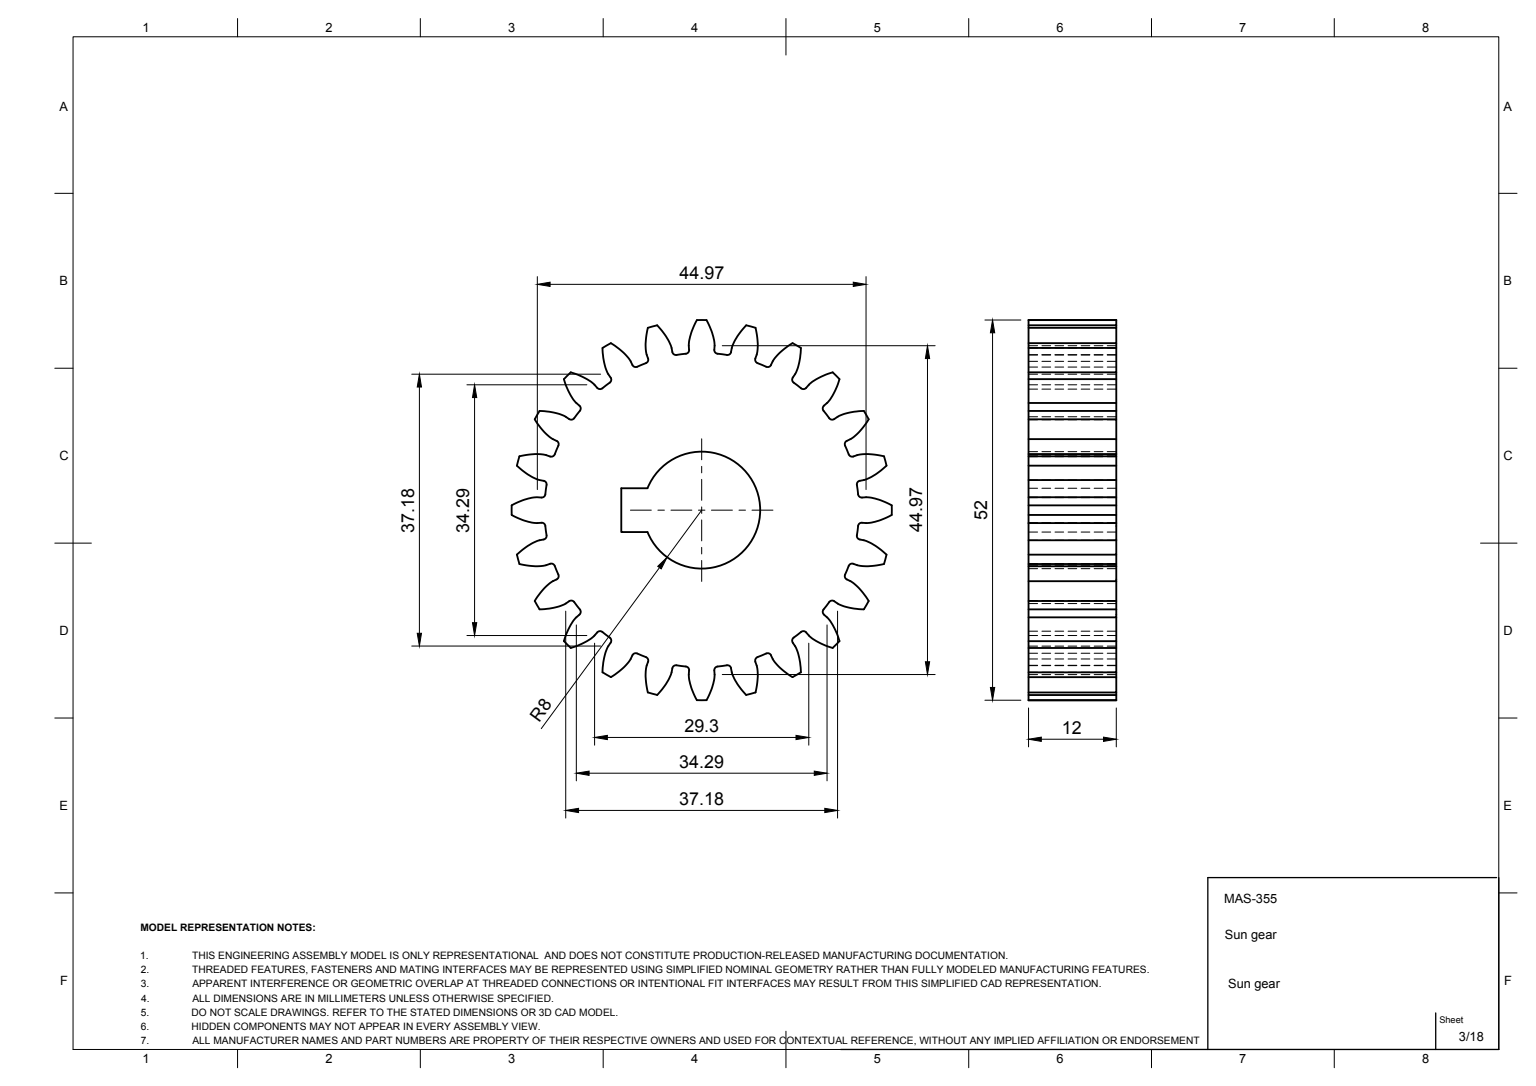
ISO-10303-21;
HEADER;
/* Generated by software containing ST-Developer
 * from STEP Tools, Inc. (www.steptools.com) 
 */

FILE_DESCRIPTION(
/* description */ ('Independent two-stage fixed-ring planetary gearbox,24/24/72 teeth,mod
ule2,20deg involutes,three planets per stage,4:1 x4:1=16:1. Native cut
-space/fillet/pattern tooth profiles derived from reusable gear blanks
; shared sun/planet/ring/carrier parts across both stages. Captured br
onze-journal input/carriers, headed retained planet pins, keyed inters
tage drive and modular keyed output interface. Native ideal gear links
; no torque, precision grade, production backlash/fits, lubrication, s
peed or life rating.'),
/* implementation_level */ '2;1');

FILE_NAME(
/* name */ 'Sun gear.step',
/* time_stamp */ '2026-11-08T19:10:00-08:00',
/* author */ (''),
/* organization */ (''),
/* preprocessor_version */ 'ST-DEVELOPER v20.2',
/* originating_system */ 'Autodesk Translation Framework v15.17.0.0',
/* authorisation */ '');

FILE_SCHEMA (('AUTOMOTIVE_DESIGN { 1 0 10303 214 3 1 1 }'));
ENDSEC;

DATA;
#10=MECHANICAL_DESIGN_GEOMETRIC_PRESENTATION_REPRESENTATION('',(#1168),#259224);
#691=(
BOUNDED_CURVE()
B_SPLINE_CURVE(5,(#175013,#175014,#175015,#175016,#175017,#175018,#175019,
#175020,#175021,#175022,#175023,#175024,#175025,#175026,#175027,#175028,
#175029,#175030,#175031,#175032,#175033,#175034,#175035,#175036,#175037,
#175038,#175039,#175040,#175041,#175042,#175043,#175044,#175045,#175046,
#175047,#175048,#175049,#175050,#175051,#175052,#175053,#175054,#175055,
#175056,#175057,#175058,#175059,#175060,#175061,#175062,#175063,#175064,
#175065,#175066,#175067,#175068,#175069,#175070,#175071,#175072,#175073,
#175074,#175075,#175076,#175077,#175078,#175079,#175080,#175081,#175082,
#175083,#175084,#175085,#175086,#175087,#175088,#175089,#175090,#175091,
#175092,#175093,#175094,#175095,#175096,#175097,#175098,#175099,#175100,
#175101,#175102,#175103,#175104,#175105,#175106,#175107,#175108,#175109,
#175110,#175111,#175112,#175113,#175114,#175115,#175116,#175117,#175118,
#175119,#175120,#175121,#175122,#175123,#175124,#175125,#175126,#175127,
#175128,#175129,#175130,#175131,#175132,#175133,#175134,#175135,#175136,
#175137,#175138,#175139,#175140,#175141,#175142,#175143,#175144,#175145,
#175146,#175147,#175148,#175149,#175150,#175151,#175152,#175153,#175154,
#175155,#175156,#175157,#175158,#175159,#175160,#175161,#175162,#175163,
#175164,#175165,#175166,#175167,#175168,#175169,#175170,#175171,#175172,
#175173,#175174,#175175,#175176,#175177,#175178,#175179,#175180,#175181,
#175182,#175183,#175184,#175185,#175186,#175187,#175188,#175189,#175190,
#175191,#175192,#175193,#175194,#175195,#175196,#175197,#175198,#175199,
#175200,#175201,#175202,#175203,#175204,#175205,#175206,#175207,#175208,
#175209,#175210,#175211,#175212,#175213,#175214,#175215,#175216,#175217),
 .UNSPECIFIED.,.F.,.F.)
B_SPLINE_CURVE_WITH_KNOTS((6,1,1,1,1,1,1,1,1,1,1,1,1,1,1,1,1,1,1,1,1,1,
1,1,1,1,1,1,1,1,1,1,1,1,1,1,1,1,1,1,1,1,1,1,1,1,1,1,1,1,1,1,1,1,1,1,1,1,
1,1,1,1,1,1,1,1,1,1,1,1,1,1,1,1,1,1,1,1,1,1,1,1,1,1,1,1,1,1,1,1,1,1,1,1,
1,1,1,1,1,1,1,1,1,1,1,1,1,1,1,1,1,1,1,1,1,1,1,1,1,1,1,1,1,1,1,1,1,1,1,1,
1,1,1,1,1,1,1,1,1,1,1,1,1,1,1,1,1,1,1,1,1,1,1,1,1,1,1,1,1,1,1,1,1,1,1,1,
1,1,1,1,1,1,1,1,1,1,1,1,1,1,1,1,1,1,1,1,1,1,1,1,1,1,1,1,1,1,1,1,1,1,6),
(0.,0.005,0.01,0.015,0.02,0.025,0.03,0.035,0.04,0.045,0.05,0.055,0.06,0.065,
0.07,0.075,0.08,0.085,0.09,0.095,0.1,0.105,0.11,0.115,0.12,0.125,0.13,0.135,
0.14,0.145,0.15,0.155,0.16,0.165,0.17,0.175,0.18,0.185,0.19,0.195,0.2,0.205,
0.21,0.215,0.22,0.225,0.23,0.235,0.24,0.245,0.25,0.255,0.26,0.265,0.27,
0.275,0.28,0.285,0.29,0.295,0.3,0.305,0.31,0.315,0.32,0.325,0.33,0.335,
0.34,0.345,0.35,0.355,0.36,0.365,0.37,0.375,0.38,0.385,0.39,0.395,0.4,0.405,
0.41,0.415,0.42,0.425,0.43,0.435,0.44,0.445,0.45,0.455,0.46,0.465,0.47,
0.475,0.48,0.485,0.49,0.495,0.5,0.505,0.51,0.515,0.52,0.525,0.53,0.535,
0.54,0.545,0.55,0.555,0.56,0.565,0.57,0.575,0.58,0.585,0.59,0.595,0.6,0.605,
0.61,0.615,0.62,0.625,0.63,0.635,0.64,0.645,0.65,0.655,0.66,0.665,0.67,
0.675,0.68,0.685,0.690000000000001,0.695000000000001,0.700000000000001,
0.705000000000001,0.710000000000001,0.715000000000001,0.720000000000001,
0.725000000000001,0.730000000000001,0.735000000000001,0.740000000000001,
0.745000000000001,0.750000000000001,0.755000000000001,0.760000000000001,
0.765000000000001,0.770000000000001,0.775000000000001,0.780000000000001,
0.785000000000001,0.790000000000001,0.795000000000001,0.800000000000001,
0.805000000000001,0.810000000000001,0.815000000000001,0.820000000000001,
0.825000000000001,0.830000000000001,0.835000000000001,0.840000000000001,
0.845000000000001,0.850000000000001,0.855000000000001,0.860000000000001,
0.865000000000001,0.870000000000001,0.875000000000001,0.880000000000001,
0.885000000000001,0.890000000000001,0.895000000000001,0.900000000000001,
0.905000000000001,0.910000000000001,0.915000000000001,0.920000000000001,
0.925000000000001,0.930000000000001,0.935000000000001,0.940000000000001,
0.945000000000001,0.950000000000001,0.955000000000001,0.960000000000001,
0.965000000000001,0.970000000000001,0.975000000000001,0.980000000000001,
0.985000000000001,0.990000000000001,0.995000000000001,1.),.UNSPECIFIED.)
CURVE()
GEOMETRIC_REPRESENTATION_ITEM()
RATIONAL_B_SPLINE_CURVE((1.,1.,1.,1.,1.,1.,1.,1.,1.,1.,1.,1.,1.,1.,1.,1.,
1.,1.,1.,1.,1.,1.,1.,1.,1.,1.,1.,1.,1.,1.,1.,1.,1.,1.,1.,1.,1.,1.,1.,1.,
1.,1.,1.,1.,1.,1.,1.,1.,1.,1.,1.,1.,1.,1.,1.,1.,1.,1.,1.,1.,1.,1.,1.,1.,
1.,1.,1.,1.,1.,1.,1.,1.,1.,1.,1.,1.,1.,1.,1.,1.,1.,1.,1.,1.,1.,1.,1.,1.,
1.,1.,1.,1.,1.,1.,1.,1.,1.,1.,1.,1.,1.,1.,1.,1.,1.,1.,1.,1.,1.,1.,1.,1.,
1.,1.,1.,1.,1.,1.,1.,1.,1.,1.,1.,1.,1.,1.,1.,1.,1.,1.,1.,1.,1.,1.,1.,1.,
1.,1.,1.,1.,1.,1.,1.,1.,1.,1.,1.,1.,1.,1.,1.,1.,1.,1.,1.,1.,1.,1.,1.,1.,
1.,1.,1.,1.,1.,1.,1.,1.,1.,1.,1.,1.,1.,1.,1.,1.,1.,1.,1.,1.,1.,1.,1.,1.,
1.,1.,1.,1.,1.,1.,1.,1.,1.,1.,1.,1.,1.,1.,1.,1.,1.,1.,1.,1.,1.))
REPRESENTATION_ITEM('')
);
#692=(
BOUNDED_CURVE()
B_SPLINE_CURVE(5,(#175221,#175222,#175223,#175224,#175225,#175226,#175227,
#175228,#175229,#175230,#175231,#175232,#175233,#175234,#175235,#175236,
#175237,#175238,#175239,#175240,#175241,#175242,#175243,#175244,#175245,
#175246,#175247,#175248,#175249,#175250,#175251,#175252,#175253,#175254,
#175255,#175256,#175257,#175258,#175259,#175260,#175261,#175262,#175263,
#175264,#175265,#175266,#175267,#175268,#175269,#175270,#175271,#175272,
#175273,#175274,#175275,#175276,#175277,#175278,#175279,#175280,#175281,
#175282,#175283,#175284,#175285,#175286,#175287,#175288,#175289,#175290,
#175291,#175292,#175293,#175294,#175295,#175296,#175297,#175298,#175299,
#175300,#175301,#175302,#175303,#175304,#175305,#175306,#175307,#175308,
#175309,#175310,#175311,#175312,#175313,#175314,#175315,#175316,#175317,
#175318,#175319,#175320,#175321,#175322,#175323,#175324,#175325,#175326,
#175327,#175328,#175329,#175330,#175331,#175332,#175333,#175334,#175335,
#175336,#175337,#175338,#175339,#175340,#175341,#175342,#175343,#175344,
#175345,#175346,#175347,#175348,#175349,#175350,#175351,#175352,#175353,
#175354,#175355,#175356,#175357,#175358,#175359,#175360,#175361,#175362,
#175363,#175364,#175365,#175366,#175367,#175368,#175369,#175370,#175371,
#175372,#175373,#175374,#175375,#175376,#175377,#175378,#175379,#175380,
#175381,#175382,#175383,#175384,#175385,#175386,#175387,#175388,#175389,
#175390,#175391,#175392,#175393,#175394,#175395,#175396,#175397,#175398,
#175399,#175400,#175401,#175402,#175403,#175404,#175405,#175406,#175407,
#175408,#175409,#175410,#175411,#175412,#175413,#175414,#175415,#175416,
#175417,#175418,#175419,#175420,#175421,#175422,#175423,#175424,#175425),
 .UNSPECIFIED.,.F.,.F.)
B_SPLINE_CURVE_WITH_KNOTS((6,1,1,1,1,1,1,1,1,1,1,1,1,1,1,1,1,1,1,1,1,1,
1,1,1,1,1,1,1,1,1,1,1,1,1,1,1,1,1,1,1,1,1,1,1,1,1,1,1,1,1,1,1,1,1,1,1,1,
1,1,1,1,1,1,1,1,1,1,1,1,1,1,1,1,1,1,1,1,1,1,1,1,1,1,1,1,1,1,1,1,1,1,1,1,
1,1,1,1,1,1,1,1,1,1,1,1,1,1,1,1,1,1,1,1,1,1,1,1,1,1,1,1,1,1,1,1,1,1,1,1,
1,1,1,1,1,1,1,1,1,1,1,1,1,1,1,1,1,1,1,1,1,1,1,1,1,1,1,1,1,1,1,1,1,1,1,1,
1,1,1,1,1,1,1,1,1,1,1,1,1,1,1,1,1,1,1,1,1,1,1,1,1,1,1,1,1,1,1,1,1,1,6),
(-1.,-0.995000000000001,-0.990000000000001,-0.985000000000001,-0.980000000000001,
-0.975000000000001,-0.970000000000001,-0.965000000000001,-0.960000000000001,
-0.955000000000001,-0.950000000000001,-0.945000000000001,-0.940000000000001,
-0.935000000000001,-0.930000000000001,-0.925000000000001,-0.920000000000001,
-0.915000000000001,-0.910000000000001,-0.905000000000001,-0.900000000000001,
-0.895000000000001,-0.890000000000001,-0.885000000000001,-0.880000000000001,
-0.875000000000001,-0.870000000000001,-0.865000000000001,-0.860000000000001,
-0.855000000000001,-0.850000000000001,-0.845000000000001,-0.840000000000001,
-0.835000000000001,-0.830000000000001,-0.825000000000001,-0.820000000000001,
-0.815000000000001,-0.810000000000001,-0.805000000000001,-0.800000000000001,
-0.795000000000001,-0.790000000000001,-0.785000000000001,-0.780000000000001,
-0.775000000000001,-0.770000000000001,-0.765000000000001,-0.760000000000001,
-0.755000000000001,-0.750000000000001,-0.745000000000001,-0.740000000000001,
-0.735000000000001,-0.730000000000001,-0.725000000000001,-0.720000000000001,
-0.715000000000001,-0.710000000000001,-0.705000000000001,-0.700000000000001,
-0.695000000000001,-0.690000000000001,-0.685,-0.68,-0.675,-0.67,-0.665,
-0.66,-0.655,-0.65,-0.645,-0.64,-0.635,-0.63,-0.625,-0.62,-0.615,-0.61,
-0.605,-0.6,-0.595,-0.59,-0.585,-0.58,-0.575,-0.57,-0.565,-0.56,-0.555,
-0.55,-0.545,-0.54,-0.535,-0.53,-0.525,-0.52,-0.515,-0.51,-0.505,-0.5,-0.495,
-0.49,-0.485,-0.48,-0.475,-0.47,-0.465,-0.46,-0.455,-0.45,-0.445,-0.44,
-0.435,-0.43,-0.425,-0.42,-0.415,-0.41,-0.405,-0.4,-0.395,-0.39,-0.385,
-0.38,-0.375,-0.37,-0.365,-0.36,-0.355,-0.35,-0.345,-0.34,-0.335,-0.33,
-0.325,-0.32,-0.315,-0.31,-0.305,-0.3,-0.295,-0.29,-0.285,-0.28,-0.275,
-0.27,-0.265,-0.26,-0.255,-0.25,-0.245,-0.24,-0.235,-0.23,-0.225,-0.22,
-0.215,-0.21,-0.205,-0.2,-0.195,-0.19,-0.185,-0.18,-0.175,-0.17,-0.165,
-0.16,-0.155,-0.15,-0.145,-0.14,-0.135,-0.13,-0.125,-0.12,-0.115,-0.11,
-0.105,-0.1,-0.095,-0.09,-0.085,-0.08,-0.075,-0.07,-0.065,-0.06,-0.055,
-0.05,-0.045,-0.04,-0.035,-0.03,-0.025,-0.02,-0.015,-0.01,-0.005,0.),
 .UNSPECIFIED.)
CURVE()
GEOMETRIC_REPRESENTATION_ITEM()
RATIONAL_B_SPLINE_CURVE((1.,1.,1.,1.,1.,1.,1.,1.,1.,1.,1.,1.,1.,1.,1.,1.,
1.,1.,1.,1.,1.,1.,1.,1.,1.,1.,1.,1.,1.,1.,1.,1.,1.,1.,1.,1.,1.,1.,1.,1.,
1.,1.,1.,1.,1.,1.,1.,1.,1.,1.,1.,1.,1.,1.,1.,1.,1.,1.,1.,1.,1.,1.,1.,1.,
1.,1.,1.,1.,1.,1.,1.,1.,1.,1.,1.,1.,1.,1.,1.,1.,1.,1.,1.,1.,1.,1.,1.,1.,
1.,1.,1.,1.,1.,1.,1.,1.,1.,1.,1.,1.,1.,1.,1.,1.,1.,1.,1.,1.,1.,1.,1.,1.,
1.,1.,1.,1.,1.,1.,1.,1.,1.,1.,1.,1.,1.,1.,1.,1.,1.,1.,1.,1.,1.,1.,1.,1.,
1.,1.,1.,1.,1.,1.,1.,1.,1.,1.,1.,1.,1.,1.,1.,1.,1.,1.,1.,1.,1.,1.,1.,1.,
1.,1.,1.,1.,1.,1.,1.,1.,1.,1.,1.,1.,1.,1.,1.,1.,1.,1.,1.,1.,1.,1.,1.,1.,
1.,1.,1.,1.,1.,1.,1.,1.,1.,1.,1.,1.,1.,1.,1.,1.,1.,1.,1.,1.,1.))
REPRESENTATION_ITEM('')
);
#693=(
BOUNDED_CURVE()
B_SPLINE_CURVE(5,(#175437,#175438,#175439,#175440,#175441,#175442,#175443,
#175444,#175445,#175446,#175447,#175448,#175449,#175450,#175451,#175452,
#175453,#175454,#175455,#175456,#175457,#175458,#175459,#175460,#175461,
#175462,#175463,#175464,#175465,#175466,#175467,#175468,#175469,#175470,
#175471,#175472,#175473,#175474,#175475,#175476,#175477,#175478,#175479,
#175480,#175481,#175482,#175483,#175484,#175485,#175486,#175487,#175488,
#175489,#175490,#175491,#175492,#175493,#175494,#175495,#175496,#175497,
#175498,#175499,#175500,#175501,#175502,#175503,#175504,#175505,#175506,
#175507,#175508,#175509,#175510,#175511,#175512,#175513,#175514,#175515,
#175516,#175517,#175518,#175519,#175520,#175521,#175522,#175523,#175524,
#175525,#175526,#175527,#175528,#175529,#175530,#175531,#175532,#175533,
#175534,#175535,#175536,#175537,#175538,#175539,#175540,#175541,#175542,
#175543,#175544,#175545,#175546,#175547,#175548,#175549,#175550,#175551,
#175552,#175553,#175554,#175555,#175556,#175557,#175558,#175559,#175560,
#175561,#175562,#175563,#175564,#175565,#175566,#175567,#175568,#175569,
#175570,#175571,#175572,#175573,#175574,#175575,#175576,#175577,#175578,
#175579,#175580,#175581,#175582,#175583,#175584,#175585,#175586,#175587,
#175588,#175589,#175590,#175591,#175592,#175593,#175594,#175595,#175596,
#175597,#175598,#175599,#175600,#175601,#175602,#175603,#175604,#175605,
#175606,#175607,#175608,#175609,#175610,#175611,#175612,#175613,#175614,
#175615,#175616,#175617,#175618,#175619,#175620,#175621,#175622,#175623,
#175624,#175625,#175626,#175627,#175628,#175629,#175630,#175631,#175632,
#175633,#175634,#175635,#175636,#175637,#175638,#175639,#175640,#175641),
 .UNSPECIFIED.,.F.,.F.)
B_SPLINE_CURVE_WITH_KNOTS((6,1,1,1,1,1,1,1,1,1,1,1,1,1,1,1,1,1,1,1,1,1,
1,1,1,1,1,1,1,1,1,1,1,1,1,1,1,1,1,1,1,1,1,1,1,1,1,1,1,1,1,1,1,1,1,1,1,1,
1,1,1,1,1,1,1,1,1,1,1,1,1,1,1,1,1,1,1,1,1,1,1,1,1,1,1,1,1,1,1,1,1,1,1,1,
1,1,1,1,1,1,1,1,1,1,1,1,1,1,1,1,1,1,1,1,1,1,1,1,1,1,1,1,1,1,1,1,1,1,1,1,
1,1,1,1,1,1,1,1,1,1,1,1,1,1,1,1,1,1,1,1,1,1,1,1,1,1,1,1,1,1,1,1,1,1,1,1,
1,1,1,1,1,1,1,1,1,1,1,1,1,1,1,1,1,1,1,1,1,1,1,1,1,1,1,1,1,1,1,1,1,1,6),
(0.,0.005,0.01,0.015,0.02,0.025,0.03,0.035,0.04,0.045,0.05,0.055,0.06,0.065,
0.07,0.075,0.08,0.085,0.09,0.095,0.1,0.105,0.11,0.115,0.12,0.125,0.13,0.135,
0.14,0.145,0.15,0.155,0.16,0.165,0.17,0.175,0.18,0.185,0.19,0.195,0.2,0.205,
0.21,0.215,0.22,0.225,0.23,0.235,0.24,0.245,0.25,0.255,0.26,0.265,0.27,
0.275,0.28,0.285,0.29,0.295,0.3,0.305,0.31,0.315,0.32,0.325,0.33,0.335,
0.34,0.345,0.35,0.355,0.36,0.365,0.37,0.375,0.38,0.385,0.39,0.395,0.4,0.405,
0.41,0.415,0.42,0.425,0.43,0.435,0.44,0.445,0.45,0.455,0.46,0.465,0.47,
0.475,0.48,0.485,0.49,0.495,0.5,0.505,0.51,0.515,0.52,0.525,0.53,0.535,
0.54,0.545,0.55,0.555,0.56,0.565,0.57,0.575,0.58,0.585,0.59,0.595,0.6,0.605,
0.61,0.615,0.62,0.625,0.63,0.635,0.64,0.645,0.65,0.655,0.66,0.665,0.67,
0.675,0.68,0.685,0.690000000000001,0.695000000000001,0.700000000000001,
0.705000000000001,0.710000000000001,0.715000000000001,0.720000000000001,
0.725000000000001,0.730000000000001,0.735000000000001,0.740000000000001,
0.745000000000001,0.750000000000001,0.755000000000001,0.760000000000001,
0.765000000000001,0.770000000000001,0.775000000000001,0.780000000000001,
0.785000000000001,0.790000000000001,0.795000000000001,0.800000000000001,
0.805000000000001,0.810000000000001,0.815000000000001,0.820000000000001,
0.825000000000001,0.830000000000001,0.835000000000001,0.840000000000001,
0.845000000000001,0.850000000000001,0.855000000000001,0.860000000000001,
0.865000000000001,0.870000000000001,0.875000000000001,0.880000000000001,
0.885000000000001,0.890000000000001,0.895000000000001,0.900000000000001,
0.905000000000001,0.910000000000001,0.915000000000001,0.920000000000001,
0.925000000000001,0.930000000000001,0.935000000000001,0.940000000000001,
0.945000000000001,0.950000000000001,0.955000000000001,0.960000000000001,
0.965000000000001,0.970000000000001,0.975000000000001,0.980000000000001,
0.985000000000001,0.990000000000001,0.995000000000001,1.),.UNSPECIFIED.)
CURVE()
GEOMETRIC_REPRESENTATION_ITEM()
RATIONAL_B_SPLINE_CURVE((1.,1.,1.,1.,1.,1.,1.,1.,1.,1.,1.,1.,1.,1.,1.,1.,
1.,1.,1.,1.,1.,1.,1.,1.,1.,1.,1.,1.,1.,1.,1.,1.,1.,1.,1.,1.,1.,1.,1.,1.,
1.,1.,1.,1.,1.,1.,1.,1.,1.,1.,1.,1.,1.,1.,1.,1.,1.,1.,1.,1.,1.,1.,1.,1.,
1.,1.,1.,1.,1.,1.,1.,1.,1.,1.,1.,1.,1.,1.,1.,1.,1.,1.,1.,1.,1.,1.,1.,1.,
1.,1.,1.,1.,1.,1.,1.,1.,1.,1.,1.,1.,1.,1.,1.,1.,1.,1.,1.,1.,1.,1.,1.,1.,
1.,1.,1.,1.,1.,1.,1.,1.,1.,1.,1.,1.,1.,1.,1.,1.,1.,1.,1.,1.,1.,1.,1.,1.,
1.,1.,1.,1.,1.,1.,1.,1.,1.,1.,1.,1.,1.,1.,1.,1.,1.,1.,1.,1.,1.,1.,1.,1.,
1.,1.,1.,1.,1.,1.,1.,1.,1.,1.,1.,1.,1.,1.,1.,1.,1.,1.,1.,1.,1.,1.,1.,1.,
1.,1.,1.,1.,1.,1.,1.,1.,1.,1.,1.,1.,1.,1.,1.,1.,1.,1.,1.,1.,1.))
REPRESENTATION_ITEM('')
);
#694=(
BOUNDED_CURVE()
B_SPLINE_CURVE(5,(#175645,#175646,#175647,#175648,#175649,#175650,#175651,
#175652,#175653,#175654,#175655,#175656,#175657,#175658,#175659,#175660,
#175661,#175662,#175663,#175664,#175665,#175666,#175667,#175668,#175669,
#175670,#175671,#175672,#175673,#175674,#175675,#175676,#175677,#175678,
#175679,#175680,#175681,#175682,#175683,#175684,#175685,#175686,#175687,
#175688,#175689,#175690,#175691,#175692,#175693,#175694,#175695,#175696,
#175697,#175698,#175699,#175700,#175701,#175702,#175703,#175704,#175705,
#175706,#175707,#175708,#175709,#175710,#175711,#175712,#175713,#175714,
#175715,#175716,#175717,#175718,#175719,#175720,#175721,#175722,#175723,
#175724,#175725,#175726,#175727,#175728,#175729,#175730,#175731,#175732,
#175733,#175734,#175735,#175736,#175737,#175738,#175739,#175740,#175741,
#175742,#175743,#175744,#175745,#175746,#175747,#175748,#175749,#175750,
#175751,#175752,#175753,#175754,#175755,#175756,#175757,#175758,#175759,
#175760,#175761,#175762,#175763,#175764,#175765,#175766,#175767,#175768,
#175769,#175770,#175771,#175772,#175773,#175774,#175775,#175776,#175777,
#175778,#175779,#175780,#175781,#175782,#175783,#175784,#175785,#175786,
#175787,#175788,#175789,#175790,#175791,#175792,#175793,#175794,#175795,
#175796,#175797,#175798,#175799,#175800,#175801,#175802,#175803,#175804,
#175805,#175806,#175807,#175808,#175809,#175810,#175811,#175812,#175813,
#175814,#175815,#175816,#175817,#175818,#175819,#175820,#175821,#175822,
#175823,#175824,#175825,#175826,#175827,#175828,#175829,#175830,#175831,
#175832,#175833,#175834,#175835,#175836,#175837,#175838,#175839,#175840,
#175841,#175842,#175843,#175844,#175845,#175846,#175847,#175848,#175849),
 .UNSPECIFIED.,.F.,.F.)
B_SPLINE_CURVE_WITH_KNOTS((6,1,1,1,1,1,1,1,1,1,1,1,1,1,1,1,1,1,1,1,1,1,
1,1,1,1,1,1,1,1,1,1,1,1,1,1,1,1,1,1,1,1,1,1,1,1,1,1,1,1,1,1,1,1,1,1,1,1,
1,1,1,1,1,1,1,1,1,1,1,1,1,1,1,1,1,1,1,1,1,1,1,1,1,1,1,1,1,1,1,1,1,1,1,1,
1,1,1,1,1,1,1,1,1,1,1,1,1,1,1,1,1,1,1,1,1,1,1,1,1,1,1,1,1,1,1,1,1,1,1,1,
1,1,1,1,1,1,1,1,1,1,1,1,1,1,1,1,1,1,1,1,1,1,1,1,1,1,1,1,1,1,1,1,1,1,1,1,
1,1,1,1,1,1,1,1,1,1,1,1,1,1,1,1,1,1,1,1,1,1,1,1,1,1,1,1,1,1,1,1,1,1,6),
(-1.,-0.995000000000001,-0.990000000000001,-0.985000000000001,-0.980000000000001,
-0.975000000000001,-0.970000000000001,-0.965000000000001,-0.960000000000001,
-0.955000000000001,-0.950000000000001,-0.945000000000001,-0.940000000000001,
-0.935000000000001,-0.930000000000001,-0.925000000000001,-0.920000000000001,
-0.915000000000001,-0.910000000000001,-0.905000000000001,-0.900000000000001,
-0.895000000000001,-0.890000000000001,-0.885000000000001,-0.880000000000001,
-0.875000000000001,-0.870000000000001,-0.865000000000001,-0.860000000000001,
-0.855000000000001,-0.850000000000001,-0.845000000000001,-0.840000000000001,
-0.835000000000001,-0.830000000000001,-0.825000000000001,-0.820000000000001,
-0.815000000000001,-0.810000000000001,-0.805000000000001,-0.800000000000001,
-0.795000000000001,-0.790000000000001,-0.785000000000001,-0.780000000000001,
-0.775000000000001,-0.770000000000001,-0.765000000000001,-0.760000000000001,
-0.755000000000001,-0.750000000000001,-0.745000000000001,-0.740000000000001,
-0.735000000000001,-0.730000000000001,-0.725000000000001,-0.720000000000001,
-0.715000000000001,-0.710000000000001,-0.705000000000001,-0.700000000000001,
-0.695000000000001,-0.690000000000001,-0.685,-0.68,-0.675,-0.67,-0.665,
-0.66,-0.655,-0.65,-0.645,-0.64,-0.635,-0.63,-0.625,-0.62,-0.615,-0.61,
-0.605,-0.6,-0.595,-0.59,-0.585,-0.58,-0.575,-0.57,-0.565,-0.56,-0.555,
-0.55,-0.545,-0.54,-0.535,-0.53,-0.525,-0.52,-0.515,-0.51,-0.505,-0.5,-0.495,
-0.49,-0.485,-0.48,-0.475,-0.47,-0.465,-0.46,-0.455,-0.45,-0.445,-0.44,
-0.435,-0.43,-0.425,-0.42,-0.415,-0.41,-0.405,-0.4,-0.395,-0.39,-0.385,
-0.38,-0.375,-0.37,-0.365,-0.36,-0.355,-0.35,-0.345,-0.34,-0.335,-0.33,
-0.325,-0.32,-0.315,-0.31,-0.305,-0.3,-0.295,-0.29,-0.285,-0.28,-0.275,
-0.27,-0.265,-0.26,-0.255,-0.25,-0.245,-0.24,-0.235,-0.23,-0.225,-0.22,
-0.215,-0.21,-0.205,-0.2,-0.195,-0.19,-0.185,-0.18,-0.175,-0.17,-0.165,
-0.16,-0.155,-0.15,-0.145,-0.14,-0.135,-0.13,-0.125,-0.12,-0.115,-0.11,
-0.105,-0.1,-0.095,-0.09,-0.085,-0.08,-0.075,-0.07,-0.065,-0.06,-0.055,
-0.05,-0.045,-0.04,-0.035,-0.03,-0.025,-0.02,-0.015,-0.01,-0.005,0.),
 .UNSPECIFIED.)
CURVE()
GEOMETRIC_REPRESENTATION_ITEM()
RATIONAL_B_SPLINE_CURVE((1.,1.,1.,1.,1.,1.,1.,1.,1.,1.,1.,1.,1.,1.,1.,1.,
1.,1.,1.,1.,1.,1.,1.,1.,1.,1.,1.,1.,1.,1.,1.,1.,1.,1.,1.,1.,1.,1.,1.,1.,
1.,1.,1.,1.,1.,1.,1.,1.,1.,1.,1.,1.,1.,1.,1.,1.,1.,1.,1.,1.,1.,1.,1.,1.,
1.,1.,1.,1.,1.,1.,1.,1.,1.,1.,1.,1.,1.,1.,1.,1.,1.,1.,1.,1.,1.,1.,1.,1.,
1.,1.,1.,1.,1.,1.,1.,1.,1.,1.,1.,1.,1.,1.,1.,1.,1.,1.,1.,1.,1.,1.,1.,1.,
1.,1.,1.,1.,1.,1.,1.,1.,1.,1.,1.,1.,1.,1.,1.,1.,1.,1.,1.,1.,1.,1.,1.,1.,
1.,1.,1.,1.,1.,1.,1.,1.,1.,1.,1.,1.,1.,1.,1.,1.,1.,1.,1.,1.,1.,1.,1.,1.,
1.,1.,1.,1.,1.,1.,1.,1.,1.,1.,1.,1.,1.,1.,1.,1.,1.,1.,1.,1.,1.,1.,1.,1.,
1.,1.,1.,1.,1.,1.,1.,1.,1.,1.,1.,1.,1.,1.,1.,1.,1.,1.,1.,1.,1.))
REPRESENTATION_ITEM('')
);
#695=(
BOUNDED_CURVE()
B_SPLINE_CURVE(5,(#175861,#175862,#175863,#175864,#175865,#175866,#175867,
#175868,#175869,#175870,#175871,#175872,#175873,#175874,#175875,#175876,
#175877,#175878,#175879,#175880,#175881,#175882,#175883,#175884,#175885,
#175886,#175887,#175888,#175889,#175890,#175891,#175892,#175893,#175894,
#175895,#175896,#175897,#175898,#175899,#175900,#175901,#175902,#175903,
#175904,#175905,#175906,#175907,#175908,#175909,#175910,#175911,#175912,
#175913,#175914,#175915,#175916,#175917,#175918,#175919,#175920,#175921,
#175922,#175923,#175924,#175925,#175926,#175927,#175928,#175929,#175930,
#175931,#175932,#175933,#175934,#175935,#175936,#175937,#175938,#175939,
#175940,#175941,#175942,#175943,#175944,#175945,#175946,#175947,#175948,
#175949,#175950,#175951,#175952,#175953,#175954,#175955,#175956,#175957,
#175958,#175959,#175960,#175961,#175962,#175963,#175964,#175965,#175966,
#175967,#175968,#175969,#175970,#175971,#175972,#175973,#175974,#175975,
#175976,#175977,#175978,#175979,#175980,#175981,#175982,#175983,#175984,
#175985,#175986,#175987,#175988,#175989,#175990,#175991,#175992,#175993,
#175994,#175995,#175996,#175997,#175998,#175999,#176000,#176001,#176002,
#176003,#176004,#176005,#176006,#176007,#176008,#176009,#176010,#176011,
#176012,#176013,#176014,#176015,#176016,#176017,#176018,#176019,#176020,
#176021,#176022,#176023,#176024,#176025,#176026,#176027,#176028,#176029,
#176030,#176031,#176032,#176033,#176034,#176035,#176036,#176037,#176038,
#176039,#176040,#176041,#176042,#176043,#176044,#176045,#176046,#176047,
#176048,#176049,#176050,#176051,#176052,#176053,#176054,#176055,#176056,
#176057,#176058,#176059,#176060,#176061,#176062,#176063,#176064,#176065),
 .UNSPECIFIED.,.F.,.F.)
B_SPLINE_CURVE_WITH_KNOTS((6,1,1,1,1,1,1,1,1,1,1,1,1,1,1,1,1,1,1,1,1,1,
1,1,1,1,1,1,1,1,1,1,1,1,1,1,1,1,1,1,1,1,1,1,1,1,1,1,1,1,1,1,1,1,1,1,1,1,
1,1,1,1,1,1,1,1,1,1,1,1,1,1,1,1,1,1,1,1,1,1,1,1,1,1,1,1,1,1,1,1,1,1,1,1,
1,1,1,1,1,1,1,1,1,1,1,1,1,1,1,1,1,1,1,1,1,1,1,1,1,1,1,1,1,1,1,1,1,1,1,1,
1,1,1,1,1,1,1,1,1,1,1,1,1,1,1,1,1,1,1,1,1,1,1,1,1,1,1,1,1,1,1,1,1,1,1,1,
1,1,1,1,1,1,1,1,1,1,1,1,1,1,1,1,1,1,1,1,1,1,1,1,1,1,1,1,1,1,1,1,1,1,6),
(0.,0.005,0.01,0.015,0.02,0.025,0.03,0.035,0.04,0.045,0.05,0.055,0.06,0.065,
0.07,0.075,0.08,0.085,0.09,0.095,0.1,0.105,0.11,0.115,0.12,0.125,0.13,0.135,
0.14,0.145,0.15,0.155,0.16,0.165,0.17,0.175,0.18,0.185,0.19,0.195,0.2,0.205,
0.21,0.215,0.22,0.225,0.23,0.235,0.24,0.245,0.25,0.255,0.26,0.265,0.27,
0.275,0.28,0.285,0.29,0.295,0.3,0.305,0.31,0.315,0.32,0.325,0.33,0.335,
0.34,0.345,0.35,0.355,0.36,0.365,0.37,0.375,0.38,0.385,0.39,0.395,0.4,0.405,
0.41,0.415,0.42,0.425,0.43,0.435,0.44,0.445,0.45,0.455,0.46,0.465,0.47,
0.475,0.48,0.485,0.49,0.495,0.5,0.505,0.51,0.515,0.52,0.525,0.53,0.535,
0.54,0.545,0.55,0.555,0.56,0.565,0.57,0.575,0.58,0.585,0.59,0.595,0.6,0.605,
0.61,0.615,0.62,0.625,0.63,0.635,0.64,0.645,0.65,0.655,0.66,0.665,0.67,
0.675,0.68,0.685,0.690000000000001,0.695000000000001,0.700000000000001,
0.705000000000001,0.710000000000001,0.715000000000001,0.720000000000001,
0.725000000000001,0.730000000000001,0.735000000000001,0.740000000000001,
0.745000000000001,0.750000000000001,0.755000000000001,0.760000000000001,
0.765000000000001,0.770000000000001,0.775000000000001,0.780000000000001,
0.785000000000001,0.790000000000001,0.795000000000001,0.800000000000001,
0.805000000000001,0.810000000000001,0.815000000000001,0.820000000000001,
0.825000000000001,0.830000000000001,0.835000000000001,0.840000000000001,
0.845000000000001,0.850000000000001,0.855000000000001,0.860000000000001,
0.865000000000001,0.870000000000001,0.875000000000001,0.880000000000001,
0.885000000000001,0.890000000000001,0.895000000000001,0.900000000000001,
0.905000000000001,0.910000000000001,0.915000000000001,0.920000000000001,
0.925000000000001,0.930000000000001,0.935000000000001,0.940000000000001,
0.945000000000001,0.950000000000001,0.955000000000001,0.960000000000001,
0.965000000000001,0.970000000000001,0.975000000000001,0.980000000000001,
0.985000000000001,0.990000000000001,0.995000000000001,1.),.UNSPECIFIED.)
CURVE()
GEOMETRIC_REPRESENTATION_ITEM()
RATIONAL_B_SPLINE_CURVE((1.,1.,1.,1.,1.,1.,1.,1.,1.,1.,1.,1.,1.,1.,1.,1.,
1.,1.,1.,1.,1.,1.,1.,1.,1.,1.,1.,1.,1.,1.,1.,1.,1.,1.,1.,1.,1.,1.,1.,1.,
1.,1.,1.,1.,1.,1.,1.,1.,1.,1.,1.,1.,1.,1.,1.,1.,1.,1.,1.,1.,1.,1.,1.,1.,
1.,1.,1.,1.,1.,1.,1.,1.,1.,1.,1.,1.,1.,1.,1.,1.,1.,1.,1.,1.,1.,1.,1.,1.,
1.,1.,1.,1.,1.,1.,1.,1.,1.,1.,1.,1.,1.,1.,1.,1.,1.,1.,1.,1.,1.,1.,1.,1.,
1.,1.,1.,1.,1.,1.,1.,1.,1.,1.,1.,1.,1.,1.,1.,1.,1.,1.,1.,1.,1.,1.,1.,1.,
1.,1.,1.,1.,1.,1.,1.,1.,1.,1.,1.,1.,1.,1.,1.,1.,1.,1.,1.,1.,1.,1.,1.,1.,
1.,1.,1.,1.,1.,1.,1.,1.,1.,1.,1.,1.,1.,1.,1.,1.,1.,1.,1.,1.,1.,1.,1.,1.,
1.,1.,1.,1.,1.,1.,1.,1.,1.,1.,1.,1.,1.,1.,1.,1.,1.,1.,1.,1.,1.))
REPRESENTATION_ITEM('')
);
#696=(
BOUNDED_CURVE()
B_SPLINE_CURVE(5,(#176069,#176070,#176071,#176072,#176073,#176074,#176075,
#176076,#176077,#176078,#176079,#176080,#176081,#176082,#176083,#176084,
#176085,#176086,#176087,#176088,#176089,#176090,#176091,#176092,#176093,
#176094,#176095,#176096,#176097,#176098,#176099,#176100,#176101,#176102,
#176103,#176104,#176105,#176106,#176107,#176108,#176109,#176110,#176111,
#176112,#176113,#176114,#176115,#176116,#176117,#176118,#176119,#176120,
#176121,#176122,#176123,#176124,#176125,#176126,#176127,#176128,#176129,
#176130,#176131,#176132,#176133,#176134,#176135,#176136,#176137,#176138,
#176139,#176140,#176141,#176142,#176143,#176144,#176145,#176146,#176147,
#176148,#176149,#176150,#176151,#176152,#176153,#176154,#176155,#176156,
#176157,#176158,#176159,#176160,#176161,#176162,#176163,#176164,#176165,
#176166,#176167,#176168,#176169,#176170,#176171,#176172,#176173,#176174,
#176175,#176176,#176177,#176178,#176179,#176180,#176181,#176182,#176183,
#176184,#176185,#176186,#176187,#176188,#176189,#176190,#176191,#176192,
#176193,#176194,#176195,#176196,#176197,#176198,#176199,#176200,#176201,
#176202,#176203,#176204,#176205,#176206,#176207,#176208,#176209,#176210,
#176211,#176212,#176213,#176214,#176215,#176216,#176217,#176218,#176219,
#176220,#176221,#176222,#176223,#176224,#176225,#176226,#176227,#176228,
#176229,#176230,#176231,#176232,#176233,#176234,#176235,#176236,#176237,
#176238,#176239,#176240,#176241,#176242,#176243,#176244,#176245,#176246,
#176247,#176248,#176249,#176250,#176251,#176252,#176253,#176254,#176255,
#176256,#176257,#176258,#176259,#176260,#176261,#176262,#176263,#176264,
#176265,#176266,#176267,#176268,#176269,#176270,#176271,#176272,#176273),
 .UNSPECIFIED.,.F.,.F.)
B_SPLINE_CURVE_WITH_KNOTS((6,1,1,1,1,1,1,1,1,1,1,1,1,1,1,1,1,1,1,1,1,1,
1,1,1,1,1,1,1,1,1,1,1,1,1,1,1,1,1,1,1,1,1,1,1,1,1,1,1,1,1,1,1,1,1,1,1,1,
1,1,1,1,1,1,1,1,1,1,1,1,1,1,1,1,1,1,1,1,1,1,1,1,1,1,1,1,1,1,1,1,1,1,1,1,
1,1,1,1,1,1,1,1,1,1,1,1,1,1,1,1,1,1,1,1,1,1,1,1,1,1,1,1,1,1,1,1,1,1,1,1,
1,1,1,1,1,1,1,1,1,1,1,1,1,1,1,1,1,1,1,1,1,1,1,1,1,1,1,1,1,1,1,1,1,1,1,1,
1,1,1,1,1,1,1,1,1,1,1,1,1,1,1,1,1,1,1,1,1,1,1,1,1,1,1,1,1,1,1,1,1,1,6),
(-1.,-0.995000000000001,-0.990000000000001,-0.985000000000001,-0.980000000000001,
-0.975000000000001,-0.970000000000001,-0.965000000000001,-0.960000000000001,
-0.955000000000001,-0.950000000000001,-0.945000000000001,-0.940000000000001,
-0.935000000000001,-0.930000000000001,-0.925000000000001,-0.920000000000001,
-0.915000000000001,-0.910000000000001,-0.905000000000001,-0.900000000000001,
-0.895000000000001,-0.890000000000001,-0.885000000000001,-0.880000000000001,
-0.875000000000001,-0.870000000000001,-0.865000000000001,-0.860000000000001,
-0.855000000000001,-0.850000000000001,-0.845000000000001,-0.840000000000001,
-0.835000000000001,-0.830000000000001,-0.825000000000001,-0.820000000000001,
-0.815000000000001,-0.810000000000001,-0.805000000000001,-0.800000000000001,
-0.795000000000001,-0.790000000000001,-0.785000000000001,-0.780000000000001,
-0.775000000000001,-0.770000000000001,-0.765000000000001,-0.760000000000001,
-0.755000000000001,-0.750000000000001,-0.745000000000001,-0.740000000000001,
-0.735000000000001,-0.730000000000001,-0.725000000000001,-0.720000000000001,
-0.715000000000001,-0.710000000000001,-0.705000000000001,-0.700000000000001,
-0.695000000000001,-0.690000000000001,-0.685,-0.68,-0.675,-0.67,-0.665,
-0.66,-0.655,-0.65,-0.645,-0.64,-0.635,-0.63,-0.625,-0.62,-0.615,-0.61,
-0.605,-0.6,-0.595,-0.59,-0.585,-0.58,-0.575,-0.57,-0.565,-0.56,-0.555,
-0.55,-0.545,-0.54,-0.535,-0.53,-0.525,-0.52,-0.515,-0.51,-0.505,-0.5,-0.495,
-0.49,-0.485,-0.48,-0.475,-0.47,-0.465,-0.46,-0.455,-0.45,-0.445,-0.44,
-0.435,-0.43,-0.425,-0.42,-0.415,-0.41,-0.405,-0.4,-0.395,-0.39,-0.385,
-0.38,-0.375,-0.37,-0.365,-0.36,-0.355,-0.35,-0.345,-0.34,-0.335,-0.33,
-0.325,-0.32,-0.315,-0.31,-0.305,-0.3,-0.295,-0.29,-0.285,-0.28,-0.275,
-0.27,-0.265,-0.26,-0.255,-0.25,-0.245,-0.24,-0.235,-0.23,-0.225,-0.22,
-0.215,-0.21,-0.205,-0.2,-0.195,-0.19,-0.185,-0.18,-0.175,-0.17,-0.165,
-0.16,-0.155,-0.15,-0.145,-0.14,-0.135,-0.13,-0.125,-0.12,-0.115,-0.11,
-0.105,-0.1,-0.095,-0.09,-0.085,-0.08,-0.075,-0.07,-0.065,-0.06,-0.055,
-0.05,-0.045,-0.04,-0.035,-0.03,-0.025,-0.02,-0.015,-0.01,-0.005,0.),
 .UNSPECIFIED.)
CURVE()
GEOMETRIC_REPRESENTATION_ITEM()
RATIONAL_B_SPLINE_CURVE((1.,1.,1.,1.,1.,1.,1.,1.,1.,1.,1.,1.,1.,1.,1.,1.,
1.,1.,1.,1.,1.,1.,1.,1.,1.,1.,1.,1.,1.,1.,1.,1.,1.,1.,1.,1.,1.,1.,1.,1.,
1.,1.,1.,1.,1.,1.,1.,1.,1.,1.,1.,1.,1.,1.,1.,1.,1.,1.,1.,1.,1.,1.,1.,1.,
1.,1.,1.,1.,1.,1.,1.,1.,1.,1.,1.,1.,1.,1.,1.,1.,1.,1.,1.,1.,1.,1.,1.,1.,
1.,1.,1.,1.,1.,1.,1.,1.,1.,1.,1.,1.,1.,1.,1.,1.,1.,1.,1.,1.,1.,1.,1.,1.,
1.,1.,1.,1.,1.,1.,1.,1.,1.,1.,1.,1.,1.,1.,1.,1.,1.,1.,1.,1.,1.,1.,1.,1.,
1.,1.,1.,1.,1.,1.,1.,1.,1.,1.,1.,1.,1.,1.,1.,1.,1.,1.,1.,1.,1.,1.,1.,1.,
1.,1.,1.,1.,1.,1.,1.,1.,1.,1.,1.,1.,1.,1.,1.,1.,1.,1.,1.,1.,1.,1.,1.,1.,
1.,1.,1.,1.,1.,1.,1.,1.,1.,1.,1.,1.,1.,1.,1.,1.,1.,1.,1.,1.,1.))
REPRESENTATION_ITEM('')
);
#697=(
BOUNDED_CURVE()
B_SPLINE_CURVE(5,(#176285,#176286,#176287,#176288,#176289,#176290,#176291,
#176292,#176293,#176294,#176295,#176296,#176297,#176298,#176299,#176300,
#176301,#176302,#176303,#176304,#176305,#176306,#176307,#176308,#176309,
#176310,#176311,#176312,#176313,#176314,#176315,#176316,#176317,#176318,
#176319,#176320,#176321,#176322,#176323,#176324,#176325,#176326,#176327,
#176328,#176329,#176330,#176331,#176332,#176333,#176334,#176335,#176336,
#176337,#176338,#176339,#176340,#176341,#176342,#176343,#176344,#176345,
#176346,#176347,#176348,#176349,#176350,#176351,#176352,#176353,#176354,
#176355,#176356,#176357,#176358,#176359,#176360,#176361,#176362,#176363,
#176364,#176365,#176366,#176367,#176368,#176369,#176370,#176371,#176372,
#176373,#176374,#176375,#176376,#176377,#176378,#176379,#176380,#176381,
#176382,#176383,#176384,#176385,#176386,#176387,#176388,#176389,#176390,
#176391,#176392,#176393,#176394,#176395,#176396,#176397,#176398,#176399,
#176400,#176401,#176402,#176403,#176404,#176405,#176406,#176407,#176408,
#176409,#176410,#176411,#176412,#176413,#176414,#176415,#176416,#176417,
#176418,#176419,#176420,#176421,#176422,#176423,#176424,#176425,#176426,
#176427,#176428,#176429,#176430,#176431,#176432,#176433,#176434,#176435,
#176436,#176437,#176438,#176439,#176440,#176441,#176442,#176443,#176444,
#176445,#176446,#176447,#176448,#176449,#176450,#176451,#176452,#176453,
#176454,#176455,#176456,#176457,#176458,#176459,#176460,#176461,#176462,
#176463,#176464,#176465,#176466,#176467,#176468,#176469,#176470,#176471,
#176472,#176473,#176474,#176475,#176476,#176477,#176478,#176479,#176480,
#176481,#176482,#176483,#176484,#176485,#176486,#176487,#176488,#176489),
 .UNSPECIFIED.,.F.,.F.)
B_SPLINE_CURVE_WITH_KNOTS((6,1,1,1,1,1,1,1,1,1,1,1,1,1,1,1,1,1,1,1,1,1,
1,1,1,1,1,1,1,1,1,1,1,1,1,1,1,1,1,1,1,1,1,1,1,1,1,1,1,1,1,1,1,1,1,1,1,1,
1,1,1,1,1,1,1,1,1,1,1,1,1,1,1,1,1,1,1,1,1,1,1,1,1,1,1,1,1,1,1,1,1,1,1,1,
1,1,1,1,1,1,1,1,1,1,1,1,1,1,1,1,1,1,1,1,1,1,1,1,1,1,1,1,1,1,1,1,1,1,1,1,
1,1,1,1,1,1,1,1,1,1,1,1,1,1,1,1,1,1,1,1,1,1,1,1,1,1,1,1,1,1,1,1,1,1,1,1,
1,1,1,1,1,1,1,1,1,1,1,1,1,1,1,1,1,1,1,1,1,1,1,1,1,1,1,1,1,1,1,1,1,1,6),
(0.,0.005,0.01,0.015,0.02,0.025,0.03,0.035,0.04,0.045,0.05,0.055,0.06,0.065,
0.07,0.075,0.08,0.085,0.09,0.095,0.1,0.105,0.11,0.115,0.12,0.125,0.13,0.135,
0.14,0.145,0.15,0.155,0.16,0.165,0.17,0.175,0.18,0.185,0.19,0.195,0.2,0.205,
0.21,0.215,0.22,0.225,0.23,0.235,0.24,0.245,0.25,0.255,0.26,0.265,0.27,
0.275,0.28,0.285,0.29,0.295,0.3,0.305,0.31,0.315,0.32,0.325,0.33,0.335,
0.34,0.345,0.35,0.355,0.36,0.365,0.37,0.375,0.38,0.385,0.39,0.395,0.4,0.405,
0.41,0.415,0.42,0.425,0.43,0.435,0.44,0.445,0.45,0.455,0.46,0.465,0.47,
0.475,0.48,0.485,0.49,0.495,0.5,0.505,0.51,0.515,0.52,0.525,0.53,0.535,
0.54,0.545,0.55,0.555,0.56,0.565,0.57,0.575,0.58,0.585,0.59,0.595,0.6,0.605,
0.61,0.615,0.62,0.625,0.63,0.635,0.64,0.645,0.65,0.655,0.66,0.665,0.67,
0.675,0.68,0.685,0.690000000000001,0.695000000000001,0.700000000000001,
0.705000000000001,0.710000000000001,0.715000000000001,0.720000000000001,
0.725000000000001,0.730000000000001,0.735000000000001,0.740000000000001,
0.745000000000001,0.750000000000001,0.755000000000001,0.760000000000001,
0.765000000000001,0.770000000000001,0.775000000000001,0.780000000000001,
0.785000000000001,0.790000000000001,0.795000000000001,0.800000000000001,
0.805000000000001,0.810000000000001,0.815000000000001,0.820000000000001,
0.825000000000001,0.830000000000001,0.835000000000001,0.840000000000001,
0.845000000000001,0.850000000000001,0.855000000000001,0.860000000000001,
0.865000000000001,0.870000000000001,0.875000000000001,0.880000000000001,
0.885000000000001,0.890000000000001,0.895000000000001,0.900000000000001,
0.905000000000001,0.910000000000001,0.915000000000001,0.920000000000001,
0.925000000000001,0.930000000000001,0.935000000000001,0.940000000000001,
0.945000000000001,0.950000000000001,0.955000000000001,0.960000000000001,
0.965000000000001,0.970000000000001,0.975000000000001,0.980000000000001,
0.985000000000001,0.990000000000001,0.995000000000001,1.),.UNSPECIFIED.)
CURVE()
GEOMETRIC_REPRESENTATION_ITEM()
RATIONAL_B_SPLINE_CURVE((1.,1.,1.,1.,1.,1.,1.,1.,1.,1.,1.,1.,1.,1.,1.,1.,
1.,1.,1.,1.,1.,1.,1.,1.,1.,1.,1.,1.,1.,1.,1.,1.,1.,1.,1.,1.,1.,1.,1.,1.,
1.,1.,1.,1.,1.,1.,1.,1.,1.,1.,1.,1.,1.,1.,1.,1.,1.,1.,1.,1.,1.,1.,1.,1.,
1.,1.,1.,1.,1.,1.,1.,1.,1.,1.,1.,1.,1.,1.,1.,1.,1.,1.,1.,1.,1.,1.,1.,1.,
1.,1.,1.,1.,1.,1.,1.,1.,1.,1.,1.,1.,1.,1.,1.,1.,1.,1.,1.,1.,1.,1.,1.,1.,
1.,1.,1.,1.,1.,1.,1.,1.,1.,1.,1.,1.,1.,1.,1.,1.,1.,1.,1.,1.,1.,1.,1.,1.,
1.,1.,1.,1.,1.,1.,1.,1.,1.,1.,1.,1.,1.,1.,1.,1.,1.,1.,1.,1.,1.,1.,1.,1.,
1.,1.,1.,1.,1.,1.,1.,1.,1.,1.,1.,1.,1.,1.,1.,1.,1.,1.,1.,1.,1.,1.,1.,1.,
1.,1.,1.,1.,1.,1.,1.,1.,1.,1.,1.,1.,1.,1.,1.,1.,1.,1.,1.,1.,1.))
REPRESENTATION_ITEM('')
);
#698=(
BOUNDED_CURVE()
B_SPLINE_CURVE(5,(#176493,#176494,#176495,#176496,#176497,#176498,#176499,
#176500,#176501,#176502,#176503,#176504,#176505,#176506,#176507,#176508,
#176509,#176510,#176511,#176512,#176513,#176514,#176515,#176516,#176517,
#176518,#176519,#176520,#176521,#176522,#176523,#176524,#176525,#176526,
#176527,#176528,#176529,#176530,#176531,#176532,#176533,#176534,#176535,
#176536,#176537,#176538,#176539,#176540,#176541,#176542,#176543,#176544,
#176545,#176546,#176547,#176548,#176549,#176550,#176551,#176552,#176553,
#176554,#176555,#176556,#176557,#176558,#176559,#176560,#176561,#176562,
#176563,#176564,#176565,#176566,#176567,#176568,#176569,#176570,#176571,
#176572,#176573,#176574,#176575,#176576,#176577,#176578,#176579,#176580,
#176581,#176582,#176583,#176584,#176585,#176586,#176587,#176588,#176589,
#176590,#176591,#176592,#176593,#176594,#176595,#176596,#176597,#176598,
#176599,#176600,#176601,#176602,#176603,#176604,#176605,#176606,#176607,
#176608,#176609,#176610,#176611,#176612,#176613,#176614,#176615,#176616,
#176617,#176618,#176619,#176620,#176621,#176622,#176623,#176624,#176625,
#176626,#176627,#176628,#176629,#176630,#176631,#176632,#176633,#176634,
#176635,#176636,#176637,#176638,#176639,#176640,#176641,#176642,#176643,
#176644,#176645,#176646,#176647,#176648,#176649,#176650,#176651,#176652,
#176653,#176654,#176655,#176656,#176657,#176658,#176659,#176660,#176661,
#176662,#176663,#176664,#176665,#176666,#176667,#176668,#176669,#176670,
#176671,#176672,#176673,#176674,#176675,#176676,#176677,#176678,#176679,
#176680,#176681,#176682,#176683,#176684,#176685,#176686,#176687,#176688,
#176689,#176690,#176691,#176692,#176693,#176694,#176695,#176696,#176697),
 .UNSPECIFIED.,.F.,.F.)
B_SPLINE_CURVE_WITH_KNOTS((6,1,1,1,1,1,1,1,1,1,1,1,1,1,1,1,1,1,1,1,1,1,
1,1,1,1,1,1,1,1,1,1,1,1,1,1,1,1,1,1,1,1,1,1,1,1,1,1,1,1,1,1,1,1,1,1,1,1,
1,1,1,1,1,1,1,1,1,1,1,1,1,1,1,1,1,1,1,1,1,1,1,1,1,1,1,1,1,1,1,1,1,1,1,1,
1,1,1,1,1,1,1,1,1,1,1,1,1,1,1,1,1,1,1,1,1,1,1,1,1,1,1,1,1,1,1,1,1,1,1,1,
1,1,1,1,1,1,1,1,1,1,1,1,1,1,1,1,1,1,1,1,1,1,1,1,1,1,1,1,1,1,1,1,1,1,1,1,
1,1,1,1,1,1,1,1,1,1,1,1,1,1,1,1,1,1,1,1,1,1,1,1,1,1,1,1,1,1,1,1,1,1,6),
(-1.,-0.995000000000001,-0.990000000000001,-0.985000000000001,-0.980000000000001,
-0.975000000000001,-0.970000000000001,-0.965000000000001,-0.960000000000001,
-0.955000000000001,-0.950000000000001,-0.945000000000001,-0.940000000000001,
-0.935000000000001,-0.930000000000001,-0.925000000000001,-0.920000000000001,
-0.915000000000001,-0.910000000000001,-0.905000000000001,-0.900000000000001,
-0.895000000000001,-0.890000000000001,-0.885000000000001,-0.880000000000001,
-0.875000000000001,-0.870000000000001,-0.865000000000001,-0.860000000000001,
-0.855000000000001,-0.850000000000001,-0.845000000000001,-0.840000000000001,
-0.835000000000001,-0.830000000000001,-0.825000000000001,-0.820000000000001,
-0.815000000000001,-0.810000000000001,-0.805000000000001,-0.800000000000001,
-0.795000000000001,-0.790000000000001,-0.785000000000001,-0.780000000000001,
-0.775000000000001,-0.770000000000001,-0.765000000000001,-0.760000000000001,
-0.755000000000001,-0.750000000000001,-0.745000000000001,-0.740000000000001,
-0.735000000000001,-0.730000000000001,-0.725000000000001,-0.720000000000001,
-0.715000000000001,-0.710000000000001,-0.705000000000001,-0.700000000000001,
-0.695000000000001,-0.690000000000001,-0.685,-0.68,-0.675,-0.67,-0.665,
-0.66,-0.655,-0.65,-0.645,-0.64,-0.635,-0.63,-0.625,-0.62,-0.615,-0.61,
-0.605,-0.6,-0.595,-0.59,-0.585,-0.58,-0.575,-0.57,-0.565,-0.56,-0.555,
-0.55,-0.545,-0.54,-0.535,-0.53,-0.525,-0.52,-0.515,-0.51,-0.505,-0.5,-0.495,
-0.49,-0.485,-0.48,-0.475,-0.47,-0.465,-0.46,-0.455,-0.45,-0.445,-0.44,
-0.435,-0.43,-0.425,-0.42,-0.415,-0.41,-0.405,-0.4,-0.395,-0.39,-0.385,
-0.38,-0.375,-0.37,-0.365,-0.36,-0.355,-0.35,-0.345,-0.34,-0.335,-0.33,
-0.325,-0.32,-0.315,-0.31,-0.305,-0.3,-0.295,-0.29,-0.285,-0.28,-0.275,
-0.27,-0.265,-0.26,-0.255,-0.25,-0.245,-0.24,-0.235,-0.23,-0.225,-0.22,
-0.215,-0.21,-0.205,-0.2,-0.195,-0.19,-0.185,-0.18,-0.175,-0.17,-0.165,
-0.16,-0.155,-0.15,-0.145,-0.14,-0.135,-0.13,-0.125,-0.12,-0.115,-0.11,
-0.105,-0.1,-0.095,-0.09,-0.085,-0.08,-0.075,-0.07,-0.065,-0.06,-0.055,
-0.05,-0.045,-0.04,-0.035,-0.03,-0.025,-0.02,-0.015,-0.01,-0.005,0.),
 .UNSPECIFIED.)
CURVE()
GEOMETRIC_REPRESENTATION_ITEM()
RATIONAL_B_SPLINE_CURVE((1.,1.,1.,1.,1.,1.,1.,1.,1.,1.,1.,1.,1.,1.,1.,1.,
1.,1.,1.,1.,1.,1.,1.,1.,1.,1.,1.,1.,1.,1.,1.,1.,1.,1.,1.,1.,1.,1.,1.,1.,
1.,1.,1.,1.,1.,1.,1.,1.,1.,1.,1.,1.,1.,1.,1.,1.,1.,1.,1.,1.,1.,1.,1.,1.,
1.,1.,1.,1.,1.,1.,1.,1.,1.,1.,1.,1.,1.,1.,1.,1.,1.,1.,1.,1.,1.,1.,1.,1.,
1.,1.,1.,1.,1.,1.,1.,1.,1.,1.,1.,1.,1.,1.,1.,1.,1.,1.,1.,1.,1.,1.,1.,1.,
1.,1.,1.,1.,1.,1.,1.,1.,1.,1.,1.,1.,1.,1.,1.,1.,1.,1.,1.,1.,1.,1.,1.,1.,
1.,1.,1.,1.,1.,1.,1.,1.,1.,1.,1.,1.,1.,1.,1.,1.,1.,1.,1.,1.,1.,1.,1.,1.,
1.,1.,1.,1.,1.,1.,1.,1.,1.,1.,1.,1.,1.,1.,1.,1.,1.,1.,1.,1.,1.,1.,1.,1.,
1.,1.,1.,1.,1.,1.,1.,1.,1.,1.,1.,1.,1.,1.,1.,1.,1.,1.,1.,1.,1.))
REPRESENTATION_ITEM('')
);
#699=(
BOUNDED_CURVE()
B_SPLINE_CURVE(5,(#176709,#176710,#176711,#176712,#176713,#176714,#176715,
#176716,#176717,#176718,#176719,#176720,#176721,#176722,#176723,#176724,
#176725,#176726,#176727,#176728,#176729,#176730,#176731,#176732,#176733,
#176734,#176735,#176736,#176737,#176738,#176739,#176740,#176741,#176742,
#176743,#176744,#176745,#176746,#176747,#176748,#176749,#176750,#176751,
#176752,#176753,#176754,#176755,#176756,#176757,#176758,#176759,#176760,
#176761,#176762,#176763,#176764,#176765,#176766,#176767,#176768,#176769,
#176770,#176771,#176772,#176773,#176774,#176775,#176776,#176777,#176778,
#176779,#176780,#176781,#176782,#176783,#176784,#176785,#176786,#176787,
#176788,#176789,#176790,#176791,#176792,#176793,#176794,#176795,#176796,
#176797,#176798,#176799,#176800,#176801,#176802,#176803,#176804,#176805,
#176806,#176807,#176808,#176809,#176810,#176811,#176812,#176813,#176814,
#176815,#176816,#176817,#176818,#176819,#176820,#176821,#176822,#176823,
#176824,#176825,#176826,#176827,#176828,#176829,#176830,#176831,#176832,
#176833,#176834,#176835,#176836,#176837,#176838,#176839,#176840,#176841,
#176842,#176843,#176844,#176845,#176846,#176847,#176848,#176849,#176850,
#176851,#176852,#176853,#176854,#176855,#176856,#176857,#176858,#176859,
#176860,#176861,#176862,#176863,#176864,#176865,#176866,#176867,#176868,
#176869,#176870,#176871,#176872,#176873,#176874,#176875,#176876,#176877,
#176878,#176879,#176880,#176881,#176882,#176883,#176884,#176885,#176886,
#176887,#176888,#176889,#176890,#176891,#176892,#176893,#176894,#176895,
#176896,#176897,#176898,#176899,#176900,#176901,#176902,#176903,#176904,
#176905,#176906,#176907,#176908,#176909,#176910,#176911,#176912,#176913),
 .UNSPECIFIED.,.F.,.F.)
B_SPLINE_CURVE_WITH_KNOTS((6,1,1,1,1,1,1,1,1,1,1,1,1,1,1,1,1,1,1,1,1,1,
1,1,1,1,1,1,1,1,1,1,1,1,1,1,1,1,1,1,1,1,1,1,1,1,1,1,1,1,1,1,1,1,1,1,1,1,
1,1,1,1,1,1,1,1,1,1,1,1,1,1,1,1,1,1,1,1,1,1,1,1,1,1,1,1,1,1,1,1,1,1,1,1,
1,1,1,1,1,1,1,1,1,1,1,1,1,1,1,1,1,1,1,1,1,1,1,1,1,1,1,1,1,1,1,1,1,1,1,1,
1,1,1,1,1,1,1,1,1,1,1,1,1,1,1,1,1,1,1,1,1,1,1,1,1,1,1,1,1,1,1,1,1,1,1,1,
1,1,1,1,1,1,1,1,1,1,1,1,1,1,1,1,1,1,1,1,1,1,1,1,1,1,1,1,1,1,1,1,1,1,6),
(0.,0.005,0.01,0.015,0.02,0.025,0.03,0.035,0.04,0.045,0.05,0.055,0.06,0.065,
0.07,0.075,0.08,0.085,0.09,0.095,0.1,0.105,0.11,0.115,0.12,0.125,0.13,0.135,
0.14,0.145,0.15,0.155,0.16,0.165,0.17,0.175,0.18,0.185,0.19,0.195,0.2,0.205,
0.21,0.215,0.22,0.225,0.23,0.235,0.24,0.245,0.25,0.255,0.26,0.265,0.27,
0.275,0.28,0.285,0.29,0.295,0.3,0.305,0.31,0.315,0.32,0.325,0.33,0.335,
0.34,0.345,0.35,0.355,0.36,0.365,0.37,0.375,0.38,0.385,0.39,0.395,0.4,0.405,
0.41,0.415,0.42,0.425,0.43,0.435,0.44,0.445,0.45,0.455,0.46,0.465,0.47,
0.475,0.48,0.485,0.49,0.495,0.5,0.505,0.51,0.515,0.52,0.525,0.53,0.535,
0.54,0.545,0.55,0.555,0.56,0.565,0.57,0.575,0.58,0.585,0.59,0.595,0.6,0.605,
0.61,0.615,0.62,0.625,0.63,0.635,0.64,0.645,0.65,0.655,0.66,0.665,0.67,
0.675,0.68,0.685,0.690000000000001,0.695000000000001,0.700000000000001,
0.705000000000001,0.710000000000001,0.715000000000001,0.720000000000001,
0.725000000000001,0.730000000000001,0.735000000000001,0.740000000000001,
0.745000000000001,0.750000000000001,0.755000000000001,0.760000000000001,
0.765000000000001,0.770000000000001,0.775000000000001,0.780000000000001,
0.785000000000001,0.790000000000001,0.795000000000001,0.800000000000001,
0.805000000000001,0.810000000000001,0.815000000000001,0.820000000000001,
0.825000000000001,0.830000000000001,0.835000000000001,0.840000000000001,
0.845000000000001,0.850000000000001,0.855000000000001,0.860000000000001,
0.865000000000001,0.870000000000001,0.875000000000001,0.880000000000001,
0.885000000000001,0.890000000000001,0.895000000000001,0.900000000000001,
0.905000000000001,0.910000000000001,0.915000000000001,0.920000000000001,
0.925000000000001,0.930000000000001,0.935000000000001,0.940000000000001,
0.945000000000001,0.950000000000001,0.955000000000001,0.960000000000001,
0.965000000000001,0.970000000000001,0.975000000000001,0.980000000000001,
0.985000000000001,0.990000000000001,0.995000000000001,1.),.UNSPECIFIED.)
CURVE()
GEOMETRIC_REPRESENTATION_ITEM()
RATIONAL_B_SPLINE_CURVE((1.,1.,1.,1.,1.,1.,1.,1.,1.,1.,1.,1.,1.,1.,1.,1.,
1.,1.,1.,1.,1.,1.,1.,1.,1.,1.,1.,1.,1.,1.,1.,1.,1.,1.,1.,1.,1.,1.,1.,1.,
1.,1.,1.,1.,1.,1.,1.,1.,1.,1.,1.,1.,1.,1.,1.,1.,1.,1.,1.,1.,1.,1.,1.,1.,
1.,1.,1.,1.,1.,1.,1.,1.,1.,1.,1.,1.,1.,1.,1.,1.,1.,1.,1.,1.,1.,1.,1.,1.,
1.,1.,1.,1.,1.,1.,1.,1.,1.,1.,1.,1.,1.,1.,1.,1.,1.,1.,1.,1.,1.,1.,1.,1.,
1.,1.,1.,1.,1.,1.,1.,1.,1.,1.,1.,1.,1.,1.,1.,1.,1.,1.,1.,1.,1.,1.,1.,1.,
1.,1.,1.,1.,1.,1.,1.,1.,1.,1.,1.,1.,1.,1.,1.,1.,1.,1.,1.,1.,1.,1.,1.,1.,
1.,1.,1.,1.,1.,1.,1.,1.,1.,1.,1.,1.,1.,1.,1.,1.,1.,1.,1.,1.,1.,1.,1.,1.,
1.,1.,1.,1.,1.,1.,1.,1.,1.,1.,1.,1.,1.,1.,1.,1.,1.,1.,1.,1.,1.))
REPRESENTATION_ITEM('')
);
#700=(
BOUNDED_CURVE()
B_SPLINE_CURVE(5,(#176917,#176918,#176919,#176920,#176921,#176922,#176923,
#176924,#176925,#176926,#176927,#176928,#176929,#176930,#176931,#176932,
#176933,#176934,#176935,#176936,#176937,#176938,#176939,#176940,#176941,
#176942,#176943,#176944,#176945,#176946,#176947,#176948,#176949,#176950,
#176951,#176952,#176953,#176954,#176955,#176956,#176957,#176958,#176959,
#176960,#176961,#176962,#176963,#176964,#176965,#176966,#176967,#176968,
#176969,#176970,#176971,#176972,#176973,#176974,#176975,#176976,#176977,
#176978,#176979,#176980,#176981,#176982,#176983,#176984,#176985,#176986,
#176987,#176988,#176989,#176990,#176991,#176992,#176993,#176994,#176995,
#176996,#176997,#176998,#176999,#177000,#177001,#177002,#177003,#177004,
#177005,#177006,#177007,#177008,#177009,#177010,#177011,#177012,#177013,
#177014,#177015,#177016,#177017,#177018,#177019,#177020,#177021,#177022,
#177023,#177024,#177025,#177026,#177027,#177028,#177029,#177030,#177031,
#177032,#177033,#177034,#177035,#177036,#177037,#177038,#177039,#177040,
#177041,#177042,#177043,#177044,#177045,#177046,#177047,#177048,#177049,
#177050,#177051,#177052,#177053,#177054,#177055,#177056,#177057,#177058,
#177059,#177060,#177061,#177062,#177063,#177064,#177065,#177066,#177067,
#177068,#177069,#177070,#177071,#177072,#177073,#177074,#177075,#177076,
#177077,#177078,#177079,#177080,#177081,#177082,#177083,#177084,#177085,
#177086,#177087,#177088,#177089,#177090,#177091,#177092,#177093,#177094,
#177095,#177096,#177097,#177098,#177099,#177100,#177101,#177102,#177103,
#177104,#177105,#177106,#177107,#177108,#177109,#177110,#177111,#177112,
#177113,#177114,#177115,#177116,#177117,#177118,#177119,#177120,#177121),
 .UNSPECIFIED.,.F.,.F.)
B_SPLINE_CURVE_WITH_KNOTS((6,1,1,1,1,1,1,1,1,1,1,1,1,1,1,1,1,1,1,1,1,1,
1,1,1,1,1,1,1,1,1,1,1,1,1,1,1,1,1,1,1,1,1,1,1,1,1,1,1,1,1,1,1,1,1,1,1,1,
1,1,1,1,1,1,1,1,1,1,1,1,1,1,1,1,1,1,1,1,1,1,1,1,1,1,1,1,1,1,1,1,1,1,1,1,
1,1,1,1,1,1,1,1,1,1,1,1,1,1,1,1,1,1,1,1,1,1,1,1,1,1,1,1,1,1,1,1,1,1,1,1,
1,1,1,1,1,1,1,1,1,1,1,1,1,1,1,1,1,1,1,1,1,1,1,1,1,1,1,1,1,1,1,1,1,1,1,1,
1,1,1,1,1,1,1,1,1,1,1,1,1,1,1,1,1,1,1,1,1,1,1,1,1,1,1,1,1,1,1,1,1,1,6),
(-1.,-0.995000000000001,-0.990000000000001,-0.985000000000001,-0.980000000000001,
-0.975000000000001,-0.970000000000001,-0.965000000000001,-0.960000000000001,
-0.955000000000001,-0.950000000000001,-0.945000000000001,-0.940000000000001,
-0.935000000000001,-0.930000000000001,-0.925000000000001,-0.920000000000001,
-0.915000000000001,-0.910000000000001,-0.905000000000001,-0.900000000000001,
-0.895000000000001,-0.890000000000001,-0.885000000000001,-0.880000000000001,
-0.875000000000001,-0.870000000000001,-0.865000000000001,-0.860000000000001,
-0.855000000000001,-0.850000000000001,-0.845000000000001,-0.840000000000001,
-0.835000000000001,-0.830000000000001,-0.825000000000001,-0.820000000000001,
-0.815000000000001,-0.810000000000001,-0.805000000000001,-0.800000000000001,
-0.795000000000001,-0.790000000000001,-0.785000000000001,-0.780000000000001,
-0.775000000000001,-0.770000000000001,-0.765000000000001,-0.760000000000001,
-0.755000000000001,-0.750000000000001,-0.745000000000001,-0.740000000000001,
-0.735000000000001,-0.730000000000001,-0.725000000000001,-0.720000000000001,
-0.715000000000001,-0.710000000000001,-0.705000000000001,-0.700000000000001,
-0.695000000000001,-0.690000000000001,-0.685,-0.68,-0.675,-0.67,-0.665,
-0.66,-0.655,-0.65,-0.645,-0.64,-0.635,-0.63,-0.625,-0.62,-0.615,-0.61,
-0.605,-0.6,-0.595,-0.59,-0.585,-0.58,-0.575,-0.57,-0.565,-0.56,-0.555,
-0.55,-0.545,-0.54,-0.535,-0.53,-0.525,-0.52,-0.515,-0.51,-0.505,-0.5,-0.495,
-0.49,-0.485,-0.48,-0.475,-0.47,-0.465,-0.46,-0.455,-0.45,-0.445,-0.44,
-0.435,-0.43,-0.425,-0.42,-0.415,-0.41,-0.405,-0.4,-0.395,-0.39,-0.385,
-0.38,-0.375,-0.37,-0.365,-0.36,-0.355,-0.35,-0.345,-0.34,-0.335,-0.33,
-0.325,-0.32,-0.315,-0.31,-0.305,-0.3,-0.295,-0.29,-0.285,-0.28,-0.275,
-0.27,-0.265,-0.26,-0.255,-0.25,-0.245,-0.24,-0.235,-0.23,-0.225,-0.22,
-0.215,-0.21,-0.205,-0.2,-0.195,-0.19,-0.185,-0.18,-0.175,-0.17,-0.165,
-0.16,-0.155,-0.15,-0.145,-0.14,-0.135,-0.13,-0.125,-0.12,-0.115,-0.11,
-0.105,-0.1,-0.095,-0.09,-0.085,-0.08,-0.075,-0.07,-0.065,-0.06,-0.055,
-0.05,-0.045,-0.04,-0.035,-0.03,-0.025,-0.02,-0.015,-0.01,-0.005,0.),
 .UNSPECIFIED.)
CURVE()
GEOMETRIC_REPRESENTATION_ITEM()
RATIONAL_B_SPLINE_CURVE((1.,1.,1.,1.,1.,1.,1.,1.,1.,1.,1.,1.,1.,1.,1.,1.,
1.,1.,1.,1.,1.,1.,1.,1.,1.,1.,1.,1.,1.,1.,1.,1.,1.,1.,1.,1.,1.,1.,1.,1.,
1.,1.,1.,1.,1.,1.,1.,1.,1.,1.,1.,1.,1.,1.,1.,1.,1.,1.,1.,1.,1.,1.,1.,1.,
1.,1.,1.,1.,1.,1.,1.,1.,1.,1.,1.,1.,1.,1.,1.,1.,1.,1.,1.,1.,1.,1.,1.,1.,
1.,1.,1.,1.,1.,1.,1.,1.,1.,1.,1.,1.,1.,1.,1.,1.,1.,1.,1.,1.,1.,1.,1.,1.,
1.,1.,1.,1.,1.,1.,1.,1.,1.,1.,1.,1.,1.,1.,1.,1.,1.,1.,1.,1.,1.,1.,1.,1.,
1.,1.,1.,1.,1.,1.,1.,1.,1.,1.,1.,1.,1.,1.,1.,1.,1.,1.,1.,1.,1.,1.,1.,1.,
1.,1.,1.,1.,1.,1.,1.,1.,1.,1.,1.,1.,1.,1.,1.,1.,1.,1.,1.,1.,1.,1.,1.,1.,
1.,1.,1.,1.,1.,1.,1.,1.,1.,1.,1.,1.,1.,1.,1.,1.,1.,1.,1.,1.,1.))
REPRESENTATION_ITEM('')
);
#701=(
BOUNDED_CURVE()
B_SPLINE_CURVE(5,(#177133,#177134,#177135,#177136,#177137,#177138,#177139,
#177140,#177141,#177142,#177143,#177144,#177145,#177146,#177147,#177148,
#177149,#177150,#177151,#177152,#177153,#177154,#177155,#177156,#177157,
#177158,#177159,#177160,#177161,#177162,#177163,#177164,#177165,#177166,
#177167,#177168,#177169,#177170,#177171,#177172,#177173,#177174,#177175,
#177176,#177177,#177178,#177179,#177180,#177181,#177182,#177183,#177184,
#177185,#177186,#177187,#177188,#177189,#177190,#177191,#177192,#177193,
#177194,#177195,#177196,#177197,#177198,#177199,#177200,#177201,#177202,
#177203,#177204,#177205,#177206,#177207,#177208,#177209,#177210,#177211,
#177212,#177213,#177214,#177215,#177216,#177217,#177218,#177219,#177220,
#177221,#177222,#177223,#177224,#177225,#177226,#177227,#177228,#177229,
#177230,#177231,#177232,#177233,#177234,#177235,#177236,#177237,#177238,
#177239,#177240,#177241,#177242,#177243,#177244,#177245,#177246,#177247,
#177248,#177249,#177250,#177251,#177252,#177253,#177254,#177255,#177256,
#177257,#177258,#177259,#177260,#177261,#177262,#177263,#177264,#177265,
#177266,#177267,#177268,#177269,#177270,#177271,#177272,#177273,#177274,
#177275,#177276,#177277,#177278,#177279,#177280,#177281,#177282,#177283,
#177284,#177285,#177286,#177287,#177288,#177289,#177290,#177291,#177292,
#177293,#177294,#177295,#177296,#177297,#177298,#177299,#177300,#177301,
#177302,#177303,#177304,#177305,#177306,#177307,#177308,#177309,#177310,
#177311,#177312,#177313,#177314,#177315,#177316,#177317,#177318,#177319,
#177320,#177321,#177322,#177323,#177324,#177325,#177326,#177327,#177328,
#177329,#177330,#177331,#177332,#177333,#177334,#177335,#177336,#177337),
 .UNSPECIFIED.,.F.,.F.)
B_SPLINE_CURVE_WITH_KNOTS((6,1,1,1,1,1,1,1,1,1,1,1,1,1,1,1,1,1,1,1,1,1,
1,1,1,1,1,1,1,1,1,1,1,1,1,1,1,1,1,1,1,1,1,1,1,1,1,1,1,1,1,1,1,1,1,1,1,1,
1,1,1,1,1,1,1,1,1,1,1,1,1,1,1,1,1,1,1,1,1,1,1,1,1,1,1,1,1,1,1,1,1,1,1,1,
1,1,1,1,1,1,1,1,1,1,1,1,1,1,1,1,1,1,1,1,1,1,1,1,1,1,1,1,1,1,1,1,1,1,1,1,
1,1,1,1,1,1,1,1,1,1,1,1,1,1,1,1,1,1,1,1,1,1,1,1,1,1,1,1,1,1,1,1,1,1,1,1,
1,1,1,1,1,1,1,1,1,1,1,1,1,1,1,1,1,1,1,1,1,1,1,1,1,1,1,1,1,1,1,1,1,1,6),
(0.,0.005,0.01,0.015,0.02,0.025,0.03,0.035,0.04,0.045,0.05,0.055,0.06,0.065,
0.07,0.075,0.08,0.085,0.09,0.095,0.1,0.105,0.11,0.115,0.12,0.125,0.13,0.135,
0.14,0.145,0.15,0.155,0.16,0.165,0.17,0.175,0.18,0.185,0.19,0.195,0.2,0.205,
0.21,0.215,0.22,0.225,0.23,0.235,0.24,0.245,0.25,0.255,0.26,0.265,0.27,
0.275,0.28,0.285,0.29,0.295,0.3,0.305,0.31,0.315,0.32,0.325,0.33,0.335,
0.34,0.345,0.35,0.355,0.36,0.365,0.37,0.375,0.38,0.385,0.39,0.395,0.4,0.405,
0.41,0.415,0.42,0.425,0.43,0.435,0.44,0.445,0.45,0.455,0.46,0.465,0.47,
0.475,0.48,0.485,0.49,0.495,0.5,0.505,0.51,0.515,0.52,0.525,0.53,0.535,
0.54,0.545,0.55,0.555,0.56,0.565,0.57,0.575,0.58,0.585,0.59,0.595,0.6,0.605,
0.61,0.615,0.62,0.625,0.63,0.635,0.64,0.645,0.65,0.655,0.66,0.665,0.67,
0.675,0.68,0.685,0.690000000000001,0.695000000000001,0.700000000000001,
0.705000000000001,0.710000000000001,0.715000000000001,0.720000000000001,
0.725000000000001,0.730000000000001,0.735000000000001,0.740000000000001,
0.745000000000001,0.750000000000001,0.755000000000001,0.760000000000001,
0.765000000000001,0.770000000000001,0.775000000000001,0.780000000000001,
0.785000000000001,0.790000000000001,0.795000000000001,0.800000000000001,
0.805000000000001,0.810000000000001,0.815000000000001,0.820000000000001,
0.825000000000001,0.830000000000001,0.835000000000001,0.840000000000001,
0.845000000000001,0.850000000000001,0.855000000000001,0.860000000000001,
0.865000000000001,0.870000000000001,0.875000000000001,0.880000000000001,
0.885000000000001,0.890000000000001,0.895000000000001,0.900000000000001,
0.905000000000001,0.910000000000001,0.915000000000001,0.920000000000001,
0.925000000000001,0.930000000000001,0.935000000000001,0.940000000000001,
0.945000000000001,0.950000000000001,0.955000000000001,0.960000000000001,
0.965000000000001,0.970000000000001,0.975000000000001,0.980000000000001,
0.985000000000001,0.990000000000001,0.995000000000001,1.),.UNSPECIFIED.)
CURVE()
GEOMETRIC_REPRESENTATION_ITEM()
RATIONAL_B_SPLINE_CURVE((1.,1.,1.,1.,1.,1.,1.,1.,1.,1.,1.,1.,1.,1.,1.,1.,
1.,1.,1.,1.,1.,1.,1.,1.,1.,1.,1.,1.,1.,1.,1.,1.,1.,1.,1.,1.,1.,1.,1.,1.,
1.,1.,1.,1.,1.,1.,1.,1.,1.,1.,1.,1.,1.,1.,1.,1.,1.,1.,1.,1.,1.,1.,1.,1.,
1.,1.,1.,1.,1.,1.,1.,1.,1.,1.,1.,1.,1.,1.,1.,1.,1.,1.,1.,1.,1.,1.,1.,1.,
1.,1.,1.,1.,1.,1.,1.,1.,1.,1.,1.,1.,1.,1.,1.,1.,1.,1.,1.,1.,1.,1.,1.,1.,
1.,1.,1.,1.,1.,1.,1.,1.,1.,1.,1.,1.,1.,1.,1.,1.,1.,1.,1.,1.,1.,1.,1.,1.,
1.,1.,1.,1.,1.,1.,1.,1.,1.,1.,1.,1.,1.,1.,1.,1.,1.,1.,1.,1.,1.,1.,1.,1.,
1.,1.,1.,1.,1.,1.,1.,1.,1.,1.,1.,1.,1.,1.,1.,1.,1.,1.,1.,1.,1.,1.,1.,1.,
1.,1.,1.,1.,1.,1.,1.,1.,1.,1.,1.,1.,1.,1.,1.,1.,1.,1.,1.,1.,1.))
REPRESENTATION_ITEM('')
);
#702=(
BOUNDED_CURVE()
B_SPLINE_CURVE(5,(#177341,#177342,#177343,#177344,#177345,#177346,#177347,
#177348,#177349,#177350,#177351,#177352,#177353,#177354,#177355,#177356,
#177357,#177358,#177359,#177360,#177361,#177362,#177363,#177364,#177365,
#177366,#177367,#177368,#177369,#177370,#177371,#177372,#177373,#177374,
#177375,#177376,#177377,#177378,#177379,#177380,#177381,#177382,#177383,
#177384,#177385,#177386,#177387,#177388,#177389,#177390,#177391,#177392,
#177393,#177394,#177395,#177396,#177397,#177398,#177399,#177400,#177401,
#177402,#177403,#177404,#177405,#177406,#177407,#177408,#177409,#177410,
#177411,#177412,#177413,#177414,#177415,#177416,#177417,#177418,#177419,
#177420,#177421,#177422,#177423,#177424,#177425,#177426,#177427,#177428,
#177429,#177430,#177431,#177432,#177433,#177434,#177435,#177436,#177437,
#177438,#177439,#177440,#177441,#177442,#177443,#177444,#177445,#177446,
#177447,#177448,#177449,#177450,#177451,#177452,#177453,#177454,#177455,
#177456,#177457,#177458,#177459,#177460,#177461,#177462,#177463,#177464,
#177465,#177466,#177467,#177468,#177469,#177470,#177471,#177472,#177473,
#177474,#177475,#177476,#177477,#177478,#177479,#177480,#177481,#177482,
#177483,#177484,#177485,#177486,#177487,#177488,#177489,#177490,#177491,
#177492,#177493,#177494,#177495,#177496,#177497,#177498,#177499,#177500,
#177501,#177502,#177503,#177504,#177505,#177506,#177507,#177508,#177509,
#177510,#177511,#177512,#177513,#177514,#177515,#177516,#177517,#177518,
#177519,#177520,#177521,#177522,#177523,#177524,#177525,#177526,#177527,
#177528,#177529,#177530,#177531,#177532,#177533,#177534,#177535,#177536,
#177537,#177538,#177539,#177540,#177541,#177542,#177543,#177544,#177545),
 .UNSPECIFIED.,.F.,.F.)
B_SPLINE_CURVE_WITH_KNOTS((6,1,1,1,1,1,1,1,1,1,1,1,1,1,1,1,1,1,1,1,1,1,
1,1,1,1,1,1,1,1,1,1,1,1,1,1,1,1,1,1,1,1,1,1,1,1,1,1,1,1,1,1,1,1,1,1,1,1,
1,1,1,1,1,1,1,1,1,1,1,1,1,1,1,1,1,1,1,1,1,1,1,1,1,1,1,1,1,1,1,1,1,1,1,1,
1,1,1,1,1,1,1,1,1,1,1,1,1,1,1,1,1,1,1,1,1,1,1,1,1,1,1,1,1,1,1,1,1,1,1,1,
1,1,1,1,1,1,1,1,1,1,1,1,1,1,1,1,1,1,1,1,1,1,1,1,1,1,1,1,1,1,1,1,1,1,1,1,
1,1,1,1,1,1,1,1,1,1,1,1,1,1,1,1,1,1,1,1,1,1,1,1,1,1,1,1,1,1,1,1,1,1,6),
(-1.,-0.995000000000001,-0.990000000000001,-0.985000000000001,-0.980000000000001,
-0.975000000000001,-0.970000000000001,-0.965000000000001,-0.960000000000001,
-0.955000000000001,-0.950000000000001,-0.945000000000001,-0.940000000000001,
-0.935000000000001,-0.930000000000001,-0.925000000000001,-0.920000000000001,
-0.915000000000001,-0.910000000000001,-0.905000000000001,-0.900000000000001,
-0.895000000000001,-0.890000000000001,-0.885000000000001,-0.880000000000001,
-0.875000000000001,-0.870000000000001,-0.865000000000001,-0.860000000000001,
-0.855000000000001,-0.850000000000001,-0.845000000000001,-0.840000000000001,
-0.835000000000001,-0.830000000000001,-0.825000000000001,-0.820000000000001,
-0.815000000000001,-0.810000000000001,-0.805000000000001,-0.800000000000001,
-0.795000000000001,-0.790000000000001,-0.785000000000001,-0.780000000000001,
-0.775000000000001,-0.770000000000001,-0.765000000000001,-0.760000000000001,
-0.755000000000001,-0.750000000000001,-0.745000000000001,-0.740000000000001,
-0.735000000000001,-0.730000000000001,-0.725000000000001,-0.720000000000001,
-0.715000000000001,-0.710000000000001,-0.705000000000001,-0.700000000000001,
-0.695000000000001,-0.690000000000001,-0.685,-0.68,-0.675,-0.67,-0.665,
-0.66,-0.655,-0.65,-0.645,-0.64,-0.635,-0.63,-0.625,-0.62,-0.615,-0.61,
-0.605,-0.6,-0.595,-0.59,-0.585,-0.58,-0.575,-0.57,-0.565,-0.56,-0.555,
-0.55,-0.545,-0.54,-0.535,-0.53,-0.525,-0.52,-0.515,-0.51,-0.505,-0.5,-0.495,
-0.49,-0.485,-0.48,-0.475,-0.47,-0.465,-0.46,-0.455,-0.45,-0.445,-0.44,
-0.435,-0.43,-0.425,-0.42,-0.415,-0.41,-0.405,-0.4,-0.395,-0.39,-0.385,
-0.38,-0.375,-0.37,-0.365,-0.36,-0.355,-0.35,-0.345,-0.34,-0.335,-0.33,
-0.325,-0.32,-0.315,-0.31,-0.305,-0.3,-0.295,-0.29,-0.285,-0.28,-0.275,
-0.27,-0.265,-0.26,-0.255,-0.25,-0.245,-0.24,-0.235,-0.23,-0.225,-0.22,
-0.215,-0.21,-0.205,-0.2,-0.195,-0.19,-0.185,-0.18,-0.175,-0.17,-0.165,
-0.16,-0.155,-0.15,-0.145,-0.14,-0.135,-0.13,-0.125,-0.12,-0.115,-0.11,
-0.105,-0.1,-0.095,-0.09,-0.085,-0.08,-0.075,-0.07,-0.065,-0.06,-0.055,
-0.05,-0.045,-0.04,-0.035,-0.03,-0.025,-0.02,-0.015,-0.01,-0.005,0.),
 .UNSPECIFIED.)
CURVE()
GEOMETRIC_REPRESENTATION_ITEM()
RATIONAL_B_SPLINE_CURVE((1.,1.,1.,1.,1.,1.,1.,1.,1.,1.,1.,1.,1.,1.,1.,1.,
1.,1.,1.,1.,1.,1.,1.,1.,1.,1.,1.,1.,1.,1.,1.,1.,1.,1.,1.,1.,1.,1.,1.,1.,
1.,1.,1.,1.,1.,1.,1.,1.,1.,1.,1.,1.,1.,1.,1.,1.,1.,1.,1.,1.,1.,1.,1.,1.,
1.,1.,1.,1.,1.,1.,1.,1.,1.,1.,1.,1.,1.,1.,1.,1.,1.,1.,1.,1.,1.,1.,1.,1.,
1.,1.,1.,1.,1.,1.,1.,1.,1.,1.,1.,1.,1.,1.,1.,1.,1.,1.,1.,1.,1.,1.,1.,1.,
1.,1.,1.,1.,1.,1.,1.,1.,1.,1.,1.,1.,1.,1.,1.,1.,1.,1.,1.,1.,1.,1.,1.,1.,
1.,1.,1.,1.,1.,1.,1.,1.,1.,1.,1.,1.,1.,1.,1.,1.,1.,1.,1.,1.,1.,1.,1.,1.,
1.,1.,1.,1.,1.,1.,1.,1.,1.,1.,1.,1.,1.,1.,1.,1.,1.,1.,1.,1.,1.,1.,1.,1.,
1.,1.,1.,1.,1.,1.,1.,1.,1.,1.,1.,1.,1.,1.,1.,1.,1.,1.,1.,1.,1.))
REPRESENTATION_ITEM('')
);
#703=(
BOUNDED_CURVE()
B_SPLINE_CURVE(5,(#177557,#177558,#177559,#177560,#177561,#177562,#177563,
#177564,#177565,#177566,#177567,#177568,#177569,#177570,#177571,#177572,
#177573,#177574,#177575,#177576,#177577,#177578,#177579,#177580,#177581,
#177582,#177583,#177584,#177585,#177586,#177587,#177588,#177589,#177590,
#177591,#177592,#177593,#177594,#177595,#177596,#177597,#177598,#177599,
#177600,#177601,#177602,#177603,#177604,#177605,#177606,#177607,#177608,
#177609,#177610,#177611,#177612,#177613,#177614,#177615,#177616,#177617,
#177618,#177619,#177620,#177621,#177622,#177623,#177624,#177625,#177626,
#177627,#177628,#177629,#177630,#177631,#177632,#177633,#177634,#177635,
#177636,#177637,#177638,#177639,#177640,#177641,#177642,#177643,#177644,
#177645,#177646,#177647,#177648,#177649,#177650,#177651,#177652,#177653,
#177654,#177655,#177656,#177657,#177658,#177659,#177660,#177661,#177662,
#177663,#177664,#177665,#177666,#177667,#177668,#177669,#177670,#177671,
#177672,#177673,#177674,#177675,#177676,#177677,#177678,#177679,#177680,
#177681,#177682,#177683,#177684,#177685,#177686,#177687,#177688,#177689,
#177690,#177691,#177692,#177693,#177694,#177695,#177696,#177697,#177698,
#177699,#177700,#177701,#177702,#177703,#177704,#177705,#177706,#177707,
#177708,#177709,#177710,#177711,#177712,#177713,#177714,#177715,#177716,
#177717,#177718,#177719,#177720,#177721,#177722,#177723,#177724,#177725,
#177726,#177727,#177728,#177729,#177730,#177731,#177732,#177733,#177734,
#177735,#177736,#177737,#177738,#177739,#177740,#177741,#177742,#177743,
#177744,#177745,#177746,#177747,#177748,#177749,#177750,#177751,#177752,
#177753,#177754,#177755,#177756,#177757,#177758,#177759,#177760,#177761),
 .UNSPECIFIED.,.F.,.F.)
B_SPLINE_CURVE_WITH_KNOTS((6,1,1,1,1,1,1,1,1,1,1,1,1,1,1,1,1,1,1,1,1,1,
1,1,1,1,1,1,1,1,1,1,1,1,1,1,1,1,1,1,1,1,1,1,1,1,1,1,1,1,1,1,1,1,1,1,1,1,
1,1,1,1,1,1,1,1,1,1,1,1,1,1,1,1,1,1,1,1,1,1,1,1,1,1,1,1,1,1,1,1,1,1,1,1,
1,1,1,1,1,1,1,1,1,1,1,1,1,1,1,1,1,1,1,1,1,1,1,1,1,1,1,1,1,1,1,1,1,1,1,1,
1,1,1,1,1,1,1,1,1,1,1,1,1,1,1,1,1,1,1,1,1,1,1,1,1,1,1,1,1,1,1,1,1,1,1,1,
1,1,1,1,1,1,1,1,1,1,1,1,1,1,1,1,1,1,1,1,1,1,1,1,1,1,1,1,1,1,1,1,1,1,6),
(0.,0.005,0.01,0.015,0.02,0.025,0.03,0.035,0.04,0.045,0.05,0.055,0.06,0.065,
0.07,0.075,0.08,0.085,0.09,0.095,0.1,0.105,0.11,0.115,0.12,0.125,0.13,0.135,
0.14,0.145,0.15,0.155,0.16,0.165,0.17,0.175,0.18,0.185,0.19,0.195,0.2,0.205,
0.21,0.215,0.22,0.225,0.23,0.235,0.24,0.245,0.25,0.255,0.26,0.265,0.27,
0.275,0.28,0.285,0.29,0.295,0.3,0.305,0.31,0.315,0.32,0.325,0.33,0.335,
0.34,0.345,0.35,0.355,0.36,0.365,0.37,0.375,0.38,0.385,0.39,0.395,0.4,0.405,
0.41,0.415,0.42,0.425,0.43,0.435,0.44,0.445,0.45,0.455,0.46,0.465,0.47,
0.475,0.48,0.485,0.49,0.495,0.5,0.505,0.51,0.515,0.52,0.525,0.53,0.535,
0.54,0.545,0.55,0.555,0.56,0.565,0.57,0.575,0.58,0.585,0.59,0.595,0.6,0.605,
0.61,0.615,0.62,0.625,0.63,0.635,0.64,0.645,0.65,0.655,0.66,0.665,0.67,
0.675,0.68,0.685,0.690000000000001,0.695000000000001,0.700000000000001,
0.705000000000001,0.710000000000001,0.715000000000001,0.720000000000001,
0.725000000000001,0.730000000000001,0.735000000000001,0.740000000000001,
0.745000000000001,0.750000000000001,0.755000000000001,0.760000000000001,
0.765000000000001,0.770000000000001,0.775000000000001,0.780000000000001,
0.785000000000001,0.790000000000001,0.795000000000001,0.800000000000001,
0.805000000000001,0.810000000000001,0.815000000000001,0.820000000000001,
0.825000000000001,0.830000000000001,0.835000000000001,0.840000000000001,
0.845000000000001,0.850000000000001,0.855000000000001,0.860000000000001,
0.865000000000001,0.870000000000001,0.875000000000001,0.880000000000001,
0.885000000000001,0.890000000000001,0.895000000000001,0.900000000000001,
0.905000000000001,0.910000000000001,0.915000000000001,0.920000000000001,
0.925000000000001,0.930000000000001,0.935000000000001,0.940000000000001,
0.945000000000001,0.950000000000001,0.955000000000001,0.960000000000001,
0.965000000000001,0.970000000000001,0.975000000000001,0.980000000000001,
0.985000000000001,0.990000000000001,0.995000000000001,1.),.UNSPECIFIED.)
CURVE()
GEOMETRIC_REPRESENTATION_ITEM()
RATIONAL_B_SPLINE_CURVE((1.,1.,1.,1.,1.,1.,1.,1.,1.,1.,1.,1.,1.,1.,1.,1.,
1.,1.,1.,1.,1.,1.,1.,1.,1.,1.,1.,1.,1.,1.,1.,1.,1.,1.,1.,1.,1.,1.,1.,1.,
1.,1.,1.,1.,1.,1.,1.,1.,1.,1.,1.,1.,1.,1.,1.,1.,1.,1.,1.,1.,1.,1.,1.,1.,
1.,1.,1.,1.,1.,1.,1.,1.,1.,1.,1.,1.,1.,1.,1.,1.,1.,1.,1.,1.,1.,1.,1.,1.,
1.,1.,1.,1.,1.,1.,1.,1.,1.,1.,1.,1.,1.,1.,1.,1.,1.,1.,1.,1.,1.,1.,1.,1.,
1.,1.,1.,1.,1.,1.,1.,1.,1.,1.,1.,1.,1.,1.,1.,1.,1.,1.,1.,1.,1.,1.,1.,1.,
1.,1.,1.,1.,1.,1.,1.,1.,1.,1.,1.,1.,1.,1.,1.,1.,1.,1.,1.,1.,1.,1.,1.,1.,
1.,1.,1.,1.,1.,1.,1.,1.,1.,1.,1.,1.,1.,1.,1.,1.,1.,1.,1.,1.,1.,1.,1.,1.,
1.,1.,1.,1.,1.,1.,1.,1.,1.,1.,1.,1.,1.,1.,1.,1.,1.,1.,1.,1.,1.))
REPRESENTATION_ITEM('')
);
#704=(
BOUNDED_CURVE()
B_SPLINE_CURVE(5,(#177765,#177766,#177767,#177768,#177769,#177770,#177771,
#177772,#177773,#177774,#177775,#177776,#177777,#177778,#177779,#177780,
#177781,#177782,#177783,#177784,#177785,#177786,#177787,#177788,#177789,
#177790,#177791,#177792,#177793,#177794,#177795,#177796,#177797,#177798,
#177799,#177800,#177801,#177802,#177803,#177804,#177805,#177806,#177807,
#177808,#177809,#177810,#177811,#177812,#177813,#177814,#177815,#177816,
#177817,#177818,#177819,#177820,#177821,#177822,#177823,#177824,#177825,
#177826,#177827,#177828,#177829,#177830,#177831,#177832,#177833,#177834,
#177835,#177836,#177837,#177838,#177839,#177840,#177841,#177842,#177843,
#177844,#177845,#177846,#177847,#177848,#177849,#177850,#177851,#177852,
#177853,#177854,#177855,#177856,#177857,#177858,#177859,#177860,#177861,
#177862,#177863,#177864,#177865,#177866,#177867,#177868,#177869,#177870,
#177871,#177872,#177873,#177874,#177875,#177876,#177877,#177878,#177879,
#177880,#177881,#177882,#177883,#177884,#177885,#177886,#177887,#177888,
#177889,#177890,#177891,#177892,#177893,#177894,#177895,#177896,#177897,
#177898,#177899,#177900,#177901,#177902,#177903,#177904,#177905,#177906,
#177907,#177908,#177909,#177910,#177911,#177912,#177913,#177914,#177915,
#177916,#177917,#177918,#177919,#177920,#177921,#177922,#177923,#177924,
#177925,#177926,#177927,#177928,#177929,#177930,#177931,#177932,#177933,
#177934,#177935,#177936,#177937,#177938,#177939,#177940,#177941,#177942,
#177943,#177944,#177945,#177946,#177947,#177948,#177949,#177950,#177951,
#177952,#177953,#177954,#177955,#177956,#177957,#177958,#177959,#177960,
#177961,#177962,#177963,#177964,#177965,#177966,#177967,#177968,#177969),
 .UNSPECIFIED.,.F.,.F.)
B_SPLINE_CURVE_WITH_KNOTS((6,1,1,1,1,1,1,1,1,1,1,1,1,1,1,1,1,1,1,1,1,1,
1,1,1,1,1,1,1,1,1,1,1,1,1,1,1,1,1,1,1,1,1,1,1,1,1,1,1,1,1,1,1,1,1,1,1,1,
1,1,1,1,1,1,1,1,1,1,1,1,1,1,1,1,1,1,1,1,1,1,1,1,1,1,1,1,1,1,1,1,1,1,1,1,
1,1,1,1,1,1,1,1,1,1,1,1,1,1,1,1,1,1,1,1,1,1,1,1,1,1,1,1,1,1,1,1,1,1,1,1,
1,1,1,1,1,1,1,1,1,1,1,1,1,1,1,1,1,1,1,1,1,1,1,1,1,1,1,1,1,1,1,1,1,1,1,1,
1,1,1,1,1,1,1,1,1,1,1,1,1,1,1,1,1,1,1,1,1,1,1,1,1,1,1,1,1,1,1,1,1,1,6),
(-1.,-0.995000000000001,-0.990000000000001,-0.985000000000001,-0.980000000000001,
-0.975000000000001,-0.970000000000001,-0.965000000000001,-0.960000000000001,
-0.955000000000001,-0.950000000000001,-0.945000000000001,-0.940000000000001,
-0.935000000000001,-0.930000000000001,-0.925000000000001,-0.920000000000001,
-0.915000000000001,-0.910000000000001,-0.905000000000001,-0.900000000000001,
-0.895000000000001,-0.890000000000001,-0.885000000000001,-0.880000000000001,
-0.875000000000001,-0.870000000000001,-0.865000000000001,-0.860000000000001,
-0.855000000000001,-0.850000000000001,-0.845000000000001,-0.840000000000001,
-0.835000000000001,-0.830000000000001,-0.825000000000001,-0.820000000000001,
-0.815000000000001,-0.810000000000001,-0.805000000000001,-0.800000000000001,
-0.795000000000001,-0.790000000000001,-0.785000000000001,-0.780000000000001,
-0.775000000000001,-0.770000000000001,-0.765000000000001,-0.760000000000001,
-0.755000000000001,-0.750000000000001,-0.745000000000001,-0.740000000000001,
-0.735000000000001,-0.730000000000001,-0.725000000000001,-0.720000000000001,
-0.715000000000001,-0.710000000000001,-0.705000000000001,-0.700000000000001,
-0.695000000000001,-0.690000000000001,-0.685,-0.68,-0.675,-0.67,-0.665,
-0.66,-0.655,-0.65,-0.645,-0.64,-0.635,-0.63,-0.625,-0.62,-0.615,-0.61,
-0.605,-0.6,-0.595,-0.59,-0.585,-0.58,-0.575,-0.57,-0.565,-0.56,-0.555,
-0.55,-0.545,-0.54,-0.535,-0.53,-0.525,-0.52,-0.515,-0.51,-0.505,-0.5,-0.495,
-0.49,-0.485,-0.48,-0.475,-0.47,-0.465,-0.46,-0.455,-0.45,-0.445,-0.44,
-0.435,-0.43,-0.425,-0.42,-0.415,-0.41,-0.405,-0.4,-0.395,-0.39,-0.385,
-0.38,-0.375,-0.37,-0.365,-0.36,-0.355,-0.35,-0.345,-0.34,-0.335,-0.33,
-0.325,-0.32,-0.315,-0.31,-0.305,-0.3,-0.295,-0.29,-0.285,-0.28,-0.275,
-0.27,-0.265,-0.26,-0.255,-0.25,-0.245,-0.24,-0.235,-0.23,-0.225,-0.22,
-0.215,-0.21,-0.205,-0.2,-0.195,-0.19,-0.185,-0.18,-0.175,-0.17,-0.165,
-0.16,-0.155,-0.15,-0.145,-0.14,-0.135,-0.13,-0.125,-0.12,-0.115,-0.11,
-0.105,-0.1,-0.095,-0.09,-0.085,-0.08,-0.075,-0.07,-0.065,-0.06,-0.055,
-0.05,-0.045,-0.04,-0.035,-0.03,-0.025,-0.02,-0.015,-0.01,-0.005,0.),
 .UNSPECIFIED.)
CURVE()
GEOMETRIC_REPRESENTATION_ITEM()
RATIONAL_B_SPLINE_CURVE((1.,1.,1.,1.,1.,1.,1.,1.,1.,1.,1.,1.,1.,1.,1.,1.,
1.,1.,1.,1.,1.,1.,1.,1.,1.,1.,1.,1.,1.,1.,1.,1.,1.,1.,1.,1.,1.,1.,1.,1.,
1.,1.,1.,1.,1.,1.,1.,1.,1.,1.,1.,1.,1.,1.,1.,1.,1.,1.,1.,1.,1.,1.,1.,1.,
1.,1.,1.,1.,1.,1.,1.,1.,1.,1.,1.,1.,1.,1.,1.,1.,1.,1.,1.,1.,1.,1.,1.,1.,
1.,1.,1.,1.,1.,1.,1.,1.,1.,1.,1.,1.,1.,1.,1.,1.,1.,1.,1.,1.,1.,1.,1.,1.,
1.,1.,1.,1.,1.,1.,1.,1.,1.,1.,1.,1.,1.,1.,1.,1.,1.,1.,1.,1.,1.,1.,1.,1.,
1.,1.,1.,1.,1.,1.,1.,1.,1.,1.,1.,1.,1.,1.,1.,1.,1.,1.,1.,1.,1.,1.,1.,1.,
1.,1.,1.,1.,1.,1.,1.,1.,1.,1.,1.,1.,1.,1.,1.,1.,1.,1.,1.,1.,1.,1.,1.,1.,
1.,1.,1.,1.,1.,1.,1.,1.,1.,1.,1.,1.,1.,1.,1.,1.,1.,1.,1.,1.,1.))
REPRESENTATION_ITEM('')
);
#705=(
BOUNDED_CURVE()
B_SPLINE_CURVE(5,(#177981,#177982,#177983,#177984,#177985,#177986,#177987,
#177988,#177989,#177990,#177991,#177992,#177993,#177994,#177995,#177996,
#177997,#177998,#177999,#178000,#178001,#178002,#178003,#178004,#178005,
#178006,#178007,#178008,#178009,#178010,#178011,#178012,#178013,#178014,
#178015,#178016,#178017,#178018,#178019,#178020,#178021,#178022,#178023,
#178024,#178025,#178026,#178027,#178028,#178029,#178030,#178031,#178032,
#178033,#178034,#178035,#178036,#178037,#178038,#178039,#178040,#178041,
#178042,#178043,#178044,#178045,#178046,#178047,#178048,#178049,#178050,
#178051,#178052,#178053,#178054,#178055,#178056,#178057,#178058,#178059,
#178060,#178061,#178062,#178063,#178064,#178065,#178066,#178067,#178068,
#178069,#178070,#178071,#178072,#178073,#178074,#178075,#178076,#178077,
#178078,#178079,#178080,#178081,#178082,#178083,#178084,#178085,#178086,
#178087,#178088,#178089,#178090,#178091,#178092,#178093,#178094,#178095,
#178096,#178097,#178098,#178099,#178100,#178101,#178102,#178103,#178104,
#178105,#178106,#178107,#178108,#178109,#178110,#178111,#178112,#178113,
#178114,#178115,#178116,#178117,#178118,#178119,#178120,#178121,#178122,
#178123,#178124,#178125,#178126,#178127,#178128,#178129,#178130,#178131,
#178132,#178133,#178134,#178135,#178136,#178137,#178138,#178139,#178140,
#178141,#178142,#178143,#178144,#178145,#178146,#178147,#178148,#178149,
#178150,#178151,#178152,#178153,#178154,#178155,#178156,#178157,#178158,
#178159,#178160,#178161,#178162,#178163,#178164,#178165,#178166,#178167,
#178168,#178169,#178170,#178171,#178172,#178173,#178174,#178175,#178176,
#178177,#178178,#178179,#178180,#178181,#178182,#178183,#178184,#178185),
 .UNSPECIFIED.,.F.,.F.)
B_SPLINE_CURVE_WITH_KNOTS((6,1,1,1,1,1,1,1,1,1,1,1,1,1,1,1,1,1,1,1,1,1,
1,1,1,1,1,1,1,1,1,1,1,1,1,1,1,1,1,1,1,1,1,1,1,1,1,1,1,1,1,1,1,1,1,1,1,1,
1,1,1,1,1,1,1,1,1,1,1,1,1,1,1,1,1,1,1,1,1,1,1,1,1,1,1,1,1,1,1,1,1,1,1,1,
1,1,1,1,1,1,1,1,1,1,1,1,1,1,1,1,1,1,1,1,1,1,1,1,1,1,1,1,1,1,1,1,1,1,1,1,
1,1,1,1,1,1,1,1,1,1,1,1,1,1,1,1,1,1,1,1,1,1,1,1,1,1,1,1,1,1,1,1,1,1,1,1,
1,1,1,1,1,1,1,1,1,1,1,1,1,1,1,1,1,1,1,1,1,1,1,1,1,1,1,1,1,1,1,1,1,1,6),
(0.,0.005,0.01,0.015,0.02,0.025,0.03,0.035,0.04,0.045,0.05,0.055,0.06,0.065,
0.07,0.075,0.08,0.085,0.09,0.095,0.1,0.105,0.11,0.115,0.12,0.125,0.13,0.135,
0.14,0.145,0.15,0.155,0.16,0.165,0.17,0.175,0.18,0.185,0.19,0.195,0.2,0.205,
0.21,0.215,0.22,0.225,0.23,0.235,0.24,0.245,0.25,0.255,0.26,0.265,0.27,
0.275,0.28,0.285,0.29,0.295,0.3,0.305,0.31,0.315,0.32,0.325,0.33,0.335,
0.34,0.345,0.35,0.355,0.36,0.365,0.37,0.375,0.38,0.385,0.39,0.395,0.4,0.405,
0.41,0.415,0.42,0.425,0.43,0.435,0.44,0.445,0.45,0.455,0.46,0.465,0.47,
0.475,0.48,0.485,0.49,0.495,0.5,0.505,0.51,0.515,0.52,0.525,0.53,0.535,
0.54,0.545,0.55,0.555,0.56,0.565,0.57,0.575,0.58,0.585,0.59,0.595,0.6,0.605,
0.61,0.615,0.62,0.625,0.63,0.635,0.64,0.645,0.65,0.655,0.66,0.665,0.67,
0.675,0.68,0.685,0.690000000000001,0.695000000000001,0.700000000000001,
0.705000000000001,0.710000000000001,0.715000000000001,0.720000000000001,
0.725000000000001,0.730000000000001,0.735000000000001,0.740000000000001,
0.745000000000001,0.750000000000001,0.755000000000001,0.760000000000001,
0.765000000000001,0.770000000000001,0.775000000000001,0.780000000000001,
0.785000000000001,0.790000000000001,0.795000000000001,0.800000000000001,
0.805000000000001,0.810000000000001,0.815000000000001,0.820000000000001,
0.825000000000001,0.830000000000001,0.835000000000001,0.840000000000001,
0.845000000000001,0.850000000000001,0.855000000000001,0.860000000000001,
0.865000000000001,0.870000000000001,0.875000000000001,0.880000000000001,
0.885000000000001,0.890000000000001,0.895000000000001,0.900000000000001,
0.905000000000001,0.910000000000001,0.915000000000001,0.920000000000001,
0.925000000000001,0.930000000000001,0.935000000000001,0.940000000000001,
0.945000000000001,0.950000000000001,0.955000000000001,0.960000000000001,
0.965000000000001,0.970000000000001,0.975000000000001,0.980000000000001,
0.985000000000001,0.990000000000001,0.995000000000001,1.),.UNSPECIFIED.)
CURVE()
GEOMETRIC_REPRESENTATION_ITEM()
RATIONAL_B_SPLINE_CURVE((1.,1.,1.,1.,1.,1.,1.,1.,1.,1.,1.,1.,1.,1.,1.,1.,
1.,1.,1.,1.,1.,1.,1.,1.,1.,1.,1.,1.,1.,1.,1.,1.,1.,1.,1.,1.,1.,1.,1.,1.,
1.,1.,1.,1.,1.,1.,1.,1.,1.,1.,1.,1.,1.,1.,1.,1.,1.,1.,1.,1.,1.,1.,1.,1.,
1.,1.,1.,1.,1.,1.,1.,1.,1.,1.,1.,1.,1.,1.,1.,1.,1.,1.,1.,1.,1.,1.,1.,1.,
1.,1.,1.,1.,1.,1.,1.,1.,1.,1.,1.,1.,1.,1.,1.,1.,1.,1.,1.,1.,1.,1.,1.,1.,
1.,1.,1.,1.,1.,1.,1.,1.,1.,1.,1.,1.,1.,1.,1.,1.,1.,1.,1.,1.,1.,1.,1.,1.,
1.,1.,1.,1.,1.,1.,1.,1.,1.,1.,1.,1.,1.,1.,1.,1.,1.,1.,1.,1.,1.,1.,1.,1.,
1.,1.,1.,1.,1.,1.,1.,1.,1.,1.,1.,1.,1.,1.,1.,1.,1.,1.,1.,1.,1.,1.,1.,1.,
1.,1.,1.,1.,1.,1.,1.,1.,1.,1.,1.,1.,1.,1.,1.,1.,1.,1.,1.,1.,1.))
REPRESENTATION_ITEM('')
);
#706=(
BOUNDED_CURVE()
B_SPLINE_CURVE(5,(#178189,#178190,#178191,#178192,#178193,#178194,#178195,
#178196,#178197,#178198,#178199,#178200,#178201,#178202,#178203,#178204,
#178205,#178206,#178207,#178208,#178209,#178210,#178211,#178212,#178213,
#178214,#178215,#178216,#178217,#178218,#178219,#178220,#178221,#178222,
#178223,#178224,#178225,#178226,#178227,#178228,#178229,#178230,#178231,
#178232,#178233,#178234,#178235,#178236,#178237,#178238,#178239,#178240,
#178241,#178242,#178243,#178244,#178245,#178246,#178247,#178248,#178249,
#178250,#178251,#178252,#178253,#178254,#178255,#178256,#178257,#178258,
#178259,#178260,#178261,#178262,#178263,#178264,#178265,#178266,#178267,
#178268,#178269,#178270,#178271,#178272,#178273,#178274,#178275,#178276,
#178277,#178278,#178279,#178280,#178281,#178282,#178283,#178284,#178285,
#178286,#178287,#178288,#178289,#178290,#178291,#178292,#178293,#178294,
#178295,#178296,#178297,#178298,#178299,#178300,#178301,#178302,#178303,
#178304,#178305,#178306,#178307,#178308,#178309,#178310,#178311,#178312,
#178313,#178314,#178315,#178316,#178317,#178318,#178319,#178320,#178321,
#178322,#178323,#178324,#178325,#178326,#178327,#178328,#178329,#178330,
#178331,#178332,#178333,#178334,#178335,#178336,#178337,#178338,#178339,
#178340,#178341,#178342,#178343,#178344,#178345,#178346,#178347,#178348,
#178349,#178350,#178351,#178352,#178353,#178354,#178355,#178356,#178357,
#178358,#178359,#178360,#178361,#178362,#178363,#178364,#178365,#178366,
#178367,#178368,#178369,#178370,#178371,#178372,#178373,#178374,#178375,
#178376,#178377,#178378,#178379,#178380,#178381,#178382,#178383,#178384,
#178385,#178386,#178387,#178388,#178389,#178390,#178391,#178392,#178393),
 .UNSPECIFIED.,.F.,.F.)
B_SPLINE_CURVE_WITH_KNOTS((6,1,1,1,1,1,1,1,1,1,1,1,1,1,1,1,1,1,1,1,1,1,
1,1,1,1,1,1,1,1,1,1,1,1,1,1,1,1,1,1,1,1,1,1,1,1,1,1,1,1,1,1,1,1,1,1,1,1,
1,1,1,1,1,1,1,1,1,1,1,1,1,1,1,1,1,1,1,1,1,1,1,1,1,1,1,1,1,1,1,1,1,1,1,1,
1,1,1,1,1,1,1,1,1,1,1,1,1,1,1,1,1,1,1,1,1,1,1,1,1,1,1,1,1,1,1,1,1,1,1,1,
1,1,1,1,1,1,1,1,1,1,1,1,1,1,1,1,1,1,1,1,1,1,1,1,1,1,1,1,1,1,1,1,1,1,1,1,
1,1,1,1,1,1,1,1,1,1,1,1,1,1,1,1,1,1,1,1,1,1,1,1,1,1,1,1,1,1,1,1,1,1,6),
(-1.,-0.995000000000001,-0.990000000000001,-0.985000000000001,-0.980000000000001,
-0.975000000000001,-0.970000000000001,-0.965000000000001,-0.960000000000001,
-0.955000000000001,-0.950000000000001,-0.945000000000001,-0.940000000000001,
-0.935000000000001,-0.930000000000001,-0.925000000000001,-0.920000000000001,
-0.915000000000001,-0.910000000000001,-0.905000000000001,-0.900000000000001,
-0.895000000000001,-0.890000000000001,-0.885000000000001,-0.880000000000001,
-0.875000000000001,-0.870000000000001,-0.865000000000001,-0.860000000000001,
-0.855000000000001,-0.850000000000001,-0.845000000000001,-0.840000000000001,
-0.835000000000001,-0.830000000000001,-0.825000000000001,-0.820000000000001,
-0.815000000000001,-0.810000000000001,-0.805000000000001,-0.800000000000001,
-0.795000000000001,-0.790000000000001,-0.785000000000001,-0.780000000000001,
-0.775000000000001,-0.770000000000001,-0.765000000000001,-0.760000000000001,
-0.755000000000001,-0.750000000000001,-0.745000000000001,-0.740000000000001,
-0.735000000000001,-0.730000000000001,-0.725000000000001,-0.720000000000001,
-0.715000000000001,-0.710000000000001,-0.705000000000001,-0.700000000000001,
-0.695000000000001,-0.690000000000001,-0.685,-0.68,-0.675,-0.67,-0.665,
-0.66,-0.655,-0.65,-0.645,-0.64,-0.635,-0.63,-0.625,-0.62,-0.615,-0.61,
-0.605,-0.6,-0.595,-0.59,-0.585,-0.58,-0.575,-0.57,-0.565,-0.56,-0.555,
-0.55,-0.545,-0.54,-0.535,-0.53,-0.525,-0.52,-0.515,-0.51,-0.505,-0.5,-0.495,
-0.49,-0.485,-0.48,-0.475,-0.47,-0.465,-0.46,-0.455,-0.45,-0.445,-0.44,
-0.435,-0.43,-0.425,-0.42,-0.415,-0.41,-0.405,-0.4,-0.395,-0.39,-0.385,
-0.38,-0.375,-0.37,-0.365,-0.36,-0.355,-0.35,-0.345,-0.34,-0.335,-0.33,
-0.325,-0.32,-0.315,-0.31,-0.305,-0.3,-0.295,-0.29,-0.285,-0.28,-0.275,
-0.27,-0.265,-0.26,-0.255,-0.25,-0.245,-0.24,-0.235,-0.23,-0.225,-0.22,
-0.215,-0.21,-0.205,-0.2,-0.195,-0.19,-0.185,-0.18,-0.175,-0.17,-0.165,
-0.16,-0.155,-0.15,-0.145,-0.14,-0.135,-0.13,-0.125,-0.12,-0.115,-0.11,
-0.105,-0.1,-0.095,-0.09,-0.085,-0.08,-0.075,-0.07,-0.065,-0.06,-0.055,
-0.05,-0.045,-0.04,-0.035,-0.03,-0.025,-0.02,-0.015,-0.01,-0.005,0.),
 .UNSPECIFIED.)
CURVE()
GEOMETRIC_REPRESENTATION_ITEM()
RATIONAL_B_SPLINE_CURVE((1.,1.,1.,1.,1.,1.,1.,1.,1.,1.,1.,1.,1.,1.,1.,1.,
1.,1.,1.,1.,1.,1.,1.,1.,1.,1.,1.,1.,1.,1.,1.,1.,1.,1.,1.,1.,1.,1.,1.,1.,
1.,1.,1.,1.,1.,1.,1.,1.,1.,1.,1.,1.,1.,1.,1.,1.,1.,1.,1.,1.,1.,1.,1.,1.,
1.,1.,1.,1.,1.,1.,1.,1.,1.,1.,1.,1.,1.,1.,1.,1.,1.,1.,1.,1.,1.,1.,1.,1.,
1.,1.,1.,1.,1.,1.,1.,1.,1.,1.,1.,1.,1.,1.,1.,1.,1.,1.,1.,1.,1.,1.,1.,1.,
1.,1.,1.,1.,1.,1.,1.,1.,1.,1.,1.,1.,1.,1.,1.,1.,1.,1.,1.,1.,1.,1.,1.,1.,
1.,1.,1.,1.,1.,1.,1.,1.,1.,1.,1.,1.,1.,1.,1.,1.,1.,1.,1.,1.,1.,1.,1.,1.,
1.,1.,1.,1.,1.,1.,1.,1.,1.,1.,1.,1.,1.,1.,1.,1.,1.,1.,1.,1.,1.,1.,1.,1.,
1.,1.,1.,1.,1.,1.,1.,1.,1.,1.,1.,1.,1.,1.,1.,1.,1.,1.,1.,1.,1.))
REPRESENTATION_ITEM('')
);
#707=(
BOUNDED_CURVE()
B_SPLINE_CURVE(5,(#178405,#178406,#178407,#178408,#178409,#178410,#178411,
#178412,#178413,#178414,#178415,#178416,#178417,#178418,#178419,#178420,
#178421,#178422,#178423,#178424,#178425,#178426,#178427,#178428,#178429,
#178430,#178431,#178432,#178433,#178434,#178435,#178436,#178437,#178438,
#178439,#178440,#178441,#178442,#178443,#178444,#178445,#178446,#178447,
#178448,#178449,#178450,#178451,#178452,#178453,#178454,#178455,#178456,
#178457,#178458,#178459,#178460,#178461,#178462,#178463,#178464,#178465,
#178466,#178467,#178468,#178469,#178470,#178471,#178472,#178473,#178474,
#178475,#178476,#178477,#178478,#178479,#178480,#178481,#178482,#178483,
#178484,#178485,#178486,#178487,#178488,#178489,#178490,#178491,#178492,
#178493,#178494,#178495,#178496,#178497,#178498,#178499,#178500,#178501,
#178502,#178503,#178504,#178505,#178506,#178507,#178508,#178509,#178510,
#178511,#178512,#178513,#178514,#178515,#178516,#178517,#178518,#178519,
#178520,#178521,#178522,#178523,#178524,#178525,#178526,#178527,#178528,
#178529,#178530,#178531,#178532,#178533,#178534,#178535,#178536,#178537,
#178538,#178539,#178540,#178541,#178542,#178543,#178544,#178545,#178546,
#178547,#178548,#178549,#178550,#178551,#178552,#178553,#178554,#178555,
#178556,#178557,#178558,#178559,#178560,#178561,#178562,#178563,#178564,
#178565,#178566,#178567,#178568,#178569,#178570,#178571,#178572,#178573,
#178574,#178575,#178576,#178577,#178578,#178579,#178580,#178581,#178582,
#178583,#178584,#178585,#178586,#178587,#178588,#178589,#178590,#178591,
#178592,#178593,#178594,#178595,#178596,#178597,#178598,#178599,#178600,
#178601,#178602,#178603,#178604,#178605,#178606,#178607,#178608,#178609),
 .UNSPECIFIED.,.F.,.F.)
B_SPLINE_CURVE_WITH_KNOTS((6,1,1,1,1,1,1,1,1,1,1,1,1,1,1,1,1,1,1,1,1,1,
1,1,1,1,1,1,1,1,1,1,1,1,1,1,1,1,1,1,1,1,1,1,1,1,1,1,1,1,1,1,1,1,1,1,1,1,
1,1,1,1,1,1,1,1,1,1,1,1,1,1,1,1,1,1,1,1,1,1,1,1,1,1,1,1,1,1,1,1,1,1,1,1,
1,1,1,1,1,1,1,1,1,1,1,1,1,1,1,1,1,1,1,1,1,1,1,1,1,1,1,1,1,1,1,1,1,1,1,1,
1,1,1,1,1,1,1,1,1,1,1,1,1,1,1,1,1,1,1,1,1,1,1,1,1,1,1,1,1,1,1,1,1,1,1,1,
1,1,1,1,1,1,1,1,1,1,1,1,1,1,1,1,1,1,1,1,1,1,1,1,1,1,1,1,1,1,1,1,1,1,6),
(0.,0.005,0.01,0.015,0.02,0.025,0.03,0.035,0.04,0.045,0.05,0.055,0.06,0.065,
0.07,0.075,0.08,0.085,0.09,0.095,0.1,0.105,0.11,0.115,0.12,0.125,0.13,0.135,
0.14,0.145,0.15,0.155,0.16,0.165,0.17,0.175,0.18,0.185,0.19,0.195,0.2,0.205,
0.21,0.215,0.22,0.225,0.23,0.235,0.24,0.245,0.25,0.255,0.26,0.265,0.27,
0.275,0.28,0.285,0.29,0.295,0.3,0.305,0.31,0.315,0.32,0.325,0.33,0.335,
0.34,0.345,0.35,0.355,0.36,0.365,0.37,0.375,0.38,0.385,0.39,0.395,0.4,0.405,
0.41,0.415,0.42,0.425,0.43,0.435,0.44,0.445,0.45,0.455,0.46,0.465,0.47,
0.475,0.48,0.485,0.49,0.495,0.5,0.505,0.51,0.515,0.52,0.525,0.53,0.535,
0.54,0.545,0.55,0.555,0.56,0.565,0.57,0.575,0.58,0.585,0.59,0.595,0.6,0.605,
0.61,0.615,0.62,0.625,0.63,0.635,0.64,0.645,0.65,0.655,0.66,0.665,0.67,
0.675,0.68,0.685,0.690000000000001,0.695000000000001,0.700000000000001,
0.705000000000001,0.710000000000001,0.715000000000001,0.720000000000001,
0.725000000000001,0.730000000000001,0.735000000000001,0.740000000000001,
0.745000000000001,0.750000000000001,0.755000000000001,0.760000000000001,
0.765000000000001,0.770000000000001,0.775000000000001,0.780000000000001,
0.785000000000001,0.790000000000001,0.795000000000001,0.800000000000001,
0.805000000000001,0.810000000000001,0.815000000000001,0.820000000000001,
0.825000000000001,0.830000000000001,0.835000000000001,0.840000000000001,
0.845000000000001,0.850000000000001,0.855000000000001,0.860000000000001,
0.865000000000001,0.870000000000001,0.875000000000001,0.880000000000001,
0.885000000000001,0.890000000000001,0.895000000000001,0.900000000000001,
0.905000000000001,0.910000000000001,0.915000000000001,0.920000000000001,
0.925000000000001,0.930000000000001,0.935000000000001,0.940000000000001,
0.945000000000001,0.950000000000001,0.955000000000001,0.960000000000001,
0.965000000000001,0.970000000000001,0.975000000000001,0.980000000000001,
0.985000000000001,0.990000000000001,0.995000000000001,1.),.UNSPECIFIED.)
CURVE()
GEOMETRIC_REPRESENTATION_ITEM()
RATIONAL_B_SPLINE_CURVE((1.,1.,1.,1.,1.,1.,1.,1.,1.,1.,1.,1.,1.,1.,1.,1.,
1.,1.,1.,1.,1.,1.,1.,1.,1.,1.,1.,1.,1.,1.,1.,1.,1.,1.,1.,1.,1.,1.,1.,1.,
1.,1.,1.,1.,1.,1.,1.,1.,1.,1.,1.,1.,1.,1.,1.,1.,1.,1.,1.,1.,1.,1.,1.,1.,
1.,1.,1.,1.,1.,1.,1.,1.,1.,1.,1.,1.,1.,1.,1.,1.,1.,1.,1.,1.,1.,1.,1.,1.,
1.,1.,1.,1.,1.,1.,1.,1.,1.,1.,1.,1.,1.,1.,1.,1.,1.,1.,1.,1.,1.,1.,1.,1.,
1.,1.,1.,1.,1.,1.,1.,1.,1.,1.,1.,1.,1.,1.,1.,1.,1.,1.,1.,1.,1.,1.,1.,1.,
1.,1.,1.,1.,1.,1.,1.,1.,1.,1.,1.,1.,1.,1.,1.,1.,1.,1.,1.,1.,1.,1.,1.,1.,
1.,1.,1.,1.,1.,1.,1.,1.,1.,1.,1.,1.,1.,1.,1.,1.,1.,1.,1.,1.,1.,1.,1.,1.,
1.,1.,1.,1.,1.,1.,1.,1.,1.,1.,1.,1.,1.,1.,1.,1.,1.,1.,1.,1.,1.))
REPRESENTATION_ITEM('')
);
#708=(
BOUNDED_CURVE()
B_SPLINE_CURVE(5,(#178613,#178614,#178615,#178616,#178617,#178618,#178619,
#178620,#178621,#178622,#178623,#178624,#178625,#178626,#178627,#178628,
#178629,#178630,#178631,#178632,#178633,#178634,#178635,#178636,#178637,
#178638,#178639,#178640,#178641,#178642,#178643,#178644,#178645,#178646,
#178647,#178648,#178649,#178650,#178651,#178652,#178653,#178654,#178655,
#178656,#178657,#178658,#178659,#178660,#178661,#178662,#178663,#178664,
#178665,#178666,#178667,#178668,#178669,#178670,#178671,#178672,#178673,
#178674,#178675,#178676,#178677,#178678,#178679,#178680,#178681,#178682,
#178683,#178684,#178685,#178686,#178687,#178688,#178689,#178690,#178691,
#178692,#178693,#178694,#178695,#178696,#178697,#178698,#178699,#178700,
#178701,#178702,#178703,#178704,#178705,#178706,#178707,#178708,#178709,
#178710,#178711,#178712,#178713,#178714,#178715,#178716,#178717,#178718,
#178719,#178720,#178721,#178722,#178723,#178724,#178725,#178726,#178727,
#178728,#178729,#178730,#178731,#178732,#178733,#178734,#178735,#178736,
#178737,#178738,#178739,#178740,#178741,#178742,#178743,#178744,#178745,
#178746,#178747,#178748,#178749,#178750,#178751,#178752,#178753,#178754,
#178755,#178756,#178757,#178758,#178759,#178760,#178761,#178762,#178763,
#178764,#178765,#178766,#178767,#178768,#178769,#178770,#178771,#178772,
#178773,#178774,#178775,#178776,#178777,#178778,#178779,#178780,#178781,
#178782,#178783,#178784,#178785,#178786,#178787,#178788,#178789,#178790,
#178791,#178792,#178793,#178794,#178795,#178796,#178797,#178798,#178799,
#178800,#178801,#178802,#178803,#178804,#178805,#178806,#178807,#178808,
#178809,#178810,#178811,#178812,#178813,#178814,#178815,#178816,#178817),
 .UNSPECIFIED.,.F.,.F.)
B_SPLINE_CURVE_WITH_KNOTS((6,1,1,1,1,1,1,1,1,1,1,1,1,1,1,1,1,1,1,1,1,1,
1,1,1,1,1,1,1,1,1,1,1,1,1,1,1,1,1,1,1,1,1,1,1,1,1,1,1,1,1,1,1,1,1,1,1,1,
1,1,1,1,1,1,1,1,1,1,1,1,1,1,1,1,1,1,1,1,1,1,1,1,1,1,1,1,1,1,1,1,1,1,1,1,
1,1,1,1,1,1,1,1,1,1,1,1,1,1,1,1,1,1,1,1,1,1,1,1,1,1,1,1,1,1,1,1,1,1,1,1,
1,1,1,1,1,1,1,1,1,1,1,1,1,1,1,1,1,1,1,1,1,1,1,1,1,1,1,1,1,1,1,1,1,1,1,1,
1,1,1,1,1,1,1,1,1,1,1,1,1,1,1,1,1,1,1,1,1,1,1,1,1,1,1,1,1,1,1,1,1,1,6),
(-1.,-0.995000000000001,-0.990000000000001,-0.985000000000001,-0.980000000000001,
-0.975000000000001,-0.970000000000001,-0.965000000000001,-0.960000000000001,
-0.955000000000001,-0.950000000000001,-0.945000000000001,-0.940000000000001,
-0.935000000000001,-0.930000000000001,-0.925000000000001,-0.920000000000001,
-0.915000000000001,-0.910000000000001,-0.905000000000001,-0.900000000000001,
-0.895000000000001,-0.890000000000001,-0.885000000000001,-0.880000000000001,
-0.875000000000001,-0.870000000000001,-0.865000000000001,-0.860000000000001,
-0.855000000000001,-0.850000000000001,-0.845000000000001,-0.840000000000001,
-0.835000000000001,-0.830000000000001,-0.825000000000001,-0.820000000000001,
-0.815000000000001,-0.810000000000001,-0.805000000000001,-0.800000000000001,
-0.795000000000001,-0.790000000000001,-0.785000000000001,-0.780000000000001,
-0.775000000000001,-0.770000000000001,-0.765000000000001,-0.760000000000001,
-0.755000000000001,-0.750000000000001,-0.745000000000001,-0.740000000000001,
-0.735000000000001,-0.730000000000001,-0.725000000000001,-0.720000000000001,
-0.715000000000001,-0.710000000000001,-0.705000000000001,-0.700000000000001,
-0.695000000000001,-0.690000000000001,-0.685,-0.68,-0.675,-0.67,-0.665,
-0.66,-0.655,-0.65,-0.645,-0.64,-0.635,-0.63,-0.625,-0.62,-0.615,-0.61,
-0.605,-0.6,-0.595,-0.59,-0.585,-0.58,-0.575,-0.57,-0.565,-0.56,-0.555,
-0.55,-0.545,-0.54,-0.535,-0.53,-0.525,-0.52,-0.515,-0.51,-0.505,-0.5,-0.495,
-0.49,-0.485,-0.48,-0.475,-0.47,-0.465,-0.46,-0.455,-0.45,-0.445,-0.44,
-0.435,-0.43,-0.425,-0.42,-0.415,-0.41,-0.405,-0.4,-0.395,-0.39,-0.385,
-0.38,-0.375,-0.37,-0.365,-0.36,-0.355,-0.35,-0.345,-0.34,-0.335,-0.33,
-0.325,-0.32,-0.315,-0.31,-0.305,-0.3,-0.295,-0.29,-0.285,-0.28,-0.275,
-0.27,-0.265,-0.26,-0.255,-0.25,-0.245,-0.24,-0.235,-0.23,-0.225,-0.22,
-0.215,-0.21,-0.205,-0.2,-0.195,-0.19,-0.185,-0.18,-0.175,-0.17,-0.165,
-0.16,-0.155,-0.15,-0.145,-0.14,-0.135,-0.13,-0.125,-0.12,-0.115,-0.11,
-0.105,-0.1,-0.095,-0.09,-0.085,-0.08,-0.075,-0.07,-0.065,-0.06,-0.055,
-0.05,-0.045,-0.04,-0.035,-0.03,-0.025,-0.02,-0.015,-0.01,-0.005,0.),
 .UNSPECIFIED.)
CURVE()
GEOMETRIC_REPRESENTATION_ITEM()
RATIONAL_B_SPLINE_CURVE((1.,1.,1.,1.,1.,1.,1.,1.,1.,1.,1.,1.,1.,1.,1.,1.,
1.,1.,1.,1.,1.,1.,1.,1.,1.,1.,1.,1.,1.,1.,1.,1.,1.,1.,1.,1.,1.,1.,1.,1.,
1.,1.,1.,1.,1.,1.,1.,1.,1.,1.,1.,1.,1.,1.,1.,1.,1.,1.,1.,1.,1.,1.,1.,1.,
1.,1.,1.,1.,1.,1.,1.,1.,1.,1.,1.,1.,1.,1.,1.,1.,1.,1.,1.,1.,1.,1.,1.,1.,
1.,1.,1.,1.,1.,1.,1.,1.,1.,1.,1.,1.,1.,1.,1.,1.,1.,1.,1.,1.,1.,1.,1.,1.,
1.,1.,1.,1.,1.,1.,1.,1.,1.,1.,1.,1.,1.,1.,1.,1.,1.,1.,1.,1.,1.,1.,1.,1.,
1.,1.,1.,1.,1.,1.,1.,1.,1.,1.,1.,1.,1.,1.,1.,1.,1.,1.,1.,1.,1.,1.,1.,1.,
1.,1.,1.,1.,1.,1.,1.,1.,1.,1.,1.,1.,1.,1.,1.,1.,1.,1.,1.,1.,1.,1.,1.,1.,
1.,1.,1.,1.,1.,1.,1.,1.,1.,1.,1.,1.,1.,1.,1.,1.,1.,1.,1.,1.,1.))
REPRESENTATION_ITEM('')
);
#709=(
BOUNDED_CURVE()
B_SPLINE_CURVE(5,(#178829,#178830,#178831,#178832,#178833,#178834,#178835,
#178836,#178837,#178838,#178839,#178840,#178841,#178842,#178843,#178844,
#178845,#178846,#178847,#178848,#178849,#178850,#178851,#178852,#178853,
#178854,#178855,#178856,#178857,#178858,#178859,#178860,#178861,#178862,
#178863,#178864,#178865,#178866,#178867,#178868,#178869,#178870,#178871,
#178872,#178873,#178874,#178875,#178876,#178877,#178878,#178879,#178880,
#178881,#178882,#178883,#178884,#178885,#178886,#178887,#178888,#178889,
#178890,#178891,#178892,#178893,#178894,#178895,#178896,#178897,#178898,
#178899,#178900,#178901,#178902,#178903,#178904,#178905,#178906,#178907,
#178908,#178909,#178910,#178911,#178912,#178913,#178914,#178915,#178916,
#178917,#178918,#178919,#178920,#178921,#178922,#178923,#178924,#178925,
#178926,#178927,#178928,#178929,#178930,#178931,#178932,#178933,#178934,
#178935,#178936,#178937,#178938,#178939,#178940,#178941,#178942,#178943,
#178944,#178945,#178946,#178947,#178948,#178949,#178950,#178951,#178952,
#178953,#178954,#178955,#178956,#178957,#178958,#178959,#178960,#178961,
#178962,#178963,#178964,#178965,#178966,#178967,#178968,#178969,#178970,
#178971,#178972,#178973,#178974,#178975,#178976,#178977,#178978,#178979,
#178980,#178981,#178982,#178983,#178984,#178985,#178986,#178987,#178988,
#178989,#178990,#178991,#178992,#178993,#178994,#178995,#178996,#178997,
#178998,#178999,#179000,#179001,#179002,#179003,#179004,#179005,#179006,
#179007,#179008,#179009,#179010,#179011,#179012,#179013,#179014,#179015,
#179016,#179017,#179018,#179019,#179020,#179021,#179022,#179023,#179024,
#179025,#179026,#179027,#179028,#179029,#179030,#179031,#179032,#179033),
 .UNSPECIFIED.,.F.,.F.)
B_SPLINE_CURVE_WITH_KNOTS((6,1,1,1,1,1,1,1,1,1,1,1,1,1,1,1,1,1,1,1,1,1,
1,1,1,1,1,1,1,1,1,1,1,1,1,1,1,1,1,1,1,1,1,1,1,1,1,1,1,1,1,1,1,1,1,1,1,1,
1,1,1,1,1,1,1,1,1,1,1,1,1,1,1,1,1,1,1,1,1,1,1,1,1,1,1,1,1,1,1,1,1,1,1,1,
1,1,1,1,1,1,1,1,1,1,1,1,1,1,1,1,1,1,1,1,1,1,1,1,1,1,1,1,1,1,1,1,1,1,1,1,
1,1,1,1,1,1,1,1,1,1,1,1,1,1,1,1,1,1,1,1,1,1,1,1,1,1,1,1,1,1,1,1,1,1,1,1,
1,1,1,1,1,1,1,1,1,1,1,1,1,1,1,1,1,1,1,1,1,1,1,1,1,1,1,1,1,1,1,1,1,1,6),
(0.,0.005,0.01,0.015,0.02,0.025,0.03,0.035,0.04,0.045,0.05,0.055,0.06,0.065,
0.07,0.075,0.08,0.085,0.09,0.095,0.1,0.105,0.11,0.115,0.12,0.125,0.13,0.135,
0.14,0.145,0.15,0.155,0.16,0.165,0.17,0.175,0.18,0.185,0.19,0.195,0.2,0.205,
0.21,0.215,0.22,0.225,0.23,0.235,0.24,0.245,0.25,0.255,0.26,0.265,0.27,
0.275,0.28,0.285,0.29,0.295,0.3,0.305,0.31,0.315,0.32,0.325,0.33,0.335,
0.34,0.345,0.35,0.355,0.36,0.365,0.37,0.375,0.38,0.385,0.39,0.395,0.4,0.405,
0.41,0.415,0.42,0.425,0.43,0.435,0.44,0.445,0.45,0.455,0.46,0.465,0.47,
0.475,0.48,0.485,0.49,0.495,0.5,0.505,0.51,0.515,0.52,0.525,0.53,0.535,
0.54,0.545,0.55,0.555,0.56,0.565,0.57,0.575,0.58,0.585,0.59,0.595,0.6,0.605,
0.61,0.615,0.62,0.625,0.63,0.635,0.64,0.645,0.65,0.655,0.66,0.665,0.67,
0.675,0.68,0.685,0.690000000000001,0.695000000000001,0.700000000000001,
0.705000000000001,0.710000000000001,0.715000000000001,0.720000000000001,
0.725000000000001,0.730000000000001,0.735000000000001,0.740000000000001,
0.745000000000001,0.750000000000001,0.755000000000001,0.760000000000001,
0.765000000000001,0.770000000000001,0.775000000000001,0.780000000000001,
0.785000000000001,0.790000000000001,0.795000000000001,0.800000000000001,
0.805000000000001,0.810000000000001,0.815000000000001,0.820000000000001,
0.825000000000001,0.830000000000001,0.835000000000001,0.840000000000001,
0.845000000000001,0.850000000000001,0.855000000000001,0.860000000000001,
0.865000000000001,0.870000000000001,0.875000000000001,0.880000000000001,
0.885000000000001,0.890000000000001,0.895000000000001,0.900000000000001,
0.905000000000001,0.910000000000001,0.915000000000001,0.920000000000001,
0.925000000000001,0.930000000000001,0.935000000000001,0.940000000000001,
0.945000000000001,0.950000000000001,0.955000000000001,0.960000000000001,
0.965000000000001,0.970000000000001,0.975000000000001,0.980000000000001,
0.985000000000001,0.990000000000001,0.995000000000001,1.),.UNSPECIFIED.)
CURVE()
GEOMETRIC_REPRESENTATION_ITEM()
RATIONAL_B_SPLINE_CURVE((1.,1.,1.,1.,1.,1.,1.,1.,1.,1.,1.,1.,1.,1.,1.,1.,
1.,1.,1.,1.,1.,1.,1.,1.,1.,1.,1.,1.,1.,1.,1.,1.,1.,1.,1.,1.,1.,1.,1.,1.,
1.,1.,1.,1.,1.,1.,1.,1.,1.,1.,1.,1.,1.,1.,1.,1.,1.,1.,1.,1.,1.,1.,1.,1.,
1.,1.,1.,1.,1.,1.,1.,1.,1.,1.,1.,1.,1.,1.,1.,1.,1.,1.,1.,1.,1.,1.,1.,1.,
1.,1.,1.,1.,1.,1.,1.,1.,1.,1.,1.,1.,1.,1.,1.,1.,1.,1.,1.,1.,1.,1.,1.,1.,
1.,1.,1.,1.,1.,1.,1.,1.,1.,1.,1.,1.,1.,1.,1.,1.,1.,1.,1.,1.,1.,1.,1.,1.,
1.,1.,1.,1.,1.,1.,1.,1.,1.,1.,1.,1.,1.,1.,1.,1.,1.,1.,1.,1.,1.,1.,1.,1.,
1.,1.,1.,1.,1.,1.,1.,1.,1.,1.,1.,1.,1.,1.,1.,1.,1.,1.,1.,1.,1.,1.,1.,1.,
1.,1.,1.,1.,1.,1.,1.,1.,1.,1.,1.,1.,1.,1.,1.,1.,1.,1.,1.,1.,1.))
REPRESENTATION_ITEM('')
);
#710=(
BOUNDED_CURVE()
B_SPLINE_CURVE(5,(#179037,#179038,#179039,#179040,#179041,#179042,#179043,
#179044,#179045,#179046,#179047,#179048,#179049,#179050,#179051,#179052,
#179053,#179054,#179055,#179056,#179057,#179058,#179059,#179060,#179061,
#179062,#179063,#179064,#179065,#179066,#179067,#179068,#179069,#179070,
#179071,#179072,#179073,#179074,#179075,#179076,#179077,#179078,#179079,
#179080,#179081,#179082,#179083,#179084,#179085,#179086,#179087,#179088,
#179089,#179090,#179091,#179092,#179093,#179094,#179095,#179096,#179097,
#179098,#179099,#179100,#179101,#179102,#179103,#179104,#179105,#179106,
#179107,#179108,#179109,#179110,#179111,#179112,#179113,#179114,#179115,
#179116,#179117,#179118,#179119,#179120,#179121,#179122,#179123,#179124,
#179125,#179126,#179127,#179128,#179129,#179130,#179131,#179132,#179133,
#179134,#179135,#179136,#179137,#179138,#179139,#179140,#179141,#179142,
#179143,#179144,#179145,#179146,#179147,#179148,#179149,#179150,#179151,
#179152,#179153,#179154,#179155,#179156,#179157,#179158,#179159,#179160,
#179161,#179162,#179163,#179164,#179165,#179166,#179167,#179168,#179169,
#179170,#179171,#179172,#179173,#179174,#179175,#179176,#179177,#179178,
#179179,#179180,#179181,#179182,#179183,#179184,#179185,#179186,#179187,
#179188,#179189,#179190,#179191,#179192,#179193,#179194,#179195,#179196,
#179197,#179198,#179199,#179200,#179201,#179202,#179203,#179204,#179205,
#179206,#179207,#179208,#179209,#179210,#179211,#179212,#179213,#179214,
#179215,#179216,#179217,#179218,#179219,#179220,#179221,#179222,#179223,
#179224,#179225,#179226,#179227,#179228,#179229,#179230,#179231,#179232,
#179233,#179234,#179235,#179236,#179237,#179238,#179239,#179240,#179241),
 .UNSPECIFIED.,.F.,.F.)
B_SPLINE_CURVE_WITH_KNOTS((6,1,1,1,1,1,1,1,1,1,1,1,1,1,1,1,1,1,1,1,1,1,
1,1,1,1,1,1,1,1,1,1,1,1,1,1,1,1,1,1,1,1,1,1,1,1,1,1,1,1,1,1,1,1,1,1,1,1,
1,1,1,1,1,1,1,1,1,1,1,1,1,1,1,1,1,1,1,1,1,1,1,1,1,1,1,1,1,1,1,1,1,1,1,1,
1,1,1,1,1,1,1,1,1,1,1,1,1,1,1,1,1,1,1,1,1,1,1,1,1,1,1,1,1,1,1,1,1,1,1,1,
1,1,1,1,1,1,1,1,1,1,1,1,1,1,1,1,1,1,1,1,1,1,1,1,1,1,1,1,1,1,1,1,1,1,1,1,
1,1,1,1,1,1,1,1,1,1,1,1,1,1,1,1,1,1,1,1,1,1,1,1,1,1,1,1,1,1,1,1,1,1,6),
(-1.,-0.995000000000001,-0.990000000000001,-0.985000000000001,-0.980000000000001,
-0.975000000000001,-0.970000000000001,-0.965000000000001,-0.960000000000001,
-0.955000000000001,-0.950000000000001,-0.945000000000001,-0.940000000000001,
-0.935000000000001,-0.930000000000001,-0.925000000000001,-0.920000000000001,
-0.915000000000001,-0.910000000000001,-0.905000000000001,-0.900000000000001,
-0.895000000000001,-0.890000000000001,-0.885000000000001,-0.880000000000001,
-0.875000000000001,-0.870000000000001,-0.865000000000001,-0.860000000000001,
-0.855000000000001,-0.850000000000001,-0.845000000000001,-0.840000000000001,
-0.835000000000001,-0.830000000000001,-0.825000000000001,-0.820000000000001,
-0.815000000000001,-0.810000000000001,-0.805000000000001,-0.800000000000001,
-0.795000000000001,-0.790000000000001,-0.785000000000001,-0.780000000000001,
-0.775000000000001,-0.770000000000001,-0.765000000000001,-0.760000000000001,
-0.755000000000001,-0.750000000000001,-0.745000000000001,-0.740000000000001,
-0.735000000000001,-0.730000000000001,-0.725000000000001,-0.720000000000001,
-0.715000000000001,-0.710000000000001,-0.705000000000001,-0.700000000000001,
-0.695000000000001,-0.690000000000001,-0.685,-0.68,-0.675,-0.67,-0.665,
-0.66,-0.655,-0.65,-0.645,-0.64,-0.635,-0.63,-0.625,-0.62,-0.615,-0.61,
-0.605,-0.6,-0.595,-0.59,-0.585,-0.58,-0.575,-0.57,-0.565,-0.56,-0.555,
-0.55,-0.545,-0.54,-0.535,-0.53,-0.525,-0.52,-0.515,-0.51,-0.505,-0.5,-0.495,
-0.49,-0.485,-0.48,-0.475,-0.47,-0.465,-0.46,-0.455,-0.45,-0.445,-0.44,
-0.435,-0.43,-0.425,-0.42,-0.415,-0.41,-0.405,-0.4,-0.395,-0.39,-0.385,
-0.38,-0.375,-0.37,-0.365,-0.36,-0.355,-0.35,-0.345,-0.34,-0.335,-0.33,
-0.325,-0.32,-0.315,-0.31,-0.305,-0.3,-0.295,-0.29,-0.285,-0.28,-0.275,
-0.27,-0.265,-0.26,-0.255,-0.25,-0.245,-0.24,-0.235,-0.23,-0.225,-0.22,
-0.215,-0.21,-0.205,-0.2,-0.195,-0.19,-0.185,-0.18,-0.175,-0.17,-0.165,
-0.16,-0.155,-0.15,-0.145,-0.14,-0.135,-0.13,-0.125,-0.12,-0.115,-0.11,
-0.105,-0.1,-0.095,-0.09,-0.085,-0.08,-0.075,-0.07,-0.065,-0.06,-0.055,
-0.05,-0.045,-0.04,-0.035,-0.03,-0.025,-0.02,-0.015,-0.01,-0.005,0.),
 .UNSPECIFIED.)
CURVE()
GEOMETRIC_REPRESENTATION_ITEM()
RATIONAL_B_SPLINE_CURVE((1.,1.,1.,1.,1.,1.,1.,1.,1.,1.,1.,1.,1.,1.,1.,1.,
1.,1.,1.,1.,1.,1.,1.,1.,1.,1.,1.,1.,1.,1.,1.,1.,1.,1.,1.,1.,1.,1.,1.,1.,
1.,1.,1.,1.,1.,1.,1.,1.,1.,1.,1.,1.,1.,1.,1.,1.,1.,1.,1.,1.,1.,1.,1.,1.,
1.,1.,1.,1.,1.,1.,1.,1.,1.,1.,1.,1.,1.,1.,1.,1.,1.,1.,1.,1.,1.,1.,1.,1.,
1.,1.,1.,1.,1.,1.,1.,1.,1.,1.,1.,1.,1.,1.,1.,1.,1.,1.,1.,1.,1.,1.,1.,1.,
1.,1.,1.,1.,1.,1.,1.,1.,1.,1.,1.,1.,1.,1.,1.,1.,1.,1.,1.,1.,1.,1.,1.,1.,
1.,1.,1.,1.,1.,1.,1.,1.,1.,1.,1.,1.,1.,1.,1.,1.,1.,1.,1.,1.,1.,1.,1.,1.,
1.,1.,1.,1.,1.,1.,1.,1.,1.,1.,1.,1.,1.,1.,1.,1.,1.,1.,1.,1.,1.,1.,1.,1.,
1.,1.,1.,1.,1.,1.,1.,1.,1.,1.,1.,1.,1.,1.,1.,1.,1.,1.,1.,1.,1.))
REPRESENTATION_ITEM('')
);
#711=(
BOUNDED_CURVE()
B_SPLINE_CURVE(5,(#179253,#179254,#179255,#179256,#179257,#179258,#179259,
#179260,#179261,#179262,#179263,#179264,#179265,#179266,#179267,#179268,
#179269,#179270,#179271,#179272,#179273,#179274,#179275,#179276,#179277,
#179278,#179279,#179280,#179281,#179282,#179283,#179284,#179285,#179286,
#179287,#179288,#179289,#179290,#179291,#179292,#179293,#179294,#179295,
#179296,#179297,#179298,#179299,#179300,#179301,#179302,#179303,#179304,
#179305,#179306,#179307,#179308,#179309,#179310,#179311,#179312,#179313,
#179314,#179315,#179316,#179317,#179318,#179319,#179320,#179321,#179322,
#179323,#179324,#179325,#179326,#179327,#179328,#179329,#179330,#179331,
#179332,#179333,#179334,#179335,#179336,#179337,#179338,#179339,#179340,
#179341,#179342,#179343,#179344,#179345,#179346,#179347,#179348,#179349,
#179350,#179351,#179352,#179353,#179354,#179355,#179356,#179357,#179358,
#179359,#179360,#179361,#179362,#179363,#179364,#179365,#179366,#179367,
#179368,#179369,#179370,#179371,#179372,#179373,#179374,#179375,#179376,
#179377,#179378,#179379,#179380,#179381,#179382,#179383,#179384,#179385,
#179386,#179387,#179388,#179389,#179390,#179391,#179392,#179393,#179394,
#179395,#179396,#179397,#179398,#179399,#179400,#179401,#179402,#179403,
#179404,#179405,#179406,#179407,#179408,#179409,#179410,#179411,#179412,
#179413,#179414,#179415,#179416,#179417,#179418,#179419,#179420,#179421,
#179422,#179423,#179424,#179425,#179426,#179427,#179428,#179429,#179430,
#179431,#179432,#179433,#179434,#179435,#179436,#179437,#179438,#179439,
#179440,#179441,#179442,#179443,#179444,#179445,#179446,#179447,#179448,
#179449,#179450,#179451,#179452,#179453,#179454,#179455,#179456,#179457),
 .UNSPECIFIED.,.F.,.F.)
B_SPLINE_CURVE_WITH_KNOTS((6,1,1,1,1,1,1,1,1,1,1,1,1,1,1,1,1,1,1,1,1,1,
1,1,1,1,1,1,1,1,1,1,1,1,1,1,1,1,1,1,1,1,1,1,1,1,1,1,1,1,1,1,1,1,1,1,1,1,
1,1,1,1,1,1,1,1,1,1,1,1,1,1,1,1,1,1,1,1,1,1,1,1,1,1,1,1,1,1,1,1,1,1,1,1,
1,1,1,1,1,1,1,1,1,1,1,1,1,1,1,1,1,1,1,1,1,1,1,1,1,1,1,1,1,1,1,1,1,1,1,1,
1,1,1,1,1,1,1,1,1,1,1,1,1,1,1,1,1,1,1,1,1,1,1,1,1,1,1,1,1,1,1,1,1,1,1,1,
1,1,1,1,1,1,1,1,1,1,1,1,1,1,1,1,1,1,1,1,1,1,1,1,1,1,1,1,1,1,1,1,1,1,6),
(0.,0.005,0.01,0.015,0.02,0.025,0.03,0.035,0.04,0.045,0.05,0.055,0.06,0.065,
0.07,0.075,0.08,0.085,0.09,0.095,0.1,0.105,0.11,0.115,0.12,0.125,0.13,0.135,
0.14,0.145,0.15,0.155,0.16,0.165,0.17,0.175,0.18,0.185,0.19,0.195,0.2,0.205,
0.21,0.215,0.22,0.225,0.23,0.235,0.24,0.245,0.25,0.255,0.26,0.265,0.27,
0.275,0.28,0.285,0.29,0.295,0.3,0.305,0.31,0.315,0.32,0.325,0.33,0.335,
0.34,0.345,0.35,0.355,0.36,0.365,0.37,0.375,0.38,0.385,0.39,0.395,0.4,0.405,
0.41,0.415,0.42,0.425,0.43,0.435,0.44,0.445,0.45,0.455,0.46,0.465,0.47,
0.475,0.48,0.485,0.49,0.495,0.5,0.505,0.51,0.515,0.52,0.525,0.53,0.535,
0.54,0.545,0.55,0.555,0.56,0.565,0.57,0.575,0.58,0.585,0.59,0.595,0.6,0.605,
0.61,0.615,0.62,0.625,0.63,0.635,0.64,0.645,0.65,0.655,0.66,0.665,0.67,
0.675,0.68,0.685,0.690000000000001,0.695000000000001,0.700000000000001,
0.705000000000001,0.710000000000001,0.715000000000001,0.720000000000001,
0.725000000000001,0.730000000000001,0.735000000000001,0.740000000000001,
0.745000000000001,0.750000000000001,0.755000000000001,0.760000000000001,
0.765000000000001,0.770000000000001,0.775000000000001,0.780000000000001,
0.785000000000001,0.790000000000001,0.795000000000001,0.800000000000001,
0.805000000000001,0.810000000000001,0.815000000000001,0.820000000000001,
0.825000000000001,0.830000000000001,0.835000000000001,0.840000000000001,
0.845000000000001,0.850000000000001,0.855000000000001,0.860000000000001,
0.865000000000001,0.870000000000001,0.875000000000001,0.880000000000001,
0.885000000000001,0.890000000000001,0.895000000000001,0.900000000000001,
0.905000000000001,0.910000000000001,0.915000000000001,0.920000000000001,
0.925000000000001,0.930000000000001,0.935000000000001,0.940000000000001,
0.945000000000001,0.950000000000001,0.955000000000001,0.960000000000001,
0.965000000000001,0.970000000000001,0.975000000000001,0.980000000000001,
0.985000000000001,0.990000000000001,0.995000000000001,1.),.UNSPECIFIED.)
CURVE()
GEOMETRIC_REPRESENTATION_ITEM()
RATIONAL_B_SPLINE_CURVE((1.,1.,1.,1.,1.,1.,1.,1.,1.,1.,1.,1.,1.,1.,1.,1.,
1.,1.,1.,1.,1.,1.,1.,1.,1.,1.,1.,1.,1.,1.,1.,1.,1.,1.,1.,1.,1.,1.,1.,1.,
1.,1.,1.,1.,1.,1.,1.,1.,1.,1.,1.,1.,1.,1.,1.,1.,1.,1.,1.,1.,1.,1.,1.,1.,
1.,1.,1.,1.,1.,1.,1.,1.,1.,1.,1.,1.,1.,1.,1.,1.,1.,1.,1.,1.,1.,1.,1.,1.,
1.,1.,1.,1.,1.,1.,1.,1.,1.,1.,1.,1.,1.,1.,1.,1.,1.,1.,1.,1.,1.,1.,1.,1.,
1.,1.,1.,1.,1.,1.,1.,1.,1.,1.,1.,1.,1.,1.,1.,1.,1.,1.,1.,1.,1.,1.,1.,1.,
1.,1.,1.,1.,1.,1.,1.,1.,1.,1.,1.,1.,1.,1.,1.,1.,1.,1.,1.,1.,1.,1.,1.,1.,
1.,1.,1.,1.,1.,1.,1.,1.,1.,1.,1.,1.,1.,1.,1.,1.,1.,1.,1.,1.,1.,1.,1.,1.,
1.,1.,1.,1.,1.,1.,1.,1.,1.,1.,1.,1.,1.,1.,1.,1.,1.,1.,1.,1.,1.))
REPRESENTATION_ITEM('')
);
#712=(
BOUNDED_CURVE()
B_SPLINE_CURVE(5,(#179461,#179462,#179463,#179464,#179465,#179466,#179467,
#179468,#179469,#179470,#179471,#179472,#179473,#179474,#179475,#179476,
#179477,#179478,#179479,#179480,#179481,#179482,#179483,#179484,#179485,
#179486,#179487,#179488,#179489,#179490,#179491,#179492,#179493,#179494,
#179495,#179496,#179497,#179498,#179499,#179500,#179501,#179502,#179503,
#179504,#179505,#179506,#179507,#179508,#179509,#179510,#179511,#179512,
#179513,#179514,#179515,#179516,#179517,#179518,#179519,#179520,#179521,
#179522,#179523,#179524,#179525,#179526,#179527,#179528,#179529,#179530,
#179531,#179532,#179533,#179534,#179535,#179536,#179537,#179538,#179539,
#179540,#179541,#179542,#179543,#179544,#179545,#179546,#179547,#179548,
#179549,#179550,#179551,#179552,#179553,#179554,#179555,#179556,#179557,
#179558,#179559,#179560,#179561,#179562,#179563,#179564,#179565,#179566,
#179567,#179568,#179569,#179570,#179571,#179572,#179573,#179574,#179575,
#179576,#179577,#179578,#179579,#179580,#179581,#179582,#179583,#179584,
#179585,#179586,#179587,#179588,#179589,#179590,#179591,#179592,#179593,
#179594,#179595,#179596,#179597,#179598,#179599,#179600,#179601,#179602,
#179603,#179604,#179605,#179606,#179607,#179608,#179609,#179610,#179611,
#179612,#179613,#179614,#179615,#179616,#179617,#179618,#179619,#179620,
#179621,#179622,#179623,#179624,#179625,#179626,#179627,#179628,#179629,
#179630,#179631,#179632,#179633,#179634,#179635,#179636,#179637,#179638,
#179639,#179640,#179641,#179642,#179643,#179644,#179645,#179646,#179647,
#179648,#179649,#179650,#179651,#179652,#179653,#179654,#179655,#179656,
#179657,#179658,#179659,#179660,#179661,#179662,#179663,#179664,#179665),
 .UNSPECIFIED.,.F.,.F.)
B_SPLINE_CURVE_WITH_KNOTS((6,1,1,1,1,1,1,1,1,1,1,1,1,1,1,1,1,1,1,1,1,1,
1,1,1,1,1,1,1,1,1,1,1,1,1,1,1,1,1,1,1,1,1,1,1,1,1,1,1,1,1,1,1,1,1,1,1,1,
1,1,1,1,1,1,1,1,1,1,1,1,1,1,1,1,1,1,1,1,1,1,1,1,1,1,1,1,1,1,1,1,1,1,1,1,
1,1,1,1,1,1,1,1,1,1,1,1,1,1,1,1,1,1,1,1,1,1,1,1,1,1,1,1,1,1,1,1,1,1,1,1,
1,1,1,1,1,1,1,1,1,1,1,1,1,1,1,1,1,1,1,1,1,1,1,1,1,1,1,1,1,1,1,1,1,1,1,1,
1,1,1,1,1,1,1,1,1,1,1,1,1,1,1,1,1,1,1,1,1,1,1,1,1,1,1,1,1,1,1,1,1,1,6),
(-1.,-0.995000000000001,-0.990000000000001,-0.985000000000001,-0.980000000000001,
-0.975000000000001,-0.970000000000001,-0.965000000000001,-0.960000000000001,
-0.955000000000001,-0.950000000000001,-0.945000000000001,-0.940000000000001,
-0.935000000000001,-0.930000000000001,-0.925000000000001,-0.920000000000001,
-0.915000000000001,-0.910000000000001,-0.905000000000001,-0.900000000000001,
-0.895000000000001,-0.890000000000001,-0.885000000000001,-0.880000000000001,
-0.875000000000001,-0.870000000000001,-0.865000000000001,-0.860000000000001,
-0.855000000000001,-0.850000000000001,-0.845000000000001,-0.840000000000001,
-0.835000000000001,-0.830000000000001,-0.825000000000001,-0.820000000000001,
-0.815000000000001,-0.810000000000001,-0.805000000000001,-0.800000000000001,
-0.795000000000001,-0.790000000000001,-0.785000000000001,-0.780000000000001,
-0.775000000000001,-0.770000000000001,-0.765000000000001,-0.760000000000001,
-0.755000000000001,-0.750000000000001,-0.745000000000001,-0.740000000000001,
-0.735000000000001,-0.730000000000001,-0.725000000000001,-0.720000000000001,
-0.715000000000001,-0.710000000000001,-0.705000000000001,-0.700000000000001,
-0.695000000000001,-0.690000000000001,-0.685,-0.68,-0.675,-0.67,-0.665,
-0.66,-0.655,-0.65,-0.645,-0.64,-0.635,-0.63,-0.625,-0.62,-0.615,-0.61,
-0.605,-0.6,-0.595,-0.59,-0.585,-0.58,-0.575,-0.57,-0.565,-0.56,-0.555,
-0.55,-0.545,-0.54,-0.535,-0.53,-0.525,-0.52,-0.515,-0.51,-0.505,-0.5,-0.495,
-0.49,-0.485,-0.48,-0.475,-0.47,-0.465,-0.46,-0.455,-0.45,-0.445,-0.44,
-0.435,-0.43,-0.425,-0.42,-0.415,-0.41,-0.405,-0.4,-0.395,-0.39,-0.385,
-0.38,-0.375,-0.37,-0.365,-0.36,-0.355,-0.35,-0.345,-0.34,-0.335,-0.33,
-0.325,-0.32,-0.315,-0.31,-0.305,-0.3,-0.295,-0.29,-0.285,-0.28,-0.275,
-0.27,-0.265,-0.26,-0.255,-0.25,-0.245,-0.24,-0.235,-0.23,-0.225,-0.22,
-0.215,-0.21,-0.205,-0.2,-0.195,-0.19,-0.185,-0.18,-0.175,-0.17,-0.165,
-0.16,-0.155,-0.15,-0.145,-0.14,-0.135,-0.13,-0.125,-0.12,-0.115,-0.11,
-0.105,-0.1,-0.095,-0.09,-0.085,-0.08,-0.075,-0.07,-0.065,-0.06,-0.055,
-0.05,-0.045,-0.04,-0.035,-0.03,-0.025,-0.02,-0.015,-0.01,-0.005,0.),
 .UNSPECIFIED.)
CURVE()
GEOMETRIC_REPRESENTATION_ITEM()
RATIONAL_B_SPLINE_CURVE((1.,1.,1.,1.,1.,1.,1.,1.,1.,1.,1.,1.,1.,1.,1.,1.,
1.,1.,1.,1.,1.,1.,1.,1.,1.,1.,1.,1.,1.,1.,1.,1.,1.,1.,1.,1.,1.,1.,1.,1.,
1.,1.,1.,1.,1.,1.,1.,1.,1.,1.,1.,1.,1.,1.,1.,1.,1.,1.,1.,1.,1.,1.,1.,1.,
1.,1.,1.,1.,1.,1.,1.,1.,1.,1.,1.,1.,1.,1.,1.,1.,1.,1.,1.,1.,1.,1.,1.,1.,
1.,1.,1.,1.,1.,1.,1.,1.,1.,1.,1.,1.,1.,1.,1.,1.,1.,1.,1.,1.,1.,1.,1.,1.,
1.,1.,1.,1.,1.,1.,1.,1.,1.,1.,1.,1.,1.,1.,1.,1.,1.,1.,1.,1.,1.,1.,1.,1.,
1.,1.,1.,1.,1.,1.,1.,1.,1.,1.,1.,1.,1.,1.,1.,1.,1.,1.,1.,1.,1.,1.,1.,1.,
1.,1.,1.,1.,1.,1.,1.,1.,1.,1.,1.,1.,1.,1.,1.,1.,1.,1.,1.,1.,1.,1.,1.,1.,
1.,1.,1.,1.,1.,1.,1.,1.,1.,1.,1.,1.,1.,1.,1.,1.,1.,1.,1.,1.,1.))
REPRESENTATION_ITEM('')
);
#713=(
BOUNDED_CURVE()
B_SPLINE_CURVE(5,(#179677,#179678,#179679,#179680,#179681,#179682,#179683,
#179684,#179685,#179686,#179687,#179688,#179689,#179690,#179691,#179692,
#179693,#179694,#179695,#179696,#179697,#179698,#179699,#179700,#179701,
#179702,#179703,#179704,#179705,#179706,#179707,#179708,#179709,#179710,
#179711,#179712,#179713,#179714,#179715,#179716,#179717,#179718,#179719,
#179720,#179721,#179722,#179723,#179724,#179725,#179726,#179727,#179728,
#179729,#179730,#179731,#179732,#179733,#179734,#179735,#179736,#179737,
#179738,#179739,#179740,#179741,#179742,#179743,#179744,#179745,#179746,
#179747,#179748,#179749,#179750,#179751,#179752,#179753,#179754,#179755,
#179756,#179757,#179758,#179759,#179760,#179761,#179762,#179763,#179764,
#179765,#179766,#179767,#179768,#179769,#179770,#179771,#179772,#179773,
#179774,#179775,#179776,#179777,#179778,#179779,#179780,#179781,#179782,
#179783,#179784,#179785,#179786,#179787,#179788,#179789,#179790,#179791,
#179792,#179793,#179794,#179795,#179796,#179797,#179798,#179799,#179800,
#179801,#179802,#179803,#179804,#179805,#179806,#179807,#179808,#179809,
#179810,#179811,#179812,#179813,#179814,#179815,#179816,#179817,#179818,
#179819,#179820,#179821,#179822,#179823,#179824,#179825,#179826,#179827,
#179828,#179829,#179830,#179831,#179832,#179833,#179834,#179835,#179836,
#179837,#179838,#179839,#179840,#179841,#179842,#179843,#179844,#179845,
#179846,#179847,#179848,#179849,#179850,#179851,#179852,#179853,#179854,
#179855,#179856,#179857,#179858,#179859,#179860,#179861,#179862,#179863,
#179864,#179865,#179866,#179867,#179868,#179869,#179870,#179871,#179872,
#179873,#179874,#179875,#179876,#179877,#179878,#179879,#179880,#179881),
 .UNSPECIFIED.,.F.,.F.)
B_SPLINE_CURVE_WITH_KNOTS((6,1,1,1,1,1,1,1,1,1,1,1,1,1,1,1,1,1,1,1,1,1,
1,1,1,1,1,1,1,1,1,1,1,1,1,1,1,1,1,1,1,1,1,1,1,1,1,1,1,1,1,1,1,1,1,1,1,1,
1,1,1,1,1,1,1,1,1,1,1,1,1,1,1,1,1,1,1,1,1,1,1,1,1,1,1,1,1,1,1,1,1,1,1,1,
1,1,1,1,1,1,1,1,1,1,1,1,1,1,1,1,1,1,1,1,1,1,1,1,1,1,1,1,1,1,1,1,1,1,1,1,
1,1,1,1,1,1,1,1,1,1,1,1,1,1,1,1,1,1,1,1,1,1,1,1,1,1,1,1,1,1,1,1,1,1,1,1,
1,1,1,1,1,1,1,1,1,1,1,1,1,1,1,1,1,1,1,1,1,1,1,1,1,1,1,1,1,1,1,1,1,1,6),
(0.,0.005,0.01,0.015,0.02,0.025,0.03,0.035,0.04,0.045,0.05,0.055,0.06,0.065,
0.07,0.075,0.08,0.085,0.09,0.095,0.1,0.105,0.11,0.115,0.12,0.125,0.13,0.135,
0.14,0.145,0.15,0.155,0.16,0.165,0.17,0.175,0.18,0.185,0.19,0.195,0.2,0.205,
0.21,0.215,0.22,0.225,0.23,0.235,0.24,0.245,0.25,0.255,0.26,0.265,0.27,
0.275,0.28,0.285,0.29,0.295,0.3,0.305,0.31,0.315,0.32,0.325,0.33,0.335,
0.34,0.345,0.35,0.355,0.36,0.365,0.37,0.375,0.38,0.385,0.39,0.395,0.4,0.405,
0.41,0.415,0.42,0.425,0.43,0.435,0.44,0.445,0.45,0.455,0.46,0.465,0.47,
0.475,0.48,0.485,0.49,0.495,0.5,0.505,0.51,0.515,0.52,0.525,0.53,0.535,
0.54,0.545,0.55,0.555,0.56,0.565,0.57,0.575,0.58,0.585,0.59,0.595,0.6,0.605,
0.61,0.615,0.62,0.625,0.63,0.635,0.64,0.645,0.65,0.655,0.66,0.665,0.67,
0.675,0.68,0.685,0.690000000000001,0.695000000000001,0.700000000000001,
0.705000000000001,0.710000000000001,0.715000000000001,0.720000000000001,
0.725000000000001,0.730000000000001,0.735000000000001,0.740000000000001,
0.745000000000001,0.750000000000001,0.755000000000001,0.760000000000001,
0.765000000000001,0.770000000000001,0.775000000000001,0.780000000000001,
0.785000000000001,0.790000000000001,0.795000000000001,0.800000000000001,
0.805000000000001,0.810000000000001,0.815000000000001,0.820000000000001,
0.825000000000001,0.830000000000001,0.835000000000001,0.840000000000001,
0.845000000000001,0.850000000000001,0.855000000000001,0.860000000000001,
0.865000000000001,0.870000000000001,0.875000000000001,0.880000000000001,
0.885000000000001,0.890000000000001,0.895000000000001,0.900000000000001,
0.905000000000001,0.910000000000001,0.915000000000001,0.920000000000001,
0.925000000000001,0.930000000000001,0.935000000000001,0.940000000000001,
0.945000000000001,0.950000000000001,0.955000000000001,0.960000000000001,
0.965000000000001,0.970000000000001,0.975000000000001,0.980000000000001,
0.985000000000001,0.990000000000001,0.995000000000001,1.),.UNSPECIFIED.)
CURVE()
GEOMETRIC_REPRESENTATION_ITEM()
RATIONAL_B_SPLINE_CURVE((1.,1.,1.,1.,1.,1.,1.,1.,1.,1.,1.,1.,1.,1.,1.,1.,
1.,1.,1.,1.,1.,1.,1.,1.,1.,1.,1.,1.,1.,1.,1.,1.,1.,1.,1.,1.,1.,1.,1.,1.,
1.,1.,1.,1.,1.,1.,1.,1.,1.,1.,1.,1.,1.,1.,1.,1.,1.,1.,1.,1.,1.,1.,1.,1.,
1.,1.,1.,1.,1.,1.,1.,1.,1.,1.,1.,1.,1.,1.,1.,1.,1.,1.,1.,1.,1.,1.,1.,1.,
1.,1.,1.,1.,1.,1.,1.,1.,1.,1.,1.,1.,1.,1.,1.,1.,1.,1.,1.,1.,1.,1.,1.,1.,
1.,1.,1.,1.,1.,1.,1.,1.,1.,1.,1.,1.,1.,1.,1.,1.,1.,1.,1.,1.,1.,1.,1.,1.,
1.,1.,1.,1.,1.,1.,1.,1.,1.,1.,1.,1.,1.,1.,1.,1.,1.,1.,1.,1.,1.,1.,1.,1.,
1.,1.,1.,1.,1.,1.,1.,1.,1.,1.,1.,1.,1.,1.,1.,1.,1.,1.,1.,1.,1.,1.,1.,1.,
1.,1.,1.,1.,1.,1.,1.,1.,1.,1.,1.,1.,1.,1.,1.,1.,1.,1.,1.,1.,1.))
REPRESENTATION_ITEM('')
);
#714=(
BOUNDED_CURVE()
B_SPLINE_CURVE(5,(#179885,#179886,#179887,#179888,#179889,#179890,#179891,
#179892,#179893,#179894,#179895,#179896,#179897,#179898,#179899,#179900,
#179901,#179902,#179903,#179904,#179905,#179906,#179907,#179908,#179909,
#179910,#179911,#179912,#179913,#179914,#179915,#179916,#179917,#179918,
#179919,#179920,#179921,#179922,#179923,#179924,#179925,#179926,#179927,
#179928,#179929,#179930,#179931,#179932,#179933,#179934,#179935,#179936,
#179937,#179938,#179939,#179940,#179941,#179942,#179943,#179944,#179945,
#179946,#179947,#179948,#179949,#179950,#179951,#179952,#179953,#179954,
#179955,#179956,#179957,#179958,#179959,#179960,#179961,#179962,#179963,
#179964,#179965,#179966,#179967,#179968,#179969,#179970,#179971,#179972,
#179973,#179974,#179975,#179976,#179977,#179978,#179979,#179980,#179981,
#179982,#179983,#179984,#179985,#179986,#179987,#179988,#179989,#179990,
#179991,#179992,#179993,#179994,#179995,#179996,#179997,#179998,#179999,
#180000,#180001,#180002,#180003,#180004,#180005,#180006,#180007,#180008,
#180009,#180010,#180011,#180012,#180013,#180014,#180015,#180016,#180017,
#180018,#180019,#180020,#180021,#180022,#180023,#180024,#180025,#180026,
#180027,#180028,#180029,#180030,#180031,#180032,#180033,#180034,#180035,
#180036,#180037,#180038,#180039,#180040,#180041,#180042,#180043,#180044,
#180045,#180046,#180047,#180048,#180049,#180050,#180051,#180052,#180053,
#180054,#180055,#180056,#180057,#180058,#180059,#180060,#180061,#180062,
#180063,#180064,#180065,#180066,#180067,#180068,#180069,#180070,#180071,
#180072,#180073,#180074,#180075,#180076,#180077,#180078,#180079,#180080,
#180081,#180082,#180083,#180084,#180085,#180086,#180087,#180088,#180089),
 .UNSPECIFIED.,.F.,.F.)
B_SPLINE_CURVE_WITH_KNOTS((6,1,1,1,1,1,1,1,1,1,1,1,1,1,1,1,1,1,1,1,1,1,
1,1,1,1,1,1,1,1,1,1,1,1,1,1,1,1,1,1,1,1,1,1,1,1,1,1,1,1,1,1,1,1,1,1,1,1,
1,1,1,1,1,1,1,1,1,1,1,1,1,1,1,1,1,1,1,1,1,1,1,1,1,1,1,1,1,1,1,1,1,1,1,1,
1,1,1,1,1,1,1,1,1,1,1,1,1,1,1,1,1,1,1,1,1,1,1,1,1,1,1,1,1,1,1,1,1,1,1,1,
1,1,1,1,1,1,1,1,1,1,1,1,1,1,1,1,1,1,1,1,1,1,1,1,1,1,1,1,1,1,1,1,1,1,1,1,
1,1,1,1,1,1,1,1,1,1,1,1,1,1,1,1,1,1,1,1,1,1,1,1,1,1,1,1,1,1,1,1,1,1,6),
(-1.,-0.995000000000001,-0.990000000000001,-0.985000000000001,-0.980000000000001,
-0.975000000000001,-0.970000000000001,-0.965000000000001,-0.960000000000001,
-0.955000000000001,-0.950000000000001,-0.945000000000001,-0.940000000000001,
-0.935000000000001,-0.930000000000001,-0.925000000000001,-0.920000000000001,
-0.915000000000001,-0.910000000000001,-0.905000000000001,-0.900000000000001,
-0.895000000000001,-0.890000000000001,-0.885000000000001,-0.880000000000001,
-0.875000000000001,-0.870000000000001,-0.865000000000001,-0.860000000000001,
-0.855000000000001,-0.850000000000001,-0.845000000000001,-0.840000000000001,
-0.835000000000001,-0.830000000000001,-0.825000000000001,-0.820000000000001,
-0.815000000000001,-0.810000000000001,-0.805000000000001,-0.800000000000001,
-0.795000000000001,-0.790000000000001,-0.785000000000001,-0.780000000000001,
-0.775000000000001,-0.770000000000001,-0.765000000000001,-0.760000000000001,
-0.755000000000001,-0.750000000000001,-0.745000000000001,-0.740000000000001,
-0.735000000000001,-0.730000000000001,-0.725000000000001,-0.720000000000001,
-0.715000000000001,-0.710000000000001,-0.705000000000001,-0.700000000000001,
-0.695000000000001,-0.690000000000001,-0.685,-0.68,-0.675,-0.67,-0.665,
-0.66,-0.655,-0.65,-0.645,-0.64,-0.635,-0.63,-0.625,-0.62,-0.615,-0.61,
-0.605,-0.6,-0.595,-0.59,-0.585,-0.58,-0.575,-0.57,-0.565,-0.56,-0.555,
-0.55,-0.545,-0.54,-0.535,-0.53,-0.525,-0.52,-0.515,-0.51,-0.505,-0.5,-0.495,
-0.49,-0.485,-0.48,-0.475,-0.47,-0.465,-0.46,-0.455,-0.45,-0.445,-0.44,
-0.435,-0.43,-0.425,-0.42,-0.415,-0.41,-0.405,-0.4,-0.395,-0.39,-0.385,
-0.38,-0.375,-0.37,-0.365,-0.36,-0.355,-0.35,-0.345,-0.34,-0.335,-0.33,
-0.325,-0.32,-0.315,-0.31,-0.305,-0.3,-0.295,-0.29,-0.285,-0.28,-0.275,
-0.27,-0.265,-0.26,-0.255,-0.25,-0.245,-0.24,-0.235,-0.23,-0.225,-0.22,
-0.215,-0.21,-0.205,-0.2,-0.195,-0.19,-0.185,-0.18,-0.175,-0.17,-0.165,
-0.16,-0.155,-0.15,-0.145,-0.14,-0.135,-0.13,-0.125,-0.12,-0.115,-0.11,
-0.105,-0.1,-0.095,-0.09,-0.085,-0.08,-0.075,-0.07,-0.065,-0.06,-0.055,
-0.05,-0.045,-0.04,-0.035,-0.03,-0.025,-0.02,-0.015,-0.01,-0.005,0.),
 .UNSPECIFIED.)
CURVE()
GEOMETRIC_REPRESENTATION_ITEM()
RATIONAL_B_SPLINE_CURVE((1.,1.,1.,1.,1.,1.,1.,1.,1.,1.,1.,1.,1.,1.,1.,1.,
1.,1.,1.,1.,1.,1.,1.,1.,1.,1.,1.,1.,1.,1.,1.,1.,1.,1.,1.,1.,1.,1.,1.,1.,
1.,1.,1.,1.,1.,1.,1.,1.,1.,1.,1.,1.,1.,1.,1.,1.,1.,1.,1.,1.,1.,1.,1.,1.,
1.,1.,1.,1.,1.,1.,1.,1.,1.,1.,1.,1.,1.,1.,1.,1.,1.,1.,1.,1.,1.,1.,1.,1.,
1.,1.,1.,1.,1.,1.,1.,1.,1.,1.,1.,1.,1.,1.,1.,1.,1.,1.,1.,1.,1.,1.,1.,1.,
1.,1.,1.,1.,1.,1.,1.,1.,1.,1.,1.,1.,1.,1.,1.,1.,1.,1.,1.,1.,1.,1.,1.,1.,
1.,1.,1.,1.,1.,1.,1.,1.,1.,1.,1.,1.,1.,1.,1.,1.,1.,1.,1.,1.,1.,1.,1.,1.,
1.,1.,1.,1.,1.,1.,1.,1.,1.,1.,1.,1.,1.,1.,1.,1.,1.,1.,1.,1.,1.,1.,1.,1.,
1.,1.,1.,1.,1.,1.,1.,1.,1.,1.,1.,1.,1.,1.,1.,1.,1.,1.,1.,1.,1.))
REPRESENTATION_ITEM('')
);
#715=(
BOUNDED_CURVE()
B_SPLINE_CURVE(5,(#180101,#180102,#180103,#180104,#180105,#180106,#180107,
#180108,#180109,#180110,#180111,#180112,#180113,#180114,#180115,#180116,
#180117,#180118,#180119,#180120,#180121,#180122,#180123,#180124,#180125,
#180126,#180127,#180128,#180129,#180130,#180131,#180132,#180133,#180134,
#180135,#180136,#180137,#180138,#180139,#180140,#180141,#180142,#180143,
#180144,#180145,#180146,#180147,#180148,#180149,#180150,#180151,#180152,
#180153,#180154,#180155,#180156,#180157,#180158,#180159,#180160,#180161,
#180162,#180163,#180164,#180165,#180166,#180167,#180168,#180169,#180170,
#180171,#180172,#180173,#180174,#180175,#180176,#180177,#180178,#180179,
#180180,#180181,#180182,#180183,#180184,#180185,#180186,#180187,#180188,
#180189,#180190,#180191,#180192,#180193,#180194,#180195,#180196,#180197,
#180198,#180199,#180200,#180201,#180202,#180203,#180204,#180205,#180206,
#180207,#180208,#180209,#180210,#180211,#180212,#180213,#180214,#180215,
#180216,#180217,#180218,#180219,#180220,#180221,#180222,#180223,#180224,
#180225,#180226,#180227,#180228,#180229,#180230,#180231,#180232,#180233,
#180234,#180235,#180236,#180237,#180238,#180239,#180240,#180241,#180242,
#180243,#180244,#180245,#180246,#180247,#180248,#180249,#180250,#180251,
#180252,#180253,#180254,#180255,#180256,#180257,#180258,#180259,#180260,
#180261,#180262,#180263,#180264,#180265,#180266,#180267,#180268,#180269,
#180270,#180271,#180272,#180273,#180274,#180275,#180276,#180277,#180278,
#180279,#180280,#180281,#180282,#180283,#180284,#180285,#180286,#180287,
#180288,#180289,#180290,#180291,#180292,#180293,#180294,#180295,#180296,
#180297,#180298,#180299,#180300,#180301,#180302,#180303,#180304,#180305),
 .UNSPECIFIED.,.F.,.F.)
B_SPLINE_CURVE_WITH_KNOTS((6,1,1,1,1,1,1,1,1,1,1,1,1,1,1,1,1,1,1,1,1,1,
1,1,1,1,1,1,1,1,1,1,1,1,1,1,1,1,1,1,1,1,1,1,1,1,1,1,1,1,1,1,1,1,1,1,1,1,
1,1,1,1,1,1,1,1,1,1,1,1,1,1,1,1,1,1,1,1,1,1,1,1,1,1,1,1,1,1,1,1,1,1,1,1,
1,1,1,1,1,1,1,1,1,1,1,1,1,1,1,1,1,1,1,1,1,1,1,1,1,1,1,1,1,1,1,1,1,1,1,1,
1,1,1,1,1,1,1,1,1,1,1,1,1,1,1,1,1,1,1,1,1,1,1,1,1,1,1,1,1,1,1,1,1,1,1,1,
1,1,1,1,1,1,1,1,1,1,1,1,1,1,1,1,1,1,1,1,1,1,1,1,1,1,1,1,1,1,1,1,1,1,6),
(0.,0.005,0.01,0.015,0.02,0.025,0.03,0.035,0.04,0.045,0.05,0.055,0.06,0.065,
0.07,0.075,0.08,0.085,0.09,0.095,0.1,0.105,0.11,0.115,0.12,0.125,0.13,0.135,
0.14,0.145,0.15,0.155,0.16,0.165,0.17,0.175,0.18,0.185,0.19,0.195,0.2,0.205,
0.21,0.215,0.22,0.225,0.23,0.235,0.24,0.245,0.25,0.255,0.26,0.265,0.27,
0.275,0.28,0.285,0.29,0.295,0.3,0.305,0.31,0.315,0.32,0.325,0.33,0.335,
0.34,0.345,0.35,0.355,0.36,0.365,0.37,0.375,0.38,0.385,0.39,0.395,0.4,0.405,
0.41,0.415,0.42,0.425,0.43,0.435,0.44,0.445,0.45,0.455,0.46,0.465,0.47,
0.475,0.48,0.485,0.49,0.495,0.5,0.505,0.51,0.515,0.52,0.525,0.53,0.535,
0.54,0.545,0.55,0.555,0.56,0.565,0.57,0.575,0.58,0.585,0.59,0.595,0.6,0.605,
0.61,0.615,0.62,0.625,0.63,0.635,0.64,0.645,0.65,0.655,0.66,0.665,0.67,
0.675,0.68,0.685,0.690000000000001,0.695000000000001,0.700000000000001,
0.705000000000001,0.710000000000001,0.715000000000001,0.720000000000001,
0.725000000000001,0.730000000000001,0.735000000000001,0.740000000000001,
0.745000000000001,0.750000000000001,0.755000000000001,0.760000000000001,
0.765000000000001,0.770000000000001,0.775000000000001,0.780000000000001,
0.785000000000001,0.790000000000001,0.795000000000001,0.800000000000001,
0.805000000000001,0.810000000000001,0.815000000000001,0.820000000000001,
0.825000000000001,0.830000000000001,0.835000000000001,0.840000000000001,
0.845000000000001,0.850000000000001,0.855000000000001,0.860000000000001,
0.865000000000001,0.870000000000001,0.875000000000001,0.880000000000001,
0.885000000000001,0.890000000000001,0.895000000000001,0.900000000000001,
0.905000000000001,0.910000000000001,0.915000000000001,0.920000000000001,
0.925000000000001,0.930000000000001,0.935000000000001,0.940000000000001,
0.945000000000001,0.950000000000001,0.955000000000001,0.960000000000001,
0.965000000000001,0.970000000000001,0.975000000000001,0.980000000000001,
0.985000000000001,0.990000000000001,0.995000000000001,1.),.UNSPECIFIED.)
CURVE()
GEOMETRIC_REPRESENTATION_ITEM()
RATIONAL_B_SPLINE_CURVE((1.,1.,1.,1.,1.,1.,1.,1.,1.,1.,1.,1.,1.,1.,1.,1.,
1.,1.,1.,1.,1.,1.,1.,1.,1.,1.,1.,1.,1.,1.,1.,1.,1.,1.,1.,1.,1.,1.,1.,1.,
1.,1.,1.,1.,1.,1.,1.,1.,1.,1.,1.,1.,1.,1.,1.,1.,1.,1.,1.,1.,1.,1.,1.,1.,
1.,1.,1.,1.,1.,1.,1.,1.,1.,1.,1.,1.,1.,1.,1.,1.,1.,1.,1.,1.,1.,1.,1.,1.,
1.,1.,1.,1.,1.,1.,1.,1.,1.,1.,1.,1.,1.,1.,1.,1.,1.,1.,1.,1.,1.,1.,1.,1.,
1.,1.,1.,1.,1.,1.,1.,1.,1.,1.,1.,1.,1.,1.,1.,1.,1.,1.,1.,1.,1.,1.,1.,1.,
1.,1.,1.,1.,1.,1.,1.,1.,1.,1.,1.,1.,1.,1.,1.,1.,1.,1.,1.,1.,1.,1.,1.,1.,
1.,1.,1.,1.,1.,1.,1.,1.,1.,1.,1.,1.,1.,1.,1.,1.,1.,1.,1.,1.,1.,1.,1.,1.,
1.,1.,1.,1.,1.,1.,1.,1.,1.,1.,1.,1.,1.,1.,1.,1.,1.,1.,1.,1.,1.))
REPRESENTATION_ITEM('')
);
#716=(
BOUNDED_CURVE()
B_SPLINE_CURVE(5,(#180309,#180310,#180311,#180312,#180313,#180314,#180315,
#180316,#180317,#180318,#180319,#180320,#180321,#180322,#180323,#180324,
#180325,#180326,#180327,#180328,#180329,#180330,#180331,#180332,#180333,
#180334,#180335,#180336,#180337,#180338,#180339,#180340,#180341,#180342,
#180343,#180344,#180345,#180346,#180347,#180348,#180349,#180350,#180351,
#180352,#180353,#180354,#180355,#180356,#180357,#180358,#180359,#180360,
#180361,#180362,#180363,#180364,#180365,#180366,#180367,#180368,#180369,
#180370,#180371,#180372,#180373,#180374,#180375,#180376,#180377,#180378,
#180379,#180380,#180381,#180382,#180383,#180384,#180385,#180386,#180387,
#180388,#180389,#180390,#180391,#180392,#180393,#180394,#180395,#180396,
#180397,#180398,#180399,#180400,#180401,#180402,#180403,#180404,#180405,
#180406,#180407,#180408,#180409,#180410,#180411,#180412,#180413,#180414,
#180415,#180416,#180417,#180418,#180419,#180420,#180421,#180422,#180423,
#180424,#180425,#180426,#180427,#180428,#180429,#180430,#180431,#180432,
#180433,#180434,#180435,#180436,#180437,#180438,#180439,#180440,#180441,
#180442,#180443,#180444,#180445,#180446,#180447,#180448,#180449,#180450,
#180451,#180452,#180453,#180454,#180455,#180456,#180457,#180458,#180459,
#180460,#180461,#180462,#180463,#180464,#180465,#180466,#180467,#180468,
#180469,#180470,#180471,#180472,#180473,#180474,#180475,#180476,#180477,
#180478,#180479,#180480,#180481,#180482,#180483,#180484,#180485,#180486,
#180487,#180488,#180489,#180490,#180491,#180492,#180493,#180494,#180495,
#180496,#180497,#180498,#180499,#180500,#180501,#180502,#180503,#180504,
#180505,#180506,#180507,#180508,#180509,#180510,#180511,#180512,#180513),
 .UNSPECIFIED.,.F.,.F.)
B_SPLINE_CURVE_WITH_KNOTS((6,1,1,1,1,1,1,1,1,1,1,1,1,1,1,1,1,1,1,1,1,1,
1,1,1,1,1,1,1,1,1,1,1,1,1,1,1,1,1,1,1,1,1,1,1,1,1,1,1,1,1,1,1,1,1,1,1,1,
1,1,1,1,1,1,1,1,1,1,1,1,1,1,1,1,1,1,1,1,1,1,1,1,1,1,1,1,1,1,1,1,1,1,1,1,
1,1,1,1,1,1,1,1,1,1,1,1,1,1,1,1,1,1,1,1,1,1,1,1,1,1,1,1,1,1,1,1,1,1,1,1,
1,1,1,1,1,1,1,1,1,1,1,1,1,1,1,1,1,1,1,1,1,1,1,1,1,1,1,1,1,1,1,1,1,1,1,1,
1,1,1,1,1,1,1,1,1,1,1,1,1,1,1,1,1,1,1,1,1,1,1,1,1,1,1,1,1,1,1,1,1,1,6),
(-1.,-0.995000000000001,-0.990000000000001,-0.985000000000001,-0.980000000000001,
-0.975000000000001,-0.970000000000001,-0.965000000000001,-0.960000000000001,
-0.955000000000001,-0.950000000000001,-0.945000000000001,-0.940000000000001,
-0.935000000000001,-0.930000000000001,-0.925000000000001,-0.920000000000001,
-0.915000000000001,-0.910000000000001,-0.905000000000001,-0.900000000000001,
-0.895000000000001,-0.890000000000001,-0.885000000000001,-0.880000000000001,
-0.875000000000001,-0.870000000000001,-0.865000000000001,-0.860000000000001,
-0.855000000000001,-0.850000000000001,-0.845000000000001,-0.840000000000001,
-0.835000000000001,-0.830000000000001,-0.825000000000001,-0.820000000000001,
-0.815000000000001,-0.810000000000001,-0.805000000000001,-0.800000000000001,
-0.795000000000001,-0.790000000000001,-0.785000000000001,-0.780000000000001,
-0.775000000000001,-0.770000000000001,-0.765000000000001,-0.760000000000001,
-0.755000000000001,-0.750000000000001,-0.745000000000001,-0.740000000000001,
-0.735000000000001,-0.730000000000001,-0.725000000000001,-0.720000000000001,
-0.715000000000001,-0.710000000000001,-0.705000000000001,-0.700000000000001,
-0.695000000000001,-0.690000000000001,-0.685,-0.68,-0.675,-0.67,-0.665,
-0.66,-0.655,-0.65,-0.645,-0.64,-0.635,-0.63,-0.625,-0.62,-0.615,-0.61,
-0.605,-0.6,-0.595,-0.59,-0.585,-0.58,-0.575,-0.57,-0.565,-0.56,-0.555,
-0.55,-0.545,-0.54,-0.535,-0.53,-0.525,-0.52,-0.515,-0.51,-0.505,-0.5,-0.495,
-0.49,-0.485,-0.48,-0.475,-0.47,-0.465,-0.46,-0.455,-0.45,-0.445,-0.44,
-0.435,-0.43,-0.425,-0.42,-0.415,-0.41,-0.405,-0.4,-0.395,-0.39,-0.385,
-0.38,-0.375,-0.37,-0.365,-0.36,-0.355,-0.35,-0.345,-0.34,-0.335,-0.33,
-0.325,-0.32,-0.315,-0.31,-0.305,-0.3,-0.295,-0.29,-0.285,-0.28,-0.275,
-0.27,-0.265,-0.26,-0.255,-0.25,-0.245,-0.24,-0.235,-0.23,-0.225,-0.22,
-0.215,-0.21,-0.205,-0.2,-0.195,-0.19,-0.185,-0.18,-0.175,-0.17,-0.165,
-0.16,-0.155,-0.15,-0.145,-0.14,-0.135,-0.13,-0.125,-0.12,-0.115,-0.11,
-0.105,-0.1,-0.095,-0.09,-0.085,-0.08,-0.075,-0.07,-0.065,-0.06,-0.055,
-0.05,-0.045,-0.04,-0.035,-0.03,-0.025,-0.02,-0.015,-0.01,-0.005,0.),
 .UNSPECIFIED.)
CURVE()
GEOMETRIC_REPRESENTATION_ITEM()
RATIONAL_B_SPLINE_CURVE((1.,1.,1.,1.,1.,1.,1.,1.,1.,1.,1.,1.,1.,1.,1.,1.,
1.,1.,1.,1.,1.,1.,1.,1.,1.,1.,1.,1.,1.,1.,1.,1.,1.,1.,1.,1.,1.,1.,1.,1.,
1.,1.,1.,1.,1.,1.,1.,1.,1.,1.,1.,1.,1.,1.,1.,1.,1.,1.,1.,1.,1.,1.,1.,1.,
1.,1.,1.,1.,1.,1.,1.,1.,1.,1.,1.,1.,1.,1.,1.,1.,1.,1.,1.,1.,1.,1.,1.,1.,
1.,1.,1.,1.,1.,1.,1.,1.,1.,1.,1.,1.,1.,1.,1.,1.,1.,1.,1.,1.,1.,1.,1.,1.,
1.,1.,1.,1.,1.,1.,1.,1.,1.,1.,1.,1.,1.,1.,1.,1.,1.,1.,1.,1.,1.,1.,1.,1.,
1.,1.,1.,1.,1.,1.,1.,1.,1.,1.,1.,1.,1.,1.,1.,1.,1.,1.,1.,1.,1.,1.,1.,1.,
1.,1.,1.,1.,1.,1.,1.,1.,1.,1.,1.,1.,1.,1.,1.,1.,1.,1.,1.,1.,1.,1.,1.,1.,
1.,1.,1.,1.,1.,1.,1.,1.,1.,1.,1.,1.,1.,1.,1.,1.,1.,1.,1.,1.,1.))
REPRESENTATION_ITEM('')
);
#717=(
BOUNDED_CURVE()
B_SPLINE_CURVE(5,(#180525,#180526,#180527,#180528,#180529,#180530,#180531,
#180532,#180533,#180534,#180535,#180536,#180537,#180538,#180539,#180540,
#180541,#180542,#180543,#180544,#180545,#180546,#180547,#180548,#180549,
#180550,#180551,#180552,#180553,#180554,#180555,#180556,#180557,#180558,
#180559,#180560,#180561,#180562,#180563,#180564,#180565,#180566,#180567,
#180568,#180569,#180570,#180571,#180572,#180573,#180574,#180575,#180576,
#180577,#180578,#180579,#180580,#180581,#180582,#180583,#180584,#180585,
#180586,#180587,#180588,#180589,#180590,#180591,#180592,#180593,#180594,
#180595,#180596,#180597,#180598,#180599,#180600,#180601,#180602,#180603,
#180604,#180605,#180606,#180607,#180608,#180609,#180610,#180611,#180612,
#180613,#180614,#180615,#180616,#180617,#180618,#180619,#180620,#180621,
#180622,#180623,#180624,#180625,#180626,#180627,#180628,#180629,#180630,
#180631,#180632,#180633,#180634,#180635,#180636,#180637,#180638,#180639,
#180640,#180641,#180642,#180643,#180644,#180645,#180646,#180647,#180648,
#180649,#180650,#180651,#180652,#180653,#180654,#180655,#180656,#180657,
#180658,#180659,#180660,#180661,#180662,#180663,#180664,#180665,#180666,
#180667,#180668,#180669,#180670,#180671,#180672,#180673,#180674,#180675,
#180676,#180677,#180678,#180679,#180680,#180681,#180682,#180683,#180684,
#180685,#180686,#180687,#180688,#180689,#180690,#180691,#180692,#180693,
#180694,#180695,#180696,#180697,#180698,#180699,#180700,#180701,#180702,
#180703,#180704,#180705,#180706,#180707,#180708,#180709,#180710,#180711,
#180712,#180713,#180714,#180715,#180716,#180717,#180718,#180719,#180720,
#180721,#180722,#180723,#180724,#180725,#180726,#180727,#180728,#180729),
 .UNSPECIFIED.,.F.,.F.)
B_SPLINE_CURVE_WITH_KNOTS((6,1,1,1,1,1,1,1,1,1,1,1,1,1,1,1,1,1,1,1,1,1,
1,1,1,1,1,1,1,1,1,1,1,1,1,1,1,1,1,1,1,1,1,1,1,1,1,1,1,1,1,1,1,1,1,1,1,1,
1,1,1,1,1,1,1,1,1,1,1,1,1,1,1,1,1,1,1,1,1,1,1,1,1,1,1,1,1,1,1,1,1,1,1,1,
1,1,1,1,1,1,1,1,1,1,1,1,1,1,1,1,1,1,1,1,1,1,1,1,1,1,1,1,1,1,1,1,1,1,1,1,
1,1,1,1,1,1,1,1,1,1,1,1,1,1,1,1,1,1,1,1,1,1,1,1,1,1,1,1,1,1,1,1,1,1,1,1,
1,1,1,1,1,1,1,1,1,1,1,1,1,1,1,1,1,1,1,1,1,1,1,1,1,1,1,1,1,1,1,1,1,1,6),
(0.,0.005,0.01,0.015,0.02,0.025,0.03,0.035,0.04,0.045,0.05,0.055,0.06,0.065,
0.07,0.075,0.08,0.085,0.09,0.095,0.1,0.105,0.11,0.115,0.12,0.125,0.13,0.135,
0.14,0.145,0.15,0.155,0.16,0.165,0.17,0.175,0.18,0.185,0.19,0.195,0.2,0.205,
0.21,0.215,0.22,0.225,0.23,0.235,0.24,0.245,0.25,0.255,0.26,0.265,0.27,
0.275,0.28,0.285,0.29,0.295,0.3,0.305,0.31,0.315,0.32,0.325,0.33,0.335,
0.34,0.345,0.35,0.355,0.36,0.365,0.37,0.375,0.38,0.385,0.39,0.395,0.4,0.405,
0.41,0.415,0.42,0.425,0.43,0.435,0.44,0.445,0.45,0.455,0.46,0.465,0.47,
0.475,0.48,0.485,0.49,0.495,0.5,0.505,0.51,0.515,0.52,0.525,0.53,0.535,
0.54,0.545,0.55,0.555,0.56,0.565,0.57,0.575,0.58,0.585,0.59,0.595,0.6,0.605,
0.61,0.615,0.62,0.625,0.63,0.635,0.64,0.645,0.65,0.655,0.66,0.665,0.67,
0.675,0.68,0.685,0.690000000000001,0.695000000000001,0.700000000000001,
0.705000000000001,0.710000000000001,0.715000000000001,0.720000000000001,
0.725000000000001,0.730000000000001,0.735000000000001,0.740000000000001,
0.745000000000001,0.750000000000001,0.755000000000001,0.760000000000001,
0.765000000000001,0.770000000000001,0.775000000000001,0.780000000000001,
0.785000000000001,0.790000000000001,0.795000000000001,0.800000000000001,
0.805000000000001,0.810000000000001,0.815000000000001,0.820000000000001,
0.825000000000001,0.830000000000001,0.835000000000001,0.840000000000001,
0.845000000000001,0.850000000000001,0.855000000000001,0.860000000000001,
0.865000000000001,0.870000000000001,0.875000000000001,0.880000000000001,
0.885000000000001,0.890000000000001,0.895000000000001,0.900000000000001,
0.905000000000001,0.910000000000001,0.915000000000001,0.920000000000001,
0.925000000000001,0.930000000000001,0.935000000000001,0.940000000000001,
0.945000000000001,0.950000000000001,0.955000000000001,0.960000000000001,
0.965000000000001,0.970000000000001,0.975000000000001,0.980000000000001,
0.985000000000001,0.990000000000001,0.995000000000001,1.),.UNSPECIFIED.)
CURVE()
GEOMETRIC_REPRESENTATION_ITEM()
RATIONAL_B_SPLINE_CURVE((1.,1.,1.,1.,1.,1.,1.,1.,1.,1.,1.,1.,1.,1.,1.,1.,
1.,1.,1.,1.,1.,1.,1.,1.,1.,1.,1.,1.,1.,1.,1.,1.,1.,1.,1.,1.,1.,1.,1.,1.,
1.,1.,1.,1.,1.,1.,1.,1.,1.,1.,1.,1.,1.,1.,1.,1.,1.,1.,1.,1.,1.,1.,1.,1.,
1.,1.,1.,1.,1.,1.,1.,1.,1.,1.,1.,1.,1.,1.,1.,1.,1.,1.,1.,1.,1.,1.,1.,1.,
1.,1.,1.,1.,1.,1.,1.,1.,1.,1.,1.,1.,1.,1.,1.,1.,1.,1.,1.,1.,1.,1.,1.,1.,
1.,1.,1.,1.,1.,1.,1.,1.,1.,1.,1.,1.,1.,1.,1.,1.,1.,1.,1.,1.,1.,1.,1.,1.,
1.,1.,1.,1.,1.,1.,1.,1.,1.,1.,1.,1.,1.,1.,1.,1.,1.,1.,1.,1.,1.,1.,1.,1.,
1.,1.,1.,1.,1.,1.,1.,1.,1.,1.,1.,1.,1.,1.,1.,1.,1.,1.,1.,1.,1.,1.,1.,1.,
1.,1.,1.,1.,1.,1.,1.,1.,1.,1.,1.,1.,1.,1.,1.,1.,1.,1.,1.,1.,1.))
REPRESENTATION_ITEM('')
);
#718=(
BOUNDED_CURVE()
B_SPLINE_CURVE(5,(#180733,#180734,#180735,#180736,#180737,#180738,#180739,
#180740,#180741,#180742,#180743,#180744,#180745,#180746,#180747,#180748,
#180749,#180750,#180751,#180752,#180753,#180754,#180755,#180756,#180757,
#180758,#180759,#180760,#180761,#180762,#180763,#180764,#180765,#180766,
#180767,#180768,#180769,#180770,#180771,#180772,#180773,#180774,#180775,
#180776,#180777,#180778,#180779,#180780,#180781,#180782,#180783,#180784,
#180785,#180786,#180787,#180788,#180789,#180790,#180791,#180792,#180793,
#180794,#180795,#180796,#180797,#180798,#180799,#180800,#180801,#180802,
#180803,#180804,#180805,#180806,#180807,#180808,#180809,#180810,#180811,
#180812,#180813,#180814,#180815,#180816,#180817,#180818,#180819,#180820,
#180821,#180822,#180823,#180824,#180825,#180826,#180827,#180828,#180829,
#180830,#180831,#180832,#180833,#180834,#180835,#180836,#180837,#180838,
#180839,#180840,#180841,#180842,#180843,#180844,#180845,#180846,#180847,
#180848,#180849,#180850,#180851,#180852,#180853,#180854,#180855,#180856,
#180857,#180858,#180859,#180860,#180861,#180862,#180863,#180864,#180865,
#180866,#180867,#180868,#180869,#180870,#180871,#180872,#180873,#180874,
#180875,#180876,#180877,#180878,#180879,#180880,#180881,#180882,#180883,
#180884,#180885,#180886,#180887,#180888,#180889,#180890,#180891,#180892,
#180893,#180894,#180895,#180896,#180897,#180898,#180899,#180900,#180901,
#180902,#180903,#180904,#180905,#180906,#180907,#180908,#180909,#180910,
#180911,#180912,#180913,#180914,#180915,#180916,#180917,#180918,#180919,
#180920,#180921,#180922,#180923,#180924,#180925,#180926,#180927,#180928,
#180929,#180930,#180931,#180932,#180933,#180934,#180935,#180936,#180937),
 .UNSPECIFIED.,.F.,.F.)
B_SPLINE_CURVE_WITH_KNOTS((6,1,1,1,1,1,1,1,1,1,1,1,1,1,1,1,1,1,1,1,1,1,
1,1,1,1,1,1,1,1,1,1,1,1,1,1,1,1,1,1,1,1,1,1,1,1,1,1,1,1,1,1,1,1,1,1,1,1,
1,1,1,1,1,1,1,1,1,1,1,1,1,1,1,1,1,1,1,1,1,1,1,1,1,1,1,1,1,1,1,1,1,1,1,1,
1,1,1,1,1,1,1,1,1,1,1,1,1,1,1,1,1,1,1,1,1,1,1,1,1,1,1,1,1,1,1,1,1,1,1,1,
1,1,1,1,1,1,1,1,1,1,1,1,1,1,1,1,1,1,1,1,1,1,1,1,1,1,1,1,1,1,1,1,1,1,1,1,
1,1,1,1,1,1,1,1,1,1,1,1,1,1,1,1,1,1,1,1,1,1,1,1,1,1,1,1,1,1,1,1,1,1,6),
(-1.,-0.995000000000001,-0.990000000000001,-0.985000000000001,-0.980000000000001,
-0.975000000000001,-0.970000000000001,-0.965000000000001,-0.960000000000001,
-0.955000000000001,-0.950000000000001,-0.945000000000001,-0.940000000000001,
-0.935000000000001,-0.930000000000001,-0.925000000000001,-0.920000000000001,
-0.915000000000001,-0.910000000000001,-0.905000000000001,-0.900000000000001,
-0.895000000000001,-0.890000000000001,-0.885000000000001,-0.880000000000001,
-0.875000000000001,-0.870000000000001,-0.865000000000001,-0.860000000000001,
-0.855000000000001,-0.850000000000001,-0.845000000000001,-0.840000000000001,
-0.835000000000001,-0.830000000000001,-0.825000000000001,-0.820000000000001,
-0.815000000000001,-0.810000000000001,-0.805000000000001,-0.800000000000001,
-0.795000000000001,-0.790000000000001,-0.785000000000001,-0.780000000000001,
-0.775000000000001,-0.770000000000001,-0.765000000000001,-0.760000000000001,
-0.755000000000001,-0.750000000000001,-0.745000000000001,-0.740000000000001,
-0.735000000000001,-0.730000000000001,-0.725000000000001,-0.720000000000001,
-0.715000000000001,-0.710000000000001,-0.705000000000001,-0.700000000000001,
-0.695000000000001,-0.690000000000001,-0.685,-0.68,-0.675,-0.67,-0.665,
-0.66,-0.655,-0.65,-0.645,-0.64,-0.635,-0.63,-0.625,-0.62,-0.615,-0.61,
-0.605,-0.6,-0.595,-0.59,-0.585,-0.58,-0.575,-0.57,-0.565,-0.56,-0.555,
-0.55,-0.545,-0.54,-0.535,-0.53,-0.525,-0.52,-0.515,-0.51,-0.505,-0.5,-0.495,
-0.49,-0.485,-0.48,-0.475,-0.47,-0.465,-0.46,-0.455,-0.45,-0.445,-0.44,
-0.435,-0.43,-0.425,-0.42,-0.415,-0.41,-0.405,-0.4,-0.395,-0.39,-0.385,
-0.38,-0.375,-0.37,-0.365,-0.36,-0.355,-0.35,-0.345,-0.34,-0.335,-0.33,
-0.325,-0.32,-0.315,-0.31,-0.305,-0.3,-0.295,-0.29,-0.285,-0.28,-0.275,
-0.27,-0.265,-0.26,-0.255,-0.25,-0.245,-0.24,-0.235,-0.23,-0.225,-0.22,
-0.215,-0.21,-0.205,-0.2,-0.195,-0.19,-0.185,-0.18,-0.175,-0.17,-0.165,
-0.16,-0.155,-0.15,-0.145,-0.14,-0.135,-0.13,-0.125,-0.12,-0.115,-0.11,
-0.105,-0.1,-0.095,-0.09,-0.085,-0.08,-0.075,-0.07,-0.065,-0.06,-0.055,
-0.05,-0.045,-0.04,-0.035,-0.03,-0.025,-0.02,-0.015,-0.01,-0.005,0.),
 .UNSPECIFIED.)
CURVE()
GEOMETRIC_REPRESENTATION_ITEM()
RATIONAL_B_SPLINE_CURVE((1.,1.,1.,1.,1.,1.,1.,1.,1.,1.,1.,1.,1.,1.,1.,1.,
1.,1.,1.,1.,1.,1.,1.,1.,1.,1.,1.,1.,1.,1.,1.,1.,1.,1.,1.,1.,1.,1.,1.,1.,
1.,1.,1.,1.,1.,1.,1.,1.,1.,1.,1.,1.,1.,1.,1.,1.,1.,1.,1.,1.,1.,1.,1.,1.,
1.,1.,1.,1.,1.,1.,1.,1.,1.,1.,1.,1.,1.,1.,1.,1.,1.,1.,1.,1.,1.,1.,1.,1.,
1.,1.,1.,1.,1.,1.,1.,1.,1.,1.,1.,1.,1.,1.,1.,1.,1.,1.,1.,1.,1.,1.,1.,1.,
1.,1.,1.,1.,1.,1.,1.,1.,1.,1.,1.,1.,1.,1.,1.,1.,1.,1.,1.,1.,1.,1.,1.,1.,
1.,1.,1.,1.,1.,1.,1.,1.,1.,1.,1.,1.,1.,1.,1.,1.,1.,1.,1.,1.,1.,1.,1.,1.,
1.,1.,1.,1.,1.,1.,1.,1.,1.,1.,1.,1.,1.,1.,1.,1.,1.,1.,1.,1.,1.,1.,1.,1.,
1.,1.,1.,1.,1.,1.,1.,1.,1.,1.,1.,1.,1.,1.,1.,1.,1.,1.,1.,1.,1.))
REPRESENTATION_ITEM('')
);
#719=(
BOUNDED_CURVE()
B_SPLINE_CURVE(5,(#180949,#180950,#180951,#180952,#180953,#180954,#180955,
#180956,#180957,#180958,#180959,#180960,#180961,#180962,#180963,#180964,
#180965,#180966,#180967,#180968,#180969,#180970,#180971,#180972,#180973,
#180974,#180975,#180976,#180977,#180978,#180979,#180980,#180981,#180982,
#180983,#180984,#180985,#180986,#180987,#180988,#180989,#180990,#180991,
#180992,#180993,#180994,#180995,#180996,#180997,#180998,#180999,#181000,
#181001,#181002,#181003,#181004,#181005,#181006,#181007,#181008,#181009,
#181010,#181011,#181012,#181013,#181014,#181015,#181016,#181017,#181018,
#181019,#181020,#181021,#181022,#181023,#181024,#181025,#181026,#181027,
#181028,#181029,#181030,#181031,#181032,#181033,#181034,#181035,#181036,
#181037,#181038,#181039,#181040,#181041,#181042,#181043,#181044,#181045,
#181046,#181047,#181048,#181049,#181050,#181051,#181052,#181053,#181054,
#181055,#181056,#181057,#181058,#181059,#181060,#181061,#181062,#181063,
#181064,#181065,#181066,#181067,#181068,#181069,#181070,#181071,#181072,
#181073,#181074,#181075,#181076,#181077,#181078,#181079,#181080,#181081,
#181082,#181083,#181084,#181085,#181086,#181087,#181088,#181089,#181090,
#181091,#181092,#181093,#181094,#181095,#181096,#181097,#181098,#181099,
#181100,#181101,#181102,#181103,#181104,#181105,#181106,#181107,#181108,
#181109,#181110,#181111,#181112,#181113,#181114,#181115,#181116,#181117,
#181118,#181119,#181120,#181121,#181122,#181123,#181124,#181125,#181126,
#181127,#181128,#181129,#181130,#181131,#181132,#181133,#181134,#181135,
#181136,#181137,#181138,#181139,#181140,#181141,#181142,#181143,#181144,
#181145,#181146,#181147,#181148,#181149,#181150,#181151,#181152,#181153),
 .UNSPECIFIED.,.F.,.F.)
B_SPLINE_CURVE_WITH_KNOTS((6,1,1,1,1,1,1,1,1,1,1,1,1,1,1,1,1,1,1,1,1,1,
1,1,1,1,1,1,1,1,1,1,1,1,1,1,1,1,1,1,1,1,1,1,1,1,1,1,1,1,1,1,1,1,1,1,1,1,
1,1,1,1,1,1,1,1,1,1,1,1,1,1,1,1,1,1,1,1,1,1,1,1,1,1,1,1,1,1,1,1,1,1,1,1,
1,1,1,1,1,1,1,1,1,1,1,1,1,1,1,1,1,1,1,1,1,1,1,1,1,1,1,1,1,1,1,1,1,1,1,1,
1,1,1,1,1,1,1,1,1,1,1,1,1,1,1,1,1,1,1,1,1,1,1,1,1,1,1,1,1,1,1,1,1,1,1,1,
1,1,1,1,1,1,1,1,1,1,1,1,1,1,1,1,1,1,1,1,1,1,1,1,1,1,1,1,1,1,1,1,1,1,6),
(0.,0.005,0.01,0.015,0.02,0.025,0.03,0.035,0.04,0.045,0.05,0.055,0.06,0.065,
0.07,0.075,0.08,0.085,0.09,0.095,0.1,0.105,0.11,0.115,0.12,0.125,0.13,0.135,
0.14,0.145,0.15,0.155,0.16,0.165,0.17,0.175,0.18,0.185,0.19,0.195,0.2,0.205,
0.21,0.215,0.22,0.225,0.23,0.235,0.24,0.245,0.25,0.255,0.26,0.265,0.27,
0.275,0.28,0.285,0.29,0.295,0.3,0.305,0.31,0.315,0.32,0.325,0.33,0.335,
0.34,0.345,0.35,0.355,0.36,0.365,0.37,0.375,0.38,0.385,0.39,0.395,0.4,0.405,
0.41,0.415,0.42,0.425,0.43,0.435,0.44,0.445,0.45,0.455,0.46,0.465,0.47,
0.475,0.48,0.485,0.49,0.495,0.5,0.505,0.51,0.515,0.52,0.525,0.53,0.535,
0.54,0.545,0.55,0.555,0.56,0.565,0.57,0.575,0.58,0.585,0.59,0.595,0.6,0.605,
0.61,0.615,0.62,0.625,0.63,0.635,0.64,0.645,0.65,0.655,0.66,0.665,0.67,
0.675,0.68,0.685,0.690000000000001,0.695000000000001,0.700000000000001,
0.705000000000001,0.710000000000001,0.715000000000001,0.720000000000001,
0.725000000000001,0.730000000000001,0.735000000000001,0.740000000000001,
0.745000000000001,0.750000000000001,0.755000000000001,0.760000000000001,
0.765000000000001,0.770000000000001,0.775000000000001,0.780000000000001,
0.785000000000001,0.790000000000001,0.795000000000001,0.800000000000001,
0.805000000000001,0.810000000000001,0.815000000000001,0.820000000000001,
0.825000000000001,0.830000000000001,0.835000000000001,0.840000000000001,
0.845000000000001,0.850000000000001,0.855000000000001,0.860000000000001,
0.865000000000001,0.870000000000001,0.875000000000001,0.880000000000001,
0.885000000000001,0.890000000000001,0.895000000000001,0.900000000000001,
0.905000000000001,0.910000000000001,0.915000000000001,0.920000000000001,
0.925000000000001,0.930000000000001,0.935000000000001,0.940000000000001,
0.945000000000001,0.950000000000001,0.955000000000001,0.960000000000001,
0.965000000000001,0.970000000000001,0.975000000000001,0.980000000000001,
0.985000000000001,0.990000000000001,0.995000000000001,1.),.UNSPECIFIED.)
CURVE()
GEOMETRIC_REPRESENTATION_ITEM()
RATIONAL_B_SPLINE_CURVE((1.,1.,1.,1.,1.,1.,1.,1.,1.,1.,1.,1.,1.,1.,1.,1.,
1.,1.,1.,1.,1.,1.,1.,1.,1.,1.,1.,1.,1.,1.,1.,1.,1.,1.,1.,1.,1.,1.,1.,1.,
1.,1.,1.,1.,1.,1.,1.,1.,1.,1.,1.,1.,1.,1.,1.,1.,1.,1.,1.,1.,1.,1.,1.,1.,
1.,1.,1.,1.,1.,1.,1.,1.,1.,1.,1.,1.,1.,1.,1.,1.,1.,1.,1.,1.,1.,1.,1.,1.,
1.,1.,1.,1.,1.,1.,1.,1.,1.,1.,1.,1.,1.,1.,1.,1.,1.,1.,1.,1.,1.,1.,1.,1.,
1.,1.,1.,1.,1.,1.,1.,1.,1.,1.,1.,1.,1.,1.,1.,1.,1.,1.,1.,1.,1.,1.,1.,1.,
1.,1.,1.,1.,1.,1.,1.,1.,1.,1.,1.,1.,1.,1.,1.,1.,1.,1.,1.,1.,1.,1.,1.,1.,
1.,1.,1.,1.,1.,1.,1.,1.,1.,1.,1.,1.,1.,1.,1.,1.,1.,1.,1.,1.,1.,1.,1.,1.,
1.,1.,1.,1.,1.,1.,1.,1.,1.,1.,1.,1.,1.,1.,1.,1.,1.,1.,1.,1.,1.))
REPRESENTATION_ITEM('')
);
#720=(
BOUNDED_CURVE()
B_SPLINE_CURVE(5,(#181157,#181158,#181159,#181160,#181161,#181162,#181163,
#181164,#181165,#181166,#181167,#181168,#181169,#181170,#181171,#181172,
#181173,#181174,#181175,#181176,#181177,#181178,#181179,#181180,#181181,
#181182,#181183,#181184,#181185,#181186,#181187,#181188,#181189,#181190,
#181191,#181192,#181193,#181194,#181195,#181196,#181197,#181198,#181199,
#181200,#181201,#181202,#181203,#181204,#181205,#181206,#181207,#181208,
#181209,#181210,#181211,#181212,#181213,#181214,#181215,#181216,#181217,
#181218,#181219,#181220,#181221,#181222,#181223,#181224,#181225,#181226,
#181227,#181228,#181229,#181230,#181231,#181232,#181233,#181234,#181235,
#181236,#181237,#181238,#181239,#181240,#181241,#181242,#181243,#181244,
#181245,#181246,#181247,#181248,#181249,#181250,#181251,#181252,#181253,
#181254,#181255,#181256,#181257,#181258,#181259,#181260,#181261,#181262,
#181263,#181264,#181265,#181266,#181267,#181268,#181269,#181270,#181271,
#181272,#181273,#181274,#181275,#181276,#181277,#181278,#181279,#181280,
#181281,#181282,#181283,#181284,#181285,#181286,#181287,#181288,#181289,
#181290,#181291,#181292,#181293,#181294,#181295,#181296,#181297,#181298,
#181299,#181300,#181301,#181302,#181303,#181304,#181305,#181306,#181307,
#181308,#181309,#181310,#181311,#181312,#181313,#181314,#181315,#181316,
#181317,#181318,#181319,#181320,#181321,#181322,#181323,#181324,#181325,
#181326,#181327,#181328,#181329,#181330,#181331,#181332,#181333,#181334,
#181335,#181336,#181337,#181338,#181339,#181340,#181341,#181342,#181343,
#181344,#181345,#181346,#181347,#181348,#181349,#181350,#181351,#181352,
#181353,#181354,#181355,#181356,#181357,#181358,#181359,#181360,#181361),
 .UNSPECIFIED.,.F.,.F.)
B_SPLINE_CURVE_WITH_KNOTS((6,1,1,1,1,1,1,1,1,1,1,1,1,1,1,1,1,1,1,1,1,1,
1,1,1,1,1,1,1,1,1,1,1,1,1,1,1,1,1,1,1,1,1,1,1,1,1,1,1,1,1,1,1,1,1,1,1,1,
1,1,1,1,1,1,1,1,1,1,1,1,1,1,1,1,1,1,1,1,1,1,1,1,1,1,1,1,1,1,1,1,1,1,1,1,
1,1,1,1,1,1,1,1,1,1,1,1,1,1,1,1,1,1,1,1,1,1,1,1,1,1,1,1,1,1,1,1,1,1,1,1,
1,1,1,1,1,1,1,1,1,1,1,1,1,1,1,1,1,1,1,1,1,1,1,1,1,1,1,1,1,1,1,1,1,1,1,1,
1,1,1,1,1,1,1,1,1,1,1,1,1,1,1,1,1,1,1,1,1,1,1,1,1,1,1,1,1,1,1,1,1,1,6),
(-1.,-0.995000000000001,-0.990000000000001,-0.985000000000001,-0.980000000000001,
-0.975000000000001,-0.970000000000001,-0.965000000000001,-0.960000000000001,
-0.955000000000001,-0.950000000000001,-0.945000000000001,-0.940000000000001,
-0.935000000000001,-0.930000000000001,-0.925000000000001,-0.920000000000001,
-0.915000000000001,-0.910000000000001,-0.905000000000001,-0.900000000000001,
-0.895000000000001,-0.890000000000001,-0.885000000000001,-0.880000000000001,
-0.875000000000001,-0.870000000000001,-0.865000000000001,-0.860000000000001,
-0.855000000000001,-0.850000000000001,-0.845000000000001,-0.840000000000001,
-0.835000000000001,-0.830000000000001,-0.825000000000001,-0.820000000000001,
-0.815000000000001,-0.810000000000001,-0.805000000000001,-0.800000000000001,
-0.795000000000001,-0.790000000000001,-0.785000000000001,-0.780000000000001,
-0.775000000000001,-0.770000000000001,-0.765000000000001,-0.760000000000001,
-0.755000000000001,-0.750000000000001,-0.745000000000001,-0.740000000000001,
-0.735000000000001,-0.730000000000001,-0.725000000000001,-0.720000000000001,
-0.715000000000001,-0.710000000000001,-0.705000000000001,-0.700000000000001,
-0.695000000000001,-0.690000000000001,-0.685,-0.68,-0.675,-0.67,-0.665,
-0.66,-0.655,-0.65,-0.645,-0.64,-0.635,-0.63,-0.625,-0.62,-0.615,-0.61,
-0.605,-0.6,-0.595,-0.59,-0.585,-0.58,-0.575,-0.57,-0.565,-0.56,-0.555,
-0.55,-0.545,-0.54,-0.535,-0.53,-0.525,-0.52,-0.515,-0.51,-0.505,-0.5,-0.495,
-0.49,-0.485,-0.48,-0.475,-0.47,-0.465,-0.46,-0.455,-0.45,-0.445,-0.44,
-0.435,-0.43,-0.425,-0.42,-0.415,-0.41,-0.405,-0.4,-0.395,-0.39,-0.385,
-0.38,-0.375,-0.37,-0.365,-0.36,-0.355,-0.35,-0.345,-0.34,-0.335,-0.33,
-0.325,-0.32,-0.315,-0.31,-0.305,-0.3,-0.295,-0.29,-0.285,-0.28,-0.275,
-0.27,-0.265,-0.26,-0.255,-0.25,-0.245,-0.24,-0.235,-0.23,-0.225,-0.22,
-0.215,-0.21,-0.205,-0.2,-0.195,-0.19,-0.185,-0.18,-0.175,-0.17,-0.165,
-0.16,-0.155,-0.15,-0.145,-0.14,-0.135,-0.13,-0.125,-0.12,-0.115,-0.11,
-0.105,-0.1,-0.095,-0.09,-0.085,-0.08,-0.075,-0.07,-0.065,-0.06,-0.055,
-0.05,-0.045,-0.04,-0.035,-0.03,-0.025,-0.02,-0.015,-0.01,-0.005,0.),
 .UNSPECIFIED.)
CURVE()
GEOMETRIC_REPRESENTATION_ITEM()
RATIONAL_B_SPLINE_CURVE((1.,1.,1.,1.,1.,1.,1.,1.,1.,1.,1.,1.,1.,1.,1.,1.,
1.,1.,1.,1.,1.,1.,1.,1.,1.,1.,1.,1.,1.,1.,1.,1.,1.,1.,1.,1.,1.,1.,1.,1.,
1.,1.,1.,1.,1.,1.,1.,1.,1.,1.,1.,1.,1.,1.,1.,1.,1.,1.,1.,1.,1.,1.,1.,1.,
1.,1.,1.,1.,1.,1.,1.,1.,1.,1.,1.,1.,1.,1.,1.,1.,1.,1.,1.,1.,1.,1.,1.,1.,
1.,1.,1.,1.,1.,1.,1.,1.,1.,1.,1.,1.,1.,1.,1.,1.,1.,1.,1.,1.,1.,1.,1.,1.,
1.,1.,1.,1.,1.,1.,1.,1.,1.,1.,1.,1.,1.,1.,1.,1.,1.,1.,1.,1.,1.,1.,1.,1.,
1.,1.,1.,1.,1.,1.,1.,1.,1.,1.,1.,1.,1.,1.,1.,1.,1.,1.,1.,1.,1.,1.,1.,1.,
1.,1.,1.,1.,1.,1.,1.,1.,1.,1.,1.,1.,1.,1.,1.,1.,1.,1.,1.,1.,1.,1.,1.,1.,
1.,1.,1.,1.,1.,1.,1.,1.,1.,1.,1.,1.,1.,1.,1.,1.,1.,1.,1.,1.,1.))
REPRESENTATION_ITEM('')
);
#721=(
BOUNDED_CURVE()
B_SPLINE_CURVE(5,(#181373,#181374,#181375,#181376,#181377,#181378,#181379,
#181380,#181381,#181382,#181383,#181384,#181385,#181386,#181387,#181388,
#181389,#181390,#181391,#181392,#181393,#181394,#181395,#181396,#181397,
#181398,#181399,#181400,#181401,#181402,#181403,#181404,#181405,#181406,
#181407,#181408,#181409,#181410,#181411,#181412,#181413,#181414,#181415,
#181416,#181417,#181418,#181419,#181420,#181421,#181422,#181423,#181424,
#181425,#181426,#181427,#181428,#181429,#181430,#181431,#181432,#181433,
#181434,#181435,#181436,#181437,#181438,#181439,#181440,#181441,#181442,
#181443,#181444,#181445,#181446,#181447,#181448,#181449,#181450,#181451,
#181452,#181453,#181454,#181455,#181456,#181457,#181458,#181459,#181460,
#181461,#181462,#181463,#181464,#181465,#181466,#181467,#181468,#181469,
#181470,#181471,#181472,#181473,#181474,#181475,#181476,#181477,#181478,
#181479,#181480,#181481,#181482,#181483,#181484,#181485,#181486,#181487,
#181488,#181489,#181490,#181491,#181492,#181493,#181494,#181495,#181496,
#181497,#181498,#181499,#181500,#181501,#181502,#181503,#181504,#181505,
#181506,#181507,#181508,#181509,#181510,#181511,#181512,#181513,#181514,
#181515,#181516,#181517,#181518,#181519,#181520,#181521,#181522,#181523,
#181524,#181525,#181526,#181527,#181528,#181529,#181530,#181531,#181532,
#181533,#181534,#181535,#181536,#181537,#181538,#181539,#181540,#181541,
#181542,#181543,#181544,#181545,#181546,#181547,#181548,#181549,#181550,
#181551,#181552,#181553,#181554,#181555,#181556,#181557,#181558,#181559,
#181560,#181561,#181562,#181563,#181564,#181565,#181566,#181567,#181568,
#181569,#181570,#181571,#181572,#181573,#181574,#181575,#181576,#181577),
 .UNSPECIFIED.,.F.,.F.)
B_SPLINE_CURVE_WITH_KNOTS((6,1,1,1,1,1,1,1,1,1,1,1,1,1,1,1,1,1,1,1,1,1,
1,1,1,1,1,1,1,1,1,1,1,1,1,1,1,1,1,1,1,1,1,1,1,1,1,1,1,1,1,1,1,1,1,1,1,1,
1,1,1,1,1,1,1,1,1,1,1,1,1,1,1,1,1,1,1,1,1,1,1,1,1,1,1,1,1,1,1,1,1,1,1,1,
1,1,1,1,1,1,1,1,1,1,1,1,1,1,1,1,1,1,1,1,1,1,1,1,1,1,1,1,1,1,1,1,1,1,1,1,
1,1,1,1,1,1,1,1,1,1,1,1,1,1,1,1,1,1,1,1,1,1,1,1,1,1,1,1,1,1,1,1,1,1,1,1,
1,1,1,1,1,1,1,1,1,1,1,1,1,1,1,1,1,1,1,1,1,1,1,1,1,1,1,1,1,1,1,1,1,1,6),
(0.,0.005,0.01,0.015,0.02,0.025,0.03,0.035,0.04,0.045,0.05,0.055,0.06,0.065,
0.07,0.075,0.08,0.085,0.09,0.095,0.1,0.105,0.11,0.115,0.12,0.125,0.13,0.135,
0.14,0.145,0.15,0.155,0.16,0.165,0.17,0.175,0.18,0.185,0.19,0.195,0.2,0.205,
0.21,0.215,0.22,0.225,0.23,0.235,0.24,0.245,0.25,0.255,0.26,0.265,0.27,
0.275,0.28,0.285,0.29,0.295,0.3,0.305,0.31,0.315,0.32,0.325,0.33,0.335,
0.34,0.345,0.35,0.355,0.36,0.365,0.37,0.375,0.38,0.385,0.39,0.395,0.4,0.405,
0.41,0.415,0.42,0.425,0.43,0.435,0.44,0.445,0.45,0.455,0.46,0.465,0.47,
0.475,0.48,0.485,0.49,0.495,0.5,0.505,0.51,0.515,0.52,0.525,0.53,0.535,
0.54,0.545,0.55,0.555,0.56,0.565,0.57,0.575,0.58,0.585,0.59,0.595,0.6,0.605,
0.61,0.615,0.62,0.625,0.63,0.635,0.64,0.645,0.65,0.655,0.66,0.665,0.67,
0.675,0.68,0.685,0.690000000000001,0.695000000000001,0.700000000000001,
0.705000000000001,0.710000000000001,0.715000000000001,0.720000000000001,
0.725000000000001,0.730000000000001,0.735000000000001,0.740000000000001,
0.745000000000001,0.750000000000001,0.755000000000001,0.760000000000001,
0.765000000000001,0.770000000000001,0.775000000000001,0.780000000000001,
0.785000000000001,0.790000000000001,0.795000000000001,0.800000000000001,
0.805000000000001,0.810000000000001,0.815000000000001,0.820000000000001,
0.825000000000001,0.830000000000001,0.835000000000001,0.840000000000001,
0.845000000000001,0.850000000000001,0.855000000000001,0.860000000000001,
0.865000000000001,0.870000000000001,0.875000000000001,0.880000000000001,
0.885000000000001,0.890000000000001,0.895000000000001,0.900000000000001,
0.905000000000001,0.910000000000001,0.915000000000001,0.920000000000001,
0.925000000000001,0.930000000000001,0.935000000000001,0.940000000000001,
0.945000000000001,0.950000000000001,0.955000000000001,0.960000000000001,
0.965000000000001,0.970000000000001,0.975000000000001,0.980000000000001,
0.985000000000001,0.990000000000001,0.995000000000001,1.),.UNSPECIFIED.)
CURVE()
GEOMETRIC_REPRESENTATION_ITEM()
RATIONAL_B_SPLINE_CURVE((1.,1.,1.,1.,1.,1.,1.,1.,1.,1.,1.,1.,1.,1.,1.,1.,
1.,1.,1.,1.,1.,1.,1.,1.,1.,1.,1.,1.,1.,1.,1.,1.,1.,1.,1.,1.,1.,1.,1.,1.,
1.,1.,1.,1.,1.,1.,1.,1.,1.,1.,1.,1.,1.,1.,1.,1.,1.,1.,1.,1.,1.,1.,1.,1.,
1.,1.,1.,1.,1.,1.,1.,1.,1.,1.,1.,1.,1.,1.,1.,1.,1.,1.,1.,1.,1.,1.,1.,1.,
1.,1.,1.,1.,1.,1.,1.,1.,1.,1.,1.,1.,1.,1.,1.,1.,1.,1.,1.,1.,1.,1.,1.,1.,
1.,1.,1.,1.,1.,1.,1.,1.,1.,1.,1.,1.,1.,1.,1.,1.,1.,1.,1.,1.,1.,1.,1.,1.,
1.,1.,1.,1.,1.,1.,1.,1.,1.,1.,1.,1.,1.,1.,1.,1.,1.,1.,1.,1.,1.,1.,1.,1.,
1.,1.,1.,1.,1.,1.,1.,1.,1.,1.,1.,1.,1.,1.,1.,1.,1.,1.,1.,1.,1.,1.,1.,1.,
1.,1.,1.,1.,1.,1.,1.,1.,1.,1.,1.,1.,1.,1.,1.,1.,1.,1.,1.,1.,1.))
REPRESENTATION_ITEM('')
);
#722=(
BOUNDED_CURVE()
B_SPLINE_CURVE(5,(#181581,#181582,#181583,#181584,#181585,#181586,#181587,
#181588,#181589,#181590,#181591,#181592,#181593,#181594,#181595,#181596,
#181597,#181598,#181599,#181600,#181601,#181602,#181603,#181604,#181605,
#181606,#181607,#181608,#181609,#181610,#181611,#181612,#181613,#181614,
#181615,#181616,#181617,#181618,#181619,#181620,#181621,#181622,#181623,
#181624,#181625,#181626,#181627,#181628,#181629,#181630,#181631,#181632,
#181633,#181634,#181635,#181636,#181637,#181638,#181639,#181640,#181641,
#181642,#181643,#181644,#181645,#181646,#181647,#181648,#181649,#181650,
#181651,#181652,#181653,#181654,#181655,#181656,#181657,#181658,#181659,
#181660,#181661,#181662,#181663,#181664,#181665,#181666,#181667,#181668,
#181669,#181670,#181671,#181672,#181673,#181674,#181675,#181676,#181677,
#181678,#181679,#181680,#181681,#181682,#181683,#181684,#181685,#181686,
#181687,#181688,#181689,#181690,#181691,#181692,#181693,#181694,#181695,
#181696,#181697,#181698,#181699,#181700,#181701,#181702,#181703,#181704,
#181705,#181706,#181707,#181708,#181709,#181710,#181711,#181712,#181713,
#181714,#181715,#181716,#181717,#181718,#181719,#181720,#181721,#181722,
#181723,#181724,#181725,#181726,#181727,#181728,#181729,#181730,#181731,
#181732,#181733,#181734,#181735,#181736,#181737,#181738,#181739,#181740,
#181741,#181742,#181743,#181744,#181745,#181746,#181747,#181748,#181749,
#181750,#181751,#181752,#181753,#181754,#181755,#181756,#181757,#181758,
#181759,#181760,#181761,#181762,#181763,#181764,#181765,#181766,#181767,
#181768,#181769,#181770,#181771,#181772,#181773,#181774,#181775,#181776,
#181777,#181778,#181779,#181780,#181781,#181782,#181783,#181784,#181785),
 .UNSPECIFIED.,.F.,.F.)
B_SPLINE_CURVE_WITH_KNOTS((6,1,1,1,1,1,1,1,1,1,1,1,1,1,1,1,1,1,1,1,1,1,
1,1,1,1,1,1,1,1,1,1,1,1,1,1,1,1,1,1,1,1,1,1,1,1,1,1,1,1,1,1,1,1,1,1,1,1,
1,1,1,1,1,1,1,1,1,1,1,1,1,1,1,1,1,1,1,1,1,1,1,1,1,1,1,1,1,1,1,1,1,1,1,1,
1,1,1,1,1,1,1,1,1,1,1,1,1,1,1,1,1,1,1,1,1,1,1,1,1,1,1,1,1,1,1,1,1,1,1,1,
1,1,1,1,1,1,1,1,1,1,1,1,1,1,1,1,1,1,1,1,1,1,1,1,1,1,1,1,1,1,1,1,1,1,1,1,
1,1,1,1,1,1,1,1,1,1,1,1,1,1,1,1,1,1,1,1,1,1,1,1,1,1,1,1,1,1,1,1,1,1,6),
(-1.,-0.995000000000001,-0.990000000000001,-0.985000000000001,-0.980000000000001,
-0.975000000000001,-0.970000000000001,-0.965000000000001,-0.960000000000001,
-0.955000000000001,-0.950000000000001,-0.945000000000001,-0.940000000000001,
-0.935000000000001,-0.930000000000001,-0.925000000000001,-0.920000000000001,
-0.915000000000001,-0.910000000000001,-0.905000000000001,-0.900000000000001,
-0.895000000000001,-0.890000000000001,-0.885000000000001,-0.880000000000001,
-0.875000000000001,-0.870000000000001,-0.865000000000001,-0.860000000000001,
-0.855000000000001,-0.850000000000001,-0.845000000000001,-0.840000000000001,
-0.835000000000001,-0.830000000000001,-0.825000000000001,-0.820000000000001,
-0.815000000000001,-0.810000000000001,-0.805000000000001,-0.800000000000001,
-0.795000000000001,-0.790000000000001,-0.785000000000001,-0.780000000000001,
-0.775000000000001,-0.770000000000001,-0.765000000000001,-0.760000000000001,
-0.755000000000001,-0.750000000000001,-0.745000000000001,-0.740000000000001,
-0.735000000000001,-0.730000000000001,-0.725000000000001,-0.720000000000001,
-0.715000000000001,-0.710000000000001,-0.705000000000001,-0.700000000000001,
-0.695000000000001,-0.690000000000001,-0.685,-0.68,-0.675,-0.67,-0.665,
-0.66,-0.655,-0.65,-0.645,-0.64,-0.635,-0.63,-0.625,-0.62,-0.615,-0.61,
-0.605,-0.6,-0.595,-0.59,-0.585,-0.58,-0.575,-0.57,-0.565,-0.56,-0.555,
-0.55,-0.545,-0.54,-0.535,-0.53,-0.525,-0.52,-0.515,-0.51,-0.505,-0.5,-0.495,
-0.49,-0.485,-0.48,-0.475,-0.47,-0.465,-0.46,-0.455,-0.45,-0.445,-0.44,
-0.435,-0.43,-0.425,-0.42,-0.415,-0.41,-0.405,-0.4,-0.395,-0.39,-0.385,
-0.38,-0.375,-0.37,-0.365,-0.36,-0.355,-0.35,-0.345,-0.34,-0.335,-0.33,
-0.325,-0.32,-0.315,-0.31,-0.305,-0.3,-0.295,-0.29,-0.285,-0.28,-0.275,
-0.27,-0.265,-0.26,-0.255,-0.25,-0.245,-0.24,-0.235,-0.23,-0.225,-0.22,
-0.215,-0.21,-0.205,-0.2,-0.195,-0.19,-0.185,-0.18,-0.175,-0.17,-0.165,
-0.16,-0.155,-0.15,-0.145,-0.14,-0.135,-0.13,-0.125,-0.12,-0.115,-0.11,
-0.105,-0.1,-0.095,-0.09,-0.085,-0.08,-0.075,-0.07,-0.065,-0.06,-0.055,
-0.05,-0.045,-0.04,-0.035,-0.03,-0.025,-0.02,-0.015,-0.01,-0.005,0.),
 .UNSPECIFIED.)
CURVE()
GEOMETRIC_REPRESENTATION_ITEM()
RATIONAL_B_SPLINE_CURVE((1.,1.,1.,1.,1.,1.,1.,1.,1.,1.,1.,1.,1.,1.,1.,1.,
1.,1.,1.,1.,1.,1.,1.,1.,1.,1.,1.,1.,1.,1.,1.,1.,1.,1.,1.,1.,1.,1.,1.,1.,
1.,1.,1.,1.,1.,1.,1.,1.,1.,1.,1.,1.,1.,1.,1.,1.,1.,1.,1.,1.,1.,1.,1.,1.,
1.,1.,1.,1.,1.,1.,1.,1.,1.,1.,1.,1.,1.,1.,1.,1.,1.,1.,1.,1.,1.,1.,1.,1.,
1.,1.,1.,1.,1.,1.,1.,1.,1.,1.,1.,1.,1.,1.,1.,1.,1.,1.,1.,1.,1.,1.,1.,1.,
1.,1.,1.,1.,1.,1.,1.,1.,1.,1.,1.,1.,1.,1.,1.,1.,1.,1.,1.,1.,1.,1.,1.,1.,
1.,1.,1.,1.,1.,1.,1.,1.,1.,1.,1.,1.,1.,1.,1.,1.,1.,1.,1.,1.,1.,1.,1.,1.,
1.,1.,1.,1.,1.,1.,1.,1.,1.,1.,1.,1.,1.,1.,1.,1.,1.,1.,1.,1.,1.,1.,1.,1.,
1.,1.,1.,1.,1.,1.,1.,1.,1.,1.,1.,1.,1.,1.,1.,1.,1.,1.,1.,1.,1.))
REPRESENTATION_ITEM('')
);
#723=(
BOUNDED_CURVE()
B_SPLINE_CURVE(5,(#181797,#181798,#181799,#181800,#181801,#181802,#181803,
#181804,#181805,#181806,#181807,#181808,#181809,#181810,#181811,#181812,
#181813,#181814,#181815,#181816,#181817,#181818,#181819,#181820,#181821,
#181822,#181823,#181824,#181825,#181826,#181827,#181828,#181829,#181830,
#181831,#181832,#181833,#181834,#181835,#181836,#181837,#181838,#181839,
#181840,#181841,#181842,#181843,#181844,#181845,#181846,#181847,#181848,
#181849,#181850,#181851,#181852,#181853,#181854,#181855,#181856,#181857,
#181858,#181859,#181860,#181861,#181862,#181863,#181864,#181865,#181866,
#181867,#181868,#181869,#181870,#181871,#181872,#181873,#181874,#181875,
#181876,#181877,#181878,#181879,#181880,#181881,#181882,#181883,#181884,
#181885,#181886,#181887,#181888,#181889,#181890,#181891,#181892,#181893,
#181894,#181895,#181896,#181897,#181898,#181899,#181900,#181901,#181902,
#181903,#181904,#181905,#181906,#181907,#181908,#181909,#181910,#181911,
#181912,#181913,#181914,#181915,#181916,#181917,#181918,#181919,#181920,
#181921,#181922,#181923,#181924,#181925,#181926,#181927,#181928,#181929,
#181930,#181931,#181932,#181933,#181934,#181935,#181936,#181937,#181938,
#181939,#181940,#181941,#181942,#181943,#181944,#181945,#181946,#181947,
#181948,#181949,#181950,#181951,#181952,#181953,#181954,#181955,#181956,
#181957,#181958,#181959,#181960,#181961,#181962,#181963,#181964,#181965,
#181966,#181967,#181968,#181969,#181970,#181971,#181972,#181973,#181974,
#181975,#181976,#181977,#181978,#181979,#181980,#181981,#181982,#181983,
#181984,#181985,#181986,#181987,#181988,#181989,#181990,#181991,#181992,
#181993,#181994,#181995,#181996,#181997,#181998,#181999,#182000,#182001),
 .UNSPECIFIED.,.F.,.F.)
B_SPLINE_CURVE_WITH_KNOTS((6,1,1,1,1,1,1,1,1,1,1,1,1,1,1,1,1,1,1,1,1,1,
1,1,1,1,1,1,1,1,1,1,1,1,1,1,1,1,1,1,1,1,1,1,1,1,1,1,1,1,1,1,1,1,1,1,1,1,
1,1,1,1,1,1,1,1,1,1,1,1,1,1,1,1,1,1,1,1,1,1,1,1,1,1,1,1,1,1,1,1,1,1,1,1,
1,1,1,1,1,1,1,1,1,1,1,1,1,1,1,1,1,1,1,1,1,1,1,1,1,1,1,1,1,1,1,1,1,1,1,1,
1,1,1,1,1,1,1,1,1,1,1,1,1,1,1,1,1,1,1,1,1,1,1,1,1,1,1,1,1,1,1,1,1,1,1,1,
1,1,1,1,1,1,1,1,1,1,1,1,1,1,1,1,1,1,1,1,1,1,1,1,1,1,1,1,1,1,1,1,1,1,6),
(0.,0.005,0.01,0.015,0.02,0.025,0.03,0.035,0.04,0.045,0.05,0.055,0.06,0.065,
0.07,0.075,0.08,0.085,0.09,0.095,0.1,0.105,0.11,0.115,0.12,0.125,0.13,0.135,
0.14,0.145,0.15,0.155,0.16,0.165,0.17,0.175,0.18,0.185,0.19,0.195,0.2,0.205,
0.21,0.215,0.22,0.225,0.23,0.235,0.24,0.245,0.25,0.255,0.26,0.265,0.27,
0.275,0.28,0.285,0.29,0.295,0.3,0.305,0.31,0.315,0.32,0.325,0.33,0.335,
0.34,0.345,0.35,0.355,0.36,0.365,0.37,0.375,0.38,0.385,0.39,0.395,0.4,0.405,
0.41,0.415,0.42,0.425,0.43,0.435,0.44,0.445,0.45,0.455,0.46,0.465,0.47,
0.475,0.48,0.485,0.49,0.495,0.5,0.505,0.51,0.515,0.52,0.525,0.53,0.535,
0.54,0.545,0.55,0.555,0.56,0.565,0.57,0.575,0.58,0.585,0.59,0.595,0.6,0.605,
0.61,0.615,0.62,0.625,0.63,0.635,0.64,0.645,0.65,0.655,0.66,0.665,0.67,
0.675,0.68,0.685,0.690000000000001,0.695000000000001,0.700000000000001,
0.705000000000001,0.710000000000001,0.715000000000001,0.720000000000001,
0.725000000000001,0.730000000000001,0.735000000000001,0.740000000000001,
0.745000000000001,0.750000000000001,0.755000000000001,0.760000000000001,
0.765000000000001,0.770000000000001,0.775000000000001,0.780000000000001,
0.785000000000001,0.790000000000001,0.795000000000001,0.800000000000001,
0.805000000000001,0.810000000000001,0.815000000000001,0.820000000000001,
0.825000000000001,0.830000000000001,0.835000000000001,0.840000000000001,
0.845000000000001,0.850000000000001,0.855000000000001,0.860000000000001,
0.865000000000001,0.870000000000001,0.875000000000001,0.880000000000001,
0.885000000000001,0.890000000000001,0.895000000000001,0.900000000000001,
0.905000000000001,0.910000000000001,0.915000000000001,0.920000000000001,
0.925000000000001,0.930000000000001,0.935000000000001,0.940000000000001,
0.945000000000001,0.950000000000001,0.955000000000001,0.960000000000001,
0.965000000000001,0.970000000000001,0.975000000000001,0.980000000000001,
0.985000000000001,0.990000000000001,0.995000000000001,1.),.UNSPECIFIED.)
CURVE()
GEOMETRIC_REPRESENTATION_ITEM()
RATIONAL_B_SPLINE_CURVE((1.,1.,1.,1.,1.,1.,1.,1.,1.,1.,1.,1.,1.,1.,1.,1.,
1.,1.,1.,1.,1.,1.,1.,1.,1.,1.,1.,1.,1.,1.,1.,1.,1.,1.,1.,1.,1.,1.,1.,1.,
1.,1.,1.,1.,1.,1.,1.,1.,1.,1.,1.,1.,1.,1.,1.,1.,1.,1.,1.,1.,1.,1.,1.,1.,
1.,1.,1.,1.,1.,1.,1.,1.,1.,1.,1.,1.,1.,1.,1.,1.,1.,1.,1.,1.,1.,1.,1.,1.,
1.,1.,1.,1.,1.,1.,1.,1.,1.,1.,1.,1.,1.,1.,1.,1.,1.,1.,1.,1.,1.,1.,1.,1.,
1.,1.,1.,1.,1.,1.,1.,1.,1.,1.,1.,1.,1.,1.,1.,1.,1.,1.,1.,1.,1.,1.,1.,1.,
1.,1.,1.,1.,1.,1.,1.,1.,1.,1.,1.,1.,1.,1.,1.,1.,1.,1.,1.,1.,1.,1.,1.,1.,
1.,1.,1.,1.,1.,1.,1.,1.,1.,1.,1.,1.,1.,1.,1.,1.,1.,1.,1.,1.,1.,1.,1.,1.,
1.,1.,1.,1.,1.,1.,1.,1.,1.,1.,1.,1.,1.,1.,1.,1.,1.,1.,1.,1.,1.))
REPRESENTATION_ITEM('')
);
#724=(
BOUNDED_CURVE()
B_SPLINE_CURVE(5,(#182005,#182006,#182007,#182008,#182009,#182010,#182011,
#182012,#182013,#182014,#182015,#182016,#182017,#182018,#182019,#182020,
#182021,#182022,#182023,#182024,#182025,#182026,#182027,#182028,#182029,
#182030,#182031,#182032,#182033,#182034,#182035,#182036,#182037,#182038,
#182039,#182040,#182041,#182042,#182043,#182044,#182045,#182046,#182047,
#182048,#182049,#182050,#182051,#182052,#182053,#182054,#182055,#182056,
#182057,#182058,#182059,#182060,#182061,#182062,#182063,#182064,#182065,
#182066,#182067,#182068,#182069,#182070,#182071,#182072,#182073,#182074,
#182075,#182076,#182077,#182078,#182079,#182080,#182081,#182082,#182083,
#182084,#182085,#182086,#182087,#182088,#182089,#182090,#182091,#182092,
#182093,#182094,#182095,#182096,#182097,#182098,#182099,#182100,#182101,
#182102,#182103,#182104,#182105,#182106,#182107,#182108,#182109,#182110,
#182111,#182112,#182113,#182114,#182115,#182116,#182117,#182118,#182119,
#182120,#182121,#182122,#182123,#182124,#182125,#182126,#182127,#182128,
#182129,#182130,#182131,#182132,#182133,#182134,#182135,#182136,#182137,
#182138,#182139,#182140,#182141,#182142,#182143,#182144,#182145,#182146,
#182147,#182148,#182149,#182150,#182151,#182152,#182153,#182154,#182155,
#182156,#182157,#182158,#182159,#182160,#182161,#182162,#182163,#182164,
#182165,#182166,#182167,#182168,#182169,#182170,#182171,#182172,#182173,
#182174,#182175,#182176,#182177,#182178,#182179,#182180,#182181,#182182,
#182183,#182184,#182185,#182186,#182187,#182188,#182189,#182190,#182191,
#182192,#182193,#182194,#182195,#182196,#182197,#182198,#182199,#182200,
#182201,#182202,#182203,#182204,#182205,#182206,#182207,#182208,#182209),
 .UNSPECIFIED.,.F.,.F.)
B_SPLINE_CURVE_WITH_KNOTS((6,1,1,1,1,1,1,1,1,1,1,1,1,1,1,1,1,1,1,1,1,1,
1,1,1,1,1,1,1,1,1,1,1,1,1,1,1,1,1,1,1,1,1,1,1,1,1,1,1,1,1,1,1,1,1,1,1,1,
1,1,1,1,1,1,1,1,1,1,1,1,1,1,1,1,1,1,1,1,1,1,1,1,1,1,1,1,1,1,1,1,1,1,1,1,
1,1,1,1,1,1,1,1,1,1,1,1,1,1,1,1,1,1,1,1,1,1,1,1,1,1,1,1,1,1,1,1,1,1,1,1,
1,1,1,1,1,1,1,1,1,1,1,1,1,1,1,1,1,1,1,1,1,1,1,1,1,1,1,1,1,1,1,1,1,1,1,1,
1,1,1,1,1,1,1,1,1,1,1,1,1,1,1,1,1,1,1,1,1,1,1,1,1,1,1,1,1,1,1,1,1,1,6),
(-1.,-0.995000000000001,-0.990000000000001,-0.985000000000001,-0.980000000000001,
-0.975000000000001,-0.970000000000001,-0.965000000000001,-0.960000000000001,
-0.955000000000001,-0.950000000000001,-0.945000000000001,-0.940000000000001,
-0.935000000000001,-0.930000000000001,-0.925000000000001,-0.920000000000001,
-0.915000000000001,-0.910000000000001,-0.905000000000001,-0.900000000000001,
-0.895000000000001,-0.890000000000001,-0.885000000000001,-0.880000000000001,
-0.875000000000001,-0.870000000000001,-0.865000000000001,-0.860000000000001,
-0.855000000000001,-0.850000000000001,-0.845000000000001,-0.840000000000001,
-0.835000000000001,-0.830000000000001,-0.825000000000001,-0.820000000000001,
-0.815000000000001,-0.810000000000001,-0.805000000000001,-0.800000000000001,
-0.795000000000001,-0.790000000000001,-0.785000000000001,-0.780000000000001,
-0.775000000000001,-0.770000000000001,-0.765000000000001,-0.760000000000001,
-0.755000000000001,-0.750000000000001,-0.745000000000001,-0.740000000000001,
-0.735000000000001,-0.730000000000001,-0.725000000000001,-0.720000000000001,
-0.715000000000001,-0.710000000000001,-0.705000000000001,-0.700000000000001,
-0.695000000000001,-0.690000000000001,-0.685,-0.68,-0.675,-0.67,-0.665,
-0.66,-0.655,-0.65,-0.645,-0.64,-0.635,-0.63,-0.625,-0.62,-0.615,-0.61,
-0.605,-0.6,-0.595,-0.59,-0.585,-0.58,-0.575,-0.57,-0.565,-0.56,-0.555,
-0.55,-0.545,-0.54,-0.535,-0.53,-0.525,-0.52,-0.515,-0.51,-0.505,-0.5,-0.495,
-0.49,-0.485,-0.48,-0.475,-0.47,-0.465,-0.46,-0.455,-0.45,-0.445,-0.44,
-0.435,-0.43,-0.425,-0.42,-0.415,-0.41,-0.405,-0.4,-0.395,-0.39,-0.385,
-0.38,-0.375,-0.37,-0.365,-0.36,-0.355,-0.35,-0.345,-0.34,-0.335,-0.33,
-0.325,-0.32,-0.315,-0.31,-0.305,-0.3,-0.295,-0.29,-0.285,-0.28,-0.275,
-0.27,-0.265,-0.26,-0.255,-0.25,-0.245,-0.24,-0.235,-0.23,-0.225,-0.22,
-0.215,-0.21,-0.205,-0.2,-0.195,-0.19,-0.185,-0.18,-0.175,-0.17,-0.165,
-0.16,-0.155,-0.15,-0.145,-0.14,-0.135,-0.13,-0.125,-0.12,-0.115,-0.11,
-0.105,-0.1,-0.095,-0.09,-0.085,-0.08,-0.075,-0.07,-0.065,-0.06,-0.055,
-0.05,-0.045,-0.04,-0.035,-0.03,-0.025,-0.02,-0.015,-0.01,-0.005,0.),
 .UNSPECIFIED.)
CURVE()
GEOMETRIC_REPRESENTATION_ITEM()
RATIONAL_B_SPLINE_CURVE((1.,1.,1.,1.,1.,1.,1.,1.,1.,1.,1.,1.,1.,1.,1.,1.,
1.,1.,1.,1.,1.,1.,1.,1.,1.,1.,1.,1.,1.,1.,1.,1.,1.,1.,1.,1.,1.,1.,1.,1.,
1.,1.,1.,1.,1.,1.,1.,1.,1.,1.,1.,1.,1.,1.,1.,1.,1.,1.,1.,1.,1.,1.,1.,1.,
1.,1.,1.,1.,1.,1.,1.,1.,1.,1.,1.,1.,1.,1.,1.,1.,1.,1.,1.,1.,1.,1.,1.,1.,
1.,1.,1.,1.,1.,1.,1.,1.,1.,1.,1.,1.,1.,1.,1.,1.,1.,1.,1.,1.,1.,1.,1.,1.,
1.,1.,1.,1.,1.,1.,1.,1.,1.,1.,1.,1.,1.,1.,1.,1.,1.,1.,1.,1.,1.,1.,1.,1.,
1.,1.,1.,1.,1.,1.,1.,1.,1.,1.,1.,1.,1.,1.,1.,1.,1.,1.,1.,1.,1.,1.,1.,1.,
1.,1.,1.,1.,1.,1.,1.,1.,1.,1.,1.,1.,1.,1.,1.,1.,1.,1.,1.,1.,1.,1.,1.,1.,
1.,1.,1.,1.,1.,1.,1.,1.,1.,1.,1.,1.,1.,1.,1.,1.,1.,1.,1.,1.,1.))
REPRESENTATION_ITEM('')
);
#725=(
BOUNDED_CURVE()
B_SPLINE_CURVE(5,(#182221,#182222,#182223,#182224,#182225,#182226,#182227,
#182228,#182229,#182230,#182231,#182232,#182233,#182234,#182235,#182236,
#182237,#182238,#182239,#182240,#182241,#182242,#182243,#182244,#182245,
#182246,#182247,#182248,#182249,#182250,#182251,#182252,#182253,#182254,
#182255,#182256,#182257,#182258,#182259,#182260,#182261,#182262,#182263,
#182264,#182265,#182266,#182267,#182268,#182269,#182270,#182271,#182272,
#182273,#182274,#182275,#182276,#182277,#182278,#182279,#182280,#182281,
#182282,#182283,#182284,#182285,#182286,#182287,#182288,#182289,#182290,
#182291,#182292,#182293,#182294,#182295,#182296,#182297,#182298,#182299,
#182300,#182301,#182302,#182303,#182304,#182305,#182306,#182307,#182308,
#182309,#182310,#182311,#182312,#182313,#182314,#182315,#182316,#182317,
#182318,#182319,#182320,#182321,#182322,#182323,#182324,#182325,#182326,
#182327,#182328,#182329,#182330,#182331,#182332,#182333,#182334,#182335,
#182336,#182337,#182338,#182339,#182340,#182341,#182342,#182343,#182344,
#182345,#182346,#182347,#182348,#182349,#182350,#182351,#182352,#182353,
#182354,#182355,#182356,#182357,#182358,#182359,#182360,#182361,#182362,
#182363,#182364,#182365,#182366,#182367,#182368,#182369,#182370,#182371,
#182372,#182373,#182374,#182375,#182376,#182377,#182378,#182379,#182380,
#182381,#182382,#182383,#182384,#182385,#182386,#182387,#182388,#182389,
#182390,#182391,#182392,#182393,#182394,#182395,#182396,#182397,#182398,
#182399,#182400,#182401,#182402,#182403,#182404,#182405,#182406,#182407,
#182408,#182409,#182410,#182411,#182412,#182413,#182414,#182415,#182416,
#182417,#182418,#182419,#182420,#182421,#182422,#182423,#182424,#182425),
 .UNSPECIFIED.,.F.,.F.)
B_SPLINE_CURVE_WITH_KNOTS((6,1,1,1,1,1,1,1,1,1,1,1,1,1,1,1,1,1,1,1,1,1,
1,1,1,1,1,1,1,1,1,1,1,1,1,1,1,1,1,1,1,1,1,1,1,1,1,1,1,1,1,1,1,1,1,1,1,1,
1,1,1,1,1,1,1,1,1,1,1,1,1,1,1,1,1,1,1,1,1,1,1,1,1,1,1,1,1,1,1,1,1,1,1,1,
1,1,1,1,1,1,1,1,1,1,1,1,1,1,1,1,1,1,1,1,1,1,1,1,1,1,1,1,1,1,1,1,1,1,1,1,
1,1,1,1,1,1,1,1,1,1,1,1,1,1,1,1,1,1,1,1,1,1,1,1,1,1,1,1,1,1,1,1,1,1,1,1,
1,1,1,1,1,1,1,1,1,1,1,1,1,1,1,1,1,1,1,1,1,1,1,1,1,1,1,1,1,1,1,1,1,1,6),
(0.,0.005,0.01,0.015,0.02,0.025,0.03,0.035,0.04,0.045,0.05,0.055,0.06,0.065,
0.07,0.075,0.08,0.085,0.09,0.095,0.1,0.105,0.11,0.115,0.12,0.125,0.13,0.135,
0.14,0.145,0.15,0.155,0.16,0.165,0.17,0.175,0.18,0.185,0.19,0.195,0.2,0.205,
0.21,0.215,0.22,0.225,0.23,0.235,0.24,0.245,0.25,0.255,0.26,0.265,0.27,
0.275,0.28,0.285,0.29,0.295,0.3,0.305,0.31,0.315,0.32,0.325,0.33,0.335,
0.34,0.345,0.35,0.355,0.36,0.365,0.37,0.375,0.38,0.385,0.39,0.395,0.4,0.405,
0.41,0.415,0.42,0.425,0.43,0.435,0.44,0.445,0.45,0.455,0.46,0.465,0.47,
0.475,0.48,0.485,0.49,0.495,0.5,0.505,0.51,0.515,0.52,0.525,0.53,0.535,
0.54,0.545,0.55,0.555,0.56,0.565,0.57,0.575,0.58,0.585,0.59,0.595,0.6,0.605,
0.61,0.615,0.62,0.625,0.63,0.635,0.64,0.645,0.65,0.655,0.66,0.665,0.67,
0.675,0.68,0.685,0.690000000000001,0.695000000000001,0.700000000000001,
0.705000000000001,0.710000000000001,0.715000000000001,0.720000000000001,
0.725000000000001,0.730000000000001,0.735000000000001,0.740000000000001,
0.745000000000001,0.750000000000001,0.755000000000001,0.760000000000001,
0.765000000000001,0.770000000000001,0.775000000000001,0.780000000000001,
0.785000000000001,0.790000000000001,0.795000000000001,0.800000000000001,
0.805000000000001,0.810000000000001,0.815000000000001,0.820000000000001,
0.825000000000001,0.830000000000001,0.835000000000001,0.840000000000001,
0.845000000000001,0.850000000000001,0.855000000000001,0.860000000000001,
0.865000000000001,0.870000000000001,0.875000000000001,0.880000000000001,
0.885000000000001,0.890000000000001,0.895000000000001,0.900000000000001,
0.905000000000001,0.910000000000001,0.915000000000001,0.920000000000001,
0.925000000000001,0.930000000000001,0.935000000000001,0.940000000000001,
0.945000000000001,0.950000000000001,0.955000000000001,0.960000000000001,
0.965000000000001,0.970000000000001,0.975000000000001,0.980000000000001,
0.985000000000001,0.990000000000001,0.995000000000001,1.),.UNSPECIFIED.)
CURVE()
GEOMETRIC_REPRESENTATION_ITEM()
RATIONAL_B_SPLINE_CURVE((1.,1.,1.,1.,1.,1.,1.,1.,1.,1.,1.,1.,1.,1.,1.,1.,
1.,1.,1.,1.,1.,1.,1.,1.,1.,1.,1.,1.,1.,1.,1.,1.,1.,1.,1.,1.,1.,1.,1.,1.,
1.,1.,1.,1.,1.,1.,1.,1.,1.,1.,1.,1.,1.,1.,1.,1.,1.,1.,1.,1.,1.,1.,1.,1.,
1.,1.,1.,1.,1.,1.,1.,1.,1.,1.,1.,1.,1.,1.,1.,1.,1.,1.,1.,1.,1.,1.,1.,1.,
1.,1.,1.,1.,1.,1.,1.,1.,1.,1.,1.,1.,1.,1.,1.,1.,1.,1.,1.,1.,1.,1.,1.,1.,
1.,1.,1.,1.,1.,1.,1.,1.,1.,1.,1.,1.,1.,1.,1.,1.,1.,1.,1.,1.,1.,1.,1.,1.,
1.,1.,1.,1.,1.,1.,1.,1.,1.,1.,1.,1.,1.,1.,1.,1.,1.,1.,1.,1.,1.,1.,1.,1.,
1.,1.,1.,1.,1.,1.,1.,1.,1.,1.,1.,1.,1.,1.,1.,1.,1.,1.,1.,1.,1.,1.,1.,1.,
1.,1.,1.,1.,1.,1.,1.,1.,1.,1.,1.,1.,1.,1.,1.,1.,1.,1.,1.,1.,1.))
REPRESENTATION_ITEM('')
);
#726=(
BOUNDED_CURVE()
B_SPLINE_CURVE(5,(#182429,#182430,#182431,#182432,#182433,#182434,#182435,
#182436,#182437,#182438,#182439,#182440,#182441,#182442,#182443,#182444,
#182445,#182446,#182447,#182448,#182449,#182450,#182451,#182452,#182453,
#182454,#182455,#182456,#182457,#182458,#182459,#182460,#182461,#182462,
#182463,#182464,#182465,#182466,#182467,#182468,#182469,#182470,#182471,
#182472,#182473,#182474,#182475,#182476,#182477,#182478,#182479,#182480,
#182481,#182482,#182483,#182484,#182485,#182486,#182487,#182488,#182489,
#182490,#182491,#182492,#182493,#182494,#182495,#182496,#182497,#182498,
#182499,#182500,#182501,#182502,#182503,#182504,#182505,#182506,#182507,
#182508,#182509,#182510,#182511,#182512,#182513,#182514,#182515,#182516,
#182517,#182518,#182519,#182520,#182521,#182522,#182523,#182524,#182525,
#182526,#182527,#182528,#182529,#182530,#182531,#182532,#182533,#182534,
#182535,#182536,#182537,#182538,#182539,#182540,#182541,#182542,#182543,
#182544,#182545,#182546,#182547,#182548,#182549,#182550,#182551,#182552,
#182553,#182554,#182555,#182556,#182557,#182558,#182559,#182560,#182561,
#182562,#182563,#182564,#182565,#182566,#182567,#182568,#182569,#182570,
#182571,#182572,#182573,#182574,#182575,#182576,#182577,#182578,#182579,
#182580,#182581,#182582,#182583,#182584,#182585,#182586,#182587,#182588,
#182589,#182590,#182591,#182592,#182593,#182594,#182595,#182596,#182597,
#182598,#182599,#182600,#182601,#182602,#182603,#182604,#182605,#182606,
#182607,#182608,#182609,#182610,#182611,#182612,#182613,#182614,#182615,
#182616,#182617,#182618,#182619,#182620,#182621,#182622,#182623,#182624,
#182625,#182626,#182627,#182628,#182629,#182630,#182631,#182632,#182633),
 .UNSPECIFIED.,.F.,.F.)
B_SPLINE_CURVE_WITH_KNOTS((6,1,1,1,1,1,1,1,1,1,1,1,1,1,1,1,1,1,1,1,1,1,
1,1,1,1,1,1,1,1,1,1,1,1,1,1,1,1,1,1,1,1,1,1,1,1,1,1,1,1,1,1,1,1,1,1,1,1,
1,1,1,1,1,1,1,1,1,1,1,1,1,1,1,1,1,1,1,1,1,1,1,1,1,1,1,1,1,1,1,1,1,1,1,1,
1,1,1,1,1,1,1,1,1,1,1,1,1,1,1,1,1,1,1,1,1,1,1,1,1,1,1,1,1,1,1,1,1,1,1,1,
1,1,1,1,1,1,1,1,1,1,1,1,1,1,1,1,1,1,1,1,1,1,1,1,1,1,1,1,1,1,1,1,1,1,1,1,
1,1,1,1,1,1,1,1,1,1,1,1,1,1,1,1,1,1,1,1,1,1,1,1,1,1,1,1,1,1,1,1,1,1,6),
(-1.,-0.995000000000001,-0.990000000000001,-0.985000000000001,-0.980000000000001,
-0.975000000000001,-0.970000000000001,-0.965000000000001,-0.960000000000001,
-0.955000000000001,-0.950000000000001,-0.945000000000001,-0.940000000000001,
-0.935000000000001,-0.930000000000001,-0.925000000000001,-0.920000000000001,
-0.915000000000001,-0.910000000000001,-0.905000000000001,-0.900000000000001,
-0.895000000000001,-0.890000000000001,-0.885000000000001,-0.880000000000001,
-0.875000000000001,-0.870000000000001,-0.865000000000001,-0.860000000000001,
-0.855000000000001,-0.850000000000001,-0.845000000000001,-0.840000000000001,
-0.835000000000001,-0.830000000000001,-0.825000000000001,-0.820000000000001,
-0.815000000000001,-0.810000000000001,-0.805000000000001,-0.800000000000001,
-0.795000000000001,-0.790000000000001,-0.785000000000001,-0.780000000000001,
-0.775000000000001,-0.770000000000001,-0.765000000000001,-0.760000000000001,
-0.755000000000001,-0.750000000000001,-0.745000000000001,-0.740000000000001,
-0.735000000000001,-0.730000000000001,-0.725000000000001,-0.720000000000001,
-0.715000000000001,-0.710000000000001,-0.705000000000001,-0.700000000000001,
-0.695000000000001,-0.690000000000001,-0.685,-0.68,-0.675,-0.67,-0.665,
-0.66,-0.655,-0.65,-0.645,-0.64,-0.635,-0.63,-0.625,-0.62,-0.615,-0.61,
-0.605,-0.6,-0.595,-0.59,-0.585,-0.58,-0.575,-0.57,-0.565,-0.56,-0.555,
-0.55,-0.545,-0.54,-0.535,-0.53,-0.525,-0.52,-0.515,-0.51,-0.505,-0.5,-0.495,
-0.49,-0.485,-0.48,-0.475,-0.47,-0.465,-0.46,-0.455,-0.45,-0.445,-0.44,
-0.435,-0.43,-0.425,-0.42,-0.415,-0.41,-0.405,-0.4,-0.395,-0.39,-0.385,
-0.38,-0.375,-0.37,-0.365,-0.36,-0.355,-0.35,-0.345,-0.34,-0.335,-0.33,
-0.325,-0.32,-0.315,-0.31,-0.305,-0.3,-0.295,-0.29,-0.285,-0.28,-0.275,
-0.27,-0.265,-0.26,-0.255,-0.25,-0.245,-0.24,-0.235,-0.23,-0.225,-0.22,
-0.215,-0.21,-0.205,-0.2,-0.195,-0.19,-0.185,-0.18,-0.175,-0.17,-0.165,
-0.16,-0.155,-0.15,-0.145,-0.14,-0.135,-0.13,-0.125,-0.12,-0.115,-0.11,
-0.105,-0.1,-0.095,-0.09,-0.085,-0.08,-0.075,-0.07,-0.065,-0.06,-0.055,
-0.05,-0.045,-0.04,-0.035,-0.03,-0.025,-0.02,-0.015,-0.01,-0.005,0.),
 .UNSPECIFIED.)
CURVE()
GEOMETRIC_REPRESENTATION_ITEM()
RATIONAL_B_SPLINE_CURVE((1.,1.,1.,1.,1.,1.,1.,1.,1.,1.,1.,1.,1.,1.,1.,1.,
1.,1.,1.,1.,1.,1.,1.,1.,1.,1.,1.,1.,1.,1.,1.,1.,1.,1.,1.,1.,1.,1.,1.,1.,
1.,1.,1.,1.,1.,1.,1.,1.,1.,1.,1.,1.,1.,1.,1.,1.,1.,1.,1.,1.,1.,1.,1.,1.,
1.,1.,1.,1.,1.,1.,1.,1.,1.,1.,1.,1.,1.,1.,1.,1.,1.,1.,1.,1.,1.,1.,1.,1.,
1.,1.,1.,1.,1.,1.,1.,1.,1.,1.,1.,1.,1.,1.,1.,1.,1.,1.,1.,1.,1.,1.,1.,1.,
1.,1.,1.,1.,1.,1.,1.,1.,1.,1.,1.,1.,1.,1.,1.,1.,1.,1.,1.,1.,1.,1.,1.,1.,
1.,1.,1.,1.,1.,1.,1.,1.,1.,1.,1.,1.,1.,1.,1.,1.,1.,1.,1.,1.,1.,1.,1.,1.,
1.,1.,1.,1.,1.,1.,1.,1.,1.,1.,1.,1.,1.,1.,1.,1.,1.,1.,1.,1.,1.,1.,1.,1.,
1.,1.,1.,1.,1.,1.,1.,1.,1.,1.,1.,1.,1.,1.,1.,1.,1.,1.,1.,1.,1.))
REPRESENTATION_ITEM('')
);
#727=(
BOUNDED_CURVE()
B_SPLINE_CURVE(5,(#182645,#182646,#182647,#182648,#182649,#182650,#182651,
#182652,#182653,#182654,#182655,#182656,#182657,#182658,#182659,#182660,
#182661,#182662,#182663,#182664,#182665,#182666,#182667,#182668,#182669,
#182670,#182671,#182672,#182673,#182674,#182675,#182676,#182677,#182678,
#182679,#182680,#182681,#182682,#182683,#182684,#182685,#182686,#182687,
#182688,#182689,#182690,#182691,#182692,#182693,#182694,#182695,#182696,
#182697,#182698,#182699,#182700,#182701,#182702,#182703,#182704,#182705,
#182706,#182707,#182708,#182709,#182710,#182711,#182712,#182713,#182714,
#182715,#182716,#182717,#182718,#182719,#182720,#182721,#182722,#182723,
#182724,#182725,#182726,#182727,#182728,#182729,#182730,#182731,#182732,
#182733,#182734,#182735,#182736,#182737,#182738,#182739,#182740,#182741,
#182742,#182743,#182744,#182745,#182746,#182747,#182748,#182749,#182750,
#182751,#182752,#182753,#182754,#182755,#182756,#182757,#182758,#182759,
#182760,#182761,#182762,#182763,#182764,#182765,#182766,#182767,#182768,
#182769,#182770,#182771,#182772,#182773,#182774,#182775,#182776,#182777,
#182778,#182779,#182780,#182781,#182782,#182783,#182784,#182785,#182786,
#182787,#182788,#182789,#182790,#182791,#182792,#182793,#182794,#182795,
#182796,#182797,#182798,#182799,#182800,#182801,#182802,#182803,#182804,
#182805,#182806,#182807,#182808,#182809,#182810,#182811,#182812,#182813,
#182814,#182815,#182816,#182817,#182818,#182819,#182820,#182821,#182822,
#182823,#182824,#182825,#182826,#182827,#182828,#182829,#182830,#182831,
#182832,#182833,#182834,#182835,#182836,#182837,#182838,#182839,#182840,
#182841,#182842,#182843,#182844,#182845,#182846,#182847,#182848,#182849),
 .UNSPECIFIED.,.F.,.F.)
B_SPLINE_CURVE_WITH_KNOTS((6,1,1,1,1,1,1,1,1,1,1,1,1,1,1,1,1,1,1,1,1,1,
1,1,1,1,1,1,1,1,1,1,1,1,1,1,1,1,1,1,1,1,1,1,1,1,1,1,1,1,1,1,1,1,1,1,1,1,
1,1,1,1,1,1,1,1,1,1,1,1,1,1,1,1,1,1,1,1,1,1,1,1,1,1,1,1,1,1,1,1,1,1,1,1,
1,1,1,1,1,1,1,1,1,1,1,1,1,1,1,1,1,1,1,1,1,1,1,1,1,1,1,1,1,1,1,1,1,1,1,1,
1,1,1,1,1,1,1,1,1,1,1,1,1,1,1,1,1,1,1,1,1,1,1,1,1,1,1,1,1,1,1,1,1,1,1,1,
1,1,1,1,1,1,1,1,1,1,1,1,1,1,1,1,1,1,1,1,1,1,1,1,1,1,1,1,1,1,1,1,1,1,6),
(0.,0.005,0.01,0.015,0.02,0.025,0.03,0.035,0.04,0.045,0.05,0.055,0.06,0.065,
0.07,0.075,0.08,0.085,0.09,0.095,0.1,0.105,0.11,0.115,0.12,0.125,0.13,0.135,
0.14,0.145,0.15,0.155,0.16,0.165,0.17,0.175,0.18,0.185,0.19,0.195,0.2,0.205,
0.21,0.215,0.22,0.225,0.23,0.235,0.24,0.245,0.25,0.255,0.26,0.265,0.27,
0.275,0.28,0.285,0.29,0.295,0.3,0.305,0.31,0.315,0.32,0.325,0.33,0.335,
0.34,0.345,0.35,0.355,0.36,0.365,0.37,0.375,0.38,0.385,0.39,0.395,0.4,0.405,
0.41,0.415,0.42,0.425,0.43,0.435,0.44,0.445,0.45,0.455,0.46,0.465,0.47,
0.475,0.48,0.485,0.49,0.495,0.5,0.505,0.51,0.515,0.52,0.525,0.53,0.535,
0.54,0.545,0.55,0.555,0.56,0.565,0.57,0.575,0.58,0.585,0.59,0.595,0.6,0.605,
0.61,0.615,0.62,0.625,0.63,0.635,0.64,0.645,0.65,0.655,0.66,0.665,0.67,
0.675,0.68,0.685,0.690000000000001,0.695000000000001,0.700000000000001,
0.705000000000001,0.710000000000001,0.715000000000001,0.720000000000001,
0.725000000000001,0.730000000000001,0.735000000000001,0.740000000000001,
0.745000000000001,0.750000000000001,0.755000000000001,0.760000000000001,
0.765000000000001,0.770000000000001,0.775000000000001,0.780000000000001,
0.785000000000001,0.790000000000001,0.795000000000001,0.800000000000001,
0.805000000000001,0.810000000000001,0.815000000000001,0.820000000000001,
0.825000000000001,0.830000000000001,0.835000000000001,0.840000000000001,
0.845000000000001,0.850000000000001,0.855000000000001,0.860000000000001,
0.865000000000001,0.870000000000001,0.875000000000001,0.880000000000001,
0.885000000000001,0.890000000000001,0.895000000000001,0.900000000000001,
0.905000000000001,0.910000000000001,0.915000000000001,0.920000000000001,
0.925000000000001,0.930000000000001,0.935000000000001,0.940000000000001,
0.945000000000001,0.950000000000001,0.955000000000001,0.960000000000001,
0.965000000000001,0.970000000000001,0.975000000000001,0.980000000000001,
0.985000000000001,0.990000000000001,0.995000000000001,1.),.UNSPECIFIED.)
CURVE()
GEOMETRIC_REPRESENTATION_ITEM()
RATIONAL_B_SPLINE_CURVE((1.,1.,1.,1.,1.,1.,1.,1.,1.,1.,1.,1.,1.,1.,1.,1.,
1.,1.,1.,1.,1.,1.,1.,1.,1.,1.,1.,1.,1.,1.,1.,1.,1.,1.,1.,1.,1.,1.,1.,1.,
1.,1.,1.,1.,1.,1.,1.,1.,1.,1.,1.,1.,1.,1.,1.,1.,1.,1.,1.,1.,1.,1.,1.,1.,
1.,1.,1.,1.,1.,1.,1.,1.,1.,1.,1.,1.,1.,1.,1.,1.,1.,1.,1.,1.,1.,1.,1.,1.,
1.,1.,1.,1.,1.,1.,1.,1.,1.,1.,1.,1.,1.,1.,1.,1.,1.,1.,1.,1.,1.,1.,1.,1.,
1.,1.,1.,1.,1.,1.,1.,1.,1.,1.,1.,1.,1.,1.,1.,1.,1.,1.,1.,1.,1.,1.,1.,1.,
1.,1.,1.,1.,1.,1.,1.,1.,1.,1.,1.,1.,1.,1.,1.,1.,1.,1.,1.,1.,1.,1.,1.,1.,
1.,1.,1.,1.,1.,1.,1.,1.,1.,1.,1.,1.,1.,1.,1.,1.,1.,1.,1.,1.,1.,1.,1.,1.,
1.,1.,1.,1.,1.,1.,1.,1.,1.,1.,1.,1.,1.,1.,1.,1.,1.,1.,1.,1.,1.))
REPRESENTATION_ITEM('')
);
#728=(
BOUNDED_CURVE()
B_SPLINE_CURVE(5,(#182853,#182854,#182855,#182856,#182857,#182858,#182859,
#182860,#182861,#182862,#182863,#182864,#182865,#182866,#182867,#182868,
#182869,#182870,#182871,#182872,#182873,#182874,#182875,#182876,#182877,
#182878,#182879,#182880,#182881,#182882,#182883,#182884,#182885,#182886,
#182887,#182888,#182889,#182890,#182891,#182892,#182893,#182894,#182895,
#182896,#182897,#182898,#182899,#182900,#182901,#182902,#182903,#182904,
#182905,#182906,#182907,#182908,#182909,#182910,#182911,#182912,#182913,
#182914,#182915,#182916,#182917,#182918,#182919,#182920,#182921,#182922,
#182923,#182924,#182925,#182926,#182927,#182928,#182929,#182930,#182931,
#182932,#182933,#182934,#182935,#182936,#182937,#182938,#182939,#182940,
#182941,#182942,#182943,#182944,#182945,#182946,#182947,#182948,#182949,
#182950,#182951,#182952,#182953,#182954,#182955,#182956,#182957,#182958,
#182959,#182960,#182961,#182962,#182963,#182964,#182965,#182966,#182967,
#182968,#182969,#182970,#182971,#182972,#182973,#182974,#182975,#182976,
#182977,#182978,#182979,#182980,#182981,#182982,#182983,#182984,#182985,
#182986,#182987,#182988,#182989,#182990,#182991,#182992,#182993,#182994,
#182995,#182996,#182997,#182998,#182999,#183000,#183001,#183002,#183003,
#183004,#183005,#183006,#183007,#183008,#183009,#183010,#183011,#183012,
#183013,#183014,#183015,#183016,#183017,#183018,#183019,#183020,#183021,
#183022,#183023,#183024,#183025,#183026,#183027,#183028,#183029,#183030,
#183031,#183032,#183033,#183034,#183035,#183036,#183037,#183038,#183039,
#183040,#183041,#183042,#183043,#183044,#183045,#183046,#183047,#183048,
#183049,#183050,#183051,#183052,#183053,#183054,#183055,#183056,#183057),
 .UNSPECIFIED.,.F.,.F.)
B_SPLINE_CURVE_WITH_KNOTS((6,1,1,1,1,1,1,1,1,1,1,1,1,1,1,1,1,1,1,1,1,1,
1,1,1,1,1,1,1,1,1,1,1,1,1,1,1,1,1,1,1,1,1,1,1,1,1,1,1,1,1,1,1,1,1,1,1,1,
1,1,1,1,1,1,1,1,1,1,1,1,1,1,1,1,1,1,1,1,1,1,1,1,1,1,1,1,1,1,1,1,1,1,1,1,
1,1,1,1,1,1,1,1,1,1,1,1,1,1,1,1,1,1,1,1,1,1,1,1,1,1,1,1,1,1,1,1,1,1,1,1,
1,1,1,1,1,1,1,1,1,1,1,1,1,1,1,1,1,1,1,1,1,1,1,1,1,1,1,1,1,1,1,1,1,1,1,1,
1,1,1,1,1,1,1,1,1,1,1,1,1,1,1,1,1,1,1,1,1,1,1,1,1,1,1,1,1,1,1,1,1,1,6),
(-1.,-0.995000000000001,-0.990000000000001,-0.985000000000001,-0.980000000000001,
-0.975000000000001,-0.970000000000001,-0.965000000000001,-0.960000000000001,
-0.955000000000001,-0.950000000000001,-0.945000000000001,-0.940000000000001,
-0.935000000000001,-0.930000000000001,-0.925000000000001,-0.920000000000001,
-0.915000000000001,-0.910000000000001,-0.905000000000001,-0.900000000000001,
-0.895000000000001,-0.890000000000001,-0.885000000000001,-0.880000000000001,
-0.875000000000001,-0.870000000000001,-0.865000000000001,-0.860000000000001,
-0.855000000000001,-0.850000000000001,-0.845000000000001,-0.840000000000001,
-0.835000000000001,-0.830000000000001,-0.825000000000001,-0.820000000000001,
-0.815000000000001,-0.810000000000001,-0.805000000000001,-0.800000000000001,
-0.795000000000001,-0.790000000000001,-0.785000000000001,-0.780000000000001,
-0.775000000000001,-0.770000000000001,-0.765000000000001,-0.760000000000001,
-0.755000000000001,-0.750000000000001,-0.745000000000001,-0.740000000000001,
-0.735000000000001,-0.730000000000001,-0.725000000000001,-0.720000000000001,
-0.715000000000001,-0.710000000000001,-0.705000000000001,-0.700000000000001,
-0.695000000000001,-0.690000000000001,-0.685,-0.68,-0.675,-0.67,-0.665,
-0.66,-0.655,-0.65,-0.645,-0.64,-0.635,-0.63,-0.625,-0.62,-0.615,-0.61,
-0.605,-0.6,-0.595,-0.59,-0.585,-0.58,-0.575,-0.57,-0.565,-0.56,-0.555,
-0.55,-0.545,-0.54,-0.535,-0.53,-0.525,-0.52,-0.515,-0.51,-0.505,-0.5,-0.495,
-0.49,-0.485,-0.48,-0.475,-0.47,-0.465,-0.46,-0.455,-0.45,-0.445,-0.44,
-0.435,-0.43,-0.425,-0.42,-0.415,-0.41,-0.405,-0.4,-0.395,-0.39,-0.385,
-0.38,-0.375,-0.37,-0.365,-0.36,-0.355,-0.35,-0.345,-0.34,-0.335,-0.33,
-0.325,-0.32,-0.315,-0.31,-0.305,-0.3,-0.295,-0.29,-0.285,-0.28,-0.275,
-0.27,-0.265,-0.26,-0.255,-0.25,-0.245,-0.24,-0.235,-0.23,-0.225,-0.22,
-0.215,-0.21,-0.205,-0.2,-0.195,-0.19,-0.185,-0.18,-0.175,-0.17,-0.165,
-0.16,-0.155,-0.15,-0.145,-0.14,-0.135,-0.13,-0.125,-0.12,-0.115,-0.11,
-0.105,-0.1,-0.095,-0.09,-0.085,-0.08,-0.075,-0.07,-0.065,-0.06,-0.055,
-0.05,-0.045,-0.04,-0.035,-0.03,-0.025,-0.02,-0.015,-0.01,-0.005,0.),
 .UNSPECIFIED.)
CURVE()
GEOMETRIC_REPRESENTATION_ITEM()
RATIONAL_B_SPLINE_CURVE((1.,1.,1.,1.,1.,1.,1.,1.,1.,1.,1.,1.,1.,1.,1.,1.,
1.,1.,1.,1.,1.,1.,1.,1.,1.,1.,1.,1.,1.,1.,1.,1.,1.,1.,1.,1.,1.,1.,1.,1.,
1.,1.,1.,1.,1.,1.,1.,1.,1.,1.,1.,1.,1.,1.,1.,1.,1.,1.,1.,1.,1.,1.,1.,1.,
1.,1.,1.,1.,1.,1.,1.,1.,1.,1.,1.,1.,1.,1.,1.,1.,1.,1.,1.,1.,1.,1.,1.,1.,
1.,1.,1.,1.,1.,1.,1.,1.,1.,1.,1.,1.,1.,1.,1.,1.,1.,1.,1.,1.,1.,1.,1.,1.,
1.,1.,1.,1.,1.,1.,1.,1.,1.,1.,1.,1.,1.,1.,1.,1.,1.,1.,1.,1.,1.,1.,1.,1.,
1.,1.,1.,1.,1.,1.,1.,1.,1.,1.,1.,1.,1.,1.,1.,1.,1.,1.,1.,1.,1.,1.,1.,1.,
1.,1.,1.,1.,1.,1.,1.,1.,1.,1.,1.,1.,1.,1.,1.,1.,1.,1.,1.,1.,1.,1.,1.,1.,
1.,1.,1.,1.,1.,1.,1.,1.,1.,1.,1.,1.,1.,1.,1.,1.,1.,1.,1.,1.,1.))
REPRESENTATION_ITEM('')
);
#729=(
BOUNDED_CURVE()
B_SPLINE_CURVE(5,(#183069,#183070,#183071,#183072,#183073,#183074,#183075,
#183076,#183077,#183078,#183079,#183080,#183081,#183082,#183083,#183084,
#183085,#183086,#183087,#183088,#183089,#183090,#183091,#183092,#183093,
#183094,#183095,#183096,#183097,#183098,#183099,#183100,#183101,#183102,
#183103,#183104,#183105,#183106,#183107,#183108,#183109,#183110,#183111,
#183112,#183113,#183114,#183115,#183116,#183117,#183118,#183119,#183120,
#183121,#183122,#183123,#183124,#183125,#183126,#183127,#183128,#183129,
#183130,#183131,#183132,#183133,#183134,#183135,#183136,#183137,#183138,
#183139,#183140,#183141,#183142,#183143,#183144,#183145,#183146,#183147,
#183148,#183149,#183150,#183151,#183152,#183153,#183154,#183155,#183156,
#183157,#183158,#183159,#183160,#183161,#183162,#183163,#183164,#183165,
#183166,#183167,#183168,#183169,#183170,#183171,#183172,#183173,#183174,
#183175,#183176,#183177,#183178,#183179,#183180,#183181,#183182,#183183,
#183184,#183185,#183186,#183187,#183188,#183189,#183190,#183191,#183192,
#183193,#183194,#183195,#183196,#183197,#183198,#183199,#183200,#183201,
#183202,#183203,#183204,#183205,#183206,#183207,#183208,#183209,#183210,
#183211,#183212,#183213,#183214,#183215,#183216,#183217,#183218,#183219,
#183220,#183221,#183222,#183223,#183224,#183225,#183226,#183227,#183228,
#183229,#183230,#183231,#183232,#183233,#183234,#183235,#183236,#183237,
#183238,#183239,#183240,#183241,#183242,#183243,#183244,#183245,#183246,
#183247,#183248,#183249,#183250,#183251,#183252,#183253,#183254,#183255,
#183256,#183257,#183258,#183259,#183260,#183261,#183262,#183263,#183264,
#183265,#183266,#183267,#183268,#183269,#183270,#183271,#183272,#183273),
 .UNSPECIFIED.,.F.,.F.)
B_SPLINE_CURVE_WITH_KNOTS((6,1,1,1,1,1,1,1,1,1,1,1,1,1,1,1,1,1,1,1,1,1,
1,1,1,1,1,1,1,1,1,1,1,1,1,1,1,1,1,1,1,1,1,1,1,1,1,1,1,1,1,1,1,1,1,1,1,1,
1,1,1,1,1,1,1,1,1,1,1,1,1,1,1,1,1,1,1,1,1,1,1,1,1,1,1,1,1,1,1,1,1,1,1,1,
1,1,1,1,1,1,1,1,1,1,1,1,1,1,1,1,1,1,1,1,1,1,1,1,1,1,1,1,1,1,1,1,1,1,1,1,
1,1,1,1,1,1,1,1,1,1,1,1,1,1,1,1,1,1,1,1,1,1,1,1,1,1,1,1,1,1,1,1,1,1,1,1,
1,1,1,1,1,1,1,1,1,1,1,1,1,1,1,1,1,1,1,1,1,1,1,1,1,1,1,1,1,1,1,1,1,1,6),
(0.,0.005,0.01,0.015,0.02,0.025,0.03,0.035,0.04,0.045,0.05,0.055,0.06,0.065,
0.07,0.075,0.08,0.085,0.09,0.095,0.1,0.105,0.11,0.115,0.12,0.125,0.13,0.135,
0.14,0.145,0.15,0.155,0.16,0.165,0.17,0.175,0.18,0.185,0.19,0.195,0.2,0.205,
0.21,0.215,0.22,0.225,0.23,0.235,0.24,0.245,0.25,0.255,0.26,0.265,0.27,
0.275,0.28,0.285,0.29,0.295,0.3,0.305,0.31,0.315,0.32,0.325,0.33,0.335,
0.34,0.345,0.35,0.355,0.36,0.365,0.37,0.375,0.38,0.385,0.39,0.395,0.4,0.405,
0.41,0.415,0.42,0.425,0.43,0.435,0.44,0.445,0.45,0.455,0.46,0.465,0.47,
0.475,0.48,0.485,0.49,0.495,0.5,0.505,0.51,0.515,0.52,0.525,0.53,0.535,
0.54,0.545,0.55,0.555,0.56,0.565,0.57,0.575,0.58,0.585,0.59,0.595,0.6,0.605,
0.61,0.615,0.62,0.625,0.63,0.635,0.64,0.645,0.65,0.655,0.66,0.665,0.67,
0.675,0.68,0.685,0.690000000000001,0.695000000000001,0.700000000000001,
0.705000000000001,0.710000000000001,0.715000000000001,0.720000000000001,
0.725000000000001,0.730000000000001,0.735000000000001,0.740000000000001,
0.745000000000001,0.750000000000001,0.755000000000001,0.760000000000001,
0.765000000000001,0.770000000000001,0.775000000000001,0.780000000000001,
0.785000000000001,0.790000000000001,0.795000000000001,0.800000000000001,
0.805000000000001,0.810000000000001,0.815000000000001,0.820000000000001,
0.825000000000001,0.830000000000001,0.835000000000001,0.840000000000001,
0.845000000000001,0.850000000000001,0.855000000000001,0.860000000000001,
0.865000000000001,0.870000000000001,0.875000000000001,0.880000000000001,
0.885000000000001,0.890000000000001,0.895000000000001,0.900000000000001,
0.905000000000001,0.910000000000001,0.915000000000001,0.920000000000001,
0.925000000000001,0.930000000000001,0.935000000000001,0.940000000000001,
0.945000000000001,0.950000000000001,0.955000000000001,0.960000000000001,
0.965000000000001,0.970000000000001,0.975000000000001,0.980000000000001,
0.985000000000001,0.990000000000001,0.995000000000001,1.),.UNSPECIFIED.)
CURVE()
GEOMETRIC_REPRESENTATION_ITEM()
RATIONAL_B_SPLINE_CURVE((1.,1.,1.,1.,1.,1.,1.,1.,1.,1.,1.,1.,1.,1.,1.,1.,
1.,1.,1.,1.,1.,1.,1.,1.,1.,1.,1.,1.,1.,1.,1.,1.,1.,1.,1.,1.,1.,1.,1.,1.,
1.,1.,1.,1.,1.,1.,1.,1.,1.,1.,1.,1.,1.,1.,1.,1.,1.,1.,1.,1.,1.,1.,1.,1.,
1.,1.,1.,1.,1.,1.,1.,1.,1.,1.,1.,1.,1.,1.,1.,1.,1.,1.,1.,1.,1.,1.,1.,1.,
1.,1.,1.,1.,1.,1.,1.,1.,1.,1.,1.,1.,1.,1.,1.,1.,1.,1.,1.,1.,1.,1.,1.,1.,
1.,1.,1.,1.,1.,1.,1.,1.,1.,1.,1.,1.,1.,1.,1.,1.,1.,1.,1.,1.,1.,1.,1.,1.,
1.,1.,1.,1.,1.,1.,1.,1.,1.,1.,1.,1.,1.,1.,1.,1.,1.,1.,1.,1.,1.,1.,1.,1.,
1.,1.,1.,1.,1.,1.,1.,1.,1.,1.,1.,1.,1.,1.,1.,1.,1.,1.,1.,1.,1.,1.,1.,1.,
1.,1.,1.,1.,1.,1.,1.,1.,1.,1.,1.,1.,1.,1.,1.,1.,1.,1.,1.,1.,1.))
REPRESENTATION_ITEM('')
);
#730=(
BOUNDED_CURVE()
B_SPLINE_CURVE(5,(#183277,#183278,#183279,#183280,#183281,#183282,#183283,
#183284,#183285,#183286,#183287,#183288,#183289,#183290,#183291,#183292,
#183293,#183294,#183295,#183296,#183297,#183298,#183299,#183300,#183301,
#183302,#183303,#183304,#183305,#183306,#183307,#183308,#183309,#183310,
#183311,#183312,#183313,#183314,#183315,#183316,#183317,#183318,#183319,
#183320,#183321,#183322,#183323,#183324,#183325,#183326,#183327,#183328,
#183329,#183330,#183331,#183332,#183333,#183334,#183335,#183336,#183337,
#183338,#183339,#183340,#183341,#183342,#183343,#183344,#183345,#183346,
#183347,#183348,#183349,#183350,#183351,#183352,#183353,#183354,#183355,
#183356,#183357,#183358,#183359,#183360,#183361,#183362,#183363,#183364,
#183365,#183366,#183367,#183368,#183369,#183370,#183371,#183372,#183373,
#183374,#183375,#183376,#183377,#183378,#183379,#183380,#183381,#183382,
#183383,#183384,#183385,#183386,#183387,#183388,#183389,#183390,#183391,
#183392,#183393,#183394,#183395,#183396,#183397,#183398,#183399,#183400,
#183401,#183402,#183403,#183404,#183405,#183406,#183407,#183408,#183409,
#183410,#183411,#183412,#183413,#183414,#183415,#183416,#183417,#183418,
#183419,#183420,#183421,#183422,#183423,#183424,#183425,#183426,#183427,
#183428,#183429,#183430,#183431,#183432,#183433,#183434,#183435,#183436,
#183437,#183438,#183439,#183440,#183441,#183442,#183443,#183444,#183445,
#183446,#183447,#183448,#183449,#183450,#183451,#183452,#183453,#183454,
#183455,#183456,#183457,#183458,#183459,#183460,#183461,#183462,#183463,
#183464,#183465,#183466,#183467,#183468,#183469,#183470,#183471,#183472,
#183473,#183474,#183475,#183476,#183477,#183478,#183479,#183480,#183481),
 .UNSPECIFIED.,.F.,.F.)
B_SPLINE_CURVE_WITH_KNOTS((6,1,1,1,1,1,1,1,1,1,1,1,1,1,1,1,1,1,1,1,1,1,
1,1,1,1,1,1,1,1,1,1,1,1,1,1,1,1,1,1,1,1,1,1,1,1,1,1,1,1,1,1,1,1,1,1,1,1,
1,1,1,1,1,1,1,1,1,1,1,1,1,1,1,1,1,1,1,1,1,1,1,1,1,1,1,1,1,1,1,1,1,1,1,1,
1,1,1,1,1,1,1,1,1,1,1,1,1,1,1,1,1,1,1,1,1,1,1,1,1,1,1,1,1,1,1,1,1,1,1,1,
1,1,1,1,1,1,1,1,1,1,1,1,1,1,1,1,1,1,1,1,1,1,1,1,1,1,1,1,1,1,1,1,1,1,1,1,
1,1,1,1,1,1,1,1,1,1,1,1,1,1,1,1,1,1,1,1,1,1,1,1,1,1,1,1,1,1,1,1,1,1,6),
(-1.,-0.995000000000001,-0.990000000000001,-0.985000000000001,-0.980000000000001,
-0.975000000000001,-0.970000000000001,-0.965000000000001,-0.960000000000001,
-0.955000000000001,-0.950000000000001,-0.945000000000001,-0.940000000000001,
-0.935000000000001,-0.930000000000001,-0.925000000000001,-0.920000000000001,
-0.915000000000001,-0.910000000000001,-0.905000000000001,-0.900000000000001,
-0.895000000000001,-0.890000000000001,-0.885000000000001,-0.880000000000001,
-0.875000000000001,-0.870000000000001,-0.865000000000001,-0.860000000000001,
-0.855000000000001,-0.850000000000001,-0.845000000000001,-0.840000000000001,
-0.835000000000001,-0.830000000000001,-0.825000000000001,-0.820000000000001,
-0.815000000000001,-0.810000000000001,-0.805000000000001,-0.800000000000001,
-0.795000000000001,-0.790000000000001,-0.785000000000001,-0.780000000000001,
-0.775000000000001,-0.770000000000001,-0.765000000000001,-0.760000000000001,
-0.755000000000001,-0.750000000000001,-0.745000000000001,-0.740000000000001,
-0.735000000000001,-0.730000000000001,-0.725000000000001,-0.720000000000001,
-0.715000000000001,-0.710000000000001,-0.705000000000001,-0.700000000000001,
-0.695000000000001,-0.690000000000001,-0.685,-0.68,-0.675,-0.67,-0.665,
-0.66,-0.655,-0.65,-0.645,-0.64,-0.635,-0.63,-0.625,-0.62,-0.615,-0.61,
-0.605,-0.6,-0.595,-0.59,-0.585,-0.58,-0.575,-0.57,-0.565,-0.56,-0.555,
-0.55,-0.545,-0.54,-0.535,-0.53,-0.525,-0.52,-0.515,-0.51,-0.505,-0.5,-0.495,
-0.49,-0.485,-0.48,-0.475,-0.47,-0.465,-0.46,-0.455,-0.45,-0.445,-0.44,
-0.435,-0.43,-0.425,-0.42,-0.415,-0.41,-0.405,-0.4,-0.395,-0.39,-0.385,
-0.38,-0.375,-0.37,-0.365,-0.36,-0.355,-0.35,-0.345,-0.34,-0.335,-0.33,
-0.325,-0.32,-0.315,-0.31,-0.305,-0.3,-0.295,-0.29,-0.285,-0.28,-0.275,
-0.27,-0.265,-0.26,-0.255,-0.25,-0.245,-0.24,-0.235,-0.23,-0.225,-0.22,
-0.215,-0.21,-0.205,-0.2,-0.195,-0.19,-0.185,-0.18,-0.175,-0.17,-0.165,
-0.16,-0.155,-0.15,-0.145,-0.14,-0.135,-0.13,-0.125,-0.12,-0.115,-0.11,
-0.105,-0.1,-0.095,-0.09,-0.085,-0.08,-0.075,-0.07,-0.065,-0.06,-0.055,
-0.05,-0.045,-0.04,-0.035,-0.03,-0.025,-0.02,-0.015,-0.01,-0.005,0.),
 .UNSPECIFIED.)
CURVE()
GEOMETRIC_REPRESENTATION_ITEM()
RATIONAL_B_SPLINE_CURVE((1.,1.,1.,1.,1.,1.,1.,1.,1.,1.,1.,1.,1.,1.,1.,1.,
1.,1.,1.,1.,1.,1.,1.,1.,1.,1.,1.,1.,1.,1.,1.,1.,1.,1.,1.,1.,1.,1.,1.,1.,
1.,1.,1.,1.,1.,1.,1.,1.,1.,1.,1.,1.,1.,1.,1.,1.,1.,1.,1.,1.,1.,1.,1.,1.,
1.,1.,1.,1.,1.,1.,1.,1.,1.,1.,1.,1.,1.,1.,1.,1.,1.,1.,1.,1.,1.,1.,1.,1.,
1.,1.,1.,1.,1.,1.,1.,1.,1.,1.,1.,1.,1.,1.,1.,1.,1.,1.,1.,1.,1.,1.,1.,1.,
1.,1.,1.,1.,1.,1.,1.,1.,1.,1.,1.,1.,1.,1.,1.,1.,1.,1.,1.,1.,1.,1.,1.,1.,
1.,1.,1.,1.,1.,1.,1.,1.,1.,1.,1.,1.,1.,1.,1.,1.,1.,1.,1.,1.,1.,1.,1.,1.,
1.,1.,1.,1.,1.,1.,1.,1.,1.,1.,1.,1.,1.,1.,1.,1.,1.,1.,1.,1.,1.,1.,1.,1.,
1.,1.,1.,1.,1.,1.,1.,1.,1.,1.,1.,1.,1.,1.,1.,1.,1.,1.,1.,1.,1.))
REPRESENTATION_ITEM('')
);
#731=(
BOUNDED_CURVE()
B_SPLINE_CURVE(5,(#183493,#183494,#183495,#183496,#183497,#183498,#183499,
#183500,#183501,#183502,#183503,#183504,#183505,#183506,#183507,#183508,
#183509,#183510,#183511,#183512,#183513,#183514,#183515,#183516,#183517,
#183518,#183519,#183520,#183521,#183522,#183523,#183524,#183525,#183526,
#183527,#183528,#183529,#183530,#183531,#183532,#183533,#183534,#183535,
#183536,#183537,#183538,#183539,#183540,#183541,#183542,#183543,#183544,
#183545,#183546,#183547,#183548,#183549,#183550,#183551,#183552,#183553,
#183554,#183555,#183556,#183557,#183558,#183559,#183560,#183561,#183562,
#183563,#183564,#183565,#183566,#183567,#183568,#183569,#183570,#183571,
#183572,#183573,#183574,#183575,#183576,#183577,#183578,#183579,#183580,
#183581,#183582,#183583,#183584,#183585,#183586,#183587,#183588,#183589,
#183590,#183591,#183592,#183593,#183594,#183595,#183596,#183597,#183598,
#183599,#183600,#183601,#183602,#183603,#183604,#183605,#183606,#183607,
#183608,#183609,#183610,#183611,#183612,#183613,#183614,#183615,#183616,
#183617,#183618,#183619,#183620,#183621,#183622,#183623,#183624,#183625,
#183626,#183627,#183628,#183629,#183630,#183631,#183632,#183633,#183634,
#183635,#183636,#183637,#183638,#183639,#183640,#183641,#183642,#183643,
#183644,#183645,#183646,#183647,#183648,#183649,#183650,#183651,#183652,
#183653,#183654,#183655,#183656,#183657,#183658,#183659,#183660,#183661,
#183662,#183663,#183664,#183665,#183666,#183667,#183668,#183669,#183670,
#183671,#183672,#183673,#183674,#183675,#183676,#183677,#183678,#183679,
#183680,#183681,#183682,#183683,#183684,#183685,#183686,#183687,#183688,
#183689,#183690,#183691,#183692,#183693,#183694,#183695,#183696,#183697),
 .UNSPECIFIED.,.F.,.F.)
B_SPLINE_CURVE_WITH_KNOTS((6,1,1,1,1,1,1,1,1,1,1,1,1,1,1,1,1,1,1,1,1,1,
1,1,1,1,1,1,1,1,1,1,1,1,1,1,1,1,1,1,1,1,1,1,1,1,1,1,1,1,1,1,1,1,1,1,1,1,
1,1,1,1,1,1,1,1,1,1,1,1,1,1,1,1,1,1,1,1,1,1,1,1,1,1,1,1,1,1,1,1,1,1,1,1,
1,1,1,1,1,1,1,1,1,1,1,1,1,1,1,1,1,1,1,1,1,1,1,1,1,1,1,1,1,1,1,1,1,1,1,1,
1,1,1,1,1,1,1,1,1,1,1,1,1,1,1,1,1,1,1,1,1,1,1,1,1,1,1,1,1,1,1,1,1,1,1,1,
1,1,1,1,1,1,1,1,1,1,1,1,1,1,1,1,1,1,1,1,1,1,1,1,1,1,1,1,1,1,1,1,1,1,6),
(0.,0.005,0.01,0.015,0.02,0.025,0.03,0.035,0.04,0.045,0.05,0.055,0.06,0.065,
0.07,0.075,0.08,0.085,0.09,0.095,0.1,0.105,0.11,0.115,0.12,0.125,0.13,0.135,
0.14,0.145,0.15,0.155,0.16,0.165,0.17,0.175,0.18,0.185,0.19,0.195,0.2,0.205,
0.21,0.215,0.22,0.225,0.23,0.235,0.24,0.245,0.25,0.255,0.26,0.265,0.27,
0.275,0.28,0.285,0.29,0.295,0.3,0.305,0.31,0.315,0.32,0.325,0.33,0.335,
0.34,0.345,0.35,0.355,0.36,0.365,0.37,0.375,0.38,0.385,0.39,0.395,0.4,0.405,
0.41,0.415,0.42,0.425,0.43,0.435,0.44,0.445,0.45,0.455,0.46,0.465,0.47,
0.475,0.48,0.485,0.49,0.495,0.5,0.505,0.51,0.515,0.52,0.525,0.53,0.535,
0.54,0.545,0.55,0.555,0.56,0.565,0.57,0.575,0.58,0.585,0.59,0.595,0.6,0.605,
0.61,0.615,0.62,0.625,0.63,0.635,0.64,0.645,0.65,0.655,0.66,0.665,0.67,
0.675,0.68,0.685,0.690000000000001,0.695000000000001,0.700000000000001,
0.705000000000001,0.710000000000001,0.715000000000001,0.720000000000001,
0.725000000000001,0.730000000000001,0.735000000000001,0.740000000000001,
0.745000000000001,0.750000000000001,0.755000000000001,0.760000000000001,
0.765000000000001,0.770000000000001,0.775000000000001,0.780000000000001,
0.785000000000001,0.790000000000001,0.795000000000001,0.800000000000001,
0.805000000000001,0.810000000000001,0.815000000000001,0.820000000000001,
0.825000000000001,0.830000000000001,0.835000000000001,0.840000000000001,
0.845000000000001,0.850000000000001,0.855000000000001,0.860000000000001,
0.865000000000001,0.870000000000001,0.875000000000001,0.880000000000001,
0.885000000000001,0.890000000000001,0.895000000000001,0.900000000000001,
0.905000000000001,0.910000000000001,0.915000000000001,0.920000000000001,
0.925000000000001,0.930000000000001,0.935000000000001,0.940000000000001,
0.945000000000001,0.950000000000001,0.955000000000001,0.960000000000001,
0.965000000000001,0.970000000000001,0.975000000000001,0.980000000000001,
0.985000000000001,0.990000000000001,0.995000000000001,1.),.UNSPECIFIED.)
CURVE()
GEOMETRIC_REPRESENTATION_ITEM()
RATIONAL_B_SPLINE_CURVE((1.,1.,1.,1.,1.,1.,1.,1.,1.,1.,1.,1.,1.,1.,1.,1.,
1.,1.,1.,1.,1.,1.,1.,1.,1.,1.,1.,1.,1.,1.,1.,1.,1.,1.,1.,1.,1.,1.,1.,1.,
1.,1.,1.,1.,1.,1.,1.,1.,1.,1.,1.,1.,1.,1.,1.,1.,1.,1.,1.,1.,1.,1.,1.,1.,
1.,1.,1.,1.,1.,1.,1.,1.,1.,1.,1.,1.,1.,1.,1.,1.,1.,1.,1.,1.,1.,1.,1.,1.,
1.,1.,1.,1.,1.,1.,1.,1.,1.,1.,1.,1.,1.,1.,1.,1.,1.,1.,1.,1.,1.,1.,1.,1.,
1.,1.,1.,1.,1.,1.,1.,1.,1.,1.,1.,1.,1.,1.,1.,1.,1.,1.,1.,1.,1.,1.,1.,1.,
1.,1.,1.,1.,1.,1.,1.,1.,1.,1.,1.,1.,1.,1.,1.,1.,1.,1.,1.,1.,1.,1.,1.,1.,
1.,1.,1.,1.,1.,1.,1.,1.,1.,1.,1.,1.,1.,1.,1.,1.,1.,1.,1.,1.,1.,1.,1.,1.,
1.,1.,1.,1.,1.,1.,1.,1.,1.,1.,1.,1.,1.,1.,1.,1.,1.,1.,1.,1.,1.))
REPRESENTATION_ITEM('')
);
#732=(
BOUNDED_CURVE()
B_SPLINE_CURVE(5,(#183701,#183702,#183703,#183704,#183705,#183706,#183707,
#183708,#183709,#183710,#183711,#183712,#183713,#183714,#183715,#183716,
#183717,#183718,#183719,#183720,#183721,#183722,#183723,#183724,#183725,
#183726,#183727,#183728,#183729,#183730,#183731,#183732,#183733,#183734,
#183735,#183736,#183737,#183738,#183739,#183740,#183741,#183742,#183743,
#183744,#183745,#183746,#183747,#183748,#183749,#183750,#183751,#183752,
#183753,#183754,#183755,#183756,#183757,#183758,#183759,#183760,#183761,
#183762,#183763,#183764,#183765,#183766,#183767,#183768,#183769,#183770,
#183771,#183772,#183773,#183774,#183775,#183776,#183777,#183778,#183779,
#183780,#183781,#183782,#183783,#183784,#183785,#183786,#183787,#183788,
#183789,#183790,#183791,#183792,#183793,#183794,#183795,#183796,#183797,
#183798,#183799,#183800,#183801,#183802,#183803,#183804,#183805,#183806,
#183807,#183808,#183809,#183810,#183811,#183812,#183813,#183814,#183815,
#183816,#183817,#183818,#183819,#183820,#183821,#183822,#183823,#183824,
#183825,#183826,#183827,#183828,#183829,#183830,#183831,#183832,#183833,
#183834,#183835,#183836,#183837,#183838,#183839,#183840,#183841,#183842,
#183843,#183844,#183845,#183846,#183847,#183848,#183849,#183850,#183851,
#183852,#183853,#183854,#183855,#183856,#183857,#183858,#183859,#183860,
#183861,#183862,#183863,#183864,#183865,#183866,#183867,#183868,#183869,
#183870,#183871,#183872,#183873,#183874,#183875,#183876,#183877,#183878,
#183879,#183880,#183881,#183882,#183883,#183884,#183885,#183886,#183887,
#183888,#183889,#183890,#183891,#183892,#183893,#183894,#183895,#183896,
#183897,#183898,#183899,#183900,#183901,#183902,#183903,#183904,#183905),
 .UNSPECIFIED.,.F.,.F.)
B_SPLINE_CURVE_WITH_KNOTS((6,1,1,1,1,1,1,1,1,1,1,1,1,1,1,1,1,1,1,1,1,1,
1,1,1,1,1,1,1,1,1,1,1,1,1,1,1,1,1,1,1,1,1,1,1,1,1,1,1,1,1,1,1,1,1,1,1,1,
1,1,1,1,1,1,1,1,1,1,1,1,1,1,1,1,1,1,1,1,1,1,1,1,1,1,1,1,1,1,1,1,1,1,1,1,
1,1,1,1,1,1,1,1,1,1,1,1,1,1,1,1,1,1,1,1,1,1,1,1,1,1,1,1,1,1,1,1,1,1,1,1,
1,1,1,1,1,1,1,1,1,1,1,1,1,1,1,1,1,1,1,1,1,1,1,1,1,1,1,1,1,1,1,1,1,1,1,1,
1,1,1,1,1,1,1,1,1,1,1,1,1,1,1,1,1,1,1,1,1,1,1,1,1,1,1,1,1,1,1,1,1,1,6),
(-1.,-0.995000000000001,-0.990000000000001,-0.985000000000001,-0.980000000000001,
-0.975000000000001,-0.970000000000001,-0.965000000000001,-0.960000000000001,
-0.955000000000001,-0.950000000000001,-0.945000000000001,-0.940000000000001,
-0.935000000000001,-0.930000000000001,-0.925000000000001,-0.920000000000001,
-0.915000000000001,-0.910000000000001,-0.905000000000001,-0.900000000000001,
-0.895000000000001,-0.890000000000001,-0.885000000000001,-0.880000000000001,
-0.875000000000001,-0.870000000000001,-0.865000000000001,-0.860000000000001,
-0.855000000000001,-0.850000000000001,-0.845000000000001,-0.840000000000001,
-0.835000000000001,-0.830000000000001,-0.825000000000001,-0.820000000000001,
-0.815000000000001,-0.810000000000001,-0.805000000000001,-0.800000000000001,
-0.795000000000001,-0.790000000000001,-0.785000000000001,-0.780000000000001,
-0.775000000000001,-0.770000000000001,-0.765000000000001,-0.760000000000001,
-0.755000000000001,-0.750000000000001,-0.745000000000001,-0.740000000000001,
-0.735000000000001,-0.730000000000001,-0.725000000000001,-0.720000000000001,
-0.715000000000001,-0.710000000000001,-0.705000000000001,-0.700000000000001,
-0.695000000000001,-0.690000000000001,-0.685,-0.68,-0.675,-0.67,-0.665,
-0.66,-0.655,-0.65,-0.645,-0.64,-0.635,-0.63,-0.625,-0.62,-0.615,-0.61,
-0.605,-0.6,-0.595,-0.59,-0.585,-0.58,-0.575,-0.57,-0.565,-0.56,-0.555,
-0.55,-0.545,-0.54,-0.535,-0.53,-0.525,-0.52,-0.515,-0.51,-0.505,-0.5,-0.495,
-0.49,-0.485,-0.48,-0.475,-0.47,-0.465,-0.46,-0.455,-0.45,-0.445,-0.44,
-0.435,-0.43,-0.425,-0.42,-0.415,-0.41,-0.405,-0.4,-0.395,-0.39,-0.385,
-0.38,-0.375,-0.37,-0.365,-0.36,-0.355,-0.35,-0.345,-0.34,-0.335,-0.33,
-0.325,-0.32,-0.315,-0.31,-0.305,-0.3,-0.295,-0.29,-0.285,-0.28,-0.275,
-0.27,-0.265,-0.26,-0.255,-0.25,-0.245,-0.24,-0.235,-0.23,-0.225,-0.22,
-0.215,-0.21,-0.205,-0.2,-0.195,-0.19,-0.185,-0.18,-0.175,-0.17,-0.165,
-0.16,-0.155,-0.15,-0.145,-0.14,-0.135,-0.13,-0.125,-0.12,-0.115,-0.11,
-0.105,-0.1,-0.095,-0.09,-0.085,-0.08,-0.075,-0.07,-0.065,-0.06,-0.055,
-0.05,-0.045,-0.04,-0.035,-0.03,-0.025,-0.02,-0.015,-0.01,-0.005,0.),
 .UNSPECIFIED.)
CURVE()
GEOMETRIC_REPRESENTATION_ITEM()
RATIONAL_B_SPLINE_CURVE((1.,1.,1.,1.,1.,1.,1.,1.,1.,1.,1.,1.,1.,1.,1.,1.,
1.,1.,1.,1.,1.,1.,1.,1.,1.,1.,1.,1.,1.,1.,1.,1.,1.,1.,1.,1.,1.,1.,1.,1.,
1.,1.,1.,1.,1.,1.,1.,1.,1.,1.,1.,1.,1.,1.,1.,1.,1.,1.,1.,1.,1.,1.,1.,1.,
1.,1.,1.,1.,1.,1.,1.,1.,1.,1.,1.,1.,1.,1.,1.,1.,1.,1.,1.,1.,1.,1.,1.,1.,
1.,1.,1.,1.,1.,1.,1.,1.,1.,1.,1.,1.,1.,1.,1.,1.,1.,1.,1.,1.,1.,1.,1.,1.,
1.,1.,1.,1.,1.,1.,1.,1.,1.,1.,1.,1.,1.,1.,1.,1.,1.,1.,1.,1.,1.,1.,1.,1.,
1.,1.,1.,1.,1.,1.,1.,1.,1.,1.,1.,1.,1.,1.,1.,1.,1.,1.,1.,1.,1.,1.,1.,1.,
1.,1.,1.,1.,1.,1.,1.,1.,1.,1.,1.,1.,1.,1.,1.,1.,1.,1.,1.,1.,1.,1.,1.,1.,
1.,1.,1.,1.,1.,1.,1.,1.,1.,1.,1.,1.,1.,1.,1.,1.,1.,1.,1.,1.,1.))
REPRESENTATION_ITEM('')
);
#733=(
BOUNDED_CURVE()
B_SPLINE_CURVE(5,(#183917,#183918,#183919,#183920,#183921,#183922,#183923,
#183924,#183925,#183926,#183927,#183928,#183929,#183930,#183931,#183932,
#183933,#183934,#183935,#183936,#183937,#183938,#183939,#183940,#183941,
#183942,#183943,#183944,#183945,#183946,#183947,#183948,#183949,#183950,
#183951,#183952,#183953,#183954,#183955,#183956,#183957,#183958,#183959,
#183960,#183961,#183962,#183963,#183964,#183965,#183966,#183967,#183968,
#183969,#183970,#183971,#183972,#183973,#183974,#183975,#183976,#183977,
#183978,#183979,#183980,#183981,#183982,#183983,#183984,#183985,#183986,
#183987,#183988,#183989,#183990,#183991,#183992,#183993,#183994,#183995,
#183996,#183997,#183998,#183999,#184000,#184001,#184002,#184003,#184004,
#184005,#184006,#184007,#184008,#184009,#184010,#184011,#184012,#184013,
#184014,#184015,#184016,#184017,#184018,#184019,#184020,#184021,#184022,
#184023,#184024,#184025,#184026,#184027,#184028,#184029,#184030,#184031,
#184032,#184033,#184034,#184035,#184036,#184037,#184038,#184039,#184040,
#184041,#184042,#184043,#184044,#184045,#184046,#184047,#184048,#184049,
#184050,#184051,#184052,#184053,#184054,#184055,#184056,#184057,#184058,
#184059,#184060,#184061,#184062,#184063,#184064,#184065,#184066,#184067,
#184068,#184069,#184070,#184071,#184072,#184073,#184074,#184075,#184076,
#184077,#184078,#184079,#184080,#184081,#184082,#184083,#184084,#184085,
#184086,#184087,#184088,#184089,#184090,#184091,#184092,#184093,#184094,
#184095,#184096,#184097,#184098,#184099,#184100,#184101,#184102,#184103,
#184104,#184105,#184106,#184107,#184108,#184109,#184110,#184111,#184112,
#184113,#184114,#184115,#184116,#184117,#184118,#184119,#184120,#184121),
 .UNSPECIFIED.,.F.,.F.)
B_SPLINE_CURVE_WITH_KNOTS((6,1,1,1,1,1,1,1,1,1,1,1,1,1,1,1,1,1,1,1,1,1,
1,1,1,1,1,1,1,1,1,1,1,1,1,1,1,1,1,1,1,1,1,1,1,1,1,1,1,1,1,1,1,1,1,1,1,1,
1,1,1,1,1,1,1,1,1,1,1,1,1,1,1,1,1,1,1,1,1,1,1,1,1,1,1,1,1,1,1,1,1,1,1,1,
1,1,1,1,1,1,1,1,1,1,1,1,1,1,1,1,1,1,1,1,1,1,1,1,1,1,1,1,1,1,1,1,1,1,1,1,
1,1,1,1,1,1,1,1,1,1,1,1,1,1,1,1,1,1,1,1,1,1,1,1,1,1,1,1,1,1,1,1,1,1,1,1,
1,1,1,1,1,1,1,1,1,1,1,1,1,1,1,1,1,1,1,1,1,1,1,1,1,1,1,1,1,1,1,1,1,1,6),
(0.,0.005,0.01,0.015,0.02,0.025,0.03,0.035,0.04,0.045,0.05,0.055,0.06,0.065,
0.07,0.075,0.08,0.085,0.09,0.095,0.1,0.105,0.11,0.115,0.12,0.125,0.13,0.135,
0.14,0.145,0.15,0.155,0.16,0.165,0.17,0.175,0.18,0.185,0.19,0.195,0.2,0.205,
0.21,0.215,0.22,0.225,0.23,0.235,0.24,0.245,0.25,0.255,0.26,0.265,0.27,
0.275,0.28,0.285,0.29,0.295,0.3,0.305,0.31,0.315,0.32,0.325,0.33,0.335,
0.34,0.345,0.35,0.355,0.36,0.365,0.37,0.375,0.38,0.385,0.39,0.395,0.4,0.405,
0.41,0.415,0.42,0.425,0.43,0.435,0.44,0.445,0.45,0.455,0.46,0.465,0.47,
0.475,0.48,0.485,0.49,0.495,0.5,0.505,0.51,0.515,0.52,0.525,0.53,0.535,
0.54,0.545,0.55,0.555,0.56,0.565,0.57,0.575,0.58,0.585,0.59,0.595,0.6,0.605,
0.61,0.615,0.62,0.625,0.63,0.635,0.64,0.645,0.65,0.655,0.66,0.665,0.67,
0.675,0.68,0.685,0.690000000000001,0.695000000000001,0.700000000000001,
0.705000000000001,0.710000000000001,0.715000000000001,0.720000000000001,
0.725000000000001,0.730000000000001,0.735000000000001,0.740000000000001,
0.745000000000001,0.750000000000001,0.755000000000001,0.760000000000001,
0.765000000000001,0.770000000000001,0.775000000000001,0.780000000000001,
0.785000000000001,0.790000000000001,0.795000000000001,0.800000000000001,
0.805000000000001,0.810000000000001,0.815000000000001,0.820000000000001,
0.825000000000001,0.830000000000001,0.835000000000001,0.840000000000001,
0.845000000000001,0.850000000000001,0.855000000000001,0.860000000000001,
0.865000000000001,0.870000000000001,0.875000000000001,0.880000000000001,
0.885000000000001,0.890000000000001,0.895000000000001,0.900000000000001,
0.905000000000001,0.910000000000001,0.915000000000001,0.920000000000001,
0.925000000000001,0.930000000000001,0.935000000000001,0.940000000000001,
0.945000000000001,0.950000000000001,0.955000000000001,0.960000000000001,
0.965000000000001,0.970000000000001,0.975000000000001,0.980000000000001,
0.985000000000001,0.990000000000001,0.995000000000001,1.),.UNSPECIFIED.)
CURVE()
GEOMETRIC_REPRESENTATION_ITEM()
RATIONAL_B_SPLINE_CURVE((1.,1.,1.,1.,1.,1.,1.,1.,1.,1.,1.,1.,1.,1.,1.,1.,
1.,1.,1.,1.,1.,1.,1.,1.,1.,1.,1.,1.,1.,1.,1.,1.,1.,1.,1.,1.,1.,1.,1.,1.,
1.,1.,1.,1.,1.,1.,1.,1.,1.,1.,1.,1.,1.,1.,1.,1.,1.,1.,1.,1.,1.,1.,1.,1.,
1.,1.,1.,1.,1.,1.,1.,1.,1.,1.,1.,1.,1.,1.,1.,1.,1.,1.,1.,1.,1.,1.,1.,1.,
1.,1.,1.,1.,1.,1.,1.,1.,1.,1.,1.,1.,1.,1.,1.,1.,1.,1.,1.,1.,1.,1.,1.,1.,
1.,1.,1.,1.,1.,1.,1.,1.,1.,1.,1.,1.,1.,1.,1.,1.,1.,1.,1.,1.,1.,1.,1.,1.,
1.,1.,1.,1.,1.,1.,1.,1.,1.,1.,1.,1.,1.,1.,1.,1.,1.,1.,1.,1.,1.,1.,1.,1.,
1.,1.,1.,1.,1.,1.,1.,1.,1.,1.,1.,1.,1.,1.,1.,1.,1.,1.,1.,1.,1.,1.,1.,1.,
1.,1.,1.,1.,1.,1.,1.,1.,1.,1.,1.,1.,1.,1.,1.,1.,1.,1.,1.,1.,1.))
REPRESENTATION_ITEM('')
);
#734=(
BOUNDED_CURVE()
B_SPLINE_CURVE(5,(#184125,#184126,#184127,#184128,#184129,#184130,#184131,
#184132,#184133,#184134,#184135,#184136,#184137,#184138,#184139,#184140,
#184141,#184142,#184143,#184144,#184145,#184146,#184147,#184148,#184149,
#184150,#184151,#184152,#184153,#184154,#184155,#184156,#184157,#184158,
#184159,#184160,#184161,#184162,#184163,#184164,#184165,#184166,#184167,
#184168,#184169,#184170,#184171,#184172,#184173,#184174,#184175,#184176,
#184177,#184178,#184179,#184180,#184181,#184182,#184183,#184184,#184185,
#184186,#184187,#184188,#184189,#184190,#184191,#184192,#184193,#184194,
#184195,#184196,#184197,#184198,#184199,#184200,#184201,#184202,#184203,
#184204,#184205,#184206,#184207,#184208,#184209,#184210,#184211,#184212,
#184213,#184214,#184215,#184216,#184217,#184218,#184219,#184220,#184221,
#184222,#184223,#184224,#184225,#184226,#184227,#184228,#184229,#184230,
#184231,#184232,#184233,#184234,#184235,#184236,#184237,#184238,#184239,
#184240,#184241,#184242,#184243,#184244,#184245,#184246,#184247,#184248,
#184249,#184250,#184251,#184252,#184253,#184254,#184255,#184256,#184257,
#184258,#184259,#184260,#184261,#184262,#184263,#184264,#184265,#184266,
#184267,#184268,#184269,#184270,#184271,#184272,#184273,#184274,#184275,
#184276,#184277,#184278,#184279,#184280,#184281,#184282,#184283,#184284,
#184285,#184286,#184287,#184288,#184289,#184290,#184291,#184292,#184293,
#184294,#184295,#184296,#184297,#184298,#184299,#184300,#184301,#184302,
#184303,#184304,#184305,#184306,#184307,#184308,#184309,#184310,#184311,
#184312,#184313,#184314,#184315,#184316,#184317,#184318,#184319,#184320,
#184321,#184322,#184323,#184324,#184325,#184326,#184327,#184328,#184329),
 .UNSPECIFIED.,.F.,.F.)
B_SPLINE_CURVE_WITH_KNOTS((6,1,1,1,1,1,1,1,1,1,1,1,1,1,1,1,1,1,1,1,1,1,
1,1,1,1,1,1,1,1,1,1,1,1,1,1,1,1,1,1,1,1,1,1,1,1,1,1,1,1,1,1,1,1,1,1,1,1,
1,1,1,1,1,1,1,1,1,1,1,1,1,1,1,1,1,1,1,1,1,1,1,1,1,1,1,1,1,1,1,1,1,1,1,1,
1,1,1,1,1,1,1,1,1,1,1,1,1,1,1,1,1,1,1,1,1,1,1,1,1,1,1,1,1,1,1,1,1,1,1,1,
1,1,1,1,1,1,1,1,1,1,1,1,1,1,1,1,1,1,1,1,1,1,1,1,1,1,1,1,1,1,1,1,1,1,1,1,
1,1,1,1,1,1,1,1,1,1,1,1,1,1,1,1,1,1,1,1,1,1,1,1,1,1,1,1,1,1,1,1,1,1,6),
(-1.,-0.995000000000001,-0.990000000000001,-0.985000000000001,-0.980000000000001,
-0.975000000000001,-0.970000000000001,-0.965000000000001,-0.960000000000001,
-0.955000000000001,-0.950000000000001,-0.945000000000001,-0.940000000000001,
-0.935000000000001,-0.930000000000001,-0.925000000000001,-0.920000000000001,
-0.915000000000001,-0.910000000000001,-0.905000000000001,-0.900000000000001,
-0.895000000000001,-0.890000000000001,-0.885000000000001,-0.880000000000001,
-0.875000000000001,-0.870000000000001,-0.865000000000001,-0.860000000000001,
-0.855000000000001,-0.850000000000001,-0.845000000000001,-0.840000000000001,
-0.835000000000001,-0.830000000000001,-0.825000000000001,-0.820000000000001,
-0.815000000000001,-0.810000000000001,-0.805000000000001,-0.800000000000001,
-0.795000000000001,-0.790000000000001,-0.785000000000001,-0.780000000000001,
-0.775000000000001,-0.770000000000001,-0.765000000000001,-0.760000000000001,
-0.755000000000001,-0.750000000000001,-0.745000000000001,-0.740000000000001,
-0.735000000000001,-0.730000000000001,-0.725000000000001,-0.720000000000001,
-0.715000000000001,-0.710000000000001,-0.705000000000001,-0.700000000000001,
-0.695000000000001,-0.690000000000001,-0.685,-0.68,-0.675,-0.67,-0.665,
-0.66,-0.655,-0.65,-0.645,-0.64,-0.635,-0.63,-0.625,-0.62,-0.615,-0.61,
-0.605,-0.6,-0.595,-0.59,-0.585,-0.58,-0.575,-0.57,-0.565,-0.56,-0.555,
-0.55,-0.545,-0.54,-0.535,-0.53,-0.525,-0.52,-0.515,-0.51,-0.505,-0.5,-0.495,
-0.49,-0.485,-0.48,-0.475,-0.47,-0.465,-0.46,-0.455,-0.45,-0.445,-0.44,
-0.435,-0.43,-0.425,-0.42,-0.415,-0.41,-0.405,-0.4,-0.395,-0.39,-0.385,
-0.38,-0.375,-0.37,-0.365,-0.36,-0.355,-0.35,-0.345,-0.34,-0.335,-0.33,
-0.325,-0.32,-0.315,-0.31,-0.305,-0.3,-0.295,-0.29,-0.285,-0.28,-0.275,
-0.27,-0.265,-0.26,-0.255,-0.25,-0.245,-0.24,-0.235,-0.23,-0.225,-0.22,
-0.215,-0.21,-0.205,-0.2,-0.195,-0.19,-0.185,-0.18,-0.175,-0.17,-0.165,
-0.16,-0.155,-0.15,-0.145,-0.14,-0.135,-0.13,-0.125,-0.12,-0.115,-0.11,
-0.105,-0.1,-0.095,-0.09,-0.085,-0.08,-0.075,-0.07,-0.065,-0.06,-0.055,
-0.05,-0.045,-0.04,-0.035,-0.03,-0.025,-0.02,-0.015,-0.01,-0.005,0.),
 .UNSPECIFIED.)
CURVE()
GEOMETRIC_REPRESENTATION_ITEM()
RATIONAL_B_SPLINE_CURVE((1.,1.,1.,1.,1.,1.,1.,1.,1.,1.,1.,1.,1.,1.,1.,1.,
1.,1.,1.,1.,1.,1.,1.,1.,1.,1.,1.,1.,1.,1.,1.,1.,1.,1.,1.,1.,1.,1.,1.,1.,
1.,1.,1.,1.,1.,1.,1.,1.,1.,1.,1.,1.,1.,1.,1.,1.,1.,1.,1.,1.,1.,1.,1.,1.,
1.,1.,1.,1.,1.,1.,1.,1.,1.,1.,1.,1.,1.,1.,1.,1.,1.,1.,1.,1.,1.,1.,1.,1.,
1.,1.,1.,1.,1.,1.,1.,1.,1.,1.,1.,1.,1.,1.,1.,1.,1.,1.,1.,1.,1.,1.,1.,1.,
1.,1.,1.,1.,1.,1.,1.,1.,1.,1.,1.,1.,1.,1.,1.,1.,1.,1.,1.,1.,1.,1.,1.,1.,
1.,1.,1.,1.,1.,1.,1.,1.,1.,1.,1.,1.,1.,1.,1.,1.,1.,1.,1.,1.,1.,1.,1.,1.,
1.,1.,1.,1.,1.,1.,1.,1.,1.,1.,1.,1.,1.,1.,1.,1.,1.,1.,1.,1.,1.,1.,1.,1.,
1.,1.,1.,1.,1.,1.,1.,1.,1.,1.,1.,1.,1.,1.,1.,1.,1.,1.,1.,1.,1.))
REPRESENTATION_ITEM('')
);
#735=(
BOUNDED_CURVE()
B_SPLINE_CURVE(5,(#184341,#184342,#184343,#184344,#184345,#184346,#184347,
#184348,#184349,#184350,#184351,#184352,#184353,#184354,#184355,#184356,
#184357,#184358,#184359,#184360,#184361,#184362,#184363,#184364,#184365,
#184366,#184367,#184368,#184369,#184370,#184371,#184372,#184373,#184374,
#184375,#184376,#184377,#184378,#184379,#184380,#184381,#184382,#184383,
#184384,#184385,#184386,#184387,#184388,#184389,#184390,#184391,#184392,
#184393,#184394,#184395,#184396,#184397,#184398,#184399,#184400,#184401,
#184402,#184403,#184404,#184405,#184406,#184407,#184408,#184409,#184410,
#184411,#184412,#184413,#184414,#184415,#184416,#184417,#184418,#184419,
#184420,#184421,#184422,#184423,#184424,#184425,#184426,#184427,#184428,
#184429,#184430,#184431,#184432,#184433,#184434,#184435,#184436,#184437,
#184438,#184439,#184440,#184441,#184442,#184443,#184444,#184445,#184446,
#184447,#184448,#184449,#184450,#184451,#184452,#184453,#184454,#184455,
#184456,#184457,#184458,#184459,#184460,#184461,#184462,#184463,#184464,
#184465,#184466,#184467,#184468,#184469,#184470,#184471,#184472,#184473,
#184474,#184475,#184476,#184477,#184478,#184479,#184480,#184481,#184482,
#184483,#184484,#184485,#184486,#184487,#184488,#184489,#184490,#184491,
#184492,#184493,#184494,#184495,#184496,#184497,#184498,#184499,#184500,
#184501,#184502,#184503,#184504,#184505,#184506,#184507,#184508,#184509,
#184510,#184511,#184512,#184513,#184514,#184515,#184516,#184517,#184518,
#184519,#184520,#184521,#184522,#184523,#184524,#184525,#184526,#184527,
#184528,#184529,#184530,#184531,#184532,#184533,#184534,#184535,#184536,
#184537,#184538,#184539,#184540,#184541,#184542,#184543,#184544,#184545),
 .UNSPECIFIED.,.F.,.F.)
B_SPLINE_CURVE_WITH_KNOTS((6,1,1,1,1,1,1,1,1,1,1,1,1,1,1,1,1,1,1,1,1,1,
1,1,1,1,1,1,1,1,1,1,1,1,1,1,1,1,1,1,1,1,1,1,1,1,1,1,1,1,1,1,1,1,1,1,1,1,
1,1,1,1,1,1,1,1,1,1,1,1,1,1,1,1,1,1,1,1,1,1,1,1,1,1,1,1,1,1,1,1,1,1,1,1,
1,1,1,1,1,1,1,1,1,1,1,1,1,1,1,1,1,1,1,1,1,1,1,1,1,1,1,1,1,1,1,1,1,1,1,1,
1,1,1,1,1,1,1,1,1,1,1,1,1,1,1,1,1,1,1,1,1,1,1,1,1,1,1,1,1,1,1,1,1,1,1,1,
1,1,1,1,1,1,1,1,1,1,1,1,1,1,1,1,1,1,1,1,1,1,1,1,1,1,1,1,1,1,1,1,1,1,6),
(0.,0.005,0.01,0.015,0.02,0.025,0.03,0.035,0.04,0.045,0.05,0.055,0.06,0.065,
0.07,0.075,0.08,0.085,0.09,0.095,0.1,0.105,0.11,0.115,0.12,0.125,0.13,0.135,
0.14,0.145,0.15,0.155,0.16,0.165,0.17,0.175,0.18,0.185,0.19,0.195,0.2,0.205,
0.21,0.215,0.22,0.225,0.23,0.235,0.24,0.245,0.25,0.255,0.26,0.265,0.27,
0.275,0.28,0.285,0.29,0.295,0.3,0.305,0.31,0.315,0.32,0.325,0.33,0.335,
0.34,0.345,0.35,0.355,0.36,0.365,0.37,0.375,0.38,0.385,0.39,0.395,0.4,0.405,
0.41,0.415,0.42,0.425,0.43,0.435,0.44,0.445,0.45,0.455,0.46,0.465,0.47,
0.475,0.48,0.485,0.49,0.495,0.5,0.505,0.51,0.515,0.52,0.525,0.53,0.535,
0.54,0.545,0.55,0.555,0.56,0.565,0.57,0.575,0.58,0.585,0.59,0.595,0.6,0.605,
0.61,0.615,0.62,0.625,0.63,0.635,0.64,0.645,0.65,0.655,0.66,0.665,0.67,
0.675,0.68,0.685,0.690000000000001,0.695000000000001,0.700000000000001,
0.705000000000001,0.710000000000001,0.715000000000001,0.720000000000001,
0.725000000000001,0.730000000000001,0.735000000000001,0.740000000000001,
0.745000000000001,0.750000000000001,0.755000000000001,0.760000000000001,
0.765000000000001,0.770000000000001,0.775000000000001,0.780000000000001,
0.785000000000001,0.790000000000001,0.795000000000001,0.800000000000001,
0.805000000000001,0.810000000000001,0.815000000000001,0.820000000000001,
0.825000000000001,0.830000000000001,0.835000000000001,0.840000000000001,
0.845000000000001,0.850000000000001,0.855000000000001,0.860000000000001,
0.865000000000001,0.870000000000001,0.875000000000001,0.880000000000001,
0.885000000000001,0.890000000000001,0.895000000000001,0.900000000000001,
0.905000000000001,0.910000000000001,0.915000000000001,0.920000000000001,
0.925000000000001,0.930000000000001,0.935000000000001,0.940000000000001,
0.945000000000001,0.950000000000001,0.955000000000001,0.960000000000001,
0.965000000000001,0.970000000000001,0.975000000000001,0.980000000000001,
0.985000000000001,0.990000000000001,0.995000000000001,1.),.UNSPECIFIED.)
CURVE()
GEOMETRIC_REPRESENTATION_ITEM()
RATIONAL_B_SPLINE_CURVE((1.,1.,1.,1.,1.,1.,1.,1.,1.,1.,1.,1.,1.,1.,1.,1.,
1.,1.,1.,1.,1.,1.,1.,1.,1.,1.,1.,1.,1.,1.,1.,1.,1.,1.,1.,1.,1.,1.,1.,1.,
1.,1.,1.,1.,1.,1.,1.,1.,1.,1.,1.,1.,1.,1.,1.,1.,1.,1.,1.,1.,1.,1.,1.,1.,
1.,1.,1.,1.,1.,1.,1.,1.,1.,1.,1.,1.,1.,1.,1.,1.,1.,1.,1.,1.,1.,1.,1.,1.,
1.,1.,1.,1.,1.,1.,1.,1.,1.,1.,1.,1.,1.,1.,1.,1.,1.,1.,1.,1.,1.,1.,1.,1.,
1.,1.,1.,1.,1.,1.,1.,1.,1.,1.,1.,1.,1.,1.,1.,1.,1.,1.,1.,1.,1.,1.,1.,1.,
1.,1.,1.,1.,1.,1.,1.,1.,1.,1.,1.,1.,1.,1.,1.,1.,1.,1.,1.,1.,1.,1.,1.,1.,
1.,1.,1.,1.,1.,1.,1.,1.,1.,1.,1.,1.,1.,1.,1.,1.,1.,1.,1.,1.,1.,1.,1.,1.,
1.,1.,1.,1.,1.,1.,1.,1.,1.,1.,1.,1.,1.,1.,1.,1.,1.,1.,1.,1.,1.))
REPRESENTATION_ITEM('')
);
#736=(
BOUNDED_CURVE()
B_SPLINE_CURVE(5,(#184549,#184550,#184551,#184552,#184553,#184554,#184555,
#184556,#184557,#184558,#184559,#184560,#184561,#184562,#184563,#184564,
#184565,#184566,#184567,#184568,#184569,#184570,#184571,#184572,#184573,
#184574,#184575,#184576,#184577,#184578,#184579,#184580,#184581,#184582,
#184583,#184584,#184585,#184586,#184587,#184588,#184589,#184590,#184591,
#184592,#184593,#184594,#184595,#184596,#184597,#184598,#184599,#184600,
#184601,#184602,#184603,#184604,#184605,#184606,#184607,#184608,#184609,
#184610,#184611,#184612,#184613,#184614,#184615,#184616,#184617,#184618,
#184619,#184620,#184621,#184622,#184623,#184624,#184625,#184626,#184627,
#184628,#184629,#184630,#184631,#184632,#184633,#184634,#184635,#184636,
#184637,#184638,#184639,#184640,#184641,#184642,#184643,#184644,#184645,
#184646,#184647,#184648,#184649,#184650,#184651,#184652,#184653,#184654,
#184655,#184656,#184657,#184658,#184659,#184660,#184661,#184662,#184663,
#184664,#184665,#184666,#184667,#184668,#184669,#184670,#184671,#184672,
#184673,#184674,#184675,#184676,#184677,#184678,#184679,#184680,#184681,
#184682,#184683,#184684,#184685,#184686,#184687,#184688,#184689,#184690,
#184691,#184692,#184693,#184694,#184695,#184696,#184697,#184698,#184699,
#184700,#184701,#184702,#184703,#184704,#184705,#184706,#184707,#184708,
#184709,#184710,#184711,#184712,#184713,#184714,#184715,#184716,#184717,
#184718,#184719,#184720,#184721,#184722,#184723,#184724,#184725,#184726,
#184727,#184728,#184729,#184730,#184731,#184732,#184733,#184734,#184735,
#184736,#184737,#184738,#184739,#184740,#184741,#184742,#184743,#184744,
#184745,#184746,#184747,#184748,#184749,#184750,#184751,#184752,#184753),
 .UNSPECIFIED.,.F.,.F.)
B_SPLINE_CURVE_WITH_KNOTS((6,1,1,1,1,1,1,1,1,1,1,1,1,1,1,1,1,1,1,1,1,1,
1,1,1,1,1,1,1,1,1,1,1,1,1,1,1,1,1,1,1,1,1,1,1,1,1,1,1,1,1,1,1,1,1,1,1,1,
1,1,1,1,1,1,1,1,1,1,1,1,1,1,1,1,1,1,1,1,1,1,1,1,1,1,1,1,1,1,1,1,1,1,1,1,
1,1,1,1,1,1,1,1,1,1,1,1,1,1,1,1,1,1,1,1,1,1,1,1,1,1,1,1,1,1,1,1,1,1,1,1,
1,1,1,1,1,1,1,1,1,1,1,1,1,1,1,1,1,1,1,1,1,1,1,1,1,1,1,1,1,1,1,1,1,1,1,1,
1,1,1,1,1,1,1,1,1,1,1,1,1,1,1,1,1,1,1,1,1,1,1,1,1,1,1,1,1,1,1,1,1,1,6),
(-1.,-0.995000000000001,-0.990000000000001,-0.985000000000001,-0.980000000000001,
-0.975000000000001,-0.970000000000001,-0.965000000000001,-0.960000000000001,
-0.955000000000001,-0.950000000000001,-0.945000000000001,-0.940000000000001,
-0.935000000000001,-0.930000000000001,-0.925000000000001,-0.920000000000001,
-0.915000000000001,-0.910000000000001,-0.905000000000001,-0.900000000000001,
-0.895000000000001,-0.890000000000001,-0.885000000000001,-0.880000000000001,
-0.875000000000001,-0.870000000000001,-0.865000000000001,-0.860000000000001,
-0.855000000000001,-0.850000000000001,-0.845000000000001,-0.840000000000001,
-0.835000000000001,-0.830000000000001,-0.825000000000001,-0.820000000000001,
-0.815000000000001,-0.810000000000001,-0.805000000000001,-0.800000000000001,
-0.795000000000001,-0.790000000000001,-0.785000000000001,-0.780000000000001,
-0.775000000000001,-0.770000000000001,-0.765000000000001,-0.760000000000001,
-0.755000000000001,-0.750000000000001,-0.745000000000001,-0.740000000000001,
-0.735000000000001,-0.730000000000001,-0.725000000000001,-0.720000000000001,
-0.715000000000001,-0.710000000000001,-0.705000000000001,-0.700000000000001,
-0.695000000000001,-0.690000000000001,-0.685,-0.68,-0.675,-0.67,-0.665,
-0.66,-0.655,-0.65,-0.645,-0.64,-0.635,-0.63,-0.625,-0.62,-0.615,-0.61,
-0.605,-0.6,-0.595,-0.59,-0.585,-0.58,-0.575,-0.57,-0.565,-0.56,-0.555,
-0.55,-0.545,-0.54,-0.535,-0.53,-0.525,-0.52,-0.515,-0.51,-0.505,-0.5,-0.495,
-0.49,-0.485,-0.48,-0.475,-0.47,-0.465,-0.46,-0.455,-0.45,-0.445,-0.44,
-0.435,-0.43,-0.425,-0.42,-0.415,-0.41,-0.405,-0.4,-0.395,-0.39,-0.385,
-0.38,-0.375,-0.37,-0.365,-0.36,-0.355,-0.35,-0.345,-0.34,-0.335,-0.33,
-0.325,-0.32,-0.315,-0.31,-0.305,-0.3,-0.295,-0.29,-0.285,-0.28,-0.275,
-0.27,-0.265,-0.26,-0.255,-0.25,-0.245,-0.24,-0.235,-0.23,-0.225,-0.22,
-0.215,-0.21,-0.205,-0.2,-0.195,-0.19,-0.185,-0.18,-0.175,-0.17,-0.165,
-0.16,-0.155,-0.15,-0.145,-0.14,-0.135,-0.13,-0.125,-0.12,-0.115,-0.11,
-0.105,-0.1,-0.095,-0.09,-0.085,-0.08,-0.075,-0.07,-0.065,-0.06,-0.055,
-0.05,-0.045,-0.04,-0.035,-0.03,-0.025,-0.02,-0.015,-0.01,-0.005,0.),
 .UNSPECIFIED.)
CURVE()
GEOMETRIC_REPRESENTATION_ITEM()
RATIONAL_B_SPLINE_CURVE((1.,1.,1.,1.,1.,1.,1.,1.,1.,1.,1.,1.,1.,1.,1.,1.,
1.,1.,1.,1.,1.,1.,1.,1.,1.,1.,1.,1.,1.,1.,1.,1.,1.,1.,1.,1.,1.,1.,1.,1.,
1.,1.,1.,1.,1.,1.,1.,1.,1.,1.,1.,1.,1.,1.,1.,1.,1.,1.,1.,1.,1.,1.,1.,1.,
1.,1.,1.,1.,1.,1.,1.,1.,1.,1.,1.,1.,1.,1.,1.,1.,1.,1.,1.,1.,1.,1.,1.,1.,
1.,1.,1.,1.,1.,1.,1.,1.,1.,1.,1.,1.,1.,1.,1.,1.,1.,1.,1.,1.,1.,1.,1.,1.,
1.,1.,1.,1.,1.,1.,1.,1.,1.,1.,1.,1.,1.,1.,1.,1.,1.,1.,1.,1.,1.,1.,1.,1.,
1.,1.,1.,1.,1.,1.,1.,1.,1.,1.,1.,1.,1.,1.,1.,1.,1.,1.,1.,1.,1.,1.,1.,1.,
1.,1.,1.,1.,1.,1.,1.,1.,1.,1.,1.,1.,1.,1.,1.,1.,1.,1.,1.,1.,1.,1.,1.,1.,
1.,1.,1.,1.,1.,1.,1.,1.,1.,1.,1.,1.,1.,1.,1.,1.,1.,1.,1.,1.,1.))
REPRESENTATION_ITEM('')
);
#737=(
BOUNDED_CURVE()
B_SPLINE_CURVE(5,(#184765,#184766,#184767,#184768,#184769,#184770,#184771,
#184772,#184773,#184774,#184775,#184776,#184777,#184778,#184779,#184780,
#184781,#184782,#184783,#184784,#184785,#184786,#184787,#184788,#184789,
#184790,#184791,#184792,#184793,#184794,#184795,#184796,#184797,#184798,
#184799,#184800,#184801,#184802,#184803,#184804,#184805,#184806,#184807,
#184808,#184809,#184810,#184811,#184812,#184813,#184814,#184815,#184816,
#184817,#184818,#184819,#184820,#184821,#184822,#184823,#184824,#184825,
#184826,#184827,#184828,#184829,#184830,#184831,#184832,#184833,#184834,
#184835,#184836,#184837,#184838,#184839,#184840,#184841,#184842,#184843,
#184844,#184845,#184846,#184847,#184848,#184849,#184850,#184851,#184852,
#184853,#184854,#184855,#184856,#184857,#184858,#184859,#184860,#184861,
#184862,#184863,#184864,#184865,#184866,#184867,#184868,#184869,#184870,
#184871,#184872,#184873,#184874,#184875,#184876,#184877,#184878,#184879,
#184880,#184881,#184882,#184883,#184884,#184885,#184886,#184887,#184888,
#184889,#184890,#184891,#184892,#184893,#184894,#184895,#184896,#184897,
#184898,#184899,#184900,#184901,#184902,#184903,#184904,#184905,#184906,
#184907,#184908,#184909,#184910,#184911,#184912,#184913,#184914,#184915,
#184916,#184917,#184918,#184919,#184920,#184921,#184922,#184923,#184924,
#184925,#184926,#184927,#184928,#184929,#184930,#184931,#184932,#184933,
#184934,#184935,#184936,#184937,#184938,#184939,#184940,#184941,#184942,
#184943,#184944,#184945,#184946,#184947,#184948,#184949,#184950,#184951,
#184952,#184953,#184954,#184955,#184956,#184957,#184958,#184959,#184960,
#184961,#184962,#184963,#184964,#184965,#184966,#184967,#184968,#184969),
 .UNSPECIFIED.,.F.,.F.)
B_SPLINE_CURVE_WITH_KNOTS((6,1,1,1,1,1,1,1,1,1,1,1,1,1,1,1,1,1,1,1,1,1,
1,1,1,1,1,1,1,1,1,1,1,1,1,1,1,1,1,1,1,1,1,1,1,1,1,1,1,1,1,1,1,1,1,1,1,1,
1,1,1,1,1,1,1,1,1,1,1,1,1,1,1,1,1,1,1,1,1,1,1,1,1,1,1,1,1,1,1,1,1,1,1,1,
1,1,1,1,1,1,1,1,1,1,1,1,1,1,1,1,1,1,1,1,1,1,1,1,1,1,1,1,1,1,1,1,1,1,1,1,
1,1,1,1,1,1,1,1,1,1,1,1,1,1,1,1,1,1,1,1,1,1,1,1,1,1,1,1,1,1,1,1,1,1,1,1,
1,1,1,1,1,1,1,1,1,1,1,1,1,1,1,1,1,1,1,1,1,1,1,1,1,1,1,1,1,1,1,1,1,1,6),
(0.,0.005,0.01,0.015,0.02,0.025,0.03,0.035,0.04,0.045,0.05,0.055,0.06,0.065,
0.07,0.075,0.08,0.085,0.09,0.095,0.1,0.105,0.11,0.115,0.12,0.125,0.13,0.135,
0.14,0.145,0.15,0.155,0.16,0.165,0.17,0.175,0.18,0.185,0.19,0.195,0.2,0.205,
0.21,0.215,0.22,0.225,0.23,0.235,0.24,0.245,0.25,0.255,0.26,0.265,0.27,
0.275,0.28,0.285,0.29,0.295,0.3,0.305,0.31,0.315,0.32,0.325,0.33,0.335,
0.34,0.345,0.35,0.355,0.36,0.365,0.37,0.375,0.38,0.385,0.39,0.395,0.4,0.405,
0.41,0.415,0.42,0.425,0.43,0.435,0.44,0.445,0.45,0.455,0.46,0.465,0.47,
0.475,0.48,0.485,0.49,0.495,0.5,0.505,0.51,0.515,0.52,0.525,0.53,0.535,
0.54,0.545,0.55,0.555,0.56,0.565,0.57,0.575,0.58,0.585,0.59,0.595,0.6,0.605,
0.61,0.615,0.62,0.625,0.63,0.635,0.64,0.645,0.65,0.655,0.66,0.665,0.67,
0.675,0.68,0.685,0.690000000000001,0.695000000000001,0.700000000000001,
0.705000000000001,0.710000000000001,0.715000000000001,0.720000000000001,
0.725000000000001,0.730000000000001,0.735000000000001,0.740000000000001,
0.745000000000001,0.750000000000001,0.755000000000001,0.760000000000001,
0.765000000000001,0.770000000000001,0.775000000000001,0.780000000000001,
0.785000000000001,0.790000000000001,0.795000000000001,0.800000000000001,
0.805000000000001,0.810000000000001,0.815000000000001,0.820000000000001,
0.825000000000001,0.830000000000001,0.835000000000001,0.840000000000001,
0.845000000000001,0.850000000000001,0.855000000000001,0.860000000000001,
0.865000000000001,0.870000000000001,0.875000000000001,0.880000000000001,
0.885000000000001,0.890000000000001,0.895000000000001,0.900000000000001,
0.905000000000001,0.910000000000001,0.915000000000001,0.920000000000001,
0.925000000000001,0.930000000000001,0.935000000000001,0.940000000000001,
0.945000000000001,0.950000000000001,0.955000000000001,0.960000000000001,
0.965000000000001,0.970000000000001,0.975000000000001,0.980000000000001,
0.985000000000001,0.990000000000001,0.995000000000001,1.),.UNSPECIFIED.)
CURVE()
GEOMETRIC_REPRESENTATION_ITEM()
RATIONAL_B_SPLINE_CURVE((1.,1.,1.,1.,1.,1.,1.,1.,1.,1.,1.,1.,1.,1.,1.,1.,
1.,1.,1.,1.,1.,1.,1.,1.,1.,1.,1.,1.,1.,1.,1.,1.,1.,1.,1.,1.,1.,1.,1.,1.,
1.,1.,1.,1.,1.,1.,1.,1.,1.,1.,1.,1.,1.,1.,1.,1.,1.,1.,1.,1.,1.,1.,1.,1.,
1.,1.,1.,1.,1.,1.,1.,1.,1.,1.,1.,1.,1.,1.,1.,1.,1.,1.,1.,1.,1.,1.,1.,1.,
1.,1.,1.,1.,1.,1.,1.,1.,1.,1.,1.,1.,1.,1.,1.,1.,1.,1.,1.,1.,1.,1.,1.,1.,
1.,1.,1.,1.,1.,1.,1.,1.,1.,1.,1.,1.,1.,1.,1.,1.,1.,1.,1.,1.,1.,1.,1.,1.,
1.,1.,1.,1.,1.,1.,1.,1.,1.,1.,1.,1.,1.,1.,1.,1.,1.,1.,1.,1.,1.,1.,1.,1.,
1.,1.,1.,1.,1.,1.,1.,1.,1.,1.,1.,1.,1.,1.,1.,1.,1.,1.,1.,1.,1.,1.,1.,1.,
1.,1.,1.,1.,1.,1.,1.,1.,1.,1.,1.,1.,1.,1.,1.,1.,1.,1.,1.,1.,1.))
REPRESENTATION_ITEM('')
);
#738=(
BOUNDED_CURVE()
B_SPLINE_CURVE(5,(#184973,#184974,#184975,#184976,#184977,#184978,#184979,
#184980,#184981,#184982,#184983,#184984,#184985,#184986,#184987,#184988,
#184989,#184990,#184991,#184992,#184993,#184994,#184995,#184996,#184997,
#184998,#184999,#185000,#185001,#185002,#185003,#185004,#185005,#185006,
#185007,#185008,#185009,#185010,#185011,#185012,#185013,#185014,#185015,
#185016,#185017,#185018,#185019,#185020,#185021,#185022,#185023,#185024,
#185025,#185026,#185027,#185028,#185029,#185030,#185031,#185032,#185033,
#185034,#185035,#185036,#185037,#185038,#185039,#185040,#185041,#185042,
#185043,#185044,#185045,#185046,#185047,#185048,#185049,#185050,#185051,
#185052,#185053,#185054,#185055,#185056,#185057,#185058,#185059,#185060,
#185061,#185062,#185063,#185064,#185065,#185066,#185067,#185068,#185069,
#185070,#185071,#185072,#185073,#185074,#185075,#185076,#185077,#185078,
#185079,#185080,#185081,#185082,#185083,#185084,#185085,#185086,#185087,
#185088,#185089,#185090,#185091,#185092,#185093,#185094,#185095,#185096,
#185097,#185098,#185099,#185100,#185101,#185102,#185103,#185104,#185105,
#185106,#185107,#185108,#185109,#185110,#185111,#185112,#185113,#185114,
#185115,#185116,#185117,#185118,#185119,#185120,#185121,#185122,#185123,
#185124,#185125,#185126,#185127,#185128,#185129,#185130,#185131,#185132,
#185133,#185134,#185135,#185136,#185137,#185138,#185139,#185140,#185141,
#185142,#185143,#185144,#185145,#185146,#185147,#185148,#185149,#185150,
#185151,#185152,#185153,#185154,#185155,#185156,#185157,#185158,#185159,
#185160,#185161,#185162,#185163,#185164,#185165,#185166,#185167,#185168,
#185169,#185170,#185171,#185172,#185173,#185174,#185175,#185176,#185177),
 .UNSPECIFIED.,.F.,.F.)
B_SPLINE_CURVE_WITH_KNOTS((6,1,1,1,1,1,1,1,1,1,1,1,1,1,1,1,1,1,1,1,1,1,
1,1,1,1,1,1,1,1,1,1,1,1,1,1,1,1,1,1,1,1,1,1,1,1,1,1,1,1,1,1,1,1,1,1,1,1,
1,1,1,1,1,1,1,1,1,1,1,1,1,1,1,1,1,1,1,1,1,1,1,1,1,1,1,1,1,1,1,1,1,1,1,1,
1,1,1,1,1,1,1,1,1,1,1,1,1,1,1,1,1,1,1,1,1,1,1,1,1,1,1,1,1,1,1,1,1,1,1,1,
1,1,1,1,1,1,1,1,1,1,1,1,1,1,1,1,1,1,1,1,1,1,1,1,1,1,1,1,1,1,1,1,1,1,1,1,
1,1,1,1,1,1,1,1,1,1,1,1,1,1,1,1,1,1,1,1,1,1,1,1,1,1,1,1,1,1,1,1,1,1,6),
(-1.,-0.995000000000001,-0.990000000000001,-0.985000000000001,-0.980000000000001,
-0.975000000000001,-0.970000000000001,-0.965000000000001,-0.960000000000001,
-0.955000000000001,-0.950000000000001,-0.945000000000001,-0.940000000000001,
-0.935000000000001,-0.930000000000001,-0.925000000000001,-0.920000000000001,
-0.915000000000001,-0.910000000000001,-0.905000000000001,-0.900000000000001,
-0.895000000000001,-0.890000000000001,-0.885000000000001,-0.880000000000001,
-0.875000000000001,-0.870000000000001,-0.865000000000001,-0.860000000000001,
-0.855000000000001,-0.850000000000001,-0.845000000000001,-0.840000000000001,
-0.835000000000001,-0.830000000000001,-0.825000000000001,-0.820000000000001,
-0.815000000000001,-0.810000000000001,-0.805000000000001,-0.800000000000001,
-0.795000000000001,-0.790000000000001,-0.785000000000001,-0.780000000000001,
-0.775000000000001,-0.770000000000001,-0.765000000000001,-0.760000000000001,
-0.755000000000001,-0.750000000000001,-0.745000000000001,-0.740000000000001,
-0.735000000000001,-0.730000000000001,-0.725000000000001,-0.720000000000001,
-0.715000000000001,-0.710000000000001,-0.705000000000001,-0.700000000000001,
-0.695000000000001,-0.690000000000001,-0.685,-0.68,-0.675,-0.67,-0.665,
-0.66,-0.655,-0.65,-0.645,-0.64,-0.635,-0.63,-0.625,-0.62,-0.615,-0.61,
-0.605,-0.6,-0.595,-0.59,-0.585,-0.58,-0.575,-0.57,-0.565,-0.56,-0.555,
-0.55,-0.545,-0.54,-0.535,-0.53,-0.525,-0.52,-0.515,-0.51,-0.505,-0.5,-0.495,
-0.49,-0.485,-0.48,-0.475,-0.47,-0.465,-0.46,-0.455,-0.45,-0.445,-0.44,
-0.435,-0.43,-0.425,-0.42,-0.415,-0.41,-0.405,-0.4,-0.395,-0.39,-0.385,
-0.38,-0.375,-0.37,-0.365,-0.36,-0.355,-0.35,-0.345,-0.34,-0.335,-0.33,
-0.325,-0.32,-0.315,-0.31,-0.305,-0.3,-0.295,-0.29,-0.285,-0.28,-0.275,
-0.27,-0.265,-0.26,-0.255,-0.25,-0.245,-0.24,-0.235,-0.23,-0.225,-0.22,
-0.215,-0.21,-0.205,-0.2,-0.195,-0.19,-0.185,-0.18,-0.175,-0.17,-0.165,
-0.16,-0.155,-0.15,-0.145,-0.14,-0.135,-0.13,-0.125,-0.12,-0.115,-0.11,
-0.105,-0.1,-0.095,-0.09,-0.085,-0.08,-0.075,-0.07,-0.065,-0.06,-0.055,
-0.05,-0.045,-0.04,-0.035,-0.03,-0.025,-0.02,-0.015,-0.01,-0.005,0.),
 .UNSPECIFIED.)
CURVE()
GEOMETRIC_REPRESENTATION_ITEM()
RATIONAL_B_SPLINE_CURVE((1.,1.,1.,1.,1.,1.,1.,1.,1.,1.,1.,1.,1.,1.,1.,1.,
1.,1.,1.,1.,1.,1.,1.,1.,1.,1.,1.,1.,1.,1.,1.,1.,1.,1.,1.,1.,1.,1.,1.,1.,
1.,1.,1.,1.,1.,1.,1.,1.,1.,1.,1.,1.,1.,1.,1.,1.,1.,1.,1.,1.,1.,1.,1.,1.,
1.,1.,1.,1.,1.,1.,1.,1.,1.,1.,1.,1.,1.,1.,1.,1.,1.,1.,1.,1.,1.,1.,1.,1.,
1.,1.,1.,1.,1.,1.,1.,1.,1.,1.,1.,1.,1.,1.,1.,1.,1.,1.,1.,1.,1.,1.,1.,1.,
1.,1.,1.,1.,1.,1.,1.,1.,1.,1.,1.,1.,1.,1.,1.,1.,1.,1.,1.,1.,1.,1.,1.,1.,
1.,1.,1.,1.,1.,1.,1.,1.,1.,1.,1.,1.,1.,1.,1.,1.,1.,1.,1.,1.,1.,1.,1.,1.,
1.,1.,1.,1.,1.,1.,1.,1.,1.,1.,1.,1.,1.,1.,1.,1.,1.,1.,1.,1.,1.,1.,1.,1.,
1.,1.,1.,1.,1.,1.,1.,1.,1.,1.,1.,1.,1.,1.,1.,1.,1.,1.,1.,1.,1.))
REPRESENTATION_ITEM('')
);
#739=(
BOUNDED_CURVE()
B_SPLINE_CURVE(5,(#186016,#186017,#186018,#186019,#186020,#186021,#186022,
#186023,#186024,#186025,#186026,#186027,#186028,#186029,#186030,#186031,
#186032,#186033,#186034,#186035,#186036,#186037,#186038,#186039,#186040,
#186041,#186042,#186043,#186044,#186045,#186046,#186047,#186048,#186049,
#186050,#186051,#186052,#186053,#186054,#186055,#186056,#186057,#186058,
#186059,#186060,#186061,#186062,#186063,#186064,#186065,#186066,#186067,
#186068,#186069,#186070,#186071,#186072,#186073,#186074,#186075,#186076,
#186077,#186078,#186079,#186080,#186081,#186082,#186083,#186084,#186085,
#186086,#186087,#186088,#186089,#186090,#186091,#186092,#186093,#186094,
#186095,#186096,#186097,#186098,#186099,#186100,#186101,#186102,#186103,
#186104,#186105,#186106,#186107,#186108,#186109,#186110,#186111,#186112,
#186113,#186114,#186115,#186116,#186117,#186118,#186119,#186120,#186121,
#186122,#186123,#186124,#186125,#186126,#186127,#186128,#186129,#186130,
#186131,#186132,#186133,#186134,#186135,#186136,#186137,#186138,#186139,
#186140,#186141,#186142,#186143,#186144,#186145,#186146,#186147,#186148,
#186149,#186150,#186151,#186152,#186153,#186154,#186155,#186156,#186157,
#186158,#186159,#186160,#186161,#186162,#186163,#186164,#186165,#186166,
#186167,#186168,#186169,#186170,#186171,#186172,#186173,#186174,#186175,
#186176,#186177,#186178,#186179,#186180,#186181,#186182,#186183,#186184,
#186185,#186186,#186187,#186188,#186189,#186190,#186191,#186192,#186193,
#186194,#186195,#186196,#186197,#186198,#186199,#186200,#186201,#186202,
#186203,#186204,#186205,#186206,#186207,#186208,#186209,#186210,#186211,
#186212,#186213,#186214,#186215,#186216,#186217,#186218,#186219,#186220),
 .UNSPECIFIED.,.F.,.F.)
B_SPLINE_CURVE_WITH_KNOTS((6,1,1,1,1,1,1,1,1,1,1,1,1,1,1,1,1,1,1,1,1,1,
1,1,1,1,1,1,1,1,1,1,1,1,1,1,1,1,1,1,1,1,1,1,1,1,1,1,1,1,1,1,1,1,1,1,1,1,
1,1,1,1,1,1,1,1,1,1,1,1,1,1,1,1,1,1,1,1,1,1,1,1,1,1,1,1,1,1,1,1,1,1,1,1,
1,1,1,1,1,1,1,1,1,1,1,1,1,1,1,1,1,1,1,1,1,1,1,1,1,1,1,1,1,1,1,1,1,1,1,1,
1,1,1,1,1,1,1,1,1,1,1,1,1,1,1,1,1,1,1,1,1,1,1,1,1,1,1,1,1,1,1,1,1,1,1,1,
1,1,1,1,1,1,1,1,1,1,1,1,1,1,1,1,1,1,1,1,1,1,1,1,1,1,1,1,1,1,1,1,1,1,6),
(-1.,-0.995000000000001,-0.990000000000001,-0.985000000000001,-0.980000000000001,
-0.975000000000001,-0.970000000000001,-0.965000000000001,-0.960000000000001,
-0.955000000000001,-0.950000000000001,-0.945000000000001,-0.940000000000001,
-0.935000000000001,-0.930000000000001,-0.925000000000001,-0.920000000000001,
-0.915000000000001,-0.910000000000001,-0.905000000000001,-0.900000000000001,
-0.895000000000001,-0.890000000000001,-0.885000000000001,-0.880000000000001,
-0.875000000000001,-0.870000000000001,-0.865000000000001,-0.860000000000001,
-0.855000000000001,-0.850000000000001,-0.845000000000001,-0.840000000000001,
-0.835000000000001,-0.830000000000001,-0.825000000000001,-0.820000000000001,
-0.815000000000001,-0.810000000000001,-0.805000000000001,-0.800000000000001,
-0.795000000000001,-0.790000000000001,-0.785000000000001,-0.780000000000001,
-0.775000000000001,-0.770000000000001,-0.765000000000001,-0.760000000000001,
-0.755000000000001,-0.750000000000001,-0.745000000000001,-0.740000000000001,
-0.735000000000001,-0.730000000000001,-0.725000000000001,-0.720000000000001,
-0.715000000000001,-0.710000000000001,-0.705000000000001,-0.700000000000001,
-0.695000000000001,-0.690000000000001,-0.685,-0.68,-0.675,-0.67,-0.665,
-0.66,-0.655,-0.65,-0.645,-0.64,-0.635,-0.63,-0.625,-0.62,-0.615,-0.61,
-0.605,-0.6,-0.595,-0.59,-0.585,-0.58,-0.575,-0.57,-0.565,-0.56,-0.555,
-0.55,-0.545,-0.54,-0.535,-0.53,-0.525,-0.52,-0.515,-0.51,-0.505,-0.5,-0.495,
-0.49,-0.485,-0.48,-0.475,-0.47,-0.465,-0.46,-0.455,-0.45,-0.445,-0.44,
-0.435,-0.43,-0.425,-0.42,-0.415,-0.41,-0.405,-0.4,-0.395,-0.39,-0.385,
-0.38,-0.375,-0.37,-0.365,-0.36,-0.355,-0.35,-0.345,-0.34,-0.335,-0.33,
-0.325,-0.32,-0.315,-0.31,-0.305,-0.3,-0.295,-0.29,-0.285,-0.28,-0.275,
-0.27,-0.265,-0.26,-0.255,-0.25,-0.245,-0.24,-0.235,-0.23,-0.225,-0.22,
-0.215,-0.21,-0.205,-0.2,-0.195,-0.19,-0.185,-0.18,-0.175,-0.17,-0.165,
-0.16,-0.155,-0.15,-0.145,-0.14,-0.135,-0.13,-0.125,-0.12,-0.115,-0.11,
-0.105,-0.1,-0.095,-0.09,-0.085,-0.08,-0.075,-0.07,-0.065,-0.06,-0.055,
-0.05,-0.045,-0.04,-0.035,-0.03,-0.025,-0.02,-0.015,-0.01,-0.005,0.),
 .UNSPECIFIED.)
CURVE()
GEOMETRIC_REPRESENTATION_ITEM()
RATIONAL_B_SPLINE_CURVE((1.,1.,1.,1.,1.,1.,1.,1.,1.,1.,1.,1.,1.,1.,1.,1.,
1.,1.,1.,1.,1.,1.,1.,1.,1.,1.,1.,1.,1.,1.,1.,1.,1.,1.,1.,1.,1.,1.,1.,1.,
1.,1.,1.,1.,1.,1.,1.,1.,1.,1.,1.,1.,1.,1.,1.,1.,1.,1.,1.,1.,1.,1.,1.,1.,
1.,1.,1.,1.,1.,1.,1.,1.,1.,1.,1.,1.,1.,1.,1.,1.,1.,1.,1.,1.,1.,1.,1.,1.,
1.,1.,1.,1.,1.,1.,1.,1.,1.,1.,1.,1.,1.,1.,1.,1.,1.,1.,1.,1.,1.,1.,1.,1.,
1.,1.,1.,1.,1.,1.,1.,1.,1.,1.,1.,1.,1.,1.,1.,1.,1.,1.,1.,1.,1.,1.,1.,1.,
1.,1.,1.,1.,1.,1.,1.,1.,1.,1.,1.,1.,1.,1.,1.,1.,1.,1.,1.,1.,1.,1.,1.,1.,
1.,1.,1.,1.,1.,1.,1.,1.,1.,1.,1.,1.,1.,1.,1.,1.,1.,1.,1.,1.,1.,1.,1.,1.,
1.,1.,1.,1.,1.,1.,1.,1.,1.,1.,1.,1.,1.,1.,1.,1.,1.,1.,1.,1.,1.))
REPRESENTATION_ITEM('')
);
#740=(
BOUNDED_CURVE()
B_SPLINE_CURVE(5,(#186633,#186634,#186635,#186636,#186637,#186638,#186639,
#186640,#186641,#186642,#186643,#186644,#186645,#186646,#186647,#186648,
#186649,#186650,#186651,#186652,#186653,#186654,#186655,#186656,#186657,
#186658,#186659,#186660,#186661,#186662,#186663,#186664,#186665,#186666,
#186667,#186668,#186669,#186670,#186671,#186672,#186673,#186674,#186675,
#186676,#186677,#186678,#186679,#186680,#186681,#186682,#186683,#186684,
#186685,#186686,#186687,#186688,#186689,#186690,#186691,#186692,#186693,
#186694,#186695,#186696,#186697,#186698,#186699,#186700,#186701,#186702,
#186703,#186704,#186705,#186706,#186707,#186708,#186709,#186710,#186711,
#186712,#186713,#186714,#186715,#186716,#186717,#186718,#186719,#186720,
#186721,#186722,#186723,#186724,#186725,#186726,#186727,#186728,#186729,
#186730,#186731,#186732,#186733,#186734,#186735,#186736,#186737,#186738,
#186739,#186740,#186741,#186742,#186743,#186744,#186745,#186746,#186747,
#186748,#186749,#186750,#186751,#186752,#186753,#186754,#186755,#186756,
#186757,#186758,#186759,#186760,#186761,#186762,#186763,#186764,#186765,
#186766,#186767,#186768,#186769,#186770,#186771,#186772,#186773,#186774,
#186775,#186776,#186777,#186778,#186779,#186780,#186781,#186782,#186783,
#186784,#186785,#186786,#186787,#186788,#186789,#186790,#186791,#186792,
#186793,#186794,#186795,#186796,#186797,#186798,#186799,#186800,#186801,
#186802,#186803,#186804,#186805,#186806,#186807,#186808,#186809,#186810,
#186811,#186812,#186813,#186814,#186815,#186816,#186817,#186818,#186819,
#186820,#186821,#186822,#186823,#186824,#186825,#186826,#186827,#186828,
#186829,#186830,#186831,#186832,#186833,#186834,#186835,#186836,#186837),
 .UNSPECIFIED.,.F.,.F.)
B_SPLINE_CURVE_WITH_KNOTS((6,1,1,1,1,1,1,1,1,1,1,1,1,1,1,1,1,1,1,1,1,1,
1,1,1,1,1,1,1,1,1,1,1,1,1,1,1,1,1,1,1,1,1,1,1,1,1,1,1,1,1,1,1,1,1,1,1,1,
1,1,1,1,1,1,1,1,1,1,1,1,1,1,1,1,1,1,1,1,1,1,1,1,1,1,1,1,1,1,1,1,1,1,1,1,
1,1,1,1,1,1,1,1,1,1,1,1,1,1,1,1,1,1,1,1,1,1,1,1,1,1,1,1,1,1,1,1,1,1,1,1,
1,1,1,1,1,1,1,1,1,1,1,1,1,1,1,1,1,1,1,1,1,1,1,1,1,1,1,1,1,1,1,1,1,1,1,1,
1,1,1,1,1,1,1,1,1,1,1,1,1,1,1,1,1,1,1,1,1,1,1,1,1,1,1,1,1,1,1,1,1,1,6),
(0.,0.005,0.01,0.015,0.02,0.025,0.03,0.035,0.04,0.045,0.05,0.055,0.06,0.065,
0.07,0.075,0.08,0.085,0.09,0.095,0.1,0.105,0.11,0.115,0.12,0.125,0.13,0.135,
0.14,0.145,0.15,0.155,0.16,0.165,0.17,0.175,0.18,0.185,0.19,0.195,0.2,0.205,
0.21,0.215,0.22,0.225,0.23,0.235,0.24,0.245,0.25,0.255,0.26,0.265,0.27,
0.275,0.28,0.285,0.29,0.295,0.3,0.305,0.31,0.315,0.32,0.325,0.33,0.335,
0.34,0.345,0.35,0.355,0.36,0.365,0.37,0.375,0.38,0.385,0.39,0.395,0.4,0.405,
0.41,0.415,0.42,0.425,0.43,0.435,0.44,0.445,0.45,0.455,0.46,0.465,0.47,
0.475,0.48,0.485,0.49,0.495,0.5,0.505,0.51,0.515,0.52,0.525,0.53,0.535,
0.54,0.545,0.55,0.555,0.56,0.565,0.57,0.575,0.58,0.585,0.59,0.595,0.6,0.605,
0.61,0.615,0.62,0.625,0.63,0.635,0.64,0.645,0.65,0.655,0.66,0.665,0.67,
0.675,0.68,0.685,0.690000000000001,0.695000000000001,0.700000000000001,
0.705000000000001,0.710000000000001,0.715000000000001,0.720000000000001,
0.725000000000001,0.730000000000001,0.735000000000001,0.740000000000001,
0.745000000000001,0.750000000000001,0.755000000000001,0.760000000000001,
0.765000000000001,0.770000000000001,0.775000000000001,0.780000000000001,
0.785000000000001,0.790000000000001,0.795000000000001,0.800000000000001,
0.805000000000001,0.810000000000001,0.815000000000001,0.820000000000001,
0.825000000000001,0.830000000000001,0.835000000000001,0.840000000000001,
0.845000000000001,0.850000000000001,0.855000000000001,0.860000000000001,
0.865000000000001,0.870000000000001,0.875000000000001,0.880000000000001,
0.885000000000001,0.890000000000001,0.895000000000001,0.900000000000001,
0.905000000000001,0.910000000000001,0.915000000000001,0.920000000000001,
0.925000000000001,0.930000000000001,0.935000000000001,0.940000000000001,
0.945000000000001,0.950000000000001,0.955000000000001,0.960000000000001,
0.965000000000001,0.970000000000001,0.975000000000001,0.980000000000001,
0.985000000000001,0.990000000000001,0.995000000000001,1.),.UNSPECIFIED.)
CURVE()
GEOMETRIC_REPRESENTATION_ITEM()
RATIONAL_B_SPLINE_CURVE((1.,1.,1.,1.,1.,1.,1.,1.,1.,1.,1.,1.,1.,1.,1.,1.,
1.,1.,1.,1.,1.,1.,1.,1.,1.,1.,1.,1.,1.,1.,1.,1.,1.,1.,1.,1.,1.,1.,1.,1.,
1.,1.,1.,1.,1.,1.,1.,1.,1.,1.,1.,1.,1.,1.,1.,1.,1.,1.,1.,1.,1.,1.,1.,1.,
1.,1.,1.,1.,1.,1.,1.,1.,1.,1.,1.,1.,1.,1.,1.,1.,1.,1.,1.,1.,1.,1.,1.,1.,
1.,1.,1.,1.,1.,1.,1.,1.,1.,1.,1.,1.,1.,1.,1.,1.,1.,1.,1.,1.,1.,1.,1.,1.,
1.,1.,1.,1.,1.,1.,1.,1.,1.,1.,1.,1.,1.,1.,1.,1.,1.,1.,1.,1.,1.,1.,1.,1.,
1.,1.,1.,1.,1.,1.,1.,1.,1.,1.,1.,1.,1.,1.,1.,1.,1.,1.,1.,1.,1.,1.,1.,1.,
1.,1.,1.,1.,1.,1.,1.,1.,1.,1.,1.,1.,1.,1.,1.,1.,1.,1.,1.,1.,1.,1.,1.,1.,
1.,1.,1.,1.,1.,1.,1.,1.,1.,1.,1.,1.,1.,1.,1.,1.,1.,1.,1.,1.,1.))
REPRESENTATION_ITEM('')
);
#741=(
BOUNDED_CURVE()
B_SPLINE_CURVE(5,(#187254,#187255,#187256,#187257,#187258,#187259,#187260,
#187261,#187262,#187263,#187264,#187265,#187266,#187267,#187268,#187269,
#187270,#187271,#187272,#187273,#187274,#187275,#187276,#187277,#187278,
#187279,#187280,#187281,#187282,#187283,#187284,#187285,#187286,#187287,
#187288,#187289,#187290,#187291,#187292,#187293,#187294,#187295,#187296,
#187297,#187298,#187299,#187300,#187301,#187302,#187303,#187304,#187305,
#187306,#187307,#187308,#187309,#187310,#187311,#187312,#187313,#187314,
#187315,#187316,#187317,#187318,#187319,#187320,#187321,#187322,#187323,
#187324,#187325,#187326,#187327,#187328,#187329,#187330,#187331,#187332,
#187333,#187334,#187335,#187336,#187337,#187338,#187339,#187340,#187341,
#187342,#187343,#187344,#187345,#187346,#187347,#187348,#187349,#187350,
#187351,#187352,#187353,#187354,#187355,#187356,#187357,#187358,#187359,
#187360,#187361,#187362,#187363,#187364,#187365,#187366,#187367,#187368,
#187369,#187370,#187371,#187372,#187373,#187374,#187375,#187376,#187377,
#187378,#187379,#187380,#187381,#187382,#187383,#187384,#187385,#187386,
#187387,#187388,#187389,#187390,#187391,#187392,#187393,#187394,#187395,
#187396,#187397,#187398,#187399,#187400,#187401,#187402,#187403,#187404,
#187405,#187406,#187407,#187408,#187409,#187410,#187411,#187412,#187413,
#187414,#187415,#187416,#187417,#187418,#187419,#187420,#187421,#187422,
#187423,#187424,#187425,#187426,#187427,#187428,#187429,#187430,#187431,
#187432,#187433,#187434,#187435,#187436,#187437,#187438,#187439,#187440,
#187441,#187442,#187443,#187444,#187445,#187446,#187447,#187448,#187449,
#187450,#187451,#187452,#187453,#187454,#187455,#187456,#187457,#187458),
 .UNSPECIFIED.,.F.,.F.)
B_SPLINE_CURVE_WITH_KNOTS((6,1,1,1,1,1,1,1,1,1,1,1,1,1,1,1,1,1,1,1,1,1,
1,1,1,1,1,1,1,1,1,1,1,1,1,1,1,1,1,1,1,1,1,1,1,1,1,1,1,1,1,1,1,1,1,1,1,1,
1,1,1,1,1,1,1,1,1,1,1,1,1,1,1,1,1,1,1,1,1,1,1,1,1,1,1,1,1,1,1,1,1,1,1,1,
1,1,1,1,1,1,1,1,1,1,1,1,1,1,1,1,1,1,1,1,1,1,1,1,1,1,1,1,1,1,1,1,1,1,1,1,
1,1,1,1,1,1,1,1,1,1,1,1,1,1,1,1,1,1,1,1,1,1,1,1,1,1,1,1,1,1,1,1,1,1,1,1,
1,1,1,1,1,1,1,1,1,1,1,1,1,1,1,1,1,1,1,1,1,1,1,1,1,1,1,1,1,1,1,1,1,1,6),
(-1.,-0.995000000000001,-0.990000000000001,-0.985000000000001,-0.980000000000001,
-0.975000000000001,-0.970000000000001,-0.965000000000001,-0.960000000000001,
-0.955000000000001,-0.950000000000001,-0.945000000000001,-0.940000000000001,
-0.935000000000001,-0.930000000000001,-0.925000000000001,-0.920000000000001,
-0.915000000000001,-0.910000000000001,-0.905000000000001,-0.900000000000001,
-0.895000000000001,-0.890000000000001,-0.885000000000001,-0.880000000000001,
-0.875000000000001,-0.870000000000001,-0.865000000000001,-0.860000000000001,
-0.855000000000001,-0.850000000000001,-0.845000000000001,-0.840000000000001,
-0.835000000000001,-0.830000000000001,-0.825000000000001,-0.820000000000001,
-0.815000000000001,-0.810000000000001,-0.805000000000001,-0.800000000000001,
-0.795000000000001,-0.790000000000001,-0.785000000000001,-0.780000000000001,
-0.775000000000001,-0.770000000000001,-0.765000000000001,-0.760000000000001,
-0.755000000000001,-0.750000000000001,-0.745000000000001,-0.740000000000001,
-0.735000000000001,-0.730000000000001,-0.725000000000001,-0.720000000000001,
-0.715000000000001,-0.710000000000001,-0.705000000000001,-0.700000000000001,
-0.695000000000001,-0.690000000000001,-0.685,-0.68,-0.675,-0.67,-0.665,
-0.66,-0.655,-0.65,-0.645,-0.64,-0.635,-0.63,-0.625,-0.62,-0.615,-0.61,
-0.605,-0.6,-0.595,-0.59,-0.585,-0.58,-0.575,-0.57,-0.565,-0.56,-0.555,
-0.55,-0.545,-0.54,-0.535,-0.53,-0.525,-0.52,-0.515,-0.51,-0.505,-0.5,-0.495,
-0.49,-0.485,-0.48,-0.475,-0.47,-0.465,-0.46,-0.455,-0.45,-0.445,-0.44,
-0.435,-0.43,-0.425,-0.42,-0.415,-0.41,-0.405,-0.4,-0.395,-0.39,-0.385,
-0.38,-0.375,-0.37,-0.365,-0.36,-0.355,-0.35,-0.345,-0.34,-0.335,-0.33,
-0.325,-0.32,-0.315,-0.31,-0.305,-0.3,-0.295,-0.29,-0.285,-0.28,-0.275,
-0.27,-0.265,-0.26,-0.255,-0.25,-0.245,-0.24,-0.235,-0.23,-0.225,-0.22,
-0.215,-0.21,-0.205,-0.2,-0.195,-0.19,-0.185,-0.18,-0.175,-0.17,-0.165,
-0.16,-0.155,-0.15,-0.145,-0.14,-0.135,-0.13,-0.125,-0.12,-0.115,-0.11,
-0.105,-0.1,-0.095,-0.09,-0.085,-0.08,-0.075,-0.07,-0.065,-0.06,-0.055,
-0.05,-0.045,-0.04,-0.035,-0.03,-0.025,-0.02,-0.015,-0.01,-0.005,0.),
 .UNSPECIFIED.)
CURVE()
GEOMETRIC_REPRESENTATION_ITEM()
RATIONAL_B_SPLINE_CURVE((1.,1.,1.,1.,1.,1.,1.,1.,1.,1.,1.,1.,1.,1.,1.,1.,
1.,1.,1.,1.,1.,1.,1.,1.,1.,1.,1.,1.,1.,1.,1.,1.,1.,1.,1.,1.,1.,1.,1.,1.,
1.,1.,1.,1.,1.,1.,1.,1.,1.,1.,1.,1.,1.,1.,1.,1.,1.,1.,1.,1.,1.,1.,1.,1.,
1.,1.,1.,1.,1.,1.,1.,1.,1.,1.,1.,1.,1.,1.,1.,1.,1.,1.,1.,1.,1.,1.,1.,1.,
1.,1.,1.,1.,1.,1.,1.,1.,1.,1.,1.,1.,1.,1.,1.,1.,1.,1.,1.,1.,1.,1.,1.,1.,
1.,1.,1.,1.,1.,1.,1.,1.,1.,1.,1.,1.,1.,1.,1.,1.,1.,1.,1.,1.,1.,1.,1.,1.,
1.,1.,1.,1.,1.,1.,1.,1.,1.,1.,1.,1.,1.,1.,1.,1.,1.,1.,1.,1.,1.,1.,1.,1.,
1.,1.,1.,1.,1.,1.,1.,1.,1.,1.,1.,1.,1.,1.,1.,1.,1.,1.,1.,1.,1.,1.,1.,1.,
1.,1.,1.,1.,1.,1.,1.,1.,1.,1.,1.,1.,1.,1.,1.,1.,1.,1.,1.,1.,1.))
REPRESENTATION_ITEM('')
);
#742=(
BOUNDED_CURVE()
B_SPLINE_CURVE(5,(#187871,#187872,#187873,#187874,#187875,#187876,#187877,
#187878,#187879,#187880,#187881,#187882,#187883,#187884,#187885,#187886,
#187887,#187888,#187889,#187890,#187891,#187892,#187893,#187894,#187895,
#187896,#187897,#187898,#187899,#187900,#187901,#187902,#187903,#187904,
#187905,#187906,#187907,#187908,#187909,#187910,#187911,#187912,#187913,
#187914,#187915,#187916,#187917,#187918,#187919,#187920,#187921,#187922,
#187923,#187924,#187925,#187926,#187927,#187928,#187929,#187930,#187931,
#187932,#187933,#187934,#187935,#187936,#187937,#187938,#187939,#187940,
#187941,#187942,#187943,#187944,#187945,#187946,#187947,#187948,#187949,
#187950,#187951,#187952,#187953,#187954,#187955,#187956,#187957,#187958,
#187959,#187960,#187961,#187962,#187963,#187964,#187965,#187966,#187967,
#187968,#187969,#187970,#187971,#187972,#187973,#187974,#187975,#187976,
#187977,#187978,#187979,#187980,#187981,#187982,#187983,#187984,#187985,
#187986,#187987,#187988,#187989,#187990,#187991,#187992,#187993,#187994,
#187995,#187996,#187997,#187998,#187999,#188000,#188001,#188002,#188003,
#188004,#188005,#188006,#188007,#188008,#188009,#188010,#188011,#188012,
#188013,#188014,#188015,#188016,#188017,#188018,#188019,#188020,#188021,
#188022,#188023,#188024,#188025,#188026,#188027,#188028,#188029,#188030,
#188031,#188032,#188033,#188034,#188035,#188036,#188037,#188038,#188039,
#188040,#188041,#188042,#188043,#188044,#188045,#188046,#188047,#188048,
#188049,#188050,#188051,#188052,#188053,#188054,#188055,#188056,#188057,
#188058,#188059,#188060,#188061,#188062,#188063,#188064,#188065,#188066,
#188067,#188068,#188069,#188070,#188071,#188072,#188073,#188074,#188075),
 .UNSPECIFIED.,.F.,.F.)
B_SPLINE_CURVE_WITH_KNOTS((6,1,1,1,1,1,1,1,1,1,1,1,1,1,1,1,1,1,1,1,1,1,
1,1,1,1,1,1,1,1,1,1,1,1,1,1,1,1,1,1,1,1,1,1,1,1,1,1,1,1,1,1,1,1,1,1,1,1,
1,1,1,1,1,1,1,1,1,1,1,1,1,1,1,1,1,1,1,1,1,1,1,1,1,1,1,1,1,1,1,1,1,1,1,1,
1,1,1,1,1,1,1,1,1,1,1,1,1,1,1,1,1,1,1,1,1,1,1,1,1,1,1,1,1,1,1,1,1,1,1,1,
1,1,1,1,1,1,1,1,1,1,1,1,1,1,1,1,1,1,1,1,1,1,1,1,1,1,1,1,1,1,1,1,1,1,1,1,
1,1,1,1,1,1,1,1,1,1,1,1,1,1,1,1,1,1,1,1,1,1,1,1,1,1,1,1,1,1,1,1,1,1,6),
(0.,0.005,0.01,0.015,0.02,0.025,0.03,0.035,0.04,0.045,0.05,0.055,0.06,0.065,
0.07,0.075,0.08,0.085,0.09,0.095,0.1,0.105,0.11,0.115,0.12,0.125,0.13,0.135,
0.14,0.145,0.15,0.155,0.16,0.165,0.17,0.175,0.18,0.185,0.19,0.195,0.2,0.205,
0.21,0.215,0.22,0.225,0.23,0.235,0.24,0.245,0.25,0.255,0.26,0.265,0.27,
0.275,0.28,0.285,0.29,0.295,0.3,0.305,0.31,0.315,0.32,0.325,0.33,0.335,
0.34,0.345,0.35,0.355,0.36,0.365,0.37,0.375,0.38,0.385,0.39,0.395,0.4,0.405,
0.41,0.415,0.42,0.425,0.43,0.435,0.44,0.445,0.45,0.455,0.46,0.465,0.47,
0.475,0.48,0.485,0.49,0.495,0.5,0.505,0.51,0.515,0.52,0.525,0.53,0.535,
0.54,0.545,0.55,0.555,0.56,0.565,0.57,0.575,0.58,0.585,0.59,0.595,0.6,0.605,
0.61,0.615,0.62,0.625,0.63,0.635,0.64,0.645,0.65,0.655,0.66,0.665,0.67,
0.675,0.68,0.685,0.690000000000001,0.695000000000001,0.700000000000001,
0.705000000000001,0.710000000000001,0.715000000000001,0.720000000000001,
0.725000000000001,0.730000000000001,0.735000000000001,0.740000000000001,
0.745000000000001,0.750000000000001,0.755000000000001,0.760000000000001,
0.765000000000001,0.770000000000001,0.775000000000001,0.780000000000001,
0.785000000000001,0.790000000000001,0.795000000000001,0.800000000000001,
0.805000000000001,0.810000000000001,0.815000000000001,0.820000000000001,
0.825000000000001,0.830000000000001,0.835000000000001,0.840000000000001,
0.845000000000001,0.850000000000001,0.855000000000001,0.860000000000001,
0.865000000000001,0.870000000000001,0.875000000000001,0.880000000000001,
0.885000000000001,0.890000000000001,0.895000000000001,0.900000000000001,
0.905000000000001,0.910000000000001,0.915000000000001,0.920000000000001,
0.925000000000001,0.930000000000001,0.935000000000001,0.940000000000001,
0.945000000000001,0.950000000000001,0.955000000000001,0.960000000000001,
0.965000000000001,0.970000000000001,0.975000000000001,0.980000000000001,
0.985000000000001,0.990000000000001,0.995000000000001,1.),.UNSPECIFIED.)
CURVE()
GEOMETRIC_REPRESENTATION_ITEM()
RATIONAL_B_SPLINE_CURVE((1.,1.,1.,1.,1.,1.,1.,1.,1.,1.,1.,1.,1.,1.,1.,1.,
1.,1.,1.,1.,1.,1.,1.,1.,1.,1.,1.,1.,1.,1.,1.,1.,1.,1.,1.,1.,1.,1.,1.,1.,
1.,1.,1.,1.,1.,1.,1.,1.,1.,1.,1.,1.,1.,1.,1.,1.,1.,1.,1.,1.,1.,1.,1.,1.,
1.,1.,1.,1.,1.,1.,1.,1.,1.,1.,1.,1.,1.,1.,1.,1.,1.,1.,1.,1.,1.,1.,1.,1.,
1.,1.,1.,1.,1.,1.,1.,1.,1.,1.,1.,1.,1.,1.,1.,1.,1.,1.,1.,1.,1.,1.,1.,1.,
1.,1.,1.,1.,1.,1.,1.,1.,1.,1.,1.,1.,1.,1.,1.,1.,1.,1.,1.,1.,1.,1.,1.,1.,
1.,1.,1.,1.,1.,1.,1.,1.,1.,1.,1.,1.,1.,1.,1.,1.,1.,1.,1.,1.,1.,1.,1.,1.,
1.,1.,1.,1.,1.,1.,1.,1.,1.,1.,1.,1.,1.,1.,1.,1.,1.,1.,1.,1.,1.,1.,1.,1.,
1.,1.,1.,1.,1.,1.,1.,1.,1.,1.,1.,1.,1.,1.,1.,1.,1.,1.,1.,1.,1.))
REPRESENTATION_ITEM('')
);
#743=(
BOUNDED_CURVE()
B_SPLINE_CURVE(5,(#188492,#188493,#188494,#188495,#188496,#188497,#188498,
#188499,#188500,#188501,#188502,#188503,#188504,#188505,#188506,#188507,
#188508,#188509,#188510,#188511,#188512,#188513,#188514,#188515,#188516,
#188517,#188518,#188519,#188520,#188521,#188522,#188523,#188524,#188525,
#188526,#188527,#188528,#188529,#188530,#188531,#188532,#188533,#188534,
#188535,#188536,#188537,#188538,#188539,#188540,#188541,#188542,#188543,
#188544,#188545,#188546,#188547,#188548,#188549,#188550,#188551,#188552,
#188553,#188554,#188555,#188556,#188557,#188558,#188559,#188560,#188561,
#188562,#188563,#188564,#188565,#188566,#188567,#188568,#188569,#188570,
#188571,#188572,#188573,#188574,#188575,#188576,#188577,#188578,#188579,
#188580,#188581,#188582,#188583,#188584,#188585,#188586,#188587,#188588,
#188589,#188590,#188591,#188592,#188593,#188594,#188595,#188596,#188597,
#188598,#188599,#188600,#188601,#188602,#188603,#188604,#188605,#188606,
#188607,#188608,#188609,#188610,#188611,#188612,#188613,#188614,#188615,
#188616,#188617,#188618,#188619,#188620,#188621,#188622,#188623,#188624,
#188625,#188626,#188627,#188628,#188629,#188630,#188631,#188632,#188633,
#188634,#188635,#188636,#188637,#188638,#188639,#188640,#188641,#188642,
#188643,#188644,#188645,#188646,#188647,#188648,#188649,#188650,#188651,
#188652,#188653,#188654,#188655,#188656,#188657,#188658,#188659,#188660,
#188661,#188662,#188663,#188664,#188665,#188666,#188667,#188668,#188669,
#188670,#188671,#188672,#188673,#188674,#188675,#188676,#188677,#188678,
#188679,#188680,#188681,#188682,#188683,#188684,#188685,#188686,#188687,
#188688,#188689,#188690,#188691,#188692,#188693,#188694,#188695,#188696),
 .UNSPECIFIED.,.F.,.F.)
B_SPLINE_CURVE_WITH_KNOTS((6,1,1,1,1,1,1,1,1,1,1,1,1,1,1,1,1,1,1,1,1,1,
1,1,1,1,1,1,1,1,1,1,1,1,1,1,1,1,1,1,1,1,1,1,1,1,1,1,1,1,1,1,1,1,1,1,1,1,
1,1,1,1,1,1,1,1,1,1,1,1,1,1,1,1,1,1,1,1,1,1,1,1,1,1,1,1,1,1,1,1,1,1,1,1,
1,1,1,1,1,1,1,1,1,1,1,1,1,1,1,1,1,1,1,1,1,1,1,1,1,1,1,1,1,1,1,1,1,1,1,1,
1,1,1,1,1,1,1,1,1,1,1,1,1,1,1,1,1,1,1,1,1,1,1,1,1,1,1,1,1,1,1,1,1,1,1,1,
1,1,1,1,1,1,1,1,1,1,1,1,1,1,1,1,1,1,1,1,1,1,1,1,1,1,1,1,1,1,1,1,1,1,6),
(-1.,-0.995000000000001,-0.990000000000001,-0.985000000000001,-0.980000000000001,
-0.975000000000001,-0.970000000000001,-0.965000000000001,-0.960000000000001,
-0.955000000000001,-0.950000000000001,-0.945000000000001,-0.940000000000001,
-0.935000000000001,-0.930000000000001,-0.925000000000001,-0.920000000000001,
-0.915000000000001,-0.910000000000001,-0.905000000000001,-0.900000000000001,
-0.895000000000001,-0.890000000000001,-0.885000000000001,-0.880000000000001,
-0.875000000000001,-0.870000000000001,-0.865000000000001,-0.860000000000001,
-0.855000000000001,-0.850000000000001,-0.845000000000001,-0.840000000000001,
-0.835000000000001,-0.830000000000001,-0.825000000000001,-0.820000000000001,
-0.815000000000001,-0.810000000000001,-0.805000000000001,-0.800000000000001,
-0.795000000000001,-0.790000000000001,-0.785000000000001,-0.780000000000001,
-0.775000000000001,-0.770000000000001,-0.765000000000001,-0.760000000000001,
-0.755000000000001,-0.750000000000001,-0.745000000000001,-0.740000000000001,
-0.735000000000001,-0.730000000000001,-0.725000000000001,-0.720000000000001,
-0.715000000000001,-0.710000000000001,-0.705000000000001,-0.700000000000001,
-0.695000000000001,-0.690000000000001,-0.685,-0.68,-0.675,-0.67,-0.665,
-0.66,-0.655,-0.65,-0.645,-0.64,-0.635,-0.63,-0.625,-0.62,-0.615,-0.61,
-0.605,-0.6,-0.595,-0.59,-0.585,-0.58,-0.575,-0.57,-0.565,-0.56,-0.555,
-0.55,-0.545,-0.54,-0.535,-0.53,-0.525,-0.52,-0.515,-0.51,-0.505,-0.5,-0.495,
-0.49,-0.485,-0.48,-0.475,-0.47,-0.465,-0.46,-0.455,-0.45,-0.445,-0.44,
-0.435,-0.43,-0.425,-0.42,-0.415,-0.41,-0.405,-0.4,-0.395,-0.39,-0.385,
-0.38,-0.375,-0.37,-0.365,-0.36,-0.355,-0.35,-0.345,-0.34,-0.335,-0.33,
-0.325,-0.32,-0.315,-0.31,-0.305,-0.3,-0.295,-0.29,-0.285,-0.28,-0.275,
-0.27,-0.265,-0.26,-0.255,-0.25,-0.245,-0.24,-0.235,-0.23,-0.225,-0.22,
-0.215,-0.21,-0.205,-0.2,-0.195,-0.19,-0.185,-0.18,-0.175,-0.17,-0.165,
-0.16,-0.155,-0.15,-0.145,-0.14,-0.135,-0.13,-0.125,-0.12,-0.115,-0.11,
-0.105,-0.1,-0.095,-0.09,-0.085,-0.08,-0.075,-0.07,-0.065,-0.06,-0.055,
-0.05,-0.045,-0.04,-0.035,-0.03,-0.025,-0.02,-0.015,-0.01,-0.005,0.),
 .UNSPECIFIED.)
CURVE()
GEOMETRIC_REPRESENTATION_ITEM()
RATIONAL_B_SPLINE_CURVE((1.,1.,1.,1.,1.,1.,1.,1.,1.,1.,1.,1.,1.,1.,1.,1.,
1.,1.,1.,1.,1.,1.,1.,1.,1.,1.,1.,1.,1.,1.,1.,1.,1.,1.,1.,1.,1.,1.,1.,1.,
1.,1.,1.,1.,1.,1.,1.,1.,1.,1.,1.,1.,1.,1.,1.,1.,1.,1.,1.,1.,1.,1.,1.,1.,
1.,1.,1.,1.,1.,1.,1.,1.,1.,1.,1.,1.,1.,1.,1.,1.,1.,1.,1.,1.,1.,1.,1.,1.,
1.,1.,1.,1.,1.,1.,1.,1.,1.,1.,1.,1.,1.,1.,1.,1.,1.,1.,1.,1.,1.,1.,1.,1.,
1.,1.,1.,1.,1.,1.,1.,1.,1.,1.,1.,1.,1.,1.,1.,1.,1.,1.,1.,1.,1.,1.,1.,1.,
1.,1.,1.,1.,1.,1.,1.,1.,1.,1.,1.,1.,1.,1.,1.,1.,1.,1.,1.,1.,1.,1.,1.,1.,
1.,1.,1.,1.,1.,1.,1.,1.,1.,1.,1.,1.,1.,1.,1.,1.,1.,1.,1.,1.,1.,1.,1.,1.,
1.,1.,1.,1.,1.,1.,1.,1.,1.,1.,1.,1.,1.,1.,1.,1.,1.,1.,1.,1.,1.))
REPRESENTATION_ITEM('')
);
#744=(
BOUNDED_CURVE()
B_SPLINE_CURVE(5,(#189109,#189110,#189111,#189112,#189113,#189114,#189115,
#189116,#189117,#189118,#189119,#189120,#189121,#189122,#189123,#189124,
#189125,#189126,#189127,#189128,#189129,#189130,#189131,#189132,#189133,
#189134,#189135,#189136,#189137,#189138,#189139,#189140,#189141,#189142,
#189143,#189144,#189145,#189146,#189147,#189148,#189149,#189150,#189151,
#189152,#189153,#189154,#189155,#189156,#189157,#189158,#189159,#189160,
#189161,#189162,#189163,#189164,#189165,#189166,#189167,#189168,#189169,
#189170,#189171,#189172,#189173,#189174,#189175,#189176,#189177,#189178,
#189179,#189180,#189181,#189182,#189183,#189184,#189185,#189186,#189187,
#189188,#189189,#189190,#189191,#189192,#189193,#189194,#189195,#189196,
#189197,#189198,#189199,#189200,#189201,#189202,#189203,#189204,#189205,
#189206,#189207,#189208,#189209,#189210,#189211,#189212,#189213,#189214,
#189215,#189216,#189217,#189218,#189219,#189220,#189221,#189222,#189223,
#189224,#189225,#189226,#189227,#189228,#189229,#189230,#189231,#189232,
#189233,#189234,#189235,#189236,#189237,#189238,#189239,#189240,#189241,
#189242,#189243,#189244,#189245,#189246,#189247,#189248,#189249,#189250,
#189251,#189252,#189253,#189254,#189255,#189256,#189257,#189258,#189259,
#189260,#189261,#189262,#189263,#189264,#189265,#189266,#189267,#189268,
#189269,#189270,#189271,#189272,#189273,#189274,#189275,#189276,#189277,
#189278,#189279,#189280,#189281,#189282,#189283,#189284,#189285,#189286,
#189287,#189288,#189289,#189290,#189291,#189292,#189293,#189294,#189295,
#189296,#189297,#189298,#189299,#189300,#189301,#189302,#189303,#189304,
#189305,#189306,#189307,#189308,#189309,#189310,#189311,#189312,#189313),
 .UNSPECIFIED.,.F.,.F.)
B_SPLINE_CURVE_WITH_KNOTS((6,1,1,1,1,1,1,1,1,1,1,1,1,1,1,1,1,1,1,1,1,1,
1,1,1,1,1,1,1,1,1,1,1,1,1,1,1,1,1,1,1,1,1,1,1,1,1,1,1,1,1,1,1,1,1,1,1,1,
1,1,1,1,1,1,1,1,1,1,1,1,1,1,1,1,1,1,1,1,1,1,1,1,1,1,1,1,1,1,1,1,1,1,1,1,
1,1,1,1,1,1,1,1,1,1,1,1,1,1,1,1,1,1,1,1,1,1,1,1,1,1,1,1,1,1,1,1,1,1,1,1,
1,1,1,1,1,1,1,1,1,1,1,1,1,1,1,1,1,1,1,1,1,1,1,1,1,1,1,1,1,1,1,1,1,1,1,1,
1,1,1,1,1,1,1,1,1,1,1,1,1,1,1,1,1,1,1,1,1,1,1,1,1,1,1,1,1,1,1,1,1,1,6),
(0.,0.005,0.01,0.015,0.02,0.025,0.03,0.035,0.04,0.045,0.05,0.055,0.06,0.065,
0.07,0.075,0.08,0.085,0.09,0.095,0.1,0.105,0.11,0.115,0.12,0.125,0.13,0.135,
0.14,0.145,0.15,0.155,0.16,0.165,0.17,0.175,0.18,0.185,0.19,0.195,0.2,0.205,
0.21,0.215,0.22,0.225,0.23,0.235,0.24,0.245,0.25,0.255,0.26,0.265,0.27,
0.275,0.28,0.285,0.29,0.295,0.3,0.305,0.31,0.315,0.32,0.325,0.33,0.335,
0.34,0.345,0.35,0.355,0.36,0.365,0.37,0.375,0.38,0.385,0.39,0.395,0.4,0.405,
0.41,0.415,0.42,0.425,0.43,0.435,0.44,0.445,0.45,0.455,0.46,0.465,0.47,
0.475,0.48,0.485,0.49,0.495,0.5,0.505,0.51,0.515,0.52,0.525,0.53,0.535,
0.54,0.545,0.55,0.555,0.56,0.565,0.57,0.575,0.58,0.585,0.59,0.595,0.6,0.605,
0.61,0.615,0.62,0.625,0.63,0.635,0.64,0.645,0.65,0.655,0.66,0.665,0.67,
0.675,0.68,0.685,0.690000000000001,0.695000000000001,0.700000000000001,
0.705000000000001,0.710000000000001,0.715000000000001,0.720000000000001,
0.725000000000001,0.730000000000001,0.735000000000001,0.740000000000001,
0.745000000000001,0.750000000000001,0.755000000000001,0.760000000000001,
0.765000000000001,0.770000000000001,0.775000000000001,0.780000000000001,
0.785000000000001,0.790000000000001,0.795000000000001,0.800000000000001,
0.805000000000001,0.810000000000001,0.815000000000001,0.820000000000001,
0.825000000000001,0.830000000000001,0.835000000000001,0.840000000000001,
0.845000000000001,0.850000000000001,0.855000000000001,0.860000000000001,
0.865000000000001,0.870000000000001,0.875000000000001,0.880000000000001,
0.885000000000001,0.890000000000001,0.895000000000001,0.900000000000001,
0.905000000000001,0.910000000000001,0.915000000000001,0.920000000000001,
0.925000000000001,0.930000000000001,0.935000000000001,0.940000000000001,
0.945000000000001,0.950000000000001,0.955000000000001,0.960000000000001,
0.965000000000001,0.970000000000001,0.975000000000001,0.980000000000001,
0.985000000000001,0.990000000000001,0.995000000000001,1.),.UNSPECIFIED.)
CURVE()
GEOMETRIC_REPRESENTATION_ITEM()
RATIONAL_B_SPLINE_CURVE((1.,1.,1.,1.,1.,1.,1.,1.,1.,1.,1.,1.,1.,1.,1.,1.,
1.,1.,1.,1.,1.,1.,1.,1.,1.,1.,1.,1.,1.,1.,1.,1.,1.,1.,1.,1.,1.,1.,1.,1.,
1.,1.,1.,1.,1.,1.,1.,1.,1.,1.,1.,1.,1.,1.,1.,1.,1.,1.,1.,1.,1.,1.,1.,1.,
1.,1.,1.,1.,1.,1.,1.,1.,1.,1.,1.,1.,1.,1.,1.,1.,1.,1.,1.,1.,1.,1.,1.,1.,
1.,1.,1.,1.,1.,1.,1.,1.,1.,1.,1.,1.,1.,1.,1.,1.,1.,1.,1.,1.,1.,1.,1.,1.,
1.,1.,1.,1.,1.,1.,1.,1.,1.,1.,1.,1.,1.,1.,1.,1.,1.,1.,1.,1.,1.,1.,1.,1.,
1.,1.,1.,1.,1.,1.,1.,1.,1.,1.,1.,1.,1.,1.,1.,1.,1.,1.,1.,1.,1.,1.,1.,1.,
1.,1.,1.,1.,1.,1.,1.,1.,1.,1.,1.,1.,1.,1.,1.,1.,1.,1.,1.,1.,1.,1.,1.,1.,
1.,1.,1.,1.,1.,1.,1.,1.,1.,1.,1.,1.,1.,1.,1.,1.,1.,1.,1.,1.,1.))
REPRESENTATION_ITEM('')
);
#745=(
BOUNDED_CURVE()
B_SPLINE_CURVE(5,(#189730,#189731,#189732,#189733,#189734,#189735,#189736,
#189737,#189738,#189739,#189740,#189741,#189742,#189743,#189744,#189745,
#189746,#189747,#189748,#189749,#189750,#189751,#189752,#189753,#189754,
#189755,#189756,#189757,#189758,#189759,#189760,#189761,#189762,#189763,
#189764,#189765,#189766,#189767,#189768,#189769,#189770,#189771,#189772,
#189773,#189774,#189775,#189776,#189777,#189778,#189779,#189780,#189781,
#189782,#189783,#189784,#189785,#189786,#189787,#189788,#189789,#189790,
#189791,#189792,#189793,#189794,#189795,#189796,#189797,#189798,#189799,
#189800,#189801,#189802,#189803,#189804,#189805,#189806,#189807,#189808,
#189809,#189810,#189811,#189812,#189813,#189814,#189815,#189816,#189817,
#189818,#189819,#189820,#189821,#189822,#189823,#189824,#189825,#189826,
#189827,#189828,#189829,#189830,#189831,#189832,#189833,#189834,#189835,
#189836,#189837,#189838,#189839,#189840,#189841,#189842,#189843,#189844,
#189845,#189846,#189847,#189848,#189849,#189850,#189851,#189852,#189853,
#189854,#189855,#189856,#189857,#189858,#189859,#189860,#189861,#189862,
#189863,#189864,#189865,#189866,#189867,#189868,#189869,#189870,#189871,
#189872,#189873,#189874,#189875,#189876,#189877,#189878,#189879,#189880,
#189881,#189882,#189883,#189884,#189885,#189886,#189887,#189888,#189889,
#189890,#189891,#189892,#189893,#189894,#189895,#189896,#189897,#189898,
#189899,#189900,#189901,#189902,#189903,#189904,#189905,#189906,#189907,
#189908,#189909,#189910,#189911,#189912,#189913,#189914,#189915,#189916,
#189917,#189918,#189919,#189920,#189921,#189922,#189923,#189924,#189925,
#189926,#189927,#189928,#189929,#189930,#189931,#189932,#189933,#189934),
 .UNSPECIFIED.,.F.,.F.)
B_SPLINE_CURVE_WITH_KNOTS((6,1,1,1,1,1,1,1,1,1,1,1,1,1,1,1,1,1,1,1,1,1,
1,1,1,1,1,1,1,1,1,1,1,1,1,1,1,1,1,1,1,1,1,1,1,1,1,1,1,1,1,1,1,1,1,1,1,1,
1,1,1,1,1,1,1,1,1,1,1,1,1,1,1,1,1,1,1,1,1,1,1,1,1,1,1,1,1,1,1,1,1,1,1,1,
1,1,1,1,1,1,1,1,1,1,1,1,1,1,1,1,1,1,1,1,1,1,1,1,1,1,1,1,1,1,1,1,1,1,1,1,
1,1,1,1,1,1,1,1,1,1,1,1,1,1,1,1,1,1,1,1,1,1,1,1,1,1,1,1,1,1,1,1,1,1,1,1,
1,1,1,1,1,1,1,1,1,1,1,1,1,1,1,1,1,1,1,1,1,1,1,1,1,1,1,1,1,1,1,1,1,1,6),
(-1.,-0.995000000000001,-0.990000000000001,-0.985000000000001,-0.980000000000001,
-0.975000000000001,-0.970000000000001,-0.965000000000001,-0.960000000000001,
-0.955000000000001,-0.950000000000001,-0.945000000000001,-0.940000000000001,
-0.935000000000001,-0.930000000000001,-0.925000000000001,-0.920000000000001,
-0.915000000000001,-0.910000000000001,-0.905000000000001,-0.900000000000001,
-0.895000000000001,-0.890000000000001,-0.885000000000001,-0.880000000000001,
-0.875000000000001,-0.870000000000001,-0.865000000000001,-0.860000000000001,
-0.855000000000001,-0.850000000000001,-0.845000000000001,-0.840000000000001,
-0.835000000000001,-0.830000000000001,-0.825000000000001,-0.820000000000001,
-0.815000000000001,-0.810000000000001,-0.805000000000001,-0.800000000000001,
-0.795000000000001,-0.790000000000001,-0.785000000000001,-0.780000000000001,
-0.775000000000001,-0.770000000000001,-0.765000000000001,-0.760000000000001,
-0.755000000000001,-0.750000000000001,-0.745000000000001,-0.740000000000001,
-0.735000000000001,-0.730000000000001,-0.725000000000001,-0.720000000000001,
-0.715000000000001,-0.710000000000001,-0.705000000000001,-0.700000000000001,
-0.695000000000001,-0.690000000000001,-0.685,-0.68,-0.675,-0.67,-0.665,
-0.66,-0.655,-0.65,-0.645,-0.64,-0.635,-0.63,-0.625,-0.62,-0.615,-0.61,
-0.605,-0.6,-0.595,-0.59,-0.585,-0.58,-0.575,-0.57,-0.565,-0.56,-0.555,
-0.55,-0.545,-0.54,-0.535,-0.53,-0.525,-0.52,-0.515,-0.51,-0.505,-0.5,-0.495,
-0.49,-0.485,-0.48,-0.475,-0.47,-0.465,-0.46,-0.455,-0.45,-0.445,-0.44,
-0.435,-0.43,-0.425,-0.42,-0.415,-0.41,-0.405,-0.4,-0.395,-0.39,-0.385,
-0.38,-0.375,-0.37,-0.365,-0.36,-0.355,-0.35,-0.345,-0.34,-0.335,-0.33,
-0.325,-0.32,-0.315,-0.31,-0.305,-0.3,-0.295,-0.29,-0.285,-0.28,-0.275,
-0.27,-0.265,-0.26,-0.255,-0.25,-0.245,-0.24,-0.235,-0.23,-0.225,-0.22,
-0.215,-0.21,-0.205,-0.2,-0.195,-0.19,-0.185,-0.18,-0.175,-0.17,-0.165,
-0.16,-0.155,-0.15,-0.145,-0.14,-0.135,-0.13,-0.125,-0.12,-0.115,-0.11,
-0.105,-0.1,-0.095,-0.09,-0.085,-0.08,-0.075,-0.07,-0.065,-0.06,-0.055,
-0.05,-0.045,-0.04,-0.035,-0.03,-0.025,-0.02,-0.015,-0.01,-0.005,0.),
 .UNSPECIFIED.)
CURVE()
GEOMETRIC_REPRESENTATION_ITEM()
RATIONAL_B_SPLINE_CURVE((1.,1.,1.,1.,1.,1.,1.,1.,1.,1.,1.,1.,1.,1.,1.,1.,
1.,1.,1.,1.,1.,1.,1.,1.,1.,1.,1.,1.,1.,1.,1.,1.,1.,1.,1.,1.,1.,1.,1.,1.,
1.,1.,1.,1.,1.,1.,1.,1.,1.,1.,1.,1.,1.,1.,1.,1.,1.,1.,1.,1.,1.,1.,1.,1.,
1.,1.,1.,1.,1.,1.,1.,1.,1.,1.,1.,1.,1.,1.,1.,1.,1.,1.,1.,1.,1.,1.,1.,1.,
1.,1.,1.,1.,1.,1.,1.,1.,1.,1.,1.,1.,1.,1.,1.,1.,1.,1.,1.,1.,1.,1.,1.,1.,
1.,1.,1.,1.,1.,1.,1.,1.,1.,1.,1.,1.,1.,1.,1.,1.,1.,1.,1.,1.,1.,1.,1.,1.,
1.,1.,1.,1.,1.,1.,1.,1.,1.,1.,1.,1.,1.,1.,1.,1.,1.,1.,1.,1.,1.,1.,1.,1.,
1.,1.,1.,1.,1.,1.,1.,1.,1.,1.,1.,1.,1.,1.,1.,1.,1.,1.,1.,1.,1.,1.,1.,1.,
1.,1.,1.,1.,1.,1.,1.,1.,1.,1.,1.,1.,1.,1.,1.,1.,1.,1.,1.,1.,1.))
REPRESENTATION_ITEM('')
);
#746=(
BOUNDED_CURVE()
B_SPLINE_CURVE(5,(#190347,#190348,#190349,#190350,#190351,#190352,#190353,
#190354,#190355,#190356,#190357,#190358,#190359,#190360,#190361,#190362,
#190363,#190364,#190365,#190366,#190367,#190368,#190369,#190370,#190371,
#190372,#190373,#190374,#190375,#190376,#190377,#190378,#190379,#190380,
#190381,#190382,#190383,#190384,#190385,#190386,#190387,#190388,#190389,
#190390,#190391,#190392,#190393,#190394,#190395,#190396,#190397,#190398,
#190399,#190400,#190401,#190402,#190403,#190404,#190405,#190406,#190407,
#190408,#190409,#190410,#190411,#190412,#190413,#190414,#190415,#190416,
#190417,#190418,#190419,#190420,#190421,#190422,#190423,#190424,#190425,
#190426,#190427,#190428,#190429,#190430,#190431,#190432,#190433,#190434,
#190435,#190436,#190437,#190438,#190439,#190440,#190441,#190442,#190443,
#190444,#190445,#190446,#190447,#190448,#190449,#190450,#190451,#190452,
#190453,#190454,#190455,#190456,#190457,#190458,#190459,#190460,#190461,
#190462,#190463,#190464,#190465,#190466,#190467,#190468,#190469,#190470,
#190471,#190472,#190473,#190474,#190475,#190476,#190477,#190478,#190479,
#190480,#190481,#190482,#190483,#190484,#190485,#190486,#190487,#190488,
#190489,#190490,#190491,#190492,#190493,#190494,#190495,#190496,#190497,
#190498,#190499,#190500,#190501,#190502,#190503,#190504,#190505,#190506,
#190507,#190508,#190509,#190510,#190511,#190512,#190513,#190514,#190515,
#190516,#190517,#190518,#190519,#190520,#190521,#190522,#190523,#190524,
#190525,#190526,#190527,#190528,#190529,#190530,#190531,#190532,#190533,
#190534,#190535,#190536,#190537,#190538,#190539,#190540,#190541,#190542,
#190543,#190544,#190545,#190546,#190547,#190548,#190549,#190550,#190551),
 .UNSPECIFIED.,.F.,.F.)
B_SPLINE_CURVE_WITH_KNOTS((6,1,1,1,1,1,1,1,1,1,1,1,1,1,1,1,1,1,1,1,1,1,
1,1,1,1,1,1,1,1,1,1,1,1,1,1,1,1,1,1,1,1,1,1,1,1,1,1,1,1,1,1,1,1,1,1,1,1,
1,1,1,1,1,1,1,1,1,1,1,1,1,1,1,1,1,1,1,1,1,1,1,1,1,1,1,1,1,1,1,1,1,1,1,1,
1,1,1,1,1,1,1,1,1,1,1,1,1,1,1,1,1,1,1,1,1,1,1,1,1,1,1,1,1,1,1,1,1,1,1,1,
1,1,1,1,1,1,1,1,1,1,1,1,1,1,1,1,1,1,1,1,1,1,1,1,1,1,1,1,1,1,1,1,1,1,1,1,
1,1,1,1,1,1,1,1,1,1,1,1,1,1,1,1,1,1,1,1,1,1,1,1,1,1,1,1,1,1,1,1,1,1,6),
(0.,0.005,0.01,0.015,0.02,0.025,0.03,0.035,0.04,0.045,0.05,0.055,0.06,0.065,
0.07,0.075,0.08,0.085,0.09,0.095,0.1,0.105,0.11,0.115,0.12,0.125,0.13,0.135,
0.14,0.145,0.15,0.155,0.16,0.165,0.17,0.175,0.18,0.185,0.19,0.195,0.2,0.205,
0.21,0.215,0.22,0.225,0.23,0.235,0.24,0.245,0.25,0.255,0.26,0.265,0.27,
0.275,0.28,0.285,0.29,0.295,0.3,0.305,0.31,0.315,0.32,0.325,0.33,0.335,
0.34,0.345,0.35,0.355,0.36,0.365,0.37,0.375,0.38,0.385,0.39,0.395,0.4,0.405,
0.41,0.415,0.42,0.425,0.43,0.435,0.44,0.445,0.45,0.455,0.46,0.465,0.47,
0.475,0.48,0.485,0.49,0.495,0.5,0.505,0.51,0.515,0.52,0.525,0.53,0.535,
0.54,0.545,0.55,0.555,0.56,0.565,0.57,0.575,0.58,0.585,0.59,0.595,0.6,0.605,
0.61,0.615,0.62,0.625,0.63,0.635,0.64,0.645,0.65,0.655,0.66,0.665,0.67,
0.675,0.68,0.685,0.690000000000001,0.695000000000001,0.700000000000001,
0.705000000000001,0.710000000000001,0.715000000000001,0.720000000000001,
0.725000000000001,0.730000000000001,0.735000000000001,0.740000000000001,
0.745000000000001,0.750000000000001,0.755000000000001,0.760000000000001,
0.765000000000001,0.770000000000001,0.775000000000001,0.780000000000001,
0.785000000000001,0.790000000000001,0.795000000000001,0.800000000000001,
0.805000000000001,0.810000000000001,0.815000000000001,0.820000000000001,
0.825000000000001,0.830000000000001,0.835000000000001,0.840000000000001,
0.845000000000001,0.850000000000001,0.855000000000001,0.860000000000001,
0.865000000000001,0.870000000000001,0.875000000000001,0.880000000000001,
0.885000000000001,0.890000000000001,0.895000000000001,0.900000000000001,
0.905000000000001,0.910000000000001,0.915000000000001,0.920000000000001,
0.925000000000001,0.930000000000001,0.935000000000001,0.940000000000001,
0.945000000000001,0.950000000000001,0.955000000000001,0.960000000000001,
0.965000000000001,0.970000000000001,0.975000000000001,0.980000000000001,
0.985000000000001,0.990000000000001,0.995000000000001,1.),.UNSPECIFIED.)
CURVE()
GEOMETRIC_REPRESENTATION_ITEM()
RATIONAL_B_SPLINE_CURVE((1.,1.,1.,1.,1.,1.,1.,1.,1.,1.,1.,1.,1.,1.,1.,1.,
1.,1.,1.,1.,1.,1.,1.,1.,1.,1.,1.,1.,1.,1.,1.,1.,1.,1.,1.,1.,1.,1.,1.,1.,
1.,1.,1.,1.,1.,1.,1.,1.,1.,1.,1.,1.,1.,1.,1.,1.,1.,1.,1.,1.,1.,1.,1.,1.,
1.,1.,1.,1.,1.,1.,1.,1.,1.,1.,1.,1.,1.,1.,1.,1.,1.,1.,1.,1.,1.,1.,1.,1.,
1.,1.,1.,1.,1.,1.,1.,1.,1.,1.,1.,1.,1.,1.,1.,1.,1.,1.,1.,1.,1.,1.,1.,1.,
1.,1.,1.,1.,1.,1.,1.,1.,1.,1.,1.,1.,1.,1.,1.,1.,1.,1.,1.,1.,1.,1.,1.,1.,
1.,1.,1.,1.,1.,1.,1.,1.,1.,1.,1.,1.,1.,1.,1.,1.,1.,1.,1.,1.,1.,1.,1.,1.,
1.,1.,1.,1.,1.,1.,1.,1.,1.,1.,1.,1.,1.,1.,1.,1.,1.,1.,1.,1.,1.,1.,1.,1.,
1.,1.,1.,1.,1.,1.,1.,1.,1.,1.,1.,1.,1.,1.,1.,1.,1.,1.,1.,1.,1.))
REPRESENTATION_ITEM('')
);
#747=(
BOUNDED_CURVE()
B_SPLINE_CURVE(5,(#190968,#190969,#190970,#190971,#190972,#190973,#190974,
#190975,#190976,#190977,#190978,#190979,#190980,#190981,#190982,#190983,
#190984,#190985,#190986,#190987,#190988,#190989,#190990,#190991,#190992,
#190993,#190994,#190995,#190996,#190997,#190998,#190999,#191000,#191001,
#191002,#191003,#191004,#191005,#191006,#191007,#191008,#191009,#191010,
#191011,#191012,#191013,#191014,#191015,#191016,#191017,#191018,#191019,
#191020,#191021,#191022,#191023,#191024,#191025,#191026,#191027,#191028,
#191029,#191030,#191031,#191032,#191033,#191034,#191035,#191036,#191037,
#191038,#191039,#191040,#191041,#191042,#191043,#191044,#191045,#191046,
#191047,#191048,#191049,#191050,#191051,#191052,#191053,#191054,#191055,
#191056,#191057,#191058,#191059,#191060,#191061,#191062,#191063,#191064,
#191065,#191066,#191067,#191068,#191069,#191070,#191071,#191072,#191073,
#191074,#191075,#191076,#191077,#191078,#191079,#191080,#191081,#191082,
#191083,#191084,#191085,#191086,#191087,#191088,#191089,#191090,#191091,
#191092,#191093,#191094,#191095,#191096,#191097,#191098,#191099,#191100,
#191101,#191102,#191103,#191104,#191105,#191106,#191107,#191108,#191109,
#191110,#191111,#191112,#191113,#191114,#191115,#191116,#191117,#191118,
#191119,#191120,#191121,#191122,#191123,#191124,#191125,#191126,#191127,
#191128,#191129,#191130,#191131,#191132,#191133,#191134,#191135,#191136,
#191137,#191138,#191139,#191140,#191141,#191142,#191143,#191144,#191145,
#191146,#191147,#191148,#191149,#191150,#191151,#191152,#191153,#191154,
#191155,#191156,#191157,#191158,#191159,#191160,#191161,#191162,#191163,
#191164,#191165,#191166,#191167,#191168,#191169,#191170,#191171,#191172),
 .UNSPECIFIED.,.F.,.F.)
B_SPLINE_CURVE_WITH_KNOTS((6,1,1,1,1,1,1,1,1,1,1,1,1,1,1,1,1,1,1,1,1,1,
1,1,1,1,1,1,1,1,1,1,1,1,1,1,1,1,1,1,1,1,1,1,1,1,1,1,1,1,1,1,1,1,1,1,1,1,
1,1,1,1,1,1,1,1,1,1,1,1,1,1,1,1,1,1,1,1,1,1,1,1,1,1,1,1,1,1,1,1,1,1,1,1,
1,1,1,1,1,1,1,1,1,1,1,1,1,1,1,1,1,1,1,1,1,1,1,1,1,1,1,1,1,1,1,1,1,1,1,1,
1,1,1,1,1,1,1,1,1,1,1,1,1,1,1,1,1,1,1,1,1,1,1,1,1,1,1,1,1,1,1,1,1,1,1,1,
1,1,1,1,1,1,1,1,1,1,1,1,1,1,1,1,1,1,1,1,1,1,1,1,1,1,1,1,1,1,1,1,1,1,6),
(-1.,-0.995000000000001,-0.990000000000001,-0.985000000000001,-0.980000000000001,
-0.975000000000001,-0.970000000000001,-0.965000000000001,-0.960000000000001,
-0.955000000000001,-0.950000000000001,-0.945000000000001,-0.940000000000001,
-0.935000000000001,-0.930000000000001,-0.925000000000001,-0.920000000000001,
-0.915000000000001,-0.910000000000001,-0.905000000000001,-0.900000000000001,
-0.895000000000001,-0.890000000000001,-0.885000000000001,-0.880000000000001,
-0.875000000000001,-0.870000000000001,-0.865000000000001,-0.860000000000001,
-0.855000000000001,-0.850000000000001,-0.845000000000001,-0.840000000000001,
-0.835000000000001,-0.830000000000001,-0.825000000000001,-0.820000000000001,
-0.815000000000001,-0.810000000000001,-0.805000000000001,-0.800000000000001,
-0.795000000000001,-0.790000000000001,-0.785000000000001,-0.780000000000001,
-0.775000000000001,-0.770000000000001,-0.765000000000001,-0.760000000000001,
-0.755000000000001,-0.750000000000001,-0.745000000000001,-0.740000000000001,
-0.735000000000001,-0.730000000000001,-0.725000000000001,-0.720000000000001,
-0.715000000000001,-0.710000000000001,-0.705000000000001,-0.700000000000001,
-0.695000000000001,-0.690000000000001,-0.685,-0.68,-0.675,-0.67,-0.665,
-0.66,-0.655,-0.65,-0.645,-0.64,-0.635,-0.63,-0.625,-0.62,-0.615,-0.61,
-0.605,-0.6,-0.595,-0.59,-0.585,-0.58,-0.575,-0.57,-0.565,-0.56,-0.555,
-0.55,-0.545,-0.54,-0.535,-0.53,-0.525,-0.52,-0.515,-0.51,-0.505,-0.5,-0.495,
-0.49,-0.485,-0.48,-0.475,-0.47,-0.465,-0.46,-0.455,-0.45,-0.445,-0.44,
-0.435,-0.43,-0.425,-0.42,-0.415,-0.41,-0.405,-0.4,-0.395,-0.39,-0.385,
-0.38,-0.375,-0.37,-0.365,-0.36,-0.355,-0.35,-0.345,-0.34,-0.335,-0.33,
-0.325,-0.32,-0.315,-0.31,-0.305,-0.3,-0.295,-0.29,-0.285,-0.28,-0.275,
-0.27,-0.265,-0.26,-0.255,-0.25,-0.245,-0.24,-0.235,-0.23,-0.225,-0.22,
-0.215,-0.21,-0.205,-0.2,-0.195,-0.19,-0.185,-0.18,-0.175,-0.17,-0.165,
-0.16,-0.155,-0.15,-0.145,-0.14,-0.135,-0.13,-0.125,-0.12,-0.115,-0.11,
-0.105,-0.1,-0.095,-0.09,-0.085,-0.08,-0.075,-0.07,-0.065,-0.06,-0.055,
-0.05,-0.045,-0.04,-0.035,-0.03,-0.025,-0.02,-0.015,-0.01,-0.005,0.),
 .UNSPECIFIED.)
CURVE()
GEOMETRIC_REPRESENTATION_ITEM()
RATIONAL_B_SPLINE_CURVE((1.,1.,1.,1.,1.,1.,1.,1.,1.,1.,1.,1.,1.,1.,1.,1.,
1.,1.,1.,1.,1.,1.,1.,1.,1.,1.,1.,1.,1.,1.,1.,1.,1.,1.,1.,1.,1.,1.,1.,1.,
1.,1.,1.,1.,1.,1.,1.,1.,1.,1.,1.,1.,1.,1.,1.,1.,1.,1.,1.,1.,1.,1.,1.,1.,
1.,1.,1.,1.,1.,1.,1.,1.,1.,1.,1.,1.,1.,1.,1.,1.,1.,1.,1.,1.,1.,1.,1.,1.,
1.,1.,1.,1.,1.,1.,1.,1.,1.,1.,1.,1.,1.,1.,1.,1.,1.,1.,1.,1.,1.,1.,1.,1.,
1.,1.,1.,1.,1.,1.,1.,1.,1.,1.,1.,1.,1.,1.,1.,1.,1.,1.,1.,1.,1.,1.,1.,1.,
1.,1.,1.,1.,1.,1.,1.,1.,1.,1.,1.,1.,1.,1.,1.,1.,1.,1.,1.,1.,1.,1.,1.,1.,
1.,1.,1.,1.,1.,1.,1.,1.,1.,1.,1.,1.,1.,1.,1.,1.,1.,1.,1.,1.,1.,1.,1.,1.,
1.,1.,1.,1.,1.,1.,1.,1.,1.,1.,1.,1.,1.,1.,1.,1.,1.,1.,1.,1.,1.))
REPRESENTATION_ITEM('')
);
#748=(
BOUNDED_CURVE()
B_SPLINE_CURVE(5,(#191585,#191586,#191587,#191588,#191589,#191590,#191591,
#191592,#191593,#191594,#191595,#191596,#191597,#191598,#191599,#191600,
#191601,#191602,#191603,#191604,#191605,#191606,#191607,#191608,#191609,
#191610,#191611,#191612,#191613,#191614,#191615,#191616,#191617,#191618,
#191619,#191620,#191621,#191622,#191623,#191624,#191625,#191626,#191627,
#191628,#191629,#191630,#191631,#191632,#191633,#191634,#191635,#191636,
#191637,#191638,#191639,#191640,#191641,#191642,#191643,#191644,#191645,
#191646,#191647,#191648,#191649,#191650,#191651,#191652,#191653,#191654,
#191655,#191656,#191657,#191658,#191659,#191660,#191661,#191662,#191663,
#191664,#191665,#191666,#191667,#191668,#191669,#191670,#191671,#191672,
#191673,#191674,#191675,#191676,#191677,#191678,#191679,#191680,#191681,
#191682,#191683,#191684,#191685,#191686,#191687,#191688,#191689,#191690,
#191691,#191692,#191693,#191694,#191695,#191696,#191697,#191698,#191699,
#191700,#191701,#191702,#191703,#191704,#191705,#191706,#191707,#191708,
#191709,#191710,#191711,#191712,#191713,#191714,#191715,#191716,#191717,
#191718,#191719,#191720,#191721,#191722,#191723,#191724,#191725,#191726,
#191727,#191728,#191729,#191730,#191731,#191732,#191733,#191734,#191735,
#191736,#191737,#191738,#191739,#191740,#191741,#191742,#191743,#191744,
#191745,#191746,#191747,#191748,#191749,#191750,#191751,#191752,#191753,
#191754,#191755,#191756,#191757,#191758,#191759,#191760,#191761,#191762,
#191763,#191764,#191765,#191766,#191767,#191768,#191769,#191770,#191771,
#191772,#191773,#191774,#191775,#191776,#191777,#191778,#191779,#191780,
#191781,#191782,#191783,#191784,#191785,#191786,#191787,#191788,#191789),
 .UNSPECIFIED.,.F.,.F.)
B_SPLINE_CURVE_WITH_KNOTS((6,1,1,1,1,1,1,1,1,1,1,1,1,1,1,1,1,1,1,1,1,1,
1,1,1,1,1,1,1,1,1,1,1,1,1,1,1,1,1,1,1,1,1,1,1,1,1,1,1,1,1,1,1,1,1,1,1,1,
1,1,1,1,1,1,1,1,1,1,1,1,1,1,1,1,1,1,1,1,1,1,1,1,1,1,1,1,1,1,1,1,1,1,1,1,
1,1,1,1,1,1,1,1,1,1,1,1,1,1,1,1,1,1,1,1,1,1,1,1,1,1,1,1,1,1,1,1,1,1,1,1,
1,1,1,1,1,1,1,1,1,1,1,1,1,1,1,1,1,1,1,1,1,1,1,1,1,1,1,1,1,1,1,1,1,1,1,1,
1,1,1,1,1,1,1,1,1,1,1,1,1,1,1,1,1,1,1,1,1,1,1,1,1,1,1,1,1,1,1,1,1,1,6),
(0.,0.005,0.01,0.015,0.02,0.025,0.03,0.035,0.04,0.045,0.05,0.055,0.06,0.065,
0.07,0.075,0.08,0.085,0.09,0.095,0.1,0.105,0.11,0.115,0.12,0.125,0.13,0.135,
0.14,0.145,0.15,0.155,0.16,0.165,0.17,0.175,0.18,0.185,0.19,0.195,0.2,0.205,
0.21,0.215,0.22,0.225,0.23,0.235,0.24,0.245,0.25,0.255,0.26,0.265,0.27,
0.275,0.28,0.285,0.29,0.295,0.3,0.305,0.31,0.315,0.32,0.325,0.33,0.335,
0.34,0.345,0.35,0.355,0.36,0.365,0.37,0.375,0.38,0.385,0.39,0.395,0.4,0.405,
0.41,0.415,0.42,0.425,0.43,0.435,0.44,0.445,0.45,0.455,0.46,0.465,0.47,
0.475,0.48,0.485,0.49,0.495,0.5,0.505,0.51,0.515,0.52,0.525,0.53,0.535,
0.54,0.545,0.55,0.555,0.56,0.565,0.57,0.575,0.58,0.585,0.59,0.595,0.6,0.605,
0.61,0.615,0.62,0.625,0.63,0.635,0.64,0.645,0.65,0.655,0.66,0.665,0.67,
0.675,0.68,0.685,0.690000000000001,0.695000000000001,0.700000000000001,
0.705000000000001,0.710000000000001,0.715000000000001,0.720000000000001,
0.725000000000001,0.730000000000001,0.735000000000001,0.740000000000001,
0.745000000000001,0.750000000000001,0.755000000000001,0.760000000000001,
0.765000000000001,0.770000000000001,0.775000000000001,0.780000000000001,
0.785000000000001,0.790000000000001,0.795000000000001,0.800000000000001,
0.805000000000001,0.810000000000001,0.815000000000001,0.820000000000001,
0.825000000000001,0.830000000000001,0.835000000000001,0.840000000000001,
0.845000000000001,0.850000000000001,0.855000000000001,0.860000000000001,
0.865000000000001,0.870000000000001,0.875000000000001,0.880000000000001,
0.885000000000001,0.890000000000001,0.895000000000001,0.900000000000001,
0.905000000000001,0.910000000000001,0.915000000000001,0.920000000000001,
0.925000000000001,0.930000000000001,0.935000000000001,0.940000000000001,
0.945000000000001,0.950000000000001,0.955000000000001,0.960000000000001,
0.965000000000001,0.970000000000001,0.975000000000001,0.980000000000001,
0.985000000000001,0.990000000000001,0.995000000000001,1.),.UNSPECIFIED.)
CURVE()
GEOMETRIC_REPRESENTATION_ITEM()
RATIONAL_B_SPLINE_CURVE((1.,1.,1.,1.,1.,1.,1.,1.,1.,1.,1.,1.,1.,1.,1.,1.,
1.,1.,1.,1.,1.,1.,1.,1.,1.,1.,1.,1.,1.,1.,1.,1.,1.,1.,1.,1.,1.,1.,1.,1.,
1.,1.,1.,1.,1.,1.,1.,1.,1.,1.,1.,1.,1.,1.,1.,1.,1.,1.,1.,1.,1.,1.,1.,1.,
1.,1.,1.,1.,1.,1.,1.,1.,1.,1.,1.,1.,1.,1.,1.,1.,1.,1.,1.,1.,1.,1.,1.,1.,
1.,1.,1.,1.,1.,1.,1.,1.,1.,1.,1.,1.,1.,1.,1.,1.,1.,1.,1.,1.,1.,1.,1.,1.,
1.,1.,1.,1.,1.,1.,1.,1.,1.,1.,1.,1.,1.,1.,1.,1.,1.,1.,1.,1.,1.,1.,1.,1.,
1.,1.,1.,1.,1.,1.,1.,1.,1.,1.,1.,1.,1.,1.,1.,1.,1.,1.,1.,1.,1.,1.,1.,1.,
1.,1.,1.,1.,1.,1.,1.,1.,1.,1.,1.,1.,1.,1.,1.,1.,1.,1.,1.,1.,1.,1.,1.,1.,
1.,1.,1.,1.,1.,1.,1.,1.,1.,1.,1.,1.,1.,1.,1.,1.,1.,1.,1.,1.,1.))
REPRESENTATION_ITEM('')
);
#749=(
BOUNDED_CURVE()
B_SPLINE_CURVE(5,(#192206,#192207,#192208,#192209,#192210,#192211,#192212,
#192213,#192214,#192215,#192216,#192217,#192218,#192219,#192220,#192221,
#192222,#192223,#192224,#192225,#192226,#192227,#192228,#192229,#192230,
#192231,#192232,#192233,#192234,#192235,#192236,#192237,#192238,#192239,
#192240,#192241,#192242,#192243,#192244,#192245,#192246,#192247,#192248,
#192249,#192250,#192251,#192252,#192253,#192254,#192255,#192256,#192257,
#192258,#192259,#192260,#192261,#192262,#192263,#192264,#192265,#192266,
#192267,#192268,#192269,#192270,#192271,#192272,#192273,#192274,#192275,
#192276,#192277,#192278,#192279,#192280,#192281,#192282,#192283,#192284,
#192285,#192286,#192287,#192288,#192289,#192290,#192291,#192292,#192293,
#192294,#192295,#192296,#192297,#192298,#192299,#192300,#192301,#192302,
#192303,#192304,#192305,#192306,#192307,#192308,#192309,#192310,#192311,
#192312,#192313,#192314,#192315,#192316,#192317,#192318,#192319,#192320,
#192321,#192322,#192323,#192324,#192325,#192326,#192327,#192328,#192329,
#192330,#192331,#192332,#192333,#192334,#192335,#192336,#192337,#192338,
#192339,#192340,#192341,#192342,#192343,#192344,#192345,#192346,#192347,
#192348,#192349,#192350,#192351,#192352,#192353,#192354,#192355,#192356,
#192357,#192358,#192359,#192360,#192361,#192362,#192363,#192364,#192365,
#192366,#192367,#192368,#192369,#192370,#192371,#192372,#192373,#192374,
#192375,#192376,#192377,#192378,#192379,#192380,#192381,#192382,#192383,
#192384,#192385,#192386,#192387,#192388,#192389,#192390,#192391,#192392,
#192393,#192394,#192395,#192396,#192397,#192398,#192399,#192400,#192401,
#192402,#192403,#192404,#192405,#192406,#192407,#192408,#192409,#192410),
 .UNSPECIFIED.,.F.,.F.)
B_SPLINE_CURVE_WITH_KNOTS((6,1,1,1,1,1,1,1,1,1,1,1,1,1,1,1,1,1,1,1,1,1,
1,1,1,1,1,1,1,1,1,1,1,1,1,1,1,1,1,1,1,1,1,1,1,1,1,1,1,1,1,1,1,1,1,1,1,1,
1,1,1,1,1,1,1,1,1,1,1,1,1,1,1,1,1,1,1,1,1,1,1,1,1,1,1,1,1,1,1,1,1,1,1,1,
1,1,1,1,1,1,1,1,1,1,1,1,1,1,1,1,1,1,1,1,1,1,1,1,1,1,1,1,1,1,1,1,1,1,1,1,
1,1,1,1,1,1,1,1,1,1,1,1,1,1,1,1,1,1,1,1,1,1,1,1,1,1,1,1,1,1,1,1,1,1,1,1,
1,1,1,1,1,1,1,1,1,1,1,1,1,1,1,1,1,1,1,1,1,1,1,1,1,1,1,1,1,1,1,1,1,1,6),
(-1.,-0.995000000000001,-0.990000000000001,-0.985000000000001,-0.980000000000001,
-0.975000000000001,-0.970000000000001,-0.965000000000001,-0.960000000000001,
-0.955000000000001,-0.950000000000001,-0.945000000000001,-0.940000000000001,
-0.935000000000001,-0.930000000000001,-0.925000000000001,-0.920000000000001,
-0.915000000000001,-0.910000000000001,-0.905000000000001,-0.900000000000001,
-0.895000000000001,-0.890000000000001,-0.885000000000001,-0.880000000000001,
-0.875000000000001,-0.870000000000001,-0.865000000000001,-0.860000000000001,
-0.855000000000001,-0.850000000000001,-0.845000000000001,-0.840000000000001,
-0.835000000000001,-0.830000000000001,-0.825000000000001,-0.820000000000001,
-0.815000000000001,-0.810000000000001,-0.805000000000001,-0.800000000000001,
-0.795000000000001,-0.790000000000001,-0.785000000000001,-0.780000000000001,
-0.775000000000001,-0.770000000000001,-0.765000000000001,-0.760000000000001,
-0.755000000000001,-0.750000000000001,-0.745000000000001,-0.740000000000001,
-0.735000000000001,-0.730000000000001,-0.725000000000001,-0.720000000000001,
-0.715000000000001,-0.710000000000001,-0.705000000000001,-0.700000000000001,
-0.695000000000001,-0.690000000000001,-0.685,-0.68,-0.675,-0.67,-0.665,
-0.66,-0.655,-0.65,-0.645,-0.64,-0.635,-0.63,-0.625,-0.62,-0.615,-0.61,
-0.605,-0.6,-0.595,-0.59,-0.585,-0.58,-0.575,-0.57,-0.565,-0.56,-0.555,
-0.55,-0.545,-0.54,-0.535,-0.53,-0.525,-0.52,-0.515,-0.51,-0.505,-0.5,-0.495,
-0.49,-0.485,-0.48,-0.475,-0.47,-0.465,-0.46,-0.455,-0.45,-0.445,-0.44,
-0.435,-0.43,-0.425,-0.42,-0.415,-0.41,-0.405,-0.4,-0.395,-0.39,-0.385,
-0.38,-0.375,-0.37,-0.365,-0.36,-0.355,-0.35,-0.345,-0.34,-0.335,-0.33,
-0.325,-0.32,-0.315,-0.31,-0.305,-0.3,-0.295,-0.29,-0.285,-0.28,-0.275,
-0.27,-0.265,-0.26,-0.255,-0.25,-0.245,-0.24,-0.235,-0.23,-0.225,-0.22,
-0.215,-0.21,-0.205,-0.2,-0.195,-0.19,-0.185,-0.18,-0.175,-0.17,-0.165,
-0.16,-0.155,-0.15,-0.145,-0.14,-0.135,-0.13,-0.125,-0.12,-0.115,-0.11,
-0.105,-0.1,-0.095,-0.09,-0.085,-0.08,-0.075,-0.07,-0.065,-0.06,-0.055,
-0.05,-0.045,-0.04,-0.035,-0.03,-0.025,-0.02,-0.015,-0.01,-0.005,0.),
 .UNSPECIFIED.)
CURVE()
GEOMETRIC_REPRESENTATION_ITEM()
RATIONAL_B_SPLINE_CURVE((1.,1.,1.,1.,1.,1.,1.,1.,1.,1.,1.,1.,1.,1.,1.,1.,
1.,1.,1.,1.,1.,1.,1.,1.,1.,1.,1.,1.,1.,1.,1.,1.,1.,1.,1.,1.,1.,1.,1.,1.,
1.,1.,1.,1.,1.,1.,1.,1.,1.,1.,1.,1.,1.,1.,1.,1.,1.,1.,1.,1.,1.,1.,1.,1.,
1.,1.,1.,1.,1.,1.,1.,1.,1.,1.,1.,1.,1.,1.,1.,1.,1.,1.,1.,1.,1.,1.,1.,1.,
1.,1.,1.,1.,1.,1.,1.,1.,1.,1.,1.,1.,1.,1.,1.,1.,1.,1.,1.,1.,1.,1.,1.,1.,
1.,1.,1.,1.,1.,1.,1.,1.,1.,1.,1.,1.,1.,1.,1.,1.,1.,1.,1.,1.,1.,1.,1.,1.,
1.,1.,1.,1.,1.,1.,1.,1.,1.,1.,1.,1.,1.,1.,1.,1.,1.,1.,1.,1.,1.,1.,1.,1.,
1.,1.,1.,1.,1.,1.,1.,1.,1.,1.,1.,1.,1.,1.,1.,1.,1.,1.,1.,1.,1.,1.,1.,1.,
1.,1.,1.,1.,1.,1.,1.,1.,1.,1.,1.,1.,1.,1.,1.,1.,1.,1.,1.,1.,1.))
REPRESENTATION_ITEM('')
);
#750=(
BOUNDED_CURVE()
B_SPLINE_CURVE(5,(#192823,#192824,#192825,#192826,#192827,#192828,#192829,
#192830,#192831,#192832,#192833,#192834,#192835,#192836,#192837,#192838,
#192839,#192840,#192841,#192842,#192843,#192844,#192845,#192846,#192847,
#192848,#192849,#192850,#192851,#192852,#192853,#192854,#192855,#192856,
#192857,#192858,#192859,#192860,#192861,#192862,#192863,#192864,#192865,
#192866,#192867,#192868,#192869,#192870,#192871,#192872,#192873,#192874,
#192875,#192876,#192877,#192878,#192879,#192880,#192881,#192882,#192883,
#192884,#192885,#192886,#192887,#192888,#192889,#192890,#192891,#192892,
#192893,#192894,#192895,#192896,#192897,#192898,#192899,#192900,#192901,
#192902,#192903,#192904,#192905,#192906,#192907,#192908,#192909,#192910,
#192911,#192912,#192913,#192914,#192915,#192916,#192917,#192918,#192919,
#192920,#192921,#192922,#192923,#192924,#192925,#192926,#192927,#192928,
#192929,#192930,#192931,#192932,#192933,#192934,#192935,#192936,#192937,
#192938,#192939,#192940,#192941,#192942,#192943,#192944,#192945,#192946,
#192947,#192948,#192949,#192950,#192951,#192952,#192953,#192954,#192955,
#192956,#192957,#192958,#192959,#192960,#192961,#192962,#192963,#192964,
#192965,#192966,#192967,#192968,#192969,#192970,#192971,#192972,#192973,
#192974,#192975,#192976,#192977,#192978,#192979,#192980,#192981,#192982,
#192983,#192984,#192985,#192986,#192987,#192988,#192989,#192990,#192991,
#192992,#192993,#192994,#192995,#192996,#192997,#192998,#192999,#193000,
#193001,#193002,#193003,#193004,#193005,#193006,#193007,#193008,#193009,
#193010,#193011,#193012,#193013,#193014,#193015,#193016,#193017,#193018,
#193019,#193020,#193021,#193022,#193023,#193024,#193025,#193026,#193027),
 .UNSPECIFIED.,.F.,.F.)
B_SPLINE_CURVE_WITH_KNOTS((6,1,1,1,1,1,1,1,1,1,1,1,1,1,1,1,1,1,1,1,1,1,
1,1,1,1,1,1,1,1,1,1,1,1,1,1,1,1,1,1,1,1,1,1,1,1,1,1,1,1,1,1,1,1,1,1,1,1,
1,1,1,1,1,1,1,1,1,1,1,1,1,1,1,1,1,1,1,1,1,1,1,1,1,1,1,1,1,1,1,1,1,1,1,1,
1,1,1,1,1,1,1,1,1,1,1,1,1,1,1,1,1,1,1,1,1,1,1,1,1,1,1,1,1,1,1,1,1,1,1,1,
1,1,1,1,1,1,1,1,1,1,1,1,1,1,1,1,1,1,1,1,1,1,1,1,1,1,1,1,1,1,1,1,1,1,1,1,
1,1,1,1,1,1,1,1,1,1,1,1,1,1,1,1,1,1,1,1,1,1,1,1,1,1,1,1,1,1,1,1,1,1,6),
(0.,0.005,0.01,0.015,0.02,0.025,0.03,0.035,0.04,0.045,0.05,0.055,0.06,0.065,
0.07,0.075,0.08,0.085,0.09,0.095,0.1,0.105,0.11,0.115,0.12,0.125,0.13,0.135,
0.14,0.145,0.15,0.155,0.16,0.165,0.17,0.175,0.18,0.185,0.19,0.195,0.2,0.205,
0.21,0.215,0.22,0.225,0.23,0.235,0.24,0.245,0.25,0.255,0.26,0.265,0.27,
0.275,0.28,0.285,0.29,0.295,0.3,0.305,0.31,0.315,0.32,0.325,0.33,0.335,
0.34,0.345,0.35,0.355,0.36,0.365,0.37,0.375,0.38,0.385,0.39,0.395,0.4,0.405,
0.41,0.415,0.42,0.425,0.43,0.435,0.44,0.445,0.45,0.455,0.46,0.465,0.47,
0.475,0.48,0.485,0.49,0.495,0.5,0.505,0.51,0.515,0.52,0.525,0.53,0.535,
0.54,0.545,0.55,0.555,0.56,0.565,0.57,0.575,0.58,0.585,0.59,0.595,0.6,0.605,
0.61,0.615,0.62,0.625,0.63,0.635,0.64,0.645,0.65,0.655,0.66,0.665,0.67,
0.675,0.68,0.685,0.690000000000001,0.695000000000001,0.700000000000001,
0.705000000000001,0.710000000000001,0.715000000000001,0.720000000000001,
0.725000000000001,0.730000000000001,0.735000000000001,0.740000000000001,
0.745000000000001,0.750000000000001,0.755000000000001,0.760000000000001,
0.765000000000001,0.770000000000001,0.775000000000001,0.780000000000001,
0.785000000000001,0.790000000000001,0.795000000000001,0.800000000000001,
0.805000000000001,0.810000000000001,0.815000000000001,0.820000000000001,
0.825000000000001,0.830000000000001,0.835000000000001,0.840000000000001,
0.845000000000001,0.850000000000001,0.855000000000001,0.860000000000001,
0.865000000000001,0.870000000000001,0.875000000000001,0.880000000000001,
0.885000000000001,0.890000000000001,0.895000000000001,0.900000000000001,
0.905000000000001,0.910000000000001,0.915000000000001,0.920000000000001,
0.925000000000001,0.930000000000001,0.935000000000001,0.940000000000001,
0.945000000000001,0.950000000000001,0.955000000000001,0.960000000000001,
0.965000000000001,0.970000000000001,0.975000000000001,0.980000000000001,
0.985000000000001,0.990000000000001,0.995000000000001,1.),.UNSPECIFIED.)
CURVE()
GEOMETRIC_REPRESENTATION_ITEM()
RATIONAL_B_SPLINE_CURVE((1.,1.,1.,1.,1.,1.,1.,1.,1.,1.,1.,1.,1.,1.,1.,1.,
1.,1.,1.,1.,1.,1.,1.,1.,1.,1.,1.,1.,1.,1.,1.,1.,1.,1.,1.,1.,1.,1.,1.,1.,
1.,1.,1.,1.,1.,1.,1.,1.,1.,1.,1.,1.,1.,1.,1.,1.,1.,1.,1.,1.,1.,1.,1.,1.,
1.,1.,1.,1.,1.,1.,1.,1.,1.,1.,1.,1.,1.,1.,1.,1.,1.,1.,1.,1.,1.,1.,1.,1.,
1.,1.,1.,1.,1.,1.,1.,1.,1.,1.,1.,1.,1.,1.,1.,1.,1.,1.,1.,1.,1.,1.,1.,1.,
1.,1.,1.,1.,1.,1.,1.,1.,1.,1.,1.,1.,1.,1.,1.,1.,1.,1.,1.,1.,1.,1.,1.,1.,
1.,1.,1.,1.,1.,1.,1.,1.,1.,1.,1.,1.,1.,1.,1.,1.,1.,1.,1.,1.,1.,1.,1.,1.,
1.,1.,1.,1.,1.,1.,1.,1.,1.,1.,1.,1.,1.,1.,1.,1.,1.,1.,1.,1.,1.,1.,1.,1.,
1.,1.,1.,1.,1.,1.,1.,1.,1.,1.,1.,1.,1.,1.,1.,1.,1.,1.,1.,1.,1.))
REPRESENTATION_ITEM('')
);
#751=(
BOUNDED_CURVE()
B_SPLINE_CURVE(5,(#193444,#193445,#193446,#193447,#193448,#193449,#193450,
#193451,#193452,#193453,#193454,#193455,#193456,#193457,#193458,#193459,
#193460,#193461,#193462,#193463,#193464,#193465,#193466,#193467,#193468,
#193469,#193470,#193471,#193472,#193473,#193474,#193475,#193476,#193477,
#193478,#193479,#193480,#193481,#193482,#193483,#193484,#193485,#193486,
#193487,#193488,#193489,#193490,#193491,#193492,#193493,#193494,#193495,
#193496,#193497,#193498,#193499,#193500,#193501,#193502,#193503,#193504,
#193505,#193506,#193507,#193508,#193509,#193510,#193511,#193512,#193513,
#193514,#193515,#193516,#193517,#193518,#193519,#193520,#193521,#193522,
#193523,#193524,#193525,#193526,#193527,#193528,#193529,#193530,#193531,
#193532,#193533,#193534,#193535,#193536,#193537,#193538,#193539,#193540,
#193541,#193542,#193543,#193544,#193545,#193546,#193547,#193548,#193549,
#193550,#193551,#193552,#193553,#193554,#193555,#193556,#193557,#193558,
#193559,#193560,#193561,#193562,#193563,#193564,#193565,#193566,#193567,
#193568,#193569,#193570,#193571,#193572,#193573,#193574,#193575,#193576,
#193577,#193578,#193579,#193580,#193581,#193582,#193583,#193584,#193585,
#193586,#193587,#193588,#193589,#193590,#193591,#193592,#193593,#193594,
#193595,#193596,#193597,#193598,#193599,#193600,#193601,#193602,#193603,
#193604,#193605,#193606,#193607,#193608,#193609,#193610,#193611,#193612,
#193613,#193614,#193615,#193616,#193617,#193618,#193619,#193620,#193621,
#193622,#193623,#193624,#193625,#193626,#193627,#193628,#193629,#193630,
#193631,#193632,#193633,#193634,#193635,#193636,#193637,#193638,#193639,
#193640,#193641,#193642,#193643,#193644,#193645,#193646,#193647,#193648),
 .UNSPECIFIED.,.F.,.F.)
B_SPLINE_CURVE_WITH_KNOTS((6,1,1,1,1,1,1,1,1,1,1,1,1,1,1,1,1,1,1,1,1,1,
1,1,1,1,1,1,1,1,1,1,1,1,1,1,1,1,1,1,1,1,1,1,1,1,1,1,1,1,1,1,1,1,1,1,1,1,
1,1,1,1,1,1,1,1,1,1,1,1,1,1,1,1,1,1,1,1,1,1,1,1,1,1,1,1,1,1,1,1,1,1,1,1,
1,1,1,1,1,1,1,1,1,1,1,1,1,1,1,1,1,1,1,1,1,1,1,1,1,1,1,1,1,1,1,1,1,1,1,1,
1,1,1,1,1,1,1,1,1,1,1,1,1,1,1,1,1,1,1,1,1,1,1,1,1,1,1,1,1,1,1,1,1,1,1,1,
1,1,1,1,1,1,1,1,1,1,1,1,1,1,1,1,1,1,1,1,1,1,1,1,1,1,1,1,1,1,1,1,1,1,6),
(-1.,-0.995000000000001,-0.990000000000001,-0.985000000000001,-0.980000000000001,
-0.975000000000001,-0.970000000000001,-0.965000000000001,-0.960000000000001,
-0.955000000000001,-0.950000000000001,-0.945000000000001,-0.940000000000001,
-0.935000000000001,-0.930000000000001,-0.925000000000001,-0.920000000000001,
-0.915000000000001,-0.910000000000001,-0.905000000000001,-0.900000000000001,
-0.895000000000001,-0.890000000000001,-0.885000000000001,-0.880000000000001,
-0.875000000000001,-0.870000000000001,-0.865000000000001,-0.860000000000001,
-0.855000000000001,-0.850000000000001,-0.845000000000001,-0.840000000000001,
-0.835000000000001,-0.830000000000001,-0.825000000000001,-0.820000000000001,
-0.815000000000001,-0.810000000000001,-0.805000000000001,-0.800000000000001,
-0.795000000000001,-0.790000000000001,-0.785000000000001,-0.780000000000001,
-0.775000000000001,-0.770000000000001,-0.765000000000001,-0.760000000000001,
-0.755000000000001,-0.750000000000001,-0.745000000000001,-0.740000000000001,
-0.735000000000001,-0.730000000000001,-0.725000000000001,-0.720000000000001,
-0.715000000000001,-0.710000000000001,-0.705000000000001,-0.700000000000001,
-0.695000000000001,-0.690000000000001,-0.685,-0.68,-0.675,-0.67,-0.665,
-0.66,-0.655,-0.65,-0.645,-0.64,-0.635,-0.63,-0.625,-0.62,-0.615,-0.61,
-0.605,-0.6,-0.595,-0.59,-0.585,-0.58,-0.575,-0.57,-0.565,-0.56,-0.555,
-0.55,-0.545,-0.54,-0.535,-0.53,-0.525,-0.52,-0.515,-0.51,-0.505,-0.5,-0.495,
-0.49,-0.485,-0.48,-0.475,-0.47,-0.465,-0.46,-0.455,-0.45,-0.445,-0.44,
-0.435,-0.43,-0.425,-0.42,-0.415,-0.41,-0.405,-0.4,-0.395,-0.39,-0.385,
-0.38,-0.375,-0.37,-0.365,-0.36,-0.355,-0.35,-0.345,-0.34,-0.335,-0.33,
-0.325,-0.32,-0.315,-0.31,-0.305,-0.3,-0.295,-0.29,-0.285,-0.28,-0.275,
-0.27,-0.265,-0.26,-0.255,-0.25,-0.245,-0.24,-0.235,-0.23,-0.225,-0.22,
-0.215,-0.21,-0.205,-0.2,-0.195,-0.19,-0.185,-0.18,-0.175,-0.17,-0.165,
-0.16,-0.155,-0.15,-0.145,-0.14,-0.135,-0.13,-0.125,-0.12,-0.115,-0.11,
-0.105,-0.1,-0.095,-0.09,-0.085,-0.08,-0.075,-0.07,-0.065,-0.06,-0.055,
-0.05,-0.045,-0.04,-0.035,-0.03,-0.025,-0.02,-0.015,-0.01,-0.005,0.),
 .UNSPECIFIED.)
CURVE()
GEOMETRIC_REPRESENTATION_ITEM()
RATIONAL_B_SPLINE_CURVE((1.,1.,1.,1.,1.,1.,1.,1.,1.,1.,1.,1.,1.,1.,1.,1.,
1.,1.,1.,1.,1.,1.,1.,1.,1.,1.,1.,1.,1.,1.,1.,1.,1.,1.,1.,1.,1.,1.,1.,1.,
1.,1.,1.,1.,1.,1.,1.,1.,1.,1.,1.,1.,1.,1.,1.,1.,1.,1.,1.,1.,1.,1.,1.,1.,
1.,1.,1.,1.,1.,1.,1.,1.,1.,1.,1.,1.,1.,1.,1.,1.,1.,1.,1.,1.,1.,1.,1.,1.,
1.,1.,1.,1.,1.,1.,1.,1.,1.,1.,1.,1.,1.,1.,1.,1.,1.,1.,1.,1.,1.,1.,1.,1.,
1.,1.,1.,1.,1.,1.,1.,1.,1.,1.,1.,1.,1.,1.,1.,1.,1.,1.,1.,1.,1.,1.,1.,1.,
1.,1.,1.,1.,1.,1.,1.,1.,1.,1.,1.,1.,1.,1.,1.,1.,1.,1.,1.,1.,1.,1.,1.,1.,
1.,1.,1.,1.,1.,1.,1.,1.,1.,1.,1.,1.,1.,1.,1.,1.,1.,1.,1.,1.,1.,1.,1.,1.,
1.,1.,1.,1.,1.,1.,1.,1.,1.,1.,1.,1.,1.,1.,1.,1.,1.,1.,1.,1.,1.))
REPRESENTATION_ITEM('')
);
#752=(
BOUNDED_CURVE()
B_SPLINE_CURVE(5,(#194061,#194062,#194063,#194064,#194065,#194066,#194067,
#194068,#194069,#194070,#194071,#194072,#194073,#194074,#194075,#194076,
#194077,#194078,#194079,#194080,#194081,#194082,#194083,#194084,#194085,
#194086,#194087,#194088,#194089,#194090,#194091,#194092,#194093,#194094,
#194095,#194096,#194097,#194098,#194099,#194100,#194101,#194102,#194103,
#194104,#194105,#194106,#194107,#194108,#194109,#194110,#194111,#194112,
#194113,#194114,#194115,#194116,#194117,#194118,#194119,#194120,#194121,
#194122,#194123,#194124,#194125,#194126,#194127,#194128,#194129,#194130,
#194131,#194132,#194133,#194134,#194135,#194136,#194137,#194138,#194139,
#194140,#194141,#194142,#194143,#194144,#194145,#194146,#194147,#194148,
#194149,#194150,#194151,#194152,#194153,#194154,#194155,#194156,#194157,
#194158,#194159,#194160,#194161,#194162,#194163,#194164,#194165,#194166,
#194167,#194168,#194169,#194170,#194171,#194172,#194173,#194174,#194175,
#194176,#194177,#194178,#194179,#194180,#194181,#194182,#194183,#194184,
#194185,#194186,#194187,#194188,#194189,#194190,#194191,#194192,#194193,
#194194,#194195,#194196,#194197,#194198,#194199,#194200,#194201,#194202,
#194203,#194204,#194205,#194206,#194207,#194208,#194209,#194210,#194211,
#194212,#194213,#194214,#194215,#194216,#194217,#194218,#194219,#194220,
#194221,#194222,#194223,#194224,#194225,#194226,#194227,#194228,#194229,
#194230,#194231,#194232,#194233,#194234,#194235,#194236,#194237,#194238,
#194239,#194240,#194241,#194242,#194243,#194244,#194245,#194246,#194247,
#194248,#194249,#194250,#194251,#194252,#194253,#194254,#194255,#194256,
#194257,#194258,#194259,#194260,#194261,#194262,#194263,#194264,#194265),
 .UNSPECIFIED.,.F.,.F.)
B_SPLINE_CURVE_WITH_KNOTS((6,1,1,1,1,1,1,1,1,1,1,1,1,1,1,1,1,1,1,1,1,1,
1,1,1,1,1,1,1,1,1,1,1,1,1,1,1,1,1,1,1,1,1,1,1,1,1,1,1,1,1,1,1,1,1,1,1,1,
1,1,1,1,1,1,1,1,1,1,1,1,1,1,1,1,1,1,1,1,1,1,1,1,1,1,1,1,1,1,1,1,1,1,1,1,
1,1,1,1,1,1,1,1,1,1,1,1,1,1,1,1,1,1,1,1,1,1,1,1,1,1,1,1,1,1,1,1,1,1,1,1,
1,1,1,1,1,1,1,1,1,1,1,1,1,1,1,1,1,1,1,1,1,1,1,1,1,1,1,1,1,1,1,1,1,1,1,1,
1,1,1,1,1,1,1,1,1,1,1,1,1,1,1,1,1,1,1,1,1,1,1,1,1,1,1,1,1,1,1,1,1,1,6),
(0.,0.005,0.01,0.015,0.02,0.025,0.03,0.035,0.04,0.045,0.05,0.055,0.06,0.065,
0.07,0.075,0.08,0.085,0.09,0.095,0.1,0.105,0.11,0.115,0.12,0.125,0.13,0.135,
0.14,0.145,0.15,0.155,0.16,0.165,0.17,0.175,0.18,0.185,0.19,0.195,0.2,0.205,
0.21,0.215,0.22,0.225,0.23,0.235,0.24,0.245,0.25,0.255,0.26,0.265,0.27,
0.275,0.28,0.285,0.29,0.295,0.3,0.305,0.31,0.315,0.32,0.325,0.33,0.335,
0.34,0.345,0.35,0.355,0.36,0.365,0.37,0.375,0.38,0.385,0.39,0.395,0.4,0.405,
0.41,0.415,0.42,0.425,0.43,0.435,0.44,0.445,0.45,0.455,0.46,0.465,0.47,
0.475,0.48,0.485,0.49,0.495,0.5,0.505,0.51,0.515,0.52,0.525,0.53,0.535,
0.54,0.545,0.55,0.555,0.56,0.565,0.57,0.575,0.58,0.585,0.59,0.595,0.6,0.605,
0.61,0.615,0.62,0.625,0.63,0.635,0.64,0.645,0.65,0.655,0.66,0.665,0.67,
0.675,0.68,0.685,0.690000000000001,0.695000000000001,0.700000000000001,
0.705000000000001,0.710000000000001,0.715000000000001,0.720000000000001,
0.725000000000001,0.730000000000001,0.735000000000001,0.740000000000001,
0.745000000000001,0.750000000000001,0.755000000000001,0.760000000000001,
0.765000000000001,0.770000000000001,0.775000000000001,0.780000000000001,
0.785000000000001,0.790000000000001,0.795000000000001,0.800000000000001,
0.805000000000001,0.810000000000001,0.815000000000001,0.820000000000001,
0.825000000000001,0.830000000000001,0.835000000000001,0.840000000000001,
0.845000000000001,0.850000000000001,0.855000000000001,0.860000000000001,
0.865000000000001,0.870000000000001,0.875000000000001,0.880000000000001,
0.885000000000001,0.890000000000001,0.895000000000001,0.900000000000001,
0.905000000000001,0.910000000000001,0.915000000000001,0.920000000000001,
0.925000000000001,0.930000000000001,0.935000000000001,0.940000000000001,
0.945000000000001,0.950000000000001,0.955000000000001,0.960000000000001,
0.965000000000001,0.970000000000001,0.975000000000001,0.980000000000001,
0.985000000000001,0.990000000000001,0.995000000000001,1.),.UNSPECIFIED.)
CURVE()
GEOMETRIC_REPRESENTATION_ITEM()
RATIONAL_B_SPLINE_CURVE((1.,1.,1.,1.,1.,1.,1.,1.,1.,1.,1.,1.,1.,1.,1.,1.,
1.,1.,1.,1.,1.,1.,1.,1.,1.,1.,1.,1.,1.,1.,1.,1.,1.,1.,1.,1.,1.,1.,1.,1.,
1.,1.,1.,1.,1.,1.,1.,1.,1.,1.,1.,1.,1.,1.,1.,1.,1.,1.,1.,1.,1.,1.,1.,1.,
1.,1.,1.,1.,1.,1.,1.,1.,1.,1.,1.,1.,1.,1.,1.,1.,1.,1.,1.,1.,1.,1.,1.,1.,
1.,1.,1.,1.,1.,1.,1.,1.,1.,1.,1.,1.,1.,1.,1.,1.,1.,1.,1.,1.,1.,1.,1.,1.,
1.,1.,1.,1.,1.,1.,1.,1.,1.,1.,1.,1.,1.,1.,1.,1.,1.,1.,1.,1.,1.,1.,1.,1.,
1.,1.,1.,1.,1.,1.,1.,1.,1.,1.,1.,1.,1.,1.,1.,1.,1.,1.,1.,1.,1.,1.,1.,1.,
1.,1.,1.,1.,1.,1.,1.,1.,1.,1.,1.,1.,1.,1.,1.,1.,1.,1.,1.,1.,1.,1.,1.,1.,
1.,1.,1.,1.,1.,1.,1.,1.,1.,1.,1.,1.,1.,1.,1.,1.,1.,1.,1.,1.,1.))
REPRESENTATION_ITEM('')
);
#753=(
BOUNDED_CURVE()
B_SPLINE_CURVE(5,(#194682,#194683,#194684,#194685,#194686,#194687,#194688,
#194689,#194690,#194691,#194692,#194693,#194694,#194695,#194696,#194697,
#194698,#194699,#194700,#194701,#194702,#194703,#194704,#194705,#194706,
#194707,#194708,#194709,#194710,#194711,#194712,#194713,#194714,#194715,
#194716,#194717,#194718,#194719,#194720,#194721,#194722,#194723,#194724,
#194725,#194726,#194727,#194728,#194729,#194730,#194731,#194732,#194733,
#194734,#194735,#194736,#194737,#194738,#194739,#194740,#194741,#194742,
#194743,#194744,#194745,#194746,#194747,#194748,#194749,#194750,#194751,
#194752,#194753,#194754,#194755,#194756,#194757,#194758,#194759,#194760,
#194761,#194762,#194763,#194764,#194765,#194766,#194767,#194768,#194769,
#194770,#194771,#194772,#194773,#194774,#194775,#194776,#194777,#194778,
#194779,#194780,#194781,#194782,#194783,#194784,#194785,#194786,#194787,
#194788,#194789,#194790,#194791,#194792,#194793,#194794,#194795,#194796,
#194797,#194798,#194799,#194800,#194801,#194802,#194803,#194804,#194805,
#194806,#194807,#194808,#194809,#194810,#194811,#194812,#194813,#194814,
#194815,#194816,#194817,#194818,#194819,#194820,#194821,#194822,#194823,
#194824,#194825,#194826,#194827,#194828,#194829,#194830,#194831,#194832,
#194833,#194834,#194835,#194836,#194837,#194838,#194839,#194840,#194841,
#194842,#194843,#194844,#194845,#194846,#194847,#194848,#194849,#194850,
#194851,#194852,#194853,#194854,#194855,#194856,#194857,#194858,#194859,
#194860,#194861,#194862,#194863,#194864,#194865,#194866,#194867,#194868,
#194869,#194870,#194871,#194872,#194873,#194874,#194875,#194876,#194877,
#194878,#194879,#194880,#194881,#194882,#194883,#194884,#194885,#194886),
 .UNSPECIFIED.,.F.,.F.)
B_SPLINE_CURVE_WITH_KNOTS((6,1,1,1,1,1,1,1,1,1,1,1,1,1,1,1,1,1,1,1,1,1,
1,1,1,1,1,1,1,1,1,1,1,1,1,1,1,1,1,1,1,1,1,1,1,1,1,1,1,1,1,1,1,1,1,1,1,1,
1,1,1,1,1,1,1,1,1,1,1,1,1,1,1,1,1,1,1,1,1,1,1,1,1,1,1,1,1,1,1,1,1,1,1,1,
1,1,1,1,1,1,1,1,1,1,1,1,1,1,1,1,1,1,1,1,1,1,1,1,1,1,1,1,1,1,1,1,1,1,1,1,
1,1,1,1,1,1,1,1,1,1,1,1,1,1,1,1,1,1,1,1,1,1,1,1,1,1,1,1,1,1,1,1,1,1,1,1,
1,1,1,1,1,1,1,1,1,1,1,1,1,1,1,1,1,1,1,1,1,1,1,1,1,1,1,1,1,1,1,1,1,1,6),
(-1.,-0.995000000000001,-0.990000000000001,-0.985000000000001,-0.980000000000001,
-0.975000000000001,-0.970000000000001,-0.965000000000001,-0.960000000000001,
-0.955000000000001,-0.950000000000001,-0.945000000000001,-0.940000000000001,
-0.935000000000001,-0.930000000000001,-0.925000000000001,-0.920000000000001,
-0.915000000000001,-0.910000000000001,-0.905000000000001,-0.900000000000001,
-0.895000000000001,-0.890000000000001,-0.885000000000001,-0.880000000000001,
-0.875000000000001,-0.870000000000001,-0.865000000000001,-0.860000000000001,
-0.855000000000001,-0.850000000000001,-0.845000000000001,-0.840000000000001,
-0.835000000000001,-0.830000000000001,-0.825000000000001,-0.820000000000001,
-0.815000000000001,-0.810000000000001,-0.805000000000001,-0.800000000000001,
-0.795000000000001,-0.790000000000001,-0.785000000000001,-0.780000000000001,
-0.775000000000001,-0.770000000000001,-0.765000000000001,-0.760000000000001,
-0.755000000000001,-0.750000000000001,-0.745000000000001,-0.740000000000001,
-0.735000000000001,-0.730000000000001,-0.725000000000001,-0.720000000000001,
-0.715000000000001,-0.710000000000001,-0.705000000000001,-0.700000000000001,
-0.695000000000001,-0.690000000000001,-0.685,-0.68,-0.675,-0.67,-0.665,
-0.66,-0.655,-0.65,-0.645,-0.64,-0.635,-0.63,-0.625,-0.62,-0.615,-0.61,
-0.605,-0.6,-0.595,-0.59,-0.585,-0.58,-0.575,-0.57,-0.565,-0.56,-0.555,
-0.55,-0.545,-0.54,-0.535,-0.53,-0.525,-0.52,-0.515,-0.51,-0.505,-0.5,-0.495,
-0.49,-0.485,-0.48,-0.475,-0.47,-0.465,-0.46,-0.455,-0.45,-0.445,-0.44,
-0.435,-0.43,-0.425,-0.42,-0.415,-0.41,-0.405,-0.4,-0.395,-0.39,-0.385,
-0.38,-0.375,-0.37,-0.365,-0.36,-0.355,-0.35,-0.345,-0.34,-0.335,-0.33,
-0.325,-0.32,-0.315,-0.31,-0.305,-0.3,-0.295,-0.29,-0.285,-0.28,-0.275,
-0.27,-0.265,-0.26,-0.255,-0.25,-0.245,-0.24,-0.235,-0.23,-0.225,-0.22,
-0.215,-0.21,-0.205,-0.2,-0.195,-0.19,-0.185,-0.18,-0.175,-0.17,-0.165,
-0.16,-0.155,-0.15,-0.145,-0.14,-0.135,-0.13,-0.125,-0.12,-0.115,-0.11,
-0.105,-0.1,-0.095,-0.09,-0.085,-0.08,-0.075,-0.07,-0.065,-0.06,-0.055,
-0.05,-0.045,-0.04,-0.035,-0.03,-0.025,-0.02,-0.015,-0.01,-0.005,0.),
 .UNSPECIFIED.)
CURVE()
GEOMETRIC_REPRESENTATION_ITEM()
RATIONAL_B_SPLINE_CURVE((1.,1.,1.,1.,1.,1.,1.,1.,1.,1.,1.,1.,1.,1.,1.,1.,
1.,1.,1.,1.,1.,1.,1.,1.,1.,1.,1.,1.,1.,1.,1.,1.,1.,1.,1.,1.,1.,1.,1.,1.,
1.,1.,1.,1.,1.,1.,1.,1.,1.,1.,1.,1.,1.,1.,1.,1.,1.,1.,1.,1.,1.,1.,1.,1.,
1.,1.,1.,1.,1.,1.,1.,1.,1.,1.,1.,1.,1.,1.,1.,1.,1.,1.,1.,1.,1.,1.,1.,1.,
1.,1.,1.,1.,1.,1.,1.,1.,1.,1.,1.,1.,1.,1.,1.,1.,1.,1.,1.,1.,1.,1.,1.,1.,
1.,1.,1.,1.,1.,1.,1.,1.,1.,1.,1.,1.,1.,1.,1.,1.,1.,1.,1.,1.,1.,1.,1.,1.,
1.,1.,1.,1.,1.,1.,1.,1.,1.,1.,1.,1.,1.,1.,1.,1.,1.,1.,1.,1.,1.,1.,1.,1.,
1.,1.,1.,1.,1.,1.,1.,1.,1.,1.,1.,1.,1.,1.,1.,1.,1.,1.,1.,1.,1.,1.,1.,1.,
1.,1.,1.,1.,1.,1.,1.,1.,1.,1.,1.,1.,1.,1.,1.,1.,1.,1.,1.,1.,1.))
REPRESENTATION_ITEM('')
);
#754=(
BOUNDED_CURVE()
B_SPLINE_CURVE(5,(#195299,#195300,#195301,#195302,#195303,#195304,#195305,
#195306,#195307,#195308,#195309,#195310,#195311,#195312,#195313,#195314,
#195315,#195316,#195317,#195318,#195319,#195320,#195321,#195322,#195323,
#195324,#195325,#195326,#195327,#195328,#195329,#195330,#195331,#195332,
#195333,#195334,#195335,#195336,#195337,#195338,#195339,#195340,#195341,
#195342,#195343,#195344,#195345,#195346,#195347,#195348,#195349,#195350,
#195351,#195352,#195353,#195354,#195355,#195356,#195357,#195358,#195359,
#195360,#195361,#195362,#195363,#195364,#195365,#195366,#195367,#195368,
#195369,#195370,#195371,#195372,#195373,#195374,#195375,#195376,#195377,
#195378,#195379,#195380,#195381,#195382,#195383,#195384,#195385,#195386,
#195387,#195388,#195389,#195390,#195391,#195392,#195393,#195394,#195395,
#195396,#195397,#195398,#195399,#195400,#195401,#195402,#195403,#195404,
#195405,#195406,#195407,#195408,#195409,#195410,#195411,#195412,#195413,
#195414,#195415,#195416,#195417,#195418,#195419,#195420,#195421,#195422,
#195423,#195424,#195425,#195426,#195427,#195428,#195429,#195430,#195431,
#195432,#195433,#195434,#195435,#195436,#195437,#195438,#195439,#195440,
#195441,#195442,#195443,#195444,#195445,#195446,#195447,#195448,#195449,
#195450,#195451,#195452,#195453,#195454,#195455,#195456,#195457,#195458,
#195459,#195460,#195461,#195462,#195463,#195464,#195465,#195466,#195467,
#195468,#195469,#195470,#195471,#195472,#195473,#195474,#195475,#195476,
#195477,#195478,#195479,#195480,#195481,#195482,#195483,#195484,#195485,
#195486,#195487,#195488,#195489,#195490,#195491,#195492,#195493,#195494,
#195495,#195496,#195497,#195498,#195499,#195500,#195501,#195502,#195503),
 .UNSPECIFIED.,.F.,.F.)
B_SPLINE_CURVE_WITH_KNOTS((6,1,1,1,1,1,1,1,1,1,1,1,1,1,1,1,1,1,1,1,1,1,
1,1,1,1,1,1,1,1,1,1,1,1,1,1,1,1,1,1,1,1,1,1,1,1,1,1,1,1,1,1,1,1,1,1,1,1,
1,1,1,1,1,1,1,1,1,1,1,1,1,1,1,1,1,1,1,1,1,1,1,1,1,1,1,1,1,1,1,1,1,1,1,1,
1,1,1,1,1,1,1,1,1,1,1,1,1,1,1,1,1,1,1,1,1,1,1,1,1,1,1,1,1,1,1,1,1,1,1,1,
1,1,1,1,1,1,1,1,1,1,1,1,1,1,1,1,1,1,1,1,1,1,1,1,1,1,1,1,1,1,1,1,1,1,1,1,
1,1,1,1,1,1,1,1,1,1,1,1,1,1,1,1,1,1,1,1,1,1,1,1,1,1,1,1,1,1,1,1,1,1,6),
(0.,0.005,0.01,0.015,0.02,0.025,0.03,0.035,0.04,0.045,0.05,0.055,0.06,0.065,
0.07,0.075,0.08,0.085,0.09,0.095,0.1,0.105,0.11,0.115,0.12,0.125,0.13,0.135,
0.14,0.145,0.15,0.155,0.16,0.165,0.17,0.175,0.18,0.185,0.19,0.195,0.2,0.205,
0.21,0.215,0.22,0.225,0.23,0.235,0.24,0.245,0.25,0.255,0.26,0.265,0.27,
0.275,0.28,0.285,0.29,0.295,0.3,0.305,0.31,0.315,0.32,0.325,0.33,0.335,
0.34,0.345,0.35,0.355,0.36,0.365,0.37,0.375,0.38,0.385,0.39,0.395,0.4,0.405,
0.41,0.415,0.42,0.425,0.43,0.435,0.44,0.445,0.45,0.455,0.46,0.465,0.47,
0.475,0.48,0.485,0.49,0.495,0.5,0.505,0.51,0.515,0.52,0.525,0.53,0.535,
0.54,0.545,0.55,0.555,0.56,0.565,0.57,0.575,0.58,0.585,0.59,0.595,0.6,0.605,
0.61,0.615,0.62,0.625,0.63,0.635,0.64,0.645,0.65,0.655,0.66,0.665,0.67,
0.675,0.68,0.685,0.690000000000001,0.695000000000001,0.700000000000001,
0.705000000000001,0.710000000000001,0.715000000000001,0.720000000000001,
0.725000000000001,0.730000000000001,0.735000000000001,0.740000000000001,
0.745000000000001,0.750000000000001,0.755000000000001,0.760000000000001,
0.765000000000001,0.770000000000001,0.775000000000001,0.780000000000001,
0.785000000000001,0.790000000000001,0.795000000000001,0.800000000000001,
0.805000000000001,0.810000000000001,0.815000000000001,0.820000000000001,
0.825000000000001,0.830000000000001,0.835000000000001,0.840000000000001,
0.845000000000001,0.850000000000001,0.855000000000001,0.860000000000001,
0.865000000000001,0.870000000000001,0.875000000000001,0.880000000000001,
0.885000000000001,0.890000000000001,0.895000000000001,0.900000000000001,
0.905000000000001,0.910000000000001,0.915000000000001,0.920000000000001,
0.925000000000001,0.930000000000001,0.935000000000001,0.940000000000001,
0.945000000000001,0.950000000000001,0.955000000000001,0.960000000000001,
0.965000000000001,0.970000000000001,0.975000000000001,0.980000000000001,
0.985000000000001,0.990000000000001,0.995000000000001,1.),.UNSPECIFIED.)
CURVE()
GEOMETRIC_REPRESENTATION_ITEM()
RATIONAL_B_SPLINE_CURVE((1.,1.,1.,1.,1.,1.,1.,1.,1.,1.,1.,1.,1.,1.,1.,1.,
1.,1.,1.,1.,1.,1.,1.,1.,1.,1.,1.,1.,1.,1.,1.,1.,1.,1.,1.,1.,1.,1.,1.,1.,
1.,1.,1.,1.,1.,1.,1.,1.,1.,1.,1.,1.,1.,1.,1.,1.,1.,1.,1.,1.,1.,1.,1.,1.,
1.,1.,1.,1.,1.,1.,1.,1.,1.,1.,1.,1.,1.,1.,1.,1.,1.,1.,1.,1.,1.,1.,1.,1.,
1.,1.,1.,1.,1.,1.,1.,1.,1.,1.,1.,1.,1.,1.,1.,1.,1.,1.,1.,1.,1.,1.,1.,1.,
1.,1.,1.,1.,1.,1.,1.,1.,1.,1.,1.,1.,1.,1.,1.,1.,1.,1.,1.,1.,1.,1.,1.,1.,
1.,1.,1.,1.,1.,1.,1.,1.,1.,1.,1.,1.,1.,1.,1.,1.,1.,1.,1.,1.,1.,1.,1.,1.,
1.,1.,1.,1.,1.,1.,1.,1.,1.,1.,1.,1.,1.,1.,1.,1.,1.,1.,1.,1.,1.,1.,1.,1.,
1.,1.,1.,1.,1.,1.,1.,1.,1.,1.,1.,1.,1.,1.,1.,1.,1.,1.,1.,1.,1.))
REPRESENTATION_ITEM('')
);
#755=(
BOUNDED_CURVE()
B_SPLINE_CURVE(5,(#195920,#195921,#195922,#195923,#195924,#195925,#195926,
#195927,#195928,#195929,#195930,#195931,#195932,#195933,#195934,#195935,
#195936,#195937,#195938,#195939,#195940,#195941,#195942,#195943,#195944,
#195945,#195946,#195947,#195948,#195949,#195950,#195951,#195952,#195953,
#195954,#195955,#195956,#195957,#195958,#195959,#195960,#195961,#195962,
#195963,#195964,#195965,#195966,#195967,#195968,#195969,#195970,#195971,
#195972,#195973,#195974,#195975,#195976,#195977,#195978,#195979,#195980,
#195981,#195982,#195983,#195984,#195985,#195986,#195987,#195988,#195989,
#195990,#195991,#195992,#195993,#195994,#195995,#195996,#195997,#195998,
#195999,#196000,#196001,#196002,#196003,#196004,#196005,#196006,#196007,
#196008,#196009,#196010,#196011,#196012,#196013,#196014,#196015,#196016,
#196017,#196018,#196019,#196020,#196021,#196022,#196023,#196024,#196025,
#196026,#196027,#196028,#196029,#196030,#196031,#196032,#196033,#196034,
#196035,#196036,#196037,#196038,#196039,#196040,#196041,#196042,#196043,
#196044,#196045,#196046,#196047,#196048,#196049,#196050,#196051,#196052,
#196053,#196054,#196055,#196056,#196057,#196058,#196059,#196060,#196061,
#196062,#196063,#196064,#196065,#196066,#196067,#196068,#196069,#196070,
#196071,#196072,#196073,#196074,#196075,#196076,#196077,#196078,#196079,
#196080,#196081,#196082,#196083,#196084,#196085,#196086,#196087,#196088,
#196089,#196090,#196091,#196092,#196093,#196094,#196095,#196096,#196097,
#196098,#196099,#196100,#196101,#196102,#196103,#196104,#196105,#196106,
#196107,#196108,#196109,#196110,#196111,#196112,#196113,#196114,#196115,
#196116,#196117,#196118,#196119,#196120,#196121,#196122,#196123,#196124),
 .UNSPECIFIED.,.F.,.F.)
B_SPLINE_CURVE_WITH_KNOTS((6,1,1,1,1,1,1,1,1,1,1,1,1,1,1,1,1,1,1,1,1,1,
1,1,1,1,1,1,1,1,1,1,1,1,1,1,1,1,1,1,1,1,1,1,1,1,1,1,1,1,1,1,1,1,1,1,1,1,
1,1,1,1,1,1,1,1,1,1,1,1,1,1,1,1,1,1,1,1,1,1,1,1,1,1,1,1,1,1,1,1,1,1,1,1,
1,1,1,1,1,1,1,1,1,1,1,1,1,1,1,1,1,1,1,1,1,1,1,1,1,1,1,1,1,1,1,1,1,1,1,1,
1,1,1,1,1,1,1,1,1,1,1,1,1,1,1,1,1,1,1,1,1,1,1,1,1,1,1,1,1,1,1,1,1,1,1,1,
1,1,1,1,1,1,1,1,1,1,1,1,1,1,1,1,1,1,1,1,1,1,1,1,1,1,1,1,1,1,1,1,1,1,6),
(-1.,-0.995000000000001,-0.990000000000001,-0.985000000000001,-0.980000000000001,
-0.975000000000001,-0.970000000000001,-0.965000000000001,-0.960000000000001,
-0.955000000000001,-0.950000000000001,-0.945000000000001,-0.940000000000001,
-0.935000000000001,-0.930000000000001,-0.925000000000001,-0.920000000000001,
-0.915000000000001,-0.910000000000001,-0.905000000000001,-0.900000000000001,
-0.895000000000001,-0.890000000000001,-0.885000000000001,-0.880000000000001,
-0.875000000000001,-0.870000000000001,-0.865000000000001,-0.860000000000001,
-0.855000000000001,-0.850000000000001,-0.845000000000001,-0.840000000000001,
-0.835000000000001,-0.830000000000001,-0.825000000000001,-0.820000000000001,
-0.815000000000001,-0.810000000000001,-0.805000000000001,-0.800000000000001,
-0.795000000000001,-0.790000000000001,-0.785000000000001,-0.780000000000001,
-0.775000000000001,-0.770000000000001,-0.765000000000001,-0.760000000000001,
-0.755000000000001,-0.750000000000001,-0.745000000000001,-0.740000000000001,
-0.735000000000001,-0.730000000000001,-0.725000000000001,-0.720000000000001,
-0.715000000000001,-0.710000000000001,-0.705000000000001,-0.700000000000001,
-0.695000000000001,-0.690000000000001,-0.685,-0.68,-0.675,-0.67,-0.665,
-0.66,-0.655,-0.65,-0.645,-0.64,-0.635,-0.63,-0.625,-0.62,-0.615,-0.61,
-0.605,-0.6,-0.595,-0.59,-0.585,-0.58,-0.575,-0.57,-0.565,-0.56,-0.555,
-0.55,-0.545,-0.54,-0.535,-0.53,-0.525,-0.52,-0.515,-0.51,-0.505,-0.5,-0.495,
-0.49,-0.485,-0.48,-0.475,-0.47,-0.465,-0.46,-0.455,-0.45,-0.445,-0.44,
-0.435,-0.43,-0.425,-0.42,-0.415,-0.41,-0.405,-0.4,-0.395,-0.39,-0.385,
-0.38,-0.375,-0.37,-0.365,-0.36,-0.355,-0.35,-0.345,-0.34,-0.335,-0.33,
-0.325,-0.32,-0.315,-0.31,-0.305,-0.3,-0.295,-0.29,-0.285,-0.28,-0.275,
-0.27,-0.265,-0.26,-0.255,-0.25,-0.245,-0.24,-0.235,-0.23,-0.225,-0.22,
-0.215,-0.21,-0.205,-0.2,-0.195,-0.19,-0.185,-0.18,-0.175,-0.17,-0.165,
-0.16,-0.155,-0.15,-0.145,-0.14,-0.135,-0.13,-0.125,-0.12,-0.115,-0.11,
-0.105,-0.1,-0.095,-0.09,-0.085,-0.08,-0.075,-0.07,-0.065,-0.06,-0.055,
-0.05,-0.045,-0.04,-0.035,-0.03,-0.025,-0.02,-0.015,-0.01,-0.005,0.),
 .UNSPECIFIED.)
CURVE()
GEOMETRIC_REPRESENTATION_ITEM()
RATIONAL_B_SPLINE_CURVE((1.,1.,1.,1.,1.,1.,1.,1.,1.,1.,1.,1.,1.,1.,1.,1.,
1.,1.,1.,1.,1.,1.,1.,1.,1.,1.,1.,1.,1.,1.,1.,1.,1.,1.,1.,1.,1.,1.,1.,1.,
1.,1.,1.,1.,1.,1.,1.,1.,1.,1.,1.,1.,1.,1.,1.,1.,1.,1.,1.,1.,1.,1.,1.,1.,
1.,1.,1.,1.,1.,1.,1.,1.,1.,1.,1.,1.,1.,1.,1.,1.,1.,1.,1.,1.,1.,1.,1.,1.,
1.,1.,1.,1.,1.,1.,1.,1.,1.,1.,1.,1.,1.,1.,1.,1.,1.,1.,1.,1.,1.,1.,1.,1.,
1.,1.,1.,1.,1.,1.,1.,1.,1.,1.,1.,1.,1.,1.,1.,1.,1.,1.,1.,1.,1.,1.,1.,1.,
1.,1.,1.,1.,1.,1.,1.,1.,1.,1.,1.,1.,1.,1.,1.,1.,1.,1.,1.,1.,1.,1.,1.,1.,
1.,1.,1.,1.,1.,1.,1.,1.,1.,1.,1.,1.,1.,1.,1.,1.,1.,1.,1.,1.,1.,1.,1.,1.,
1.,1.,1.,1.,1.,1.,1.,1.,1.,1.,1.,1.,1.,1.,1.,1.,1.,1.,1.,1.,1.))
REPRESENTATION_ITEM('')
);
#756=(
BOUNDED_CURVE()
B_SPLINE_CURVE(5,(#196537,#196538,#196539,#196540,#196541,#196542,#196543,
#196544,#196545,#196546,#196547,#196548,#196549,#196550,#196551,#196552,
#196553,#196554,#196555,#196556,#196557,#196558,#196559,#196560,#196561,
#196562,#196563,#196564,#196565,#196566,#196567,#196568,#196569,#196570,
#196571,#196572,#196573,#196574,#196575,#196576,#196577,#196578,#196579,
#196580,#196581,#196582,#196583,#196584,#196585,#196586,#196587,#196588,
#196589,#196590,#196591,#196592,#196593,#196594,#196595,#196596,#196597,
#196598,#196599,#196600,#196601,#196602,#196603,#196604,#196605,#196606,
#196607,#196608,#196609,#196610,#196611,#196612,#196613,#196614,#196615,
#196616,#196617,#196618,#196619,#196620,#196621,#196622,#196623,#196624,
#196625,#196626,#196627,#196628,#196629,#196630,#196631,#196632,#196633,
#196634,#196635,#196636,#196637,#196638,#196639,#196640,#196641,#196642,
#196643,#196644,#196645,#196646,#196647,#196648,#196649,#196650,#196651,
#196652,#196653,#196654,#196655,#196656,#196657,#196658,#196659,#196660,
#196661,#196662,#196663,#196664,#196665,#196666,#196667,#196668,#196669,
#196670,#196671,#196672,#196673,#196674,#196675,#196676,#196677,#196678,
#196679,#196680,#196681,#196682,#196683,#196684,#196685,#196686,#196687,
#196688,#196689,#196690,#196691,#196692,#196693,#196694,#196695,#196696,
#196697,#196698,#196699,#196700,#196701,#196702,#196703,#196704,#196705,
#196706,#196707,#196708,#196709,#196710,#196711,#196712,#196713,#196714,
#196715,#196716,#196717,#196718,#196719,#196720,#196721,#196722,#196723,
#196724,#196725,#196726,#196727,#196728,#196729,#196730,#196731,#196732,
#196733,#196734,#196735,#196736,#196737,#196738,#196739,#196740,#196741),
 .UNSPECIFIED.,.F.,.F.)
B_SPLINE_CURVE_WITH_KNOTS((6,1,1,1,1,1,1,1,1,1,1,1,1,1,1,1,1,1,1,1,1,1,
1,1,1,1,1,1,1,1,1,1,1,1,1,1,1,1,1,1,1,1,1,1,1,1,1,1,1,1,1,1,1,1,1,1,1,1,
1,1,1,1,1,1,1,1,1,1,1,1,1,1,1,1,1,1,1,1,1,1,1,1,1,1,1,1,1,1,1,1,1,1,1,1,
1,1,1,1,1,1,1,1,1,1,1,1,1,1,1,1,1,1,1,1,1,1,1,1,1,1,1,1,1,1,1,1,1,1,1,1,
1,1,1,1,1,1,1,1,1,1,1,1,1,1,1,1,1,1,1,1,1,1,1,1,1,1,1,1,1,1,1,1,1,1,1,1,
1,1,1,1,1,1,1,1,1,1,1,1,1,1,1,1,1,1,1,1,1,1,1,1,1,1,1,1,1,1,1,1,1,1,6),
(0.,0.005,0.01,0.015,0.02,0.025,0.03,0.035,0.04,0.045,0.05,0.055,0.06,0.065,
0.07,0.075,0.08,0.085,0.09,0.095,0.1,0.105,0.11,0.115,0.12,0.125,0.13,0.135,
0.14,0.145,0.15,0.155,0.16,0.165,0.17,0.175,0.18,0.185,0.19,0.195,0.2,0.205,
0.21,0.215,0.22,0.225,0.23,0.235,0.24,0.245,0.25,0.255,0.26,0.265,0.27,
0.275,0.28,0.285,0.29,0.295,0.3,0.305,0.31,0.315,0.32,0.325,0.33,0.335,
0.34,0.345,0.35,0.355,0.36,0.365,0.37,0.375,0.38,0.385,0.39,0.395,0.4,0.405,
0.41,0.415,0.42,0.425,0.43,0.435,0.44,0.445,0.45,0.455,0.46,0.465,0.47,
0.475,0.48,0.485,0.49,0.495,0.5,0.505,0.51,0.515,0.52,0.525,0.53,0.535,
0.54,0.545,0.55,0.555,0.56,0.565,0.57,0.575,0.58,0.585,0.59,0.595,0.6,0.605,
0.61,0.615,0.62,0.625,0.63,0.635,0.64,0.645,0.65,0.655,0.66,0.665,0.67,
0.675,0.68,0.685,0.690000000000001,0.695000000000001,0.700000000000001,
0.705000000000001,0.710000000000001,0.715000000000001,0.720000000000001,
0.725000000000001,0.730000000000001,0.735000000000001,0.740000000000001,
0.745000000000001,0.750000000000001,0.755000000000001,0.760000000000001,
0.765000000000001,0.770000000000001,0.775000000000001,0.780000000000001,
0.785000000000001,0.790000000000001,0.795000000000001,0.800000000000001,
0.805000000000001,0.810000000000001,0.815000000000001,0.820000000000001,
0.825000000000001,0.830000000000001,0.835000000000001,0.840000000000001,
0.845000000000001,0.850000000000001,0.855000000000001,0.860000000000001,
0.865000000000001,0.870000000000001,0.875000000000001,0.880000000000001,
0.885000000000001,0.890000000000001,0.895000000000001,0.900000000000001,
0.905000000000001,0.910000000000001,0.915000000000001,0.920000000000001,
0.925000000000001,0.930000000000001,0.935000000000001,0.940000000000001,
0.945000000000001,0.950000000000001,0.955000000000001,0.960000000000001,
0.965000000000001,0.970000000000001,0.975000000000001,0.980000000000001,
0.985000000000001,0.990000000000001,0.995000000000001,1.),.UNSPECIFIED.)
CURVE()
GEOMETRIC_REPRESENTATION_ITEM()
RATIONAL_B_SPLINE_CURVE((1.,1.,1.,1.,1.,1.,1.,1.,1.,1.,1.,1.,1.,1.,1.,1.,
1.,1.,1.,1.,1.,1.,1.,1.,1.,1.,1.,1.,1.,1.,1.,1.,1.,1.,1.,1.,1.,1.,1.,1.,
1.,1.,1.,1.,1.,1.,1.,1.,1.,1.,1.,1.,1.,1.,1.,1.,1.,1.,1.,1.,1.,1.,1.,1.,
1.,1.,1.,1.,1.,1.,1.,1.,1.,1.,1.,1.,1.,1.,1.,1.,1.,1.,1.,1.,1.,1.,1.,1.,
1.,1.,1.,1.,1.,1.,1.,1.,1.,1.,1.,1.,1.,1.,1.,1.,1.,1.,1.,1.,1.,1.,1.,1.,
1.,1.,1.,1.,1.,1.,1.,1.,1.,1.,1.,1.,1.,1.,1.,1.,1.,1.,1.,1.,1.,1.,1.,1.,
1.,1.,1.,1.,1.,1.,1.,1.,1.,1.,1.,1.,1.,1.,1.,1.,1.,1.,1.,1.,1.,1.,1.,1.,
1.,1.,1.,1.,1.,1.,1.,1.,1.,1.,1.,1.,1.,1.,1.,1.,1.,1.,1.,1.,1.,1.,1.,1.,
1.,1.,1.,1.,1.,1.,1.,1.,1.,1.,1.,1.,1.,1.,1.,1.,1.,1.,1.,1.,1.))
REPRESENTATION_ITEM('')
);
#757=(
BOUNDED_CURVE()
B_SPLINE_CURVE(5,(#197158,#197159,#197160,#197161,#197162,#197163,#197164,
#197165,#197166,#197167,#197168,#197169,#197170,#197171,#197172,#197173,
#197174,#197175,#197176,#197177,#197178,#197179,#197180,#197181,#197182,
#197183,#197184,#197185,#197186,#197187,#197188,#197189,#197190,#197191,
#197192,#197193,#197194,#197195,#197196,#197197,#197198,#197199,#197200,
#197201,#197202,#197203,#197204,#197205,#197206,#197207,#197208,#197209,
#197210,#197211,#197212,#197213,#197214,#197215,#197216,#197217,#197218,
#197219,#197220,#197221,#197222,#197223,#197224,#197225,#197226,#197227,
#197228,#197229,#197230,#197231,#197232,#197233,#197234,#197235,#197236,
#197237,#197238,#197239,#197240,#197241,#197242,#197243,#197244,#197245,
#197246,#197247,#197248,#197249,#197250,#197251,#197252,#197253,#197254,
#197255,#197256,#197257,#197258,#197259,#197260,#197261,#197262,#197263,
#197264,#197265,#197266,#197267,#197268,#197269,#197270,#197271,#197272,
#197273,#197274,#197275,#197276,#197277,#197278,#197279,#197280,#197281,
#197282,#197283,#197284,#197285,#197286,#197287,#197288,#197289,#197290,
#197291,#197292,#197293,#197294,#197295,#197296,#197297,#197298,#197299,
#197300,#197301,#197302,#197303,#197304,#197305,#197306,#197307,#197308,
#197309,#197310,#197311,#197312,#197313,#197314,#197315,#197316,#197317,
#197318,#197319,#197320,#197321,#197322,#197323,#197324,#197325,#197326,
#197327,#197328,#197329,#197330,#197331,#197332,#197333,#197334,#197335,
#197336,#197337,#197338,#197339,#197340,#197341,#197342,#197343,#197344,
#197345,#197346,#197347,#197348,#197349,#197350,#197351,#197352,#197353,
#197354,#197355,#197356,#197357,#197358,#197359,#197360,#197361,#197362),
 .UNSPECIFIED.,.F.,.F.)
B_SPLINE_CURVE_WITH_KNOTS((6,1,1,1,1,1,1,1,1,1,1,1,1,1,1,1,1,1,1,1,1,1,
1,1,1,1,1,1,1,1,1,1,1,1,1,1,1,1,1,1,1,1,1,1,1,1,1,1,1,1,1,1,1,1,1,1,1,1,
1,1,1,1,1,1,1,1,1,1,1,1,1,1,1,1,1,1,1,1,1,1,1,1,1,1,1,1,1,1,1,1,1,1,1,1,
1,1,1,1,1,1,1,1,1,1,1,1,1,1,1,1,1,1,1,1,1,1,1,1,1,1,1,1,1,1,1,1,1,1,1,1,
1,1,1,1,1,1,1,1,1,1,1,1,1,1,1,1,1,1,1,1,1,1,1,1,1,1,1,1,1,1,1,1,1,1,1,1,
1,1,1,1,1,1,1,1,1,1,1,1,1,1,1,1,1,1,1,1,1,1,1,1,1,1,1,1,1,1,1,1,1,1,6),
(-1.,-0.995000000000001,-0.990000000000001,-0.985000000000001,-0.980000000000001,
-0.975000000000001,-0.970000000000001,-0.965000000000001,-0.960000000000001,
-0.955000000000001,-0.950000000000001,-0.945000000000001,-0.940000000000001,
-0.935000000000001,-0.930000000000001,-0.925000000000001,-0.920000000000001,
-0.915000000000001,-0.910000000000001,-0.905000000000001,-0.900000000000001,
-0.895000000000001,-0.890000000000001,-0.885000000000001,-0.880000000000001,
-0.875000000000001,-0.870000000000001,-0.865000000000001,-0.860000000000001,
-0.855000000000001,-0.850000000000001,-0.845000000000001,-0.840000000000001,
-0.835000000000001,-0.830000000000001,-0.825000000000001,-0.820000000000001,
-0.815000000000001,-0.810000000000001,-0.805000000000001,-0.800000000000001,
-0.795000000000001,-0.790000000000001,-0.785000000000001,-0.780000000000001,
-0.775000000000001,-0.770000000000001,-0.765000000000001,-0.760000000000001,
-0.755000000000001,-0.750000000000001,-0.745000000000001,-0.740000000000001,
-0.735000000000001,-0.730000000000001,-0.725000000000001,-0.720000000000001,
-0.715000000000001,-0.710000000000001,-0.705000000000001,-0.700000000000001,
-0.695000000000001,-0.690000000000001,-0.685,-0.68,-0.675,-0.67,-0.665,
-0.66,-0.655,-0.65,-0.645,-0.64,-0.635,-0.63,-0.625,-0.62,-0.615,-0.61,
-0.605,-0.6,-0.595,-0.59,-0.585,-0.58,-0.575,-0.57,-0.565,-0.56,-0.555,
-0.55,-0.545,-0.54,-0.535,-0.53,-0.525,-0.52,-0.515,-0.51,-0.505,-0.5,-0.495,
-0.49,-0.485,-0.48,-0.475,-0.47,-0.465,-0.46,-0.455,-0.45,-0.445,-0.44,
-0.435,-0.43,-0.425,-0.42,-0.415,-0.41,-0.405,-0.4,-0.395,-0.39,-0.385,
-0.38,-0.375,-0.37,-0.365,-0.36,-0.355,-0.35,-0.345,-0.34,-0.335,-0.33,
-0.325,-0.32,-0.315,-0.31,-0.305,-0.3,-0.295,-0.29,-0.285,-0.28,-0.275,
-0.27,-0.265,-0.26,-0.255,-0.25,-0.245,-0.24,-0.235,-0.23,-0.225,-0.22,
-0.215,-0.21,-0.205,-0.2,-0.195,-0.19,-0.185,-0.18,-0.175,-0.17,-0.165,
-0.16,-0.155,-0.15,-0.145,-0.14,-0.135,-0.13,-0.125,-0.12,-0.115,-0.11,
-0.105,-0.1,-0.095,-0.09,-0.085,-0.08,-0.075,-0.07,-0.065,-0.06,-0.055,
-0.05,-0.045,-0.04,-0.035,-0.03,-0.025,-0.02,-0.015,-0.01,-0.005,0.),
 .UNSPECIFIED.)
CURVE()
GEOMETRIC_REPRESENTATION_ITEM()
RATIONAL_B_SPLINE_CURVE((1.,1.,1.,1.,1.,1.,1.,1.,1.,1.,1.,1.,1.,1.,1.,1.,
1.,1.,1.,1.,1.,1.,1.,1.,1.,1.,1.,1.,1.,1.,1.,1.,1.,1.,1.,1.,1.,1.,1.,1.,
1.,1.,1.,1.,1.,1.,1.,1.,1.,1.,1.,1.,1.,1.,1.,1.,1.,1.,1.,1.,1.,1.,1.,1.,
1.,1.,1.,1.,1.,1.,1.,1.,1.,1.,1.,1.,1.,1.,1.,1.,1.,1.,1.,1.,1.,1.,1.,1.,
1.,1.,1.,1.,1.,1.,1.,1.,1.,1.,1.,1.,1.,1.,1.,1.,1.,1.,1.,1.,1.,1.,1.,1.,
1.,1.,1.,1.,1.,1.,1.,1.,1.,1.,1.,1.,1.,1.,1.,1.,1.,1.,1.,1.,1.,1.,1.,1.,
1.,1.,1.,1.,1.,1.,1.,1.,1.,1.,1.,1.,1.,1.,1.,1.,1.,1.,1.,1.,1.,1.,1.,1.,
1.,1.,1.,1.,1.,1.,1.,1.,1.,1.,1.,1.,1.,1.,1.,1.,1.,1.,1.,1.,1.,1.,1.,1.,
1.,1.,1.,1.,1.,1.,1.,1.,1.,1.,1.,1.,1.,1.,1.,1.,1.,1.,1.,1.,1.))
REPRESENTATION_ITEM('')
);
#758=(
BOUNDED_CURVE()
B_SPLINE_CURVE(5,(#197775,#197776,#197777,#197778,#197779,#197780,#197781,
#197782,#197783,#197784,#197785,#197786,#197787,#197788,#197789,#197790,
#197791,#197792,#197793,#197794,#197795,#197796,#197797,#197798,#197799,
#197800,#197801,#197802,#197803,#197804,#197805,#197806,#197807,#197808,
#197809,#197810,#197811,#197812,#197813,#197814,#197815,#197816,#197817,
#197818,#197819,#197820,#197821,#197822,#197823,#197824,#197825,#197826,
#197827,#197828,#197829,#197830,#197831,#197832,#197833,#197834,#197835,
#197836,#197837,#197838,#197839,#197840,#197841,#197842,#197843,#197844,
#197845,#197846,#197847,#197848,#197849,#197850,#197851,#197852,#197853,
#197854,#197855,#197856,#197857,#197858,#197859,#197860,#197861,#197862,
#197863,#197864,#197865,#197866,#197867,#197868,#197869,#197870,#197871,
#197872,#197873,#197874,#197875,#197876,#197877,#197878,#197879,#197880,
#197881,#197882,#197883,#197884,#197885,#197886,#197887,#197888,#197889,
#197890,#197891,#197892,#197893,#197894,#197895,#197896,#197897,#197898,
#197899,#197900,#197901,#197902,#197903,#197904,#197905,#197906,#197907,
#197908,#197909,#197910,#197911,#197912,#197913,#197914,#197915,#197916,
#197917,#197918,#197919,#197920,#197921,#197922,#197923,#197924,#197925,
#197926,#197927,#197928,#197929,#197930,#197931,#197932,#197933,#197934,
#197935,#197936,#197937,#197938,#197939,#197940,#197941,#197942,#197943,
#197944,#197945,#197946,#197947,#197948,#197949,#197950,#197951,#197952,
#197953,#197954,#197955,#197956,#197957,#197958,#197959,#197960,#197961,
#197962,#197963,#197964,#197965,#197966,#197967,#197968,#197969,#197970,
#197971,#197972,#197973,#197974,#197975,#197976,#197977,#197978,#197979),
 .UNSPECIFIED.,.F.,.F.)
B_SPLINE_CURVE_WITH_KNOTS((6,1,1,1,1,1,1,1,1,1,1,1,1,1,1,1,1,1,1,1,1,1,
1,1,1,1,1,1,1,1,1,1,1,1,1,1,1,1,1,1,1,1,1,1,1,1,1,1,1,1,1,1,1,1,1,1,1,1,
1,1,1,1,1,1,1,1,1,1,1,1,1,1,1,1,1,1,1,1,1,1,1,1,1,1,1,1,1,1,1,1,1,1,1,1,
1,1,1,1,1,1,1,1,1,1,1,1,1,1,1,1,1,1,1,1,1,1,1,1,1,1,1,1,1,1,1,1,1,1,1,1,
1,1,1,1,1,1,1,1,1,1,1,1,1,1,1,1,1,1,1,1,1,1,1,1,1,1,1,1,1,1,1,1,1,1,1,1,
1,1,1,1,1,1,1,1,1,1,1,1,1,1,1,1,1,1,1,1,1,1,1,1,1,1,1,1,1,1,1,1,1,1,6),
(0.,0.005,0.01,0.015,0.02,0.025,0.03,0.035,0.04,0.045,0.05,0.055,0.06,0.065,
0.07,0.075,0.08,0.085,0.09,0.095,0.1,0.105,0.11,0.115,0.12,0.125,0.13,0.135,
0.14,0.145,0.15,0.155,0.16,0.165,0.17,0.175,0.18,0.185,0.19,0.195,0.2,0.205,
0.21,0.215,0.22,0.225,0.23,0.235,0.24,0.245,0.25,0.255,0.26,0.265,0.27,
0.275,0.28,0.285,0.29,0.295,0.3,0.305,0.31,0.315,0.32,0.325,0.33,0.335,
0.34,0.345,0.35,0.355,0.36,0.365,0.37,0.375,0.38,0.385,0.39,0.395,0.4,0.405,
0.41,0.415,0.42,0.425,0.43,0.435,0.44,0.445,0.45,0.455,0.46,0.465,0.47,
0.475,0.48,0.485,0.49,0.495,0.5,0.505,0.51,0.515,0.52,0.525,0.53,0.535,
0.54,0.545,0.55,0.555,0.56,0.565,0.57,0.575,0.58,0.585,0.59,0.595,0.6,0.605,
0.61,0.615,0.62,0.625,0.63,0.635,0.64,0.645,0.65,0.655,0.66,0.665,0.67,
0.675,0.68,0.685,0.690000000000001,0.695000000000001,0.700000000000001,
0.705000000000001,0.710000000000001,0.715000000000001,0.720000000000001,
0.725000000000001,0.730000000000001,0.735000000000001,0.740000000000001,
0.745000000000001,0.750000000000001,0.755000000000001,0.760000000000001,
0.765000000000001,0.770000000000001,0.775000000000001,0.780000000000001,
0.785000000000001,0.790000000000001,0.795000000000001,0.800000000000001,
0.805000000000001,0.810000000000001,0.815000000000001,0.820000000000001,
0.825000000000001,0.830000000000001,0.835000000000001,0.840000000000001,
0.845000000000001,0.850000000000001,0.855000000000001,0.860000000000001,
0.865000000000001,0.870000000000001,0.875000000000001,0.880000000000001,
0.885000000000001,0.890000000000001,0.895000000000001,0.900000000000001,
0.905000000000001,0.910000000000001,0.915000000000001,0.920000000000001,
0.925000000000001,0.930000000000001,0.935000000000001,0.940000000000001,
0.945000000000001,0.950000000000001,0.955000000000001,0.960000000000001,
0.965000000000001,0.970000000000001,0.975000000000001,0.980000000000001,
0.985000000000001,0.990000000000001,0.995000000000001,1.),.UNSPECIFIED.)
CURVE()
GEOMETRIC_REPRESENTATION_ITEM()
RATIONAL_B_SPLINE_CURVE((1.,1.,1.,1.,1.,1.,1.,1.,1.,1.,1.,1.,1.,1.,1.,1.,
1.,1.,1.,1.,1.,1.,1.,1.,1.,1.,1.,1.,1.,1.,1.,1.,1.,1.,1.,1.,1.,1.,1.,1.,
1.,1.,1.,1.,1.,1.,1.,1.,1.,1.,1.,1.,1.,1.,1.,1.,1.,1.,1.,1.,1.,1.,1.,1.,
1.,1.,1.,1.,1.,1.,1.,1.,1.,1.,1.,1.,1.,1.,1.,1.,1.,1.,1.,1.,1.,1.,1.,1.,
1.,1.,1.,1.,1.,1.,1.,1.,1.,1.,1.,1.,1.,1.,1.,1.,1.,1.,1.,1.,1.,1.,1.,1.,
1.,1.,1.,1.,1.,1.,1.,1.,1.,1.,1.,1.,1.,1.,1.,1.,1.,1.,1.,1.,1.,1.,1.,1.,
1.,1.,1.,1.,1.,1.,1.,1.,1.,1.,1.,1.,1.,1.,1.,1.,1.,1.,1.,1.,1.,1.,1.,1.,
1.,1.,1.,1.,1.,1.,1.,1.,1.,1.,1.,1.,1.,1.,1.,1.,1.,1.,1.,1.,1.,1.,1.,1.,
1.,1.,1.,1.,1.,1.,1.,1.,1.,1.,1.,1.,1.,1.,1.,1.,1.,1.,1.,1.,1.))
REPRESENTATION_ITEM('')
);
#759=(
BOUNDED_CURVE()
B_SPLINE_CURVE(5,(#198396,#198397,#198398,#198399,#198400,#198401,#198402,
#198403,#198404,#198405,#198406,#198407,#198408,#198409,#198410,#198411,
#198412,#198413,#198414,#198415,#198416,#198417,#198418,#198419,#198420,
#198421,#198422,#198423,#198424,#198425,#198426,#198427,#198428,#198429,
#198430,#198431,#198432,#198433,#198434,#198435,#198436,#198437,#198438,
#198439,#198440,#198441,#198442,#198443,#198444,#198445,#198446,#198447,
#198448,#198449,#198450,#198451,#198452,#198453,#198454,#198455,#198456,
#198457,#198458,#198459,#198460,#198461,#198462,#198463,#198464,#198465,
#198466,#198467,#198468,#198469,#198470,#198471,#198472,#198473,#198474,
#198475,#198476,#198477,#198478,#198479,#198480,#198481,#198482,#198483,
#198484,#198485,#198486,#198487,#198488,#198489,#198490,#198491,#198492,
#198493,#198494,#198495,#198496,#198497,#198498,#198499,#198500,#198501,
#198502,#198503,#198504,#198505,#198506,#198507,#198508,#198509,#198510,
#198511,#198512,#198513,#198514,#198515,#198516,#198517,#198518,#198519,
#198520,#198521,#198522,#198523,#198524,#198525,#198526,#198527,#198528,
#198529,#198530,#198531,#198532,#198533,#198534,#198535,#198536,#198537,
#198538,#198539,#198540,#198541,#198542,#198543,#198544,#198545,#198546,
#198547,#198548,#198549,#198550,#198551,#198552,#198553,#198554,#198555,
#198556,#198557,#198558,#198559,#198560,#198561,#198562,#198563,#198564,
#198565,#198566,#198567,#198568,#198569,#198570,#198571,#198572,#198573,
#198574,#198575,#198576,#198577,#198578,#198579,#198580,#198581,#198582,
#198583,#198584,#198585,#198586,#198587,#198588,#198589,#198590,#198591,
#198592,#198593,#198594,#198595,#198596,#198597,#198598,#198599,#198600),
 .UNSPECIFIED.,.F.,.F.)
B_SPLINE_CURVE_WITH_KNOTS((6,1,1,1,1,1,1,1,1,1,1,1,1,1,1,1,1,1,1,1,1,1,
1,1,1,1,1,1,1,1,1,1,1,1,1,1,1,1,1,1,1,1,1,1,1,1,1,1,1,1,1,1,1,1,1,1,1,1,
1,1,1,1,1,1,1,1,1,1,1,1,1,1,1,1,1,1,1,1,1,1,1,1,1,1,1,1,1,1,1,1,1,1,1,1,
1,1,1,1,1,1,1,1,1,1,1,1,1,1,1,1,1,1,1,1,1,1,1,1,1,1,1,1,1,1,1,1,1,1,1,1,
1,1,1,1,1,1,1,1,1,1,1,1,1,1,1,1,1,1,1,1,1,1,1,1,1,1,1,1,1,1,1,1,1,1,1,1,
1,1,1,1,1,1,1,1,1,1,1,1,1,1,1,1,1,1,1,1,1,1,1,1,1,1,1,1,1,1,1,1,1,1,6),
(-1.,-0.995000000000001,-0.990000000000001,-0.985000000000001,-0.980000000000001,
-0.975000000000001,-0.970000000000001,-0.965000000000001,-0.960000000000001,
-0.955000000000001,-0.950000000000001,-0.945000000000001,-0.940000000000001,
-0.935000000000001,-0.930000000000001,-0.925000000000001,-0.920000000000001,
-0.915000000000001,-0.910000000000001,-0.905000000000001,-0.900000000000001,
-0.895000000000001,-0.890000000000001,-0.885000000000001,-0.880000000000001,
-0.875000000000001,-0.870000000000001,-0.865000000000001,-0.860000000000001,
-0.855000000000001,-0.850000000000001,-0.845000000000001,-0.840000000000001,
-0.835000000000001,-0.830000000000001,-0.825000000000001,-0.820000000000001,
-0.815000000000001,-0.810000000000001,-0.805000000000001,-0.800000000000001,
-0.795000000000001,-0.790000000000001,-0.785000000000001,-0.780000000000001,
-0.775000000000001,-0.770000000000001,-0.765000000000001,-0.760000000000001,
-0.755000000000001,-0.750000000000001,-0.745000000000001,-0.740000000000001,
-0.735000000000001,-0.730000000000001,-0.725000000000001,-0.720000000000001,
-0.715000000000001,-0.710000000000001,-0.705000000000001,-0.700000000000001,
-0.695000000000001,-0.690000000000001,-0.685,-0.68,-0.675,-0.67,-0.665,
-0.66,-0.655,-0.65,-0.645,-0.64,-0.635,-0.63,-0.625,-0.62,-0.615,-0.61,
-0.605,-0.6,-0.595,-0.59,-0.585,-0.58,-0.575,-0.57,-0.565,-0.56,-0.555,
-0.55,-0.545,-0.54,-0.535,-0.53,-0.525,-0.52,-0.515,-0.51,-0.505,-0.5,-0.495,
-0.49,-0.485,-0.48,-0.475,-0.47,-0.465,-0.46,-0.455,-0.45,-0.445,-0.44,
-0.435,-0.43,-0.425,-0.42,-0.415,-0.41,-0.405,-0.4,-0.395,-0.39,-0.385,
-0.38,-0.375,-0.37,-0.365,-0.36,-0.355,-0.35,-0.345,-0.34,-0.335,-0.33,
-0.325,-0.32,-0.315,-0.31,-0.305,-0.3,-0.295,-0.29,-0.285,-0.28,-0.275,
-0.27,-0.265,-0.26,-0.255,-0.25,-0.245,-0.24,-0.235,-0.23,-0.225,-0.22,
-0.215,-0.21,-0.205,-0.2,-0.195,-0.19,-0.185,-0.18,-0.175,-0.17,-0.165,
-0.16,-0.155,-0.15,-0.145,-0.14,-0.135,-0.13,-0.125,-0.12,-0.115,-0.11,
-0.105,-0.1,-0.095,-0.09,-0.085,-0.08,-0.075,-0.07,-0.065,-0.06,-0.055,
-0.05,-0.045,-0.04,-0.035,-0.03,-0.025,-0.02,-0.015,-0.01,-0.005,0.),
 .UNSPECIFIED.)
CURVE()
GEOMETRIC_REPRESENTATION_ITEM()
RATIONAL_B_SPLINE_CURVE((1.,1.,1.,1.,1.,1.,1.,1.,1.,1.,1.,1.,1.,1.,1.,1.,
1.,1.,1.,1.,1.,1.,1.,1.,1.,1.,1.,1.,1.,1.,1.,1.,1.,1.,1.,1.,1.,1.,1.,1.,
1.,1.,1.,1.,1.,1.,1.,1.,1.,1.,1.,1.,1.,1.,1.,1.,1.,1.,1.,1.,1.,1.,1.,1.,
1.,1.,1.,1.,1.,1.,1.,1.,1.,1.,1.,1.,1.,1.,1.,1.,1.,1.,1.,1.,1.,1.,1.,1.,
1.,1.,1.,1.,1.,1.,1.,1.,1.,1.,1.,1.,1.,1.,1.,1.,1.,1.,1.,1.,1.,1.,1.,1.,
1.,1.,1.,1.,1.,1.,1.,1.,1.,1.,1.,1.,1.,1.,1.,1.,1.,1.,1.,1.,1.,1.,1.,1.,
1.,1.,1.,1.,1.,1.,1.,1.,1.,1.,1.,1.,1.,1.,1.,1.,1.,1.,1.,1.,1.,1.,1.,1.,
1.,1.,1.,1.,1.,1.,1.,1.,1.,1.,1.,1.,1.,1.,1.,1.,1.,1.,1.,1.,1.,1.,1.,1.,
1.,1.,1.,1.,1.,1.,1.,1.,1.,1.,1.,1.,1.,1.,1.,1.,1.,1.,1.,1.,1.))
REPRESENTATION_ITEM('')
);
#760=(
BOUNDED_CURVE()
B_SPLINE_CURVE(5,(#199013,#199014,#199015,#199016,#199017,#199018,#199019,
#199020,#199021,#199022,#199023,#199024,#199025,#199026,#199027,#199028,
#199029,#199030,#199031,#199032,#199033,#199034,#199035,#199036,#199037,
#199038,#199039,#199040,#199041,#199042,#199043,#199044,#199045,#199046,
#199047,#199048,#199049,#199050,#199051,#199052,#199053,#199054,#199055,
#199056,#199057,#199058,#199059,#199060,#199061,#199062,#199063,#199064,
#199065,#199066,#199067,#199068,#199069,#199070,#199071,#199072,#199073,
#199074,#199075,#199076,#199077,#199078,#199079,#199080,#199081,#199082,
#199083,#199084,#199085,#199086,#199087,#199088,#199089,#199090,#199091,
#199092,#199093,#199094,#199095,#199096,#199097,#199098,#199099,#199100,
#199101,#199102,#199103,#199104,#199105,#199106,#199107,#199108,#199109,
#199110,#199111,#199112,#199113,#199114,#199115,#199116,#199117,#199118,
#199119,#199120,#199121,#199122,#199123,#199124,#199125,#199126,#199127,
#199128,#199129,#199130,#199131,#199132,#199133,#199134,#199135,#199136,
#199137,#199138,#199139,#199140,#199141,#199142,#199143,#199144,#199145,
#199146,#199147,#199148,#199149,#199150,#199151,#199152,#199153,#199154,
#199155,#199156,#199157,#199158,#199159,#199160,#199161,#199162,#199163,
#199164,#199165,#199166,#199167,#199168,#199169,#199170,#199171,#199172,
#199173,#199174,#199175,#199176,#199177,#199178,#199179,#199180,#199181,
#199182,#199183,#199184,#199185,#199186,#199187,#199188,#199189,#199190,
#199191,#199192,#199193,#199194,#199195,#199196,#199197,#199198,#199199,
#199200,#199201,#199202,#199203,#199204,#199205,#199206,#199207,#199208,
#199209,#199210,#199211,#199212,#199213,#199214,#199215,#199216,#199217),
 .UNSPECIFIED.,.F.,.F.)
B_SPLINE_CURVE_WITH_KNOTS((6,1,1,1,1,1,1,1,1,1,1,1,1,1,1,1,1,1,1,1,1,1,
1,1,1,1,1,1,1,1,1,1,1,1,1,1,1,1,1,1,1,1,1,1,1,1,1,1,1,1,1,1,1,1,1,1,1,1,
1,1,1,1,1,1,1,1,1,1,1,1,1,1,1,1,1,1,1,1,1,1,1,1,1,1,1,1,1,1,1,1,1,1,1,1,
1,1,1,1,1,1,1,1,1,1,1,1,1,1,1,1,1,1,1,1,1,1,1,1,1,1,1,1,1,1,1,1,1,1,1,1,
1,1,1,1,1,1,1,1,1,1,1,1,1,1,1,1,1,1,1,1,1,1,1,1,1,1,1,1,1,1,1,1,1,1,1,1,
1,1,1,1,1,1,1,1,1,1,1,1,1,1,1,1,1,1,1,1,1,1,1,1,1,1,1,1,1,1,1,1,1,1,6),
(0.,0.005,0.01,0.015,0.02,0.025,0.03,0.035,0.04,0.045,0.05,0.055,0.06,0.065,
0.07,0.075,0.08,0.085,0.09,0.095,0.1,0.105,0.11,0.115,0.12,0.125,0.13,0.135,
0.14,0.145,0.15,0.155,0.16,0.165,0.17,0.175,0.18,0.185,0.19,0.195,0.2,0.205,
0.21,0.215,0.22,0.225,0.23,0.235,0.24,0.245,0.25,0.255,0.26,0.265,0.27,
0.275,0.28,0.285,0.29,0.295,0.3,0.305,0.31,0.315,0.32,0.325,0.33,0.335,
0.34,0.345,0.35,0.355,0.36,0.365,0.37,0.375,0.38,0.385,0.39,0.395,0.4,0.405,
0.41,0.415,0.42,0.425,0.43,0.435,0.44,0.445,0.45,0.455,0.46,0.465,0.47,
0.475,0.48,0.485,0.49,0.495,0.5,0.505,0.51,0.515,0.52,0.525,0.53,0.535,
0.54,0.545,0.55,0.555,0.56,0.565,0.57,0.575,0.58,0.585,0.59,0.595,0.6,0.605,
0.61,0.615,0.62,0.625,0.63,0.635,0.64,0.645,0.65,0.655,0.66,0.665,0.67,
0.675,0.68,0.685,0.690000000000001,0.695000000000001,0.700000000000001,
0.705000000000001,0.710000000000001,0.715000000000001,0.720000000000001,
0.725000000000001,0.730000000000001,0.735000000000001,0.740000000000001,
0.745000000000001,0.750000000000001,0.755000000000001,0.760000000000001,
0.765000000000001,0.770000000000001,0.775000000000001,0.780000000000001,
0.785000000000001,0.790000000000001,0.795000000000001,0.800000000000001,
0.805000000000001,0.810000000000001,0.815000000000001,0.820000000000001,
0.825000000000001,0.830000000000001,0.835000000000001,0.840000000000001,
0.845000000000001,0.850000000000001,0.855000000000001,0.860000000000001,
0.865000000000001,0.870000000000001,0.875000000000001,0.880000000000001,
0.885000000000001,0.890000000000001,0.895000000000001,0.900000000000001,
0.905000000000001,0.910000000000001,0.915000000000001,0.920000000000001,
0.925000000000001,0.930000000000001,0.935000000000001,0.940000000000001,
0.945000000000001,0.950000000000001,0.955000000000001,0.960000000000001,
0.965000000000001,0.970000000000001,0.975000000000001,0.980000000000001,
0.985000000000001,0.990000000000001,0.995000000000001,1.),.UNSPECIFIED.)
CURVE()
GEOMETRIC_REPRESENTATION_ITEM()
RATIONAL_B_SPLINE_CURVE((1.,1.,1.,1.,1.,1.,1.,1.,1.,1.,1.,1.,1.,1.,1.,1.,
1.,1.,1.,1.,1.,1.,1.,1.,1.,1.,1.,1.,1.,1.,1.,1.,1.,1.,1.,1.,1.,1.,1.,1.,
1.,1.,1.,1.,1.,1.,1.,1.,1.,1.,1.,1.,1.,1.,1.,1.,1.,1.,1.,1.,1.,1.,1.,1.,
1.,1.,1.,1.,1.,1.,1.,1.,1.,1.,1.,1.,1.,1.,1.,1.,1.,1.,1.,1.,1.,1.,1.,1.,
1.,1.,1.,1.,1.,1.,1.,1.,1.,1.,1.,1.,1.,1.,1.,1.,1.,1.,1.,1.,1.,1.,1.,1.,
1.,1.,1.,1.,1.,1.,1.,1.,1.,1.,1.,1.,1.,1.,1.,1.,1.,1.,1.,1.,1.,1.,1.,1.,
1.,1.,1.,1.,1.,1.,1.,1.,1.,1.,1.,1.,1.,1.,1.,1.,1.,1.,1.,1.,1.,1.,1.,1.,
1.,1.,1.,1.,1.,1.,1.,1.,1.,1.,1.,1.,1.,1.,1.,1.,1.,1.,1.,1.,1.,1.,1.,1.,
1.,1.,1.,1.,1.,1.,1.,1.,1.,1.,1.,1.,1.,1.,1.,1.,1.,1.,1.,1.,1.))
REPRESENTATION_ITEM('')
);
#761=(
BOUNDED_CURVE()
B_SPLINE_CURVE(5,(#199634,#199635,#199636,#199637,#199638,#199639,#199640,
#199641,#199642,#199643,#199644,#199645,#199646,#199647,#199648,#199649,
#199650,#199651,#199652,#199653,#199654,#199655,#199656,#199657,#199658,
#199659,#199660,#199661,#199662,#199663,#199664,#199665,#199666,#199667,
#199668,#199669,#199670,#199671,#199672,#199673,#199674,#199675,#199676,
#199677,#199678,#199679,#199680,#199681,#199682,#199683,#199684,#199685,
#199686,#199687,#199688,#199689,#199690,#199691,#199692,#199693,#199694,
#199695,#199696,#199697,#199698,#199699,#199700,#199701,#199702,#199703,
#199704,#199705,#199706,#199707,#199708,#199709,#199710,#199711,#199712,
#199713,#199714,#199715,#199716,#199717,#199718,#199719,#199720,#199721,
#199722,#199723,#199724,#199725,#199726,#199727,#199728,#199729,#199730,
#199731,#199732,#199733,#199734,#199735,#199736,#199737,#199738,#199739,
#199740,#199741,#199742,#199743,#199744,#199745,#199746,#199747,#199748,
#199749,#199750,#199751,#199752,#199753,#199754,#199755,#199756,#199757,
#199758,#199759,#199760,#199761,#199762,#199763,#199764,#199765,#199766,
#199767,#199768,#199769,#199770,#199771,#199772,#199773,#199774,#199775,
#199776,#199777,#199778,#199779,#199780,#199781,#199782,#199783,#199784,
#199785,#199786,#199787,#199788,#199789,#199790,#199791,#199792,#199793,
#199794,#199795,#199796,#199797,#199798,#199799,#199800,#199801,#199802,
#199803,#199804,#199805,#199806,#199807,#199808,#199809,#199810,#199811,
#199812,#199813,#199814,#199815,#199816,#199817,#199818,#199819,#199820,
#199821,#199822,#199823,#199824,#199825,#199826,#199827,#199828,#199829,
#199830,#199831,#199832,#199833,#199834,#199835,#199836,#199837,#199838),
 .UNSPECIFIED.,.F.,.F.)
B_SPLINE_CURVE_WITH_KNOTS((6,1,1,1,1,1,1,1,1,1,1,1,1,1,1,1,1,1,1,1,1,1,
1,1,1,1,1,1,1,1,1,1,1,1,1,1,1,1,1,1,1,1,1,1,1,1,1,1,1,1,1,1,1,1,1,1,1,1,
1,1,1,1,1,1,1,1,1,1,1,1,1,1,1,1,1,1,1,1,1,1,1,1,1,1,1,1,1,1,1,1,1,1,1,1,
1,1,1,1,1,1,1,1,1,1,1,1,1,1,1,1,1,1,1,1,1,1,1,1,1,1,1,1,1,1,1,1,1,1,1,1,
1,1,1,1,1,1,1,1,1,1,1,1,1,1,1,1,1,1,1,1,1,1,1,1,1,1,1,1,1,1,1,1,1,1,1,1,
1,1,1,1,1,1,1,1,1,1,1,1,1,1,1,1,1,1,1,1,1,1,1,1,1,1,1,1,1,1,1,1,1,1,6),
(-1.,-0.995000000000001,-0.990000000000001,-0.985000000000001,-0.980000000000001,
-0.975000000000001,-0.970000000000001,-0.965000000000001,-0.960000000000001,
-0.955000000000001,-0.950000000000001,-0.945000000000001,-0.940000000000001,
-0.935000000000001,-0.930000000000001,-0.925000000000001,-0.920000000000001,
-0.915000000000001,-0.910000000000001,-0.905000000000001,-0.900000000000001,
-0.895000000000001,-0.890000000000001,-0.885000000000001,-0.880000000000001,
-0.875000000000001,-0.870000000000001,-0.865000000000001,-0.860000000000001,
-0.855000000000001,-0.850000000000001,-0.845000000000001,-0.840000000000001,
-0.835000000000001,-0.830000000000001,-0.825000000000001,-0.820000000000001,
-0.815000000000001,-0.810000000000001,-0.805000000000001,-0.800000000000001,
-0.795000000000001,-0.790000000000001,-0.785000000000001,-0.780000000000001,
-0.775000000000001,-0.770000000000001,-0.765000000000001,-0.760000000000001,
-0.755000000000001,-0.750000000000001,-0.745000000000001,-0.740000000000001,
-0.735000000000001,-0.730000000000001,-0.725000000000001,-0.720000000000001,
-0.715000000000001,-0.710000000000001,-0.705000000000001,-0.700000000000001,
-0.695000000000001,-0.690000000000001,-0.685,-0.68,-0.675,-0.67,-0.665,
-0.66,-0.655,-0.65,-0.645,-0.64,-0.635,-0.63,-0.625,-0.62,-0.615,-0.61,
-0.605,-0.6,-0.595,-0.59,-0.585,-0.58,-0.575,-0.57,-0.565,-0.56,-0.555,
-0.55,-0.545,-0.54,-0.535,-0.53,-0.525,-0.52,-0.515,-0.51,-0.505,-0.5,-0.495,
-0.49,-0.485,-0.48,-0.475,-0.47,-0.465,-0.46,-0.455,-0.45,-0.445,-0.44,
-0.435,-0.43,-0.425,-0.42,-0.415,-0.41,-0.405,-0.4,-0.395,-0.39,-0.385,
-0.38,-0.375,-0.37,-0.365,-0.36,-0.355,-0.35,-0.345,-0.34,-0.335,-0.33,
-0.325,-0.32,-0.315,-0.31,-0.305,-0.3,-0.295,-0.29,-0.285,-0.28,-0.275,
-0.27,-0.265,-0.26,-0.255,-0.25,-0.245,-0.24,-0.235,-0.23,-0.225,-0.22,
-0.215,-0.21,-0.205,-0.2,-0.195,-0.19,-0.185,-0.18,-0.175,-0.17,-0.165,
-0.16,-0.155,-0.15,-0.145,-0.14,-0.135,-0.13,-0.125,-0.12,-0.115,-0.11,
-0.105,-0.1,-0.095,-0.09,-0.085,-0.08,-0.075,-0.07,-0.065,-0.06,-0.055,
-0.05,-0.045,-0.04,-0.035,-0.03,-0.025,-0.02,-0.015,-0.01,-0.005,0.),
 .UNSPECIFIED.)
CURVE()
GEOMETRIC_REPRESENTATION_ITEM()
RATIONAL_B_SPLINE_CURVE((1.,1.,1.,1.,1.,1.,1.,1.,1.,1.,1.,1.,1.,1.,1.,1.,
1.,1.,1.,1.,1.,1.,1.,1.,1.,1.,1.,1.,1.,1.,1.,1.,1.,1.,1.,1.,1.,1.,1.,1.,
1.,1.,1.,1.,1.,1.,1.,1.,1.,1.,1.,1.,1.,1.,1.,1.,1.,1.,1.,1.,1.,1.,1.,1.,
1.,1.,1.,1.,1.,1.,1.,1.,1.,1.,1.,1.,1.,1.,1.,1.,1.,1.,1.,1.,1.,1.,1.,1.,
1.,1.,1.,1.,1.,1.,1.,1.,1.,1.,1.,1.,1.,1.,1.,1.,1.,1.,1.,1.,1.,1.,1.,1.,
1.,1.,1.,1.,1.,1.,1.,1.,1.,1.,1.,1.,1.,1.,1.,1.,1.,1.,1.,1.,1.,1.,1.,1.,
1.,1.,1.,1.,1.,1.,1.,1.,1.,1.,1.,1.,1.,1.,1.,1.,1.,1.,1.,1.,1.,1.,1.,1.,
1.,1.,1.,1.,1.,1.,1.,1.,1.,1.,1.,1.,1.,1.,1.,1.,1.,1.,1.,1.,1.,1.,1.,1.,
1.,1.,1.,1.,1.,1.,1.,1.,1.,1.,1.,1.,1.,1.,1.,1.,1.,1.,1.,1.,1.))
REPRESENTATION_ITEM('')
);
#762=(
BOUNDED_CURVE()
B_SPLINE_CURVE(5,(#200251,#200252,#200253,#200254,#200255,#200256,#200257,
#200258,#200259,#200260,#200261,#200262,#200263,#200264,#200265,#200266,
#200267,#200268,#200269,#200270,#200271,#200272,#200273,#200274,#200275,
#200276,#200277,#200278,#200279,#200280,#200281,#200282,#200283,#200284,
#200285,#200286,#200287,#200288,#200289,#200290,#200291,#200292,#200293,
#200294,#200295,#200296,#200297,#200298,#200299,#200300,#200301,#200302,
#200303,#200304,#200305,#200306,#200307,#200308,#200309,#200310,#200311,
#200312,#200313,#200314,#200315,#200316,#200317,#200318,#200319,#200320,
#200321,#200322,#200323,#200324,#200325,#200326,#200327,#200328,#200329,
#200330,#200331,#200332,#200333,#200334,#200335,#200336,#200337,#200338,
#200339,#200340,#200341,#200342,#200343,#200344,#200345,#200346,#200347,
#200348,#200349,#200350,#200351,#200352,#200353,#200354,#200355,#200356,
#200357,#200358,#200359,#200360,#200361,#200362,#200363,#200364,#200365,
#200366,#200367,#200368,#200369,#200370,#200371,#200372,#200373,#200374,
#200375,#200376,#200377,#200378,#200379,#200380,#200381,#200382,#200383,
#200384,#200385,#200386,#200387,#200388,#200389,#200390,#200391,#200392,
#200393,#200394,#200395,#200396,#200397,#200398,#200399,#200400,#200401,
#200402,#200403,#200404,#200405,#200406,#200407,#200408,#200409,#200410,
#200411,#200412,#200413,#200414,#200415,#200416,#200417,#200418,#200419,
#200420,#200421,#200422,#200423,#200424,#200425,#200426,#200427,#200428,
#200429,#200430,#200431,#200432,#200433,#200434,#200435,#200436,#200437,
#200438,#200439,#200440,#200441,#200442,#200443,#200444,#200445,#200446,
#200447,#200448,#200449,#200450,#200451,#200452,#200453,#200454,#200455),
 .UNSPECIFIED.,.F.,.F.)
B_SPLINE_CURVE_WITH_KNOTS((6,1,1,1,1,1,1,1,1,1,1,1,1,1,1,1,1,1,1,1,1,1,
1,1,1,1,1,1,1,1,1,1,1,1,1,1,1,1,1,1,1,1,1,1,1,1,1,1,1,1,1,1,1,1,1,1,1,1,
1,1,1,1,1,1,1,1,1,1,1,1,1,1,1,1,1,1,1,1,1,1,1,1,1,1,1,1,1,1,1,1,1,1,1,1,
1,1,1,1,1,1,1,1,1,1,1,1,1,1,1,1,1,1,1,1,1,1,1,1,1,1,1,1,1,1,1,1,1,1,1,1,
1,1,1,1,1,1,1,1,1,1,1,1,1,1,1,1,1,1,1,1,1,1,1,1,1,1,1,1,1,1,1,1,1,1,1,1,
1,1,1,1,1,1,1,1,1,1,1,1,1,1,1,1,1,1,1,1,1,1,1,1,1,1,1,1,1,1,1,1,1,1,6),
(0.,0.005,0.01,0.015,0.02,0.025,0.03,0.035,0.04,0.045,0.05,0.055,0.06,0.065,
0.07,0.075,0.08,0.085,0.09,0.095,0.1,0.105,0.11,0.115,0.12,0.125,0.13,0.135,
0.14,0.145,0.15,0.155,0.16,0.165,0.17,0.175,0.18,0.185,0.19,0.195,0.2,0.205,
0.21,0.215,0.22,0.225,0.23,0.235,0.24,0.245,0.25,0.255,0.26,0.265,0.27,
0.275,0.28,0.285,0.29,0.295,0.3,0.305,0.31,0.315,0.32,0.325,0.33,0.335,
0.34,0.345,0.35,0.355,0.36,0.365,0.37,0.375,0.38,0.385,0.39,0.395,0.4,0.405,
0.41,0.415,0.42,0.425,0.43,0.435,0.44,0.445,0.45,0.455,0.46,0.465,0.47,
0.475,0.48,0.485,0.49,0.495,0.5,0.505,0.51,0.515,0.52,0.525,0.53,0.535,
0.54,0.545,0.55,0.555,0.56,0.565,0.57,0.575,0.58,0.585,0.59,0.595,0.6,0.605,
0.61,0.615,0.62,0.625,0.63,0.635,0.64,0.645,0.65,0.655,0.66,0.665,0.67,
0.675,0.68,0.685,0.690000000000001,0.695000000000001,0.700000000000001,
0.705000000000001,0.710000000000001,0.715000000000001,0.720000000000001,
0.725000000000001,0.730000000000001,0.735000000000001,0.740000000000001,
0.745000000000001,0.750000000000001,0.755000000000001,0.760000000000001,
0.765000000000001,0.770000000000001,0.775000000000001,0.780000000000001,
0.785000000000001,0.790000000000001,0.795000000000001,0.800000000000001,
0.805000000000001,0.810000000000001,0.815000000000001,0.820000000000001,
0.825000000000001,0.830000000000001,0.835000000000001,0.840000000000001,
0.845000000000001,0.850000000000001,0.855000000000001,0.860000000000001,
0.865000000000001,0.870000000000001,0.875000000000001,0.880000000000001,
0.885000000000001,0.890000000000001,0.895000000000001,0.900000000000001,
0.905000000000001,0.910000000000001,0.915000000000001,0.920000000000001,
0.925000000000001,0.930000000000001,0.935000000000001,0.940000000000001,
0.945000000000001,0.950000000000001,0.955000000000001,0.960000000000001,
0.965000000000001,0.970000000000001,0.975000000000001,0.980000000000001,
0.985000000000001,0.990000000000001,0.995000000000001,1.),.UNSPECIFIED.)
CURVE()
GEOMETRIC_REPRESENTATION_ITEM()
RATIONAL_B_SPLINE_CURVE((1.,1.,1.,1.,1.,1.,1.,1.,1.,1.,1.,1.,1.,1.,1.,1.,
1.,1.,1.,1.,1.,1.,1.,1.,1.,1.,1.,1.,1.,1.,1.,1.,1.,1.,1.,1.,1.,1.,1.,1.,
1.,1.,1.,1.,1.,1.,1.,1.,1.,1.,1.,1.,1.,1.,1.,1.,1.,1.,1.,1.,1.,1.,1.,1.,
1.,1.,1.,1.,1.,1.,1.,1.,1.,1.,1.,1.,1.,1.,1.,1.,1.,1.,1.,1.,1.,1.,1.,1.,
1.,1.,1.,1.,1.,1.,1.,1.,1.,1.,1.,1.,1.,1.,1.,1.,1.,1.,1.,1.,1.,1.,1.,1.,
1.,1.,1.,1.,1.,1.,1.,1.,1.,1.,1.,1.,1.,1.,1.,1.,1.,1.,1.,1.,1.,1.,1.,1.,
1.,1.,1.,1.,1.,1.,1.,1.,1.,1.,1.,1.,1.,1.,1.,1.,1.,1.,1.,1.,1.,1.,1.,1.,
1.,1.,1.,1.,1.,1.,1.,1.,1.,1.,1.,1.,1.,1.,1.,1.,1.,1.,1.,1.,1.,1.,1.,1.,
1.,1.,1.,1.,1.,1.,1.,1.,1.,1.,1.,1.,1.,1.,1.,1.,1.,1.,1.,1.,1.))
REPRESENTATION_ITEM('')
);
#763=(
BOUNDED_CURVE()
B_SPLINE_CURVE(5,(#200872,#200873,#200874,#200875,#200876,#200877,#200878,
#200879,#200880,#200881,#200882,#200883,#200884,#200885,#200886,#200887,
#200888,#200889,#200890,#200891,#200892,#200893,#200894,#200895,#200896,
#200897,#200898,#200899,#200900,#200901,#200902,#200903,#200904,#200905,
#200906,#200907,#200908,#200909,#200910,#200911,#200912,#200913,#200914,
#200915,#200916,#200917,#200918,#200919,#200920,#200921,#200922,#200923,
#200924,#200925,#200926,#200927,#200928,#200929,#200930,#200931,#200932,
#200933,#200934,#200935,#200936,#200937,#200938,#200939,#200940,#200941,
#200942,#200943,#200944,#200945,#200946,#200947,#200948,#200949,#200950,
#200951,#200952,#200953,#200954,#200955,#200956,#200957,#200958,#200959,
#200960,#200961,#200962,#200963,#200964,#200965,#200966,#200967,#200968,
#200969,#200970,#200971,#200972,#200973,#200974,#200975,#200976,#200977,
#200978,#200979,#200980,#200981,#200982,#200983,#200984,#200985,#200986,
#200987,#200988,#200989,#200990,#200991,#200992,#200993,#200994,#200995,
#200996,#200997,#200998,#200999,#201000,#201001,#201002,#201003,#201004,
#201005,#201006,#201007,#201008,#201009,#201010,#201011,#201012,#201013,
#201014,#201015,#201016,#201017,#201018,#201019,#201020,#201021,#201022,
#201023,#201024,#201025,#201026,#201027,#201028,#201029,#201030,#201031,
#201032,#201033,#201034,#201035,#201036,#201037,#201038,#201039,#201040,
#201041,#201042,#201043,#201044,#201045,#201046,#201047,#201048,#201049,
#201050,#201051,#201052,#201053,#201054,#201055,#201056,#201057,#201058,
#201059,#201060,#201061,#201062,#201063,#201064,#201065,#201066,#201067,
#201068,#201069,#201070,#201071,#201072,#201073,#201074,#201075,#201076),
 .UNSPECIFIED.,.F.,.F.)
B_SPLINE_CURVE_WITH_KNOTS((6,1,1,1,1,1,1,1,1,1,1,1,1,1,1,1,1,1,1,1,1,1,
1,1,1,1,1,1,1,1,1,1,1,1,1,1,1,1,1,1,1,1,1,1,1,1,1,1,1,1,1,1,1,1,1,1,1,1,
1,1,1,1,1,1,1,1,1,1,1,1,1,1,1,1,1,1,1,1,1,1,1,1,1,1,1,1,1,1,1,1,1,1,1,1,
1,1,1,1,1,1,1,1,1,1,1,1,1,1,1,1,1,1,1,1,1,1,1,1,1,1,1,1,1,1,1,1,1,1,1,1,
1,1,1,1,1,1,1,1,1,1,1,1,1,1,1,1,1,1,1,1,1,1,1,1,1,1,1,1,1,1,1,1,1,1,1,1,
1,1,1,1,1,1,1,1,1,1,1,1,1,1,1,1,1,1,1,1,1,1,1,1,1,1,1,1,1,1,1,1,1,1,6),
(-1.,-0.995000000000001,-0.990000000000001,-0.985000000000001,-0.980000000000001,
-0.975000000000001,-0.970000000000001,-0.965000000000001,-0.960000000000001,
-0.955000000000001,-0.950000000000001,-0.945000000000001,-0.940000000000001,
-0.935000000000001,-0.930000000000001,-0.925000000000001,-0.920000000000001,
-0.915000000000001,-0.910000000000001,-0.905000000000001,-0.900000000000001,
-0.895000000000001,-0.890000000000001,-0.885000000000001,-0.880000000000001,
-0.875000000000001,-0.870000000000001,-0.865000000000001,-0.860000000000001,
-0.855000000000001,-0.850000000000001,-0.845000000000001,-0.840000000000001,
-0.835000000000001,-0.830000000000001,-0.825000000000001,-0.820000000000001,
-0.815000000000001,-0.810000000000001,-0.805000000000001,-0.800000000000001,
-0.795000000000001,-0.790000000000001,-0.785000000000001,-0.780000000000001,
-0.775000000000001,-0.770000000000001,-0.765000000000001,-0.760000000000001,
-0.755000000000001,-0.750000000000001,-0.745000000000001,-0.740000000000001,
-0.735000000000001,-0.730000000000001,-0.725000000000001,-0.720000000000001,
-0.715000000000001,-0.710000000000001,-0.705000000000001,-0.700000000000001,
-0.695000000000001,-0.690000000000001,-0.685,-0.68,-0.675,-0.67,-0.665,
-0.66,-0.655,-0.65,-0.645,-0.64,-0.635,-0.63,-0.625,-0.62,-0.615,-0.61,
-0.605,-0.6,-0.595,-0.59,-0.585,-0.58,-0.575,-0.57,-0.565,-0.56,-0.555,
-0.55,-0.545,-0.54,-0.535,-0.53,-0.525,-0.52,-0.515,-0.51,-0.505,-0.5,-0.495,
-0.49,-0.485,-0.48,-0.475,-0.47,-0.465,-0.46,-0.455,-0.45,-0.445,-0.44,
-0.435,-0.43,-0.425,-0.42,-0.415,-0.41,-0.405,-0.4,-0.395,-0.39,-0.385,
-0.38,-0.375,-0.37,-0.365,-0.36,-0.355,-0.35,-0.345,-0.34,-0.335,-0.33,
-0.325,-0.32,-0.315,-0.31,-0.305,-0.3,-0.295,-0.29,-0.285,-0.28,-0.275,
-0.27,-0.265,-0.26,-0.255,-0.25,-0.245,-0.24,-0.235,-0.23,-0.225,-0.22,
-0.215,-0.21,-0.205,-0.2,-0.195,-0.19,-0.185,-0.18,-0.175,-0.17,-0.165,
-0.16,-0.155,-0.15,-0.145,-0.14,-0.135,-0.13,-0.125,-0.12,-0.115,-0.11,
-0.105,-0.1,-0.095,-0.09,-0.085,-0.08,-0.075,-0.07,-0.065,-0.06,-0.055,
-0.05,-0.045,-0.04,-0.035,-0.03,-0.025,-0.02,-0.015,-0.01,-0.005,0.),
 .UNSPECIFIED.)
CURVE()
GEOMETRIC_REPRESENTATION_ITEM()
RATIONAL_B_SPLINE_CURVE((1.,1.,1.,1.,1.,1.,1.,1.,1.,1.,1.,1.,1.,1.,1.,1.,
1.,1.,1.,1.,1.,1.,1.,1.,1.,1.,1.,1.,1.,1.,1.,1.,1.,1.,1.,1.,1.,1.,1.,1.,
1.,1.,1.,1.,1.,1.,1.,1.,1.,1.,1.,1.,1.,1.,1.,1.,1.,1.,1.,1.,1.,1.,1.,1.,
1.,1.,1.,1.,1.,1.,1.,1.,1.,1.,1.,1.,1.,1.,1.,1.,1.,1.,1.,1.,1.,1.,1.,1.,
1.,1.,1.,1.,1.,1.,1.,1.,1.,1.,1.,1.,1.,1.,1.,1.,1.,1.,1.,1.,1.,1.,1.,1.,
1.,1.,1.,1.,1.,1.,1.,1.,1.,1.,1.,1.,1.,1.,1.,1.,1.,1.,1.,1.,1.,1.,1.,1.,
1.,1.,1.,1.,1.,1.,1.,1.,1.,1.,1.,1.,1.,1.,1.,1.,1.,1.,1.,1.,1.,1.,1.,1.,
1.,1.,1.,1.,1.,1.,1.,1.,1.,1.,1.,1.,1.,1.,1.,1.,1.,1.,1.,1.,1.,1.,1.,1.,
1.,1.,1.,1.,1.,1.,1.,1.,1.,1.,1.,1.,1.,1.,1.,1.,1.,1.,1.,1.,1.))
REPRESENTATION_ITEM('')
);
#764=(
BOUNDED_CURVE()
B_SPLINE_CURVE(5,(#201489,#201490,#201491,#201492,#201493,#201494,#201495,
#201496,#201497,#201498,#201499,#201500,#201501,#201502,#201503,#201504,
#201505,#201506,#201507,#201508,#201509,#201510,#201511,#201512,#201513,
#201514,#201515,#201516,#201517,#201518,#201519,#201520,#201521,#201522,
#201523,#201524,#201525,#201526,#201527,#201528,#201529,#201530,#201531,
#201532,#201533,#201534,#201535,#201536,#201537,#201538,#201539,#201540,
#201541,#201542,#201543,#201544,#201545,#201546,#201547,#201548,#201549,
#201550,#201551,#201552,#201553,#201554,#201555,#201556,#201557,#201558,
#201559,#201560,#201561,#201562,#201563,#201564,#201565,#201566,#201567,
#201568,#201569,#201570,#201571,#201572,#201573,#201574,#201575,#201576,
#201577,#201578,#201579,#201580,#201581,#201582,#201583,#201584,#201585,
#201586,#201587,#201588,#201589,#201590,#201591,#201592,#201593,#201594,
#201595,#201596,#201597,#201598,#201599,#201600,#201601,#201602,#201603,
#201604,#201605,#201606,#201607,#201608,#201609,#201610,#201611,#201612,
#201613,#201614,#201615,#201616,#201617,#201618,#201619,#201620,#201621,
#201622,#201623,#201624,#201625,#201626,#201627,#201628,#201629,#201630,
#201631,#201632,#201633,#201634,#201635,#201636,#201637,#201638,#201639,
#201640,#201641,#201642,#201643,#201644,#201645,#201646,#201647,#201648,
#201649,#201650,#201651,#201652,#201653,#201654,#201655,#201656,#201657,
#201658,#201659,#201660,#201661,#201662,#201663,#201664,#201665,#201666,
#201667,#201668,#201669,#201670,#201671,#201672,#201673,#201674,#201675,
#201676,#201677,#201678,#201679,#201680,#201681,#201682,#201683,#201684,
#201685,#201686,#201687,#201688,#201689,#201690,#201691,#201692,#201693),
 .UNSPECIFIED.,.F.,.F.)
B_SPLINE_CURVE_WITH_KNOTS((6,1,1,1,1,1,1,1,1,1,1,1,1,1,1,1,1,1,1,1,1,1,
1,1,1,1,1,1,1,1,1,1,1,1,1,1,1,1,1,1,1,1,1,1,1,1,1,1,1,1,1,1,1,1,1,1,1,1,
1,1,1,1,1,1,1,1,1,1,1,1,1,1,1,1,1,1,1,1,1,1,1,1,1,1,1,1,1,1,1,1,1,1,1,1,
1,1,1,1,1,1,1,1,1,1,1,1,1,1,1,1,1,1,1,1,1,1,1,1,1,1,1,1,1,1,1,1,1,1,1,1,
1,1,1,1,1,1,1,1,1,1,1,1,1,1,1,1,1,1,1,1,1,1,1,1,1,1,1,1,1,1,1,1,1,1,1,1,
1,1,1,1,1,1,1,1,1,1,1,1,1,1,1,1,1,1,1,1,1,1,1,1,1,1,1,1,1,1,1,1,1,1,6),
(0.,0.005,0.01,0.015,0.02,0.025,0.03,0.035,0.04,0.045,0.05,0.055,0.06,0.065,
0.07,0.075,0.08,0.085,0.09,0.095,0.1,0.105,0.11,0.115,0.12,0.125,0.13,0.135,
0.14,0.145,0.15,0.155,0.16,0.165,0.17,0.175,0.18,0.185,0.19,0.195,0.2,0.205,
0.21,0.215,0.22,0.225,0.23,0.235,0.24,0.245,0.25,0.255,0.26,0.265,0.27,
0.275,0.28,0.285,0.29,0.295,0.3,0.305,0.31,0.315,0.32,0.325,0.33,0.335,
0.34,0.345,0.35,0.355,0.36,0.365,0.37,0.375,0.38,0.385,0.39,0.395,0.4,0.405,
0.41,0.415,0.42,0.425,0.43,0.435,0.44,0.445,0.45,0.455,0.46,0.465,0.47,
0.475,0.48,0.485,0.49,0.495,0.5,0.505,0.51,0.515,0.52,0.525,0.53,0.535,
0.54,0.545,0.55,0.555,0.56,0.565,0.57,0.575,0.58,0.585,0.59,0.595,0.6,0.605,
0.61,0.615,0.62,0.625,0.63,0.635,0.64,0.645,0.65,0.655,0.66,0.665,0.67,
0.675,0.68,0.685,0.690000000000001,0.695000000000001,0.700000000000001,
0.705000000000001,0.710000000000001,0.715000000000001,0.720000000000001,
0.725000000000001,0.730000000000001,0.735000000000001,0.740000000000001,
0.745000000000001,0.750000000000001,0.755000000000001,0.760000000000001,
0.765000000000001,0.770000000000001,0.775000000000001,0.780000000000001,
0.785000000000001,0.790000000000001,0.795000000000001,0.800000000000001,
0.805000000000001,0.810000000000001,0.815000000000001,0.820000000000001,
0.825000000000001,0.830000000000001,0.835000000000001,0.840000000000001,
0.845000000000001,0.850000000000001,0.855000000000001,0.860000000000001,
0.865000000000001,0.870000000000001,0.875000000000001,0.880000000000001,
0.885000000000001,0.890000000000001,0.895000000000001,0.900000000000001,
0.905000000000001,0.910000000000001,0.915000000000001,0.920000000000001,
0.925000000000001,0.930000000000001,0.935000000000001,0.940000000000001,
0.945000000000001,0.950000000000001,0.955000000000001,0.960000000000001,
0.965000000000001,0.970000000000001,0.975000000000001,0.980000000000001,
0.985000000000001,0.990000000000001,0.995000000000001,1.),.UNSPECIFIED.)
CURVE()
GEOMETRIC_REPRESENTATION_ITEM()
RATIONAL_B_SPLINE_CURVE((1.,1.,1.,1.,1.,1.,1.,1.,1.,1.,1.,1.,1.,1.,1.,1.,
1.,1.,1.,1.,1.,1.,1.,1.,1.,1.,1.,1.,1.,1.,1.,1.,1.,1.,1.,1.,1.,1.,1.,1.,
1.,1.,1.,1.,1.,1.,1.,1.,1.,1.,1.,1.,1.,1.,1.,1.,1.,1.,1.,1.,1.,1.,1.,1.,
1.,1.,1.,1.,1.,1.,1.,1.,1.,1.,1.,1.,1.,1.,1.,1.,1.,1.,1.,1.,1.,1.,1.,1.,
1.,1.,1.,1.,1.,1.,1.,1.,1.,1.,1.,1.,1.,1.,1.,1.,1.,1.,1.,1.,1.,1.,1.,1.,
1.,1.,1.,1.,1.,1.,1.,1.,1.,1.,1.,1.,1.,1.,1.,1.,1.,1.,1.,1.,1.,1.,1.,1.,
1.,1.,1.,1.,1.,1.,1.,1.,1.,1.,1.,1.,1.,1.,1.,1.,1.,1.,1.,1.,1.,1.,1.,1.,
1.,1.,1.,1.,1.,1.,1.,1.,1.,1.,1.,1.,1.,1.,1.,1.,1.,1.,1.,1.,1.,1.,1.,1.,
1.,1.,1.,1.,1.,1.,1.,1.,1.,1.,1.,1.,1.,1.,1.,1.,1.,1.,1.,1.,1.))
REPRESENTATION_ITEM('')
);
#765=(
BOUNDED_CURVE()
B_SPLINE_CURVE(5,(#202110,#202111,#202112,#202113,#202114,#202115,#202116,
#202117,#202118,#202119,#202120,#202121,#202122,#202123,#202124,#202125,
#202126,#202127,#202128,#202129,#202130,#202131,#202132,#202133,#202134,
#202135,#202136,#202137,#202138,#202139,#202140,#202141,#202142,#202143,
#202144,#202145,#202146,#202147,#202148,#202149,#202150,#202151,#202152,
#202153,#202154,#202155,#202156,#202157,#202158,#202159,#202160,#202161,
#202162,#202163,#202164,#202165,#202166,#202167,#202168,#202169,#202170,
#202171,#202172,#202173,#202174,#202175,#202176,#202177,#202178,#202179,
#202180,#202181,#202182,#202183,#202184,#202185,#202186,#202187,#202188,
#202189,#202190,#202191,#202192,#202193,#202194,#202195,#202196,#202197,
#202198,#202199,#202200,#202201,#202202,#202203,#202204,#202205,#202206,
#202207,#202208,#202209,#202210,#202211,#202212,#202213,#202214,#202215,
#202216,#202217,#202218,#202219,#202220,#202221,#202222,#202223,#202224,
#202225,#202226,#202227,#202228,#202229,#202230,#202231,#202232,#202233,
#202234,#202235,#202236,#202237,#202238,#202239,#202240,#202241,#202242,
#202243,#202244,#202245,#202246,#202247,#202248,#202249,#202250,#202251,
#202252,#202253,#202254,#202255,#202256,#202257,#202258,#202259,#202260,
#202261,#202262,#202263,#202264,#202265,#202266,#202267,#202268,#202269,
#202270,#202271,#202272,#202273,#202274,#202275,#202276,#202277,#202278,
#202279,#202280,#202281,#202282,#202283,#202284,#202285,#202286,#202287,
#202288,#202289,#202290,#202291,#202292,#202293,#202294,#202295,#202296,
#202297,#202298,#202299,#202300,#202301,#202302,#202303,#202304,#202305,
#202306,#202307,#202308,#202309,#202310,#202311,#202312,#202313,#202314),
 .UNSPECIFIED.,.F.,.F.)
B_SPLINE_CURVE_WITH_KNOTS((6,1,1,1,1,1,1,1,1,1,1,1,1,1,1,1,1,1,1,1,1,1,
1,1,1,1,1,1,1,1,1,1,1,1,1,1,1,1,1,1,1,1,1,1,1,1,1,1,1,1,1,1,1,1,1,1,1,1,
1,1,1,1,1,1,1,1,1,1,1,1,1,1,1,1,1,1,1,1,1,1,1,1,1,1,1,1,1,1,1,1,1,1,1,1,
1,1,1,1,1,1,1,1,1,1,1,1,1,1,1,1,1,1,1,1,1,1,1,1,1,1,1,1,1,1,1,1,1,1,1,1,
1,1,1,1,1,1,1,1,1,1,1,1,1,1,1,1,1,1,1,1,1,1,1,1,1,1,1,1,1,1,1,1,1,1,1,1,
1,1,1,1,1,1,1,1,1,1,1,1,1,1,1,1,1,1,1,1,1,1,1,1,1,1,1,1,1,1,1,1,1,1,6),
(-1.,-0.995000000000001,-0.990000000000001,-0.985000000000001,-0.980000000000001,
-0.975000000000001,-0.970000000000001,-0.965000000000001,-0.960000000000001,
-0.955000000000001,-0.950000000000001,-0.945000000000001,-0.940000000000001,
-0.935000000000001,-0.930000000000001,-0.925000000000001,-0.920000000000001,
-0.915000000000001,-0.910000000000001,-0.905000000000001,-0.900000000000001,
-0.895000000000001,-0.890000000000001,-0.885000000000001,-0.880000000000001,
-0.875000000000001,-0.870000000000001,-0.865000000000001,-0.860000000000001,
-0.855000000000001,-0.850000000000001,-0.845000000000001,-0.840000000000001,
-0.835000000000001,-0.830000000000001,-0.825000000000001,-0.820000000000001,
-0.815000000000001,-0.810000000000001,-0.805000000000001,-0.800000000000001,
-0.795000000000001,-0.790000000000001,-0.785000000000001,-0.780000000000001,
-0.775000000000001,-0.770000000000001,-0.765000000000001,-0.760000000000001,
-0.755000000000001,-0.750000000000001,-0.745000000000001,-0.740000000000001,
-0.735000000000001,-0.730000000000001,-0.725000000000001,-0.720000000000001,
-0.715000000000001,-0.710000000000001,-0.705000000000001,-0.700000000000001,
-0.695000000000001,-0.690000000000001,-0.685,-0.68,-0.675,-0.67,-0.665,
-0.66,-0.655,-0.65,-0.645,-0.64,-0.635,-0.63,-0.625,-0.62,-0.615,-0.61,
-0.605,-0.6,-0.595,-0.59,-0.585,-0.58,-0.575,-0.57,-0.565,-0.56,-0.555,
-0.55,-0.545,-0.54,-0.535,-0.53,-0.525,-0.52,-0.515,-0.51,-0.505,-0.5,-0.495,
-0.49,-0.485,-0.48,-0.475,-0.47,-0.465,-0.46,-0.455,-0.45,-0.445,-0.44,
-0.435,-0.43,-0.425,-0.42,-0.415,-0.41,-0.405,-0.4,-0.395,-0.39,-0.385,
-0.38,-0.375,-0.37,-0.365,-0.36,-0.355,-0.35,-0.345,-0.34,-0.335,-0.33,
-0.325,-0.32,-0.315,-0.31,-0.305,-0.3,-0.295,-0.29,-0.285,-0.28,-0.275,
-0.27,-0.265,-0.26,-0.255,-0.25,-0.245,-0.24,-0.235,-0.23,-0.225,-0.22,
-0.215,-0.21,-0.205,-0.2,-0.195,-0.19,-0.185,-0.18,-0.175,-0.17,-0.165,
-0.16,-0.155,-0.15,-0.145,-0.14,-0.135,-0.13,-0.125,-0.12,-0.115,-0.11,
-0.105,-0.1,-0.095,-0.09,-0.085,-0.08,-0.075,-0.07,-0.065,-0.06,-0.055,
-0.05,-0.045,-0.04,-0.035,-0.03,-0.025,-0.02,-0.015,-0.01,-0.005,0.),
 .UNSPECIFIED.)
CURVE()
GEOMETRIC_REPRESENTATION_ITEM()
RATIONAL_B_SPLINE_CURVE((1.,1.,1.,1.,1.,1.,1.,1.,1.,1.,1.,1.,1.,1.,1.,1.,
1.,1.,1.,1.,1.,1.,1.,1.,1.,1.,1.,1.,1.,1.,1.,1.,1.,1.,1.,1.,1.,1.,1.,1.,
1.,1.,1.,1.,1.,1.,1.,1.,1.,1.,1.,1.,1.,1.,1.,1.,1.,1.,1.,1.,1.,1.,1.,1.,
1.,1.,1.,1.,1.,1.,1.,1.,1.,1.,1.,1.,1.,1.,1.,1.,1.,1.,1.,1.,1.,1.,1.,1.,
1.,1.,1.,1.,1.,1.,1.,1.,1.,1.,1.,1.,1.,1.,1.,1.,1.,1.,1.,1.,1.,1.,1.,1.,
1.,1.,1.,1.,1.,1.,1.,1.,1.,1.,1.,1.,1.,1.,1.,1.,1.,1.,1.,1.,1.,1.,1.,1.,
1.,1.,1.,1.,1.,1.,1.,1.,1.,1.,1.,1.,1.,1.,1.,1.,1.,1.,1.,1.,1.,1.,1.,1.,
1.,1.,1.,1.,1.,1.,1.,1.,1.,1.,1.,1.,1.,1.,1.,1.,1.,1.,1.,1.,1.,1.,1.,1.,
1.,1.,1.,1.,1.,1.,1.,1.,1.,1.,1.,1.,1.,1.,1.,1.,1.,1.,1.,1.,1.))
REPRESENTATION_ITEM('')
);
#766=(
BOUNDED_CURVE()
B_SPLINE_CURVE(5,(#202727,#202728,#202729,#202730,#202731,#202732,#202733,
#202734,#202735,#202736,#202737,#202738,#202739,#202740,#202741,#202742,
#202743,#202744,#202745,#202746,#202747,#202748,#202749,#202750,#202751,
#202752,#202753,#202754,#202755,#202756,#202757,#202758,#202759,#202760,
#202761,#202762,#202763,#202764,#202765,#202766,#202767,#202768,#202769,
#202770,#202771,#202772,#202773,#202774,#202775,#202776,#202777,#202778,
#202779,#202780,#202781,#202782,#202783,#202784,#202785,#202786,#202787,
#202788,#202789,#202790,#202791,#202792,#202793,#202794,#202795,#202796,
#202797,#202798,#202799,#202800,#202801,#202802,#202803,#202804,#202805,
#202806,#202807,#202808,#202809,#202810,#202811,#202812,#202813,#202814,
#202815,#202816,#202817,#202818,#202819,#202820,#202821,#202822,#202823,
#202824,#202825,#202826,#202827,#202828,#202829,#202830,#202831,#202832,
#202833,#202834,#202835,#202836,#202837,#202838,#202839,#202840,#202841,
#202842,#202843,#202844,#202845,#202846,#202847,#202848,#202849,#202850,
#202851,#202852,#202853,#202854,#202855,#202856,#202857,#202858,#202859,
#202860,#202861,#202862,#202863,#202864,#202865,#202866,#202867,#202868,
#202869,#202870,#202871,#202872,#202873,#202874,#202875,#202876,#202877,
#202878,#202879,#202880,#202881,#202882,#202883,#202884,#202885,#202886,
#202887,#202888,#202889,#202890,#202891,#202892,#202893,#202894,#202895,
#202896,#202897,#202898,#202899,#202900,#202901,#202902,#202903,#202904,
#202905,#202906,#202907,#202908,#202909,#202910,#202911,#202912,#202913,
#202914,#202915,#202916,#202917,#202918,#202919,#202920,#202921,#202922,
#202923,#202924,#202925,#202926,#202927,#202928,#202929,#202930,#202931),
 .UNSPECIFIED.,.F.,.F.)
B_SPLINE_CURVE_WITH_KNOTS((6,1,1,1,1,1,1,1,1,1,1,1,1,1,1,1,1,1,1,1,1,1,
1,1,1,1,1,1,1,1,1,1,1,1,1,1,1,1,1,1,1,1,1,1,1,1,1,1,1,1,1,1,1,1,1,1,1,1,
1,1,1,1,1,1,1,1,1,1,1,1,1,1,1,1,1,1,1,1,1,1,1,1,1,1,1,1,1,1,1,1,1,1,1,1,
1,1,1,1,1,1,1,1,1,1,1,1,1,1,1,1,1,1,1,1,1,1,1,1,1,1,1,1,1,1,1,1,1,1,1,1,
1,1,1,1,1,1,1,1,1,1,1,1,1,1,1,1,1,1,1,1,1,1,1,1,1,1,1,1,1,1,1,1,1,1,1,1,
1,1,1,1,1,1,1,1,1,1,1,1,1,1,1,1,1,1,1,1,1,1,1,1,1,1,1,1,1,1,1,1,1,1,6),
(0.,0.005,0.01,0.015,0.02,0.025,0.03,0.035,0.04,0.045,0.05,0.055,0.06,0.065,
0.07,0.075,0.08,0.085,0.09,0.095,0.1,0.105,0.11,0.115,0.12,0.125,0.13,0.135,
0.14,0.145,0.15,0.155,0.16,0.165,0.17,0.175,0.18,0.185,0.19,0.195,0.2,0.205,
0.21,0.215,0.22,0.225,0.23,0.235,0.24,0.245,0.25,0.255,0.26,0.265,0.27,
0.275,0.28,0.285,0.29,0.295,0.3,0.305,0.31,0.315,0.32,0.325,0.33,0.335,
0.34,0.345,0.35,0.355,0.36,0.365,0.37,0.375,0.38,0.385,0.39,0.395,0.4,0.405,
0.41,0.415,0.42,0.425,0.43,0.435,0.44,0.445,0.45,0.455,0.46,0.465,0.47,
0.475,0.48,0.485,0.49,0.495,0.5,0.505,0.51,0.515,0.52,0.525,0.53,0.535,
0.54,0.545,0.55,0.555,0.56,0.565,0.57,0.575,0.58,0.585,0.59,0.595,0.6,0.605,
0.61,0.615,0.62,0.625,0.63,0.635,0.64,0.645,0.65,0.655,0.66,0.665,0.67,
0.675,0.68,0.685,0.690000000000001,0.695000000000001,0.700000000000001,
0.705000000000001,0.710000000000001,0.715000000000001,0.720000000000001,
0.725000000000001,0.730000000000001,0.735000000000001,0.740000000000001,
0.745000000000001,0.750000000000001,0.755000000000001,0.760000000000001,
0.765000000000001,0.770000000000001,0.775000000000001,0.780000000000001,
0.785000000000001,0.790000000000001,0.795000000000001,0.800000000000001,
0.805000000000001,0.810000000000001,0.815000000000001,0.820000000000001,
0.825000000000001,0.830000000000001,0.835000000000001,0.840000000000001,
0.845000000000001,0.850000000000001,0.855000000000001,0.860000000000001,
0.865000000000001,0.870000000000001,0.875000000000001,0.880000000000001,
0.885000000000001,0.890000000000001,0.895000000000001,0.900000000000001,
0.905000000000001,0.910000000000001,0.915000000000001,0.920000000000001,
0.925000000000001,0.930000000000001,0.935000000000001,0.940000000000001,
0.945000000000001,0.950000000000001,0.955000000000001,0.960000000000001,
0.965000000000001,0.970000000000001,0.975000000000001,0.980000000000001,
0.985000000000001,0.990000000000001,0.995000000000001,1.),.UNSPECIFIED.)
CURVE()
GEOMETRIC_REPRESENTATION_ITEM()
RATIONAL_B_SPLINE_CURVE((1.,1.,1.,1.,1.,1.,1.,1.,1.,1.,1.,1.,1.,1.,1.,1.,
1.,1.,1.,1.,1.,1.,1.,1.,1.,1.,1.,1.,1.,1.,1.,1.,1.,1.,1.,1.,1.,1.,1.,1.,
1.,1.,1.,1.,1.,1.,1.,1.,1.,1.,1.,1.,1.,1.,1.,1.,1.,1.,1.,1.,1.,1.,1.,1.,
1.,1.,1.,1.,1.,1.,1.,1.,1.,1.,1.,1.,1.,1.,1.,1.,1.,1.,1.,1.,1.,1.,1.,1.,
1.,1.,1.,1.,1.,1.,1.,1.,1.,1.,1.,1.,1.,1.,1.,1.,1.,1.,1.,1.,1.,1.,1.,1.,
1.,1.,1.,1.,1.,1.,1.,1.,1.,1.,1.,1.,1.,1.,1.,1.,1.,1.,1.,1.,1.,1.,1.,1.,
1.,1.,1.,1.,1.,1.,1.,1.,1.,1.,1.,1.,1.,1.,1.,1.,1.,1.,1.,1.,1.,1.,1.,1.,
1.,1.,1.,1.,1.,1.,1.,1.,1.,1.,1.,1.,1.,1.,1.,1.,1.,1.,1.,1.,1.,1.,1.,1.,
1.,1.,1.,1.,1.,1.,1.,1.,1.,1.,1.,1.,1.,1.,1.,1.,1.,1.,1.,1.,1.))
REPRESENTATION_ITEM('')
);
#767=(
BOUNDED_CURVE()
B_SPLINE_CURVE(5,(#203348,#203349,#203350,#203351,#203352,#203353,#203354,
#203355,#203356,#203357,#203358,#203359,#203360,#203361,#203362,#203363,
#203364,#203365,#203366,#203367,#203368,#203369,#203370,#203371,#203372,
#203373,#203374,#203375,#203376,#203377,#203378,#203379,#203380,#203381,
#203382,#203383,#203384,#203385,#203386,#203387,#203388,#203389,#203390,
#203391,#203392,#203393,#203394,#203395,#203396,#203397,#203398,#203399,
#203400,#203401,#203402,#203403,#203404,#203405,#203406,#203407,#203408,
#203409,#203410,#203411,#203412,#203413,#203414,#203415,#203416,#203417,
#203418,#203419,#203420,#203421,#203422,#203423,#203424,#203425,#203426,
#203427,#203428,#203429,#203430,#203431,#203432,#203433,#203434,#203435,
#203436,#203437,#203438,#203439,#203440,#203441,#203442,#203443,#203444,
#203445,#203446,#203447,#203448,#203449,#203450,#203451,#203452,#203453,
#203454,#203455,#203456,#203457,#203458,#203459,#203460,#203461,#203462,
#203463,#203464,#203465,#203466,#203467,#203468,#203469,#203470,#203471,
#203472,#203473,#203474,#203475,#203476,#203477,#203478,#203479,#203480,
#203481,#203482,#203483,#203484,#203485,#203486,#203487,#203488,#203489,
#203490,#203491,#203492,#203493,#203494,#203495,#203496,#203497,#203498,
#203499,#203500,#203501,#203502,#203503,#203504,#203505,#203506,#203507,
#203508,#203509,#203510,#203511,#203512,#203513,#203514,#203515,#203516,
#203517,#203518,#203519,#203520,#203521,#203522,#203523,#203524,#203525,
#203526,#203527,#203528,#203529,#203530,#203531,#203532,#203533,#203534,
#203535,#203536,#203537,#203538,#203539,#203540,#203541,#203542,#203543,
#203544,#203545,#203546,#203547,#203548,#203549,#203550,#203551,#203552),
 .UNSPECIFIED.,.F.,.F.)
B_SPLINE_CURVE_WITH_KNOTS((6,1,1,1,1,1,1,1,1,1,1,1,1,1,1,1,1,1,1,1,1,1,
1,1,1,1,1,1,1,1,1,1,1,1,1,1,1,1,1,1,1,1,1,1,1,1,1,1,1,1,1,1,1,1,1,1,1,1,
1,1,1,1,1,1,1,1,1,1,1,1,1,1,1,1,1,1,1,1,1,1,1,1,1,1,1,1,1,1,1,1,1,1,1,1,
1,1,1,1,1,1,1,1,1,1,1,1,1,1,1,1,1,1,1,1,1,1,1,1,1,1,1,1,1,1,1,1,1,1,1,1,
1,1,1,1,1,1,1,1,1,1,1,1,1,1,1,1,1,1,1,1,1,1,1,1,1,1,1,1,1,1,1,1,1,1,1,1,
1,1,1,1,1,1,1,1,1,1,1,1,1,1,1,1,1,1,1,1,1,1,1,1,1,1,1,1,1,1,1,1,1,1,6),
(-1.,-0.995000000000001,-0.990000000000001,-0.985000000000001,-0.980000000000001,
-0.975000000000001,-0.970000000000001,-0.965000000000001,-0.960000000000001,
-0.955000000000001,-0.950000000000001,-0.945000000000001,-0.940000000000001,
-0.935000000000001,-0.930000000000001,-0.925000000000001,-0.920000000000001,
-0.915000000000001,-0.910000000000001,-0.905000000000001,-0.900000000000001,
-0.895000000000001,-0.890000000000001,-0.885000000000001,-0.880000000000001,
-0.875000000000001,-0.870000000000001,-0.865000000000001,-0.860000000000001,
-0.855000000000001,-0.850000000000001,-0.845000000000001,-0.840000000000001,
-0.835000000000001,-0.830000000000001,-0.825000000000001,-0.820000000000001,
-0.815000000000001,-0.810000000000001,-0.805000000000001,-0.800000000000001,
-0.795000000000001,-0.790000000000001,-0.785000000000001,-0.780000000000001,
-0.775000000000001,-0.770000000000001,-0.765000000000001,-0.760000000000001,
-0.755000000000001,-0.750000000000001,-0.745000000000001,-0.740000000000001,
-0.735000000000001,-0.730000000000001,-0.725000000000001,-0.720000000000001,
-0.715000000000001,-0.710000000000001,-0.705000000000001,-0.700000000000001,
-0.695000000000001,-0.690000000000001,-0.685,-0.68,-0.675,-0.67,-0.665,
-0.66,-0.655,-0.65,-0.645,-0.64,-0.635,-0.63,-0.625,-0.62,-0.615,-0.61,
-0.605,-0.6,-0.595,-0.59,-0.585,-0.58,-0.575,-0.57,-0.565,-0.56,-0.555,
-0.55,-0.545,-0.54,-0.535,-0.53,-0.525,-0.52,-0.515,-0.51,-0.505,-0.5,-0.495,
-0.49,-0.485,-0.48,-0.475,-0.47,-0.465,-0.46,-0.455,-0.45,-0.445,-0.44,
-0.435,-0.43,-0.425,-0.42,-0.415,-0.41,-0.405,-0.4,-0.395,-0.39,-0.385,
-0.38,-0.375,-0.37,-0.365,-0.36,-0.355,-0.35,-0.345,-0.34,-0.335,-0.33,
-0.325,-0.32,-0.315,-0.31,-0.305,-0.3,-0.295,-0.29,-0.285,-0.28,-0.275,
-0.27,-0.265,-0.26,-0.255,-0.25,-0.245,-0.24,-0.235,-0.23,-0.225,-0.22,
-0.215,-0.21,-0.205,-0.2,-0.195,-0.19,-0.185,-0.18,-0.175,-0.17,-0.165,
-0.16,-0.155,-0.15,-0.145,-0.14,-0.135,-0.13,-0.125,-0.12,-0.115,-0.11,
-0.105,-0.1,-0.095,-0.09,-0.085,-0.08,-0.075,-0.07,-0.065,-0.06,-0.055,
-0.05,-0.045,-0.04,-0.035,-0.03,-0.025,-0.02,-0.015,-0.01,-0.005,0.),
 .UNSPECIFIED.)
CURVE()
GEOMETRIC_REPRESENTATION_ITEM()
RATIONAL_B_SPLINE_CURVE((1.,1.,1.,1.,1.,1.,1.,1.,1.,1.,1.,1.,1.,1.,1.,1.,
1.,1.,1.,1.,1.,1.,1.,1.,1.,1.,1.,1.,1.,1.,1.,1.,1.,1.,1.,1.,1.,1.,1.,1.,
1.,1.,1.,1.,1.,1.,1.,1.,1.,1.,1.,1.,1.,1.,1.,1.,1.,1.,1.,1.,1.,1.,1.,1.,
1.,1.,1.,1.,1.,1.,1.,1.,1.,1.,1.,1.,1.,1.,1.,1.,1.,1.,1.,1.,1.,1.,1.,1.,
1.,1.,1.,1.,1.,1.,1.,1.,1.,1.,1.,1.,1.,1.,1.,1.,1.,1.,1.,1.,1.,1.,1.,1.,
1.,1.,1.,1.,1.,1.,1.,1.,1.,1.,1.,1.,1.,1.,1.,1.,1.,1.,1.,1.,1.,1.,1.,1.,
1.,1.,1.,1.,1.,1.,1.,1.,1.,1.,1.,1.,1.,1.,1.,1.,1.,1.,1.,1.,1.,1.,1.,1.,
1.,1.,1.,1.,1.,1.,1.,1.,1.,1.,1.,1.,1.,1.,1.,1.,1.,1.,1.,1.,1.,1.,1.,1.,
1.,1.,1.,1.,1.,1.,1.,1.,1.,1.,1.,1.,1.,1.,1.,1.,1.,1.,1.,1.,1.))
REPRESENTATION_ITEM('')
);
#768=(
BOUNDED_CURVE()
B_SPLINE_CURVE(5,(#203965,#203966,#203967,#203968,#203969,#203970,#203971,
#203972,#203973,#203974,#203975,#203976,#203977,#203978,#203979,#203980,
#203981,#203982,#203983,#203984,#203985,#203986,#203987,#203988,#203989,
#203990,#203991,#203992,#203993,#203994,#203995,#203996,#203997,#203998,
#203999,#204000,#204001,#204002,#204003,#204004,#204005,#204006,#204007,
#204008,#204009,#204010,#204011,#204012,#204013,#204014,#204015,#204016,
#204017,#204018,#204019,#204020,#204021,#204022,#204023,#204024,#204025,
#204026,#204027,#204028,#204029,#204030,#204031,#204032,#204033,#204034,
#204035,#204036,#204037,#204038,#204039,#204040,#204041,#204042,#204043,
#204044,#204045,#204046,#204047,#204048,#204049,#204050,#204051,#204052,
#204053,#204054,#204055,#204056,#204057,#204058,#204059,#204060,#204061,
#204062,#204063,#204064,#204065,#204066,#204067,#204068,#204069,#204070,
#204071,#204072,#204073,#204074,#204075,#204076,#204077,#204078,#204079,
#204080,#204081,#204082,#204083,#204084,#204085,#204086,#204087,#204088,
#204089,#204090,#204091,#204092,#204093,#204094,#204095,#204096,#204097,
#204098,#204099,#204100,#204101,#204102,#204103,#204104,#204105,#204106,
#204107,#204108,#204109,#204110,#204111,#204112,#204113,#204114,#204115,
#204116,#204117,#204118,#204119,#204120,#204121,#204122,#204123,#204124,
#204125,#204126,#204127,#204128,#204129,#204130,#204131,#204132,#204133,
#204134,#204135,#204136,#204137,#204138,#204139,#204140,#204141,#204142,
#204143,#204144,#204145,#204146,#204147,#204148,#204149,#204150,#204151,
#204152,#204153,#204154,#204155,#204156,#204157,#204158,#204159,#204160,
#204161,#204162,#204163,#204164,#204165,#204166,#204167,#204168,#204169),
 .UNSPECIFIED.,.F.,.F.)
B_SPLINE_CURVE_WITH_KNOTS((6,1,1,1,1,1,1,1,1,1,1,1,1,1,1,1,1,1,1,1,1,1,
1,1,1,1,1,1,1,1,1,1,1,1,1,1,1,1,1,1,1,1,1,1,1,1,1,1,1,1,1,1,1,1,1,1,1,1,
1,1,1,1,1,1,1,1,1,1,1,1,1,1,1,1,1,1,1,1,1,1,1,1,1,1,1,1,1,1,1,1,1,1,1,1,
1,1,1,1,1,1,1,1,1,1,1,1,1,1,1,1,1,1,1,1,1,1,1,1,1,1,1,1,1,1,1,1,1,1,1,1,
1,1,1,1,1,1,1,1,1,1,1,1,1,1,1,1,1,1,1,1,1,1,1,1,1,1,1,1,1,1,1,1,1,1,1,1,
1,1,1,1,1,1,1,1,1,1,1,1,1,1,1,1,1,1,1,1,1,1,1,1,1,1,1,1,1,1,1,1,1,1,6),
(0.,0.005,0.01,0.015,0.02,0.025,0.03,0.035,0.04,0.045,0.05,0.055,0.06,0.065,
0.07,0.075,0.08,0.085,0.09,0.095,0.1,0.105,0.11,0.115,0.12,0.125,0.13,0.135,
0.14,0.145,0.15,0.155,0.16,0.165,0.17,0.175,0.18,0.185,0.19,0.195,0.2,0.205,
0.21,0.215,0.22,0.225,0.23,0.235,0.24,0.245,0.25,0.255,0.26,0.265,0.27,
0.275,0.28,0.285,0.29,0.295,0.3,0.305,0.31,0.315,0.32,0.325,0.33,0.335,
0.34,0.345,0.35,0.355,0.36,0.365,0.37,0.375,0.38,0.385,0.39,0.395,0.4,0.405,
0.41,0.415,0.42,0.425,0.43,0.435,0.44,0.445,0.45,0.455,0.46,0.465,0.47,
0.475,0.48,0.485,0.49,0.495,0.5,0.505,0.51,0.515,0.52,0.525,0.53,0.535,
0.54,0.545,0.55,0.555,0.56,0.565,0.57,0.575,0.58,0.585,0.59,0.595,0.6,0.605,
0.61,0.615,0.62,0.625,0.63,0.635,0.64,0.645,0.65,0.655,0.66,0.665,0.67,
0.675,0.68,0.685,0.690000000000001,0.695000000000001,0.700000000000001,
0.705000000000001,0.710000000000001,0.715000000000001,0.720000000000001,
0.725000000000001,0.730000000000001,0.735000000000001,0.740000000000001,
0.745000000000001,0.750000000000001,0.755000000000001,0.760000000000001,
0.765000000000001,0.770000000000001,0.775000000000001,0.780000000000001,
0.785000000000001,0.790000000000001,0.795000000000001,0.800000000000001,
0.805000000000001,0.810000000000001,0.815000000000001,0.820000000000001,
0.825000000000001,0.830000000000001,0.835000000000001,0.840000000000001,
0.845000000000001,0.850000000000001,0.855000000000001,0.860000000000001,
0.865000000000001,0.870000000000001,0.875000000000001,0.880000000000001,
0.885000000000001,0.890000000000001,0.895000000000001,0.900000000000001,
0.905000000000001,0.910000000000001,0.915000000000001,0.920000000000001,
0.925000000000001,0.930000000000001,0.935000000000001,0.940000000000001,
0.945000000000001,0.950000000000001,0.955000000000001,0.960000000000001,
0.965000000000001,0.970000000000001,0.975000000000001,0.980000000000001,
0.985000000000001,0.990000000000001,0.995000000000001,1.),.UNSPECIFIED.)
CURVE()
GEOMETRIC_REPRESENTATION_ITEM()
RATIONAL_B_SPLINE_CURVE((1.,1.,1.,1.,1.,1.,1.,1.,1.,1.,1.,1.,1.,1.,1.,1.,
1.,1.,1.,1.,1.,1.,1.,1.,1.,1.,1.,1.,1.,1.,1.,1.,1.,1.,1.,1.,1.,1.,1.,1.,
1.,1.,1.,1.,1.,1.,1.,1.,1.,1.,1.,1.,1.,1.,1.,1.,1.,1.,1.,1.,1.,1.,1.,1.,
1.,1.,1.,1.,1.,1.,1.,1.,1.,1.,1.,1.,1.,1.,1.,1.,1.,1.,1.,1.,1.,1.,1.,1.,
1.,1.,1.,1.,1.,1.,1.,1.,1.,1.,1.,1.,1.,1.,1.,1.,1.,1.,1.,1.,1.,1.,1.,1.,
1.,1.,1.,1.,1.,1.,1.,1.,1.,1.,1.,1.,1.,1.,1.,1.,1.,1.,1.,1.,1.,1.,1.,1.,
1.,1.,1.,1.,1.,1.,1.,1.,1.,1.,1.,1.,1.,1.,1.,1.,1.,1.,1.,1.,1.,1.,1.,1.,
1.,1.,1.,1.,1.,1.,1.,1.,1.,1.,1.,1.,1.,1.,1.,1.,1.,1.,1.,1.,1.,1.,1.,1.,
1.,1.,1.,1.,1.,1.,1.,1.,1.,1.,1.,1.,1.,1.,1.,1.,1.,1.,1.,1.,1.))
REPRESENTATION_ITEM('')
);
#769=(
BOUNDED_CURVE()
B_SPLINE_CURVE(5,(#204586,#204587,#204588,#204589,#204590,#204591,#204592,
#204593,#204594,#204595,#204596,#204597,#204598,#204599,#204600,#204601,
#204602,#204603,#204604,#204605,#204606,#204607,#204608,#204609,#204610,
#204611,#204612,#204613,#204614,#204615,#204616,#204617,#204618,#204619,
#204620,#204621,#204622,#204623,#204624,#204625,#204626,#204627,#204628,
#204629,#204630,#204631,#204632,#204633,#204634,#204635,#204636,#204637,
#204638,#204639,#204640,#204641,#204642,#204643,#204644,#204645,#204646,
#204647,#204648,#204649,#204650,#204651,#204652,#204653,#204654,#204655,
#204656,#204657,#204658,#204659,#204660,#204661,#204662,#204663,#204664,
#204665,#204666,#204667,#204668,#204669,#204670,#204671,#204672,#204673,
#204674,#204675,#204676,#204677,#204678,#204679,#204680,#204681,#204682,
#204683,#204684,#204685,#204686,#204687,#204688,#204689,#204690,#204691,
#204692,#204693,#204694,#204695,#204696,#204697,#204698,#204699,#204700,
#204701,#204702,#204703,#204704,#204705,#204706,#204707,#204708,#204709,
#204710,#204711,#204712,#204713,#204714,#204715,#204716,#204717,#204718,
#204719,#204720,#204721,#204722,#204723,#204724,#204725,#204726,#204727,
#204728,#204729,#204730,#204731,#204732,#204733,#204734,#204735,#204736,
#204737,#204738,#204739,#204740,#204741,#204742,#204743,#204744,#204745,
#204746,#204747,#204748,#204749,#204750,#204751,#204752,#204753,#204754,
#204755,#204756,#204757,#204758,#204759,#204760,#204761,#204762,#204763,
#204764,#204765,#204766,#204767,#204768,#204769,#204770,#204771,#204772,
#204773,#204774,#204775,#204776,#204777,#204778,#204779,#204780,#204781,
#204782,#204783,#204784,#204785,#204786,#204787,#204788,#204789,#204790),
 .UNSPECIFIED.,.F.,.F.)
B_SPLINE_CURVE_WITH_KNOTS((6,1,1,1,1,1,1,1,1,1,1,1,1,1,1,1,1,1,1,1,1,1,
1,1,1,1,1,1,1,1,1,1,1,1,1,1,1,1,1,1,1,1,1,1,1,1,1,1,1,1,1,1,1,1,1,1,1,1,
1,1,1,1,1,1,1,1,1,1,1,1,1,1,1,1,1,1,1,1,1,1,1,1,1,1,1,1,1,1,1,1,1,1,1,1,
1,1,1,1,1,1,1,1,1,1,1,1,1,1,1,1,1,1,1,1,1,1,1,1,1,1,1,1,1,1,1,1,1,1,1,1,
1,1,1,1,1,1,1,1,1,1,1,1,1,1,1,1,1,1,1,1,1,1,1,1,1,1,1,1,1,1,1,1,1,1,1,1,
1,1,1,1,1,1,1,1,1,1,1,1,1,1,1,1,1,1,1,1,1,1,1,1,1,1,1,1,1,1,1,1,1,1,6),
(-1.,-0.995000000000001,-0.990000000000001,-0.985000000000001,-0.980000000000001,
-0.975000000000001,-0.970000000000001,-0.965000000000001,-0.960000000000001,
-0.955000000000001,-0.950000000000001,-0.945000000000001,-0.940000000000001,
-0.935000000000001,-0.930000000000001,-0.925000000000001,-0.920000000000001,
-0.915000000000001,-0.910000000000001,-0.905000000000001,-0.900000000000001,
-0.895000000000001,-0.890000000000001,-0.885000000000001,-0.880000000000001,
-0.875000000000001,-0.870000000000001,-0.865000000000001,-0.860000000000001,
-0.855000000000001,-0.850000000000001,-0.845000000000001,-0.840000000000001,
-0.835000000000001,-0.830000000000001,-0.825000000000001,-0.820000000000001,
-0.815000000000001,-0.810000000000001,-0.805000000000001,-0.800000000000001,
-0.795000000000001,-0.790000000000001,-0.785000000000001,-0.780000000000001,
-0.775000000000001,-0.770000000000001,-0.765000000000001,-0.760000000000001,
-0.755000000000001,-0.750000000000001,-0.745000000000001,-0.740000000000001,
-0.735000000000001,-0.730000000000001,-0.725000000000001,-0.720000000000001,
-0.715000000000001,-0.710000000000001,-0.705000000000001,-0.700000000000001,
-0.695000000000001,-0.690000000000001,-0.685,-0.68,-0.675,-0.67,-0.665,
-0.66,-0.655,-0.65,-0.645,-0.64,-0.635,-0.63,-0.625,-0.62,-0.615,-0.61,
-0.605,-0.6,-0.595,-0.59,-0.585,-0.58,-0.575,-0.57,-0.565,-0.56,-0.555,
-0.55,-0.545,-0.54,-0.535,-0.53,-0.525,-0.52,-0.515,-0.51,-0.505,-0.5,-0.495,
-0.49,-0.485,-0.48,-0.475,-0.47,-0.465,-0.46,-0.455,-0.45,-0.445,-0.44,
-0.435,-0.43,-0.425,-0.42,-0.415,-0.41,-0.405,-0.4,-0.395,-0.39,-0.385,
-0.38,-0.375,-0.37,-0.365,-0.36,-0.355,-0.35,-0.345,-0.34,-0.335,-0.33,
-0.325,-0.32,-0.315,-0.31,-0.305,-0.3,-0.295,-0.29,-0.285,-0.28,-0.275,
-0.27,-0.265,-0.26,-0.255,-0.25,-0.245,-0.24,-0.235,-0.23,-0.225,-0.22,
-0.215,-0.21,-0.205,-0.2,-0.195,-0.19,-0.185,-0.18,-0.175,-0.17,-0.165,
-0.16,-0.155,-0.15,-0.145,-0.14,-0.135,-0.13,-0.125,-0.12,-0.115,-0.11,
-0.105,-0.1,-0.095,-0.09,-0.085,-0.08,-0.075,-0.07,-0.065,-0.06,-0.055,
-0.05,-0.045,-0.04,-0.035,-0.03,-0.025,-0.02,-0.015,-0.01,-0.005,0.),
 .UNSPECIFIED.)
CURVE()
GEOMETRIC_REPRESENTATION_ITEM()
RATIONAL_B_SPLINE_CURVE((1.,1.,1.,1.,1.,1.,1.,1.,1.,1.,1.,1.,1.,1.,1.,1.,
1.,1.,1.,1.,1.,1.,1.,1.,1.,1.,1.,1.,1.,1.,1.,1.,1.,1.,1.,1.,1.,1.,1.,1.,
1.,1.,1.,1.,1.,1.,1.,1.,1.,1.,1.,1.,1.,1.,1.,1.,1.,1.,1.,1.,1.,1.,1.,1.,
1.,1.,1.,1.,1.,1.,1.,1.,1.,1.,1.,1.,1.,1.,1.,1.,1.,1.,1.,1.,1.,1.,1.,1.,
1.,1.,1.,1.,1.,1.,1.,1.,1.,1.,1.,1.,1.,1.,1.,1.,1.,1.,1.,1.,1.,1.,1.,1.,
1.,1.,1.,1.,1.,1.,1.,1.,1.,1.,1.,1.,1.,1.,1.,1.,1.,1.,1.,1.,1.,1.,1.,1.,
1.,1.,1.,1.,1.,1.,1.,1.,1.,1.,1.,1.,1.,1.,1.,1.,1.,1.,1.,1.,1.,1.,1.,1.,
1.,1.,1.,1.,1.,1.,1.,1.,1.,1.,1.,1.,1.,1.,1.,1.,1.,1.,1.,1.,1.,1.,1.,1.,
1.,1.,1.,1.,1.,1.,1.,1.,1.,1.,1.,1.,1.,1.,1.,1.,1.,1.,1.,1.,1.))
REPRESENTATION_ITEM('')
);
#770=(
BOUNDED_CURVE()
B_SPLINE_CURVE(5,(#205203,#205204,#205205,#205206,#205207,#205208,#205209,
#205210,#205211,#205212,#205213,#205214,#205215,#205216,#205217,#205218,
#205219,#205220,#205221,#205222,#205223,#205224,#205225,#205226,#205227,
#205228,#205229,#205230,#205231,#205232,#205233,#205234,#205235,#205236,
#205237,#205238,#205239,#205240,#205241,#205242,#205243,#205244,#205245,
#205246,#205247,#205248,#205249,#205250,#205251,#205252,#205253,#205254,
#205255,#205256,#205257,#205258,#205259,#205260,#205261,#205262,#205263,
#205264,#205265,#205266,#205267,#205268,#205269,#205270,#205271,#205272,
#205273,#205274,#205275,#205276,#205277,#205278,#205279,#205280,#205281,
#205282,#205283,#205284,#205285,#205286,#205287,#205288,#205289,#205290,
#205291,#205292,#205293,#205294,#205295,#205296,#205297,#205298,#205299,
#205300,#205301,#205302,#205303,#205304,#205305,#205306,#205307,#205308,
#205309,#205310,#205311,#205312,#205313,#205314,#205315,#205316,#205317,
#205318,#205319,#205320,#205321,#205322,#205323,#205324,#205325,#205326,
#205327,#205328,#205329,#205330,#205331,#205332,#205333,#205334,#205335,
#205336,#205337,#205338,#205339,#205340,#205341,#205342,#205343,#205344,
#205345,#205346,#205347,#205348,#205349,#205350,#205351,#205352,#205353,
#205354,#205355,#205356,#205357,#205358,#205359,#205360,#205361,#205362,
#205363,#205364,#205365,#205366,#205367,#205368,#205369,#205370,#205371,
#205372,#205373,#205374,#205375,#205376,#205377,#205378,#205379,#205380,
#205381,#205382,#205383,#205384,#205385,#205386,#205387,#205388,#205389,
#205390,#205391,#205392,#205393,#205394,#205395,#205396,#205397,#205398,
#205399,#205400,#205401,#205402,#205403,#205404,#205405,#205406,#205407),
 .UNSPECIFIED.,.F.,.F.)
B_SPLINE_CURVE_WITH_KNOTS((6,1,1,1,1,1,1,1,1,1,1,1,1,1,1,1,1,1,1,1,1,1,
1,1,1,1,1,1,1,1,1,1,1,1,1,1,1,1,1,1,1,1,1,1,1,1,1,1,1,1,1,1,1,1,1,1,1,1,
1,1,1,1,1,1,1,1,1,1,1,1,1,1,1,1,1,1,1,1,1,1,1,1,1,1,1,1,1,1,1,1,1,1,1,1,
1,1,1,1,1,1,1,1,1,1,1,1,1,1,1,1,1,1,1,1,1,1,1,1,1,1,1,1,1,1,1,1,1,1,1,1,
1,1,1,1,1,1,1,1,1,1,1,1,1,1,1,1,1,1,1,1,1,1,1,1,1,1,1,1,1,1,1,1,1,1,1,1,
1,1,1,1,1,1,1,1,1,1,1,1,1,1,1,1,1,1,1,1,1,1,1,1,1,1,1,1,1,1,1,1,1,1,6),
(0.,0.005,0.01,0.015,0.02,0.025,0.03,0.035,0.04,0.045,0.05,0.055,0.06,0.065,
0.07,0.075,0.08,0.085,0.09,0.095,0.1,0.105,0.11,0.115,0.12,0.125,0.13,0.135,
0.14,0.145,0.15,0.155,0.16,0.165,0.17,0.175,0.18,0.185,0.19,0.195,0.2,0.205,
0.21,0.215,0.22,0.225,0.23,0.235,0.24,0.245,0.25,0.255,0.26,0.265,0.27,
0.275,0.28,0.285,0.29,0.295,0.3,0.305,0.31,0.315,0.32,0.325,0.33,0.335,
0.34,0.345,0.35,0.355,0.36,0.365,0.37,0.375,0.38,0.385,0.39,0.395,0.4,0.405,
0.41,0.415,0.42,0.425,0.43,0.435,0.44,0.445,0.45,0.455,0.46,0.465,0.47,
0.475,0.48,0.485,0.49,0.495,0.5,0.505,0.51,0.515,0.52,0.525,0.53,0.535,
0.54,0.545,0.55,0.555,0.56,0.565,0.57,0.575,0.58,0.585,0.59,0.595,0.6,0.605,
0.61,0.615,0.62,0.625,0.63,0.635,0.64,0.645,0.65,0.655,0.66,0.665,0.67,
0.675,0.68,0.685,0.690000000000001,0.695000000000001,0.700000000000001,
0.705000000000001,0.710000000000001,0.715000000000001,0.720000000000001,
0.725000000000001,0.730000000000001,0.735000000000001,0.740000000000001,
0.745000000000001,0.750000000000001,0.755000000000001,0.760000000000001,
0.765000000000001,0.770000000000001,0.775000000000001,0.780000000000001,
0.785000000000001,0.790000000000001,0.795000000000001,0.800000000000001,
0.805000000000001,0.810000000000001,0.815000000000001,0.820000000000001,
0.825000000000001,0.830000000000001,0.835000000000001,0.840000000000001,
0.845000000000001,0.850000000000001,0.855000000000001,0.860000000000001,
0.865000000000001,0.870000000000001,0.875000000000001,0.880000000000001,
0.885000000000001,0.890000000000001,0.895000000000001,0.900000000000001,
0.905000000000001,0.910000000000001,0.915000000000001,0.920000000000001,
0.925000000000001,0.930000000000001,0.935000000000001,0.940000000000001,
0.945000000000001,0.950000000000001,0.955000000000001,0.960000000000001,
0.965000000000001,0.970000000000001,0.975000000000001,0.980000000000001,
0.985000000000001,0.990000000000001,0.995000000000001,1.),.UNSPECIFIED.)
CURVE()
GEOMETRIC_REPRESENTATION_ITEM()
RATIONAL_B_SPLINE_CURVE((1.,1.,1.,1.,1.,1.,1.,1.,1.,1.,1.,1.,1.,1.,1.,1.,
1.,1.,1.,1.,1.,1.,1.,1.,1.,1.,1.,1.,1.,1.,1.,1.,1.,1.,1.,1.,1.,1.,1.,1.,
1.,1.,1.,1.,1.,1.,1.,1.,1.,1.,1.,1.,1.,1.,1.,1.,1.,1.,1.,1.,1.,1.,1.,1.,
1.,1.,1.,1.,1.,1.,1.,1.,1.,1.,1.,1.,1.,1.,1.,1.,1.,1.,1.,1.,1.,1.,1.,1.,
1.,1.,1.,1.,1.,1.,1.,1.,1.,1.,1.,1.,1.,1.,1.,1.,1.,1.,1.,1.,1.,1.,1.,1.,
1.,1.,1.,1.,1.,1.,1.,1.,1.,1.,1.,1.,1.,1.,1.,1.,1.,1.,1.,1.,1.,1.,1.,1.,
1.,1.,1.,1.,1.,1.,1.,1.,1.,1.,1.,1.,1.,1.,1.,1.,1.,1.,1.,1.,1.,1.,1.,1.,
1.,1.,1.,1.,1.,1.,1.,1.,1.,1.,1.,1.,1.,1.,1.,1.,1.,1.,1.,1.,1.,1.,1.,1.,
1.,1.,1.,1.,1.,1.,1.,1.,1.,1.,1.,1.,1.,1.,1.,1.,1.,1.,1.,1.,1.))
REPRESENTATION_ITEM('')
);
#771=(
BOUNDED_CURVE()
B_SPLINE_CURVE(5,(#205824,#205825,#205826,#205827,#205828,#205829,#205830,
#205831,#205832,#205833,#205834,#205835,#205836,#205837,#205838,#205839,
#205840,#205841,#205842,#205843,#205844,#205845,#205846,#205847,#205848,
#205849,#205850,#205851,#205852,#205853,#205854,#205855,#205856,#205857,
#205858,#205859,#205860,#205861,#205862,#205863,#205864,#205865,#205866,
#205867,#205868,#205869,#205870,#205871,#205872,#205873,#205874,#205875,
#205876,#205877,#205878,#205879,#205880,#205881,#205882,#205883,#205884,
#205885,#205886,#205887,#205888,#205889,#205890,#205891,#205892,#205893,
#205894,#205895,#205896,#205897,#205898,#205899,#205900,#205901,#205902,
#205903,#205904,#205905,#205906,#205907,#205908,#205909,#205910,#205911,
#205912,#205913,#205914,#205915,#205916,#205917,#205918,#205919,#205920,
#205921,#205922,#205923,#205924,#205925,#205926,#205927,#205928,#205929,
#205930,#205931,#205932,#205933,#205934,#205935,#205936,#205937,#205938,
#205939,#205940,#205941,#205942,#205943,#205944,#205945,#205946,#205947,
#205948,#205949,#205950,#205951,#205952,#205953,#205954,#205955,#205956,
#205957,#205958,#205959,#205960,#205961,#205962,#205963,#205964,#205965,
#205966,#205967,#205968,#205969,#205970,#205971,#205972,#205973,#205974,
#205975,#205976,#205977,#205978,#205979,#205980,#205981,#205982,#205983,
#205984,#205985,#205986,#205987,#205988,#205989,#205990,#205991,#205992,
#205993,#205994,#205995,#205996,#205997,#205998,#205999,#206000,#206001,
#206002,#206003,#206004,#206005,#206006,#206007,#206008,#206009,#206010,
#206011,#206012,#206013,#206014,#206015,#206016,#206017,#206018,#206019,
#206020,#206021,#206022,#206023,#206024,#206025,#206026,#206027,#206028),
 .UNSPECIFIED.,.F.,.F.)
B_SPLINE_CURVE_WITH_KNOTS((6,1,1,1,1,1,1,1,1,1,1,1,1,1,1,1,1,1,1,1,1,1,
1,1,1,1,1,1,1,1,1,1,1,1,1,1,1,1,1,1,1,1,1,1,1,1,1,1,1,1,1,1,1,1,1,1,1,1,
1,1,1,1,1,1,1,1,1,1,1,1,1,1,1,1,1,1,1,1,1,1,1,1,1,1,1,1,1,1,1,1,1,1,1,1,
1,1,1,1,1,1,1,1,1,1,1,1,1,1,1,1,1,1,1,1,1,1,1,1,1,1,1,1,1,1,1,1,1,1,1,1,
1,1,1,1,1,1,1,1,1,1,1,1,1,1,1,1,1,1,1,1,1,1,1,1,1,1,1,1,1,1,1,1,1,1,1,1,
1,1,1,1,1,1,1,1,1,1,1,1,1,1,1,1,1,1,1,1,1,1,1,1,1,1,1,1,1,1,1,1,1,1,6),
(-1.,-0.995000000000001,-0.990000000000001,-0.985000000000001,-0.980000000000001,
-0.975000000000001,-0.970000000000001,-0.965000000000001,-0.960000000000001,
-0.955000000000001,-0.950000000000001,-0.945000000000001,-0.940000000000001,
-0.935000000000001,-0.930000000000001,-0.925000000000001,-0.920000000000001,
-0.915000000000001,-0.910000000000001,-0.905000000000001,-0.900000000000001,
-0.895000000000001,-0.890000000000001,-0.885000000000001,-0.880000000000001,
-0.875000000000001,-0.870000000000001,-0.865000000000001,-0.860000000000001,
-0.855000000000001,-0.850000000000001,-0.845000000000001,-0.840000000000001,
-0.835000000000001,-0.830000000000001,-0.825000000000001,-0.820000000000001,
-0.815000000000001,-0.810000000000001,-0.805000000000001,-0.800000000000001,
-0.795000000000001,-0.790000000000001,-0.785000000000001,-0.780000000000001,
-0.775000000000001,-0.770000000000001,-0.765000000000001,-0.760000000000001,
-0.755000000000001,-0.750000000000001,-0.745000000000001,-0.740000000000001,
-0.735000000000001,-0.730000000000001,-0.725000000000001,-0.720000000000001,
-0.715000000000001,-0.710000000000001,-0.705000000000001,-0.700000000000001,
-0.695000000000001,-0.690000000000001,-0.685,-0.68,-0.675,-0.67,-0.665,
-0.66,-0.655,-0.65,-0.645,-0.64,-0.635,-0.63,-0.625,-0.62,-0.615,-0.61,
-0.605,-0.6,-0.595,-0.59,-0.585,-0.58,-0.575,-0.57,-0.565,-0.56,-0.555,
-0.55,-0.545,-0.54,-0.535,-0.53,-0.525,-0.52,-0.515,-0.51,-0.505,-0.5,-0.495,
-0.49,-0.485,-0.48,-0.475,-0.47,-0.465,-0.46,-0.455,-0.45,-0.445,-0.44,
-0.435,-0.43,-0.425,-0.42,-0.415,-0.41,-0.405,-0.4,-0.395,-0.39,-0.385,
-0.38,-0.375,-0.37,-0.365,-0.36,-0.355,-0.35,-0.345,-0.34,-0.335,-0.33,
-0.325,-0.32,-0.315,-0.31,-0.305,-0.3,-0.295,-0.29,-0.285,-0.28,-0.275,
-0.27,-0.265,-0.26,-0.255,-0.25,-0.245,-0.24,-0.235,-0.23,-0.225,-0.22,
-0.215,-0.21,-0.205,-0.2,-0.195,-0.19,-0.185,-0.18,-0.175,-0.17,-0.165,
-0.16,-0.155,-0.15,-0.145,-0.14,-0.135,-0.13,-0.125,-0.12,-0.115,-0.11,
-0.105,-0.1,-0.095,-0.09,-0.085,-0.08,-0.075,-0.07,-0.065,-0.06,-0.055,
-0.05,-0.045,-0.04,-0.035,-0.03,-0.025,-0.02,-0.015,-0.01,-0.005,0.),
 .UNSPECIFIED.)
CURVE()
GEOMETRIC_REPRESENTATION_ITEM()
RATIONAL_B_SPLINE_CURVE((1.,1.,1.,1.,1.,1.,1.,1.,1.,1.,1.,1.,1.,1.,1.,1.,
1.,1.,1.,1.,1.,1.,1.,1.,1.,1.,1.,1.,1.,1.,1.,1.,1.,1.,1.,1.,1.,1.,1.,1.,
1.,1.,1.,1.,1.,1.,1.,1.,1.,1.,1.,1.,1.,1.,1.,1.,1.,1.,1.,1.,1.,1.,1.,1.,
1.,1.,1.,1.,1.,1.,1.,1.,1.,1.,1.,1.,1.,1.,1.,1.,1.,1.,1.,1.,1.,1.,1.,1.,
1.,1.,1.,1.,1.,1.,1.,1.,1.,1.,1.,1.,1.,1.,1.,1.,1.,1.,1.,1.,1.,1.,1.,1.,
1.,1.,1.,1.,1.,1.,1.,1.,1.,1.,1.,1.,1.,1.,1.,1.,1.,1.,1.,1.,1.,1.,1.,1.,
1.,1.,1.,1.,1.,1.,1.,1.,1.,1.,1.,1.,1.,1.,1.,1.,1.,1.,1.,1.,1.,1.,1.,1.,
1.,1.,1.,1.,1.,1.,1.,1.,1.,1.,1.,1.,1.,1.,1.,1.,1.,1.,1.,1.,1.,1.,1.,1.,
1.,1.,1.,1.,1.,1.,1.,1.,1.,1.,1.,1.,1.,1.,1.,1.,1.,1.,1.,1.,1.))
REPRESENTATION_ITEM('')
);
#772=(
BOUNDED_CURVE()
B_SPLINE_CURVE(5,(#206441,#206442,#206443,#206444,#206445,#206446,#206447,
#206448,#206449,#206450,#206451,#206452,#206453,#206454,#206455,#206456,
#206457,#206458,#206459,#206460,#206461,#206462,#206463,#206464,#206465,
#206466,#206467,#206468,#206469,#206470,#206471,#206472,#206473,#206474,
#206475,#206476,#206477,#206478,#206479,#206480,#206481,#206482,#206483,
#206484,#206485,#206486,#206487,#206488,#206489,#206490,#206491,#206492,
#206493,#206494,#206495,#206496,#206497,#206498,#206499,#206500,#206501,
#206502,#206503,#206504,#206505,#206506,#206507,#206508,#206509,#206510,
#206511,#206512,#206513,#206514,#206515,#206516,#206517,#206518,#206519,
#206520,#206521,#206522,#206523,#206524,#206525,#206526,#206527,#206528,
#206529,#206530,#206531,#206532,#206533,#206534,#206535,#206536,#206537,
#206538,#206539,#206540,#206541,#206542,#206543,#206544,#206545,#206546,
#206547,#206548,#206549,#206550,#206551,#206552,#206553,#206554,#206555,
#206556,#206557,#206558,#206559,#206560,#206561,#206562,#206563,#206564,
#206565,#206566,#206567,#206568,#206569,#206570,#206571,#206572,#206573,
#206574,#206575,#206576,#206577,#206578,#206579,#206580,#206581,#206582,
#206583,#206584,#206585,#206586,#206587,#206588,#206589,#206590,#206591,
#206592,#206593,#206594,#206595,#206596,#206597,#206598,#206599,#206600,
#206601,#206602,#206603,#206604,#206605,#206606,#206607,#206608,#206609,
#206610,#206611,#206612,#206613,#206614,#206615,#206616,#206617,#206618,
#206619,#206620,#206621,#206622,#206623,#206624,#206625,#206626,#206627,
#206628,#206629,#206630,#206631,#206632,#206633,#206634,#206635,#206636,
#206637,#206638,#206639,#206640,#206641,#206642,#206643,#206644,#206645),
 .UNSPECIFIED.,.F.,.F.)
B_SPLINE_CURVE_WITH_KNOTS((6,1,1,1,1,1,1,1,1,1,1,1,1,1,1,1,1,1,1,1,1,1,
1,1,1,1,1,1,1,1,1,1,1,1,1,1,1,1,1,1,1,1,1,1,1,1,1,1,1,1,1,1,1,1,1,1,1,1,
1,1,1,1,1,1,1,1,1,1,1,1,1,1,1,1,1,1,1,1,1,1,1,1,1,1,1,1,1,1,1,1,1,1,1,1,
1,1,1,1,1,1,1,1,1,1,1,1,1,1,1,1,1,1,1,1,1,1,1,1,1,1,1,1,1,1,1,1,1,1,1,1,
1,1,1,1,1,1,1,1,1,1,1,1,1,1,1,1,1,1,1,1,1,1,1,1,1,1,1,1,1,1,1,1,1,1,1,1,
1,1,1,1,1,1,1,1,1,1,1,1,1,1,1,1,1,1,1,1,1,1,1,1,1,1,1,1,1,1,1,1,1,1,6),
(0.,0.005,0.01,0.015,0.02,0.025,0.03,0.035,0.04,0.045,0.05,0.055,0.06,0.065,
0.07,0.075,0.08,0.085,0.09,0.095,0.1,0.105,0.11,0.115,0.12,0.125,0.13,0.135,
0.14,0.145,0.15,0.155,0.16,0.165,0.17,0.175,0.18,0.185,0.19,0.195,0.2,0.205,
0.21,0.215,0.22,0.225,0.23,0.235,0.24,0.245,0.25,0.255,0.26,0.265,0.27,
0.275,0.28,0.285,0.29,0.295,0.3,0.305,0.31,0.315,0.32,0.325,0.33,0.335,
0.34,0.345,0.35,0.355,0.36,0.365,0.37,0.375,0.38,0.385,0.39,0.395,0.4,0.405,
0.41,0.415,0.42,0.425,0.43,0.435,0.44,0.445,0.45,0.455,0.46,0.465,0.47,
0.475,0.48,0.485,0.49,0.495,0.5,0.505,0.51,0.515,0.52,0.525,0.53,0.535,
0.54,0.545,0.55,0.555,0.56,0.565,0.57,0.575,0.58,0.585,0.59,0.595,0.6,0.605,
0.61,0.615,0.62,0.625,0.63,0.635,0.64,0.645,0.65,0.655,0.66,0.665,0.67,
0.675,0.68,0.685,0.690000000000001,0.695000000000001,0.700000000000001,
0.705000000000001,0.710000000000001,0.715000000000001,0.720000000000001,
0.725000000000001,0.730000000000001,0.735000000000001,0.740000000000001,
0.745000000000001,0.750000000000001,0.755000000000001,0.760000000000001,
0.765000000000001,0.770000000000001,0.775000000000001,0.780000000000001,
0.785000000000001,0.790000000000001,0.795000000000001,0.800000000000001,
0.805000000000001,0.810000000000001,0.815000000000001,0.820000000000001,
0.825000000000001,0.830000000000001,0.835000000000001,0.840000000000001,
0.845000000000001,0.850000000000001,0.855000000000001,0.860000000000001,
0.865000000000001,0.870000000000001,0.875000000000001,0.880000000000001,
0.885000000000001,0.890000000000001,0.895000000000001,0.900000000000001,
0.905000000000001,0.910000000000001,0.915000000000001,0.920000000000001,
0.925000000000001,0.930000000000001,0.935000000000001,0.940000000000001,
0.945000000000001,0.950000000000001,0.955000000000001,0.960000000000001,
0.965000000000001,0.970000000000001,0.975000000000001,0.980000000000001,
0.985000000000001,0.990000000000001,0.995000000000001,1.),.UNSPECIFIED.)
CURVE()
GEOMETRIC_REPRESENTATION_ITEM()
RATIONAL_B_SPLINE_CURVE((1.,1.,1.,1.,1.,1.,1.,1.,1.,1.,1.,1.,1.,1.,1.,1.,
1.,1.,1.,1.,1.,1.,1.,1.,1.,1.,1.,1.,1.,1.,1.,1.,1.,1.,1.,1.,1.,1.,1.,1.,
1.,1.,1.,1.,1.,1.,1.,1.,1.,1.,1.,1.,1.,1.,1.,1.,1.,1.,1.,1.,1.,1.,1.,1.,
1.,1.,1.,1.,1.,1.,1.,1.,1.,1.,1.,1.,1.,1.,1.,1.,1.,1.,1.,1.,1.,1.,1.,1.,
1.,1.,1.,1.,1.,1.,1.,1.,1.,1.,1.,1.,1.,1.,1.,1.,1.,1.,1.,1.,1.,1.,1.,1.,
1.,1.,1.,1.,1.,1.,1.,1.,1.,1.,1.,1.,1.,1.,1.,1.,1.,1.,1.,1.,1.,1.,1.,1.,
1.,1.,1.,1.,1.,1.,1.,1.,1.,1.,1.,1.,1.,1.,1.,1.,1.,1.,1.,1.,1.,1.,1.,1.,
1.,1.,1.,1.,1.,1.,1.,1.,1.,1.,1.,1.,1.,1.,1.,1.,1.,1.,1.,1.,1.,1.,1.,1.,
1.,1.,1.,1.,1.,1.,1.,1.,1.,1.,1.,1.,1.,1.,1.,1.,1.,1.,1.,1.,1.))
REPRESENTATION_ITEM('')
);
#773=(
BOUNDED_CURVE()
B_SPLINE_CURVE(5,(#207062,#207063,#207064,#207065,#207066,#207067,#207068,
#207069,#207070,#207071,#207072,#207073,#207074,#207075,#207076,#207077,
#207078,#207079,#207080,#207081,#207082,#207083,#207084,#207085,#207086,
#207087,#207088,#207089,#207090,#207091,#207092,#207093,#207094,#207095,
#207096,#207097,#207098,#207099,#207100,#207101,#207102,#207103,#207104,
#207105,#207106,#207107,#207108,#207109,#207110,#207111,#207112,#207113,
#207114,#207115,#207116,#207117,#207118,#207119,#207120,#207121,#207122,
#207123,#207124,#207125,#207126,#207127,#207128,#207129,#207130,#207131,
#207132,#207133,#207134,#207135,#207136,#207137,#207138,#207139,#207140,
#207141,#207142,#207143,#207144,#207145,#207146,#207147,#207148,#207149,
#207150,#207151,#207152,#207153,#207154,#207155,#207156,#207157,#207158,
#207159,#207160,#207161,#207162,#207163,#207164,#207165,#207166,#207167,
#207168,#207169,#207170,#207171,#207172,#207173,#207174,#207175,#207176,
#207177,#207178,#207179,#207180,#207181,#207182,#207183,#207184,#207185,
#207186,#207187,#207188,#207189,#207190,#207191,#207192,#207193,#207194,
#207195,#207196,#207197,#207198,#207199,#207200,#207201,#207202,#207203,
#207204,#207205,#207206,#207207,#207208,#207209,#207210,#207211,#207212,
#207213,#207214,#207215,#207216,#207217,#207218,#207219,#207220,#207221,
#207222,#207223,#207224,#207225,#207226,#207227,#207228,#207229,#207230,
#207231,#207232,#207233,#207234,#207235,#207236,#207237,#207238,#207239,
#207240,#207241,#207242,#207243,#207244,#207245,#207246,#207247,#207248,
#207249,#207250,#207251,#207252,#207253,#207254,#207255,#207256,#207257,
#207258,#207259,#207260,#207261,#207262,#207263,#207264,#207265,#207266),
 .UNSPECIFIED.,.F.,.F.)
B_SPLINE_CURVE_WITH_KNOTS((6,1,1,1,1,1,1,1,1,1,1,1,1,1,1,1,1,1,1,1,1,1,
1,1,1,1,1,1,1,1,1,1,1,1,1,1,1,1,1,1,1,1,1,1,1,1,1,1,1,1,1,1,1,1,1,1,1,1,
1,1,1,1,1,1,1,1,1,1,1,1,1,1,1,1,1,1,1,1,1,1,1,1,1,1,1,1,1,1,1,1,1,1,1,1,
1,1,1,1,1,1,1,1,1,1,1,1,1,1,1,1,1,1,1,1,1,1,1,1,1,1,1,1,1,1,1,1,1,1,1,1,
1,1,1,1,1,1,1,1,1,1,1,1,1,1,1,1,1,1,1,1,1,1,1,1,1,1,1,1,1,1,1,1,1,1,1,1,
1,1,1,1,1,1,1,1,1,1,1,1,1,1,1,1,1,1,1,1,1,1,1,1,1,1,1,1,1,1,1,1,1,1,6),
(-1.,-0.995000000000001,-0.990000000000001,-0.985000000000001,-0.980000000000001,
-0.975000000000001,-0.970000000000001,-0.965000000000001,-0.960000000000001,
-0.955000000000001,-0.950000000000001,-0.945000000000001,-0.940000000000001,
-0.935000000000001,-0.930000000000001,-0.925000000000001,-0.920000000000001,
-0.915000000000001,-0.910000000000001,-0.905000000000001,-0.900000000000001,
-0.895000000000001,-0.890000000000001,-0.885000000000001,-0.880000000000001,
-0.875000000000001,-0.870000000000001,-0.865000000000001,-0.860000000000001,
-0.855000000000001,-0.850000000000001,-0.845000000000001,-0.840000000000001,
-0.835000000000001,-0.830000000000001,-0.825000000000001,-0.820000000000001,
-0.815000000000001,-0.810000000000001,-0.805000000000001,-0.800000000000001,
-0.795000000000001,-0.790000000000001,-0.785000000000001,-0.780000000000001,
-0.775000000000001,-0.770000000000001,-0.765000000000001,-0.760000000000001,
-0.755000000000001,-0.750000000000001,-0.745000000000001,-0.740000000000001,
-0.735000000000001,-0.730000000000001,-0.725000000000001,-0.720000000000001,
-0.715000000000001,-0.710000000000001,-0.705000000000001,-0.700000000000001,
-0.695000000000001,-0.690000000000001,-0.685,-0.68,-0.675,-0.67,-0.665,
-0.66,-0.655,-0.65,-0.645,-0.64,-0.635,-0.63,-0.625,-0.62,-0.615,-0.61,
-0.605,-0.6,-0.595,-0.59,-0.585,-0.58,-0.575,-0.57,-0.565,-0.56,-0.555,
-0.55,-0.545,-0.54,-0.535,-0.53,-0.525,-0.52,-0.515,-0.51,-0.505,-0.5,-0.495,
-0.49,-0.485,-0.48,-0.475,-0.47,-0.465,-0.46,-0.455,-0.45,-0.445,-0.44,
-0.435,-0.43,-0.425,-0.42,-0.415,-0.41,-0.405,-0.4,-0.395,-0.39,-0.385,
-0.38,-0.375,-0.37,-0.365,-0.36,-0.355,-0.35,-0.345,-0.34,-0.335,-0.33,
-0.325,-0.32,-0.315,-0.31,-0.305,-0.3,-0.295,-0.29,-0.285,-0.28,-0.275,
-0.27,-0.265,-0.26,-0.255,-0.25,-0.245,-0.24,-0.235,-0.23,-0.225,-0.22,
-0.215,-0.21,-0.205,-0.2,-0.195,-0.19,-0.185,-0.18,-0.175,-0.17,-0.165,
-0.16,-0.155,-0.15,-0.145,-0.14,-0.135,-0.13,-0.125,-0.12,-0.115,-0.11,
-0.105,-0.1,-0.095,-0.09,-0.085,-0.08,-0.075,-0.07,-0.065,-0.06,-0.055,
-0.05,-0.045,-0.04,-0.035,-0.03,-0.025,-0.02,-0.015,-0.01,-0.005,0.),
 .UNSPECIFIED.)
CURVE()
GEOMETRIC_REPRESENTATION_ITEM()
RATIONAL_B_SPLINE_CURVE((1.,1.,1.,1.,1.,1.,1.,1.,1.,1.,1.,1.,1.,1.,1.,1.,
1.,1.,1.,1.,1.,1.,1.,1.,1.,1.,1.,1.,1.,1.,1.,1.,1.,1.,1.,1.,1.,1.,1.,1.,
1.,1.,1.,1.,1.,1.,1.,1.,1.,1.,1.,1.,1.,1.,1.,1.,1.,1.,1.,1.,1.,1.,1.,1.,
1.,1.,1.,1.,1.,1.,1.,1.,1.,1.,1.,1.,1.,1.,1.,1.,1.,1.,1.,1.,1.,1.,1.,1.,
1.,1.,1.,1.,1.,1.,1.,1.,1.,1.,1.,1.,1.,1.,1.,1.,1.,1.,1.,1.,1.,1.,1.,1.,
1.,1.,1.,1.,1.,1.,1.,1.,1.,1.,1.,1.,1.,1.,1.,1.,1.,1.,1.,1.,1.,1.,1.,1.,
1.,1.,1.,1.,1.,1.,1.,1.,1.,1.,1.,1.,1.,1.,1.,1.,1.,1.,1.,1.,1.,1.,1.,1.,
1.,1.,1.,1.,1.,1.,1.,1.,1.,1.,1.,1.,1.,1.,1.,1.,1.,1.,1.,1.,1.,1.,1.,1.,
1.,1.,1.,1.,1.,1.,1.,1.,1.,1.,1.,1.,1.,1.,1.,1.,1.,1.,1.,1.,1.))
REPRESENTATION_ITEM('')
);
#774=(
BOUNDED_CURVE()
B_SPLINE_CURVE(5,(#207679,#207680,#207681,#207682,#207683,#207684,#207685,
#207686,#207687,#207688,#207689,#207690,#207691,#207692,#207693,#207694,
#207695,#207696,#207697,#207698,#207699,#207700,#207701,#207702,#207703,
#207704,#207705,#207706,#207707,#207708,#207709,#207710,#207711,#207712,
#207713,#207714,#207715,#207716,#207717,#207718,#207719,#207720,#207721,
#207722,#207723,#207724,#207725,#207726,#207727,#207728,#207729,#207730,
#207731,#207732,#207733,#207734,#207735,#207736,#207737,#207738,#207739,
#207740,#207741,#207742,#207743,#207744,#207745,#207746,#207747,#207748,
#207749,#207750,#207751,#207752,#207753,#207754,#207755,#207756,#207757,
#207758,#207759,#207760,#207761,#207762,#207763,#207764,#207765,#207766,
#207767,#207768,#207769,#207770,#207771,#207772,#207773,#207774,#207775,
#207776,#207777,#207778,#207779,#207780,#207781,#207782,#207783,#207784,
#207785,#207786,#207787,#207788,#207789,#207790,#207791,#207792,#207793,
#207794,#207795,#207796,#207797,#207798,#207799,#207800,#207801,#207802,
#207803,#207804,#207805,#207806,#207807,#207808,#207809,#207810,#207811,
#207812,#207813,#207814,#207815,#207816,#207817,#207818,#207819,#207820,
#207821,#207822,#207823,#207824,#207825,#207826,#207827,#207828,#207829,
#207830,#207831,#207832,#207833,#207834,#207835,#207836,#207837,#207838,
#207839,#207840,#207841,#207842,#207843,#207844,#207845,#207846,#207847,
#207848,#207849,#207850,#207851,#207852,#207853,#207854,#207855,#207856,
#207857,#207858,#207859,#207860,#207861,#207862,#207863,#207864,#207865,
#207866,#207867,#207868,#207869,#207870,#207871,#207872,#207873,#207874,
#207875,#207876,#207877,#207878,#207879,#207880,#207881,#207882,#207883),
 .UNSPECIFIED.,.F.,.F.)
B_SPLINE_CURVE_WITH_KNOTS((6,1,1,1,1,1,1,1,1,1,1,1,1,1,1,1,1,1,1,1,1,1,
1,1,1,1,1,1,1,1,1,1,1,1,1,1,1,1,1,1,1,1,1,1,1,1,1,1,1,1,1,1,1,1,1,1,1,1,
1,1,1,1,1,1,1,1,1,1,1,1,1,1,1,1,1,1,1,1,1,1,1,1,1,1,1,1,1,1,1,1,1,1,1,1,
1,1,1,1,1,1,1,1,1,1,1,1,1,1,1,1,1,1,1,1,1,1,1,1,1,1,1,1,1,1,1,1,1,1,1,1,
1,1,1,1,1,1,1,1,1,1,1,1,1,1,1,1,1,1,1,1,1,1,1,1,1,1,1,1,1,1,1,1,1,1,1,1,
1,1,1,1,1,1,1,1,1,1,1,1,1,1,1,1,1,1,1,1,1,1,1,1,1,1,1,1,1,1,1,1,1,1,6),
(0.,0.005,0.01,0.015,0.02,0.025,0.03,0.035,0.04,0.045,0.05,0.055,0.06,0.065,
0.07,0.075,0.08,0.085,0.09,0.095,0.1,0.105,0.11,0.115,0.12,0.125,0.13,0.135,
0.14,0.145,0.15,0.155,0.16,0.165,0.17,0.175,0.18,0.185,0.19,0.195,0.2,0.205,
0.21,0.215,0.22,0.225,0.23,0.235,0.24,0.245,0.25,0.255,0.26,0.265,0.27,
0.275,0.28,0.285,0.29,0.295,0.3,0.305,0.31,0.315,0.32,0.325,0.33,0.335,
0.34,0.345,0.35,0.355,0.36,0.365,0.37,0.375,0.38,0.385,0.39,0.395,0.4,0.405,
0.41,0.415,0.42,0.425,0.43,0.435,0.44,0.445,0.45,0.455,0.46,0.465,0.47,
0.475,0.48,0.485,0.49,0.495,0.5,0.505,0.51,0.515,0.52,0.525,0.53,0.535,
0.54,0.545,0.55,0.555,0.56,0.565,0.57,0.575,0.58,0.585,0.59,0.595,0.6,0.605,
0.61,0.615,0.62,0.625,0.63,0.635,0.64,0.645,0.65,0.655,0.66,0.665,0.67,
0.675,0.68,0.685,0.690000000000001,0.695000000000001,0.700000000000001,
0.705000000000001,0.710000000000001,0.715000000000001,0.720000000000001,
0.725000000000001,0.730000000000001,0.735000000000001,0.740000000000001,
0.745000000000001,0.750000000000001,0.755000000000001,0.760000000000001,
0.765000000000001,0.770000000000001,0.775000000000001,0.780000000000001,
0.785000000000001,0.790000000000001,0.795000000000001,0.800000000000001,
0.805000000000001,0.810000000000001,0.815000000000001,0.820000000000001,
0.825000000000001,0.830000000000001,0.835000000000001,0.840000000000001,
0.845000000000001,0.850000000000001,0.855000000000001,0.860000000000001,
0.865000000000001,0.870000000000001,0.875000000000001,0.880000000000001,
0.885000000000001,0.890000000000001,0.895000000000001,0.900000000000001,
0.905000000000001,0.910000000000001,0.915000000000001,0.920000000000001,
0.925000000000001,0.930000000000001,0.935000000000001,0.940000000000001,
0.945000000000001,0.950000000000001,0.955000000000001,0.960000000000001,
0.965000000000001,0.970000000000001,0.975000000000001,0.980000000000001,
0.985000000000001,0.990000000000001,0.995000000000001,1.),.UNSPECIFIED.)
CURVE()
GEOMETRIC_REPRESENTATION_ITEM()
RATIONAL_B_SPLINE_CURVE((1.,1.,1.,1.,1.,1.,1.,1.,1.,1.,1.,1.,1.,1.,1.,1.,
1.,1.,1.,1.,1.,1.,1.,1.,1.,1.,1.,1.,1.,1.,1.,1.,1.,1.,1.,1.,1.,1.,1.,1.,
1.,1.,1.,1.,1.,1.,1.,1.,1.,1.,1.,1.,1.,1.,1.,1.,1.,1.,1.,1.,1.,1.,1.,1.,
1.,1.,1.,1.,1.,1.,1.,1.,1.,1.,1.,1.,1.,1.,1.,1.,1.,1.,1.,1.,1.,1.,1.,1.,
1.,1.,1.,1.,1.,1.,1.,1.,1.,1.,1.,1.,1.,1.,1.,1.,1.,1.,1.,1.,1.,1.,1.,1.,
1.,1.,1.,1.,1.,1.,1.,1.,1.,1.,1.,1.,1.,1.,1.,1.,1.,1.,1.,1.,1.,1.,1.,1.,
1.,1.,1.,1.,1.,1.,1.,1.,1.,1.,1.,1.,1.,1.,1.,1.,1.,1.,1.,1.,1.,1.,1.,1.,
1.,1.,1.,1.,1.,1.,1.,1.,1.,1.,1.,1.,1.,1.,1.,1.,1.,1.,1.,1.,1.,1.,1.,1.,
1.,1.,1.,1.,1.,1.,1.,1.,1.,1.,1.,1.,1.,1.,1.,1.,1.,1.,1.,1.,1.))
REPRESENTATION_ITEM('')
);
#775=(
BOUNDED_CURVE()
B_SPLINE_CURVE(5,(#208300,#208301,#208302,#208303,#208304,#208305,#208306,
#208307,#208308,#208309,#208310,#208311,#208312,#208313,#208314,#208315,
#208316,#208317,#208318,#208319,#208320,#208321,#208322,#208323,#208324,
#208325,#208326,#208327,#208328,#208329,#208330,#208331,#208332,#208333,
#208334,#208335,#208336,#208337,#208338,#208339,#208340,#208341,#208342,
#208343,#208344,#208345,#208346,#208347,#208348,#208349,#208350,#208351,
#208352,#208353,#208354,#208355,#208356,#208357,#208358,#208359,#208360,
#208361,#208362,#208363,#208364,#208365,#208366,#208367,#208368,#208369,
#208370,#208371,#208372,#208373,#208374,#208375,#208376,#208377,#208378,
#208379,#208380,#208381,#208382,#208383,#208384,#208385,#208386,#208387,
#208388,#208389,#208390,#208391,#208392,#208393,#208394,#208395,#208396,
#208397,#208398,#208399,#208400,#208401,#208402,#208403,#208404,#208405,
#208406,#208407,#208408,#208409,#208410,#208411,#208412,#208413,#208414,
#208415,#208416,#208417,#208418,#208419,#208420,#208421,#208422,#208423,
#208424,#208425,#208426,#208427,#208428,#208429,#208430,#208431,#208432,
#208433,#208434,#208435,#208436,#208437,#208438,#208439,#208440,#208441,
#208442,#208443,#208444,#208445,#208446,#208447,#208448,#208449,#208450,
#208451,#208452,#208453,#208454,#208455,#208456,#208457,#208458,#208459,
#208460,#208461,#208462,#208463,#208464,#208465,#208466,#208467,#208468,
#208469,#208470,#208471,#208472,#208473,#208474,#208475,#208476,#208477,
#208478,#208479,#208480,#208481,#208482,#208483,#208484,#208485,#208486,
#208487,#208488,#208489,#208490,#208491,#208492,#208493,#208494,#208495,
#208496,#208497,#208498,#208499,#208500,#208501,#208502,#208503,#208504),
 .UNSPECIFIED.,.F.,.F.)
B_SPLINE_CURVE_WITH_KNOTS((6,1,1,1,1,1,1,1,1,1,1,1,1,1,1,1,1,1,1,1,1,1,
1,1,1,1,1,1,1,1,1,1,1,1,1,1,1,1,1,1,1,1,1,1,1,1,1,1,1,1,1,1,1,1,1,1,1,1,
1,1,1,1,1,1,1,1,1,1,1,1,1,1,1,1,1,1,1,1,1,1,1,1,1,1,1,1,1,1,1,1,1,1,1,1,
1,1,1,1,1,1,1,1,1,1,1,1,1,1,1,1,1,1,1,1,1,1,1,1,1,1,1,1,1,1,1,1,1,1,1,1,
1,1,1,1,1,1,1,1,1,1,1,1,1,1,1,1,1,1,1,1,1,1,1,1,1,1,1,1,1,1,1,1,1,1,1,1,
1,1,1,1,1,1,1,1,1,1,1,1,1,1,1,1,1,1,1,1,1,1,1,1,1,1,1,1,1,1,1,1,1,1,6),
(-1.,-0.995000000000001,-0.990000000000001,-0.985000000000001,-0.980000000000001,
-0.975000000000001,-0.970000000000001,-0.965000000000001,-0.960000000000001,
-0.955000000000001,-0.950000000000001,-0.945000000000001,-0.940000000000001,
-0.935000000000001,-0.930000000000001,-0.925000000000001,-0.920000000000001,
-0.915000000000001,-0.910000000000001,-0.905000000000001,-0.900000000000001,
-0.895000000000001,-0.890000000000001,-0.885000000000001,-0.880000000000001,
-0.875000000000001,-0.870000000000001,-0.865000000000001,-0.860000000000001,
-0.855000000000001,-0.850000000000001,-0.845000000000001,-0.840000000000001,
-0.835000000000001,-0.830000000000001,-0.825000000000001,-0.820000000000001,
-0.815000000000001,-0.810000000000001,-0.805000000000001,-0.800000000000001,
-0.795000000000001,-0.790000000000001,-0.785000000000001,-0.780000000000001,
-0.775000000000001,-0.770000000000001,-0.765000000000001,-0.760000000000001,
-0.755000000000001,-0.750000000000001,-0.745000000000001,-0.740000000000001,
-0.735000000000001,-0.730000000000001,-0.725000000000001,-0.720000000000001,
-0.715000000000001,-0.710000000000001,-0.705000000000001,-0.700000000000001,
-0.695000000000001,-0.690000000000001,-0.685,-0.68,-0.675,-0.67,-0.665,
-0.66,-0.655,-0.65,-0.645,-0.64,-0.635,-0.63,-0.625,-0.62,-0.615,-0.61,
-0.605,-0.6,-0.595,-0.59,-0.585,-0.58,-0.575,-0.57,-0.565,-0.56,-0.555,
-0.55,-0.545,-0.54,-0.535,-0.53,-0.525,-0.52,-0.515,-0.51,-0.505,-0.5,-0.495,
-0.49,-0.485,-0.48,-0.475,-0.47,-0.465,-0.46,-0.455,-0.45,-0.445,-0.44,
-0.435,-0.43,-0.425,-0.42,-0.415,-0.41,-0.405,-0.4,-0.395,-0.39,-0.385,
-0.38,-0.375,-0.37,-0.365,-0.36,-0.355,-0.35,-0.345,-0.34,-0.335,-0.33,
-0.325,-0.32,-0.315,-0.31,-0.305,-0.3,-0.295,-0.29,-0.285,-0.28,-0.275,
-0.27,-0.265,-0.26,-0.255,-0.25,-0.245,-0.24,-0.235,-0.23,-0.225,-0.22,
-0.215,-0.21,-0.205,-0.2,-0.195,-0.19,-0.185,-0.18,-0.175,-0.17,-0.165,
-0.16,-0.155,-0.15,-0.145,-0.14,-0.135,-0.13,-0.125,-0.12,-0.115,-0.11,
-0.105,-0.1,-0.095,-0.09,-0.085,-0.08,-0.075,-0.07,-0.065,-0.06,-0.055,
-0.05,-0.045,-0.04,-0.035,-0.03,-0.025,-0.02,-0.015,-0.01,-0.005,0.),
 .UNSPECIFIED.)
CURVE()
GEOMETRIC_REPRESENTATION_ITEM()
RATIONAL_B_SPLINE_CURVE((1.,1.,1.,1.,1.,1.,1.,1.,1.,1.,1.,1.,1.,1.,1.,1.,
1.,1.,1.,1.,1.,1.,1.,1.,1.,1.,1.,1.,1.,1.,1.,1.,1.,1.,1.,1.,1.,1.,1.,1.,
1.,1.,1.,1.,1.,1.,1.,1.,1.,1.,1.,1.,1.,1.,1.,1.,1.,1.,1.,1.,1.,1.,1.,1.,
1.,1.,1.,1.,1.,1.,1.,1.,1.,1.,1.,1.,1.,1.,1.,1.,1.,1.,1.,1.,1.,1.,1.,1.,
1.,1.,1.,1.,1.,1.,1.,1.,1.,1.,1.,1.,1.,1.,1.,1.,1.,1.,1.,1.,1.,1.,1.,1.,
1.,1.,1.,1.,1.,1.,1.,1.,1.,1.,1.,1.,1.,1.,1.,1.,1.,1.,1.,1.,1.,1.,1.,1.,
1.,1.,1.,1.,1.,1.,1.,1.,1.,1.,1.,1.,1.,1.,1.,1.,1.,1.,1.,1.,1.,1.,1.,1.,
1.,1.,1.,1.,1.,1.,1.,1.,1.,1.,1.,1.,1.,1.,1.,1.,1.,1.,1.,1.,1.,1.,1.,1.,
1.,1.,1.,1.,1.,1.,1.,1.,1.,1.,1.,1.,1.,1.,1.,1.,1.,1.,1.,1.,1.))
REPRESENTATION_ITEM('')
);
#776=(
BOUNDED_CURVE()
B_SPLINE_CURVE(5,(#208917,#208918,#208919,#208920,#208921,#208922,#208923,
#208924,#208925,#208926,#208927,#208928,#208929,#208930,#208931,#208932,
#208933,#208934,#208935,#208936,#208937,#208938,#208939,#208940,#208941,
#208942,#208943,#208944,#208945,#208946,#208947,#208948,#208949,#208950,
#208951,#208952,#208953,#208954,#208955,#208956,#208957,#208958,#208959,
#208960,#208961,#208962,#208963,#208964,#208965,#208966,#208967,#208968,
#208969,#208970,#208971,#208972,#208973,#208974,#208975,#208976,#208977,
#208978,#208979,#208980,#208981,#208982,#208983,#208984,#208985,#208986,
#208987,#208988,#208989,#208990,#208991,#208992,#208993,#208994,#208995,
#208996,#208997,#208998,#208999,#209000,#209001,#209002,#209003,#209004,
#209005,#209006,#209007,#209008,#209009,#209010,#209011,#209012,#209013,
#209014,#209015,#209016,#209017,#209018,#209019,#209020,#209021,#209022,
#209023,#209024,#209025,#209026,#209027,#209028,#209029,#209030,#209031,
#209032,#209033,#209034,#209035,#209036,#209037,#209038,#209039,#209040,
#209041,#209042,#209043,#209044,#209045,#209046,#209047,#209048,#209049,
#209050,#209051,#209052,#209053,#209054,#209055,#209056,#209057,#209058,
#209059,#209060,#209061,#209062,#209063,#209064,#209065,#209066,#209067,
#209068,#209069,#209070,#209071,#209072,#209073,#209074,#209075,#209076,
#209077,#209078,#209079,#209080,#209081,#209082,#209083,#209084,#209085,
#209086,#209087,#209088,#209089,#209090,#209091,#209092,#209093,#209094,
#209095,#209096,#209097,#209098,#209099,#209100,#209101,#209102,#209103,
#209104,#209105,#209106,#209107,#209108,#209109,#209110,#209111,#209112,
#209113,#209114,#209115,#209116,#209117,#209118,#209119,#209120,#209121),
 .UNSPECIFIED.,.F.,.F.)
B_SPLINE_CURVE_WITH_KNOTS((6,1,1,1,1,1,1,1,1,1,1,1,1,1,1,1,1,1,1,1,1,1,
1,1,1,1,1,1,1,1,1,1,1,1,1,1,1,1,1,1,1,1,1,1,1,1,1,1,1,1,1,1,1,1,1,1,1,1,
1,1,1,1,1,1,1,1,1,1,1,1,1,1,1,1,1,1,1,1,1,1,1,1,1,1,1,1,1,1,1,1,1,1,1,1,
1,1,1,1,1,1,1,1,1,1,1,1,1,1,1,1,1,1,1,1,1,1,1,1,1,1,1,1,1,1,1,1,1,1,1,1,
1,1,1,1,1,1,1,1,1,1,1,1,1,1,1,1,1,1,1,1,1,1,1,1,1,1,1,1,1,1,1,1,1,1,1,1,
1,1,1,1,1,1,1,1,1,1,1,1,1,1,1,1,1,1,1,1,1,1,1,1,1,1,1,1,1,1,1,1,1,1,6),
(0.,0.005,0.01,0.015,0.02,0.025,0.03,0.035,0.04,0.045,0.05,0.055,0.06,0.065,
0.07,0.075,0.08,0.085,0.09,0.095,0.1,0.105,0.11,0.115,0.12,0.125,0.13,0.135,
0.14,0.145,0.15,0.155,0.16,0.165,0.17,0.175,0.18,0.185,0.19,0.195,0.2,0.205,
0.21,0.215,0.22,0.225,0.23,0.235,0.24,0.245,0.25,0.255,0.26,0.265,0.27,
0.275,0.28,0.285,0.29,0.295,0.3,0.305,0.31,0.315,0.32,0.325,0.33,0.335,
0.34,0.345,0.35,0.355,0.36,0.365,0.37,0.375,0.38,0.385,0.39,0.395,0.4,0.405,
0.41,0.415,0.42,0.425,0.43,0.435,0.44,0.445,0.45,0.455,0.46,0.465,0.47,
0.475,0.48,0.485,0.49,0.495,0.5,0.505,0.51,0.515,0.52,0.525,0.53,0.535,
0.54,0.545,0.55,0.555,0.56,0.565,0.57,0.575,0.58,0.585,0.59,0.595,0.6,0.605,
0.61,0.615,0.62,0.625,0.63,0.635,0.64,0.645,0.65,0.655,0.66,0.665,0.67,
0.675,0.68,0.685,0.690000000000001,0.695000000000001,0.700000000000001,
0.705000000000001,0.710000000000001,0.715000000000001,0.720000000000001,
0.725000000000001,0.730000000000001,0.735000000000001,0.740000000000001,
0.745000000000001,0.750000000000001,0.755000000000001,0.760000000000001,
0.765000000000001,0.770000000000001,0.775000000000001,0.780000000000001,
0.785000000000001,0.790000000000001,0.795000000000001,0.800000000000001,
0.805000000000001,0.810000000000001,0.815000000000001,0.820000000000001,
0.825000000000001,0.830000000000001,0.835000000000001,0.840000000000001,
0.845000000000001,0.850000000000001,0.855000000000001,0.860000000000001,
0.865000000000001,0.870000000000001,0.875000000000001,0.880000000000001,
0.885000000000001,0.890000000000001,0.895000000000001,0.900000000000001,
0.905000000000001,0.910000000000001,0.915000000000001,0.920000000000001,
0.925000000000001,0.930000000000001,0.935000000000001,0.940000000000001,
0.945000000000001,0.950000000000001,0.955000000000001,0.960000000000001,
0.965000000000001,0.970000000000001,0.975000000000001,0.980000000000001,
0.985000000000001,0.990000000000001,0.995000000000001,1.),.UNSPECIFIED.)
CURVE()
GEOMETRIC_REPRESENTATION_ITEM()
RATIONAL_B_SPLINE_CURVE((1.,1.,1.,1.,1.,1.,1.,1.,1.,1.,1.,1.,1.,1.,1.,1.,
1.,1.,1.,1.,1.,1.,1.,1.,1.,1.,1.,1.,1.,1.,1.,1.,1.,1.,1.,1.,1.,1.,1.,1.,
1.,1.,1.,1.,1.,1.,1.,1.,1.,1.,1.,1.,1.,1.,1.,1.,1.,1.,1.,1.,1.,1.,1.,1.,
1.,1.,1.,1.,1.,1.,1.,1.,1.,1.,1.,1.,1.,1.,1.,1.,1.,1.,1.,1.,1.,1.,1.,1.,
1.,1.,1.,1.,1.,1.,1.,1.,1.,1.,1.,1.,1.,1.,1.,1.,1.,1.,1.,1.,1.,1.,1.,1.,
1.,1.,1.,1.,1.,1.,1.,1.,1.,1.,1.,1.,1.,1.,1.,1.,1.,1.,1.,1.,1.,1.,1.,1.,
1.,1.,1.,1.,1.,1.,1.,1.,1.,1.,1.,1.,1.,1.,1.,1.,1.,1.,1.,1.,1.,1.,1.,1.,
1.,1.,1.,1.,1.,1.,1.,1.,1.,1.,1.,1.,1.,1.,1.,1.,1.,1.,1.,1.,1.,1.,1.,1.,
1.,1.,1.,1.,1.,1.,1.,1.,1.,1.,1.,1.,1.,1.,1.,1.,1.,1.,1.,1.,1.))
REPRESENTATION_ITEM('')
);
#777=(
BOUNDED_CURVE()
B_SPLINE_CURVE(5,(#209538,#209539,#209540,#209541,#209542,#209543,#209544,
#209545,#209546,#209547,#209548,#209549,#209550,#209551,#209552,#209553,
#209554,#209555,#209556,#209557,#209558,#209559,#209560,#209561,#209562,
#209563,#209564,#209565,#209566,#209567,#209568,#209569,#209570,#209571,
#209572,#209573,#209574,#209575,#209576,#209577,#209578,#209579,#209580,
#209581,#209582,#209583,#209584,#209585,#209586,#209587,#209588,#209589,
#209590,#209591,#209592,#209593,#209594,#209595,#209596,#209597,#209598,
#209599,#209600,#209601,#209602,#209603,#209604,#209605,#209606,#209607,
#209608,#209609,#209610,#209611,#209612,#209613,#209614,#209615,#209616,
#209617,#209618,#209619,#209620,#209621,#209622,#209623,#209624,#209625,
#209626,#209627,#209628,#209629,#209630,#209631,#209632,#209633,#209634,
#209635,#209636,#209637,#209638,#209639,#209640,#209641,#209642,#209643,
#209644,#209645,#209646,#209647,#209648,#209649,#209650,#209651,#209652,
#209653,#209654,#209655,#209656,#209657,#209658,#209659,#209660,#209661,
#209662,#209663,#209664,#209665,#209666,#209667,#209668,#209669,#209670,
#209671,#209672,#209673,#209674,#209675,#209676,#209677,#209678,#209679,
#209680,#209681,#209682,#209683,#209684,#209685,#209686,#209687,#209688,
#209689,#209690,#209691,#209692,#209693,#209694,#209695,#209696,#209697,
#209698,#209699,#209700,#209701,#209702,#209703,#209704,#209705,#209706,
#209707,#209708,#209709,#209710,#209711,#209712,#209713,#209714,#209715,
#209716,#209717,#209718,#209719,#209720,#209721,#209722,#209723,#209724,
#209725,#209726,#209727,#209728,#209729,#209730,#209731,#209732,#209733,
#209734,#209735,#209736,#209737,#209738,#209739,#209740,#209741,#209742),
 .UNSPECIFIED.,.F.,.F.)
B_SPLINE_CURVE_WITH_KNOTS((6,1,1,1,1,1,1,1,1,1,1,1,1,1,1,1,1,1,1,1,1,1,
1,1,1,1,1,1,1,1,1,1,1,1,1,1,1,1,1,1,1,1,1,1,1,1,1,1,1,1,1,1,1,1,1,1,1,1,
1,1,1,1,1,1,1,1,1,1,1,1,1,1,1,1,1,1,1,1,1,1,1,1,1,1,1,1,1,1,1,1,1,1,1,1,
1,1,1,1,1,1,1,1,1,1,1,1,1,1,1,1,1,1,1,1,1,1,1,1,1,1,1,1,1,1,1,1,1,1,1,1,
1,1,1,1,1,1,1,1,1,1,1,1,1,1,1,1,1,1,1,1,1,1,1,1,1,1,1,1,1,1,1,1,1,1,1,1,
1,1,1,1,1,1,1,1,1,1,1,1,1,1,1,1,1,1,1,1,1,1,1,1,1,1,1,1,1,1,1,1,1,1,6),
(-1.,-0.995000000000001,-0.990000000000001,-0.985000000000001,-0.980000000000001,
-0.975000000000001,-0.970000000000001,-0.965000000000001,-0.960000000000001,
-0.955000000000001,-0.950000000000001,-0.945000000000001,-0.940000000000001,
-0.935000000000001,-0.930000000000001,-0.925000000000001,-0.920000000000001,
-0.915000000000001,-0.910000000000001,-0.905000000000001,-0.900000000000001,
-0.895000000000001,-0.890000000000001,-0.885000000000001,-0.880000000000001,
-0.875000000000001,-0.870000000000001,-0.865000000000001,-0.860000000000001,
-0.855000000000001,-0.850000000000001,-0.845000000000001,-0.840000000000001,
-0.835000000000001,-0.830000000000001,-0.825000000000001,-0.820000000000001,
-0.815000000000001,-0.810000000000001,-0.805000000000001,-0.800000000000001,
-0.795000000000001,-0.790000000000001,-0.785000000000001,-0.780000000000001,
-0.775000000000001,-0.770000000000001,-0.765000000000001,-0.760000000000001,
-0.755000000000001,-0.750000000000001,-0.745000000000001,-0.740000000000001,
-0.735000000000001,-0.730000000000001,-0.725000000000001,-0.720000000000001,
-0.715000000000001,-0.710000000000001,-0.705000000000001,-0.700000000000001,
-0.695000000000001,-0.690000000000001,-0.685,-0.68,-0.675,-0.67,-0.665,
-0.66,-0.655,-0.65,-0.645,-0.64,-0.635,-0.63,-0.625,-0.62,-0.615,-0.61,
-0.605,-0.6,-0.595,-0.59,-0.585,-0.58,-0.575,-0.57,-0.565,-0.56,-0.555,
-0.55,-0.545,-0.54,-0.535,-0.53,-0.525,-0.52,-0.515,-0.51,-0.505,-0.5,-0.495,
-0.49,-0.485,-0.48,-0.475,-0.47,-0.465,-0.46,-0.455,-0.45,-0.445,-0.44,
-0.435,-0.43,-0.425,-0.42,-0.415,-0.41,-0.405,-0.4,-0.395,-0.39,-0.385,
-0.38,-0.375,-0.37,-0.365,-0.36,-0.355,-0.35,-0.345,-0.34,-0.335,-0.33,
-0.325,-0.32,-0.315,-0.31,-0.305,-0.3,-0.295,-0.29,-0.285,-0.28,-0.275,
-0.27,-0.265,-0.26,-0.255,-0.25,-0.245,-0.24,-0.235,-0.23,-0.225,-0.22,
-0.215,-0.21,-0.205,-0.2,-0.195,-0.19,-0.185,-0.18,-0.175,-0.17,-0.165,
-0.16,-0.155,-0.15,-0.145,-0.14,-0.135,-0.13,-0.125,-0.12,-0.115,-0.11,
-0.105,-0.1,-0.095,-0.09,-0.085,-0.08,-0.075,-0.07,-0.065,-0.06,-0.055,
-0.05,-0.045,-0.04,-0.035,-0.03,-0.025,-0.02,-0.015,-0.01,-0.005,0.),
 .UNSPECIFIED.)
CURVE()
GEOMETRIC_REPRESENTATION_ITEM()
RATIONAL_B_SPLINE_CURVE((1.,1.,1.,1.,1.,1.,1.,1.,1.,1.,1.,1.,1.,1.,1.,1.,
1.,1.,1.,1.,1.,1.,1.,1.,1.,1.,1.,1.,1.,1.,1.,1.,1.,1.,1.,1.,1.,1.,1.,1.,
1.,1.,1.,1.,1.,1.,1.,1.,1.,1.,1.,1.,1.,1.,1.,1.,1.,1.,1.,1.,1.,1.,1.,1.,
1.,1.,1.,1.,1.,1.,1.,1.,1.,1.,1.,1.,1.,1.,1.,1.,1.,1.,1.,1.,1.,1.,1.,1.,
1.,1.,1.,1.,1.,1.,1.,1.,1.,1.,1.,1.,1.,1.,1.,1.,1.,1.,1.,1.,1.,1.,1.,1.,
1.,1.,1.,1.,1.,1.,1.,1.,1.,1.,1.,1.,1.,1.,1.,1.,1.,1.,1.,1.,1.,1.,1.,1.,
1.,1.,1.,1.,1.,1.,1.,1.,1.,1.,1.,1.,1.,1.,1.,1.,1.,1.,1.,1.,1.,1.,1.,1.,
1.,1.,1.,1.,1.,1.,1.,1.,1.,1.,1.,1.,1.,1.,1.,1.,1.,1.,1.,1.,1.,1.,1.,1.,
1.,1.,1.,1.,1.,1.,1.,1.,1.,1.,1.,1.,1.,1.,1.,1.,1.,1.,1.,1.,1.))
REPRESENTATION_ITEM('')
);
#778=(
BOUNDED_CURVE()
B_SPLINE_CURVE(5,(#210155,#210156,#210157,#210158,#210159,#210160,#210161,
#210162,#210163,#210164,#210165,#210166,#210167,#210168,#210169,#210170,
#210171,#210172,#210173,#210174,#210175,#210176,#210177,#210178,#210179,
#210180,#210181,#210182,#210183,#210184,#210185,#210186,#210187,#210188,
#210189,#210190,#210191,#210192,#210193,#210194,#210195,#210196,#210197,
#210198,#210199,#210200,#210201,#210202,#210203,#210204,#210205,#210206,
#210207,#210208,#210209,#210210,#210211,#210212,#210213,#210214,#210215,
#210216,#210217,#210218,#210219,#210220,#210221,#210222,#210223,#210224,
#210225,#210226,#210227,#210228,#210229,#210230,#210231,#210232,#210233,
#210234,#210235,#210236,#210237,#210238,#210239,#210240,#210241,#210242,
#210243,#210244,#210245,#210246,#210247,#210248,#210249,#210250,#210251,
#210252,#210253,#210254,#210255,#210256,#210257,#210258,#210259,#210260,
#210261,#210262,#210263,#210264,#210265,#210266,#210267,#210268,#210269,
#210270,#210271,#210272,#210273,#210274,#210275,#210276,#210277,#210278,
#210279,#210280,#210281,#210282,#210283,#210284,#210285,#210286,#210287,
#210288,#210289,#210290,#210291,#210292,#210293,#210294,#210295,#210296,
#210297,#210298,#210299,#210300,#210301,#210302,#210303,#210304,#210305,
#210306,#210307,#210308,#210309,#210310,#210311,#210312,#210313,#210314,
#210315,#210316,#210317,#210318,#210319,#210320,#210321,#210322,#210323,
#210324,#210325,#210326,#210327,#210328,#210329,#210330,#210331,#210332,
#210333,#210334,#210335,#210336,#210337,#210338,#210339,#210340,#210341,
#210342,#210343,#210344,#210345,#210346,#210347,#210348,#210349,#210350,
#210351,#210352,#210353,#210354,#210355,#210356,#210357,#210358,#210359),
 .UNSPECIFIED.,.F.,.F.)
B_SPLINE_CURVE_WITH_KNOTS((6,1,1,1,1,1,1,1,1,1,1,1,1,1,1,1,1,1,1,1,1,1,
1,1,1,1,1,1,1,1,1,1,1,1,1,1,1,1,1,1,1,1,1,1,1,1,1,1,1,1,1,1,1,1,1,1,1,1,
1,1,1,1,1,1,1,1,1,1,1,1,1,1,1,1,1,1,1,1,1,1,1,1,1,1,1,1,1,1,1,1,1,1,1,1,
1,1,1,1,1,1,1,1,1,1,1,1,1,1,1,1,1,1,1,1,1,1,1,1,1,1,1,1,1,1,1,1,1,1,1,1,
1,1,1,1,1,1,1,1,1,1,1,1,1,1,1,1,1,1,1,1,1,1,1,1,1,1,1,1,1,1,1,1,1,1,1,1,
1,1,1,1,1,1,1,1,1,1,1,1,1,1,1,1,1,1,1,1,1,1,1,1,1,1,1,1,1,1,1,1,1,1,6),
(0.,0.005,0.01,0.015,0.02,0.025,0.03,0.035,0.04,0.045,0.05,0.055,0.06,0.065,
0.07,0.075,0.08,0.085,0.09,0.095,0.1,0.105,0.11,0.115,0.12,0.125,0.13,0.135,
0.14,0.145,0.15,0.155,0.16,0.165,0.17,0.175,0.18,0.185,0.19,0.195,0.2,0.205,
0.21,0.215,0.22,0.225,0.23,0.235,0.24,0.245,0.25,0.255,0.26,0.265,0.27,
0.275,0.28,0.285,0.29,0.295,0.3,0.305,0.31,0.315,0.32,0.325,0.33,0.335,
0.34,0.345,0.35,0.355,0.36,0.365,0.37,0.375,0.38,0.385,0.39,0.395,0.4,0.405,
0.41,0.415,0.42,0.425,0.43,0.435,0.44,0.445,0.45,0.455,0.46,0.465,0.47,
0.475,0.48,0.485,0.49,0.495,0.5,0.505,0.51,0.515,0.52,0.525,0.53,0.535,
0.54,0.545,0.55,0.555,0.56,0.565,0.57,0.575,0.58,0.585,0.59,0.595,0.6,0.605,
0.61,0.615,0.62,0.625,0.63,0.635,0.64,0.645,0.65,0.655,0.66,0.665,0.67,
0.675,0.68,0.685,0.690000000000001,0.695000000000001,0.700000000000001,
0.705000000000001,0.710000000000001,0.715000000000001,0.720000000000001,
0.725000000000001,0.730000000000001,0.735000000000001,0.740000000000001,
0.745000000000001,0.750000000000001,0.755000000000001,0.760000000000001,
0.765000000000001,0.770000000000001,0.775000000000001,0.780000000000001,
0.785000000000001,0.790000000000001,0.795000000000001,0.800000000000001,
0.805000000000001,0.810000000000001,0.815000000000001,0.820000000000001,
0.825000000000001,0.830000000000001,0.835000000000001,0.840000000000001,
0.845000000000001,0.850000000000001,0.855000000000001,0.860000000000001,
0.865000000000001,0.870000000000001,0.875000000000001,0.880000000000001,
0.885000000000001,0.890000000000001,0.895000000000001,0.900000000000001,
0.905000000000001,0.910000000000001,0.915000000000001,0.920000000000001,
0.925000000000001,0.930000000000001,0.935000000000001,0.940000000000001,
0.945000000000001,0.950000000000001,0.955000000000001,0.960000000000001,
0.965000000000001,0.970000000000001,0.975000000000001,0.980000000000001,
0.985000000000001,0.990000000000001,0.995000000000001,1.),.UNSPECIFIED.)
CURVE()
GEOMETRIC_REPRESENTATION_ITEM()
RATIONAL_B_SPLINE_CURVE((1.,1.,1.,1.,1.,1.,1.,1.,1.,1.,1.,1.,1.,1.,1.,1.,
1.,1.,1.,1.,1.,1.,1.,1.,1.,1.,1.,1.,1.,1.,1.,1.,1.,1.,1.,1.,1.,1.,1.,1.,
1.,1.,1.,1.,1.,1.,1.,1.,1.,1.,1.,1.,1.,1.,1.,1.,1.,1.,1.,1.,1.,1.,1.,1.,
1.,1.,1.,1.,1.,1.,1.,1.,1.,1.,1.,1.,1.,1.,1.,1.,1.,1.,1.,1.,1.,1.,1.,1.,
1.,1.,1.,1.,1.,1.,1.,1.,1.,1.,1.,1.,1.,1.,1.,1.,1.,1.,1.,1.,1.,1.,1.,1.,
1.,1.,1.,1.,1.,1.,1.,1.,1.,1.,1.,1.,1.,1.,1.,1.,1.,1.,1.,1.,1.,1.,1.,1.,
1.,1.,1.,1.,1.,1.,1.,1.,1.,1.,1.,1.,1.,1.,1.,1.,1.,1.,1.,1.,1.,1.,1.,1.,
1.,1.,1.,1.,1.,1.,1.,1.,1.,1.,1.,1.,1.,1.,1.,1.,1.,1.,1.,1.,1.,1.,1.,1.,
1.,1.,1.,1.,1.,1.,1.,1.,1.,1.,1.,1.,1.,1.,1.,1.,1.,1.,1.,1.,1.))
REPRESENTATION_ITEM('')
);
#779=(
BOUNDED_CURVE()
B_SPLINE_CURVE(5,(#210776,#210777,#210778,#210779,#210780,#210781,#210782,
#210783,#210784,#210785,#210786,#210787,#210788,#210789,#210790,#210791,
#210792,#210793,#210794,#210795,#210796,#210797,#210798,#210799,#210800,
#210801,#210802,#210803,#210804,#210805,#210806,#210807,#210808,#210809,
#210810,#210811,#210812,#210813,#210814,#210815,#210816,#210817,#210818,
#210819,#210820,#210821,#210822,#210823,#210824,#210825,#210826,#210827,
#210828,#210829,#210830,#210831,#210832,#210833,#210834,#210835,#210836,
#210837,#210838,#210839,#210840,#210841,#210842,#210843,#210844,#210845,
#210846,#210847,#210848,#210849,#210850,#210851,#210852,#210853,#210854,
#210855,#210856,#210857,#210858,#210859,#210860,#210861,#210862,#210863,
#210864,#210865,#210866,#210867,#210868,#210869,#210870,#210871,#210872,
#210873,#210874,#210875,#210876,#210877,#210878,#210879,#210880,#210881,
#210882,#210883,#210884,#210885,#210886,#210887,#210888,#210889,#210890,
#210891,#210892,#210893,#210894,#210895,#210896,#210897,#210898,#210899,
#210900,#210901,#210902,#210903,#210904,#210905,#210906,#210907,#210908,
#210909,#210910,#210911,#210912,#210913,#210914,#210915,#210916,#210917,
#210918,#210919,#210920,#210921,#210922,#210923,#210924,#210925,#210926,
#210927,#210928,#210929,#210930,#210931,#210932,#210933,#210934,#210935,
#210936,#210937,#210938,#210939,#210940,#210941,#210942,#210943,#210944,
#210945,#210946,#210947,#210948,#210949,#210950,#210951,#210952,#210953,
#210954,#210955,#210956,#210957,#210958,#210959,#210960,#210961,#210962,
#210963,#210964,#210965,#210966,#210967,#210968,#210969,#210970,#210971,
#210972,#210973,#210974,#210975,#210976,#210977,#210978,#210979,#210980),
 .UNSPECIFIED.,.F.,.F.)
B_SPLINE_CURVE_WITH_KNOTS((6,1,1,1,1,1,1,1,1,1,1,1,1,1,1,1,1,1,1,1,1,1,
1,1,1,1,1,1,1,1,1,1,1,1,1,1,1,1,1,1,1,1,1,1,1,1,1,1,1,1,1,1,1,1,1,1,1,1,
1,1,1,1,1,1,1,1,1,1,1,1,1,1,1,1,1,1,1,1,1,1,1,1,1,1,1,1,1,1,1,1,1,1,1,1,
1,1,1,1,1,1,1,1,1,1,1,1,1,1,1,1,1,1,1,1,1,1,1,1,1,1,1,1,1,1,1,1,1,1,1,1,
1,1,1,1,1,1,1,1,1,1,1,1,1,1,1,1,1,1,1,1,1,1,1,1,1,1,1,1,1,1,1,1,1,1,1,1,
1,1,1,1,1,1,1,1,1,1,1,1,1,1,1,1,1,1,1,1,1,1,1,1,1,1,1,1,1,1,1,1,1,1,6),
(-1.,-0.995000000000001,-0.990000000000001,-0.985000000000001,-0.980000000000001,
-0.975000000000001,-0.970000000000001,-0.965000000000001,-0.960000000000001,
-0.955000000000001,-0.950000000000001,-0.945000000000001,-0.940000000000001,
-0.935000000000001,-0.930000000000001,-0.925000000000001,-0.920000000000001,
-0.915000000000001,-0.910000000000001,-0.905000000000001,-0.900000000000001,
-0.895000000000001,-0.890000000000001,-0.885000000000001,-0.880000000000001,
-0.875000000000001,-0.870000000000001,-0.865000000000001,-0.860000000000001,
-0.855000000000001,-0.850000000000001,-0.845000000000001,-0.840000000000001,
-0.835000000000001,-0.830000000000001,-0.825000000000001,-0.820000000000001,
-0.815000000000001,-0.810000000000001,-0.805000000000001,-0.800000000000001,
-0.795000000000001,-0.790000000000001,-0.785000000000001,-0.780000000000001,
-0.775000000000001,-0.770000000000001,-0.765000000000001,-0.760000000000001,
-0.755000000000001,-0.750000000000001,-0.745000000000001,-0.740000000000001,
-0.735000000000001,-0.730000000000001,-0.725000000000001,-0.720000000000001,
-0.715000000000001,-0.710000000000001,-0.705000000000001,-0.700000000000001,
-0.695000000000001,-0.690000000000001,-0.685,-0.68,-0.675,-0.67,-0.665,
-0.66,-0.655,-0.65,-0.645,-0.64,-0.635,-0.63,-0.625,-0.62,-0.615,-0.61,
-0.605,-0.6,-0.595,-0.59,-0.585,-0.58,-0.575,-0.57,-0.565,-0.56,-0.555,
-0.55,-0.545,-0.54,-0.535,-0.53,-0.525,-0.52,-0.515,-0.51,-0.505,-0.5,-0.495,
-0.49,-0.485,-0.48,-0.475,-0.47,-0.465,-0.46,-0.455,-0.45,-0.445,-0.44,
-0.435,-0.43,-0.425,-0.42,-0.415,-0.41,-0.405,-0.4,-0.395,-0.39,-0.385,
-0.38,-0.375,-0.37,-0.365,-0.36,-0.355,-0.35,-0.345,-0.34,-0.335,-0.33,
-0.325,-0.32,-0.315,-0.31,-0.305,-0.3,-0.295,-0.29,-0.285,-0.28,-0.275,
-0.27,-0.265,-0.26,-0.255,-0.25,-0.245,-0.24,-0.235,-0.23,-0.225,-0.22,
-0.215,-0.21,-0.205,-0.2,-0.195,-0.19,-0.185,-0.18,-0.175,-0.17,-0.165,
-0.16,-0.155,-0.15,-0.145,-0.14,-0.135,-0.13,-0.125,-0.12,-0.115,-0.11,
-0.105,-0.1,-0.095,-0.09,-0.085,-0.08,-0.075,-0.07,-0.065,-0.06,-0.055,
-0.05,-0.045,-0.04,-0.035,-0.03,-0.025,-0.02,-0.015,-0.01,-0.005,0.),
 .UNSPECIFIED.)
CURVE()
GEOMETRIC_REPRESENTATION_ITEM()
RATIONAL_B_SPLINE_CURVE((1.,1.,1.,1.,1.,1.,1.,1.,1.,1.,1.,1.,1.,1.,1.,1.,
1.,1.,1.,1.,1.,1.,1.,1.,1.,1.,1.,1.,1.,1.,1.,1.,1.,1.,1.,1.,1.,1.,1.,1.,
1.,1.,1.,1.,1.,1.,1.,1.,1.,1.,1.,1.,1.,1.,1.,1.,1.,1.,1.,1.,1.,1.,1.,1.,
1.,1.,1.,1.,1.,1.,1.,1.,1.,1.,1.,1.,1.,1.,1.,1.,1.,1.,1.,1.,1.,1.,1.,1.,
1.,1.,1.,1.,1.,1.,1.,1.,1.,1.,1.,1.,1.,1.,1.,1.,1.,1.,1.,1.,1.,1.,1.,1.,
1.,1.,1.,1.,1.,1.,1.,1.,1.,1.,1.,1.,1.,1.,1.,1.,1.,1.,1.,1.,1.,1.,1.,1.,
1.,1.,1.,1.,1.,1.,1.,1.,1.,1.,1.,1.,1.,1.,1.,1.,1.,1.,1.,1.,1.,1.,1.,1.,
1.,1.,1.,1.,1.,1.,1.,1.,1.,1.,1.,1.,1.,1.,1.,1.,1.,1.,1.,1.,1.,1.,1.,1.,
1.,1.,1.,1.,1.,1.,1.,1.,1.,1.,1.,1.,1.,1.,1.,1.,1.,1.,1.,1.,1.))
REPRESENTATION_ITEM('')
);
#780=(
BOUNDED_CURVE()
B_SPLINE_CURVE(5,(#211393,#211394,#211395,#211396,#211397,#211398,#211399,
#211400,#211401,#211402,#211403,#211404,#211405,#211406,#211407,#211408,
#211409,#211410,#211411,#211412,#211413,#211414,#211415,#211416,#211417,
#211418,#211419,#211420,#211421,#211422,#211423,#211424,#211425,#211426,
#211427,#211428,#211429,#211430,#211431,#211432,#211433,#211434,#211435,
#211436,#211437,#211438,#211439,#211440,#211441,#211442,#211443,#211444,
#211445,#211446,#211447,#211448,#211449,#211450,#211451,#211452,#211453,
#211454,#211455,#211456,#211457,#211458,#211459,#211460,#211461,#211462,
#211463,#211464,#211465,#211466,#211467,#211468,#211469,#211470,#211471,
#211472,#211473,#211474,#211475,#211476,#211477,#211478,#211479,#211480,
#211481,#211482,#211483,#211484,#211485,#211486,#211487,#211488,#211489,
#211490,#211491,#211492,#211493,#211494,#211495,#211496,#211497,#211498,
#211499,#211500,#211501,#211502,#211503,#211504,#211505,#211506,#211507,
#211508,#211509,#211510,#211511,#211512,#211513,#211514,#211515,#211516,
#211517,#211518,#211519,#211520,#211521,#211522,#211523,#211524,#211525,
#211526,#211527,#211528,#211529,#211530,#211531,#211532,#211533,#211534,
#211535,#211536,#211537,#211538,#211539,#211540,#211541,#211542,#211543,
#211544,#211545,#211546,#211547,#211548,#211549,#211550,#211551,#211552,
#211553,#211554,#211555,#211556,#211557,#211558,#211559,#211560,#211561,
#211562,#211563,#211564,#211565,#211566,#211567,#211568,#211569,#211570,
#211571,#211572,#211573,#211574,#211575,#211576,#211577,#211578,#211579,
#211580,#211581,#211582,#211583,#211584,#211585,#211586,#211587,#211588,
#211589,#211590,#211591,#211592,#211593,#211594,#211595,#211596,#211597),
 .UNSPECIFIED.,.F.,.F.)
B_SPLINE_CURVE_WITH_KNOTS((6,1,1,1,1,1,1,1,1,1,1,1,1,1,1,1,1,1,1,1,1,1,
1,1,1,1,1,1,1,1,1,1,1,1,1,1,1,1,1,1,1,1,1,1,1,1,1,1,1,1,1,1,1,1,1,1,1,1,
1,1,1,1,1,1,1,1,1,1,1,1,1,1,1,1,1,1,1,1,1,1,1,1,1,1,1,1,1,1,1,1,1,1,1,1,
1,1,1,1,1,1,1,1,1,1,1,1,1,1,1,1,1,1,1,1,1,1,1,1,1,1,1,1,1,1,1,1,1,1,1,1,
1,1,1,1,1,1,1,1,1,1,1,1,1,1,1,1,1,1,1,1,1,1,1,1,1,1,1,1,1,1,1,1,1,1,1,1,
1,1,1,1,1,1,1,1,1,1,1,1,1,1,1,1,1,1,1,1,1,1,1,1,1,1,1,1,1,1,1,1,1,1,6),
(0.,0.005,0.01,0.015,0.02,0.025,0.03,0.035,0.04,0.045,0.05,0.055,0.06,0.065,
0.07,0.075,0.08,0.085,0.09,0.095,0.1,0.105,0.11,0.115,0.12,0.125,0.13,0.135,
0.14,0.145,0.15,0.155,0.16,0.165,0.17,0.175,0.18,0.185,0.19,0.195,0.2,0.205,
0.21,0.215,0.22,0.225,0.23,0.235,0.24,0.245,0.25,0.255,0.26,0.265,0.27,
0.275,0.28,0.285,0.29,0.295,0.3,0.305,0.31,0.315,0.32,0.325,0.33,0.335,
0.34,0.345,0.35,0.355,0.36,0.365,0.37,0.375,0.38,0.385,0.39,0.395,0.4,0.405,
0.41,0.415,0.42,0.425,0.43,0.435,0.44,0.445,0.45,0.455,0.46,0.465,0.47,
0.475,0.48,0.485,0.49,0.495,0.5,0.505,0.51,0.515,0.52,0.525,0.53,0.535,
0.54,0.545,0.55,0.555,0.56,0.565,0.57,0.575,0.58,0.585,0.59,0.595,0.6,0.605,
0.61,0.615,0.62,0.625,0.63,0.635,0.64,0.645,0.65,0.655,0.66,0.665,0.67,
0.675,0.68,0.685,0.690000000000001,0.695000000000001,0.700000000000001,
0.705000000000001,0.710000000000001,0.715000000000001,0.720000000000001,
0.725000000000001,0.730000000000001,0.735000000000001,0.740000000000001,
0.745000000000001,0.750000000000001,0.755000000000001,0.760000000000001,
0.765000000000001,0.770000000000001,0.775000000000001,0.780000000000001,
0.785000000000001,0.790000000000001,0.795000000000001,0.800000000000001,
0.805000000000001,0.810000000000001,0.815000000000001,0.820000000000001,
0.825000000000001,0.830000000000001,0.835000000000001,0.840000000000001,
0.845000000000001,0.850000000000001,0.855000000000001,0.860000000000001,
0.865000000000001,0.870000000000001,0.875000000000001,0.880000000000001,
0.885000000000001,0.890000000000001,0.895000000000001,0.900000000000001,
0.905000000000001,0.910000000000001,0.915000000000001,0.920000000000001,
0.925000000000001,0.930000000000001,0.935000000000001,0.940000000000001,
0.945000000000001,0.950000000000001,0.955000000000001,0.960000000000001,
0.965000000000001,0.970000000000001,0.975000000000001,0.980000000000001,
0.985000000000001,0.990000000000001,0.995000000000001,1.),.UNSPECIFIED.)
CURVE()
GEOMETRIC_REPRESENTATION_ITEM()
RATIONAL_B_SPLINE_CURVE((1.,1.,1.,1.,1.,1.,1.,1.,1.,1.,1.,1.,1.,1.,1.,1.,
1.,1.,1.,1.,1.,1.,1.,1.,1.,1.,1.,1.,1.,1.,1.,1.,1.,1.,1.,1.,1.,1.,1.,1.,
1.,1.,1.,1.,1.,1.,1.,1.,1.,1.,1.,1.,1.,1.,1.,1.,1.,1.,1.,1.,1.,1.,1.,1.,
1.,1.,1.,1.,1.,1.,1.,1.,1.,1.,1.,1.,1.,1.,1.,1.,1.,1.,1.,1.,1.,1.,1.,1.,
1.,1.,1.,1.,1.,1.,1.,1.,1.,1.,1.,1.,1.,1.,1.,1.,1.,1.,1.,1.,1.,1.,1.,1.,
1.,1.,1.,1.,1.,1.,1.,1.,1.,1.,1.,1.,1.,1.,1.,1.,1.,1.,1.,1.,1.,1.,1.,1.,
1.,1.,1.,1.,1.,1.,1.,1.,1.,1.,1.,1.,1.,1.,1.,1.,1.,1.,1.,1.,1.,1.,1.,1.,
1.,1.,1.,1.,1.,1.,1.,1.,1.,1.,1.,1.,1.,1.,1.,1.,1.,1.,1.,1.,1.,1.,1.,1.,
1.,1.,1.,1.,1.,1.,1.,1.,1.,1.,1.,1.,1.,1.,1.,1.,1.,1.,1.,1.,1.))
REPRESENTATION_ITEM('')
);
#781=(
BOUNDED_CURVE()
B_SPLINE_CURVE(5,(#212014,#212015,#212016,#212017,#212018,#212019,#212020,
#212021,#212022,#212023,#212024,#212025,#212026,#212027,#212028,#212029,
#212030,#212031,#212032,#212033,#212034,#212035,#212036,#212037,#212038,
#212039,#212040,#212041,#212042,#212043,#212044,#212045,#212046,#212047,
#212048,#212049,#212050,#212051,#212052,#212053,#212054,#212055,#212056,
#212057,#212058,#212059,#212060,#212061,#212062,#212063,#212064,#212065,
#212066,#212067,#212068,#212069,#212070,#212071,#212072,#212073,#212074,
#212075,#212076,#212077,#212078,#212079,#212080,#212081,#212082,#212083,
#212084,#212085,#212086,#212087,#212088,#212089,#212090,#212091,#212092,
#212093,#212094,#212095,#212096,#212097,#212098,#212099,#212100,#212101,
#212102,#212103,#212104,#212105,#212106,#212107,#212108,#212109,#212110,
#212111,#212112,#212113,#212114,#212115,#212116,#212117,#212118,#212119,
#212120,#212121,#212122,#212123,#212124,#212125,#212126,#212127,#212128,
#212129,#212130,#212131,#212132,#212133,#212134,#212135,#212136,#212137,
#212138,#212139,#212140,#212141,#212142,#212143,#212144,#212145,#212146,
#212147,#212148,#212149,#212150,#212151,#212152,#212153,#212154,#212155,
#212156,#212157,#212158,#212159,#212160,#212161,#212162,#212163,#212164,
#212165,#212166,#212167,#212168,#212169,#212170,#212171,#212172,#212173,
#212174,#212175,#212176,#212177,#212178,#212179,#212180,#212181,#212182,
#212183,#212184,#212185,#212186,#212187,#212188,#212189,#212190,#212191,
#212192,#212193,#212194,#212195,#212196,#212197,#212198,#212199,#212200,
#212201,#212202,#212203,#212204,#212205,#212206,#212207,#212208,#212209,
#212210,#212211,#212212,#212213,#212214,#212215,#212216,#212217,#212218),
 .UNSPECIFIED.,.F.,.F.)
B_SPLINE_CURVE_WITH_KNOTS((6,1,1,1,1,1,1,1,1,1,1,1,1,1,1,1,1,1,1,1,1,1,
1,1,1,1,1,1,1,1,1,1,1,1,1,1,1,1,1,1,1,1,1,1,1,1,1,1,1,1,1,1,1,1,1,1,1,1,
1,1,1,1,1,1,1,1,1,1,1,1,1,1,1,1,1,1,1,1,1,1,1,1,1,1,1,1,1,1,1,1,1,1,1,1,
1,1,1,1,1,1,1,1,1,1,1,1,1,1,1,1,1,1,1,1,1,1,1,1,1,1,1,1,1,1,1,1,1,1,1,1,
1,1,1,1,1,1,1,1,1,1,1,1,1,1,1,1,1,1,1,1,1,1,1,1,1,1,1,1,1,1,1,1,1,1,1,1,
1,1,1,1,1,1,1,1,1,1,1,1,1,1,1,1,1,1,1,1,1,1,1,1,1,1,1,1,1,1,1,1,1,1,6),
(-1.,-0.995000000000001,-0.990000000000001,-0.985000000000001,-0.980000000000001,
-0.975000000000001,-0.970000000000001,-0.965000000000001,-0.960000000000001,
-0.955000000000001,-0.950000000000001,-0.945000000000001,-0.940000000000001,
-0.935000000000001,-0.930000000000001,-0.925000000000001,-0.920000000000001,
-0.915000000000001,-0.910000000000001,-0.905000000000001,-0.900000000000001,
-0.895000000000001,-0.890000000000001,-0.885000000000001,-0.880000000000001,
-0.875000000000001,-0.870000000000001,-0.865000000000001,-0.860000000000001,
-0.855000000000001,-0.850000000000001,-0.845000000000001,-0.840000000000001,
-0.835000000000001,-0.830000000000001,-0.825000000000001,-0.820000000000001,
-0.815000000000001,-0.810000000000001,-0.805000000000001,-0.800000000000001,
-0.795000000000001,-0.790000000000001,-0.785000000000001,-0.780000000000001,
-0.775000000000001,-0.770000000000001,-0.765000000000001,-0.760000000000001,
-0.755000000000001,-0.750000000000001,-0.745000000000001,-0.740000000000001,
-0.735000000000001,-0.730000000000001,-0.725000000000001,-0.720000000000001,
-0.715000000000001,-0.710000000000001,-0.705000000000001,-0.700000000000001,
-0.695000000000001,-0.690000000000001,-0.685,-0.68,-0.675,-0.67,-0.665,
-0.66,-0.655,-0.65,-0.645,-0.64,-0.635,-0.63,-0.625,-0.62,-0.615,-0.61,
-0.605,-0.6,-0.595,-0.59,-0.585,-0.58,-0.575,-0.57,-0.565,-0.56,-0.555,
-0.55,-0.545,-0.54,-0.535,-0.53,-0.525,-0.52,-0.515,-0.51,-0.505,-0.5,-0.495,
-0.49,-0.485,-0.48,-0.475,-0.47,-0.465,-0.46,-0.455,-0.45,-0.445,-0.44,
-0.435,-0.43,-0.425,-0.42,-0.415,-0.41,-0.405,-0.4,-0.395,-0.39,-0.385,
-0.38,-0.375,-0.37,-0.365,-0.36,-0.355,-0.35,-0.345,-0.34,-0.335,-0.33,
-0.325,-0.32,-0.315,-0.31,-0.305,-0.3,-0.295,-0.29,-0.285,-0.28,-0.275,
-0.27,-0.265,-0.26,-0.255,-0.25,-0.245,-0.24,-0.235,-0.23,-0.225,-0.22,
-0.215,-0.21,-0.205,-0.2,-0.195,-0.19,-0.185,-0.18,-0.175,-0.17,-0.165,
-0.16,-0.155,-0.15,-0.145,-0.14,-0.135,-0.13,-0.125,-0.12,-0.115,-0.11,
-0.105,-0.1,-0.095,-0.09,-0.085,-0.08,-0.075,-0.07,-0.065,-0.06,-0.055,
-0.05,-0.045,-0.04,-0.035,-0.03,-0.025,-0.02,-0.015,-0.01,-0.005,0.),
 .UNSPECIFIED.)
CURVE()
GEOMETRIC_REPRESENTATION_ITEM()
RATIONAL_B_SPLINE_CURVE((1.,1.,1.,1.,1.,1.,1.,1.,1.,1.,1.,1.,1.,1.,1.,1.,
1.,1.,1.,1.,1.,1.,1.,1.,1.,1.,1.,1.,1.,1.,1.,1.,1.,1.,1.,1.,1.,1.,1.,1.,
1.,1.,1.,1.,1.,1.,1.,1.,1.,1.,1.,1.,1.,1.,1.,1.,1.,1.,1.,1.,1.,1.,1.,1.,
1.,1.,1.,1.,1.,1.,1.,1.,1.,1.,1.,1.,1.,1.,1.,1.,1.,1.,1.,1.,1.,1.,1.,1.,
1.,1.,1.,1.,1.,1.,1.,1.,1.,1.,1.,1.,1.,1.,1.,1.,1.,1.,1.,1.,1.,1.,1.,1.,
1.,1.,1.,1.,1.,1.,1.,1.,1.,1.,1.,1.,1.,1.,1.,1.,1.,1.,1.,1.,1.,1.,1.,1.,
1.,1.,1.,1.,1.,1.,1.,1.,1.,1.,1.,1.,1.,1.,1.,1.,1.,1.,1.,1.,1.,1.,1.,1.,
1.,1.,1.,1.,1.,1.,1.,1.,1.,1.,1.,1.,1.,1.,1.,1.,1.,1.,1.,1.,1.,1.,1.,1.,
1.,1.,1.,1.,1.,1.,1.,1.,1.,1.,1.,1.,1.,1.,1.,1.,1.,1.,1.,1.,1.))
REPRESENTATION_ITEM('')
);
#782=(
BOUNDED_CURVE()
B_SPLINE_CURVE(5,(#212631,#212632,#212633,#212634,#212635,#212636,#212637,
#212638,#212639,#212640,#212641,#212642,#212643,#212644,#212645,#212646,
#212647,#212648,#212649,#212650,#212651,#212652,#212653,#212654,#212655,
#212656,#212657,#212658,#212659,#212660,#212661,#212662,#212663,#212664,
#212665,#212666,#212667,#212668,#212669,#212670,#212671,#212672,#212673,
#212674,#212675,#212676,#212677,#212678,#212679,#212680,#212681,#212682,
#212683,#212684,#212685,#212686,#212687,#212688,#212689,#212690,#212691,
#212692,#212693,#212694,#212695,#212696,#212697,#212698,#212699,#212700,
#212701,#212702,#212703,#212704,#212705,#212706,#212707,#212708,#212709,
#212710,#212711,#212712,#212713,#212714,#212715,#212716,#212717,#212718,
#212719,#212720,#212721,#212722,#212723,#212724,#212725,#212726,#212727,
#212728,#212729,#212730,#212731,#212732,#212733,#212734,#212735,#212736,
#212737,#212738,#212739,#212740,#212741,#212742,#212743,#212744,#212745,
#212746,#212747,#212748,#212749,#212750,#212751,#212752,#212753,#212754,
#212755,#212756,#212757,#212758,#212759,#212760,#212761,#212762,#212763,
#212764,#212765,#212766,#212767,#212768,#212769,#212770,#212771,#212772,
#212773,#212774,#212775,#212776,#212777,#212778,#212779,#212780,#212781,
#212782,#212783,#212784,#212785,#212786,#212787,#212788,#212789,#212790,
#212791,#212792,#212793,#212794,#212795,#212796,#212797,#212798,#212799,
#212800,#212801,#212802,#212803,#212804,#212805,#212806,#212807,#212808,
#212809,#212810,#212811,#212812,#212813,#212814,#212815,#212816,#212817,
#212818,#212819,#212820,#212821,#212822,#212823,#212824,#212825,#212826,
#212827,#212828,#212829,#212830,#212831,#212832,#212833,#212834,#212835),
 .UNSPECIFIED.,.F.,.F.)
B_SPLINE_CURVE_WITH_KNOTS((6,1,1,1,1,1,1,1,1,1,1,1,1,1,1,1,1,1,1,1,1,1,
1,1,1,1,1,1,1,1,1,1,1,1,1,1,1,1,1,1,1,1,1,1,1,1,1,1,1,1,1,1,1,1,1,1,1,1,
1,1,1,1,1,1,1,1,1,1,1,1,1,1,1,1,1,1,1,1,1,1,1,1,1,1,1,1,1,1,1,1,1,1,1,1,
1,1,1,1,1,1,1,1,1,1,1,1,1,1,1,1,1,1,1,1,1,1,1,1,1,1,1,1,1,1,1,1,1,1,1,1,
1,1,1,1,1,1,1,1,1,1,1,1,1,1,1,1,1,1,1,1,1,1,1,1,1,1,1,1,1,1,1,1,1,1,1,1,
1,1,1,1,1,1,1,1,1,1,1,1,1,1,1,1,1,1,1,1,1,1,1,1,1,1,1,1,1,1,1,1,1,1,6),
(0.,0.005,0.01,0.015,0.02,0.025,0.03,0.035,0.04,0.045,0.05,0.055,0.06,0.065,
0.07,0.075,0.08,0.085,0.09,0.095,0.1,0.105,0.11,0.115,0.12,0.125,0.13,0.135,
0.14,0.145,0.15,0.155,0.16,0.165,0.17,0.175,0.18,0.185,0.19,0.195,0.2,0.205,
0.21,0.215,0.22,0.225,0.23,0.235,0.24,0.245,0.25,0.255,0.26,0.265,0.27,
0.275,0.28,0.285,0.29,0.295,0.3,0.305,0.31,0.315,0.32,0.325,0.33,0.335,
0.34,0.345,0.35,0.355,0.36,0.365,0.37,0.375,0.38,0.385,0.39,0.395,0.4,0.405,
0.41,0.415,0.42,0.425,0.43,0.435,0.44,0.445,0.45,0.455,0.46,0.465,0.47,
0.475,0.48,0.485,0.49,0.495,0.5,0.505,0.51,0.515,0.52,0.525,0.53,0.535,
0.54,0.545,0.55,0.555,0.56,0.565,0.57,0.575,0.58,0.585,0.59,0.595,0.6,0.605,
0.61,0.615,0.62,0.625,0.63,0.635,0.64,0.645,0.65,0.655,0.66,0.665,0.67,
0.675,0.68,0.685,0.690000000000001,0.695000000000001,0.700000000000001,
0.705000000000001,0.710000000000001,0.715000000000001,0.720000000000001,
0.725000000000001,0.730000000000001,0.735000000000001,0.740000000000001,
0.745000000000001,0.750000000000001,0.755000000000001,0.760000000000001,
0.765000000000001,0.770000000000001,0.775000000000001,0.780000000000001,
0.785000000000001,0.790000000000001,0.795000000000001,0.800000000000001,
0.805000000000001,0.810000000000001,0.815000000000001,0.820000000000001,
0.825000000000001,0.830000000000001,0.835000000000001,0.840000000000001,
0.845000000000001,0.850000000000001,0.855000000000001,0.860000000000001,
0.865000000000001,0.870000000000001,0.875000000000001,0.880000000000001,
0.885000000000001,0.890000000000001,0.895000000000001,0.900000000000001,
0.905000000000001,0.910000000000001,0.915000000000001,0.920000000000001,
0.925000000000001,0.930000000000001,0.935000000000001,0.940000000000001,
0.945000000000001,0.950000000000001,0.955000000000001,0.960000000000001,
0.965000000000001,0.970000000000001,0.975000000000001,0.980000000000001,
0.985000000000001,0.990000000000001,0.995000000000001,1.),.UNSPECIFIED.)
CURVE()
GEOMETRIC_REPRESENTATION_ITEM()
RATIONAL_B_SPLINE_CURVE((1.,1.,1.,1.,1.,1.,1.,1.,1.,1.,1.,1.,1.,1.,1.,1.,
1.,1.,1.,1.,1.,1.,1.,1.,1.,1.,1.,1.,1.,1.,1.,1.,1.,1.,1.,1.,1.,1.,1.,1.,
1.,1.,1.,1.,1.,1.,1.,1.,1.,1.,1.,1.,1.,1.,1.,1.,1.,1.,1.,1.,1.,1.,1.,1.,
1.,1.,1.,1.,1.,1.,1.,1.,1.,1.,1.,1.,1.,1.,1.,1.,1.,1.,1.,1.,1.,1.,1.,1.,
1.,1.,1.,1.,1.,1.,1.,1.,1.,1.,1.,1.,1.,1.,1.,1.,1.,1.,1.,1.,1.,1.,1.,1.,
1.,1.,1.,1.,1.,1.,1.,1.,1.,1.,1.,1.,1.,1.,1.,1.,1.,1.,1.,1.,1.,1.,1.,1.,
1.,1.,1.,1.,1.,1.,1.,1.,1.,1.,1.,1.,1.,1.,1.,1.,1.,1.,1.,1.,1.,1.,1.,1.,
1.,1.,1.,1.,1.,1.,1.,1.,1.,1.,1.,1.,1.,1.,1.,1.,1.,1.,1.,1.,1.,1.,1.,1.,
1.,1.,1.,1.,1.,1.,1.,1.,1.,1.,1.,1.,1.,1.,1.,1.,1.,1.,1.,1.,1.))
REPRESENTATION_ITEM('')
);
#783=(
BOUNDED_CURVE()
B_SPLINE_CURVE(5,(#213252,#213253,#213254,#213255,#213256,#213257,#213258,
#213259,#213260,#213261,#213262,#213263,#213264,#213265,#213266,#213267,
#213268,#213269,#213270,#213271,#213272,#213273,#213274,#213275,#213276,
#213277,#213278,#213279,#213280,#213281,#213282,#213283,#213284,#213285,
#213286,#213287,#213288,#213289,#213290,#213291,#213292,#213293,#213294,
#213295,#213296,#213297,#213298,#213299,#213300,#213301,#213302,#213303,
#213304,#213305,#213306,#213307,#213308,#213309,#213310,#213311,#213312,
#213313,#213314,#213315,#213316,#213317,#213318,#213319,#213320,#213321,
#213322,#213323,#213324,#213325,#213326,#213327,#213328,#213329,#213330,
#213331,#213332,#213333,#213334,#213335,#213336,#213337,#213338,#213339,
#213340,#213341,#213342,#213343,#213344,#213345,#213346,#213347,#213348,
#213349,#213350,#213351,#213352,#213353,#213354,#213355,#213356,#213357,
#213358,#213359,#213360,#213361,#213362,#213363,#213364,#213365,#213366,
#213367,#213368,#213369,#213370,#213371,#213372,#213373,#213374,#213375,
#213376,#213377,#213378,#213379,#213380,#213381,#213382,#213383,#213384,
#213385,#213386,#213387,#213388,#213389,#213390,#213391,#213392,#213393,
#213394,#213395,#213396,#213397,#213398,#213399,#213400,#213401,#213402,
#213403,#213404,#213405,#213406,#213407,#213408,#213409,#213410,#213411,
#213412,#213413,#213414,#213415,#213416,#213417,#213418,#213419,#213420,
#213421,#213422,#213423,#213424,#213425,#213426,#213427,#213428,#213429,
#213430,#213431,#213432,#213433,#213434,#213435,#213436,#213437,#213438,
#213439,#213440,#213441,#213442,#213443,#213444,#213445,#213446,#213447,
#213448,#213449,#213450,#213451,#213452,#213453,#213454,#213455,#213456),
 .UNSPECIFIED.,.F.,.F.)
B_SPLINE_CURVE_WITH_KNOTS((6,1,1,1,1,1,1,1,1,1,1,1,1,1,1,1,1,1,1,1,1,1,
1,1,1,1,1,1,1,1,1,1,1,1,1,1,1,1,1,1,1,1,1,1,1,1,1,1,1,1,1,1,1,1,1,1,1,1,
1,1,1,1,1,1,1,1,1,1,1,1,1,1,1,1,1,1,1,1,1,1,1,1,1,1,1,1,1,1,1,1,1,1,1,1,
1,1,1,1,1,1,1,1,1,1,1,1,1,1,1,1,1,1,1,1,1,1,1,1,1,1,1,1,1,1,1,1,1,1,1,1,
1,1,1,1,1,1,1,1,1,1,1,1,1,1,1,1,1,1,1,1,1,1,1,1,1,1,1,1,1,1,1,1,1,1,1,1,
1,1,1,1,1,1,1,1,1,1,1,1,1,1,1,1,1,1,1,1,1,1,1,1,1,1,1,1,1,1,1,1,1,1,6),
(-1.,-0.995000000000001,-0.990000000000001,-0.985000000000001,-0.980000000000001,
-0.975000000000001,-0.970000000000001,-0.965000000000001,-0.960000000000001,
-0.955000000000001,-0.950000000000001,-0.945000000000001,-0.940000000000001,
-0.935000000000001,-0.930000000000001,-0.925000000000001,-0.920000000000001,
-0.915000000000001,-0.910000000000001,-0.905000000000001,-0.900000000000001,
-0.895000000000001,-0.890000000000001,-0.885000000000001,-0.880000000000001,
-0.875000000000001,-0.870000000000001,-0.865000000000001,-0.860000000000001,
-0.855000000000001,-0.850000000000001,-0.845000000000001,-0.840000000000001,
-0.835000000000001,-0.830000000000001,-0.825000000000001,-0.820000000000001,
-0.815000000000001,-0.810000000000001,-0.805000000000001,-0.800000000000001,
-0.795000000000001,-0.790000000000001,-0.785000000000001,-0.780000000000001,
-0.775000000000001,-0.770000000000001,-0.765000000000001,-0.760000000000001,
-0.755000000000001,-0.750000000000001,-0.745000000000001,-0.740000000000001,
-0.735000000000001,-0.730000000000001,-0.725000000000001,-0.720000000000001,
-0.715000000000001,-0.710000000000001,-0.705000000000001,-0.700000000000001,
-0.695000000000001,-0.690000000000001,-0.685,-0.68,-0.675,-0.67,-0.665,
-0.66,-0.655,-0.65,-0.645,-0.64,-0.635,-0.63,-0.625,-0.62,-0.615,-0.61,
-0.605,-0.6,-0.595,-0.59,-0.585,-0.58,-0.575,-0.57,-0.565,-0.56,-0.555,
-0.55,-0.545,-0.54,-0.535,-0.53,-0.525,-0.52,-0.515,-0.51,-0.505,-0.5,-0.495,
-0.49,-0.485,-0.48,-0.475,-0.47,-0.465,-0.46,-0.455,-0.45,-0.445,-0.44,
-0.435,-0.43,-0.425,-0.42,-0.415,-0.41,-0.405,-0.4,-0.395,-0.39,-0.385,
-0.38,-0.375,-0.37,-0.365,-0.36,-0.355,-0.35,-0.345,-0.34,-0.335,-0.33,
-0.325,-0.32,-0.315,-0.31,-0.305,-0.3,-0.295,-0.29,-0.285,-0.28,-0.275,
-0.27,-0.265,-0.26,-0.255,-0.25,-0.245,-0.24,-0.235,-0.23,-0.225,-0.22,
-0.215,-0.21,-0.205,-0.2,-0.195,-0.19,-0.185,-0.18,-0.175,-0.17,-0.165,
-0.16,-0.155,-0.15,-0.145,-0.14,-0.135,-0.13,-0.125,-0.12,-0.115,-0.11,
-0.105,-0.1,-0.095,-0.09,-0.085,-0.08,-0.075,-0.07,-0.065,-0.06,-0.055,
-0.05,-0.045,-0.04,-0.035,-0.03,-0.025,-0.02,-0.015,-0.01,-0.005,0.),
 .UNSPECIFIED.)
CURVE()
GEOMETRIC_REPRESENTATION_ITEM()
RATIONAL_B_SPLINE_CURVE((1.,1.,1.,1.,1.,1.,1.,1.,1.,1.,1.,1.,1.,1.,1.,1.,
1.,1.,1.,1.,1.,1.,1.,1.,1.,1.,1.,1.,1.,1.,1.,1.,1.,1.,1.,1.,1.,1.,1.,1.,
1.,1.,1.,1.,1.,1.,1.,1.,1.,1.,1.,1.,1.,1.,1.,1.,1.,1.,1.,1.,1.,1.,1.,1.,
1.,1.,1.,1.,1.,1.,1.,1.,1.,1.,1.,1.,1.,1.,1.,1.,1.,1.,1.,1.,1.,1.,1.,1.,
1.,1.,1.,1.,1.,1.,1.,1.,1.,1.,1.,1.,1.,1.,1.,1.,1.,1.,1.,1.,1.,1.,1.,1.,
1.,1.,1.,1.,1.,1.,1.,1.,1.,1.,1.,1.,1.,1.,1.,1.,1.,1.,1.,1.,1.,1.,1.,1.,
1.,1.,1.,1.,1.,1.,1.,1.,1.,1.,1.,1.,1.,1.,1.,1.,1.,1.,1.,1.,1.,1.,1.,1.,
1.,1.,1.,1.,1.,1.,1.,1.,1.,1.,1.,1.,1.,1.,1.,1.,1.,1.,1.,1.,1.,1.,1.,1.,
1.,1.,1.,1.,1.,1.,1.,1.,1.,1.,1.,1.,1.,1.,1.,1.,1.,1.,1.,1.,1.))
REPRESENTATION_ITEM('')
);
#784=(
BOUNDED_CURVE()
B_SPLINE_CURVE(5,(#213869,#213870,#213871,#213872,#213873,#213874,#213875,
#213876,#213877,#213878,#213879,#213880,#213881,#213882,#213883,#213884,
#213885,#213886,#213887,#213888,#213889,#213890,#213891,#213892,#213893,
#213894,#213895,#213896,#213897,#213898,#213899,#213900,#213901,#213902,
#213903,#213904,#213905,#213906,#213907,#213908,#213909,#213910,#213911,
#213912,#213913,#213914,#213915,#213916,#213917,#213918,#213919,#213920,
#213921,#213922,#213923,#213924,#213925,#213926,#213927,#213928,#213929,
#213930,#213931,#213932,#213933,#213934,#213935,#213936,#213937,#213938,
#213939,#213940,#213941,#213942,#213943,#213944,#213945,#213946,#213947,
#213948,#213949,#213950,#213951,#213952,#213953,#213954,#213955,#213956,
#213957,#213958,#213959,#213960,#213961,#213962,#213963,#213964,#213965,
#213966,#213967,#213968,#213969,#213970,#213971,#213972,#213973,#213974,
#213975,#213976,#213977,#213978,#213979,#213980,#213981,#213982,#213983,
#213984,#213985,#213986,#213987,#213988,#213989,#213990,#213991,#213992,
#213993,#213994,#213995,#213996,#213997,#213998,#213999,#214000,#214001,
#214002,#214003,#214004,#214005,#214006,#214007,#214008,#214009,#214010,
#214011,#214012,#214013,#214014,#214015,#214016,#214017,#214018,#214019,
#214020,#214021,#214022,#214023,#214024,#214025,#214026,#214027,#214028,
#214029,#214030,#214031,#214032,#214033,#214034,#214035,#214036,#214037,
#214038,#214039,#214040,#214041,#214042,#214043,#214044,#214045,#214046,
#214047,#214048,#214049,#214050,#214051,#214052,#214053,#214054,#214055,
#214056,#214057,#214058,#214059,#214060,#214061,#214062,#214063,#214064,
#214065,#214066,#214067,#214068,#214069,#214070,#214071,#214072,#214073),
 .UNSPECIFIED.,.F.,.F.)
B_SPLINE_CURVE_WITH_KNOTS((6,1,1,1,1,1,1,1,1,1,1,1,1,1,1,1,1,1,1,1,1,1,
1,1,1,1,1,1,1,1,1,1,1,1,1,1,1,1,1,1,1,1,1,1,1,1,1,1,1,1,1,1,1,1,1,1,1,1,
1,1,1,1,1,1,1,1,1,1,1,1,1,1,1,1,1,1,1,1,1,1,1,1,1,1,1,1,1,1,1,1,1,1,1,1,
1,1,1,1,1,1,1,1,1,1,1,1,1,1,1,1,1,1,1,1,1,1,1,1,1,1,1,1,1,1,1,1,1,1,1,1,
1,1,1,1,1,1,1,1,1,1,1,1,1,1,1,1,1,1,1,1,1,1,1,1,1,1,1,1,1,1,1,1,1,1,1,1,
1,1,1,1,1,1,1,1,1,1,1,1,1,1,1,1,1,1,1,1,1,1,1,1,1,1,1,1,1,1,1,1,1,1,6),
(0.,0.005,0.01,0.015,0.02,0.025,0.03,0.035,0.04,0.045,0.05,0.055,0.06,0.065,
0.07,0.075,0.08,0.085,0.09,0.095,0.1,0.105,0.11,0.115,0.12,0.125,0.13,0.135,
0.14,0.145,0.15,0.155,0.16,0.165,0.17,0.175,0.18,0.185,0.19,0.195,0.2,0.205,
0.21,0.215,0.22,0.225,0.23,0.235,0.24,0.245,0.25,0.255,0.26,0.265,0.27,
0.275,0.28,0.285,0.29,0.295,0.3,0.305,0.31,0.315,0.32,0.325,0.33,0.335,
0.34,0.345,0.35,0.355,0.36,0.365,0.37,0.375,0.38,0.385,0.39,0.395,0.4,0.405,
0.41,0.415,0.42,0.425,0.43,0.435,0.44,0.445,0.45,0.455,0.46,0.465,0.47,
0.475,0.48,0.485,0.49,0.495,0.5,0.505,0.51,0.515,0.52,0.525,0.53,0.535,
0.54,0.545,0.55,0.555,0.56,0.565,0.57,0.575,0.58,0.585,0.59,0.595,0.6,0.605,
0.61,0.615,0.62,0.625,0.63,0.635,0.64,0.645,0.65,0.655,0.66,0.665,0.67,
0.675,0.68,0.685,0.690000000000001,0.695000000000001,0.700000000000001,
0.705000000000001,0.710000000000001,0.715000000000001,0.720000000000001,
0.725000000000001,0.730000000000001,0.735000000000001,0.740000000000001,
0.745000000000001,0.750000000000001,0.755000000000001,0.760000000000001,
0.765000000000001,0.770000000000001,0.775000000000001,0.780000000000001,
0.785000000000001,0.790000000000001,0.795000000000001,0.800000000000001,
0.805000000000001,0.810000000000001,0.815000000000001,0.820000000000001,
0.825000000000001,0.830000000000001,0.835000000000001,0.840000000000001,
0.845000000000001,0.850000000000001,0.855000000000001,0.860000000000001,
0.865000000000001,0.870000000000001,0.875000000000001,0.880000000000001,
0.885000000000001,0.890000000000001,0.895000000000001,0.900000000000001,
0.905000000000001,0.910000000000001,0.915000000000001,0.920000000000001,
0.925000000000001,0.930000000000001,0.935000000000001,0.940000000000001,
0.945000000000001,0.950000000000001,0.955000000000001,0.960000000000001,
0.965000000000001,0.970000000000001,0.975000000000001,0.980000000000001,
0.985000000000001,0.990000000000001,0.995000000000001,1.),.UNSPECIFIED.)
CURVE()
GEOMETRIC_REPRESENTATION_ITEM()
RATIONAL_B_SPLINE_CURVE((1.,1.,1.,1.,1.,1.,1.,1.,1.,1.,1.,1.,1.,1.,1.,1.,
1.,1.,1.,1.,1.,1.,1.,1.,1.,1.,1.,1.,1.,1.,1.,1.,1.,1.,1.,1.,1.,1.,1.,1.,
1.,1.,1.,1.,1.,1.,1.,1.,1.,1.,1.,1.,1.,1.,1.,1.,1.,1.,1.,1.,1.,1.,1.,1.,
1.,1.,1.,1.,1.,1.,1.,1.,1.,1.,1.,1.,1.,1.,1.,1.,1.,1.,1.,1.,1.,1.,1.,1.,
1.,1.,1.,1.,1.,1.,1.,1.,1.,1.,1.,1.,1.,1.,1.,1.,1.,1.,1.,1.,1.,1.,1.,1.,
1.,1.,1.,1.,1.,1.,1.,1.,1.,1.,1.,1.,1.,1.,1.,1.,1.,1.,1.,1.,1.,1.,1.,1.,
1.,1.,1.,1.,1.,1.,1.,1.,1.,1.,1.,1.,1.,1.,1.,1.,1.,1.,1.,1.,1.,1.,1.,1.,
1.,1.,1.,1.,1.,1.,1.,1.,1.,1.,1.,1.,1.,1.,1.,1.,1.,1.,1.,1.,1.,1.,1.,1.,
1.,1.,1.,1.,1.,1.,1.,1.,1.,1.,1.,1.,1.,1.,1.,1.,1.,1.,1.,1.,1.))
REPRESENTATION_ITEM('')
);
#785=(
BOUNDED_CURVE()
B_SPLINE_CURVE(5,(#214101,#214102,#214103,#214104,#214105,#214106,#214107,
#214108,#214109,#214110,#214111,#214112,#214113,#214114,#214115,#214116,
#214117,#214118,#214119,#214120,#214121,#214122,#214123,#214124,#214125,
#214126,#214127,#214128,#214129,#214130,#214131,#214132,#214133,#214134,
#214135,#214136,#214137,#214138,#214139,#214140,#214141,#214142,#214143,
#214144,#214145,#214146,#214147,#214148,#214149,#214150,#214151,#214152,
#214153,#214154,#214155,#214156,#214157,#214158,#214159,#214160,#214161,
#214162,#214163,#214164,#214165,#214166,#214167,#214168,#214169,#214170,
#214171,#214172,#214173,#214174,#214175,#214176,#214177,#214178,#214179,
#214180,#214181,#214182,#214183,#214184,#214185,#214186,#214187,#214188,
#214189,#214190,#214191,#214192,#214193,#214194,#214195,#214196,#214197,
#214198,#214199,#214200,#214201,#214202,#214203,#214204,#214205,#214206,
#214207,#214208,#214209,#214210,#214211,#214212,#214213,#214214,#214215,
#214216,#214217,#214218,#214219,#214220,#214221,#214222,#214223,#214224,
#214225,#214226,#214227,#214228,#214229,#214230,#214231,#214232,#214233,
#214234,#214235,#214236,#214237,#214238,#214239,#214240,#214241,#214242,
#214243,#214244,#214245,#214246,#214247,#214248,#214249,#214250,#214251,
#214252,#214253,#214254,#214255,#214256,#214257,#214258,#214259,#214260,
#214261,#214262,#214263,#214264,#214265,#214266,#214267,#214268,#214269,
#214270,#214271,#214272,#214273,#214274,#214275,#214276,#214277,#214278,
#214279,#214280,#214281,#214282,#214283,#214284,#214285,#214286,#214287,
#214288,#214289,#214290,#214291,#214292,#214293,#214294,#214295,#214296,
#214297,#214298,#214299,#214300,#214301,#214302,#214303,#214304,#214305),
 .UNSPECIFIED.,.F.,.F.)
B_SPLINE_CURVE_WITH_KNOTS((6,1,1,1,1,1,1,1,1,1,1,1,1,1,1,1,1,1,1,1,1,1,
1,1,1,1,1,1,1,1,1,1,1,1,1,1,1,1,1,1,1,1,1,1,1,1,1,1,1,1,1,1,1,1,1,1,1,1,
1,1,1,1,1,1,1,1,1,1,1,1,1,1,1,1,1,1,1,1,1,1,1,1,1,1,1,1,1,1,1,1,1,1,1,1,
1,1,1,1,1,1,1,1,1,1,1,1,1,1,1,1,1,1,1,1,1,1,1,1,1,1,1,1,1,1,1,1,1,1,1,1,
1,1,1,1,1,1,1,1,1,1,1,1,1,1,1,1,1,1,1,1,1,1,1,1,1,1,1,1,1,1,1,1,1,1,1,1,
1,1,1,1,1,1,1,1,1,1,1,1,1,1,1,1,1,1,1,1,1,1,1,1,1,1,1,1,1,1,1,1,1,1,6),
(-1.,-0.995000000000001,-0.990000000000001,-0.985000000000001,-0.980000000000001,
-0.975000000000001,-0.970000000000001,-0.965000000000001,-0.960000000000001,
-0.955000000000001,-0.950000000000001,-0.945000000000001,-0.940000000000001,
-0.935000000000001,-0.930000000000001,-0.925000000000001,-0.920000000000001,
-0.915000000000001,-0.910000000000001,-0.905000000000001,-0.900000000000001,
-0.895000000000001,-0.890000000000001,-0.885000000000001,-0.880000000000001,
-0.875000000000001,-0.870000000000001,-0.865000000000001,-0.860000000000001,
-0.855000000000001,-0.850000000000001,-0.845000000000001,-0.840000000000001,
-0.835000000000001,-0.830000000000001,-0.825000000000001,-0.820000000000001,
-0.815000000000001,-0.810000000000001,-0.805000000000001,-0.800000000000001,
-0.795000000000001,-0.790000000000001,-0.785000000000001,-0.780000000000001,
-0.775000000000001,-0.770000000000001,-0.765000000000001,-0.760000000000001,
-0.755000000000001,-0.750000000000001,-0.745000000000001,-0.740000000000001,
-0.735000000000001,-0.730000000000001,-0.725000000000001,-0.720000000000001,
-0.715000000000001,-0.710000000000001,-0.705000000000001,-0.700000000000001,
-0.695000000000001,-0.690000000000001,-0.685,-0.68,-0.675,-0.67,-0.665,
-0.66,-0.655,-0.65,-0.645,-0.64,-0.635,-0.63,-0.625,-0.62,-0.615,-0.61,
-0.605,-0.6,-0.595,-0.59,-0.585,-0.58,-0.575,-0.57,-0.565,-0.56,-0.555,
-0.55,-0.545,-0.54,-0.535,-0.53,-0.525,-0.52,-0.515,-0.51,-0.505,-0.5,-0.495,
-0.49,-0.485,-0.48,-0.475,-0.47,-0.465,-0.46,-0.455,-0.45,-0.445,-0.44,
-0.435,-0.43,-0.425,-0.42,-0.415,-0.41,-0.405,-0.4,-0.395,-0.39,-0.385,
-0.38,-0.375,-0.37,-0.365,-0.36,-0.355,-0.35,-0.345,-0.34,-0.335,-0.33,
-0.325,-0.32,-0.315,-0.31,-0.305,-0.3,-0.295,-0.29,-0.285,-0.28,-0.275,
-0.27,-0.265,-0.26,-0.255,-0.25,-0.245,-0.24,-0.235,-0.23,-0.225,-0.22,
-0.215,-0.21,-0.205,-0.2,-0.195,-0.19,-0.185,-0.18,-0.175,-0.17,-0.165,
-0.16,-0.155,-0.15,-0.145,-0.14,-0.135,-0.13,-0.125,-0.12,-0.115,-0.11,
-0.105,-0.1,-0.095,-0.09,-0.085,-0.08,-0.075,-0.07,-0.065,-0.06,-0.055,
-0.05,-0.045,-0.04,-0.035,-0.03,-0.025,-0.02,-0.015,-0.01,-0.005,0.),
 .UNSPECIFIED.)
CURVE()
GEOMETRIC_REPRESENTATION_ITEM()
RATIONAL_B_SPLINE_CURVE((1.,1.,1.,1.,1.,1.,1.,1.,1.,1.,1.,1.,1.,1.,1.,1.,
1.,1.,1.,1.,1.,1.,1.,1.,1.,1.,1.,1.,1.,1.,1.,1.,1.,1.,1.,1.,1.,1.,1.,1.,
1.,1.,1.,1.,1.,1.,1.,1.,1.,1.,1.,1.,1.,1.,1.,1.,1.,1.,1.,1.,1.,1.,1.,1.,
1.,1.,1.,1.,1.,1.,1.,1.,1.,1.,1.,1.,1.,1.,1.,1.,1.,1.,1.,1.,1.,1.,1.,1.,
1.,1.,1.,1.,1.,1.,1.,1.,1.,1.,1.,1.,1.,1.,1.,1.,1.,1.,1.,1.,1.,1.,1.,1.,
1.,1.,1.,1.,1.,1.,1.,1.,1.,1.,1.,1.,1.,1.,1.,1.,1.,1.,1.,1.,1.,1.,1.,1.,
1.,1.,1.,1.,1.,1.,1.,1.,1.,1.,1.,1.,1.,1.,1.,1.,1.,1.,1.,1.,1.,1.,1.,1.,
1.,1.,1.,1.,1.,1.,1.,1.,1.,1.,1.,1.,1.,1.,1.,1.,1.,1.,1.,1.,1.,1.,1.,1.,
1.,1.,1.,1.,1.,1.,1.,1.,1.,1.,1.,1.,1.,1.,1.,1.,1.,1.,1.,1.,1.))
REPRESENTATION_ITEM('')
);
#786=(
BOUNDED_CURVE()
B_SPLINE_CURVE(5,(#214317,#214318,#214319,#214320,#214321,#214322,#214323,
#214324,#214325,#214326,#214327,#214328,#214329,#214330,#214331,#214332,
#214333,#214334,#214335,#214336,#214337,#214338,#214339,#214340,#214341,
#214342,#214343,#214344,#214345,#214346,#214347,#214348,#214349,#214350,
#214351,#214352,#214353,#214354,#214355,#214356,#214357,#214358,#214359,
#214360,#214361,#214362,#214363,#214364,#214365,#214366,#214367,#214368,
#214369,#214370,#214371,#214372,#214373,#214374,#214375,#214376,#214377,
#214378,#214379,#214380,#214381,#214382,#214383,#214384,#214385,#214386,
#214387,#214388,#214389,#214390,#214391,#214392,#214393,#214394,#214395,
#214396,#214397,#214398,#214399,#214400,#214401,#214402,#214403,#214404,
#214405,#214406,#214407,#214408,#214409,#214410,#214411,#214412,#214413,
#214414,#214415,#214416,#214417,#214418,#214419,#214420,#214421,#214422,
#214423,#214424,#214425,#214426,#214427,#214428,#214429,#214430,#214431,
#214432,#214433,#214434,#214435,#214436,#214437,#214438,#214439,#214440,
#214441,#214442,#214443,#214444,#214445,#214446,#214447,#214448,#214449,
#214450,#214451,#214452,#214453,#214454,#214455,#214456,#214457,#214458,
#214459,#214460,#214461,#214462,#214463,#214464,#214465,#214466,#214467,
#214468,#214469,#214470,#214471,#214472,#214473,#214474,#214475,#214476,
#214477,#214478,#214479,#214480,#214481,#214482,#214483,#214484,#214485,
#214486,#214487,#214488,#214489,#214490,#214491,#214492,#214493,#214494,
#214495,#214496,#214497,#214498,#214499,#214500,#214501,#214502,#214503,
#214504,#214505,#214506,#214507,#214508,#214509,#214510,#214511,#214512,
#214513,#214514,#214515,#214516,#214517,#214518,#214519,#214520,#214521),
 .UNSPECIFIED.,.F.,.F.)
B_SPLINE_CURVE_WITH_KNOTS((6,1,1,1,1,1,1,1,1,1,1,1,1,1,1,1,1,1,1,1,1,1,
1,1,1,1,1,1,1,1,1,1,1,1,1,1,1,1,1,1,1,1,1,1,1,1,1,1,1,1,1,1,1,1,1,1,1,1,
1,1,1,1,1,1,1,1,1,1,1,1,1,1,1,1,1,1,1,1,1,1,1,1,1,1,1,1,1,1,1,1,1,1,1,1,
1,1,1,1,1,1,1,1,1,1,1,1,1,1,1,1,1,1,1,1,1,1,1,1,1,1,1,1,1,1,1,1,1,1,1,1,
1,1,1,1,1,1,1,1,1,1,1,1,1,1,1,1,1,1,1,1,1,1,1,1,1,1,1,1,1,1,1,1,1,1,1,1,
1,1,1,1,1,1,1,1,1,1,1,1,1,1,1,1,1,1,1,1,1,1,1,1,1,1,1,1,1,1,1,1,1,1,6),
(0.,0.005,0.01,0.015,0.02,0.025,0.03,0.035,0.04,0.045,0.05,0.055,0.06,0.065,
0.07,0.075,0.08,0.085,0.09,0.095,0.1,0.105,0.11,0.115,0.12,0.125,0.13,0.135,
0.14,0.145,0.15,0.155,0.16,0.165,0.17,0.175,0.18,0.185,0.19,0.195,0.2,0.205,
0.21,0.215,0.22,0.225,0.23,0.235,0.24,0.245,0.25,0.255,0.26,0.265,0.27,
0.275,0.28,0.285,0.29,0.295,0.3,0.305,0.31,0.315,0.32,0.325,0.33,0.335,
0.34,0.345,0.35,0.355,0.36,0.365,0.37,0.375,0.38,0.385,0.39,0.395,0.4,0.405,
0.41,0.415,0.42,0.425,0.43,0.435,0.44,0.445,0.45,0.455,0.46,0.465,0.47,
0.475,0.48,0.485,0.49,0.495,0.5,0.505,0.51,0.515,0.52,0.525,0.53,0.535,
0.54,0.545,0.55,0.555,0.56,0.565,0.57,0.575,0.58,0.585,0.59,0.595,0.6,0.605,
0.61,0.615,0.62,0.625,0.63,0.635,0.64,0.645,0.65,0.655,0.66,0.665,0.67,
0.675,0.68,0.685,0.690000000000001,0.695000000000001,0.700000000000001,
0.705000000000001,0.710000000000001,0.715000000000001,0.720000000000001,
0.725000000000001,0.730000000000001,0.735000000000001,0.740000000000001,
0.745000000000001,0.750000000000001,0.755000000000001,0.760000000000001,
0.765000000000001,0.770000000000001,0.775000000000001,0.780000000000001,
0.785000000000001,0.790000000000001,0.795000000000001,0.800000000000001,
0.805000000000001,0.810000000000001,0.815000000000001,0.820000000000001,
0.825000000000001,0.830000000000001,0.835000000000001,0.840000000000001,
0.845000000000001,0.850000000000001,0.855000000000001,0.860000000000001,
0.865000000000001,0.870000000000001,0.875000000000001,0.880000000000001,
0.885000000000001,0.890000000000001,0.895000000000001,0.900000000000001,
0.905000000000001,0.910000000000001,0.915000000000001,0.920000000000001,
0.925000000000001,0.930000000000001,0.935000000000001,0.940000000000001,
0.945000000000001,0.950000000000001,0.955000000000001,0.960000000000001,
0.965000000000001,0.970000000000001,0.975000000000001,0.980000000000001,
0.985000000000001,0.990000000000001,0.995000000000001,1.),.UNSPECIFIED.)
CURVE()
GEOMETRIC_REPRESENTATION_ITEM()
RATIONAL_B_SPLINE_CURVE((1.,1.,1.,1.,1.,1.,1.,1.,1.,1.,1.,1.,1.,1.,1.,1.,
1.,1.,1.,1.,1.,1.,1.,1.,1.,1.,1.,1.,1.,1.,1.,1.,1.,1.,1.,1.,1.,1.,1.,1.,
1.,1.,1.,1.,1.,1.,1.,1.,1.,1.,1.,1.,1.,1.,1.,1.,1.,1.,1.,1.,1.,1.,1.,1.,
1.,1.,1.,1.,1.,1.,1.,1.,1.,1.,1.,1.,1.,1.,1.,1.,1.,1.,1.,1.,1.,1.,1.,1.,
1.,1.,1.,1.,1.,1.,1.,1.,1.,1.,1.,1.,1.,1.,1.,1.,1.,1.,1.,1.,1.,1.,1.,1.,
1.,1.,1.,1.,1.,1.,1.,1.,1.,1.,1.,1.,1.,1.,1.,1.,1.,1.,1.,1.,1.,1.,1.,1.,
1.,1.,1.,1.,1.,1.,1.,1.,1.,1.,1.,1.,1.,1.,1.,1.,1.,1.,1.,1.,1.,1.,1.,1.,
1.,1.,1.,1.,1.,1.,1.,1.,1.,1.,1.,1.,1.,1.,1.,1.,1.,1.,1.,1.,1.,1.,1.,1.,
1.,1.,1.,1.,1.,1.,1.,1.,1.,1.,1.,1.,1.,1.,1.,1.,1.,1.,1.,1.,1.))
REPRESENTATION_ITEM('')
);
#1027=(
BOUNDED_SURFACE()
B_SPLINE_SURFACE(5,1,((#185605,#185606),(#185607,#185608),(#185609,#185610),
(#185611,#185612),(#185613,#185614),(#185615,#185616),(#185617,#185618),
(#185619,#185620),(#185621,#185622),(#185623,#185624),(#185625,#185626),
(#185627,#185628),(#185629,#185630),(#185631,#185632),(#185633,#185634),
(#185635,#185636),(#185637,#185638),(#185639,#185640),(#185641,#185642),
(#185643,#185644),(#185645,#185646),(#185647,#185648),(#185649,#185650),
(#185651,#185652),(#185653,#185654),(#185655,#185656),(#185657,#185658),
(#185659,#185660),(#185661,#185662),(#185663,#185664),(#185665,#185666),
(#185667,#185668),(#185669,#185670),(#185671,#185672),(#185673,#185674),
(#185675,#185676),(#185677,#185678),(#185679,#185680),(#185681,#185682),
(#185683,#185684),(#185685,#185686),(#185687,#185688),(#185689,#185690),
(#185691,#185692),(#185693,#185694),(#185695,#185696),(#185697,#185698),
(#185699,#185700),(#185701,#185702),(#185703,#185704),(#185705,#185706),
(#185707,#185708),(#185709,#185710),(#185711,#185712),(#185713,#185714),
(#185715,#185716),(#185717,#185718),(#185719,#185720),(#185721,#185722),
(#185723,#185724),(#185725,#185726),(#185727,#185728),(#185729,#185730),
(#185731,#185732),(#185733,#185734),(#185735,#185736),(#185737,#185738),
(#185739,#185740),(#185741,#185742),(#185743,#185744),(#185745,#185746),
(#185747,#185748),(#185749,#185750),(#185751,#185752),(#185753,#185754),
(#185755,#185756),(#185757,#185758),(#185759,#185760),(#185761,#185762),
(#185763,#185764),(#185765,#185766),(#185767,#185768),(#185769,#185770),
(#185771,#185772),(#185773,#185774),(#185775,#185776),(#185777,#185778),
(#185779,#185780),(#185781,#185782),(#185783,#185784),(#185785,#185786),
(#185787,#185788),(#185789,#185790),(#185791,#185792),(#185793,#185794),
(#185795,#185796),(#185797,#185798),(#185799,#185800),(#185801,#185802),
(#185803,#185804),(#185805,#185806),(#185807,#185808),(#185809,#185810),
(#185811,#185812),(#185813,#185814),(#185815,#185816),(#185817,#185818),
(#185819,#185820),(#185821,#185822),(#185823,#185824),(#185825,#185826),
(#185827,#185828),(#185829,#185830),(#185831,#185832),(#185833,#185834),
(#185835,#185836),(#185837,#185838),(#185839,#185840),(#185841,#185842),
(#185843,#185844),(#185845,#185846),(#185847,#185848),(#185849,#185850),
(#185851,#185852),(#185853,#185854),(#185855,#185856),(#185857,#185858),
(#185859,#185860),(#185861,#185862),(#185863,#185864),(#185865,#185866),
(#185867,#185868),(#185869,#185870),(#185871,#185872),(#185873,#185874),
(#185875,#185876),(#185877,#185878),(#185879,#185880),(#185881,#185882),
(#185883,#185884),(#185885,#185886),(#185887,#185888),(#185889,#185890),
(#185891,#185892),(#185893,#185894),(#185895,#185896),(#185897,#185898),
(#185899,#185900),(#185901,#185902),(#185903,#185904),(#185905,#185906),
(#185907,#185908),(#185909,#185910),(#185911,#185912),(#185913,#185914),
(#185915,#185916),(#185917,#185918),(#185919,#185920),(#185921,#185922),
(#185923,#185924),(#185925,#185926),(#185927,#185928),(#185929,#185930),
(#185931,#185932),(#185933,#185934),(#185935,#185936),(#185937,#185938),
(#185939,#185940),(#185941,#185942),(#185943,#185944),(#185945,#185946),
(#185947,#185948),(#185949,#185950),(#185951,#185952),(#185953,#185954),
(#185955,#185956),(#185957,#185958),(#185959,#185960),(#185961,#185962),
(#185963,#185964),(#185965,#185966),(#185967,#185968),(#185969,#185970),
(#185971,#185972),(#185973,#185974),(#185975,#185976),(#185977,#185978),
(#185979,#185980),(#185981,#185982),(#185983,#185984),(#185985,#185986),
(#185987,#185988),(#185989,#185990),(#185991,#185992),(#185993,#185994),
(#185995,#185996),(#185997,#185998),(#185999,#186000),(#186001,#186002),
(#186003,#186004),(#186005,#186006),(#186007,#186008),(#186009,#186010),
(#186011,#186012),(#186013,#186014)),.UNSPECIFIED.,.F.,.F.,.F.)
B_SPLINE_SURFACE_WITH_KNOTS((6,1,1,1,1,1,1,1,1,1,1,1,1,1,1,1,1,1,1,1,1,
1,1,1,1,1,1,1,1,1,1,1,1,1,1,1,1,1,1,1,1,1,1,1,1,1,1,1,1,1,1,1,1,1,1,1,1,
1,1,1,1,1,1,1,1,1,1,1,1,1,1,1,1,1,1,1,1,1,1,1,1,1,1,1,1,1,1,1,1,1,1,1,1,
1,1,1,1,1,1,1,1,1,1,1,1,1,1,1,1,1,1,1,1,1,1,1,1,1,1,1,1,1,1,1,1,1,1,1,1,
1,1,1,1,1,1,1,1,1,1,1,1,1,1,1,1,1,1,1,1,1,1,1,1,1,1,1,1,1,1,1,1,1,1,1,1,
1,1,1,1,1,1,1,1,1,1,1,1,1,1,1,1,1,1,1,1,1,1,1,1,1,1,1,1,1,1,1,1,1,1,1,6),
(2,2),(-1.,-0.995000000000001,-0.990000000000001,-0.985000000000001,-0.980000000000001,
-0.975000000000001,-0.970000000000001,-0.965000000000001,-0.960000000000001,
-0.955000000000001,-0.950000000000001,-0.945000000000001,-0.940000000000001,
-0.935000000000001,-0.930000000000001,-0.925000000000001,-0.920000000000001,
-0.915000000000001,-0.910000000000001,-0.905000000000001,-0.900000000000001,
-0.895000000000001,-0.890000000000001,-0.885000000000001,-0.880000000000001,
-0.875000000000001,-0.870000000000001,-0.865000000000001,-0.860000000000001,
-0.855000000000001,-0.850000000000001,-0.845000000000001,-0.840000000000001,
-0.835000000000001,-0.830000000000001,-0.825000000000001,-0.820000000000001,
-0.815000000000001,-0.810000000000001,-0.805000000000001,-0.800000000000001,
-0.795000000000001,-0.790000000000001,-0.785000000000001,-0.780000000000001,
-0.775000000000001,-0.770000000000001,-0.765000000000001,-0.760000000000001,
-0.755000000000001,-0.750000000000001,-0.745000000000001,-0.740000000000001,
-0.735000000000001,-0.730000000000001,-0.725000000000001,-0.720000000000001,
-0.715000000000001,-0.710000000000001,-0.705000000000001,-0.700000000000001,
-0.695000000000001,-0.690000000000001,-0.685,-0.68,-0.675,-0.67,-0.665,
-0.66,-0.655,-0.65,-0.645,-0.64,-0.635,-0.63,-0.625,-0.62,-0.615,-0.61,
-0.605,-0.6,-0.595,-0.59,-0.585,-0.58,-0.575,-0.57,-0.565,-0.56,-0.555,
-0.55,-0.545,-0.54,-0.535,-0.53,-0.525,-0.52,-0.515,-0.51,-0.505,-0.5,-0.495,
-0.49,-0.485,-0.48,-0.475,-0.47,-0.465,-0.46,-0.455,-0.45,-0.445,-0.44,
-0.435,-0.43,-0.425,-0.42,-0.415,-0.41,-0.405,-0.4,-0.395,-0.39,-0.385,
-0.38,-0.375,-0.37,-0.365,-0.36,-0.355,-0.35,-0.345,-0.34,-0.335,-0.33,
-0.325,-0.32,-0.315,-0.31,-0.305,-0.3,-0.295,-0.29,-0.285,-0.28,-0.275,
-0.27,-0.265,-0.26,-0.255,-0.25,-0.245,-0.24,-0.235,-0.23,-0.225,-0.22,
-0.215,-0.21,-0.205,-0.2,-0.195,-0.19,-0.185,-0.18,-0.175,-0.17,-0.165,
-0.16,-0.155,-0.15,-0.145,-0.14,-0.135,-0.13,-0.125,-0.12,-0.115,-0.11,
-0.105,-0.1,-0.095,-0.09,-0.085,-0.08,-0.075,-0.07,-0.065,-0.06,-0.055,
-0.05,-0.045,-0.04,-0.035,-0.03,-0.025,-0.02,-0.015,-0.01,-0.005,0.),(0.,
1.2),.UNSPECIFIED.)
GEOMETRIC_REPRESENTATION_ITEM()
RATIONAL_B_SPLINE_SURFACE(((1.,1.),(1.,1.),(1.,1.),(1.,1.),(1.,1.),(1.,
1.),(1.,1.),(1.,1.),(1.,1.),(1.,1.),(1.,1.),(1.,1.),(1.,1.),(1.,1.),(1.,
1.),(1.,1.),(1.,1.),(1.,1.),(1.,1.),(1.,1.),(1.,1.),(1.,1.),(1.,1.),(1.,
1.),(1.,1.),(1.,1.),(1.,1.),(1.,1.),(1.,1.),(1.,1.),(1.,1.),(1.,1.),(1.,
1.),(1.,1.),(1.,1.),(1.,1.),(1.,1.),(1.,1.),(1.,1.),(1.,1.),(1.,1.),(1.,
1.),(1.,1.),(1.,1.),(1.,1.),(1.,1.),(1.,1.),(1.,1.),(1.,1.),(1.,1.),(1.,
1.),(1.,1.),(1.,1.),(1.,1.),(1.,1.),(1.,1.),(1.,1.),(1.,1.),(1.,1.),(1.,
1.),(1.,1.),(1.,1.),(1.,1.),(1.,1.),(1.,1.),(1.,1.),(1.,1.),(1.,1.),(1.,
1.),(1.,1.),(1.,1.),(1.,1.),(1.,1.),(1.,1.),(1.,1.),(1.,1.),(1.,1.),(1.,
1.),(1.,1.),(1.,1.),(1.,1.),(1.,1.),(1.,1.),(1.,1.),(1.,1.),(1.,1.),(1.,
1.),(1.,1.),(1.,1.),(1.,1.),(1.,1.),(1.,1.),(1.,1.),(1.,1.),(1.,1.),(1.,
1.),(1.,1.),(1.,1.),(1.,1.),(1.,1.),(1.,1.),(1.,1.),(1.,1.),(1.,1.),(1.,
1.),(1.,1.),(1.,1.),(1.,1.),(1.,1.),(1.,1.),(1.,1.),(1.,1.),(1.,1.),(1.,
1.),(1.,1.),(1.,1.),(1.,1.),(1.,1.),(1.,1.),(1.,1.),(1.,1.),(1.,1.),(1.,
1.),(1.,1.),(1.,1.),(1.,1.),(1.,1.),(1.,1.),(1.,1.),(1.,1.),(1.,1.),(1.,
1.),(1.,1.),(1.,1.),(1.,1.),(1.,1.),(1.,1.),(1.,1.),(1.,1.),(1.,1.),(1.,
1.),(1.,1.),(1.,1.),(1.,1.),(1.,1.),(1.,1.),(1.,1.),(1.,1.),(1.,1.),(1.,
1.),(1.,1.),(1.,1.),(1.,1.),(1.,1.),(1.,1.),(1.,1.),(1.,1.),(1.,1.),(1.,
1.),(1.,1.),(1.,1.),(1.,1.),(1.,1.),(1.,1.),(1.,1.),(1.,1.),(1.,1.),(1.,
1.),(1.,1.),(1.,1.),(1.,1.),(1.,1.),(1.,1.),(1.,1.),(1.,1.),(1.,1.),(1.,
1.),(1.,1.),(1.,1.),(1.,1.),(1.,1.),(1.,1.),(1.,1.),(1.,1.),(1.,1.),(1.,
1.),(1.,1.),(1.,1.),(1.,1.),(1.,1.),(1.,1.),(1.,1.),(1.,1.),(1.,1.),(1.,
1.),(1.,1.),(1.,1.),(1.,1.),(1.,1.),(1.,1.),(1.,1.),(1.,1.),(1.,1.),(1.,
1.),(1.,1.)))
REPRESENTATION_ITEM('')
SURFACE()
);
#1028=(
BOUNDED_SURFACE()
B_SPLINE_SURFACE(5,1,((#186222,#186223),(#186224,#186225),(#186226,#186227),
(#186228,#186229),(#186230,#186231),(#186232,#186233),(#186234,#186235),
(#186236,#186237),(#186238,#186239),(#186240,#186241),(#186242,#186243),
(#186244,#186245),(#186246,#186247),(#186248,#186249),(#186250,#186251),
(#186252,#186253),(#186254,#186255),(#186256,#186257),(#186258,#186259),
(#186260,#186261),(#186262,#186263),(#186264,#186265),(#186266,#186267),
(#186268,#186269),(#186270,#186271),(#186272,#186273),(#186274,#186275),
(#186276,#186277),(#186278,#186279),(#186280,#186281),(#186282,#186283),
(#186284,#186285),(#186286,#186287),(#186288,#186289),(#186290,#186291),
(#186292,#186293),(#186294,#186295),(#186296,#186297),(#186298,#186299),
(#186300,#186301),(#186302,#186303),(#186304,#186305),(#186306,#186307),
(#186308,#186309),(#186310,#186311),(#186312,#186313),(#186314,#186315),
(#186316,#186317),(#186318,#186319),(#186320,#186321),(#186322,#186323),
(#186324,#186325),(#186326,#186327),(#186328,#186329),(#186330,#186331),
(#186332,#186333),(#186334,#186335),(#186336,#186337),(#186338,#186339),
(#186340,#186341),(#186342,#186343),(#186344,#186345),(#186346,#186347),
(#186348,#186349),(#186350,#186351),(#186352,#186353),(#186354,#186355),
(#186356,#186357),(#186358,#186359),(#186360,#186361),(#186362,#186363),
(#186364,#186365),(#186366,#186367),(#186368,#186369),(#186370,#186371),
(#186372,#186373),(#186374,#186375),(#186376,#186377),(#186378,#186379),
(#186380,#186381),(#186382,#186383),(#186384,#186385),(#186386,#186387),
(#186388,#186389),(#186390,#186391),(#186392,#186393),(#186394,#186395),
(#186396,#186397),(#186398,#186399),(#186400,#186401),(#186402,#186403),
(#186404,#186405),(#186406,#186407),(#186408,#186409),(#186410,#186411),
(#186412,#186413),(#186414,#186415),(#186416,#186417),(#186418,#186419),
(#186420,#186421),(#186422,#186423),(#186424,#186425),(#186426,#186427),
(#186428,#186429),(#186430,#186431),(#186432,#186433),(#186434,#186435),
(#186436,#186437),(#186438,#186439),(#186440,#186441),(#186442,#186443),
(#186444,#186445),(#186446,#186447),(#186448,#186449),(#186450,#186451),
(#186452,#186453),(#186454,#186455),(#186456,#186457),(#186458,#186459),
(#186460,#186461),(#186462,#186463),(#186464,#186465),(#186466,#186467),
(#186468,#186469),(#186470,#186471),(#186472,#186473),(#186474,#186475),
(#186476,#186477),(#186478,#186479),(#186480,#186481),(#186482,#186483),
(#186484,#186485),(#186486,#186487),(#186488,#186489),(#186490,#186491),
(#186492,#186493),(#186494,#186495),(#186496,#186497),(#186498,#186499),
(#186500,#186501),(#186502,#186503),(#186504,#186505),(#186506,#186507),
(#186508,#186509),(#186510,#186511),(#186512,#186513),(#186514,#186515),
(#186516,#186517),(#186518,#186519),(#186520,#186521),(#186522,#186523),
(#186524,#186525),(#186526,#186527),(#186528,#186529),(#186530,#186531),
(#186532,#186533),(#186534,#186535),(#186536,#186537),(#186538,#186539),
(#186540,#186541),(#186542,#186543),(#186544,#186545),(#186546,#186547),
(#186548,#186549),(#186550,#186551),(#186552,#186553),(#186554,#186555),
(#186556,#186557),(#186558,#186559),(#186560,#186561),(#186562,#186563),
(#186564,#186565),(#186566,#186567),(#186568,#186569),(#186570,#186571),
(#186572,#186573),(#186574,#186575),(#186576,#186577),(#186578,#186579),
(#186580,#186581),(#186582,#186583),(#186584,#186585),(#186586,#186587),
(#186588,#186589),(#186590,#186591),(#186592,#186593),(#186594,#186595),
(#186596,#186597),(#186598,#186599),(#186600,#186601),(#186602,#186603),
(#186604,#186605),(#186606,#186607),(#186608,#186609),(#186610,#186611),
(#186612,#186613),(#186614,#186615),(#186616,#186617),(#186618,#186619),
(#186620,#186621),(#186622,#186623),(#186624,#186625),(#186626,#186627),
(#186628,#186629),(#186630,#186631)),.UNSPECIFIED.,.F.,.F.,.F.)
B_SPLINE_SURFACE_WITH_KNOTS((6,1,1,1,1,1,1,1,1,1,1,1,1,1,1,1,1,1,1,1,1,
1,1,1,1,1,1,1,1,1,1,1,1,1,1,1,1,1,1,1,1,1,1,1,1,1,1,1,1,1,1,1,1,1,1,1,1,
1,1,1,1,1,1,1,1,1,1,1,1,1,1,1,1,1,1,1,1,1,1,1,1,1,1,1,1,1,1,1,1,1,1,1,1,
1,1,1,1,1,1,1,1,1,1,1,1,1,1,1,1,1,1,1,1,1,1,1,1,1,1,1,1,1,1,1,1,1,1,1,1,
1,1,1,1,1,1,1,1,1,1,1,1,1,1,1,1,1,1,1,1,1,1,1,1,1,1,1,1,1,1,1,1,1,1,1,1,
1,1,1,1,1,1,1,1,1,1,1,1,1,1,1,1,1,1,1,1,1,1,1,1,1,1,1,1,1,1,1,1,1,1,1,6),
(2,2),(0.,0.005,0.01,0.015,0.02,0.025,0.03,0.035,0.04,0.045,0.05,0.055,
0.06,0.065,0.07,0.075,0.08,0.085,0.09,0.095,0.1,0.105,0.11,0.115,0.12,0.125,
0.13,0.135,0.14,0.145,0.15,0.155,0.16,0.165,0.17,0.175,0.18,0.185,0.19,
0.195,0.2,0.205,0.21,0.215,0.22,0.225,0.23,0.235,0.24,0.245,0.25,0.255,
0.26,0.265,0.27,0.275,0.28,0.285,0.29,0.295,0.3,0.305,0.31,0.315,0.32,0.325,
0.33,0.335,0.34,0.345,0.35,0.355,0.36,0.365,0.37,0.375,0.38,0.385,0.39,
0.395,0.4,0.405,0.41,0.415,0.42,0.425,0.43,0.435,0.44,0.445,0.45,0.455,
0.46,0.465,0.47,0.475,0.48,0.485,0.49,0.495,0.5,0.505,0.51,0.515,0.52,0.525,
0.53,0.535,0.54,0.545,0.55,0.555,0.56,0.565,0.57,0.575,0.58,0.585,0.59,
0.595,0.6,0.605,0.61,0.615,0.62,0.625,0.63,0.635,0.64,0.645,0.65,0.655,
0.66,0.665,0.67,0.675,0.68,0.685,0.690000000000001,0.695000000000001,0.700000000000001,
0.705000000000001,0.710000000000001,0.715000000000001,0.720000000000001,
0.725000000000001,0.730000000000001,0.735000000000001,0.740000000000001,
0.745000000000001,0.750000000000001,0.755000000000001,0.760000000000001,
0.765000000000001,0.770000000000001,0.775000000000001,0.780000000000001,
0.785000000000001,0.790000000000001,0.795000000000001,0.800000000000001,
0.805000000000001,0.810000000000001,0.815000000000001,0.820000000000001,
0.825000000000001,0.830000000000001,0.835000000000001,0.840000000000001,
0.845000000000001,0.850000000000001,0.855000000000001,0.860000000000001,
0.865000000000001,0.870000000000001,0.875000000000001,0.880000000000001,
0.885000000000001,0.890000000000001,0.895000000000001,0.900000000000001,
0.905000000000001,0.910000000000001,0.915000000000001,0.920000000000001,
0.925000000000001,0.930000000000001,0.935000000000001,0.940000000000001,
0.945000000000001,0.950000000000001,0.955000000000001,0.960000000000001,
0.965000000000001,0.970000000000001,0.975000000000001,0.980000000000001,
0.985000000000001,0.990000000000001,0.995000000000001,1.),(0.,1.2),
 .UNSPECIFIED.)
GEOMETRIC_REPRESENTATION_ITEM()
RATIONAL_B_SPLINE_SURFACE(((1.,1.),(1.,1.),(1.,1.),(1.,1.),(1.,1.),(1.,
1.),(1.,1.),(1.,1.),(1.,1.),(1.,1.),(1.,1.),(1.,1.),(1.,1.),(1.,1.),(1.,
1.),(1.,1.),(1.,1.),(1.,1.),(1.,1.),(1.,1.),(1.,1.),(1.,1.),(1.,1.),(1.,
1.),(1.,1.),(1.,1.),(1.,1.),(1.,1.),(1.,1.),(1.,1.),(1.,1.),(1.,1.),(1.,
1.),(1.,1.),(1.,1.),(1.,1.),(1.,1.),(1.,1.),(1.,1.),(1.,1.),(1.,1.),(1.,
1.),(1.,1.),(1.,1.),(1.,1.),(1.,1.),(1.,1.),(1.,1.),(1.,1.),(1.,1.),(1.,
1.),(1.,1.),(1.,1.),(1.,1.),(1.,1.),(1.,1.),(1.,1.),(1.,1.),(1.,1.),(1.,
1.),(1.,1.),(1.,1.),(1.,1.),(1.,1.),(1.,1.),(1.,1.),(1.,1.),(1.,1.),(1.,
1.),(1.,1.),(1.,1.),(1.,1.),(1.,1.),(1.,1.),(1.,1.),(1.,1.),(1.,1.),(1.,
1.),(1.,1.),(1.,1.),(1.,1.),(1.,1.),(1.,1.),(1.,1.),(1.,1.),(1.,1.),(1.,
1.),(1.,1.),(1.,1.),(1.,1.),(1.,1.),(1.,1.),(1.,1.),(1.,1.),(1.,1.),(1.,
1.),(1.,1.),(1.,1.),(1.,1.),(1.,1.),(1.,1.),(1.,1.),(1.,1.),(1.,1.),(1.,
1.),(1.,1.),(1.,1.),(1.,1.),(1.,1.),(1.,1.),(1.,1.),(1.,1.),(1.,1.),(1.,
1.),(1.,1.),(1.,1.),(1.,1.),(1.,1.),(1.,1.),(1.,1.),(1.,1.),(1.,1.),(1.,
1.),(1.,1.),(1.,1.),(1.,1.),(1.,1.),(1.,1.),(1.,1.),(1.,1.),(1.,1.),(1.,
1.),(1.,1.),(1.,1.),(1.,1.),(1.,1.),(1.,1.),(1.,1.),(1.,1.),(1.,1.),(1.,
1.),(1.,1.),(1.,1.),(1.,1.),(1.,1.),(1.,1.),(1.,1.),(1.,1.),(1.,1.),(1.,
1.),(1.,1.),(1.,1.),(1.,1.),(1.,1.),(1.,1.),(1.,1.),(1.,1.),(1.,1.),(1.,
1.),(1.,1.),(1.,1.),(1.,1.),(1.,1.),(1.,1.),(1.,1.),(1.,1.),(1.,1.),(1.,
1.),(1.,1.),(1.,1.),(1.,1.),(1.,1.),(1.,1.),(1.,1.),(1.,1.),(1.,1.),(1.,
1.),(1.,1.),(1.,1.),(1.,1.),(1.,1.),(1.,1.),(1.,1.),(1.,1.),(1.,1.),(1.,
1.),(1.,1.),(1.,1.),(1.,1.),(1.,1.),(1.,1.),(1.,1.),(1.,1.),(1.,1.),(1.,
1.),(1.,1.),(1.,1.),(1.,1.),(1.,1.),(1.,1.),(1.,1.),(1.,1.),(1.,1.),(1.,
1.),(1.,1.)))
REPRESENTATION_ITEM('')
SURFACE()
);
#1029=(
BOUNDED_SURFACE()
B_SPLINE_SURFACE(5,1,((#186843,#186844),(#186845,#186846),(#186847,#186848),
(#186849,#186850),(#186851,#186852),(#186853,#186854),(#186855,#186856),
(#186857,#186858),(#186859,#186860),(#186861,#186862),(#186863,#186864),
(#186865,#186866),(#186867,#186868),(#186869,#186870),(#186871,#186872),
(#186873,#186874),(#186875,#186876),(#186877,#186878),(#186879,#186880),
(#186881,#186882),(#186883,#186884),(#186885,#186886),(#186887,#186888),
(#186889,#186890),(#186891,#186892),(#186893,#186894),(#186895,#186896),
(#186897,#186898),(#186899,#186900),(#186901,#186902),(#186903,#186904),
(#186905,#186906),(#186907,#186908),(#186909,#186910),(#186911,#186912),
(#186913,#186914),(#186915,#186916),(#186917,#186918),(#186919,#186920),
(#186921,#186922),(#186923,#186924),(#186925,#186926),(#186927,#186928),
(#186929,#186930),(#186931,#186932),(#186933,#186934),(#186935,#186936),
(#186937,#186938),(#186939,#186940),(#186941,#186942),(#186943,#186944),
(#186945,#186946),(#186947,#186948),(#186949,#186950),(#186951,#186952),
(#186953,#186954),(#186955,#186956),(#186957,#186958),(#186959,#186960),
(#186961,#186962),(#186963,#186964),(#186965,#186966),(#186967,#186968),
(#186969,#186970),(#186971,#186972),(#186973,#186974),(#186975,#186976),
(#186977,#186978),(#186979,#186980),(#186981,#186982),(#186983,#186984),
(#186985,#186986),(#186987,#186988),(#186989,#186990),(#186991,#186992),
(#186993,#186994),(#186995,#186996),(#186997,#186998),(#186999,#187000),
(#187001,#187002),(#187003,#187004),(#187005,#187006),(#187007,#187008),
(#187009,#187010),(#187011,#187012),(#187013,#187014),(#187015,#187016),
(#187017,#187018),(#187019,#187020),(#187021,#187022),(#187023,#187024),
(#187025,#187026),(#187027,#187028),(#187029,#187030),(#187031,#187032),
(#187033,#187034),(#187035,#187036),(#187037,#187038),(#187039,#187040),
(#187041,#187042),(#187043,#187044),(#187045,#187046),(#187047,#187048),
(#187049,#187050),(#187051,#187052),(#187053,#187054),(#187055,#187056),
(#187057,#187058),(#187059,#187060),(#187061,#187062),(#187063,#187064),
(#187065,#187066),(#187067,#187068),(#187069,#187070),(#187071,#187072),
(#187073,#187074),(#187075,#187076),(#187077,#187078),(#187079,#187080),
(#187081,#187082),(#187083,#187084),(#187085,#187086),(#187087,#187088),
(#187089,#187090),(#187091,#187092),(#187093,#187094),(#187095,#187096),
(#187097,#187098),(#187099,#187100),(#187101,#187102),(#187103,#187104),
(#187105,#187106),(#187107,#187108),(#187109,#187110),(#187111,#187112),
(#187113,#187114),(#187115,#187116),(#187117,#187118),(#187119,#187120),
(#187121,#187122),(#187123,#187124),(#187125,#187126),(#187127,#187128),
(#187129,#187130),(#187131,#187132),(#187133,#187134),(#187135,#187136),
(#187137,#187138),(#187139,#187140),(#187141,#187142),(#187143,#187144),
(#187145,#187146),(#187147,#187148),(#187149,#187150),(#187151,#187152),
(#187153,#187154),(#187155,#187156),(#187157,#187158),(#187159,#187160),
(#187161,#187162),(#187163,#187164),(#187165,#187166),(#187167,#187168),
(#187169,#187170),(#187171,#187172),(#187173,#187174),(#187175,#187176),
(#187177,#187178),(#187179,#187180),(#187181,#187182),(#187183,#187184),
(#187185,#187186),(#187187,#187188),(#187189,#187190),(#187191,#187192),
(#187193,#187194),(#187195,#187196),(#187197,#187198),(#187199,#187200),
(#187201,#187202),(#187203,#187204),(#187205,#187206),(#187207,#187208),
(#187209,#187210),(#187211,#187212),(#187213,#187214),(#187215,#187216),
(#187217,#187218),(#187219,#187220),(#187221,#187222),(#187223,#187224),
(#187225,#187226),(#187227,#187228),(#187229,#187230),(#187231,#187232),
(#187233,#187234),(#187235,#187236),(#187237,#187238),(#187239,#187240),
(#187241,#187242),(#187243,#187244),(#187245,#187246),(#187247,#187248),
(#187249,#187250),(#187251,#187252)),.UNSPECIFIED.,.F.,.F.,.F.)
B_SPLINE_SURFACE_WITH_KNOTS((6,1,1,1,1,1,1,1,1,1,1,1,1,1,1,1,1,1,1,1,1,
1,1,1,1,1,1,1,1,1,1,1,1,1,1,1,1,1,1,1,1,1,1,1,1,1,1,1,1,1,1,1,1,1,1,1,1,
1,1,1,1,1,1,1,1,1,1,1,1,1,1,1,1,1,1,1,1,1,1,1,1,1,1,1,1,1,1,1,1,1,1,1,1,
1,1,1,1,1,1,1,1,1,1,1,1,1,1,1,1,1,1,1,1,1,1,1,1,1,1,1,1,1,1,1,1,1,1,1,1,
1,1,1,1,1,1,1,1,1,1,1,1,1,1,1,1,1,1,1,1,1,1,1,1,1,1,1,1,1,1,1,1,1,1,1,1,
1,1,1,1,1,1,1,1,1,1,1,1,1,1,1,1,1,1,1,1,1,1,1,1,1,1,1,1,1,1,1,1,1,1,1,6),
(2,2),(-1.,-0.995000000000001,-0.990000000000001,-0.985000000000001,-0.980000000000001,
-0.975000000000001,-0.970000000000001,-0.965000000000001,-0.960000000000001,
-0.955000000000001,-0.950000000000001,-0.945000000000001,-0.940000000000001,
-0.935000000000001,-0.930000000000001,-0.925000000000001,-0.920000000000001,
-0.915000000000001,-0.910000000000001,-0.905000000000001,-0.900000000000001,
-0.895000000000001,-0.890000000000001,-0.885000000000001,-0.880000000000001,
-0.875000000000001,-0.870000000000001,-0.865000000000001,-0.860000000000001,
-0.855000000000001,-0.850000000000001,-0.845000000000001,-0.840000000000001,
-0.835000000000001,-0.830000000000001,-0.825000000000001,-0.820000000000001,
-0.815000000000001,-0.810000000000001,-0.805000000000001,-0.800000000000001,
-0.795000000000001,-0.790000000000001,-0.785000000000001,-0.780000000000001,
-0.775000000000001,-0.770000000000001,-0.765000000000001,-0.760000000000001,
-0.755000000000001,-0.750000000000001,-0.745000000000001,-0.740000000000001,
-0.735000000000001,-0.730000000000001,-0.725000000000001,-0.720000000000001,
-0.715000000000001,-0.710000000000001,-0.705000000000001,-0.700000000000001,
-0.695000000000001,-0.690000000000001,-0.685,-0.68,-0.675,-0.67,-0.665,
-0.66,-0.655,-0.65,-0.645,-0.64,-0.635,-0.63,-0.625,-0.62,-0.615,-0.61,
-0.605,-0.6,-0.595,-0.59,-0.585,-0.58,-0.575,-0.57,-0.565,-0.56,-0.555,
-0.55,-0.545,-0.54,-0.535,-0.53,-0.525,-0.52,-0.515,-0.51,-0.505,-0.5,-0.495,
-0.49,-0.485,-0.48,-0.475,-0.47,-0.465,-0.46,-0.455,-0.45,-0.445,-0.44,
-0.435,-0.43,-0.425,-0.42,-0.415,-0.41,-0.405,-0.4,-0.395,-0.39,-0.385,
-0.38,-0.375,-0.37,-0.365,-0.36,-0.355,-0.35,-0.345,-0.34,-0.335,-0.33,
-0.325,-0.32,-0.315,-0.31,-0.305,-0.3,-0.295,-0.29,-0.285,-0.28,-0.275,
-0.27,-0.265,-0.26,-0.255,-0.25,-0.245,-0.24,-0.235,-0.23,-0.225,-0.22,
-0.215,-0.21,-0.205,-0.2,-0.195,-0.19,-0.185,-0.18,-0.175,-0.17,-0.165,
-0.16,-0.155,-0.15,-0.145,-0.14,-0.135,-0.13,-0.125,-0.12,-0.115,-0.11,
-0.105,-0.1,-0.095,-0.09,-0.085,-0.08,-0.075,-0.07,-0.065,-0.06,-0.055,
-0.05,-0.045,-0.04,-0.035,-0.03,-0.025,-0.02,-0.015,-0.01,-0.005,0.),(0.,
1.2),.UNSPECIFIED.)
GEOMETRIC_REPRESENTATION_ITEM()
RATIONAL_B_SPLINE_SURFACE(((1.,1.),(1.,1.),(1.,1.),(1.,1.),(1.,1.),(1.,
1.),(1.,1.),(1.,1.),(1.,1.),(1.,1.),(1.,1.),(1.,1.),(1.,1.),(1.,1.),(1.,
1.),(1.,1.),(1.,1.),(1.,1.),(1.,1.),(1.,1.),(1.,1.),(1.,1.),(1.,1.),(1.,
1.),(1.,1.),(1.,1.),(1.,1.),(1.,1.),(1.,1.),(1.,1.),(1.,1.),(1.,1.),(1.,
1.),(1.,1.),(1.,1.),(1.,1.),(1.,1.),(1.,1.),(1.,1.),(1.,1.),(1.,1.),(1.,
1.),(1.,1.),(1.,1.),(1.,1.),(1.,1.),(1.,1.),(1.,1.),(1.,1.),(1.,1.),(1.,
1.),(1.,1.),(1.,1.),(1.,1.),(1.,1.),(1.,1.),(1.,1.),(1.,1.),(1.,1.),(1.,
1.),(1.,1.),(1.,1.),(1.,1.),(1.,1.),(1.,1.),(1.,1.),(1.,1.),(1.,1.),(1.,
1.),(1.,1.),(1.,1.),(1.,1.),(1.,1.),(1.,1.),(1.,1.),(1.,1.),(1.,1.),(1.,
1.),(1.,1.),(1.,1.),(1.,1.),(1.,1.),(1.,1.),(1.,1.),(1.,1.),(1.,1.),(1.,
1.),(1.,1.),(1.,1.),(1.,1.),(1.,1.),(1.,1.),(1.,1.),(1.,1.),(1.,1.),(1.,
1.),(1.,1.),(1.,1.),(1.,1.),(1.,1.),(1.,1.),(1.,1.),(1.,1.),(1.,1.),(1.,
1.),(1.,1.),(1.,1.),(1.,1.),(1.,1.),(1.,1.),(1.,1.),(1.,1.),(1.,1.),(1.,
1.),(1.,1.),(1.,1.),(1.,1.),(1.,1.),(1.,1.),(1.,1.),(1.,1.),(1.,1.),(1.,
1.),(1.,1.),(1.,1.),(1.,1.),(1.,1.),(1.,1.),(1.,1.),(1.,1.),(1.,1.),(1.,
1.),(1.,1.),(1.,1.),(1.,1.),(1.,1.),(1.,1.),(1.,1.),(1.,1.),(1.,1.),(1.,
1.),(1.,1.),(1.,1.),(1.,1.),(1.,1.),(1.,1.),(1.,1.),(1.,1.),(1.,1.),(1.,
1.),(1.,1.),(1.,1.),(1.,1.),(1.,1.),(1.,1.),(1.,1.),(1.,1.),(1.,1.),(1.,
1.),(1.,1.),(1.,1.),(1.,1.),(1.,1.),(1.,1.),(1.,1.),(1.,1.),(1.,1.),(1.,
1.),(1.,1.),(1.,1.),(1.,1.),(1.,1.),(1.,1.),(1.,1.),(1.,1.),(1.,1.),(1.,
1.),(1.,1.),(1.,1.),(1.,1.),(1.,1.),(1.,1.),(1.,1.),(1.,1.),(1.,1.),(1.,
1.),(1.,1.),(1.,1.),(1.,1.),(1.,1.),(1.,1.),(1.,1.),(1.,1.),(1.,1.),(1.,
1.),(1.,1.),(1.,1.),(1.,1.),(1.,1.),(1.,1.),(1.,1.),(1.,1.),(1.,1.),(1.,
1.),(1.,1.)))
REPRESENTATION_ITEM('')
SURFACE()
);
#1030=(
BOUNDED_SURFACE()
B_SPLINE_SURFACE(5,1,((#187460,#187461),(#187462,#187463),(#187464,#187465),
(#187466,#187467),(#187468,#187469),(#187470,#187471),(#187472,#187473),
(#187474,#187475),(#187476,#187477),(#187478,#187479),(#187480,#187481),
(#187482,#187483),(#187484,#187485),(#187486,#187487),(#187488,#187489),
(#187490,#187491),(#187492,#187493),(#187494,#187495),(#187496,#187497),
(#187498,#187499),(#187500,#187501),(#187502,#187503),(#187504,#187505),
(#187506,#187507),(#187508,#187509),(#187510,#187511),(#187512,#187513),
(#187514,#187515),(#187516,#187517),(#187518,#187519),(#187520,#187521),
(#187522,#187523),(#187524,#187525),(#187526,#187527),(#187528,#187529),
(#187530,#187531),(#187532,#187533),(#187534,#187535),(#187536,#187537),
(#187538,#187539),(#187540,#187541),(#187542,#187543),(#187544,#187545),
(#187546,#187547),(#187548,#187549),(#187550,#187551),(#187552,#187553),
(#187554,#187555),(#187556,#187557),(#187558,#187559),(#187560,#187561),
(#187562,#187563),(#187564,#187565),(#187566,#187567),(#187568,#187569),
(#187570,#187571),(#187572,#187573),(#187574,#187575),(#187576,#187577),
(#187578,#187579),(#187580,#187581),(#187582,#187583),(#187584,#187585),
(#187586,#187587),(#187588,#187589),(#187590,#187591),(#187592,#187593),
(#187594,#187595),(#187596,#187597),(#187598,#187599),(#187600,#187601),
(#187602,#187603),(#187604,#187605),(#187606,#187607),(#187608,#187609),
(#187610,#187611),(#187612,#187613),(#187614,#187615),(#187616,#187617),
(#187618,#187619),(#187620,#187621),(#187622,#187623),(#187624,#187625),
(#187626,#187627),(#187628,#187629),(#187630,#187631),(#187632,#187633),
(#187634,#187635),(#187636,#187637),(#187638,#187639),(#187640,#187641),
(#187642,#187643),(#187644,#187645),(#187646,#187647),(#187648,#187649),
(#187650,#187651),(#187652,#187653),(#187654,#187655),(#187656,#187657),
(#187658,#187659),(#187660,#187661),(#187662,#187663),(#187664,#187665),
(#187666,#187667),(#187668,#187669),(#187670,#187671),(#187672,#187673),
(#187674,#187675),(#187676,#187677),(#187678,#187679),(#187680,#187681),
(#187682,#187683),(#187684,#187685),(#187686,#187687),(#187688,#187689),
(#187690,#187691),(#187692,#187693),(#187694,#187695),(#187696,#187697),
(#187698,#187699),(#187700,#187701),(#187702,#187703),(#187704,#187705),
(#187706,#187707),(#187708,#187709),(#187710,#187711),(#187712,#187713),
(#187714,#187715),(#187716,#187717),(#187718,#187719),(#187720,#187721),
(#187722,#187723),(#187724,#187725),(#187726,#187727),(#187728,#187729),
(#187730,#187731),(#187732,#187733),(#187734,#187735),(#187736,#187737),
(#187738,#187739),(#187740,#187741),(#187742,#187743),(#187744,#187745),
(#187746,#187747),(#187748,#187749),(#187750,#187751),(#187752,#187753),
(#187754,#187755),(#187756,#187757),(#187758,#187759),(#187760,#187761),
(#187762,#187763),(#187764,#187765),(#187766,#187767),(#187768,#187769),
(#187770,#187771),(#187772,#187773),(#187774,#187775),(#187776,#187777),
(#187778,#187779),(#187780,#187781),(#187782,#187783),(#187784,#187785),
(#187786,#187787),(#187788,#187789),(#187790,#187791),(#187792,#187793),
(#187794,#187795),(#187796,#187797),(#187798,#187799),(#187800,#187801),
(#187802,#187803),(#187804,#187805),(#187806,#187807),(#187808,#187809),
(#187810,#187811),(#187812,#187813),(#187814,#187815),(#187816,#187817),
(#187818,#187819),(#187820,#187821),(#187822,#187823),(#187824,#187825),
(#187826,#187827),(#187828,#187829),(#187830,#187831),(#187832,#187833),
(#187834,#187835),(#187836,#187837),(#187838,#187839),(#187840,#187841),
(#187842,#187843),(#187844,#187845),(#187846,#187847),(#187848,#187849),
(#187850,#187851),(#187852,#187853),(#187854,#187855),(#187856,#187857),
(#187858,#187859),(#187860,#187861),(#187862,#187863),(#187864,#187865),
(#187866,#187867),(#187868,#187869)),.UNSPECIFIED.,.F.,.F.,.F.)
B_SPLINE_SURFACE_WITH_KNOTS((6,1,1,1,1,1,1,1,1,1,1,1,1,1,1,1,1,1,1,1,1,
1,1,1,1,1,1,1,1,1,1,1,1,1,1,1,1,1,1,1,1,1,1,1,1,1,1,1,1,1,1,1,1,1,1,1,1,
1,1,1,1,1,1,1,1,1,1,1,1,1,1,1,1,1,1,1,1,1,1,1,1,1,1,1,1,1,1,1,1,1,1,1,1,
1,1,1,1,1,1,1,1,1,1,1,1,1,1,1,1,1,1,1,1,1,1,1,1,1,1,1,1,1,1,1,1,1,1,1,1,
1,1,1,1,1,1,1,1,1,1,1,1,1,1,1,1,1,1,1,1,1,1,1,1,1,1,1,1,1,1,1,1,1,1,1,1,
1,1,1,1,1,1,1,1,1,1,1,1,1,1,1,1,1,1,1,1,1,1,1,1,1,1,1,1,1,1,1,1,1,1,1,6),
(2,2),(0.,0.005,0.01,0.015,0.02,0.025,0.03,0.035,0.04,0.045,0.05,0.055,
0.06,0.065,0.07,0.075,0.08,0.085,0.09,0.095,0.1,0.105,0.11,0.115,0.12,0.125,
0.13,0.135,0.14,0.145,0.15,0.155,0.16,0.165,0.17,0.175,0.18,0.185,0.19,
0.195,0.2,0.205,0.21,0.215,0.22,0.225,0.23,0.235,0.24,0.245,0.25,0.255,
0.26,0.265,0.27,0.275,0.28,0.285,0.29,0.295,0.3,0.305,0.31,0.315,0.32,0.325,
0.33,0.335,0.34,0.345,0.35,0.355,0.36,0.365,0.37,0.375,0.38,0.385,0.39,
0.395,0.4,0.405,0.41,0.415,0.42,0.425,0.43,0.435,0.44,0.445,0.45,0.455,
0.46,0.465,0.47,0.475,0.48,0.485,0.49,0.495,0.5,0.505,0.51,0.515,0.52,0.525,
0.53,0.535,0.54,0.545,0.55,0.555,0.56,0.565,0.57,0.575,0.58,0.585,0.59,
0.595,0.6,0.605,0.61,0.615,0.62,0.625,0.63,0.635,0.64,0.645,0.65,0.655,
0.66,0.665,0.67,0.675,0.68,0.685,0.690000000000001,0.695000000000001,0.700000000000001,
0.705000000000001,0.710000000000001,0.715000000000001,0.720000000000001,
0.725000000000001,0.730000000000001,0.735000000000001,0.740000000000001,
0.745000000000001,0.750000000000001,0.755000000000001,0.760000000000001,
0.765000000000001,0.770000000000001,0.775000000000001,0.780000000000001,
0.785000000000001,0.790000000000001,0.795000000000001,0.800000000000001,
0.805000000000001,0.810000000000001,0.815000000000001,0.820000000000001,
0.825000000000001,0.830000000000001,0.835000000000001,0.840000000000001,
0.845000000000001,0.850000000000001,0.855000000000001,0.860000000000001,
0.865000000000001,0.870000000000001,0.875000000000001,0.880000000000001,
0.885000000000001,0.890000000000001,0.895000000000001,0.900000000000001,
0.905000000000001,0.910000000000001,0.915000000000001,0.920000000000001,
0.925000000000001,0.930000000000001,0.935000000000001,0.940000000000001,
0.945000000000001,0.950000000000001,0.955000000000001,0.960000000000001,
0.965000000000001,0.970000000000001,0.975000000000001,0.980000000000001,
0.985000000000001,0.990000000000001,0.995000000000001,1.),(0.,1.2),
 .UNSPECIFIED.)
GEOMETRIC_REPRESENTATION_ITEM()
RATIONAL_B_SPLINE_SURFACE(((1.,1.),(1.,1.),(1.,1.),(1.,1.),(1.,1.),(1.,
1.),(1.,1.),(1.,1.),(1.,1.),(1.,1.),(1.,1.),(1.,1.),(1.,1.),(1.,1.),(1.,
1.),(1.,1.),(1.,1.),(1.,1.),(1.,1.),(1.,1.),(1.,1.),(1.,1.),(1.,1.),(1.,
1.),(1.,1.),(1.,1.),(1.,1.),(1.,1.),(1.,1.),(1.,1.),(1.,1.),(1.,1.),(1.,
1.),(1.,1.),(1.,1.),(1.,1.),(1.,1.),(1.,1.),(1.,1.),(1.,1.),(1.,1.),(1.,
1.),(1.,1.),(1.,1.),(1.,1.),(1.,1.),(1.,1.),(1.,1.),(1.,1.),(1.,1.),(1.,
1.),(1.,1.),(1.,1.),(1.,1.),(1.,1.),(1.,1.),(1.,1.),(1.,1.),(1.,1.),(1.,
1.),(1.,1.),(1.,1.),(1.,1.),(1.,1.),(1.,1.),(1.,1.),(1.,1.),(1.,1.),(1.,
1.),(1.,1.),(1.,1.),(1.,1.),(1.,1.),(1.,1.),(1.,1.),(1.,1.),(1.,1.),(1.,
1.),(1.,1.),(1.,1.),(1.,1.),(1.,1.),(1.,1.),(1.,1.),(1.,1.),(1.,1.),(1.,
1.),(1.,1.),(1.,1.),(1.,1.),(1.,1.),(1.,1.),(1.,1.),(1.,1.),(1.,1.),(1.,
1.),(1.,1.),(1.,1.),(1.,1.),(1.,1.),(1.,1.),(1.,1.),(1.,1.),(1.,1.),(1.,
1.),(1.,1.),(1.,1.),(1.,1.),(1.,1.),(1.,1.),(1.,1.),(1.,1.),(1.,1.),(1.,
1.),(1.,1.),(1.,1.),(1.,1.),(1.,1.),(1.,1.),(1.,1.),(1.,1.),(1.,1.),(1.,
1.),(1.,1.),(1.,1.),(1.,1.),(1.,1.),(1.,1.),(1.,1.),(1.,1.),(1.,1.),(1.,
1.),(1.,1.),(1.,1.),(1.,1.),(1.,1.),(1.,1.),(1.,1.),(1.,1.),(1.,1.),(1.,
1.),(1.,1.),(1.,1.),(1.,1.),(1.,1.),(1.,1.),(1.,1.),(1.,1.),(1.,1.),(1.,
1.),(1.,1.),(1.,1.),(1.,1.),(1.,1.),(1.,1.),(1.,1.),(1.,1.),(1.,1.),(1.,
1.),(1.,1.),(1.,1.),(1.,1.),(1.,1.),(1.,1.),(1.,1.),(1.,1.),(1.,1.),(1.,
1.),(1.,1.),(1.,1.),(1.,1.),(1.,1.),(1.,1.),(1.,1.),(1.,1.),(1.,1.),(1.,
1.),(1.,1.),(1.,1.),(1.,1.),(1.,1.),(1.,1.),(1.,1.),(1.,1.),(1.,1.),(1.,
1.),(1.,1.),(1.,1.),(1.,1.),(1.,1.),(1.,1.),(1.,1.),(1.,1.),(1.,1.),(1.,
1.),(1.,1.),(1.,1.),(1.,1.),(1.,1.),(1.,1.),(1.,1.),(1.,1.),(1.,1.),(1.,
1.),(1.,1.)))
REPRESENTATION_ITEM('')
SURFACE()
);
#1031=(
BOUNDED_SURFACE()
B_SPLINE_SURFACE(5,1,((#188081,#188082),(#188083,#188084),(#188085,#188086),
(#188087,#188088),(#188089,#188090),(#188091,#188092),(#188093,#188094),
(#188095,#188096),(#188097,#188098),(#188099,#188100),(#188101,#188102),
(#188103,#188104),(#188105,#188106),(#188107,#188108),(#188109,#188110),
(#188111,#188112),(#188113,#188114),(#188115,#188116),(#188117,#188118),
(#188119,#188120),(#188121,#188122),(#188123,#188124),(#188125,#188126),
(#188127,#188128),(#188129,#188130),(#188131,#188132),(#188133,#188134),
(#188135,#188136),(#188137,#188138),(#188139,#188140),(#188141,#188142),
(#188143,#188144),(#188145,#188146),(#188147,#188148),(#188149,#188150),
(#188151,#188152),(#188153,#188154),(#188155,#188156),(#188157,#188158),
(#188159,#188160),(#188161,#188162),(#188163,#188164),(#188165,#188166),
(#188167,#188168),(#188169,#188170),(#188171,#188172),(#188173,#188174),
(#188175,#188176),(#188177,#188178),(#188179,#188180),(#188181,#188182),
(#188183,#188184),(#188185,#188186),(#188187,#188188),(#188189,#188190),
(#188191,#188192),(#188193,#188194),(#188195,#188196),(#188197,#188198),
(#188199,#188200),(#188201,#188202),(#188203,#188204),(#188205,#188206),
(#188207,#188208),(#188209,#188210),(#188211,#188212),(#188213,#188214),
(#188215,#188216),(#188217,#188218),(#188219,#188220),(#188221,#188222),
(#188223,#188224),(#188225,#188226),(#188227,#188228),(#188229,#188230),
(#188231,#188232),(#188233,#188234),(#188235,#188236),(#188237,#188238),
(#188239,#188240),(#188241,#188242),(#188243,#188244),(#188245,#188246),
(#188247,#188248),(#188249,#188250),(#188251,#188252),(#188253,#188254),
(#188255,#188256),(#188257,#188258),(#188259,#188260),(#188261,#188262),
(#188263,#188264),(#188265,#188266),(#188267,#188268),(#188269,#188270),
(#188271,#188272),(#188273,#188274),(#188275,#188276),(#188277,#188278),
(#188279,#188280),(#188281,#188282),(#188283,#188284),(#188285,#188286),
(#188287,#188288),(#188289,#188290),(#188291,#188292),(#188293,#188294),
(#188295,#188296),(#188297,#188298),(#188299,#188300),(#188301,#188302),
(#188303,#188304),(#188305,#188306),(#188307,#188308),(#188309,#188310),
(#188311,#188312),(#188313,#188314),(#188315,#188316),(#188317,#188318),
(#188319,#188320),(#188321,#188322),(#188323,#188324),(#188325,#188326),
(#188327,#188328),(#188329,#188330),(#188331,#188332),(#188333,#188334),
(#188335,#188336),(#188337,#188338),(#188339,#188340),(#188341,#188342),
(#188343,#188344),(#188345,#188346),(#188347,#188348),(#188349,#188350),
(#188351,#188352),(#188353,#188354),(#188355,#188356),(#188357,#188358),
(#188359,#188360),(#188361,#188362),(#188363,#188364),(#188365,#188366),
(#188367,#188368),(#188369,#188370),(#188371,#188372),(#188373,#188374),
(#188375,#188376),(#188377,#188378),(#188379,#188380),(#188381,#188382),
(#188383,#188384),(#188385,#188386),(#188387,#188388),(#188389,#188390),
(#188391,#188392),(#188393,#188394),(#188395,#188396),(#188397,#188398),
(#188399,#188400),(#188401,#188402),(#188403,#188404),(#188405,#188406),
(#188407,#188408),(#188409,#188410),(#188411,#188412),(#188413,#188414),
(#188415,#188416),(#188417,#188418),(#188419,#188420),(#188421,#188422),
(#188423,#188424),(#188425,#188426),(#188427,#188428),(#188429,#188430),
(#188431,#188432),(#188433,#188434),(#188435,#188436),(#188437,#188438),
(#188439,#188440),(#188441,#188442),(#188443,#188444),(#188445,#188446),
(#188447,#188448),(#188449,#188450),(#188451,#188452),(#188453,#188454),
(#188455,#188456),(#188457,#188458),(#188459,#188460),(#188461,#188462),
(#188463,#188464),(#188465,#188466),(#188467,#188468),(#188469,#188470),
(#188471,#188472),(#188473,#188474),(#188475,#188476),(#188477,#188478),
(#188479,#188480),(#188481,#188482),(#188483,#188484),(#188485,#188486),
(#188487,#188488),(#188489,#188490)),.UNSPECIFIED.,.F.,.F.,.F.)
B_SPLINE_SURFACE_WITH_KNOTS((6,1,1,1,1,1,1,1,1,1,1,1,1,1,1,1,1,1,1,1,1,
1,1,1,1,1,1,1,1,1,1,1,1,1,1,1,1,1,1,1,1,1,1,1,1,1,1,1,1,1,1,1,1,1,1,1,1,
1,1,1,1,1,1,1,1,1,1,1,1,1,1,1,1,1,1,1,1,1,1,1,1,1,1,1,1,1,1,1,1,1,1,1,1,
1,1,1,1,1,1,1,1,1,1,1,1,1,1,1,1,1,1,1,1,1,1,1,1,1,1,1,1,1,1,1,1,1,1,1,1,
1,1,1,1,1,1,1,1,1,1,1,1,1,1,1,1,1,1,1,1,1,1,1,1,1,1,1,1,1,1,1,1,1,1,1,1,
1,1,1,1,1,1,1,1,1,1,1,1,1,1,1,1,1,1,1,1,1,1,1,1,1,1,1,1,1,1,1,1,1,1,1,6),
(2,2),(-1.,-0.995000000000001,-0.990000000000001,-0.985000000000001,-0.980000000000001,
-0.975000000000001,-0.970000000000001,-0.965000000000001,-0.960000000000001,
-0.955000000000001,-0.950000000000001,-0.945000000000001,-0.940000000000001,
-0.935000000000001,-0.930000000000001,-0.925000000000001,-0.920000000000001,
-0.915000000000001,-0.910000000000001,-0.905000000000001,-0.900000000000001,
-0.895000000000001,-0.890000000000001,-0.885000000000001,-0.880000000000001,
-0.875000000000001,-0.870000000000001,-0.865000000000001,-0.860000000000001,
-0.855000000000001,-0.850000000000001,-0.845000000000001,-0.840000000000001,
-0.835000000000001,-0.830000000000001,-0.825000000000001,-0.820000000000001,
-0.815000000000001,-0.810000000000001,-0.805000000000001,-0.800000000000001,
-0.795000000000001,-0.790000000000001,-0.785000000000001,-0.780000000000001,
-0.775000000000001,-0.770000000000001,-0.765000000000001,-0.760000000000001,
-0.755000000000001,-0.750000000000001,-0.745000000000001,-0.740000000000001,
-0.735000000000001,-0.730000000000001,-0.725000000000001,-0.720000000000001,
-0.715000000000001,-0.710000000000001,-0.705000000000001,-0.700000000000001,
-0.695000000000001,-0.690000000000001,-0.685,-0.68,-0.675,-0.67,-0.665,
-0.66,-0.655,-0.65,-0.645,-0.64,-0.635,-0.63,-0.625,-0.62,-0.615,-0.61,
-0.605,-0.6,-0.595,-0.59,-0.585,-0.58,-0.575,-0.57,-0.565,-0.56,-0.555,
-0.55,-0.545,-0.54,-0.535,-0.53,-0.525,-0.52,-0.515,-0.51,-0.505,-0.5,-0.495,
-0.49,-0.485,-0.48,-0.475,-0.47,-0.465,-0.46,-0.455,-0.45,-0.445,-0.44,
-0.435,-0.43,-0.425,-0.42,-0.415,-0.41,-0.405,-0.4,-0.395,-0.39,-0.385,
-0.38,-0.375,-0.37,-0.365,-0.36,-0.355,-0.35,-0.345,-0.34,-0.335,-0.33,
-0.325,-0.32,-0.315,-0.31,-0.305,-0.3,-0.295,-0.29,-0.285,-0.28,-0.275,
-0.27,-0.265,-0.26,-0.255,-0.25,-0.245,-0.24,-0.235,-0.23,-0.225,-0.22,
-0.215,-0.21,-0.205,-0.2,-0.195,-0.19,-0.185,-0.18,-0.175,-0.17,-0.165,
-0.16,-0.155,-0.15,-0.145,-0.14,-0.135,-0.13,-0.125,-0.12,-0.115,-0.11,
-0.105,-0.1,-0.095,-0.09,-0.085,-0.08,-0.075,-0.07,-0.065,-0.06,-0.055,
-0.05,-0.045,-0.04,-0.035,-0.03,-0.025,-0.02,-0.015,-0.01,-0.005,0.),(0.,
1.2),.UNSPECIFIED.)
GEOMETRIC_REPRESENTATION_ITEM()
RATIONAL_B_SPLINE_SURFACE(((1.,1.),(1.,1.),(1.,1.),(1.,1.),(1.,1.),(1.,
1.),(1.,1.),(1.,1.),(1.,1.),(1.,1.),(1.,1.),(1.,1.),(1.,1.),(1.,1.),(1.,
1.),(1.,1.),(1.,1.),(1.,1.),(1.,1.),(1.,1.),(1.,1.),(1.,1.),(1.,1.),(1.,
1.),(1.,1.),(1.,1.),(1.,1.),(1.,1.),(1.,1.),(1.,1.),(1.,1.),(1.,1.),(1.,
1.),(1.,1.),(1.,1.),(1.,1.),(1.,1.),(1.,1.),(1.,1.),(1.,1.),(1.,1.),(1.,
1.),(1.,1.),(1.,1.),(1.,1.),(1.,1.),(1.,1.),(1.,1.),(1.,1.),(1.,1.),(1.,
1.),(1.,1.),(1.,1.),(1.,1.),(1.,1.),(1.,1.),(1.,1.),(1.,1.),(1.,1.),(1.,
1.),(1.,1.),(1.,1.),(1.,1.),(1.,1.),(1.,1.),(1.,1.),(1.,1.),(1.,1.),(1.,
1.),(1.,1.),(1.,1.),(1.,1.),(1.,1.),(1.,1.),(1.,1.),(1.,1.),(1.,1.),(1.,
1.),(1.,1.),(1.,1.),(1.,1.),(1.,1.),(1.,1.),(1.,1.),(1.,1.),(1.,1.),(1.,
1.),(1.,1.),(1.,1.),(1.,1.),(1.,1.),(1.,1.),(1.,1.),(1.,1.),(1.,1.),(1.,
1.),(1.,1.),(1.,1.),(1.,1.),(1.,1.),(1.,1.),(1.,1.),(1.,1.),(1.,1.),(1.,
1.),(1.,1.),(1.,1.),(1.,1.),(1.,1.),(1.,1.),(1.,1.),(1.,1.),(1.,1.),(1.,
1.),(1.,1.),(1.,1.),(1.,1.),(1.,1.),(1.,1.),(1.,1.),(1.,1.),(1.,1.),(1.,
1.),(1.,1.),(1.,1.),(1.,1.),(1.,1.),(1.,1.),(1.,1.),(1.,1.),(1.,1.),(1.,
1.),(1.,1.),(1.,1.),(1.,1.),(1.,1.),(1.,1.),(1.,1.),(1.,1.),(1.,1.),(1.,
1.),(1.,1.),(1.,1.),(1.,1.),(1.,1.),(1.,1.),(1.,1.),(1.,1.),(1.,1.),(1.,
1.),(1.,1.),(1.,1.),(1.,1.),(1.,1.),(1.,1.),(1.,1.),(1.,1.),(1.,1.),(1.,
1.),(1.,1.),(1.,1.),(1.,1.),(1.,1.),(1.,1.),(1.,1.),(1.,1.),(1.,1.),(1.,
1.),(1.,1.),(1.,1.),(1.,1.),(1.,1.),(1.,1.),(1.,1.),(1.,1.),(1.,1.),(1.,
1.),(1.,1.),(1.,1.),(1.,1.),(1.,1.),(1.,1.),(1.,1.),(1.,1.),(1.,1.),(1.,
1.),(1.,1.),(1.,1.),(1.,1.),(1.,1.),(1.,1.),(1.,1.),(1.,1.),(1.,1.),(1.,
1.),(1.,1.),(1.,1.),(1.,1.),(1.,1.),(1.,1.),(1.,1.),(1.,1.),(1.,1.),(1.,
1.),(1.,1.)))
REPRESENTATION_ITEM('')
SURFACE()
);
#1032=(
BOUNDED_SURFACE()
B_SPLINE_SURFACE(5,1,((#188698,#188699),(#188700,#188701),(#188702,#188703),
(#188704,#188705),(#188706,#188707),(#188708,#188709),(#188710,#188711),
(#188712,#188713),(#188714,#188715),(#188716,#188717),(#188718,#188719),
(#188720,#188721),(#188722,#188723),(#188724,#188725),(#188726,#188727),
(#188728,#188729),(#188730,#188731),(#188732,#188733),(#188734,#188735),
(#188736,#188737),(#188738,#188739),(#188740,#188741),(#188742,#188743),
(#188744,#188745),(#188746,#188747),(#188748,#188749),(#188750,#188751),
(#188752,#188753),(#188754,#188755),(#188756,#188757),(#188758,#188759),
(#188760,#188761),(#188762,#188763),(#188764,#188765),(#188766,#188767),
(#188768,#188769),(#188770,#188771),(#188772,#188773),(#188774,#188775),
(#188776,#188777),(#188778,#188779),(#188780,#188781),(#188782,#188783),
(#188784,#188785),(#188786,#188787),(#188788,#188789),(#188790,#188791),
(#188792,#188793),(#188794,#188795),(#188796,#188797),(#188798,#188799),
(#188800,#188801),(#188802,#188803),(#188804,#188805),(#188806,#188807),
(#188808,#188809),(#188810,#188811),(#188812,#188813),(#188814,#188815),
(#188816,#188817),(#188818,#188819),(#188820,#188821),(#188822,#188823),
(#188824,#188825),(#188826,#188827),(#188828,#188829),(#188830,#188831),
(#188832,#188833),(#188834,#188835),(#188836,#188837),(#188838,#188839),
(#188840,#188841),(#188842,#188843),(#188844,#188845),(#188846,#188847),
(#188848,#188849),(#188850,#188851),(#188852,#188853),(#188854,#188855),
(#188856,#188857),(#188858,#188859),(#188860,#188861),(#188862,#188863),
(#188864,#188865),(#188866,#188867),(#188868,#188869),(#188870,#188871),
(#188872,#188873),(#188874,#188875),(#188876,#188877),(#188878,#188879),
(#188880,#188881),(#188882,#188883),(#188884,#188885),(#188886,#188887),
(#188888,#188889),(#188890,#188891),(#188892,#188893),(#188894,#188895),
(#188896,#188897),(#188898,#188899),(#188900,#188901),(#188902,#188903),
(#188904,#188905),(#188906,#188907),(#188908,#188909),(#188910,#188911),
(#188912,#188913),(#188914,#188915),(#188916,#188917),(#188918,#188919),
(#188920,#188921),(#188922,#188923),(#188924,#188925),(#188926,#188927),
(#188928,#188929),(#188930,#188931),(#188932,#188933),(#188934,#188935),
(#188936,#188937),(#188938,#188939),(#188940,#188941),(#188942,#188943),
(#188944,#188945),(#188946,#188947),(#188948,#188949),(#188950,#188951),
(#188952,#188953),(#188954,#188955),(#188956,#188957),(#188958,#188959),
(#188960,#188961),(#188962,#188963),(#188964,#188965),(#188966,#188967),
(#188968,#188969),(#188970,#188971),(#188972,#188973),(#188974,#188975),
(#188976,#188977),(#188978,#188979),(#188980,#188981),(#188982,#188983),
(#188984,#188985),(#188986,#188987),(#188988,#188989),(#188990,#188991),
(#188992,#188993),(#188994,#188995),(#188996,#188997),(#188998,#188999),
(#189000,#189001),(#189002,#189003),(#189004,#189005),(#189006,#189007),
(#189008,#189009),(#189010,#189011),(#189012,#189013),(#189014,#189015),
(#189016,#189017),(#189018,#189019),(#189020,#189021),(#189022,#189023),
(#189024,#189025),(#189026,#189027),(#189028,#189029),(#189030,#189031),
(#189032,#189033),(#189034,#189035),(#189036,#189037),(#189038,#189039),
(#189040,#189041),(#189042,#189043),(#189044,#189045),(#189046,#189047),
(#189048,#189049),(#189050,#189051),(#189052,#189053),(#189054,#189055),
(#189056,#189057),(#189058,#189059),(#189060,#189061),(#189062,#189063),
(#189064,#189065),(#189066,#189067),(#189068,#189069),(#189070,#189071),
(#189072,#189073),(#189074,#189075),(#189076,#189077),(#189078,#189079),
(#189080,#189081),(#189082,#189083),(#189084,#189085),(#189086,#189087),
(#189088,#189089),(#189090,#189091),(#189092,#189093),(#189094,#189095),
(#189096,#189097),(#189098,#189099),(#189100,#189101),(#189102,#189103),
(#189104,#189105),(#189106,#189107)),.UNSPECIFIED.,.F.,.F.,.F.)
B_SPLINE_SURFACE_WITH_KNOTS((6,1,1,1,1,1,1,1,1,1,1,1,1,1,1,1,1,1,1,1,1,
1,1,1,1,1,1,1,1,1,1,1,1,1,1,1,1,1,1,1,1,1,1,1,1,1,1,1,1,1,1,1,1,1,1,1,1,
1,1,1,1,1,1,1,1,1,1,1,1,1,1,1,1,1,1,1,1,1,1,1,1,1,1,1,1,1,1,1,1,1,1,1,1,
1,1,1,1,1,1,1,1,1,1,1,1,1,1,1,1,1,1,1,1,1,1,1,1,1,1,1,1,1,1,1,1,1,1,1,1,
1,1,1,1,1,1,1,1,1,1,1,1,1,1,1,1,1,1,1,1,1,1,1,1,1,1,1,1,1,1,1,1,1,1,1,1,
1,1,1,1,1,1,1,1,1,1,1,1,1,1,1,1,1,1,1,1,1,1,1,1,1,1,1,1,1,1,1,1,1,1,1,6),
(2,2),(0.,0.005,0.01,0.015,0.02,0.025,0.03,0.035,0.04,0.045,0.05,0.055,
0.06,0.065,0.07,0.075,0.08,0.085,0.09,0.095,0.1,0.105,0.11,0.115,0.12,0.125,
0.13,0.135,0.14,0.145,0.15,0.155,0.16,0.165,0.17,0.175,0.18,0.185,0.19,
0.195,0.2,0.205,0.21,0.215,0.22,0.225,0.23,0.235,0.24,0.245,0.25,0.255,
0.26,0.265,0.27,0.275,0.28,0.285,0.29,0.295,0.3,0.305,0.31,0.315,0.32,0.325,
0.33,0.335,0.34,0.345,0.35,0.355,0.36,0.365,0.37,0.375,0.38,0.385,0.39,
0.395,0.4,0.405,0.41,0.415,0.42,0.425,0.43,0.435,0.44,0.445,0.45,0.455,
0.46,0.465,0.47,0.475,0.48,0.485,0.49,0.495,0.5,0.505,0.51,0.515,0.52,0.525,
0.53,0.535,0.54,0.545,0.55,0.555,0.56,0.565,0.57,0.575,0.58,0.585,0.59,
0.595,0.6,0.605,0.61,0.615,0.62,0.625,0.63,0.635,0.64,0.645,0.65,0.655,
0.66,0.665,0.67,0.675,0.68,0.685,0.690000000000001,0.695000000000001,0.700000000000001,
0.705000000000001,0.710000000000001,0.715000000000001,0.720000000000001,
0.725000000000001,0.730000000000001,0.735000000000001,0.740000000000001,
0.745000000000001,0.750000000000001,0.755000000000001,0.760000000000001,
0.765000000000001,0.770000000000001,0.775000000000001,0.780000000000001,
0.785000000000001,0.790000000000001,0.795000000000001,0.800000000000001,
0.805000000000001,0.810000000000001,0.815000000000001,0.820000000000001,
0.825000000000001,0.830000000000001,0.835000000000001,0.840000000000001,
0.845000000000001,0.850000000000001,0.855000000000001,0.860000000000001,
0.865000000000001,0.870000000000001,0.875000000000001,0.880000000000001,
0.885000000000001,0.890000000000001,0.895000000000001,0.900000000000001,
0.905000000000001,0.910000000000001,0.915000000000001,0.920000000000001,
0.925000000000001,0.930000000000001,0.935000000000001,0.940000000000001,
0.945000000000001,0.950000000000001,0.955000000000001,0.960000000000001,
0.965000000000001,0.970000000000001,0.975000000000001,0.980000000000001,
0.985000000000001,0.990000000000001,0.995000000000001,1.),(0.,1.2),
 .UNSPECIFIED.)
GEOMETRIC_REPRESENTATION_ITEM()
RATIONAL_B_SPLINE_SURFACE(((1.,1.),(1.,1.),(1.,1.),(1.,1.),(1.,1.),(1.,
1.),(1.,1.),(1.,1.),(1.,1.),(1.,1.),(1.,1.),(1.,1.),(1.,1.),(1.,1.),(1.,
1.),(1.,1.),(1.,1.),(1.,1.),(1.,1.),(1.,1.),(1.,1.),(1.,1.),(1.,1.),(1.,
1.),(1.,1.),(1.,1.),(1.,1.),(1.,1.),(1.,1.),(1.,1.),(1.,1.),(1.,1.),(1.,
1.),(1.,1.),(1.,1.),(1.,1.),(1.,1.),(1.,1.),(1.,1.),(1.,1.),(1.,1.),(1.,
1.),(1.,1.),(1.,1.),(1.,1.),(1.,1.),(1.,1.),(1.,1.),(1.,1.),(1.,1.),(1.,
1.),(1.,1.),(1.,1.),(1.,1.),(1.,1.),(1.,1.),(1.,1.),(1.,1.),(1.,1.),(1.,
1.),(1.,1.),(1.,1.),(1.,1.),(1.,1.),(1.,1.),(1.,1.),(1.,1.),(1.,1.),(1.,
1.),(1.,1.),(1.,1.),(1.,1.),(1.,1.),(1.,1.),(1.,1.),(1.,1.),(1.,1.),(1.,
1.),(1.,1.),(1.,1.),(1.,1.),(1.,1.),(1.,1.),(1.,1.),(1.,1.),(1.,1.),(1.,
1.),(1.,1.),(1.,1.),(1.,1.),(1.,1.),(1.,1.),(1.,1.),(1.,1.),(1.,1.),(1.,
1.),(1.,1.),(1.,1.),(1.,1.),(1.,1.),(1.,1.),(1.,1.),(1.,1.),(1.,1.),(1.,
1.),(1.,1.),(1.,1.),(1.,1.),(1.,1.),(1.,1.),(1.,1.),(1.,1.),(1.,1.),(1.,
1.),(1.,1.),(1.,1.),(1.,1.),(1.,1.),(1.,1.),(1.,1.),(1.,1.),(1.,1.),(1.,
1.),(1.,1.),(1.,1.),(1.,1.),(1.,1.),(1.,1.),(1.,1.),(1.,1.),(1.,1.),(1.,
1.),(1.,1.),(1.,1.),(1.,1.),(1.,1.),(1.,1.),(1.,1.),(1.,1.),(1.,1.),(1.,
1.),(1.,1.),(1.,1.),(1.,1.),(1.,1.),(1.,1.),(1.,1.),(1.,1.),(1.,1.),(1.,
1.),(1.,1.),(1.,1.),(1.,1.),(1.,1.),(1.,1.),(1.,1.),(1.,1.),(1.,1.),(1.,
1.),(1.,1.),(1.,1.),(1.,1.),(1.,1.),(1.,1.),(1.,1.),(1.,1.),(1.,1.),(1.,
1.),(1.,1.),(1.,1.),(1.,1.),(1.,1.),(1.,1.),(1.,1.),(1.,1.),(1.,1.),(1.,
1.),(1.,1.),(1.,1.),(1.,1.),(1.,1.),(1.,1.),(1.,1.),(1.,1.),(1.,1.),(1.,
1.),(1.,1.),(1.,1.),(1.,1.),(1.,1.),(1.,1.),(1.,1.),(1.,1.),(1.,1.),(1.,
1.),(1.,1.),(1.,1.),(1.,1.),(1.,1.),(1.,1.),(1.,1.),(1.,1.),(1.,1.),(1.,
1.),(1.,1.)))
REPRESENTATION_ITEM('')
SURFACE()
);
#1033=(
BOUNDED_SURFACE()
B_SPLINE_SURFACE(5,1,((#189319,#189320),(#189321,#189322),(#189323,#189324),
(#189325,#189326),(#189327,#189328),(#189329,#189330),(#189331,#189332),
(#189333,#189334),(#189335,#189336),(#189337,#189338),(#189339,#189340),
(#189341,#189342),(#189343,#189344),(#189345,#189346),(#189347,#189348),
(#189349,#189350),(#189351,#189352),(#189353,#189354),(#189355,#189356),
(#189357,#189358),(#189359,#189360),(#189361,#189362),(#189363,#189364),
(#189365,#189366),(#189367,#189368),(#189369,#189370),(#189371,#189372),
(#189373,#189374),(#189375,#189376),(#189377,#189378),(#189379,#189380),
(#189381,#189382),(#189383,#189384),(#189385,#189386),(#189387,#189388),
(#189389,#189390),(#189391,#189392),(#189393,#189394),(#189395,#189396),
(#189397,#189398),(#189399,#189400),(#189401,#189402),(#189403,#189404),
(#189405,#189406),(#189407,#189408),(#189409,#189410),(#189411,#189412),
(#189413,#189414),(#189415,#189416),(#189417,#189418),(#189419,#189420),
(#189421,#189422),(#189423,#189424),(#189425,#189426),(#189427,#189428),
(#189429,#189430),(#189431,#189432),(#189433,#189434),(#189435,#189436),
(#189437,#189438),(#189439,#189440),(#189441,#189442),(#189443,#189444),
(#189445,#189446),(#189447,#189448),(#189449,#189450),(#189451,#189452),
(#189453,#189454),(#189455,#189456),(#189457,#189458),(#189459,#189460),
(#189461,#189462),(#189463,#189464),(#189465,#189466),(#189467,#189468),
(#189469,#189470),(#189471,#189472),(#189473,#189474),(#189475,#189476),
(#189477,#189478),(#189479,#189480),(#189481,#189482),(#189483,#189484),
(#189485,#189486),(#189487,#189488),(#189489,#189490),(#189491,#189492),
(#189493,#189494),(#189495,#189496),(#189497,#189498),(#189499,#189500),
(#189501,#189502),(#189503,#189504),(#189505,#189506),(#189507,#189508),
(#189509,#189510),(#189511,#189512),(#189513,#189514),(#189515,#189516),
(#189517,#189518),(#189519,#189520),(#189521,#189522),(#189523,#189524),
(#189525,#189526),(#189527,#189528),(#189529,#189530),(#189531,#189532),
(#189533,#189534),(#189535,#189536),(#189537,#189538),(#189539,#189540),
(#189541,#189542),(#189543,#189544),(#189545,#189546),(#189547,#189548),
(#189549,#189550),(#189551,#189552),(#189553,#189554),(#189555,#189556),
(#189557,#189558),(#189559,#189560),(#189561,#189562),(#189563,#189564),
(#189565,#189566),(#189567,#189568),(#189569,#189570),(#189571,#189572),
(#189573,#189574),(#189575,#189576),(#189577,#189578),(#189579,#189580),
(#189581,#189582),(#189583,#189584),(#189585,#189586),(#189587,#189588),
(#189589,#189590),(#189591,#189592),(#189593,#189594),(#189595,#189596),
(#189597,#189598),(#189599,#189600),(#189601,#189602),(#189603,#189604),
(#189605,#189606),(#189607,#189608),(#189609,#189610),(#189611,#189612),
(#189613,#189614),(#189615,#189616),(#189617,#189618),(#189619,#189620),
(#189621,#189622),(#189623,#189624),(#189625,#189626),(#189627,#189628),
(#189629,#189630),(#189631,#189632),(#189633,#189634),(#189635,#189636),
(#189637,#189638),(#189639,#189640),(#189641,#189642),(#189643,#189644),
(#189645,#189646),(#189647,#189648),(#189649,#189650),(#189651,#189652),
(#189653,#189654),(#189655,#189656),(#189657,#189658),(#189659,#189660),
(#189661,#189662),(#189663,#189664),(#189665,#189666),(#189667,#189668),
(#189669,#189670),(#189671,#189672),(#189673,#189674),(#189675,#189676),
(#189677,#189678),(#189679,#189680),(#189681,#189682),(#189683,#189684),
(#189685,#189686),(#189687,#189688),(#189689,#189690),(#189691,#189692),
(#189693,#189694),(#189695,#189696),(#189697,#189698),(#189699,#189700),
(#189701,#189702),(#189703,#189704),(#189705,#189706),(#189707,#189708),
(#189709,#189710),(#189711,#189712),(#189713,#189714),(#189715,#189716),
(#189717,#189718),(#189719,#189720),(#189721,#189722),(#189723,#189724),
(#189725,#189726),(#189727,#189728)),.UNSPECIFIED.,.F.,.F.,.F.)
B_SPLINE_SURFACE_WITH_KNOTS((6,1,1,1,1,1,1,1,1,1,1,1,1,1,1,1,1,1,1,1,1,
1,1,1,1,1,1,1,1,1,1,1,1,1,1,1,1,1,1,1,1,1,1,1,1,1,1,1,1,1,1,1,1,1,1,1,1,
1,1,1,1,1,1,1,1,1,1,1,1,1,1,1,1,1,1,1,1,1,1,1,1,1,1,1,1,1,1,1,1,1,1,1,1,
1,1,1,1,1,1,1,1,1,1,1,1,1,1,1,1,1,1,1,1,1,1,1,1,1,1,1,1,1,1,1,1,1,1,1,1,
1,1,1,1,1,1,1,1,1,1,1,1,1,1,1,1,1,1,1,1,1,1,1,1,1,1,1,1,1,1,1,1,1,1,1,1,
1,1,1,1,1,1,1,1,1,1,1,1,1,1,1,1,1,1,1,1,1,1,1,1,1,1,1,1,1,1,1,1,1,1,1,6),
(2,2),(-1.,-0.995000000000001,-0.990000000000001,-0.985000000000001,-0.980000000000001,
-0.975000000000001,-0.970000000000001,-0.965000000000001,-0.960000000000001,
-0.955000000000001,-0.950000000000001,-0.945000000000001,-0.940000000000001,
-0.935000000000001,-0.930000000000001,-0.925000000000001,-0.920000000000001,
-0.915000000000001,-0.910000000000001,-0.905000000000001,-0.900000000000001,
-0.895000000000001,-0.890000000000001,-0.885000000000001,-0.880000000000001,
-0.875000000000001,-0.870000000000001,-0.865000000000001,-0.860000000000001,
-0.855000000000001,-0.850000000000001,-0.845000000000001,-0.840000000000001,
-0.835000000000001,-0.830000000000001,-0.825000000000001,-0.820000000000001,
-0.815000000000001,-0.810000000000001,-0.805000000000001,-0.800000000000001,
-0.795000000000001,-0.790000000000001,-0.785000000000001,-0.780000000000001,
-0.775000000000001,-0.770000000000001,-0.765000000000001,-0.760000000000001,
-0.755000000000001,-0.750000000000001,-0.745000000000001,-0.740000000000001,
-0.735000000000001,-0.730000000000001,-0.725000000000001,-0.720000000000001,
-0.715000000000001,-0.710000000000001,-0.705000000000001,-0.700000000000001,
-0.695000000000001,-0.690000000000001,-0.685,-0.68,-0.675,-0.67,-0.665,
-0.66,-0.655,-0.65,-0.645,-0.64,-0.635,-0.63,-0.625,-0.62,-0.615,-0.61,
-0.605,-0.6,-0.595,-0.59,-0.585,-0.58,-0.575,-0.57,-0.565,-0.56,-0.555,
-0.55,-0.545,-0.54,-0.535,-0.53,-0.525,-0.52,-0.515,-0.51,-0.505,-0.5,-0.495,
-0.49,-0.485,-0.48,-0.475,-0.47,-0.465,-0.46,-0.455,-0.45,-0.445,-0.44,
-0.435,-0.43,-0.425,-0.42,-0.415,-0.41,-0.405,-0.4,-0.395,-0.39,-0.385,
-0.38,-0.375,-0.37,-0.365,-0.36,-0.355,-0.35,-0.345,-0.34,-0.335,-0.33,
-0.325,-0.32,-0.315,-0.31,-0.305,-0.3,-0.295,-0.29,-0.285,-0.28,-0.275,
-0.27,-0.265,-0.26,-0.255,-0.25,-0.245,-0.24,-0.235,-0.23,-0.225,-0.22,
-0.215,-0.21,-0.205,-0.2,-0.195,-0.19,-0.185,-0.18,-0.175,-0.17,-0.165,
-0.16,-0.155,-0.15,-0.145,-0.14,-0.135,-0.13,-0.125,-0.12,-0.115,-0.11,
-0.105,-0.1,-0.095,-0.09,-0.085,-0.08,-0.075,-0.07,-0.065,-0.06,-0.055,
-0.05,-0.045,-0.04,-0.035,-0.03,-0.025,-0.02,-0.015,-0.01,-0.005,0.),(0.,
1.2),.UNSPECIFIED.)
GEOMETRIC_REPRESENTATION_ITEM()
RATIONAL_B_SPLINE_SURFACE(((1.,1.),(1.,1.),(1.,1.),(1.,1.),(1.,1.),(1.,
1.),(1.,1.),(1.,1.),(1.,1.),(1.,1.),(1.,1.),(1.,1.),(1.,1.),(1.,1.),(1.,
1.),(1.,1.),(1.,1.),(1.,1.),(1.,1.),(1.,1.),(1.,1.),(1.,1.),(1.,1.),(1.,
1.),(1.,1.),(1.,1.),(1.,1.),(1.,1.),(1.,1.),(1.,1.),(1.,1.),(1.,1.),(1.,
1.),(1.,1.),(1.,1.),(1.,1.),(1.,1.),(1.,1.),(1.,1.),(1.,1.),(1.,1.),(1.,
1.),(1.,1.),(1.,1.),(1.,1.),(1.,1.),(1.,1.),(1.,1.),(1.,1.),(1.,1.),(1.,
1.),(1.,1.),(1.,1.),(1.,1.),(1.,1.),(1.,1.),(1.,1.),(1.,1.),(1.,1.),(1.,
1.),(1.,1.),(1.,1.),(1.,1.),(1.,1.),(1.,1.),(1.,1.),(1.,1.),(1.,1.),(1.,
1.),(1.,1.),(1.,1.),(1.,1.),(1.,1.),(1.,1.),(1.,1.),(1.,1.),(1.,1.),(1.,
1.),(1.,1.),(1.,1.),(1.,1.),(1.,1.),(1.,1.),(1.,1.),(1.,1.),(1.,1.),(1.,
1.),(1.,1.),(1.,1.),(1.,1.),(1.,1.),(1.,1.),(1.,1.),(1.,1.),(1.,1.),(1.,
1.),(1.,1.),(1.,1.),(1.,1.),(1.,1.),(1.,1.),(1.,1.),(1.,1.),(1.,1.),(1.,
1.),(1.,1.),(1.,1.),(1.,1.),(1.,1.),(1.,1.),(1.,1.),(1.,1.),(1.,1.),(1.,
1.),(1.,1.),(1.,1.),(1.,1.),(1.,1.),(1.,1.),(1.,1.),(1.,1.),(1.,1.),(1.,
1.),(1.,1.),(1.,1.),(1.,1.),(1.,1.),(1.,1.),(1.,1.),(1.,1.),(1.,1.),(1.,
1.),(1.,1.),(1.,1.),(1.,1.),(1.,1.),(1.,1.),(1.,1.),(1.,1.),(1.,1.),(1.,
1.),(1.,1.),(1.,1.),(1.,1.),(1.,1.),(1.,1.),(1.,1.),(1.,1.),(1.,1.),(1.,
1.),(1.,1.),(1.,1.),(1.,1.),(1.,1.),(1.,1.),(1.,1.),(1.,1.),(1.,1.),(1.,
1.),(1.,1.),(1.,1.),(1.,1.),(1.,1.),(1.,1.),(1.,1.),(1.,1.),(1.,1.),(1.,
1.),(1.,1.),(1.,1.),(1.,1.),(1.,1.),(1.,1.),(1.,1.),(1.,1.),(1.,1.),(1.,
1.),(1.,1.),(1.,1.),(1.,1.),(1.,1.),(1.,1.),(1.,1.),(1.,1.),(1.,1.),(1.,
1.),(1.,1.),(1.,1.),(1.,1.),(1.,1.),(1.,1.),(1.,1.),(1.,1.),(1.,1.),(1.,
1.),(1.,1.),(1.,1.),(1.,1.),(1.,1.),(1.,1.),(1.,1.),(1.,1.),(1.,1.),(1.,
1.),(1.,1.)))
REPRESENTATION_ITEM('')
SURFACE()
);
#1034=(
BOUNDED_SURFACE()
B_SPLINE_SURFACE(5,1,((#189936,#189937),(#189938,#189939),(#189940,#189941),
(#189942,#189943),(#189944,#189945),(#189946,#189947),(#189948,#189949),
(#189950,#189951),(#189952,#189953),(#189954,#189955),(#189956,#189957),
(#189958,#189959),(#189960,#189961),(#189962,#189963),(#189964,#189965),
(#189966,#189967),(#189968,#189969),(#189970,#189971),(#189972,#189973),
(#189974,#189975),(#189976,#189977),(#189978,#189979),(#189980,#189981),
(#189982,#189983),(#189984,#189985),(#189986,#189987),(#189988,#189989),
(#189990,#189991),(#189992,#189993),(#189994,#189995),(#189996,#189997),
(#189998,#189999),(#190000,#190001),(#190002,#190003),(#190004,#190005),
(#190006,#190007),(#190008,#190009),(#190010,#190011),(#190012,#190013),
(#190014,#190015),(#190016,#190017),(#190018,#190019),(#190020,#190021),
(#190022,#190023),(#190024,#190025),(#190026,#190027),(#190028,#190029),
(#190030,#190031),(#190032,#190033),(#190034,#190035),(#190036,#190037),
(#190038,#190039),(#190040,#190041),(#190042,#190043),(#190044,#190045),
(#190046,#190047),(#190048,#190049),(#190050,#190051),(#190052,#190053),
(#190054,#190055),(#190056,#190057),(#190058,#190059),(#190060,#190061),
(#190062,#190063),(#190064,#190065),(#190066,#190067),(#190068,#190069),
(#190070,#190071),(#190072,#190073),(#190074,#190075),(#190076,#190077),
(#190078,#190079),(#190080,#190081),(#190082,#190083),(#190084,#190085),
(#190086,#190087),(#190088,#190089),(#190090,#190091),(#190092,#190093),
(#190094,#190095),(#190096,#190097),(#190098,#190099),(#190100,#190101),
(#190102,#190103),(#190104,#190105),(#190106,#190107),(#190108,#190109),
(#190110,#190111),(#190112,#190113),(#190114,#190115),(#190116,#190117),
(#190118,#190119),(#190120,#190121),(#190122,#190123),(#190124,#190125),
(#190126,#190127),(#190128,#190129),(#190130,#190131),(#190132,#190133),
(#190134,#190135),(#190136,#190137),(#190138,#190139),(#190140,#190141),
(#190142,#190143),(#190144,#190145),(#190146,#190147),(#190148,#190149),
(#190150,#190151),(#190152,#190153),(#190154,#190155),(#190156,#190157),
(#190158,#190159),(#190160,#190161),(#190162,#190163),(#190164,#190165),
(#190166,#190167),(#190168,#190169),(#190170,#190171),(#190172,#190173),
(#190174,#190175),(#190176,#190177),(#190178,#190179),(#190180,#190181),
(#190182,#190183),(#190184,#190185),(#190186,#190187),(#190188,#190189),
(#190190,#190191),(#190192,#190193),(#190194,#190195),(#190196,#190197),
(#190198,#190199),(#190200,#190201),(#190202,#190203),(#190204,#190205),
(#190206,#190207),(#190208,#190209),(#190210,#190211),(#190212,#190213),
(#190214,#190215),(#190216,#190217),(#190218,#190219),(#190220,#190221),
(#190222,#190223),(#190224,#190225),(#190226,#190227),(#190228,#190229),
(#190230,#190231),(#190232,#190233),(#190234,#190235),(#190236,#190237),
(#190238,#190239),(#190240,#190241),(#190242,#190243),(#190244,#190245),
(#190246,#190247),(#190248,#190249),(#190250,#190251),(#190252,#190253),
(#190254,#190255),(#190256,#190257),(#190258,#190259),(#190260,#190261),
(#190262,#190263),(#190264,#190265),(#190266,#190267),(#190268,#190269),
(#190270,#190271),(#190272,#190273),(#190274,#190275),(#190276,#190277),
(#190278,#190279),(#190280,#190281),(#190282,#190283),(#190284,#190285),
(#190286,#190287),(#190288,#190289),(#190290,#190291),(#190292,#190293),
(#190294,#190295),(#190296,#190297),(#190298,#190299),(#190300,#190301),
(#190302,#190303),(#190304,#190305),(#190306,#190307),(#190308,#190309),
(#190310,#190311),(#190312,#190313),(#190314,#190315),(#190316,#190317),
(#190318,#190319),(#190320,#190321),(#190322,#190323),(#190324,#190325),
(#190326,#190327),(#190328,#190329),(#190330,#190331),(#190332,#190333),
(#190334,#190335),(#190336,#190337),(#190338,#190339),(#190340,#190341),
(#190342,#190343),(#190344,#190345)),.UNSPECIFIED.,.F.,.F.,.F.)
B_SPLINE_SURFACE_WITH_KNOTS((6,1,1,1,1,1,1,1,1,1,1,1,1,1,1,1,1,1,1,1,1,
1,1,1,1,1,1,1,1,1,1,1,1,1,1,1,1,1,1,1,1,1,1,1,1,1,1,1,1,1,1,1,1,1,1,1,1,
1,1,1,1,1,1,1,1,1,1,1,1,1,1,1,1,1,1,1,1,1,1,1,1,1,1,1,1,1,1,1,1,1,1,1,1,
1,1,1,1,1,1,1,1,1,1,1,1,1,1,1,1,1,1,1,1,1,1,1,1,1,1,1,1,1,1,1,1,1,1,1,1,
1,1,1,1,1,1,1,1,1,1,1,1,1,1,1,1,1,1,1,1,1,1,1,1,1,1,1,1,1,1,1,1,1,1,1,1,
1,1,1,1,1,1,1,1,1,1,1,1,1,1,1,1,1,1,1,1,1,1,1,1,1,1,1,1,1,1,1,1,1,1,1,6),
(2,2),(0.,0.005,0.01,0.015,0.02,0.025,0.03,0.035,0.04,0.045,0.05,0.055,
0.06,0.065,0.07,0.075,0.08,0.085,0.09,0.095,0.1,0.105,0.11,0.115,0.12,0.125,
0.13,0.135,0.14,0.145,0.15,0.155,0.16,0.165,0.17,0.175,0.18,0.185,0.19,
0.195,0.2,0.205,0.21,0.215,0.22,0.225,0.23,0.235,0.24,0.245,0.25,0.255,
0.26,0.265,0.27,0.275,0.28,0.285,0.29,0.295,0.3,0.305,0.31,0.315,0.32,0.325,
0.33,0.335,0.34,0.345,0.35,0.355,0.36,0.365,0.37,0.375,0.38,0.385,0.39,
0.395,0.4,0.405,0.41,0.415,0.42,0.425,0.43,0.435,0.44,0.445,0.45,0.455,
0.46,0.465,0.47,0.475,0.48,0.485,0.49,0.495,0.5,0.505,0.51,0.515,0.52,0.525,
0.53,0.535,0.54,0.545,0.55,0.555,0.56,0.565,0.57,0.575,0.58,0.585,0.59,
0.595,0.6,0.605,0.61,0.615,0.62,0.625,0.63,0.635,0.64,0.645,0.65,0.655,
0.66,0.665,0.67,0.675,0.68,0.685,0.690000000000001,0.695000000000001,0.700000000000001,
0.705000000000001,0.710000000000001,0.715000000000001,0.720000000000001,
0.725000000000001,0.730000000000001,0.735000000000001,0.740000000000001,
0.745000000000001,0.750000000000001,0.755000000000001,0.760000000000001,
0.765000000000001,0.770000000000001,0.775000000000001,0.780000000000001,
0.785000000000001,0.790000000000001,0.795000000000001,0.800000000000001,
0.805000000000001,0.810000000000001,0.815000000000001,0.820000000000001,
0.825000000000001,0.830000000000001,0.835000000000001,0.840000000000001,
0.845000000000001,0.850000000000001,0.855000000000001,0.860000000000001,
0.865000000000001,0.870000000000001,0.875000000000001,0.880000000000001,
0.885000000000001,0.890000000000001,0.895000000000001,0.900000000000001,
0.905000000000001,0.910000000000001,0.915000000000001,0.920000000000001,
0.925000000000001,0.930000000000001,0.935000000000001,0.940000000000001,
0.945000000000001,0.950000000000001,0.955000000000001,0.960000000000001,
0.965000000000001,0.970000000000001,0.975000000000001,0.980000000000001,
0.985000000000001,0.990000000000001,0.995000000000001,1.),(0.,1.2),
 .UNSPECIFIED.)
GEOMETRIC_REPRESENTATION_ITEM()
RATIONAL_B_SPLINE_SURFACE(((1.,1.),(1.,1.),(1.,1.),(1.,1.),(1.,1.),(1.,
1.),(1.,1.),(1.,1.),(1.,1.),(1.,1.),(1.,1.),(1.,1.),(1.,1.),(1.,1.),(1.,
1.),(1.,1.),(1.,1.),(1.,1.),(1.,1.),(1.,1.),(1.,1.),(1.,1.),(1.,1.),(1.,
1.),(1.,1.),(1.,1.),(1.,1.),(1.,1.),(1.,1.),(1.,1.),(1.,1.),(1.,1.),(1.,
1.),(1.,1.),(1.,1.),(1.,1.),(1.,1.),(1.,1.),(1.,1.),(1.,1.),(1.,1.),(1.,
1.),(1.,1.),(1.,1.),(1.,1.),(1.,1.),(1.,1.),(1.,1.),(1.,1.),(1.,1.),(1.,
1.),(1.,1.),(1.,1.),(1.,1.),(1.,1.),(1.,1.),(1.,1.),(1.,1.),(1.,1.),(1.,
1.),(1.,1.),(1.,1.),(1.,1.),(1.,1.),(1.,1.),(1.,1.),(1.,1.),(1.,1.),(1.,
1.),(1.,1.),(1.,1.),(1.,1.),(1.,1.),(1.,1.),(1.,1.),(1.,1.),(1.,1.),(1.,
1.),(1.,1.),(1.,1.),(1.,1.),(1.,1.),(1.,1.),(1.,1.),(1.,1.),(1.,1.),(1.,
1.),(1.,1.),(1.,1.),(1.,1.),(1.,1.),(1.,1.),(1.,1.),(1.,1.),(1.,1.),(1.,
1.),(1.,1.),(1.,1.),(1.,1.),(1.,1.),(1.,1.),(1.,1.),(1.,1.),(1.,1.),(1.,
1.),(1.,1.),(1.,1.),(1.,1.),(1.,1.),(1.,1.),(1.,1.),(1.,1.),(1.,1.),(1.,
1.),(1.,1.),(1.,1.),(1.,1.),(1.,1.),(1.,1.),(1.,1.),(1.,1.),(1.,1.),(1.,
1.),(1.,1.),(1.,1.),(1.,1.),(1.,1.),(1.,1.),(1.,1.),(1.,1.),(1.,1.),(1.,
1.),(1.,1.),(1.,1.),(1.,1.),(1.,1.),(1.,1.),(1.,1.),(1.,1.),(1.,1.),(1.,
1.),(1.,1.),(1.,1.),(1.,1.),(1.,1.),(1.,1.),(1.,1.),(1.,1.),(1.,1.),(1.,
1.),(1.,1.),(1.,1.),(1.,1.),(1.,1.),(1.,1.),(1.,1.),(1.,1.),(1.,1.),(1.,
1.),(1.,1.),(1.,1.),(1.,1.),(1.,1.),(1.,1.),(1.,1.),(1.,1.),(1.,1.),(1.,
1.),(1.,1.),(1.,1.),(1.,1.),(1.,1.),(1.,1.),(1.,1.),(1.,1.),(1.,1.),(1.,
1.),(1.,1.),(1.,1.),(1.,1.),(1.,1.),(1.,1.),(1.,1.),(1.,1.),(1.,1.),(1.,
1.),(1.,1.),(1.,1.),(1.,1.),(1.,1.),(1.,1.),(1.,1.),(1.,1.),(1.,1.),(1.,
1.),(1.,1.),(1.,1.),(1.,1.),(1.,1.),(1.,1.),(1.,1.),(1.,1.),(1.,1.),(1.,
1.),(1.,1.)))
REPRESENTATION_ITEM('')
SURFACE()
);
#1035=(
BOUNDED_SURFACE()
B_SPLINE_SURFACE(5,1,((#190557,#190558),(#190559,#190560),(#190561,#190562),
(#190563,#190564),(#190565,#190566),(#190567,#190568),(#190569,#190570),
(#190571,#190572),(#190573,#190574),(#190575,#190576),(#190577,#190578),
(#190579,#190580),(#190581,#190582),(#190583,#190584),(#190585,#190586),
(#190587,#190588),(#190589,#190590),(#190591,#190592),(#190593,#190594),
(#190595,#190596),(#190597,#190598),(#190599,#190600),(#190601,#190602),
(#190603,#190604),(#190605,#190606),(#190607,#190608),(#190609,#190610),
(#190611,#190612),(#190613,#190614),(#190615,#190616),(#190617,#190618),
(#190619,#190620),(#190621,#190622),(#190623,#190624),(#190625,#190626),
(#190627,#190628),(#190629,#190630),(#190631,#190632),(#190633,#190634),
(#190635,#190636),(#190637,#190638),(#190639,#190640),(#190641,#190642),
(#190643,#190644),(#190645,#190646),(#190647,#190648),(#190649,#190650),
(#190651,#190652),(#190653,#190654),(#190655,#190656),(#190657,#190658),
(#190659,#190660),(#190661,#190662),(#190663,#190664),(#190665,#190666),
(#190667,#190668),(#190669,#190670),(#190671,#190672),(#190673,#190674),
(#190675,#190676),(#190677,#190678),(#190679,#190680),(#190681,#190682),
(#190683,#190684),(#190685,#190686),(#190687,#190688),(#190689,#190690),
(#190691,#190692),(#190693,#190694),(#190695,#190696),(#190697,#190698),
(#190699,#190700),(#190701,#190702),(#190703,#190704),(#190705,#190706),
(#190707,#190708),(#190709,#190710),(#190711,#190712),(#190713,#190714),
(#190715,#190716),(#190717,#190718),(#190719,#190720),(#190721,#190722),
(#190723,#190724),(#190725,#190726),(#190727,#190728),(#190729,#190730),
(#190731,#190732),(#190733,#190734),(#190735,#190736),(#190737,#190738),
(#190739,#190740),(#190741,#190742),(#190743,#190744),(#190745,#190746),
(#190747,#190748),(#190749,#190750),(#190751,#190752),(#190753,#190754),
(#190755,#190756),(#190757,#190758),(#190759,#190760),(#190761,#190762),
(#190763,#190764),(#190765,#190766),(#190767,#190768),(#190769,#190770),
(#190771,#190772),(#190773,#190774),(#190775,#190776),(#190777,#190778),
(#190779,#190780),(#190781,#190782),(#190783,#190784),(#190785,#190786),
(#190787,#190788),(#190789,#190790),(#190791,#190792),(#190793,#190794),
(#190795,#190796),(#190797,#190798),(#190799,#190800),(#190801,#190802),
(#190803,#190804),(#190805,#190806),(#190807,#190808),(#190809,#190810),
(#190811,#190812),(#190813,#190814),(#190815,#190816),(#190817,#190818),
(#190819,#190820),(#190821,#190822),(#190823,#190824),(#190825,#190826),
(#190827,#190828),(#190829,#190830),(#190831,#190832),(#190833,#190834),
(#190835,#190836),(#190837,#190838),(#190839,#190840),(#190841,#190842),
(#190843,#190844),(#190845,#190846),(#190847,#190848),(#190849,#190850),
(#190851,#190852),(#190853,#190854),(#190855,#190856),(#190857,#190858),
(#190859,#190860),(#190861,#190862),(#190863,#190864),(#190865,#190866),
(#190867,#190868),(#190869,#190870),(#190871,#190872),(#190873,#190874),
(#190875,#190876),(#190877,#190878),(#190879,#190880),(#190881,#190882),
(#190883,#190884),(#190885,#190886),(#190887,#190888),(#190889,#190890),
(#190891,#190892),(#190893,#190894),(#190895,#190896),(#190897,#190898),
(#190899,#190900),(#190901,#190902),(#190903,#190904),(#190905,#190906),
(#190907,#190908),(#190909,#190910),(#190911,#190912),(#190913,#190914),
(#190915,#190916),(#190917,#190918),(#190919,#190920),(#190921,#190922),
(#190923,#190924),(#190925,#190926),(#190927,#190928),(#190929,#190930),
(#190931,#190932),(#190933,#190934),(#190935,#190936),(#190937,#190938),
(#190939,#190940),(#190941,#190942),(#190943,#190944),(#190945,#190946),
(#190947,#190948),(#190949,#190950),(#190951,#190952),(#190953,#190954),
(#190955,#190956),(#190957,#190958),(#190959,#190960),(#190961,#190962),
(#190963,#190964),(#190965,#190966)),.UNSPECIFIED.,.F.,.F.,.F.)
B_SPLINE_SURFACE_WITH_KNOTS((6,1,1,1,1,1,1,1,1,1,1,1,1,1,1,1,1,1,1,1,1,
1,1,1,1,1,1,1,1,1,1,1,1,1,1,1,1,1,1,1,1,1,1,1,1,1,1,1,1,1,1,1,1,1,1,1,1,
1,1,1,1,1,1,1,1,1,1,1,1,1,1,1,1,1,1,1,1,1,1,1,1,1,1,1,1,1,1,1,1,1,1,1,1,
1,1,1,1,1,1,1,1,1,1,1,1,1,1,1,1,1,1,1,1,1,1,1,1,1,1,1,1,1,1,1,1,1,1,1,1,
1,1,1,1,1,1,1,1,1,1,1,1,1,1,1,1,1,1,1,1,1,1,1,1,1,1,1,1,1,1,1,1,1,1,1,1,
1,1,1,1,1,1,1,1,1,1,1,1,1,1,1,1,1,1,1,1,1,1,1,1,1,1,1,1,1,1,1,1,1,1,1,6),
(2,2),(-1.,-0.995000000000001,-0.990000000000001,-0.985000000000001,-0.980000000000001,
-0.975000000000001,-0.970000000000001,-0.965000000000001,-0.960000000000001,
-0.955000000000001,-0.950000000000001,-0.945000000000001,-0.940000000000001,
-0.935000000000001,-0.930000000000001,-0.925000000000001,-0.920000000000001,
-0.915000000000001,-0.910000000000001,-0.905000000000001,-0.900000000000001,
-0.895000000000001,-0.890000000000001,-0.885000000000001,-0.880000000000001,
-0.875000000000001,-0.870000000000001,-0.865000000000001,-0.860000000000001,
-0.855000000000001,-0.850000000000001,-0.845000000000001,-0.840000000000001,
-0.835000000000001,-0.830000000000001,-0.825000000000001,-0.820000000000001,
-0.815000000000001,-0.810000000000001,-0.805000000000001,-0.800000000000001,
-0.795000000000001,-0.790000000000001,-0.785000000000001,-0.780000000000001,
-0.775000000000001,-0.770000000000001,-0.765000000000001,-0.760000000000001,
-0.755000000000001,-0.750000000000001,-0.745000000000001,-0.740000000000001,
-0.735000000000001,-0.730000000000001,-0.725000000000001,-0.720000000000001,
-0.715000000000001,-0.710000000000001,-0.705000000000001,-0.700000000000001,
-0.695000000000001,-0.690000000000001,-0.685,-0.68,-0.675,-0.67,-0.665,
-0.66,-0.655,-0.65,-0.645,-0.64,-0.635,-0.63,-0.625,-0.62,-0.615,-0.61,
-0.605,-0.6,-0.595,-0.59,-0.585,-0.58,-0.575,-0.57,-0.565,-0.56,-0.555,
-0.55,-0.545,-0.54,-0.535,-0.53,-0.525,-0.52,-0.515,-0.51,-0.505,-0.5,-0.495,
-0.49,-0.485,-0.48,-0.475,-0.47,-0.465,-0.46,-0.455,-0.45,-0.445,-0.44,
-0.435,-0.43,-0.425,-0.42,-0.415,-0.41,-0.405,-0.4,-0.395,-0.39,-0.385,
-0.38,-0.375,-0.37,-0.365,-0.36,-0.355,-0.35,-0.345,-0.34,-0.335,-0.33,
-0.325,-0.32,-0.315,-0.31,-0.305,-0.3,-0.295,-0.29,-0.285,-0.28,-0.275,
-0.27,-0.265,-0.26,-0.255,-0.25,-0.245,-0.24,-0.235,-0.23,-0.225,-0.22,
-0.215,-0.21,-0.205,-0.2,-0.195,-0.19,-0.185,-0.18,-0.175,-0.17,-0.165,
-0.16,-0.155,-0.15,-0.145,-0.14,-0.135,-0.13,-0.125,-0.12,-0.115,-0.11,
-0.105,-0.1,-0.095,-0.09,-0.085,-0.08,-0.075,-0.07,-0.065,-0.06,-0.055,
-0.05,-0.045,-0.04,-0.035,-0.03,-0.025,-0.02,-0.015,-0.01,-0.005,0.),(0.,
1.2),.UNSPECIFIED.)
GEOMETRIC_REPRESENTATION_ITEM()
RATIONAL_B_SPLINE_SURFACE(((1.,1.),(1.,1.),(1.,1.),(1.,1.),(1.,1.),(1.,
1.),(1.,1.),(1.,1.),(1.,1.),(1.,1.),(1.,1.),(1.,1.),(1.,1.),(1.,1.),(1.,
1.),(1.,1.),(1.,1.),(1.,1.),(1.,1.),(1.,1.),(1.,1.),(1.,1.),(1.,1.),(1.,
1.),(1.,1.),(1.,1.),(1.,1.),(1.,1.),(1.,1.),(1.,1.),(1.,1.),(1.,1.),(1.,
1.),(1.,1.),(1.,1.),(1.,1.),(1.,1.),(1.,1.),(1.,1.),(1.,1.),(1.,1.),(1.,
1.),(1.,1.),(1.,1.),(1.,1.),(1.,1.),(1.,1.),(1.,1.),(1.,1.),(1.,1.),(1.,
1.),(1.,1.),(1.,1.),(1.,1.),(1.,1.),(1.,1.),(1.,1.),(1.,1.),(1.,1.),(1.,
1.),(1.,1.),(1.,1.),(1.,1.),(1.,1.),(1.,1.),(1.,1.),(1.,1.),(1.,1.),(1.,
1.),(1.,1.),(1.,1.),(1.,1.),(1.,1.),(1.,1.),(1.,1.),(1.,1.),(1.,1.),(1.,
1.),(1.,1.),(1.,1.),(1.,1.),(1.,1.),(1.,1.),(1.,1.),(1.,1.),(1.,1.),(1.,
1.),(1.,1.),(1.,1.),(1.,1.),(1.,1.),(1.,1.),(1.,1.),(1.,1.),(1.,1.),(1.,
1.),(1.,1.),(1.,1.),(1.,1.),(1.,1.),(1.,1.),(1.,1.),(1.,1.),(1.,1.),(1.,
1.),(1.,1.),(1.,1.),(1.,1.),(1.,1.),(1.,1.),(1.,1.),(1.,1.),(1.,1.),(1.,
1.),(1.,1.),(1.,1.),(1.,1.),(1.,1.),(1.,1.),(1.,1.),(1.,1.),(1.,1.),(1.,
1.),(1.,1.),(1.,1.),(1.,1.),(1.,1.),(1.,1.),(1.,1.),(1.,1.),(1.,1.),(1.,
1.),(1.,1.),(1.,1.),(1.,1.),(1.,1.),(1.,1.),(1.,1.),(1.,1.),(1.,1.),(1.,
1.),(1.,1.),(1.,1.),(1.,1.),(1.,1.),(1.,1.),(1.,1.),(1.,1.),(1.,1.),(1.,
1.),(1.,1.),(1.,1.),(1.,1.),(1.,1.),(1.,1.),(1.,1.),(1.,1.),(1.,1.),(1.,
1.),(1.,1.),(1.,1.),(1.,1.),(1.,1.),(1.,1.),(1.,1.),(1.,1.),(1.,1.),(1.,
1.),(1.,1.),(1.,1.),(1.,1.),(1.,1.),(1.,1.),(1.,1.),(1.,1.),(1.,1.),(1.,
1.),(1.,1.),(1.,1.),(1.,1.),(1.,1.),(1.,1.),(1.,1.),(1.,1.),(1.,1.),(1.,
1.),(1.,1.),(1.,1.),(1.,1.),(1.,1.),(1.,1.),(1.,1.),(1.,1.),(1.,1.),(1.,
1.),(1.,1.),(1.,1.),(1.,1.),(1.,1.),(1.,1.),(1.,1.),(1.,1.),(1.,1.),(1.,
1.),(1.,1.)))
REPRESENTATION_ITEM('')
SURFACE()
);
#1036=(
BOUNDED_SURFACE()
B_SPLINE_SURFACE(5,1,((#191174,#191175),(#191176,#191177),(#191178,#191179),
(#191180,#191181),(#191182,#191183),(#191184,#191185),(#191186,#191187),
(#191188,#191189),(#191190,#191191),(#191192,#191193),(#191194,#191195),
(#191196,#191197),(#191198,#191199),(#191200,#191201),(#191202,#191203),
(#191204,#191205),(#191206,#191207),(#191208,#191209),(#191210,#191211),
(#191212,#191213),(#191214,#191215),(#191216,#191217),(#191218,#191219),
(#191220,#191221),(#191222,#191223),(#191224,#191225),(#191226,#191227),
(#191228,#191229),(#191230,#191231),(#191232,#191233),(#191234,#191235),
(#191236,#191237),(#191238,#191239),(#191240,#191241),(#191242,#191243),
(#191244,#191245),(#191246,#191247),(#191248,#191249),(#191250,#191251),
(#191252,#191253),(#191254,#191255),(#191256,#191257),(#191258,#191259),
(#191260,#191261),(#191262,#191263),(#191264,#191265),(#191266,#191267),
(#191268,#191269),(#191270,#191271),(#191272,#191273),(#191274,#191275),
(#191276,#191277),(#191278,#191279),(#191280,#191281),(#191282,#191283),
(#191284,#191285),(#191286,#191287),(#191288,#191289),(#191290,#191291),
(#191292,#191293),(#191294,#191295),(#191296,#191297),(#191298,#191299),
(#191300,#191301),(#191302,#191303),(#191304,#191305),(#191306,#191307),
(#191308,#191309),(#191310,#191311),(#191312,#191313),(#191314,#191315),
(#191316,#191317),(#191318,#191319),(#191320,#191321),(#191322,#191323),
(#191324,#191325),(#191326,#191327),(#191328,#191329),(#191330,#191331),
(#191332,#191333),(#191334,#191335),(#191336,#191337),(#191338,#191339),
(#191340,#191341),(#191342,#191343),(#191344,#191345),(#191346,#191347),
(#191348,#191349),(#191350,#191351),(#191352,#191353),(#191354,#191355),
(#191356,#191357),(#191358,#191359),(#191360,#191361),(#191362,#191363),
(#191364,#191365),(#191366,#191367),(#191368,#191369),(#191370,#191371),
(#191372,#191373),(#191374,#191375),(#191376,#191377),(#191378,#191379),
(#191380,#191381),(#191382,#191383),(#191384,#191385),(#191386,#191387),
(#191388,#191389),(#191390,#191391),(#191392,#191393),(#191394,#191395),
(#191396,#191397),(#191398,#191399),(#191400,#191401),(#191402,#191403),
(#191404,#191405),(#191406,#191407),(#191408,#191409),(#191410,#191411),
(#191412,#191413),(#191414,#191415),(#191416,#191417),(#191418,#191419),
(#191420,#191421),(#191422,#191423),(#191424,#191425),(#191426,#191427),
(#191428,#191429),(#191430,#191431),(#191432,#191433),(#191434,#191435),
(#191436,#191437),(#191438,#191439),(#191440,#191441),(#191442,#191443),
(#191444,#191445),(#191446,#191447),(#191448,#191449),(#191450,#191451),
(#191452,#191453),(#191454,#191455),(#191456,#191457),(#191458,#191459),
(#191460,#191461),(#191462,#191463),(#191464,#191465),(#191466,#191467),
(#191468,#191469),(#191470,#191471),(#191472,#191473),(#191474,#191475),
(#191476,#191477),(#191478,#191479),(#191480,#191481),(#191482,#191483),
(#191484,#191485),(#191486,#191487),(#191488,#191489),(#191490,#191491),
(#191492,#191493),(#191494,#191495),(#191496,#191497),(#191498,#191499),
(#191500,#191501),(#191502,#191503),(#191504,#191505),(#191506,#191507),
(#191508,#191509),(#191510,#191511),(#191512,#191513),(#191514,#191515),
(#191516,#191517),(#191518,#191519),(#191520,#191521),(#191522,#191523),
(#191524,#191525),(#191526,#191527),(#191528,#191529),(#191530,#191531),
(#191532,#191533),(#191534,#191535),(#191536,#191537),(#191538,#191539),
(#191540,#191541),(#191542,#191543),(#191544,#191545),(#191546,#191547),
(#191548,#191549),(#191550,#191551),(#191552,#191553),(#191554,#191555),
(#191556,#191557),(#191558,#191559),(#191560,#191561),(#191562,#191563),
(#191564,#191565),(#191566,#191567),(#191568,#191569),(#191570,#191571),
(#191572,#191573),(#191574,#191575),(#191576,#191577),(#191578,#191579),
(#191580,#191581),(#191582,#191583)),.UNSPECIFIED.,.F.,.F.,.F.)
B_SPLINE_SURFACE_WITH_KNOTS((6,1,1,1,1,1,1,1,1,1,1,1,1,1,1,1,1,1,1,1,1,
1,1,1,1,1,1,1,1,1,1,1,1,1,1,1,1,1,1,1,1,1,1,1,1,1,1,1,1,1,1,1,1,1,1,1,1,
1,1,1,1,1,1,1,1,1,1,1,1,1,1,1,1,1,1,1,1,1,1,1,1,1,1,1,1,1,1,1,1,1,1,1,1,
1,1,1,1,1,1,1,1,1,1,1,1,1,1,1,1,1,1,1,1,1,1,1,1,1,1,1,1,1,1,1,1,1,1,1,1,
1,1,1,1,1,1,1,1,1,1,1,1,1,1,1,1,1,1,1,1,1,1,1,1,1,1,1,1,1,1,1,1,1,1,1,1,
1,1,1,1,1,1,1,1,1,1,1,1,1,1,1,1,1,1,1,1,1,1,1,1,1,1,1,1,1,1,1,1,1,1,1,6),
(2,2),(0.,0.005,0.01,0.015,0.02,0.025,0.03,0.035,0.04,0.045,0.05,0.055,
0.06,0.065,0.07,0.075,0.08,0.085,0.09,0.095,0.1,0.105,0.11,0.115,0.12,0.125,
0.13,0.135,0.14,0.145,0.15,0.155,0.16,0.165,0.17,0.175,0.18,0.185,0.19,
0.195,0.2,0.205,0.21,0.215,0.22,0.225,0.23,0.235,0.24,0.245,0.25,0.255,
0.26,0.265,0.27,0.275,0.28,0.285,0.29,0.295,0.3,0.305,0.31,0.315,0.32,0.325,
0.33,0.335,0.34,0.345,0.35,0.355,0.36,0.365,0.37,0.375,0.38,0.385,0.39,
0.395,0.4,0.405,0.41,0.415,0.42,0.425,0.43,0.435,0.44,0.445,0.45,0.455,
0.46,0.465,0.47,0.475,0.48,0.485,0.49,0.495,0.5,0.505,0.51,0.515,0.52,0.525,
0.53,0.535,0.54,0.545,0.55,0.555,0.56,0.565,0.57,0.575,0.58,0.585,0.59,
0.595,0.6,0.605,0.61,0.615,0.62,0.625,0.63,0.635,0.64,0.645,0.65,0.655,
0.66,0.665,0.67,0.675,0.68,0.685,0.690000000000001,0.695000000000001,0.700000000000001,
0.705000000000001,0.710000000000001,0.715000000000001,0.720000000000001,
0.725000000000001,0.730000000000001,0.735000000000001,0.740000000000001,
0.745000000000001,0.750000000000001,0.755000000000001,0.760000000000001,
0.765000000000001,0.770000000000001,0.775000000000001,0.780000000000001,
0.785000000000001,0.790000000000001,0.795000000000001,0.800000000000001,
0.805000000000001,0.810000000000001,0.815000000000001,0.820000000000001,
0.825000000000001,0.830000000000001,0.835000000000001,0.840000000000001,
0.845000000000001,0.850000000000001,0.855000000000001,0.860000000000001,
0.865000000000001,0.870000000000001,0.875000000000001,0.880000000000001,
0.885000000000001,0.890000000000001,0.895000000000001,0.900000000000001,
0.905000000000001,0.910000000000001,0.915000000000001,0.920000000000001,
0.925000000000001,0.930000000000001,0.935000000000001,0.940000000000001,
0.945000000000001,0.950000000000001,0.955000000000001,0.960000000000001,
0.965000000000001,0.970000000000001,0.975000000000001,0.980000000000001,
0.985000000000001,0.990000000000001,0.995000000000001,1.),(0.,1.2),
 .UNSPECIFIED.)
GEOMETRIC_REPRESENTATION_ITEM()
RATIONAL_B_SPLINE_SURFACE(((1.,1.),(1.,1.),(1.,1.),(1.,1.),(1.,1.),(1.,
1.),(1.,1.),(1.,1.),(1.,1.),(1.,1.),(1.,1.),(1.,1.),(1.,1.),(1.,1.),(1.,
1.),(1.,1.),(1.,1.),(1.,1.),(1.,1.),(1.,1.),(1.,1.),(1.,1.),(1.,1.),(1.,
1.),(1.,1.),(1.,1.),(1.,1.),(1.,1.),(1.,1.),(1.,1.),(1.,1.),(1.,1.),(1.,
1.),(1.,1.),(1.,1.),(1.,1.),(1.,1.),(1.,1.),(1.,1.),(1.,1.),(1.,1.),(1.,
1.),(1.,1.),(1.,1.),(1.,1.),(1.,1.),(1.,1.),(1.,1.),(1.,1.),(1.,1.),(1.,
1.),(1.,1.),(1.,1.),(1.,1.),(1.,1.),(1.,1.),(1.,1.),(1.,1.),(1.,1.),(1.,
1.),(1.,1.),(1.,1.),(1.,1.),(1.,1.),(1.,1.),(1.,1.),(1.,1.),(1.,1.),(1.,
1.),(1.,1.),(1.,1.),(1.,1.),(1.,1.),(1.,1.),(1.,1.),(1.,1.),(1.,1.),(1.,
1.),(1.,1.),(1.,1.),(1.,1.),(1.,1.),(1.,1.),(1.,1.),(1.,1.),(1.,1.),(1.,
1.),(1.,1.),(1.,1.),(1.,1.),(1.,1.),(1.,1.),(1.,1.),(1.,1.),(1.,1.),(1.,
1.),(1.,1.),(1.,1.),(1.,1.),(1.,1.),(1.,1.),(1.,1.),(1.,1.),(1.,1.),(1.,
1.),(1.,1.),(1.,1.),(1.,1.),(1.,1.),(1.,1.),(1.,1.),(1.,1.),(1.,1.),(1.,
1.),(1.,1.),(1.,1.),(1.,1.),(1.,1.),(1.,1.),(1.,1.),(1.,1.),(1.,1.),(1.,
1.),(1.,1.),(1.,1.),(1.,1.),(1.,1.),(1.,1.),(1.,1.),(1.,1.),(1.,1.),(1.,
1.),(1.,1.),(1.,1.),(1.,1.),(1.,1.),(1.,1.),(1.,1.),(1.,1.),(1.,1.),(1.,
1.),(1.,1.),(1.,1.),(1.,1.),(1.,1.),(1.,1.),(1.,1.),(1.,1.),(1.,1.),(1.,
1.),(1.,1.),(1.,1.),(1.,1.),(1.,1.),(1.,1.),(1.,1.),(1.,1.),(1.,1.),(1.,
1.),(1.,1.),(1.,1.),(1.,1.),(1.,1.),(1.,1.),(1.,1.),(1.,1.),(1.,1.),(1.,
1.),(1.,1.),(1.,1.),(1.,1.),(1.,1.),(1.,1.),(1.,1.),(1.,1.),(1.,1.),(1.,
1.),(1.,1.),(1.,1.),(1.,1.),(1.,1.),(1.,1.),(1.,1.),(1.,1.),(1.,1.),(1.,
1.),(1.,1.),(1.,1.),(1.,1.),(1.,1.),(1.,1.),(1.,1.),(1.,1.),(1.,1.),(1.,
1.),(1.,1.),(1.,1.),(1.,1.),(1.,1.),(1.,1.),(1.,1.),(1.,1.),(1.,1.),(1.,
1.),(1.,1.)))
REPRESENTATION_ITEM('')
SURFACE()
);
#1037=(
BOUNDED_SURFACE()
B_SPLINE_SURFACE(5,1,((#191795,#191796),(#191797,#191798),(#191799,#191800),
(#191801,#191802),(#191803,#191804),(#191805,#191806),(#191807,#191808),
(#191809,#191810),(#191811,#191812),(#191813,#191814),(#191815,#191816),
(#191817,#191818),(#191819,#191820),(#191821,#191822),(#191823,#191824),
(#191825,#191826),(#191827,#191828),(#191829,#191830),(#191831,#191832),
(#191833,#191834),(#191835,#191836),(#191837,#191838),(#191839,#191840),
(#191841,#191842),(#191843,#191844),(#191845,#191846),(#191847,#191848),
(#191849,#191850),(#191851,#191852),(#191853,#191854),(#191855,#191856),
(#191857,#191858),(#191859,#191860),(#191861,#191862),(#191863,#191864),
(#191865,#191866),(#191867,#191868),(#191869,#191870),(#191871,#191872),
(#191873,#191874),(#191875,#191876),(#191877,#191878),(#191879,#191880),
(#191881,#191882),(#191883,#191884),(#191885,#191886),(#191887,#191888),
(#191889,#191890),(#191891,#191892),(#191893,#191894),(#191895,#191896),
(#191897,#191898),(#191899,#191900),(#191901,#191902),(#191903,#191904),
(#191905,#191906),(#191907,#191908),(#191909,#191910),(#191911,#191912),
(#191913,#191914),(#191915,#191916),(#191917,#191918),(#191919,#191920),
(#191921,#191922),(#191923,#191924),(#191925,#191926),(#191927,#191928),
(#191929,#191930),(#191931,#191932),(#191933,#191934),(#191935,#191936),
(#191937,#191938),(#191939,#191940),(#191941,#191942),(#191943,#191944),
(#191945,#191946),(#191947,#191948),(#191949,#191950),(#191951,#191952),
(#191953,#191954),(#191955,#191956),(#191957,#191958),(#191959,#191960),
(#191961,#191962),(#191963,#191964),(#191965,#191966),(#191967,#191968),
(#191969,#191970),(#191971,#191972),(#191973,#191974),(#191975,#191976),
(#191977,#191978),(#191979,#191980),(#191981,#191982),(#191983,#191984),
(#191985,#191986),(#191987,#191988),(#191989,#191990),(#191991,#191992),
(#191993,#191994),(#191995,#191996),(#191997,#191998),(#191999,#192000),
(#192001,#192002),(#192003,#192004),(#192005,#192006),(#192007,#192008),
(#192009,#192010),(#192011,#192012),(#192013,#192014),(#192015,#192016),
(#192017,#192018),(#192019,#192020),(#192021,#192022),(#192023,#192024),
(#192025,#192026),(#192027,#192028),(#192029,#192030),(#192031,#192032),
(#192033,#192034),(#192035,#192036),(#192037,#192038),(#192039,#192040),
(#192041,#192042),(#192043,#192044),(#192045,#192046),(#192047,#192048),
(#192049,#192050),(#192051,#192052),(#192053,#192054),(#192055,#192056),
(#192057,#192058),(#192059,#192060),(#192061,#192062),(#192063,#192064),
(#192065,#192066),(#192067,#192068),(#192069,#192070),(#192071,#192072),
(#192073,#192074),(#192075,#192076),(#192077,#192078),(#192079,#192080),
(#192081,#192082),(#192083,#192084),(#192085,#192086),(#192087,#192088),
(#192089,#192090),(#192091,#192092),(#192093,#192094),(#192095,#192096),
(#192097,#192098),(#192099,#192100),(#192101,#192102),(#192103,#192104),
(#192105,#192106),(#192107,#192108),(#192109,#192110),(#192111,#192112),
(#192113,#192114),(#192115,#192116),(#192117,#192118),(#192119,#192120),
(#192121,#192122),(#192123,#192124),(#192125,#192126),(#192127,#192128),
(#192129,#192130),(#192131,#192132),(#192133,#192134),(#192135,#192136),
(#192137,#192138),(#192139,#192140),(#192141,#192142),(#192143,#192144),
(#192145,#192146),(#192147,#192148),(#192149,#192150),(#192151,#192152),
(#192153,#192154),(#192155,#192156),(#192157,#192158),(#192159,#192160),
(#192161,#192162),(#192163,#192164),(#192165,#192166),(#192167,#192168),
(#192169,#192170),(#192171,#192172),(#192173,#192174),(#192175,#192176),
(#192177,#192178),(#192179,#192180),(#192181,#192182),(#192183,#192184),
(#192185,#192186),(#192187,#192188),(#192189,#192190),(#192191,#192192),
(#192193,#192194),(#192195,#192196),(#192197,#192198),(#192199,#192200),
(#192201,#192202),(#192203,#192204)),.UNSPECIFIED.,.F.,.F.,.F.)
B_SPLINE_SURFACE_WITH_KNOTS((6,1,1,1,1,1,1,1,1,1,1,1,1,1,1,1,1,1,1,1,1,
1,1,1,1,1,1,1,1,1,1,1,1,1,1,1,1,1,1,1,1,1,1,1,1,1,1,1,1,1,1,1,1,1,1,1,1,
1,1,1,1,1,1,1,1,1,1,1,1,1,1,1,1,1,1,1,1,1,1,1,1,1,1,1,1,1,1,1,1,1,1,1,1,
1,1,1,1,1,1,1,1,1,1,1,1,1,1,1,1,1,1,1,1,1,1,1,1,1,1,1,1,1,1,1,1,1,1,1,1,
1,1,1,1,1,1,1,1,1,1,1,1,1,1,1,1,1,1,1,1,1,1,1,1,1,1,1,1,1,1,1,1,1,1,1,1,
1,1,1,1,1,1,1,1,1,1,1,1,1,1,1,1,1,1,1,1,1,1,1,1,1,1,1,1,1,1,1,1,1,1,1,6),
(2,2),(-1.,-0.995000000000001,-0.990000000000001,-0.985000000000001,-0.980000000000001,
-0.975000000000001,-0.970000000000001,-0.965000000000001,-0.960000000000001,
-0.955000000000001,-0.950000000000001,-0.945000000000001,-0.940000000000001,
-0.935000000000001,-0.930000000000001,-0.925000000000001,-0.920000000000001,
-0.915000000000001,-0.910000000000001,-0.905000000000001,-0.900000000000001,
-0.895000000000001,-0.890000000000001,-0.885000000000001,-0.880000000000001,
-0.875000000000001,-0.870000000000001,-0.865000000000001,-0.860000000000001,
-0.855000000000001,-0.850000000000001,-0.845000000000001,-0.840000000000001,
-0.835000000000001,-0.830000000000001,-0.825000000000001,-0.820000000000001,
-0.815000000000001,-0.810000000000001,-0.805000000000001,-0.800000000000001,
-0.795000000000001,-0.790000000000001,-0.785000000000001,-0.780000000000001,
-0.775000000000001,-0.770000000000001,-0.765000000000001,-0.760000000000001,
-0.755000000000001,-0.750000000000001,-0.745000000000001,-0.740000000000001,
-0.735000000000001,-0.730000000000001,-0.725000000000001,-0.720000000000001,
-0.715000000000001,-0.710000000000001,-0.705000000000001,-0.700000000000001,
-0.695000000000001,-0.690000000000001,-0.685,-0.68,-0.675,-0.67,-0.665,
-0.66,-0.655,-0.65,-0.645,-0.64,-0.635,-0.63,-0.625,-0.62,-0.615,-0.61,
-0.605,-0.6,-0.595,-0.59,-0.585,-0.58,-0.575,-0.57,-0.565,-0.56,-0.555,
-0.55,-0.545,-0.54,-0.535,-0.53,-0.525,-0.52,-0.515,-0.51,-0.505,-0.5,-0.495,
-0.49,-0.485,-0.48,-0.475,-0.47,-0.465,-0.46,-0.455,-0.45,-0.445,-0.44,
-0.435,-0.43,-0.425,-0.42,-0.415,-0.41,-0.405,-0.4,-0.395,-0.39,-0.385,
-0.38,-0.375,-0.37,-0.365,-0.36,-0.355,-0.35,-0.345,-0.34,-0.335,-0.33,
-0.325,-0.32,-0.315,-0.31,-0.305,-0.3,-0.295,-0.29,-0.285,-0.28,-0.275,
-0.27,-0.265,-0.26,-0.255,-0.25,-0.245,-0.24,-0.235,-0.23,-0.225,-0.22,
-0.215,-0.21,-0.205,-0.2,-0.195,-0.19,-0.185,-0.18,-0.175,-0.17,-0.165,
-0.16,-0.155,-0.15,-0.145,-0.14,-0.135,-0.13,-0.125,-0.12,-0.115,-0.11,
-0.105,-0.1,-0.095,-0.09,-0.085,-0.08,-0.075,-0.07,-0.065,-0.06,-0.055,
-0.05,-0.045,-0.04,-0.035,-0.03,-0.025,-0.02,-0.015,-0.01,-0.005,0.),(0.,
1.2),.UNSPECIFIED.)
GEOMETRIC_REPRESENTATION_ITEM()
RATIONAL_B_SPLINE_SURFACE(((1.,1.),(1.,1.),(1.,1.),(1.,1.),(1.,1.),(1.,
1.),(1.,1.),(1.,1.),(1.,1.),(1.,1.),(1.,1.),(1.,1.),(1.,1.),(1.,1.),(1.,
1.),(1.,1.),(1.,1.),(1.,1.),(1.,1.),(1.,1.),(1.,1.),(1.,1.),(1.,1.),(1.,
1.),(1.,1.),(1.,1.),(1.,1.),(1.,1.),(1.,1.),(1.,1.),(1.,1.),(1.,1.),(1.,
1.),(1.,1.),(1.,1.),(1.,1.),(1.,1.),(1.,1.),(1.,1.),(1.,1.),(1.,1.),(1.,
1.),(1.,1.),(1.,1.),(1.,1.),(1.,1.),(1.,1.),(1.,1.),(1.,1.),(1.,1.),(1.,
1.),(1.,1.),(1.,1.),(1.,1.),(1.,1.),(1.,1.),(1.,1.),(1.,1.),(1.,1.),(1.,
1.),(1.,1.),(1.,1.),(1.,1.),(1.,1.),(1.,1.),(1.,1.),(1.,1.),(1.,1.),(1.,
1.),(1.,1.),(1.,1.),(1.,1.),(1.,1.),(1.,1.),(1.,1.),(1.,1.),(1.,1.),(1.,
1.),(1.,1.),(1.,1.),(1.,1.),(1.,1.),(1.,1.),(1.,1.),(1.,1.),(1.,1.),(1.,
1.),(1.,1.),(1.,1.),(1.,1.),(1.,1.),(1.,1.),(1.,1.),(1.,1.),(1.,1.),(1.,
1.),(1.,1.),(1.,1.),(1.,1.),(1.,1.),(1.,1.),(1.,1.),(1.,1.),(1.,1.),(1.,
1.),(1.,1.),(1.,1.),(1.,1.),(1.,1.),(1.,1.),(1.,1.),(1.,1.),(1.,1.),(1.,
1.),(1.,1.),(1.,1.),(1.,1.),(1.,1.),(1.,1.),(1.,1.),(1.,1.),(1.,1.),(1.,
1.),(1.,1.),(1.,1.),(1.,1.),(1.,1.),(1.,1.),(1.,1.),(1.,1.),(1.,1.),(1.,
1.),(1.,1.),(1.,1.),(1.,1.),(1.,1.),(1.,1.),(1.,1.),(1.,1.),(1.,1.),(1.,
1.),(1.,1.),(1.,1.),(1.,1.),(1.,1.),(1.,1.),(1.,1.),(1.,1.),(1.,1.),(1.,
1.),(1.,1.),(1.,1.),(1.,1.),(1.,1.),(1.,1.),(1.,1.),(1.,1.),(1.,1.),(1.,
1.),(1.,1.),(1.,1.),(1.,1.),(1.,1.),(1.,1.),(1.,1.),(1.,1.),(1.,1.),(1.,
1.),(1.,1.),(1.,1.),(1.,1.),(1.,1.),(1.,1.),(1.,1.),(1.,1.),(1.,1.),(1.,
1.),(1.,1.),(1.,1.),(1.,1.),(1.,1.),(1.,1.),(1.,1.),(1.,1.),(1.,1.),(1.,
1.),(1.,1.),(1.,1.),(1.,1.),(1.,1.),(1.,1.),(1.,1.),(1.,1.),(1.,1.),(1.,
1.),(1.,1.),(1.,1.),(1.,1.),(1.,1.),(1.,1.),(1.,1.),(1.,1.),(1.,1.),(1.,
1.),(1.,1.)))
REPRESENTATION_ITEM('')
SURFACE()
);
#1038=(
BOUNDED_SURFACE()
B_SPLINE_SURFACE(5,1,((#192412,#192413),(#192414,#192415),(#192416,#192417),
(#192418,#192419),(#192420,#192421),(#192422,#192423),(#192424,#192425),
(#192426,#192427),(#192428,#192429),(#192430,#192431),(#192432,#192433),
(#192434,#192435),(#192436,#192437),(#192438,#192439),(#192440,#192441),
(#192442,#192443),(#192444,#192445),(#192446,#192447),(#192448,#192449),
(#192450,#192451),(#192452,#192453),(#192454,#192455),(#192456,#192457),
(#192458,#192459),(#192460,#192461),(#192462,#192463),(#192464,#192465),
(#192466,#192467),(#192468,#192469),(#192470,#192471),(#192472,#192473),
(#192474,#192475),(#192476,#192477),(#192478,#192479),(#192480,#192481),
(#192482,#192483),(#192484,#192485),(#192486,#192487),(#192488,#192489),
(#192490,#192491),(#192492,#192493),(#192494,#192495),(#192496,#192497),
(#192498,#192499),(#192500,#192501),(#192502,#192503),(#192504,#192505),
(#192506,#192507),(#192508,#192509),(#192510,#192511),(#192512,#192513),
(#192514,#192515),(#192516,#192517),(#192518,#192519),(#192520,#192521),
(#192522,#192523),(#192524,#192525),(#192526,#192527),(#192528,#192529),
(#192530,#192531),(#192532,#192533),(#192534,#192535),(#192536,#192537),
(#192538,#192539),(#192540,#192541),(#192542,#192543),(#192544,#192545),
(#192546,#192547),(#192548,#192549),(#192550,#192551),(#192552,#192553),
(#192554,#192555),(#192556,#192557),(#192558,#192559),(#192560,#192561),
(#192562,#192563),(#192564,#192565),(#192566,#192567),(#192568,#192569),
(#192570,#192571),(#192572,#192573),(#192574,#192575),(#192576,#192577),
(#192578,#192579),(#192580,#192581),(#192582,#192583),(#192584,#192585),
(#192586,#192587),(#192588,#192589),(#192590,#192591),(#192592,#192593),
(#192594,#192595),(#192596,#192597),(#192598,#192599),(#192600,#192601),
(#192602,#192603),(#192604,#192605),(#192606,#192607),(#192608,#192609),
(#192610,#192611),(#192612,#192613),(#192614,#192615),(#192616,#192617),
(#192618,#192619),(#192620,#192621),(#192622,#192623),(#192624,#192625),
(#192626,#192627),(#192628,#192629),(#192630,#192631),(#192632,#192633),
(#192634,#192635),(#192636,#192637),(#192638,#192639),(#192640,#192641),
(#192642,#192643),(#192644,#192645),(#192646,#192647),(#192648,#192649),
(#192650,#192651),(#192652,#192653),(#192654,#192655),(#192656,#192657),
(#192658,#192659),(#192660,#192661),(#192662,#192663),(#192664,#192665),
(#192666,#192667),(#192668,#192669),(#192670,#192671),(#192672,#192673),
(#192674,#192675),(#192676,#192677),(#192678,#192679),(#192680,#192681),
(#192682,#192683),(#192684,#192685),(#192686,#192687),(#192688,#192689),
(#192690,#192691),(#192692,#192693),(#192694,#192695),(#192696,#192697),
(#192698,#192699),(#192700,#192701),(#192702,#192703),(#192704,#192705),
(#192706,#192707),(#192708,#192709),(#192710,#192711),(#192712,#192713),
(#192714,#192715),(#192716,#192717),(#192718,#192719),(#192720,#192721),
(#192722,#192723),(#192724,#192725),(#192726,#192727),(#192728,#192729),
(#192730,#192731),(#192732,#192733),(#192734,#192735),(#192736,#192737),
(#192738,#192739),(#192740,#192741),(#192742,#192743),(#192744,#192745),
(#192746,#192747),(#192748,#192749),(#192750,#192751),(#192752,#192753),
(#192754,#192755),(#192756,#192757),(#192758,#192759),(#192760,#192761),
(#192762,#192763),(#192764,#192765),(#192766,#192767),(#192768,#192769),
(#192770,#192771),(#192772,#192773),(#192774,#192775),(#192776,#192777),
(#192778,#192779),(#192780,#192781),(#192782,#192783),(#192784,#192785),
(#192786,#192787),(#192788,#192789),(#192790,#192791),(#192792,#192793),
(#192794,#192795),(#192796,#192797),(#192798,#192799),(#192800,#192801),
(#192802,#192803),(#192804,#192805),(#192806,#192807),(#192808,#192809),
(#192810,#192811),(#192812,#192813),(#192814,#192815),(#192816,#192817),
(#192818,#192819),(#192820,#192821)),.UNSPECIFIED.,.F.,.F.,.F.)
B_SPLINE_SURFACE_WITH_KNOTS((6,1,1,1,1,1,1,1,1,1,1,1,1,1,1,1,1,1,1,1,1,
1,1,1,1,1,1,1,1,1,1,1,1,1,1,1,1,1,1,1,1,1,1,1,1,1,1,1,1,1,1,1,1,1,1,1,1,
1,1,1,1,1,1,1,1,1,1,1,1,1,1,1,1,1,1,1,1,1,1,1,1,1,1,1,1,1,1,1,1,1,1,1,1,
1,1,1,1,1,1,1,1,1,1,1,1,1,1,1,1,1,1,1,1,1,1,1,1,1,1,1,1,1,1,1,1,1,1,1,1,
1,1,1,1,1,1,1,1,1,1,1,1,1,1,1,1,1,1,1,1,1,1,1,1,1,1,1,1,1,1,1,1,1,1,1,1,
1,1,1,1,1,1,1,1,1,1,1,1,1,1,1,1,1,1,1,1,1,1,1,1,1,1,1,1,1,1,1,1,1,1,1,6),
(2,2),(0.,0.005,0.01,0.015,0.02,0.025,0.03,0.035,0.04,0.045,0.05,0.055,
0.06,0.065,0.07,0.075,0.08,0.085,0.09,0.095,0.1,0.105,0.11,0.115,0.12,0.125,
0.13,0.135,0.14,0.145,0.15,0.155,0.16,0.165,0.17,0.175,0.18,0.185,0.19,
0.195,0.2,0.205,0.21,0.215,0.22,0.225,0.23,0.235,0.24,0.245,0.25,0.255,
0.26,0.265,0.27,0.275,0.28,0.285,0.29,0.295,0.3,0.305,0.31,0.315,0.32,0.325,
0.33,0.335,0.34,0.345,0.35,0.355,0.36,0.365,0.37,0.375,0.38,0.385,0.39,
0.395,0.4,0.405,0.41,0.415,0.42,0.425,0.43,0.435,0.44,0.445,0.45,0.455,
0.46,0.465,0.47,0.475,0.48,0.485,0.49,0.495,0.5,0.505,0.51,0.515,0.52,0.525,
0.53,0.535,0.54,0.545,0.55,0.555,0.56,0.565,0.57,0.575,0.58,0.585,0.59,
0.595,0.6,0.605,0.61,0.615,0.62,0.625,0.63,0.635,0.64,0.645,0.65,0.655,
0.66,0.665,0.67,0.675,0.68,0.685,0.690000000000001,0.695000000000001,0.700000000000001,
0.705000000000001,0.710000000000001,0.715000000000001,0.720000000000001,
0.725000000000001,0.730000000000001,0.735000000000001,0.740000000000001,
0.745000000000001,0.750000000000001,0.755000000000001,0.760000000000001,
0.765000000000001,0.770000000000001,0.775000000000001,0.780000000000001,
0.785000000000001,0.790000000000001,0.795000000000001,0.800000000000001,
0.805000000000001,0.810000000000001,0.815000000000001,0.820000000000001,
0.825000000000001,0.830000000000001,0.835000000000001,0.840000000000001,
0.845000000000001,0.850000000000001,0.855000000000001,0.860000000000001,
0.865000000000001,0.870000000000001,0.875000000000001,0.880000000000001,
0.885000000000001,0.890000000000001,0.895000000000001,0.900000000000001,
0.905000000000001,0.910000000000001,0.915000000000001,0.920000000000001,
0.925000000000001,0.930000000000001,0.935000000000001,0.940000000000001,
0.945000000000001,0.950000000000001,0.955000000000001,0.960000000000001,
0.965000000000001,0.970000000000001,0.975000000000001,0.980000000000001,
0.985000000000001,0.990000000000001,0.995000000000001,1.),(0.,1.2),
 .UNSPECIFIED.)
GEOMETRIC_REPRESENTATION_ITEM()
RATIONAL_B_SPLINE_SURFACE(((1.,1.),(1.,1.),(1.,1.),(1.,1.),(1.,1.),(1.,
1.),(1.,1.),(1.,1.),(1.,1.),(1.,1.),(1.,1.),(1.,1.),(1.,1.),(1.,1.),(1.,
1.),(1.,1.),(1.,1.),(1.,1.),(1.,1.),(1.,1.),(1.,1.),(1.,1.),(1.,1.),(1.,
1.),(1.,1.),(1.,1.),(1.,1.),(1.,1.),(1.,1.),(1.,1.),(1.,1.),(1.,1.),(1.,
1.),(1.,1.),(1.,1.),(1.,1.),(1.,1.),(1.,1.),(1.,1.),(1.,1.),(1.,1.),(1.,
1.),(1.,1.),(1.,1.),(1.,1.),(1.,1.),(1.,1.),(1.,1.),(1.,1.),(1.,1.),(1.,
1.),(1.,1.),(1.,1.),(1.,1.),(1.,1.),(1.,1.),(1.,1.),(1.,1.),(1.,1.),(1.,
1.),(1.,1.),(1.,1.),(1.,1.),(1.,1.),(1.,1.),(1.,1.),(1.,1.),(1.,1.),(1.,
1.),(1.,1.),(1.,1.),(1.,1.),(1.,1.),(1.,1.),(1.,1.),(1.,1.),(1.,1.),(1.,
1.),(1.,1.),(1.,1.),(1.,1.),(1.,1.),(1.,1.),(1.,1.),(1.,1.),(1.,1.),(1.,
1.),(1.,1.),(1.,1.),(1.,1.),(1.,1.),(1.,1.),(1.,1.),(1.,1.),(1.,1.),(1.,
1.),(1.,1.),(1.,1.),(1.,1.),(1.,1.),(1.,1.),(1.,1.),(1.,1.),(1.,1.),(1.,
1.),(1.,1.),(1.,1.),(1.,1.),(1.,1.),(1.,1.),(1.,1.),(1.,1.),(1.,1.),(1.,
1.),(1.,1.),(1.,1.),(1.,1.),(1.,1.),(1.,1.),(1.,1.),(1.,1.),(1.,1.),(1.,
1.),(1.,1.),(1.,1.),(1.,1.),(1.,1.),(1.,1.),(1.,1.),(1.,1.),(1.,1.),(1.,
1.),(1.,1.),(1.,1.),(1.,1.),(1.,1.),(1.,1.),(1.,1.),(1.,1.),(1.,1.),(1.,
1.),(1.,1.),(1.,1.),(1.,1.),(1.,1.),(1.,1.),(1.,1.),(1.,1.),(1.,1.),(1.,
1.),(1.,1.),(1.,1.),(1.,1.),(1.,1.),(1.,1.),(1.,1.),(1.,1.),(1.,1.),(1.,
1.),(1.,1.),(1.,1.),(1.,1.),(1.,1.),(1.,1.),(1.,1.),(1.,1.),(1.,1.),(1.,
1.),(1.,1.),(1.,1.),(1.,1.),(1.,1.),(1.,1.),(1.,1.),(1.,1.),(1.,1.),(1.,
1.),(1.,1.),(1.,1.),(1.,1.),(1.,1.),(1.,1.),(1.,1.),(1.,1.),(1.,1.),(1.,
1.),(1.,1.),(1.,1.),(1.,1.),(1.,1.),(1.,1.),(1.,1.),(1.,1.),(1.,1.),(1.,
1.),(1.,1.),(1.,1.),(1.,1.),(1.,1.),(1.,1.),(1.,1.),(1.,1.),(1.,1.),(1.,
1.),(1.,1.)))
REPRESENTATION_ITEM('')
SURFACE()
);
#1039=(
BOUNDED_SURFACE()
B_SPLINE_SURFACE(5,1,((#193033,#193034),(#193035,#193036),(#193037,#193038),
(#193039,#193040),(#193041,#193042),(#193043,#193044),(#193045,#193046),
(#193047,#193048),(#193049,#193050),(#193051,#193052),(#193053,#193054),
(#193055,#193056),(#193057,#193058),(#193059,#193060),(#193061,#193062),
(#193063,#193064),(#193065,#193066),(#193067,#193068),(#193069,#193070),
(#193071,#193072),(#193073,#193074),(#193075,#193076),(#193077,#193078),
(#193079,#193080),(#193081,#193082),(#193083,#193084),(#193085,#193086),
(#193087,#193088),(#193089,#193090),(#193091,#193092),(#193093,#193094),
(#193095,#193096),(#193097,#193098),(#193099,#193100),(#193101,#193102),
(#193103,#193104),(#193105,#193106),(#193107,#193108),(#193109,#193110),
(#193111,#193112),(#193113,#193114),(#193115,#193116),(#193117,#193118),
(#193119,#193120),(#193121,#193122),(#193123,#193124),(#193125,#193126),
(#193127,#193128),(#193129,#193130),(#193131,#193132),(#193133,#193134),
(#193135,#193136),(#193137,#193138),(#193139,#193140),(#193141,#193142),
(#193143,#193144),(#193145,#193146),(#193147,#193148),(#193149,#193150),
(#193151,#193152),(#193153,#193154),(#193155,#193156),(#193157,#193158),
(#193159,#193160),(#193161,#193162),(#193163,#193164),(#193165,#193166),
(#193167,#193168),(#193169,#193170),(#193171,#193172),(#193173,#193174),
(#193175,#193176),(#193177,#193178),(#193179,#193180),(#193181,#193182),
(#193183,#193184),(#193185,#193186),(#193187,#193188),(#193189,#193190),
(#193191,#193192),(#193193,#193194),(#193195,#193196),(#193197,#193198),
(#193199,#193200),(#193201,#193202),(#193203,#193204),(#193205,#193206),
(#193207,#193208),(#193209,#193210),(#193211,#193212),(#193213,#193214),
(#193215,#193216),(#193217,#193218),(#193219,#193220),(#193221,#193222),
(#193223,#193224),(#193225,#193226),(#193227,#193228),(#193229,#193230),
(#193231,#193232),(#193233,#193234),(#193235,#193236),(#193237,#193238),
(#193239,#193240),(#193241,#193242),(#193243,#193244),(#193245,#193246),
(#193247,#193248),(#193249,#193250),(#193251,#193252),(#193253,#193254),
(#193255,#193256),(#193257,#193258),(#193259,#193260),(#193261,#193262),
(#193263,#193264),(#193265,#193266),(#193267,#193268),(#193269,#193270),
(#193271,#193272),(#193273,#193274),(#193275,#193276),(#193277,#193278),
(#193279,#193280),(#193281,#193282),(#193283,#193284),(#193285,#193286),
(#193287,#193288),(#193289,#193290),(#193291,#193292),(#193293,#193294),
(#193295,#193296),(#193297,#193298),(#193299,#193300),(#193301,#193302),
(#193303,#193304),(#193305,#193306),(#193307,#193308),(#193309,#193310),
(#193311,#193312),(#193313,#193314),(#193315,#193316),(#193317,#193318),
(#193319,#193320),(#193321,#193322),(#193323,#193324),(#193325,#193326),
(#193327,#193328),(#193329,#193330),(#193331,#193332),(#193333,#193334),
(#193335,#193336),(#193337,#193338),(#193339,#193340),(#193341,#193342),
(#193343,#193344),(#193345,#193346),(#193347,#193348),(#193349,#193350),
(#193351,#193352),(#193353,#193354),(#193355,#193356),(#193357,#193358),
(#193359,#193360),(#193361,#193362),(#193363,#193364),(#193365,#193366),
(#193367,#193368),(#193369,#193370),(#193371,#193372),(#193373,#193374),
(#193375,#193376),(#193377,#193378),(#193379,#193380),(#193381,#193382),
(#193383,#193384),(#193385,#193386),(#193387,#193388),(#193389,#193390),
(#193391,#193392),(#193393,#193394),(#193395,#193396),(#193397,#193398),
(#193399,#193400),(#193401,#193402),(#193403,#193404),(#193405,#193406),
(#193407,#193408),(#193409,#193410),(#193411,#193412),(#193413,#193414),
(#193415,#193416),(#193417,#193418),(#193419,#193420),(#193421,#193422),
(#193423,#193424),(#193425,#193426),(#193427,#193428),(#193429,#193430),
(#193431,#193432),(#193433,#193434),(#193435,#193436),(#193437,#193438),
(#193439,#193440),(#193441,#193442)),.UNSPECIFIED.,.F.,.F.,.F.)
B_SPLINE_SURFACE_WITH_KNOTS((6,1,1,1,1,1,1,1,1,1,1,1,1,1,1,1,1,1,1,1,1,
1,1,1,1,1,1,1,1,1,1,1,1,1,1,1,1,1,1,1,1,1,1,1,1,1,1,1,1,1,1,1,1,1,1,1,1,
1,1,1,1,1,1,1,1,1,1,1,1,1,1,1,1,1,1,1,1,1,1,1,1,1,1,1,1,1,1,1,1,1,1,1,1,
1,1,1,1,1,1,1,1,1,1,1,1,1,1,1,1,1,1,1,1,1,1,1,1,1,1,1,1,1,1,1,1,1,1,1,1,
1,1,1,1,1,1,1,1,1,1,1,1,1,1,1,1,1,1,1,1,1,1,1,1,1,1,1,1,1,1,1,1,1,1,1,1,
1,1,1,1,1,1,1,1,1,1,1,1,1,1,1,1,1,1,1,1,1,1,1,1,1,1,1,1,1,1,1,1,1,1,1,6),
(2,2),(-1.,-0.995000000000001,-0.990000000000001,-0.985000000000001,-0.980000000000001,
-0.975000000000001,-0.970000000000001,-0.965000000000001,-0.960000000000001,
-0.955000000000001,-0.950000000000001,-0.945000000000001,-0.940000000000001,
-0.935000000000001,-0.930000000000001,-0.925000000000001,-0.920000000000001,
-0.915000000000001,-0.910000000000001,-0.905000000000001,-0.900000000000001,
-0.895000000000001,-0.890000000000001,-0.885000000000001,-0.880000000000001,
-0.875000000000001,-0.870000000000001,-0.865000000000001,-0.860000000000001,
-0.855000000000001,-0.850000000000001,-0.845000000000001,-0.840000000000001,
-0.835000000000001,-0.830000000000001,-0.825000000000001,-0.820000000000001,
-0.815000000000001,-0.810000000000001,-0.805000000000001,-0.800000000000001,
-0.795000000000001,-0.790000000000001,-0.785000000000001,-0.780000000000001,
-0.775000000000001,-0.770000000000001,-0.765000000000001,-0.760000000000001,
-0.755000000000001,-0.750000000000001,-0.745000000000001,-0.740000000000001,
-0.735000000000001,-0.730000000000001,-0.725000000000001,-0.720000000000001,
-0.715000000000001,-0.710000000000001,-0.705000000000001,-0.700000000000001,
-0.695000000000001,-0.690000000000001,-0.685,-0.68,-0.675,-0.67,-0.665,
-0.66,-0.655,-0.65,-0.645,-0.64,-0.635,-0.63,-0.625,-0.62,-0.615,-0.61,
-0.605,-0.6,-0.595,-0.59,-0.585,-0.58,-0.575,-0.57,-0.565,-0.56,-0.555,
-0.55,-0.545,-0.54,-0.535,-0.53,-0.525,-0.52,-0.515,-0.51,-0.505,-0.5,-0.495,
-0.49,-0.485,-0.48,-0.475,-0.47,-0.465,-0.46,-0.455,-0.45,-0.445,-0.44,
-0.435,-0.43,-0.425,-0.42,-0.415,-0.41,-0.405,-0.4,-0.395,-0.39,-0.385,
-0.38,-0.375,-0.37,-0.365,-0.36,-0.355,-0.35,-0.345,-0.34,-0.335,-0.33,
-0.325,-0.32,-0.315,-0.31,-0.305,-0.3,-0.295,-0.29,-0.285,-0.28,-0.275,
-0.27,-0.265,-0.26,-0.255,-0.25,-0.245,-0.24,-0.235,-0.23,-0.225,-0.22,
-0.215,-0.21,-0.205,-0.2,-0.195,-0.19,-0.185,-0.18,-0.175,-0.17,-0.165,
-0.16,-0.155,-0.15,-0.145,-0.14,-0.135,-0.13,-0.125,-0.12,-0.115,-0.11,
-0.105,-0.1,-0.095,-0.09,-0.085,-0.08,-0.075,-0.07,-0.065,-0.06,-0.055,
-0.05,-0.045,-0.04,-0.035,-0.03,-0.025,-0.02,-0.015,-0.01,-0.005,0.),(0.,
1.2),.UNSPECIFIED.)
GEOMETRIC_REPRESENTATION_ITEM()
RATIONAL_B_SPLINE_SURFACE(((1.,1.),(1.,1.),(1.,1.),(1.,1.),(1.,1.),(1.,
1.),(1.,1.),(1.,1.),(1.,1.),(1.,1.),(1.,1.),(1.,1.),(1.,1.),(1.,1.),(1.,
1.),(1.,1.),(1.,1.),(1.,1.),(1.,1.),(1.,1.),(1.,1.),(1.,1.),(1.,1.),(1.,
1.),(1.,1.),(1.,1.),(1.,1.),(1.,1.),(1.,1.),(1.,1.),(1.,1.),(1.,1.),(1.,
1.),(1.,1.),(1.,1.),(1.,1.),(1.,1.),(1.,1.),(1.,1.),(1.,1.),(1.,1.),(1.,
1.),(1.,1.),(1.,1.),(1.,1.),(1.,1.),(1.,1.),(1.,1.),(1.,1.),(1.,1.),(1.,
1.),(1.,1.),(1.,1.),(1.,1.),(1.,1.),(1.,1.),(1.,1.),(1.,1.),(1.,1.),(1.,
1.),(1.,1.),(1.,1.),(1.,1.),(1.,1.),(1.,1.),(1.,1.),(1.,1.),(1.,1.),(1.,
1.),(1.,1.),(1.,1.),(1.,1.),(1.,1.),(1.,1.),(1.,1.),(1.,1.),(1.,1.),(1.,
1.),(1.,1.),(1.,1.),(1.,1.),(1.,1.),(1.,1.),(1.,1.),(1.,1.),(1.,1.),(1.,
1.),(1.,1.),(1.,1.),(1.,1.),(1.,1.),(1.,1.),(1.,1.),(1.,1.),(1.,1.),(1.,
1.),(1.,1.),(1.,1.),(1.,1.),(1.,1.),(1.,1.),(1.,1.),(1.,1.),(1.,1.),(1.,
1.),(1.,1.),(1.,1.),(1.,1.),(1.,1.),(1.,1.),(1.,1.),(1.,1.),(1.,1.),(1.,
1.),(1.,1.),(1.,1.),(1.,1.),(1.,1.),(1.,1.),(1.,1.),(1.,1.),(1.,1.),(1.,
1.),(1.,1.),(1.,1.),(1.,1.),(1.,1.),(1.,1.),(1.,1.),(1.,1.),(1.,1.),(1.,
1.),(1.,1.),(1.,1.),(1.,1.),(1.,1.),(1.,1.),(1.,1.),(1.,1.),(1.,1.),(1.,
1.),(1.,1.),(1.,1.),(1.,1.),(1.,1.),(1.,1.),(1.,1.),(1.,1.),(1.,1.),(1.,
1.),(1.,1.),(1.,1.),(1.,1.),(1.,1.),(1.,1.),(1.,1.),(1.,1.),(1.,1.),(1.,
1.),(1.,1.),(1.,1.),(1.,1.),(1.,1.),(1.,1.),(1.,1.),(1.,1.),(1.,1.),(1.,
1.),(1.,1.),(1.,1.),(1.,1.),(1.,1.),(1.,1.),(1.,1.),(1.,1.),(1.,1.),(1.,
1.),(1.,1.),(1.,1.),(1.,1.),(1.,1.),(1.,1.),(1.,1.),(1.,1.),(1.,1.),(1.,
1.),(1.,1.),(1.,1.),(1.,1.),(1.,1.),(1.,1.),(1.,1.),(1.,1.),(1.,1.),(1.,
1.),(1.,1.),(1.,1.),(1.,1.),(1.,1.),(1.,1.),(1.,1.),(1.,1.),(1.,1.),(1.,
1.),(1.,1.)))
REPRESENTATION_ITEM('')
SURFACE()
);
#1040=(
BOUNDED_SURFACE()
B_SPLINE_SURFACE(5,1,((#193650,#193651),(#193652,#193653),(#193654,#193655),
(#193656,#193657),(#193658,#193659),(#193660,#193661),(#193662,#193663),
(#193664,#193665),(#193666,#193667),(#193668,#193669),(#193670,#193671),
(#193672,#193673),(#193674,#193675),(#193676,#193677),(#193678,#193679),
(#193680,#193681),(#193682,#193683),(#193684,#193685),(#193686,#193687),
(#193688,#193689),(#193690,#193691),(#193692,#193693),(#193694,#193695),
(#193696,#193697),(#193698,#193699),(#193700,#193701),(#193702,#193703),
(#193704,#193705),(#193706,#193707),(#193708,#193709),(#193710,#193711),
(#193712,#193713),(#193714,#193715),(#193716,#193717),(#193718,#193719),
(#193720,#193721),(#193722,#193723),(#193724,#193725),(#193726,#193727),
(#193728,#193729),(#193730,#193731),(#193732,#193733),(#193734,#193735),
(#193736,#193737),(#193738,#193739),(#193740,#193741),(#193742,#193743),
(#193744,#193745),(#193746,#193747),(#193748,#193749),(#193750,#193751),
(#193752,#193753),(#193754,#193755),(#193756,#193757),(#193758,#193759),
(#193760,#193761),(#193762,#193763),(#193764,#193765),(#193766,#193767),
(#193768,#193769),(#193770,#193771),(#193772,#193773),(#193774,#193775),
(#193776,#193777),(#193778,#193779),(#193780,#193781),(#193782,#193783),
(#193784,#193785),(#193786,#193787),(#193788,#193789),(#193790,#193791),
(#193792,#193793),(#193794,#193795),(#193796,#193797),(#193798,#193799),
(#193800,#193801),(#193802,#193803),(#193804,#193805),(#193806,#193807),
(#193808,#193809),(#193810,#193811),(#193812,#193813),(#193814,#193815),
(#193816,#193817),(#193818,#193819),(#193820,#193821),(#193822,#193823),
(#193824,#193825),(#193826,#193827),(#193828,#193829),(#193830,#193831),
(#193832,#193833),(#193834,#193835),(#193836,#193837),(#193838,#193839),
(#193840,#193841),(#193842,#193843),(#193844,#193845),(#193846,#193847),
(#193848,#193849),(#193850,#193851),(#193852,#193853),(#193854,#193855),
(#193856,#193857),(#193858,#193859),(#193860,#193861),(#193862,#193863),
(#193864,#193865),(#193866,#193867),(#193868,#193869),(#193870,#193871),
(#193872,#193873),(#193874,#193875),(#193876,#193877),(#193878,#193879),
(#193880,#193881),(#193882,#193883),(#193884,#193885),(#193886,#193887),
(#193888,#193889),(#193890,#193891),(#193892,#193893),(#193894,#193895),
(#193896,#193897),(#193898,#193899),(#193900,#193901),(#193902,#193903),
(#193904,#193905),(#193906,#193907),(#193908,#193909),(#193910,#193911),
(#193912,#193913),(#193914,#193915),(#193916,#193917),(#193918,#193919),
(#193920,#193921),(#193922,#193923),(#193924,#193925),(#193926,#193927),
(#193928,#193929),(#193930,#193931),(#193932,#193933),(#193934,#193935),
(#193936,#193937),(#193938,#193939),(#193940,#193941),(#193942,#193943),
(#193944,#193945),(#193946,#193947),(#193948,#193949),(#193950,#193951),
(#193952,#193953),(#193954,#193955),(#193956,#193957),(#193958,#193959),
(#193960,#193961),(#193962,#193963),(#193964,#193965),(#193966,#193967),
(#193968,#193969),(#193970,#193971),(#193972,#193973),(#193974,#193975),
(#193976,#193977),(#193978,#193979),(#193980,#193981),(#193982,#193983),
(#193984,#193985),(#193986,#193987),(#193988,#193989),(#193990,#193991),
(#193992,#193993),(#193994,#193995),(#193996,#193997),(#193998,#193999),
(#194000,#194001),(#194002,#194003),(#194004,#194005),(#194006,#194007),
(#194008,#194009),(#194010,#194011),(#194012,#194013),(#194014,#194015),
(#194016,#194017),(#194018,#194019),(#194020,#194021),(#194022,#194023),
(#194024,#194025),(#194026,#194027),(#194028,#194029),(#194030,#194031),
(#194032,#194033),(#194034,#194035),(#194036,#194037),(#194038,#194039),
(#194040,#194041),(#194042,#194043),(#194044,#194045),(#194046,#194047),
(#194048,#194049),(#194050,#194051),(#194052,#194053),(#194054,#194055),
(#194056,#194057),(#194058,#194059)),.UNSPECIFIED.,.F.,.F.,.F.)
B_SPLINE_SURFACE_WITH_KNOTS((6,1,1,1,1,1,1,1,1,1,1,1,1,1,1,1,1,1,1,1,1,
1,1,1,1,1,1,1,1,1,1,1,1,1,1,1,1,1,1,1,1,1,1,1,1,1,1,1,1,1,1,1,1,1,1,1,1,
1,1,1,1,1,1,1,1,1,1,1,1,1,1,1,1,1,1,1,1,1,1,1,1,1,1,1,1,1,1,1,1,1,1,1,1,
1,1,1,1,1,1,1,1,1,1,1,1,1,1,1,1,1,1,1,1,1,1,1,1,1,1,1,1,1,1,1,1,1,1,1,1,
1,1,1,1,1,1,1,1,1,1,1,1,1,1,1,1,1,1,1,1,1,1,1,1,1,1,1,1,1,1,1,1,1,1,1,1,
1,1,1,1,1,1,1,1,1,1,1,1,1,1,1,1,1,1,1,1,1,1,1,1,1,1,1,1,1,1,1,1,1,1,1,6),
(2,2),(0.,0.005,0.01,0.015,0.02,0.025,0.03,0.035,0.04,0.045,0.05,0.055,
0.06,0.065,0.07,0.075,0.08,0.085,0.09,0.095,0.1,0.105,0.11,0.115,0.12,0.125,
0.13,0.135,0.14,0.145,0.15,0.155,0.16,0.165,0.17,0.175,0.18,0.185,0.19,
0.195,0.2,0.205,0.21,0.215,0.22,0.225,0.23,0.235,0.24,0.245,0.25,0.255,
0.26,0.265,0.27,0.275,0.28,0.285,0.29,0.295,0.3,0.305,0.31,0.315,0.32,0.325,
0.33,0.335,0.34,0.345,0.35,0.355,0.36,0.365,0.37,0.375,0.38,0.385,0.39,
0.395,0.4,0.405,0.41,0.415,0.42,0.425,0.43,0.435,0.44,0.445,0.45,0.455,
0.46,0.465,0.47,0.475,0.48,0.485,0.49,0.495,0.5,0.505,0.51,0.515,0.52,0.525,
0.53,0.535,0.54,0.545,0.55,0.555,0.56,0.565,0.57,0.575,0.58,0.585,0.59,
0.595,0.6,0.605,0.61,0.615,0.62,0.625,0.63,0.635,0.64,0.645,0.65,0.655,
0.66,0.665,0.67,0.675,0.68,0.685,0.690000000000001,0.695000000000001,0.700000000000001,
0.705000000000001,0.710000000000001,0.715000000000001,0.720000000000001,
0.725000000000001,0.730000000000001,0.735000000000001,0.740000000000001,
0.745000000000001,0.750000000000001,0.755000000000001,0.760000000000001,
0.765000000000001,0.770000000000001,0.775000000000001,0.780000000000001,
0.785000000000001,0.790000000000001,0.795000000000001,0.800000000000001,
0.805000000000001,0.810000000000001,0.815000000000001,0.820000000000001,
0.825000000000001,0.830000000000001,0.835000000000001,0.840000000000001,
0.845000000000001,0.850000000000001,0.855000000000001,0.860000000000001,
0.865000000000001,0.870000000000001,0.875000000000001,0.880000000000001,
0.885000000000001,0.890000000000001,0.895000000000001,0.900000000000001,
0.905000000000001,0.910000000000001,0.915000000000001,0.920000000000001,
0.925000000000001,0.930000000000001,0.935000000000001,0.940000000000001,
0.945000000000001,0.950000000000001,0.955000000000001,0.960000000000001,
0.965000000000001,0.970000000000001,0.975000000000001,0.980000000000001,
0.985000000000001,0.990000000000001,0.995000000000001,1.),(0.,1.2),
 .UNSPECIFIED.)
GEOMETRIC_REPRESENTATION_ITEM()
RATIONAL_B_SPLINE_SURFACE(((1.,1.),(1.,1.),(1.,1.),(1.,1.),(1.,1.),(1.,
1.),(1.,1.),(1.,1.),(1.,1.),(1.,1.),(1.,1.),(1.,1.),(1.,1.),(1.,1.),(1.,
1.),(1.,1.),(1.,1.),(1.,1.),(1.,1.),(1.,1.),(1.,1.),(1.,1.),(1.,1.),(1.,
1.),(1.,1.),(1.,1.),(1.,1.),(1.,1.),(1.,1.),(1.,1.),(1.,1.),(1.,1.),(1.,
1.),(1.,1.),(1.,1.),(1.,1.),(1.,1.),(1.,1.),(1.,1.),(1.,1.),(1.,1.),(1.,
1.),(1.,1.),(1.,1.),(1.,1.),(1.,1.),(1.,1.),(1.,1.),(1.,1.),(1.,1.),(1.,
1.),(1.,1.),(1.,1.),(1.,1.),(1.,1.),(1.,1.),(1.,1.),(1.,1.),(1.,1.),(1.,
1.),(1.,1.),(1.,1.),(1.,1.),(1.,1.),(1.,1.),(1.,1.),(1.,1.),(1.,1.),(1.,
1.),(1.,1.),(1.,1.),(1.,1.),(1.,1.),(1.,1.),(1.,1.),(1.,1.),(1.,1.),(1.,
1.),(1.,1.),(1.,1.),(1.,1.),(1.,1.),(1.,1.),(1.,1.),(1.,1.),(1.,1.),(1.,
1.),(1.,1.),(1.,1.),(1.,1.),(1.,1.),(1.,1.),(1.,1.),(1.,1.),(1.,1.),(1.,
1.),(1.,1.),(1.,1.),(1.,1.),(1.,1.),(1.,1.),(1.,1.),(1.,1.),(1.,1.),(1.,
1.),(1.,1.),(1.,1.),(1.,1.),(1.,1.),(1.,1.),(1.,1.),(1.,1.),(1.,1.),(1.,
1.),(1.,1.),(1.,1.),(1.,1.),(1.,1.),(1.,1.),(1.,1.),(1.,1.),(1.,1.),(1.,
1.),(1.,1.),(1.,1.),(1.,1.),(1.,1.),(1.,1.),(1.,1.),(1.,1.),(1.,1.),(1.,
1.),(1.,1.),(1.,1.),(1.,1.),(1.,1.),(1.,1.),(1.,1.),(1.,1.),(1.,1.),(1.,
1.),(1.,1.),(1.,1.),(1.,1.),(1.,1.),(1.,1.),(1.,1.),(1.,1.),(1.,1.),(1.,
1.),(1.,1.),(1.,1.),(1.,1.),(1.,1.),(1.,1.),(1.,1.),(1.,1.),(1.,1.),(1.,
1.),(1.,1.),(1.,1.),(1.,1.),(1.,1.),(1.,1.),(1.,1.),(1.,1.),(1.,1.),(1.,
1.),(1.,1.),(1.,1.),(1.,1.),(1.,1.),(1.,1.),(1.,1.),(1.,1.),(1.,1.),(1.,
1.),(1.,1.),(1.,1.),(1.,1.),(1.,1.),(1.,1.),(1.,1.),(1.,1.),(1.,1.),(1.,
1.),(1.,1.),(1.,1.),(1.,1.),(1.,1.),(1.,1.),(1.,1.),(1.,1.),(1.,1.),(1.,
1.),(1.,1.),(1.,1.),(1.,1.),(1.,1.),(1.,1.),(1.,1.),(1.,1.),(1.,1.),(1.,
1.),(1.,1.)))
REPRESENTATION_ITEM('')
SURFACE()
);
#1041=(
BOUNDED_SURFACE()
B_SPLINE_SURFACE(5,1,((#194271,#194272),(#194273,#194274),(#194275,#194276),
(#194277,#194278),(#194279,#194280),(#194281,#194282),(#194283,#194284),
(#194285,#194286),(#194287,#194288),(#194289,#194290),(#194291,#194292),
(#194293,#194294),(#194295,#194296),(#194297,#194298),(#194299,#194300),
(#194301,#194302),(#194303,#194304),(#194305,#194306),(#194307,#194308),
(#194309,#194310),(#194311,#194312),(#194313,#194314),(#194315,#194316),
(#194317,#194318),(#194319,#194320),(#194321,#194322),(#194323,#194324),
(#194325,#194326),(#194327,#194328),(#194329,#194330),(#194331,#194332),
(#194333,#194334),(#194335,#194336),(#194337,#194338),(#194339,#194340),
(#194341,#194342),(#194343,#194344),(#194345,#194346),(#194347,#194348),
(#194349,#194350),(#194351,#194352),(#194353,#194354),(#194355,#194356),
(#194357,#194358),(#194359,#194360),(#194361,#194362),(#194363,#194364),
(#194365,#194366),(#194367,#194368),(#194369,#194370),(#194371,#194372),
(#194373,#194374),(#194375,#194376),(#194377,#194378),(#194379,#194380),
(#194381,#194382),(#194383,#194384),(#194385,#194386),(#194387,#194388),
(#194389,#194390),(#194391,#194392),(#194393,#194394),(#194395,#194396),
(#194397,#194398),(#194399,#194400),(#194401,#194402),(#194403,#194404),
(#194405,#194406),(#194407,#194408),(#194409,#194410),(#194411,#194412),
(#194413,#194414),(#194415,#194416),(#194417,#194418),(#194419,#194420),
(#194421,#194422),(#194423,#194424),(#194425,#194426),(#194427,#194428),
(#194429,#194430),(#194431,#194432),(#194433,#194434),(#194435,#194436),
(#194437,#194438),(#194439,#194440),(#194441,#194442),(#194443,#194444),
(#194445,#194446),(#194447,#194448),(#194449,#194450),(#194451,#194452),
(#194453,#194454),(#194455,#194456),(#194457,#194458),(#194459,#194460),
(#194461,#194462),(#194463,#194464),(#194465,#194466),(#194467,#194468),
(#194469,#194470),(#194471,#194472),(#194473,#194474),(#194475,#194476),
(#194477,#194478),(#194479,#194480),(#194481,#194482),(#194483,#194484),
(#194485,#194486),(#194487,#194488),(#194489,#194490),(#194491,#194492),
(#194493,#194494),(#194495,#194496),(#194497,#194498),(#194499,#194500),
(#194501,#194502),(#194503,#194504),(#194505,#194506),(#194507,#194508),
(#194509,#194510),(#194511,#194512),(#194513,#194514),(#194515,#194516),
(#194517,#194518),(#194519,#194520),(#194521,#194522),(#194523,#194524),
(#194525,#194526),(#194527,#194528),(#194529,#194530),(#194531,#194532),
(#194533,#194534),(#194535,#194536),(#194537,#194538),(#194539,#194540),
(#194541,#194542),(#194543,#194544),(#194545,#194546),(#194547,#194548),
(#194549,#194550),(#194551,#194552),(#194553,#194554),(#194555,#194556),
(#194557,#194558),(#194559,#194560),(#194561,#194562),(#194563,#194564),
(#194565,#194566),(#194567,#194568),(#194569,#194570),(#194571,#194572),
(#194573,#194574),(#194575,#194576),(#194577,#194578),(#194579,#194580),
(#194581,#194582),(#194583,#194584),(#194585,#194586),(#194587,#194588),
(#194589,#194590),(#194591,#194592),(#194593,#194594),(#194595,#194596),
(#194597,#194598),(#194599,#194600),(#194601,#194602),(#194603,#194604),
(#194605,#194606),(#194607,#194608),(#194609,#194610),(#194611,#194612),
(#194613,#194614),(#194615,#194616),(#194617,#194618),(#194619,#194620),
(#194621,#194622),(#194623,#194624),(#194625,#194626),(#194627,#194628),
(#194629,#194630),(#194631,#194632),(#194633,#194634),(#194635,#194636),
(#194637,#194638),(#194639,#194640),(#194641,#194642),(#194643,#194644),
(#194645,#194646),(#194647,#194648),(#194649,#194650),(#194651,#194652),
(#194653,#194654),(#194655,#194656),(#194657,#194658),(#194659,#194660),
(#194661,#194662),(#194663,#194664),(#194665,#194666),(#194667,#194668),
(#194669,#194670),(#194671,#194672),(#194673,#194674),(#194675,#194676),
(#194677,#194678),(#194679,#194680)),.UNSPECIFIED.,.F.,.F.,.F.)
B_SPLINE_SURFACE_WITH_KNOTS((6,1,1,1,1,1,1,1,1,1,1,1,1,1,1,1,1,1,1,1,1,
1,1,1,1,1,1,1,1,1,1,1,1,1,1,1,1,1,1,1,1,1,1,1,1,1,1,1,1,1,1,1,1,1,1,1,1,
1,1,1,1,1,1,1,1,1,1,1,1,1,1,1,1,1,1,1,1,1,1,1,1,1,1,1,1,1,1,1,1,1,1,1,1,
1,1,1,1,1,1,1,1,1,1,1,1,1,1,1,1,1,1,1,1,1,1,1,1,1,1,1,1,1,1,1,1,1,1,1,1,
1,1,1,1,1,1,1,1,1,1,1,1,1,1,1,1,1,1,1,1,1,1,1,1,1,1,1,1,1,1,1,1,1,1,1,1,
1,1,1,1,1,1,1,1,1,1,1,1,1,1,1,1,1,1,1,1,1,1,1,1,1,1,1,1,1,1,1,1,1,1,1,6),
(2,2),(-1.,-0.995000000000001,-0.990000000000001,-0.985000000000001,-0.980000000000001,
-0.975000000000001,-0.970000000000001,-0.965000000000001,-0.960000000000001,
-0.955000000000001,-0.950000000000001,-0.945000000000001,-0.940000000000001,
-0.935000000000001,-0.930000000000001,-0.925000000000001,-0.920000000000001,
-0.915000000000001,-0.910000000000001,-0.905000000000001,-0.900000000000001,
-0.895000000000001,-0.890000000000001,-0.885000000000001,-0.880000000000001,
-0.875000000000001,-0.870000000000001,-0.865000000000001,-0.860000000000001,
-0.855000000000001,-0.850000000000001,-0.845000000000001,-0.840000000000001,
-0.835000000000001,-0.830000000000001,-0.825000000000001,-0.820000000000001,
-0.815000000000001,-0.810000000000001,-0.805000000000001,-0.800000000000001,
-0.795000000000001,-0.790000000000001,-0.785000000000001,-0.780000000000001,
-0.775000000000001,-0.770000000000001,-0.765000000000001,-0.760000000000001,
-0.755000000000001,-0.750000000000001,-0.745000000000001,-0.740000000000001,
-0.735000000000001,-0.730000000000001,-0.725000000000001,-0.720000000000001,
-0.715000000000001,-0.710000000000001,-0.705000000000001,-0.700000000000001,
-0.695000000000001,-0.690000000000001,-0.685,-0.68,-0.675,-0.67,-0.665,
-0.66,-0.655,-0.65,-0.645,-0.64,-0.635,-0.63,-0.625,-0.62,-0.615,-0.61,
-0.605,-0.6,-0.595,-0.59,-0.585,-0.58,-0.575,-0.57,-0.565,-0.56,-0.555,
-0.55,-0.545,-0.54,-0.535,-0.53,-0.525,-0.52,-0.515,-0.51,-0.505,-0.5,-0.495,
-0.49,-0.485,-0.48,-0.475,-0.47,-0.465,-0.46,-0.455,-0.45,-0.445,-0.44,
-0.435,-0.43,-0.425,-0.42,-0.415,-0.41,-0.405,-0.4,-0.395,-0.39,-0.385,
-0.38,-0.375,-0.37,-0.365,-0.36,-0.355,-0.35,-0.345,-0.34,-0.335,-0.33,
-0.325,-0.32,-0.315,-0.31,-0.305,-0.3,-0.295,-0.29,-0.285,-0.28,-0.275,
-0.27,-0.265,-0.26,-0.255,-0.25,-0.245,-0.24,-0.235,-0.23,-0.225,-0.22,
-0.215,-0.21,-0.205,-0.2,-0.195,-0.19,-0.185,-0.18,-0.175,-0.17,-0.165,
-0.16,-0.155,-0.15,-0.145,-0.14,-0.135,-0.13,-0.125,-0.12,-0.115,-0.11,
-0.105,-0.1,-0.095,-0.09,-0.085,-0.08,-0.075,-0.07,-0.065,-0.06,-0.055,
-0.05,-0.045,-0.04,-0.035,-0.03,-0.025,-0.02,-0.015,-0.01,-0.005,0.),(0.,
1.2),.UNSPECIFIED.)
GEOMETRIC_REPRESENTATION_ITEM()
RATIONAL_B_SPLINE_SURFACE(((1.,1.),(1.,1.),(1.,1.),(1.,1.),(1.,1.),(1.,
1.),(1.,1.),(1.,1.),(1.,1.),(1.,1.),(1.,1.),(1.,1.),(1.,1.),(1.,1.),(1.,
1.),(1.,1.),(1.,1.),(1.,1.),(1.,1.),(1.,1.),(1.,1.),(1.,1.),(1.,1.),(1.,
1.),(1.,1.),(1.,1.),(1.,1.),(1.,1.),(1.,1.),(1.,1.),(1.,1.),(1.,1.),(1.,
1.),(1.,1.),(1.,1.),(1.,1.),(1.,1.),(1.,1.),(1.,1.),(1.,1.),(1.,1.),(1.,
1.),(1.,1.),(1.,1.),(1.,1.),(1.,1.),(1.,1.),(1.,1.),(1.,1.),(1.,1.),(1.,
1.),(1.,1.),(1.,1.),(1.,1.),(1.,1.),(1.,1.),(1.,1.),(1.,1.),(1.,1.),(1.,
1.),(1.,1.),(1.,1.),(1.,1.),(1.,1.),(1.,1.),(1.,1.),(1.,1.),(1.,1.),(1.,
1.),(1.,1.),(1.,1.),(1.,1.),(1.,1.),(1.,1.),(1.,1.),(1.,1.),(1.,1.),(1.,
1.),(1.,1.),(1.,1.),(1.,1.),(1.,1.),(1.,1.),(1.,1.),(1.,1.),(1.,1.),(1.,
1.),(1.,1.),(1.,1.),(1.,1.),(1.,1.),(1.,1.),(1.,1.),(1.,1.),(1.,1.),(1.,
1.),(1.,1.),(1.,1.),(1.,1.),(1.,1.),(1.,1.),(1.,1.),(1.,1.),(1.,1.),(1.,
1.),(1.,1.),(1.,1.),(1.,1.),(1.,1.),(1.,1.),(1.,1.),(1.,1.),(1.,1.),(1.,
1.),(1.,1.),(1.,1.),(1.,1.),(1.,1.),(1.,1.),(1.,1.),(1.,1.),(1.,1.),(1.,
1.),(1.,1.),(1.,1.),(1.,1.),(1.,1.),(1.,1.),(1.,1.),(1.,1.),(1.,1.),(1.,
1.),(1.,1.),(1.,1.),(1.,1.),(1.,1.),(1.,1.),(1.,1.),(1.,1.),(1.,1.),(1.,
1.),(1.,1.),(1.,1.),(1.,1.),(1.,1.),(1.,1.),(1.,1.),(1.,1.),(1.,1.),(1.,
1.),(1.,1.),(1.,1.),(1.,1.),(1.,1.),(1.,1.),(1.,1.),(1.,1.),(1.,1.),(1.,
1.),(1.,1.),(1.,1.),(1.,1.),(1.,1.),(1.,1.),(1.,1.),(1.,1.),(1.,1.),(1.,
1.),(1.,1.),(1.,1.),(1.,1.),(1.,1.),(1.,1.),(1.,1.),(1.,1.),(1.,1.),(1.,
1.),(1.,1.),(1.,1.),(1.,1.),(1.,1.),(1.,1.),(1.,1.),(1.,1.),(1.,1.),(1.,
1.),(1.,1.),(1.,1.),(1.,1.),(1.,1.),(1.,1.),(1.,1.),(1.,1.),(1.,1.),(1.,
1.),(1.,1.),(1.,1.),(1.,1.),(1.,1.),(1.,1.),(1.,1.),(1.,1.),(1.,1.),(1.,
1.),(1.,1.)))
REPRESENTATION_ITEM('')
SURFACE()
);
#1042=(
BOUNDED_SURFACE()
B_SPLINE_SURFACE(5,1,((#194888,#194889),(#194890,#194891),(#194892,#194893),
(#194894,#194895),(#194896,#194897),(#194898,#194899),(#194900,#194901),
(#194902,#194903),(#194904,#194905),(#194906,#194907),(#194908,#194909),
(#194910,#194911),(#194912,#194913),(#194914,#194915),(#194916,#194917),
(#194918,#194919),(#194920,#194921),(#194922,#194923),(#194924,#194925),
(#194926,#194927),(#194928,#194929),(#194930,#194931),(#194932,#194933),
(#194934,#194935),(#194936,#194937),(#194938,#194939),(#194940,#194941),
(#194942,#194943),(#194944,#194945),(#194946,#194947),(#194948,#194949),
(#194950,#194951),(#194952,#194953),(#194954,#194955),(#194956,#194957),
(#194958,#194959),(#194960,#194961),(#194962,#194963),(#194964,#194965),
(#194966,#194967),(#194968,#194969),(#194970,#194971),(#194972,#194973),
(#194974,#194975),(#194976,#194977),(#194978,#194979),(#194980,#194981),
(#194982,#194983),(#194984,#194985),(#194986,#194987),(#194988,#194989),
(#194990,#194991),(#194992,#194993),(#194994,#194995),(#194996,#194997),
(#194998,#194999),(#195000,#195001),(#195002,#195003),(#195004,#195005),
(#195006,#195007),(#195008,#195009),(#195010,#195011),(#195012,#195013),
(#195014,#195015),(#195016,#195017),(#195018,#195019),(#195020,#195021),
(#195022,#195023),(#195024,#195025),(#195026,#195027),(#195028,#195029),
(#195030,#195031),(#195032,#195033),(#195034,#195035),(#195036,#195037),
(#195038,#195039),(#195040,#195041),(#195042,#195043),(#195044,#195045),
(#195046,#195047),(#195048,#195049),(#195050,#195051),(#195052,#195053),
(#195054,#195055),(#195056,#195057),(#195058,#195059),(#195060,#195061),
(#195062,#195063),(#195064,#195065),(#195066,#195067),(#195068,#195069),
(#195070,#195071),(#195072,#195073),(#195074,#195075),(#195076,#195077),
(#195078,#195079),(#195080,#195081),(#195082,#195083),(#195084,#195085),
(#195086,#195087),(#195088,#195089),(#195090,#195091),(#195092,#195093),
(#195094,#195095),(#195096,#195097),(#195098,#195099),(#195100,#195101),
(#195102,#195103),(#195104,#195105),(#195106,#195107),(#195108,#195109),
(#195110,#195111),(#195112,#195113),(#195114,#195115),(#195116,#195117),
(#195118,#195119),(#195120,#195121),(#195122,#195123),(#195124,#195125),
(#195126,#195127),(#195128,#195129),(#195130,#195131),(#195132,#195133),
(#195134,#195135),(#195136,#195137),(#195138,#195139),(#195140,#195141),
(#195142,#195143),(#195144,#195145),(#195146,#195147),(#195148,#195149),
(#195150,#195151),(#195152,#195153),(#195154,#195155),(#195156,#195157),
(#195158,#195159),(#195160,#195161),(#195162,#195163),(#195164,#195165),
(#195166,#195167),(#195168,#195169),(#195170,#195171),(#195172,#195173),
(#195174,#195175),(#195176,#195177),(#195178,#195179),(#195180,#195181),
(#195182,#195183),(#195184,#195185),(#195186,#195187),(#195188,#195189),
(#195190,#195191),(#195192,#195193),(#195194,#195195),(#195196,#195197),
(#195198,#195199),(#195200,#195201),(#195202,#195203),(#195204,#195205),
(#195206,#195207),(#195208,#195209),(#195210,#195211),(#195212,#195213),
(#195214,#195215),(#195216,#195217),(#195218,#195219),(#195220,#195221),
(#195222,#195223),(#195224,#195225),(#195226,#195227),(#195228,#195229),
(#195230,#195231),(#195232,#195233),(#195234,#195235),(#195236,#195237),
(#195238,#195239),(#195240,#195241),(#195242,#195243),(#195244,#195245),
(#195246,#195247),(#195248,#195249),(#195250,#195251),(#195252,#195253),
(#195254,#195255),(#195256,#195257),(#195258,#195259),(#195260,#195261),
(#195262,#195263),(#195264,#195265),(#195266,#195267),(#195268,#195269),
(#195270,#195271),(#195272,#195273),(#195274,#195275),(#195276,#195277),
(#195278,#195279),(#195280,#195281),(#195282,#195283),(#195284,#195285),
(#195286,#195287),(#195288,#195289),(#195290,#195291),(#195292,#195293),
(#195294,#195295),(#195296,#195297)),.UNSPECIFIED.,.F.,.F.,.F.)
B_SPLINE_SURFACE_WITH_KNOTS((6,1,1,1,1,1,1,1,1,1,1,1,1,1,1,1,1,1,1,1,1,
1,1,1,1,1,1,1,1,1,1,1,1,1,1,1,1,1,1,1,1,1,1,1,1,1,1,1,1,1,1,1,1,1,1,1,1,
1,1,1,1,1,1,1,1,1,1,1,1,1,1,1,1,1,1,1,1,1,1,1,1,1,1,1,1,1,1,1,1,1,1,1,1,
1,1,1,1,1,1,1,1,1,1,1,1,1,1,1,1,1,1,1,1,1,1,1,1,1,1,1,1,1,1,1,1,1,1,1,1,
1,1,1,1,1,1,1,1,1,1,1,1,1,1,1,1,1,1,1,1,1,1,1,1,1,1,1,1,1,1,1,1,1,1,1,1,
1,1,1,1,1,1,1,1,1,1,1,1,1,1,1,1,1,1,1,1,1,1,1,1,1,1,1,1,1,1,1,1,1,1,1,6),
(2,2),(0.,0.005,0.01,0.015,0.02,0.025,0.03,0.035,0.04,0.045,0.05,0.055,
0.06,0.065,0.07,0.075,0.08,0.085,0.09,0.095,0.1,0.105,0.11,0.115,0.12,0.125,
0.13,0.135,0.14,0.145,0.15,0.155,0.16,0.165,0.17,0.175,0.18,0.185,0.19,
0.195,0.2,0.205,0.21,0.215,0.22,0.225,0.23,0.235,0.24,0.245,0.25,0.255,
0.26,0.265,0.27,0.275,0.28,0.285,0.29,0.295,0.3,0.305,0.31,0.315,0.32,0.325,
0.33,0.335,0.34,0.345,0.35,0.355,0.36,0.365,0.37,0.375,0.38,0.385,0.39,
0.395,0.4,0.405,0.41,0.415,0.42,0.425,0.43,0.435,0.44,0.445,0.45,0.455,
0.46,0.465,0.47,0.475,0.48,0.485,0.49,0.495,0.5,0.505,0.51,0.515,0.52,0.525,
0.53,0.535,0.54,0.545,0.55,0.555,0.56,0.565,0.57,0.575,0.58,0.585,0.59,
0.595,0.6,0.605,0.61,0.615,0.62,0.625,0.63,0.635,0.64,0.645,0.65,0.655,
0.66,0.665,0.67,0.675,0.68,0.685,0.690000000000001,0.695000000000001,0.700000000000001,
0.705000000000001,0.710000000000001,0.715000000000001,0.720000000000001,
0.725000000000001,0.730000000000001,0.735000000000001,0.740000000000001,
0.745000000000001,0.750000000000001,0.755000000000001,0.760000000000001,
0.765000000000001,0.770000000000001,0.775000000000001,0.780000000000001,
0.785000000000001,0.790000000000001,0.795000000000001,0.800000000000001,
0.805000000000001,0.810000000000001,0.815000000000001,0.820000000000001,
0.825000000000001,0.830000000000001,0.835000000000001,0.840000000000001,
0.845000000000001,0.850000000000001,0.855000000000001,0.860000000000001,
0.865000000000001,0.870000000000001,0.875000000000001,0.880000000000001,
0.885000000000001,0.890000000000001,0.895000000000001,0.900000000000001,
0.905000000000001,0.910000000000001,0.915000000000001,0.920000000000001,
0.925000000000001,0.930000000000001,0.935000000000001,0.940000000000001,
0.945000000000001,0.950000000000001,0.955000000000001,0.960000000000001,
0.965000000000001,0.970000000000001,0.975000000000001,0.980000000000001,
0.985000000000001,0.990000000000001,0.995000000000001,1.),(0.,1.2),
 .UNSPECIFIED.)
GEOMETRIC_REPRESENTATION_ITEM()
RATIONAL_B_SPLINE_SURFACE(((1.,1.),(1.,1.),(1.,1.),(1.,1.),(1.,1.),(1.,
1.),(1.,1.),(1.,1.),(1.,1.),(1.,1.),(1.,1.),(1.,1.),(1.,1.),(1.,1.),(1.,
1.),(1.,1.),(1.,1.),(1.,1.),(1.,1.),(1.,1.),(1.,1.),(1.,1.),(1.,1.),(1.,
1.),(1.,1.),(1.,1.),(1.,1.),(1.,1.),(1.,1.),(1.,1.),(1.,1.),(1.,1.),(1.,
1.),(1.,1.),(1.,1.),(1.,1.),(1.,1.),(1.,1.),(1.,1.),(1.,1.),(1.,1.),(1.,
1.),(1.,1.),(1.,1.),(1.,1.),(1.,1.),(1.,1.),(1.,1.),(1.,1.),(1.,1.),(1.,
1.),(1.,1.),(1.,1.),(1.,1.),(1.,1.),(1.,1.),(1.,1.),(1.,1.),(1.,1.),(1.,
1.),(1.,1.),(1.,1.),(1.,1.),(1.,1.),(1.,1.),(1.,1.),(1.,1.),(1.,1.),(1.,
1.),(1.,1.),(1.,1.),(1.,1.),(1.,1.),(1.,1.),(1.,1.),(1.,1.),(1.,1.),(1.,
1.),(1.,1.),(1.,1.),(1.,1.),(1.,1.),(1.,1.),(1.,1.),(1.,1.),(1.,1.),(1.,
1.),(1.,1.),(1.,1.),(1.,1.),(1.,1.),(1.,1.),(1.,1.),(1.,1.),(1.,1.),(1.,
1.),(1.,1.),(1.,1.),(1.,1.),(1.,1.),(1.,1.),(1.,1.),(1.,1.),(1.,1.),(1.,
1.),(1.,1.),(1.,1.),(1.,1.),(1.,1.),(1.,1.),(1.,1.),(1.,1.),(1.,1.),(1.,
1.),(1.,1.),(1.,1.),(1.,1.),(1.,1.),(1.,1.),(1.,1.),(1.,1.),(1.,1.),(1.,
1.),(1.,1.),(1.,1.),(1.,1.),(1.,1.),(1.,1.),(1.,1.),(1.,1.),(1.,1.),(1.,
1.),(1.,1.),(1.,1.),(1.,1.),(1.,1.),(1.,1.),(1.,1.),(1.,1.),(1.,1.),(1.,
1.),(1.,1.),(1.,1.),(1.,1.),(1.,1.),(1.,1.),(1.,1.),(1.,1.),(1.,1.),(1.,
1.),(1.,1.),(1.,1.),(1.,1.),(1.,1.),(1.,1.),(1.,1.),(1.,1.),(1.,1.),(1.,
1.),(1.,1.),(1.,1.),(1.,1.),(1.,1.),(1.,1.),(1.,1.),(1.,1.),(1.,1.),(1.,
1.),(1.,1.),(1.,1.),(1.,1.),(1.,1.),(1.,1.),(1.,1.),(1.,1.),(1.,1.),(1.,
1.),(1.,1.),(1.,1.),(1.,1.),(1.,1.),(1.,1.),(1.,1.),(1.,1.),(1.,1.),(1.,
1.),(1.,1.),(1.,1.),(1.,1.),(1.,1.),(1.,1.),(1.,1.),(1.,1.),(1.,1.),(1.,
1.),(1.,1.),(1.,1.),(1.,1.),(1.,1.),(1.,1.),(1.,1.),(1.,1.),(1.,1.),(1.,
1.),(1.,1.)))
REPRESENTATION_ITEM('')
SURFACE()
);
#1043=(
BOUNDED_SURFACE()
B_SPLINE_SURFACE(5,1,((#195509,#195510),(#195511,#195512),(#195513,#195514),
(#195515,#195516),(#195517,#195518),(#195519,#195520),(#195521,#195522),
(#195523,#195524),(#195525,#195526),(#195527,#195528),(#195529,#195530),
(#195531,#195532),(#195533,#195534),(#195535,#195536),(#195537,#195538),
(#195539,#195540),(#195541,#195542),(#195543,#195544),(#195545,#195546),
(#195547,#195548),(#195549,#195550),(#195551,#195552),(#195553,#195554),
(#195555,#195556),(#195557,#195558),(#195559,#195560),(#195561,#195562),
(#195563,#195564),(#195565,#195566),(#195567,#195568),(#195569,#195570),
(#195571,#195572),(#195573,#195574),(#195575,#195576),(#195577,#195578),
(#195579,#195580),(#195581,#195582),(#195583,#195584),(#195585,#195586),
(#195587,#195588),(#195589,#195590),(#195591,#195592),(#195593,#195594),
(#195595,#195596),(#195597,#195598),(#195599,#195600),(#195601,#195602),
(#195603,#195604),(#195605,#195606),(#195607,#195608),(#195609,#195610),
(#195611,#195612),(#195613,#195614),(#195615,#195616),(#195617,#195618),
(#195619,#195620),(#195621,#195622),(#195623,#195624),(#195625,#195626),
(#195627,#195628),(#195629,#195630),(#195631,#195632),(#195633,#195634),
(#195635,#195636),(#195637,#195638),(#195639,#195640),(#195641,#195642),
(#195643,#195644),(#195645,#195646),(#195647,#195648),(#195649,#195650),
(#195651,#195652),(#195653,#195654),(#195655,#195656),(#195657,#195658),
(#195659,#195660),(#195661,#195662),(#195663,#195664),(#195665,#195666),
(#195667,#195668),(#195669,#195670),(#195671,#195672),(#195673,#195674),
(#195675,#195676),(#195677,#195678),(#195679,#195680),(#195681,#195682),
(#195683,#195684),(#195685,#195686),(#195687,#195688),(#195689,#195690),
(#195691,#195692),(#195693,#195694),(#195695,#195696),(#195697,#195698),
(#195699,#195700),(#195701,#195702),(#195703,#195704),(#195705,#195706),
(#195707,#195708),(#195709,#195710),(#195711,#195712),(#195713,#195714),
(#195715,#195716),(#195717,#195718),(#195719,#195720),(#195721,#195722),
(#195723,#195724),(#195725,#195726),(#195727,#195728),(#195729,#195730),
(#195731,#195732),(#195733,#195734),(#195735,#195736),(#195737,#195738),
(#195739,#195740),(#195741,#195742),(#195743,#195744),(#195745,#195746),
(#195747,#195748),(#195749,#195750),(#195751,#195752),(#195753,#195754),
(#195755,#195756),(#195757,#195758),(#195759,#195760),(#195761,#195762),
(#195763,#195764),(#195765,#195766),(#195767,#195768),(#195769,#195770),
(#195771,#195772),(#195773,#195774),(#195775,#195776),(#195777,#195778),
(#195779,#195780),(#195781,#195782),(#195783,#195784),(#195785,#195786),
(#195787,#195788),(#195789,#195790),(#195791,#195792),(#195793,#195794),
(#195795,#195796),(#195797,#195798),(#195799,#195800),(#195801,#195802),
(#195803,#195804),(#195805,#195806),(#195807,#195808),(#195809,#195810),
(#195811,#195812),(#195813,#195814),(#195815,#195816),(#195817,#195818),
(#195819,#195820),(#195821,#195822),(#195823,#195824),(#195825,#195826),
(#195827,#195828),(#195829,#195830),(#195831,#195832),(#195833,#195834),
(#195835,#195836),(#195837,#195838),(#195839,#195840),(#195841,#195842),
(#195843,#195844),(#195845,#195846),(#195847,#195848),(#195849,#195850),
(#195851,#195852),(#195853,#195854),(#195855,#195856),(#195857,#195858),
(#195859,#195860),(#195861,#195862),(#195863,#195864),(#195865,#195866),
(#195867,#195868),(#195869,#195870),(#195871,#195872),(#195873,#195874),
(#195875,#195876),(#195877,#195878),(#195879,#195880),(#195881,#195882),
(#195883,#195884),(#195885,#195886),(#195887,#195888),(#195889,#195890),
(#195891,#195892),(#195893,#195894),(#195895,#195896),(#195897,#195898),
(#195899,#195900),(#195901,#195902),(#195903,#195904),(#195905,#195906),
(#195907,#195908),(#195909,#195910),(#195911,#195912),(#195913,#195914),
(#195915,#195916),(#195917,#195918)),.UNSPECIFIED.,.F.,.F.,.F.)
B_SPLINE_SURFACE_WITH_KNOTS((6,1,1,1,1,1,1,1,1,1,1,1,1,1,1,1,1,1,1,1,1,
1,1,1,1,1,1,1,1,1,1,1,1,1,1,1,1,1,1,1,1,1,1,1,1,1,1,1,1,1,1,1,1,1,1,1,1,
1,1,1,1,1,1,1,1,1,1,1,1,1,1,1,1,1,1,1,1,1,1,1,1,1,1,1,1,1,1,1,1,1,1,1,1,
1,1,1,1,1,1,1,1,1,1,1,1,1,1,1,1,1,1,1,1,1,1,1,1,1,1,1,1,1,1,1,1,1,1,1,1,
1,1,1,1,1,1,1,1,1,1,1,1,1,1,1,1,1,1,1,1,1,1,1,1,1,1,1,1,1,1,1,1,1,1,1,1,
1,1,1,1,1,1,1,1,1,1,1,1,1,1,1,1,1,1,1,1,1,1,1,1,1,1,1,1,1,1,1,1,1,1,1,6),
(2,2),(-1.,-0.995000000000001,-0.990000000000001,-0.985000000000001,-0.980000000000001,
-0.975000000000001,-0.970000000000001,-0.965000000000001,-0.960000000000001,
-0.955000000000001,-0.950000000000001,-0.945000000000001,-0.940000000000001,
-0.935000000000001,-0.930000000000001,-0.925000000000001,-0.920000000000001,
-0.915000000000001,-0.910000000000001,-0.905000000000001,-0.900000000000001,
-0.895000000000001,-0.890000000000001,-0.885000000000001,-0.880000000000001,
-0.875000000000001,-0.870000000000001,-0.865000000000001,-0.860000000000001,
-0.855000000000001,-0.850000000000001,-0.845000000000001,-0.840000000000001,
-0.835000000000001,-0.830000000000001,-0.825000000000001,-0.820000000000001,
-0.815000000000001,-0.810000000000001,-0.805000000000001,-0.800000000000001,
-0.795000000000001,-0.790000000000001,-0.785000000000001,-0.780000000000001,
-0.775000000000001,-0.770000000000001,-0.765000000000001,-0.760000000000001,
-0.755000000000001,-0.750000000000001,-0.745000000000001,-0.740000000000001,
-0.735000000000001,-0.730000000000001,-0.725000000000001,-0.720000000000001,
-0.715000000000001,-0.710000000000001,-0.705000000000001,-0.700000000000001,
-0.695000000000001,-0.690000000000001,-0.685,-0.68,-0.675,-0.67,-0.665,
-0.66,-0.655,-0.65,-0.645,-0.64,-0.635,-0.63,-0.625,-0.62,-0.615,-0.61,
-0.605,-0.6,-0.595,-0.59,-0.585,-0.58,-0.575,-0.57,-0.565,-0.56,-0.555,
-0.55,-0.545,-0.54,-0.535,-0.53,-0.525,-0.52,-0.515,-0.51,-0.505,-0.5,-0.495,
-0.49,-0.485,-0.48,-0.475,-0.47,-0.465,-0.46,-0.455,-0.45,-0.445,-0.44,
-0.435,-0.43,-0.425,-0.42,-0.415,-0.41,-0.405,-0.4,-0.395,-0.39,-0.385,
-0.38,-0.375,-0.37,-0.365,-0.36,-0.355,-0.35,-0.345,-0.34,-0.335,-0.33,
-0.325,-0.32,-0.315,-0.31,-0.305,-0.3,-0.295,-0.29,-0.285,-0.28,-0.275,
-0.27,-0.265,-0.26,-0.255,-0.25,-0.245,-0.24,-0.235,-0.23,-0.225,-0.22,
-0.215,-0.21,-0.205,-0.2,-0.195,-0.19,-0.185,-0.18,-0.175,-0.17,-0.165,
-0.16,-0.155,-0.15,-0.145,-0.14,-0.135,-0.13,-0.125,-0.12,-0.115,-0.11,
-0.105,-0.1,-0.095,-0.09,-0.085,-0.08,-0.075,-0.07,-0.065,-0.06,-0.055,
-0.05,-0.045,-0.04,-0.035,-0.03,-0.025,-0.02,-0.015,-0.01,-0.005,0.),(0.,
1.2),.UNSPECIFIED.)
GEOMETRIC_REPRESENTATION_ITEM()
RATIONAL_B_SPLINE_SURFACE(((1.,1.),(1.,1.),(1.,1.),(1.,1.),(1.,1.),(1.,
1.),(1.,1.),(1.,1.),(1.,1.),(1.,1.),(1.,1.),(1.,1.),(1.,1.),(1.,1.),(1.,
1.),(1.,1.),(1.,1.),(1.,1.),(1.,1.),(1.,1.),(1.,1.),(1.,1.),(1.,1.),(1.,
1.),(1.,1.),(1.,1.),(1.,1.),(1.,1.),(1.,1.),(1.,1.),(1.,1.),(1.,1.),(1.,
1.),(1.,1.),(1.,1.),(1.,1.),(1.,1.),(1.,1.),(1.,1.),(1.,1.),(1.,1.),(1.,
1.),(1.,1.),(1.,1.),(1.,1.),(1.,1.),(1.,1.),(1.,1.),(1.,1.),(1.,1.),(1.,
1.),(1.,1.),(1.,1.),(1.,1.),(1.,1.),(1.,1.),(1.,1.),(1.,1.),(1.,1.),(1.,
1.),(1.,1.),(1.,1.),(1.,1.),(1.,1.),(1.,1.),(1.,1.),(1.,1.),(1.,1.),(1.,
1.),(1.,1.),(1.,1.),(1.,1.),(1.,1.),(1.,1.),(1.,1.),(1.,1.),(1.,1.),(1.,
1.),(1.,1.),(1.,1.),(1.,1.),(1.,1.),(1.,1.),(1.,1.),(1.,1.),(1.,1.),(1.,
1.),(1.,1.),(1.,1.),(1.,1.),(1.,1.),(1.,1.),(1.,1.),(1.,1.),(1.,1.),(1.,
1.),(1.,1.),(1.,1.),(1.,1.),(1.,1.),(1.,1.),(1.,1.),(1.,1.),(1.,1.),(1.,
1.),(1.,1.),(1.,1.),(1.,1.),(1.,1.),(1.,1.),(1.,1.),(1.,1.),(1.,1.),(1.,
1.),(1.,1.),(1.,1.),(1.,1.),(1.,1.),(1.,1.),(1.,1.),(1.,1.),(1.,1.),(1.,
1.),(1.,1.),(1.,1.),(1.,1.),(1.,1.),(1.,1.),(1.,1.),(1.,1.),(1.,1.),(1.,
1.),(1.,1.),(1.,1.),(1.,1.),(1.,1.),(1.,1.),(1.,1.),(1.,1.),(1.,1.),(1.,
1.),(1.,1.),(1.,1.),(1.,1.),(1.,1.),(1.,1.),(1.,1.),(1.,1.),(1.,1.),(1.,
1.),(1.,1.),(1.,1.),(1.,1.),(1.,1.),(1.,1.),(1.,1.),(1.,1.),(1.,1.),(1.,
1.),(1.,1.),(1.,1.),(1.,1.),(1.,1.),(1.,1.),(1.,1.),(1.,1.),(1.,1.),(1.,
1.),(1.,1.),(1.,1.),(1.,1.),(1.,1.),(1.,1.),(1.,1.),(1.,1.),(1.,1.),(1.,
1.),(1.,1.),(1.,1.),(1.,1.),(1.,1.),(1.,1.),(1.,1.),(1.,1.),(1.,1.),(1.,
1.),(1.,1.),(1.,1.),(1.,1.),(1.,1.),(1.,1.),(1.,1.),(1.,1.),(1.,1.),(1.,
1.),(1.,1.),(1.,1.),(1.,1.),(1.,1.),(1.,1.),(1.,1.),(1.,1.),(1.,1.),(1.,
1.),(1.,1.)))
REPRESENTATION_ITEM('')
SURFACE()
);
#1044=(
BOUNDED_SURFACE()
B_SPLINE_SURFACE(5,1,((#196126,#196127),(#196128,#196129),(#196130,#196131),
(#196132,#196133),(#196134,#196135),(#196136,#196137),(#196138,#196139),
(#196140,#196141),(#196142,#196143),(#196144,#196145),(#196146,#196147),
(#196148,#196149),(#196150,#196151),(#196152,#196153),(#196154,#196155),
(#196156,#196157),(#196158,#196159),(#196160,#196161),(#196162,#196163),
(#196164,#196165),(#196166,#196167),(#196168,#196169),(#196170,#196171),
(#196172,#196173),(#196174,#196175),(#196176,#196177),(#196178,#196179),
(#196180,#196181),(#196182,#196183),(#196184,#196185),(#196186,#196187),
(#196188,#196189),(#196190,#196191),(#196192,#196193),(#196194,#196195),
(#196196,#196197),(#196198,#196199),(#196200,#196201),(#196202,#196203),
(#196204,#196205),(#196206,#196207),(#196208,#196209),(#196210,#196211),
(#196212,#196213),(#196214,#196215),(#196216,#196217),(#196218,#196219),
(#196220,#196221),(#196222,#196223),(#196224,#196225),(#196226,#196227),
(#196228,#196229),(#196230,#196231),(#196232,#196233),(#196234,#196235),
(#196236,#196237),(#196238,#196239),(#196240,#196241),(#196242,#196243),
(#196244,#196245),(#196246,#196247),(#196248,#196249),(#196250,#196251),
(#196252,#196253),(#196254,#196255),(#196256,#196257),(#196258,#196259),
(#196260,#196261),(#196262,#196263),(#196264,#196265),(#196266,#196267),
(#196268,#196269),(#196270,#196271),(#196272,#196273),(#196274,#196275),
(#196276,#196277),(#196278,#196279),(#196280,#196281),(#196282,#196283),
(#196284,#196285),(#196286,#196287),(#196288,#196289),(#196290,#196291),
(#196292,#196293),(#196294,#196295),(#196296,#196297),(#196298,#196299),
(#196300,#196301),(#196302,#196303),(#196304,#196305),(#196306,#196307),
(#196308,#196309),(#196310,#196311),(#196312,#196313),(#196314,#196315),
(#196316,#196317),(#196318,#196319),(#196320,#196321),(#196322,#196323),
(#196324,#196325),(#196326,#196327),(#196328,#196329),(#196330,#196331),
(#196332,#196333),(#196334,#196335),(#196336,#196337),(#196338,#196339),
(#196340,#196341),(#196342,#196343),(#196344,#196345),(#196346,#196347),
(#196348,#196349),(#196350,#196351),(#196352,#196353),(#196354,#196355),
(#196356,#196357),(#196358,#196359),(#196360,#196361),(#196362,#196363),
(#196364,#196365),(#196366,#196367),(#196368,#196369),(#196370,#196371),
(#196372,#196373),(#196374,#196375),(#196376,#196377),(#196378,#196379),
(#196380,#196381),(#196382,#196383),(#196384,#196385),(#196386,#196387),
(#196388,#196389),(#196390,#196391),(#196392,#196393),(#196394,#196395),
(#196396,#196397),(#196398,#196399),(#196400,#196401),(#196402,#196403),
(#196404,#196405),(#196406,#196407),(#196408,#196409),(#196410,#196411),
(#196412,#196413),(#196414,#196415),(#196416,#196417),(#196418,#196419),
(#196420,#196421),(#196422,#196423),(#196424,#196425),(#196426,#196427),
(#196428,#196429),(#196430,#196431),(#196432,#196433),(#196434,#196435),
(#196436,#196437),(#196438,#196439),(#196440,#196441),(#196442,#196443),
(#196444,#196445),(#196446,#196447),(#196448,#196449),(#196450,#196451),
(#196452,#196453),(#196454,#196455),(#196456,#196457),(#196458,#196459),
(#196460,#196461),(#196462,#196463),(#196464,#196465),(#196466,#196467),
(#196468,#196469),(#196470,#196471),(#196472,#196473),(#196474,#196475),
(#196476,#196477),(#196478,#196479),(#196480,#196481),(#196482,#196483),
(#196484,#196485),(#196486,#196487),(#196488,#196489),(#196490,#196491),
(#196492,#196493),(#196494,#196495),(#196496,#196497),(#196498,#196499),
(#196500,#196501),(#196502,#196503),(#196504,#196505),(#196506,#196507),
(#196508,#196509),(#196510,#196511),(#196512,#196513),(#196514,#196515),
(#196516,#196517),(#196518,#196519),(#196520,#196521),(#196522,#196523),
(#196524,#196525),(#196526,#196527),(#196528,#196529),(#196530,#196531),
(#196532,#196533),(#196534,#196535)),.UNSPECIFIED.,.F.,.F.,.F.)
B_SPLINE_SURFACE_WITH_KNOTS((6,1,1,1,1,1,1,1,1,1,1,1,1,1,1,1,1,1,1,1,1,
1,1,1,1,1,1,1,1,1,1,1,1,1,1,1,1,1,1,1,1,1,1,1,1,1,1,1,1,1,1,1,1,1,1,1,1,
1,1,1,1,1,1,1,1,1,1,1,1,1,1,1,1,1,1,1,1,1,1,1,1,1,1,1,1,1,1,1,1,1,1,1,1,
1,1,1,1,1,1,1,1,1,1,1,1,1,1,1,1,1,1,1,1,1,1,1,1,1,1,1,1,1,1,1,1,1,1,1,1,
1,1,1,1,1,1,1,1,1,1,1,1,1,1,1,1,1,1,1,1,1,1,1,1,1,1,1,1,1,1,1,1,1,1,1,1,
1,1,1,1,1,1,1,1,1,1,1,1,1,1,1,1,1,1,1,1,1,1,1,1,1,1,1,1,1,1,1,1,1,1,1,6),
(2,2),(0.,0.005,0.01,0.015,0.02,0.025,0.03,0.035,0.04,0.045,0.05,0.055,
0.06,0.065,0.07,0.075,0.08,0.085,0.09,0.095,0.1,0.105,0.11,0.115,0.12,0.125,
0.13,0.135,0.14,0.145,0.15,0.155,0.16,0.165,0.17,0.175,0.18,0.185,0.19,
0.195,0.2,0.205,0.21,0.215,0.22,0.225,0.23,0.235,0.24,0.245,0.25,0.255,
0.26,0.265,0.27,0.275,0.28,0.285,0.29,0.295,0.3,0.305,0.31,0.315,0.32,0.325,
0.33,0.335,0.34,0.345,0.35,0.355,0.36,0.365,0.37,0.375,0.38,0.385,0.39,
0.395,0.4,0.405,0.41,0.415,0.42,0.425,0.43,0.435,0.44,0.445,0.45,0.455,
0.46,0.465,0.47,0.475,0.48,0.485,0.49,0.495,0.5,0.505,0.51,0.515,0.52,0.525,
0.53,0.535,0.54,0.545,0.55,0.555,0.56,0.565,0.57,0.575,0.58,0.585,0.59,
0.595,0.6,0.605,0.61,0.615,0.62,0.625,0.63,0.635,0.64,0.645,0.65,0.655,
0.66,0.665,0.67,0.675,0.68,0.685,0.690000000000001,0.695000000000001,0.700000000000001,
0.705000000000001,0.710000000000001,0.715000000000001,0.720000000000001,
0.725000000000001,0.730000000000001,0.735000000000001,0.740000000000001,
0.745000000000001,0.750000000000001,0.755000000000001,0.760000000000001,
0.765000000000001,0.770000000000001,0.775000000000001,0.780000000000001,
0.785000000000001,0.790000000000001,0.795000000000001,0.800000000000001,
0.805000000000001,0.810000000000001,0.815000000000001,0.820000000000001,
0.825000000000001,0.830000000000001,0.835000000000001,0.840000000000001,
0.845000000000001,0.850000000000001,0.855000000000001,0.860000000000001,
0.865000000000001,0.870000000000001,0.875000000000001,0.880000000000001,
0.885000000000001,0.890000000000001,0.895000000000001,0.900000000000001,
0.905000000000001,0.910000000000001,0.915000000000001,0.920000000000001,
0.925000000000001,0.930000000000001,0.935000000000001,0.940000000000001,
0.945000000000001,0.950000000000001,0.955000000000001,0.960000000000001,
0.965000000000001,0.970000000000001,0.975000000000001,0.980000000000001,
0.985000000000001,0.990000000000001,0.995000000000001,1.),(0.,1.2),
 .UNSPECIFIED.)
GEOMETRIC_REPRESENTATION_ITEM()
RATIONAL_B_SPLINE_SURFACE(((1.,1.),(1.,1.),(1.,1.),(1.,1.),(1.,1.),(1.,
1.),(1.,1.),(1.,1.),(1.,1.),(1.,1.),(1.,1.),(1.,1.),(1.,1.),(1.,1.),(1.,
1.),(1.,1.),(1.,1.),(1.,1.),(1.,1.),(1.,1.),(1.,1.),(1.,1.),(1.,1.),(1.,
1.),(1.,1.),(1.,1.),(1.,1.),(1.,1.),(1.,1.),(1.,1.),(1.,1.),(1.,1.),(1.,
1.),(1.,1.),(1.,1.),(1.,1.),(1.,1.),(1.,1.),(1.,1.),(1.,1.),(1.,1.),(1.,
1.),(1.,1.),(1.,1.),(1.,1.),(1.,1.),(1.,1.),(1.,1.),(1.,1.),(1.,1.),(1.,
1.),(1.,1.),(1.,1.),(1.,1.),(1.,1.),(1.,1.),(1.,1.),(1.,1.),(1.,1.),(1.,
1.),(1.,1.),(1.,1.),(1.,1.),(1.,1.),(1.,1.),(1.,1.),(1.,1.),(1.,1.),(1.,
1.),(1.,1.),(1.,1.),(1.,1.),(1.,1.),(1.,1.),(1.,1.),(1.,1.),(1.,1.),(1.,
1.),(1.,1.),(1.,1.),(1.,1.),(1.,1.),(1.,1.),(1.,1.),(1.,1.),(1.,1.),(1.,
1.),(1.,1.),(1.,1.),(1.,1.),(1.,1.),(1.,1.),(1.,1.),(1.,1.),(1.,1.),(1.,
1.),(1.,1.),(1.,1.),(1.,1.),(1.,1.),(1.,1.),(1.,1.),(1.,1.),(1.,1.),(1.,
1.),(1.,1.),(1.,1.),(1.,1.),(1.,1.),(1.,1.),(1.,1.),(1.,1.),(1.,1.),(1.,
1.),(1.,1.),(1.,1.),(1.,1.),(1.,1.),(1.,1.),(1.,1.),(1.,1.),(1.,1.),(1.,
1.),(1.,1.),(1.,1.),(1.,1.),(1.,1.),(1.,1.),(1.,1.),(1.,1.),(1.,1.),(1.,
1.),(1.,1.),(1.,1.),(1.,1.),(1.,1.),(1.,1.),(1.,1.),(1.,1.),(1.,1.),(1.,
1.),(1.,1.),(1.,1.),(1.,1.),(1.,1.),(1.,1.),(1.,1.),(1.,1.),(1.,1.),(1.,
1.),(1.,1.),(1.,1.),(1.,1.),(1.,1.),(1.,1.),(1.,1.),(1.,1.),(1.,1.),(1.,
1.),(1.,1.),(1.,1.),(1.,1.),(1.,1.),(1.,1.),(1.,1.),(1.,1.),(1.,1.),(1.,
1.),(1.,1.),(1.,1.),(1.,1.),(1.,1.),(1.,1.),(1.,1.),(1.,1.),(1.,1.),(1.,
1.),(1.,1.),(1.,1.),(1.,1.),(1.,1.),(1.,1.),(1.,1.),(1.,1.),(1.,1.),(1.,
1.),(1.,1.),(1.,1.),(1.,1.),(1.,1.),(1.,1.),(1.,1.),(1.,1.),(1.,1.),(1.,
1.),(1.,1.),(1.,1.),(1.,1.),(1.,1.),(1.,1.),(1.,1.),(1.,1.),(1.,1.),(1.,
1.),(1.,1.)))
REPRESENTATION_ITEM('')
SURFACE()
);
#1045=(
BOUNDED_SURFACE()
B_SPLINE_SURFACE(5,1,((#196747,#196748),(#196749,#196750),(#196751,#196752),
(#196753,#196754),(#196755,#196756),(#196757,#196758),(#196759,#196760),
(#196761,#196762),(#196763,#196764),(#196765,#196766),(#196767,#196768),
(#196769,#196770),(#196771,#196772),(#196773,#196774),(#196775,#196776),
(#196777,#196778),(#196779,#196780),(#196781,#196782),(#196783,#196784),
(#196785,#196786),(#196787,#196788),(#196789,#196790),(#196791,#196792),
(#196793,#196794),(#196795,#196796),(#196797,#196798),(#196799,#196800),
(#196801,#196802),(#196803,#196804),(#196805,#196806),(#196807,#196808),
(#196809,#196810),(#196811,#196812),(#196813,#196814),(#196815,#196816),
(#196817,#196818),(#196819,#196820),(#196821,#196822),(#196823,#196824),
(#196825,#196826),(#196827,#196828),(#196829,#196830),(#196831,#196832),
(#196833,#196834),(#196835,#196836),(#196837,#196838),(#196839,#196840),
(#196841,#196842),(#196843,#196844),(#196845,#196846),(#196847,#196848),
(#196849,#196850),(#196851,#196852),(#196853,#196854),(#196855,#196856),
(#196857,#196858),(#196859,#196860),(#196861,#196862),(#196863,#196864),
(#196865,#196866),(#196867,#196868),(#196869,#196870),(#196871,#196872),
(#196873,#196874),(#196875,#196876),(#196877,#196878),(#196879,#196880),
(#196881,#196882),(#196883,#196884),(#196885,#196886),(#196887,#196888),
(#196889,#196890),(#196891,#196892),(#196893,#196894),(#196895,#196896),
(#196897,#196898),(#196899,#196900),(#196901,#196902),(#196903,#196904),
(#196905,#196906),(#196907,#196908),(#196909,#196910),(#196911,#196912),
(#196913,#196914),(#196915,#196916),(#196917,#196918),(#196919,#196920),
(#196921,#196922),(#196923,#196924),(#196925,#196926),(#196927,#196928),
(#196929,#196930),(#196931,#196932),(#196933,#196934),(#196935,#196936),
(#196937,#196938),(#196939,#196940),(#196941,#196942),(#196943,#196944),
(#196945,#196946),(#196947,#196948),(#196949,#196950),(#196951,#196952),
(#196953,#196954),(#196955,#196956),(#196957,#196958),(#196959,#196960),
(#196961,#196962),(#196963,#196964),(#196965,#196966),(#196967,#196968),
(#196969,#196970),(#196971,#196972),(#196973,#196974),(#196975,#196976),
(#196977,#196978),(#196979,#196980),(#196981,#196982),(#196983,#196984),
(#196985,#196986),(#196987,#196988),(#196989,#196990),(#196991,#196992),
(#196993,#196994),(#196995,#196996),(#196997,#196998),(#196999,#197000),
(#197001,#197002),(#197003,#197004),(#197005,#197006),(#197007,#197008),
(#197009,#197010),(#197011,#197012),(#197013,#197014),(#197015,#197016),
(#197017,#197018),(#197019,#197020),(#197021,#197022),(#197023,#197024),
(#197025,#197026),(#197027,#197028),(#197029,#197030),(#197031,#197032),
(#197033,#197034),(#197035,#197036),(#197037,#197038),(#197039,#197040),
(#197041,#197042),(#197043,#197044),(#197045,#197046),(#197047,#197048),
(#197049,#197050),(#197051,#197052),(#197053,#197054),(#197055,#197056),
(#197057,#197058),(#197059,#197060),(#197061,#197062),(#197063,#197064),
(#197065,#197066),(#197067,#197068),(#197069,#197070),(#197071,#197072),
(#197073,#197074),(#197075,#197076),(#197077,#197078),(#197079,#197080),
(#197081,#197082),(#197083,#197084),(#197085,#197086),(#197087,#197088),
(#197089,#197090),(#197091,#197092),(#197093,#197094),(#197095,#197096),
(#197097,#197098),(#197099,#197100),(#197101,#197102),(#197103,#197104),
(#197105,#197106),(#197107,#197108),(#197109,#197110),(#197111,#197112),
(#197113,#197114),(#197115,#197116),(#197117,#197118),(#197119,#197120),
(#197121,#197122),(#197123,#197124),(#197125,#197126),(#197127,#197128),
(#197129,#197130),(#197131,#197132),(#197133,#197134),(#197135,#197136),
(#197137,#197138),(#197139,#197140),(#197141,#197142),(#197143,#197144),
(#197145,#197146),(#197147,#197148),(#197149,#197150),(#197151,#197152),
(#197153,#197154),(#197155,#197156)),.UNSPECIFIED.,.F.,.F.,.F.)
B_SPLINE_SURFACE_WITH_KNOTS((6,1,1,1,1,1,1,1,1,1,1,1,1,1,1,1,1,1,1,1,1,
1,1,1,1,1,1,1,1,1,1,1,1,1,1,1,1,1,1,1,1,1,1,1,1,1,1,1,1,1,1,1,1,1,1,1,1,
1,1,1,1,1,1,1,1,1,1,1,1,1,1,1,1,1,1,1,1,1,1,1,1,1,1,1,1,1,1,1,1,1,1,1,1,
1,1,1,1,1,1,1,1,1,1,1,1,1,1,1,1,1,1,1,1,1,1,1,1,1,1,1,1,1,1,1,1,1,1,1,1,
1,1,1,1,1,1,1,1,1,1,1,1,1,1,1,1,1,1,1,1,1,1,1,1,1,1,1,1,1,1,1,1,1,1,1,1,
1,1,1,1,1,1,1,1,1,1,1,1,1,1,1,1,1,1,1,1,1,1,1,1,1,1,1,1,1,1,1,1,1,1,1,6),
(2,2),(-1.,-0.995000000000001,-0.990000000000001,-0.985000000000001,-0.980000000000001,
-0.975000000000001,-0.970000000000001,-0.965000000000001,-0.960000000000001,
-0.955000000000001,-0.950000000000001,-0.945000000000001,-0.940000000000001,
-0.935000000000001,-0.930000000000001,-0.925000000000001,-0.920000000000001,
-0.915000000000001,-0.910000000000001,-0.905000000000001,-0.900000000000001,
-0.895000000000001,-0.890000000000001,-0.885000000000001,-0.880000000000001,
-0.875000000000001,-0.870000000000001,-0.865000000000001,-0.860000000000001,
-0.855000000000001,-0.850000000000001,-0.845000000000001,-0.840000000000001,
-0.835000000000001,-0.830000000000001,-0.825000000000001,-0.820000000000001,
-0.815000000000001,-0.810000000000001,-0.805000000000001,-0.800000000000001,
-0.795000000000001,-0.790000000000001,-0.785000000000001,-0.780000000000001,
-0.775000000000001,-0.770000000000001,-0.765000000000001,-0.760000000000001,
-0.755000000000001,-0.750000000000001,-0.745000000000001,-0.740000000000001,
-0.735000000000001,-0.730000000000001,-0.725000000000001,-0.720000000000001,
-0.715000000000001,-0.710000000000001,-0.705000000000001,-0.700000000000001,
-0.695000000000001,-0.690000000000001,-0.685,-0.68,-0.675,-0.67,-0.665,
-0.66,-0.655,-0.65,-0.645,-0.64,-0.635,-0.63,-0.625,-0.62,-0.615,-0.61,
-0.605,-0.6,-0.595,-0.59,-0.585,-0.58,-0.575,-0.57,-0.565,-0.56,-0.555,
-0.55,-0.545,-0.54,-0.535,-0.53,-0.525,-0.52,-0.515,-0.51,-0.505,-0.5,-0.495,
-0.49,-0.485,-0.48,-0.475,-0.47,-0.465,-0.46,-0.455,-0.45,-0.445,-0.44,
-0.435,-0.43,-0.425,-0.42,-0.415,-0.41,-0.405,-0.4,-0.395,-0.39,-0.385,
-0.38,-0.375,-0.37,-0.365,-0.36,-0.355,-0.35,-0.345,-0.34,-0.335,-0.33,
-0.325,-0.32,-0.315,-0.31,-0.305,-0.3,-0.295,-0.29,-0.285,-0.28,-0.275,
-0.27,-0.265,-0.26,-0.255,-0.25,-0.245,-0.24,-0.235,-0.23,-0.225,-0.22,
-0.215,-0.21,-0.205,-0.2,-0.195,-0.19,-0.185,-0.18,-0.175,-0.17,-0.165,
-0.16,-0.155,-0.15,-0.145,-0.14,-0.135,-0.13,-0.125,-0.12,-0.115,-0.11,
-0.105,-0.1,-0.095,-0.09,-0.085,-0.08,-0.075,-0.07,-0.065,-0.06,-0.055,
-0.05,-0.045,-0.04,-0.035,-0.03,-0.025,-0.02,-0.015,-0.01,-0.005,0.),(0.,
1.2),.UNSPECIFIED.)
GEOMETRIC_REPRESENTATION_ITEM()
RATIONAL_B_SPLINE_SURFACE(((1.,1.),(1.,1.),(1.,1.),(1.,1.),(1.,1.),(1.,
1.),(1.,1.),(1.,1.),(1.,1.),(1.,1.),(1.,1.),(1.,1.),(1.,1.),(1.,1.),(1.,
1.),(1.,1.),(1.,1.),(1.,1.),(1.,1.),(1.,1.),(1.,1.),(1.,1.),(1.,1.),(1.,
1.),(1.,1.),(1.,1.),(1.,1.),(1.,1.),(1.,1.),(1.,1.),(1.,1.),(1.,1.),(1.,
1.),(1.,1.),(1.,1.),(1.,1.),(1.,1.),(1.,1.),(1.,1.),(1.,1.),(1.,1.),(1.,
1.),(1.,1.),(1.,1.),(1.,1.),(1.,1.),(1.,1.),(1.,1.),(1.,1.),(1.,1.),(1.,
1.),(1.,1.),(1.,1.),(1.,1.),(1.,1.),(1.,1.),(1.,1.),(1.,1.),(1.,1.),(1.,
1.),(1.,1.),(1.,1.),(1.,1.),(1.,1.),(1.,1.),(1.,1.),(1.,1.),(1.,1.),(1.,
1.),(1.,1.),(1.,1.),(1.,1.),(1.,1.),(1.,1.),(1.,1.),(1.,1.),(1.,1.),(1.,
1.),(1.,1.),(1.,1.),(1.,1.),(1.,1.),(1.,1.),(1.,1.),(1.,1.),(1.,1.),(1.,
1.),(1.,1.),(1.,1.),(1.,1.),(1.,1.),(1.,1.),(1.,1.),(1.,1.),(1.,1.),(1.,
1.),(1.,1.),(1.,1.),(1.,1.),(1.,1.),(1.,1.),(1.,1.),(1.,1.),(1.,1.),(1.,
1.),(1.,1.),(1.,1.),(1.,1.),(1.,1.),(1.,1.),(1.,1.),(1.,1.),(1.,1.),(1.,
1.),(1.,1.),(1.,1.),(1.,1.),(1.,1.),(1.,1.),(1.,1.),(1.,1.),(1.,1.),(1.,
1.),(1.,1.),(1.,1.),(1.,1.),(1.,1.),(1.,1.),(1.,1.),(1.,1.),(1.,1.),(1.,
1.),(1.,1.),(1.,1.),(1.,1.),(1.,1.),(1.,1.),(1.,1.),(1.,1.),(1.,1.),(1.,
1.),(1.,1.),(1.,1.),(1.,1.),(1.,1.),(1.,1.),(1.,1.),(1.,1.),(1.,1.),(1.,
1.),(1.,1.),(1.,1.),(1.,1.),(1.,1.),(1.,1.),(1.,1.),(1.,1.),(1.,1.),(1.,
1.),(1.,1.),(1.,1.),(1.,1.),(1.,1.),(1.,1.),(1.,1.),(1.,1.),(1.,1.),(1.,
1.),(1.,1.),(1.,1.),(1.,1.),(1.,1.),(1.,1.),(1.,1.),(1.,1.),(1.,1.),(1.,
1.),(1.,1.),(1.,1.),(1.,1.),(1.,1.),(1.,1.),(1.,1.),(1.,1.),(1.,1.),(1.,
1.),(1.,1.),(1.,1.),(1.,1.),(1.,1.),(1.,1.),(1.,1.),(1.,1.),(1.,1.),(1.,
1.),(1.,1.),(1.,1.),(1.,1.),(1.,1.),(1.,1.),(1.,1.),(1.,1.),(1.,1.),(1.,
1.),(1.,1.)))
REPRESENTATION_ITEM('')
SURFACE()
);
#1046=(
BOUNDED_SURFACE()
B_SPLINE_SURFACE(5,1,((#197364,#197365),(#197366,#197367),(#197368,#197369),
(#197370,#197371),(#197372,#197373),(#197374,#197375),(#197376,#197377),
(#197378,#197379),(#197380,#197381),(#197382,#197383),(#197384,#197385),
(#197386,#197387),(#197388,#197389),(#197390,#197391),(#197392,#197393),
(#197394,#197395),(#197396,#197397),(#197398,#197399),(#197400,#197401),
(#197402,#197403),(#197404,#197405),(#197406,#197407),(#197408,#197409),
(#197410,#197411),(#197412,#197413),(#197414,#197415),(#197416,#197417),
(#197418,#197419),(#197420,#197421),(#197422,#197423),(#197424,#197425),
(#197426,#197427),(#197428,#197429),(#197430,#197431),(#197432,#197433),
(#197434,#197435),(#197436,#197437),(#197438,#197439),(#197440,#197441),
(#197442,#197443),(#197444,#197445),(#197446,#197447),(#197448,#197449),
(#197450,#197451),(#197452,#197453),(#197454,#197455),(#197456,#197457),
(#197458,#197459),(#197460,#197461),(#197462,#197463),(#197464,#197465),
(#197466,#197467),(#197468,#197469),(#197470,#197471),(#197472,#197473),
(#197474,#197475),(#197476,#197477),(#197478,#197479),(#197480,#197481),
(#197482,#197483),(#197484,#197485),(#197486,#197487),(#197488,#197489),
(#197490,#197491),(#197492,#197493),(#197494,#197495),(#197496,#197497),
(#197498,#197499),(#197500,#197501),(#197502,#197503),(#197504,#197505),
(#197506,#197507),(#197508,#197509),(#197510,#197511),(#197512,#197513),
(#197514,#197515),(#197516,#197517),(#197518,#197519),(#197520,#197521),
(#197522,#197523),(#197524,#197525),(#197526,#197527),(#197528,#197529),
(#197530,#197531),(#197532,#197533),(#197534,#197535),(#197536,#197537),
(#197538,#197539),(#197540,#197541),(#197542,#197543),(#197544,#197545),
(#197546,#197547),(#197548,#197549),(#197550,#197551),(#197552,#197553),
(#197554,#197555),(#197556,#197557),(#197558,#197559),(#197560,#197561),
(#197562,#197563),(#197564,#197565),(#197566,#197567),(#197568,#197569),
(#197570,#197571),(#197572,#197573),(#197574,#197575),(#197576,#197577),
(#197578,#197579),(#197580,#197581),(#197582,#197583),(#197584,#197585),
(#197586,#197587),(#197588,#197589),(#197590,#197591),(#197592,#197593),
(#197594,#197595),(#197596,#197597),(#197598,#197599),(#197600,#197601),
(#197602,#197603),(#197604,#197605),(#197606,#197607),(#197608,#197609),
(#197610,#197611),(#197612,#197613),(#197614,#197615),(#197616,#197617),
(#197618,#197619),(#197620,#197621),(#197622,#197623),(#197624,#197625),
(#197626,#197627),(#197628,#197629),(#197630,#197631),(#197632,#197633),
(#197634,#197635),(#197636,#197637),(#197638,#197639),(#197640,#197641),
(#197642,#197643),(#197644,#197645),(#197646,#197647),(#197648,#197649),
(#197650,#197651),(#197652,#197653),(#197654,#197655),(#197656,#197657),
(#197658,#197659),(#197660,#197661),(#197662,#197663),(#197664,#197665),
(#197666,#197667),(#197668,#197669),(#197670,#197671),(#197672,#197673),
(#197674,#197675),(#197676,#197677),(#197678,#197679),(#197680,#197681),
(#197682,#197683),(#197684,#197685),(#197686,#197687),(#197688,#197689),
(#197690,#197691),(#197692,#197693),(#197694,#197695),(#197696,#197697),
(#197698,#197699),(#197700,#197701),(#197702,#197703),(#197704,#197705),
(#197706,#197707),(#197708,#197709),(#197710,#197711),(#197712,#197713),
(#197714,#197715),(#197716,#197717),(#197718,#197719),(#197720,#197721),
(#197722,#197723),(#197724,#197725),(#197726,#197727),(#197728,#197729),
(#197730,#197731),(#197732,#197733),(#197734,#197735),(#197736,#197737),
(#197738,#197739),(#197740,#197741),(#197742,#197743),(#197744,#197745),
(#197746,#197747),(#197748,#197749),(#197750,#197751),(#197752,#197753),
(#197754,#197755),(#197756,#197757),(#197758,#197759),(#197760,#197761),
(#197762,#197763),(#197764,#197765),(#197766,#197767),(#197768,#197769),
(#197770,#197771),(#197772,#197773)),.UNSPECIFIED.,.F.,.F.,.F.)
B_SPLINE_SURFACE_WITH_KNOTS((6,1,1,1,1,1,1,1,1,1,1,1,1,1,1,1,1,1,1,1,1,
1,1,1,1,1,1,1,1,1,1,1,1,1,1,1,1,1,1,1,1,1,1,1,1,1,1,1,1,1,1,1,1,1,1,1,1,
1,1,1,1,1,1,1,1,1,1,1,1,1,1,1,1,1,1,1,1,1,1,1,1,1,1,1,1,1,1,1,1,1,1,1,1,
1,1,1,1,1,1,1,1,1,1,1,1,1,1,1,1,1,1,1,1,1,1,1,1,1,1,1,1,1,1,1,1,1,1,1,1,
1,1,1,1,1,1,1,1,1,1,1,1,1,1,1,1,1,1,1,1,1,1,1,1,1,1,1,1,1,1,1,1,1,1,1,1,
1,1,1,1,1,1,1,1,1,1,1,1,1,1,1,1,1,1,1,1,1,1,1,1,1,1,1,1,1,1,1,1,1,1,1,6),
(2,2),(0.,0.005,0.01,0.015,0.02,0.025,0.03,0.035,0.04,0.045,0.05,0.055,
0.06,0.065,0.07,0.075,0.08,0.085,0.09,0.095,0.1,0.105,0.11,0.115,0.12,0.125,
0.13,0.135,0.14,0.145,0.15,0.155,0.16,0.165,0.17,0.175,0.18,0.185,0.19,
0.195,0.2,0.205,0.21,0.215,0.22,0.225,0.23,0.235,0.24,0.245,0.25,0.255,
0.26,0.265,0.27,0.275,0.28,0.285,0.29,0.295,0.3,0.305,0.31,0.315,0.32,0.325,
0.33,0.335,0.34,0.345,0.35,0.355,0.36,0.365,0.37,0.375,0.38,0.385,0.39,
0.395,0.4,0.405,0.41,0.415,0.42,0.425,0.43,0.435,0.44,0.445,0.45,0.455,
0.46,0.465,0.47,0.475,0.48,0.485,0.49,0.495,0.5,0.505,0.51,0.515,0.52,0.525,
0.53,0.535,0.54,0.545,0.55,0.555,0.56,0.565,0.57,0.575,0.58,0.585,0.59,
0.595,0.6,0.605,0.61,0.615,0.62,0.625,0.63,0.635,0.64,0.645,0.65,0.655,
0.66,0.665,0.67,0.675,0.68,0.685,0.690000000000001,0.695000000000001,0.700000000000001,
0.705000000000001,0.710000000000001,0.715000000000001,0.720000000000001,
0.725000000000001,0.730000000000001,0.735000000000001,0.740000000000001,
0.745000000000001,0.750000000000001,0.755000000000001,0.760000000000001,
0.765000000000001,0.770000000000001,0.775000000000001,0.780000000000001,
0.785000000000001,0.790000000000001,0.795000000000001,0.800000000000001,
0.805000000000001,0.810000000000001,0.815000000000001,0.820000000000001,
0.825000000000001,0.830000000000001,0.835000000000001,0.840000000000001,
0.845000000000001,0.850000000000001,0.855000000000001,0.860000000000001,
0.865000000000001,0.870000000000001,0.875000000000001,0.880000000000001,
0.885000000000001,0.890000000000001,0.895000000000001,0.900000000000001,
0.905000000000001,0.910000000000001,0.915000000000001,0.920000000000001,
0.925000000000001,0.930000000000001,0.935000000000001,0.940000000000001,
0.945000000000001,0.950000000000001,0.955000000000001,0.960000000000001,
0.965000000000001,0.970000000000001,0.975000000000001,0.980000000000001,
0.985000000000001,0.990000000000001,0.995000000000001,1.),(0.,1.2),
 .UNSPECIFIED.)
GEOMETRIC_REPRESENTATION_ITEM()
RATIONAL_B_SPLINE_SURFACE(((1.,1.),(1.,1.),(1.,1.),(1.,1.),(1.,1.),(1.,
1.),(1.,1.),(1.,1.),(1.,1.),(1.,1.),(1.,1.),(1.,1.),(1.,1.),(1.,1.),(1.,
1.),(1.,1.),(1.,1.),(1.,1.),(1.,1.),(1.,1.),(1.,1.),(1.,1.),(1.,1.),(1.,
1.),(1.,1.),(1.,1.),(1.,1.),(1.,1.),(1.,1.),(1.,1.),(1.,1.),(1.,1.),(1.,
1.),(1.,1.),(1.,1.),(1.,1.),(1.,1.),(1.,1.),(1.,1.),(1.,1.),(1.,1.),(1.,
1.),(1.,1.),(1.,1.),(1.,1.),(1.,1.),(1.,1.),(1.,1.),(1.,1.),(1.,1.),(1.,
1.),(1.,1.),(1.,1.),(1.,1.),(1.,1.),(1.,1.),(1.,1.),(1.,1.),(1.,1.),(1.,
1.),(1.,1.),(1.,1.),(1.,1.),(1.,1.),(1.,1.),(1.,1.),(1.,1.),(1.,1.),(1.,
1.),(1.,1.),(1.,1.),(1.,1.),(1.,1.),(1.,1.),(1.,1.),(1.,1.),(1.,1.),(1.,
1.),(1.,1.),(1.,1.),(1.,1.),(1.,1.),(1.,1.),(1.,1.),(1.,1.),(1.,1.),(1.,
1.),(1.,1.),(1.,1.),(1.,1.),(1.,1.),(1.,1.),(1.,1.),(1.,1.),(1.,1.),(1.,
1.),(1.,1.),(1.,1.),(1.,1.),(1.,1.),(1.,1.),(1.,1.),(1.,1.),(1.,1.),(1.,
1.),(1.,1.),(1.,1.),(1.,1.),(1.,1.),(1.,1.),(1.,1.),(1.,1.),(1.,1.),(1.,
1.),(1.,1.),(1.,1.),(1.,1.),(1.,1.),(1.,1.),(1.,1.),(1.,1.),(1.,1.),(1.,
1.),(1.,1.),(1.,1.),(1.,1.),(1.,1.),(1.,1.),(1.,1.),(1.,1.),(1.,1.),(1.,
1.),(1.,1.),(1.,1.),(1.,1.),(1.,1.),(1.,1.),(1.,1.),(1.,1.),(1.,1.),(1.,
1.),(1.,1.),(1.,1.),(1.,1.),(1.,1.),(1.,1.),(1.,1.),(1.,1.),(1.,1.),(1.,
1.),(1.,1.),(1.,1.),(1.,1.),(1.,1.),(1.,1.),(1.,1.),(1.,1.),(1.,1.),(1.,
1.),(1.,1.),(1.,1.),(1.,1.),(1.,1.),(1.,1.),(1.,1.),(1.,1.),(1.,1.),(1.,
1.),(1.,1.),(1.,1.),(1.,1.),(1.,1.),(1.,1.),(1.,1.),(1.,1.),(1.,1.),(1.,
1.),(1.,1.),(1.,1.),(1.,1.),(1.,1.),(1.,1.),(1.,1.),(1.,1.),(1.,1.),(1.,
1.),(1.,1.),(1.,1.),(1.,1.),(1.,1.),(1.,1.),(1.,1.),(1.,1.),(1.,1.),(1.,
1.),(1.,1.),(1.,1.),(1.,1.),(1.,1.),(1.,1.),(1.,1.),(1.,1.),(1.,1.),(1.,
1.),(1.,1.)))
REPRESENTATION_ITEM('')
SURFACE()
);
#1047=(
BOUNDED_SURFACE()
B_SPLINE_SURFACE(5,1,((#197985,#197986),(#197987,#197988),(#197989,#197990),
(#197991,#197992),(#197993,#197994),(#197995,#197996),(#197997,#197998),
(#197999,#198000),(#198001,#198002),(#198003,#198004),(#198005,#198006),
(#198007,#198008),(#198009,#198010),(#198011,#198012),(#198013,#198014),
(#198015,#198016),(#198017,#198018),(#198019,#198020),(#198021,#198022),
(#198023,#198024),(#198025,#198026),(#198027,#198028),(#198029,#198030),
(#198031,#198032),(#198033,#198034),(#198035,#198036),(#198037,#198038),
(#198039,#198040),(#198041,#198042),(#198043,#198044),(#198045,#198046),
(#198047,#198048),(#198049,#198050),(#198051,#198052),(#198053,#198054),
(#198055,#198056),(#198057,#198058),(#198059,#198060),(#198061,#198062),
(#198063,#198064),(#198065,#198066),(#198067,#198068),(#198069,#198070),
(#198071,#198072),(#198073,#198074),(#198075,#198076),(#198077,#198078),
(#198079,#198080),(#198081,#198082),(#198083,#198084),(#198085,#198086),
(#198087,#198088),(#198089,#198090),(#198091,#198092),(#198093,#198094),
(#198095,#198096),(#198097,#198098),(#198099,#198100),(#198101,#198102),
(#198103,#198104),(#198105,#198106),(#198107,#198108),(#198109,#198110),
(#198111,#198112),(#198113,#198114),(#198115,#198116),(#198117,#198118),
(#198119,#198120),(#198121,#198122),(#198123,#198124),(#198125,#198126),
(#198127,#198128),(#198129,#198130),(#198131,#198132),(#198133,#198134),
(#198135,#198136),(#198137,#198138),(#198139,#198140),(#198141,#198142),
(#198143,#198144),(#198145,#198146),(#198147,#198148),(#198149,#198150),
(#198151,#198152),(#198153,#198154),(#198155,#198156),(#198157,#198158),
(#198159,#198160),(#198161,#198162),(#198163,#198164),(#198165,#198166),
(#198167,#198168),(#198169,#198170),(#198171,#198172),(#198173,#198174),
(#198175,#198176),(#198177,#198178),(#198179,#198180),(#198181,#198182),
(#198183,#198184),(#198185,#198186),(#198187,#198188),(#198189,#198190),
(#198191,#198192),(#198193,#198194),(#198195,#198196),(#198197,#198198),
(#198199,#198200),(#198201,#198202),(#198203,#198204),(#198205,#198206),
(#198207,#198208),(#198209,#198210),(#198211,#198212),(#198213,#198214),
(#198215,#198216),(#198217,#198218),(#198219,#198220),(#198221,#198222),
(#198223,#198224),(#198225,#198226),(#198227,#198228),(#198229,#198230),
(#198231,#198232),(#198233,#198234),(#198235,#198236),(#198237,#198238),
(#198239,#198240),(#198241,#198242),(#198243,#198244),(#198245,#198246),
(#198247,#198248),(#198249,#198250),(#198251,#198252),(#198253,#198254),
(#198255,#198256),(#198257,#198258),(#198259,#198260),(#198261,#198262),
(#198263,#198264),(#198265,#198266),(#198267,#198268),(#198269,#198270),
(#198271,#198272),(#198273,#198274),(#198275,#198276),(#198277,#198278),
(#198279,#198280),(#198281,#198282),(#198283,#198284),(#198285,#198286),
(#198287,#198288),(#198289,#198290),(#198291,#198292),(#198293,#198294),
(#198295,#198296),(#198297,#198298),(#198299,#198300),(#198301,#198302),
(#198303,#198304),(#198305,#198306),(#198307,#198308),(#198309,#198310),
(#198311,#198312),(#198313,#198314),(#198315,#198316),(#198317,#198318),
(#198319,#198320),(#198321,#198322),(#198323,#198324),(#198325,#198326),
(#198327,#198328),(#198329,#198330),(#198331,#198332),(#198333,#198334),
(#198335,#198336),(#198337,#198338),(#198339,#198340),(#198341,#198342),
(#198343,#198344),(#198345,#198346),(#198347,#198348),(#198349,#198350),
(#198351,#198352),(#198353,#198354),(#198355,#198356),(#198357,#198358),
(#198359,#198360),(#198361,#198362),(#198363,#198364),(#198365,#198366),
(#198367,#198368),(#198369,#198370),(#198371,#198372),(#198373,#198374),
(#198375,#198376),(#198377,#198378),(#198379,#198380),(#198381,#198382),
(#198383,#198384),(#198385,#198386),(#198387,#198388),(#198389,#198390),
(#198391,#198392),(#198393,#198394)),.UNSPECIFIED.,.F.,.F.,.F.)
B_SPLINE_SURFACE_WITH_KNOTS((6,1,1,1,1,1,1,1,1,1,1,1,1,1,1,1,1,1,1,1,1,
1,1,1,1,1,1,1,1,1,1,1,1,1,1,1,1,1,1,1,1,1,1,1,1,1,1,1,1,1,1,1,1,1,1,1,1,
1,1,1,1,1,1,1,1,1,1,1,1,1,1,1,1,1,1,1,1,1,1,1,1,1,1,1,1,1,1,1,1,1,1,1,1,
1,1,1,1,1,1,1,1,1,1,1,1,1,1,1,1,1,1,1,1,1,1,1,1,1,1,1,1,1,1,1,1,1,1,1,1,
1,1,1,1,1,1,1,1,1,1,1,1,1,1,1,1,1,1,1,1,1,1,1,1,1,1,1,1,1,1,1,1,1,1,1,1,
1,1,1,1,1,1,1,1,1,1,1,1,1,1,1,1,1,1,1,1,1,1,1,1,1,1,1,1,1,1,1,1,1,1,1,6),
(2,2),(-1.,-0.995000000000001,-0.990000000000001,-0.985000000000001,-0.980000000000001,
-0.975000000000001,-0.970000000000001,-0.965000000000001,-0.960000000000001,
-0.955000000000001,-0.950000000000001,-0.945000000000001,-0.940000000000001,
-0.935000000000001,-0.930000000000001,-0.925000000000001,-0.920000000000001,
-0.915000000000001,-0.910000000000001,-0.905000000000001,-0.900000000000001,
-0.895000000000001,-0.890000000000001,-0.885000000000001,-0.880000000000001,
-0.875000000000001,-0.870000000000001,-0.865000000000001,-0.860000000000001,
-0.855000000000001,-0.850000000000001,-0.845000000000001,-0.840000000000001,
-0.835000000000001,-0.830000000000001,-0.825000000000001,-0.820000000000001,
-0.815000000000001,-0.810000000000001,-0.805000000000001,-0.800000000000001,
-0.795000000000001,-0.790000000000001,-0.785000000000001,-0.780000000000001,
-0.775000000000001,-0.770000000000001,-0.765000000000001,-0.760000000000001,
-0.755000000000001,-0.750000000000001,-0.745000000000001,-0.740000000000001,
-0.735000000000001,-0.730000000000001,-0.725000000000001,-0.720000000000001,
-0.715000000000001,-0.710000000000001,-0.705000000000001,-0.700000000000001,
-0.695000000000001,-0.690000000000001,-0.685,-0.68,-0.675,-0.67,-0.665,
-0.66,-0.655,-0.65,-0.645,-0.64,-0.635,-0.63,-0.625,-0.62,-0.615,-0.61,
-0.605,-0.6,-0.595,-0.59,-0.585,-0.58,-0.575,-0.57,-0.565,-0.56,-0.555,
-0.55,-0.545,-0.54,-0.535,-0.53,-0.525,-0.52,-0.515,-0.51,-0.505,-0.5,-0.495,
-0.49,-0.485,-0.48,-0.475,-0.47,-0.465,-0.46,-0.455,-0.45,-0.445,-0.44,
-0.435,-0.43,-0.425,-0.42,-0.415,-0.41,-0.405,-0.4,-0.395,-0.39,-0.385,
-0.38,-0.375,-0.37,-0.365,-0.36,-0.355,-0.35,-0.345,-0.34,-0.335,-0.33,
-0.325,-0.32,-0.315,-0.31,-0.305,-0.3,-0.295,-0.29,-0.285,-0.28,-0.275,
-0.27,-0.265,-0.26,-0.255,-0.25,-0.245,-0.24,-0.235,-0.23,-0.225,-0.22,
-0.215,-0.21,-0.205,-0.2,-0.195,-0.19,-0.185,-0.18,-0.175,-0.17,-0.165,
-0.16,-0.155,-0.15,-0.145,-0.14,-0.135,-0.13,-0.125,-0.12,-0.115,-0.11,
-0.105,-0.1,-0.095,-0.09,-0.085,-0.08,-0.075,-0.07,-0.065,-0.06,-0.055,
-0.05,-0.045,-0.04,-0.035,-0.03,-0.025,-0.02,-0.015,-0.01,-0.005,0.),(0.,
1.2),.UNSPECIFIED.)
GEOMETRIC_REPRESENTATION_ITEM()
RATIONAL_B_SPLINE_SURFACE(((1.,1.),(1.,1.),(1.,1.),(1.,1.),(1.,1.),(1.,
1.),(1.,1.),(1.,1.),(1.,1.),(1.,1.),(1.,1.),(1.,1.),(1.,1.),(1.,1.),(1.,
1.),(1.,1.),(1.,1.),(1.,1.),(1.,1.),(1.,1.),(1.,1.),(1.,1.),(1.,1.),(1.,
1.),(1.,1.),(1.,1.),(1.,1.),(1.,1.),(1.,1.),(1.,1.),(1.,1.),(1.,1.),(1.,
1.),(1.,1.),(1.,1.),(1.,1.),(1.,1.),(1.,1.),(1.,1.),(1.,1.),(1.,1.),(1.,
1.),(1.,1.),(1.,1.),(1.,1.),(1.,1.),(1.,1.),(1.,1.),(1.,1.),(1.,1.),(1.,
1.),(1.,1.),(1.,1.),(1.,1.),(1.,1.),(1.,1.),(1.,1.),(1.,1.),(1.,1.),(1.,
1.),(1.,1.),(1.,1.),(1.,1.),(1.,1.),(1.,1.),(1.,1.),(1.,1.),(1.,1.),(1.,
1.),(1.,1.),(1.,1.),(1.,1.),(1.,1.),(1.,1.),(1.,1.),(1.,1.),(1.,1.),(1.,
1.),(1.,1.),(1.,1.),(1.,1.),(1.,1.),(1.,1.),(1.,1.),(1.,1.),(1.,1.),(1.,
1.),(1.,1.),(1.,1.),(1.,1.),(1.,1.),(1.,1.),(1.,1.),(1.,1.),(1.,1.),(1.,
1.),(1.,1.),(1.,1.),(1.,1.),(1.,1.),(1.,1.),(1.,1.),(1.,1.),(1.,1.),(1.,
1.),(1.,1.),(1.,1.),(1.,1.),(1.,1.),(1.,1.),(1.,1.),(1.,1.),(1.,1.),(1.,
1.),(1.,1.),(1.,1.),(1.,1.),(1.,1.),(1.,1.),(1.,1.),(1.,1.),(1.,1.),(1.,
1.),(1.,1.),(1.,1.),(1.,1.),(1.,1.),(1.,1.),(1.,1.),(1.,1.),(1.,1.),(1.,
1.),(1.,1.),(1.,1.),(1.,1.),(1.,1.),(1.,1.),(1.,1.),(1.,1.),(1.,1.),(1.,
1.),(1.,1.),(1.,1.),(1.,1.),(1.,1.),(1.,1.),(1.,1.),(1.,1.),(1.,1.),(1.,
1.),(1.,1.),(1.,1.),(1.,1.),(1.,1.),(1.,1.),(1.,1.),(1.,1.),(1.,1.),(1.,
1.),(1.,1.),(1.,1.),(1.,1.),(1.,1.),(1.,1.),(1.,1.),(1.,1.),(1.,1.),(1.,
1.),(1.,1.),(1.,1.),(1.,1.),(1.,1.),(1.,1.),(1.,1.),(1.,1.),(1.,1.),(1.,
1.),(1.,1.),(1.,1.),(1.,1.),(1.,1.),(1.,1.),(1.,1.),(1.,1.),(1.,1.),(1.,
1.),(1.,1.),(1.,1.),(1.,1.),(1.,1.),(1.,1.),(1.,1.),(1.,1.),(1.,1.),(1.,
1.),(1.,1.),(1.,1.),(1.,1.),(1.,1.),(1.,1.),(1.,1.),(1.,1.),(1.,1.),(1.,
1.),(1.,1.)))
REPRESENTATION_ITEM('')
SURFACE()
);
#1048=(
BOUNDED_SURFACE()
B_SPLINE_SURFACE(5,1,((#198602,#198603),(#198604,#198605),(#198606,#198607),
(#198608,#198609),(#198610,#198611),(#198612,#198613),(#198614,#198615),
(#198616,#198617),(#198618,#198619),(#198620,#198621),(#198622,#198623),
(#198624,#198625),(#198626,#198627),(#198628,#198629),(#198630,#198631),
(#198632,#198633),(#198634,#198635),(#198636,#198637),(#198638,#198639),
(#198640,#198641),(#198642,#198643),(#198644,#198645),(#198646,#198647),
(#198648,#198649),(#198650,#198651),(#198652,#198653),(#198654,#198655),
(#198656,#198657),(#198658,#198659),(#198660,#198661),(#198662,#198663),
(#198664,#198665),(#198666,#198667),(#198668,#198669),(#198670,#198671),
(#198672,#198673),(#198674,#198675),(#198676,#198677),(#198678,#198679),
(#198680,#198681),(#198682,#198683),(#198684,#198685),(#198686,#198687),
(#198688,#198689),(#198690,#198691),(#198692,#198693),(#198694,#198695),
(#198696,#198697),(#198698,#198699),(#198700,#198701),(#198702,#198703),
(#198704,#198705),(#198706,#198707),(#198708,#198709),(#198710,#198711),
(#198712,#198713),(#198714,#198715),(#198716,#198717),(#198718,#198719),
(#198720,#198721),(#198722,#198723),(#198724,#198725),(#198726,#198727),
(#198728,#198729),(#198730,#198731),(#198732,#198733),(#198734,#198735),
(#198736,#198737),(#198738,#198739),(#198740,#198741),(#198742,#198743),
(#198744,#198745),(#198746,#198747),(#198748,#198749),(#198750,#198751),
(#198752,#198753),(#198754,#198755),(#198756,#198757),(#198758,#198759),
(#198760,#198761),(#198762,#198763),(#198764,#198765),(#198766,#198767),
(#198768,#198769),(#198770,#198771),(#198772,#198773),(#198774,#198775),
(#198776,#198777),(#198778,#198779),(#198780,#198781),(#198782,#198783),
(#198784,#198785),(#198786,#198787),(#198788,#198789),(#198790,#198791),
(#198792,#198793),(#198794,#198795),(#198796,#198797),(#198798,#198799),
(#198800,#198801),(#198802,#198803),(#198804,#198805),(#198806,#198807),
(#198808,#198809),(#198810,#198811),(#198812,#198813),(#198814,#198815),
(#198816,#198817),(#198818,#198819),(#198820,#198821),(#198822,#198823),
(#198824,#198825),(#198826,#198827),(#198828,#198829),(#198830,#198831),
(#198832,#198833),(#198834,#198835),(#198836,#198837),(#198838,#198839),
(#198840,#198841),(#198842,#198843),(#198844,#198845),(#198846,#198847),
(#198848,#198849),(#198850,#198851),(#198852,#198853),(#198854,#198855),
(#198856,#198857),(#198858,#198859),(#198860,#198861),(#198862,#198863),
(#198864,#198865),(#198866,#198867),(#198868,#198869),(#198870,#198871),
(#198872,#198873),(#198874,#198875),(#198876,#198877),(#198878,#198879),
(#198880,#198881),(#198882,#198883),(#198884,#198885),(#198886,#198887),
(#198888,#198889),(#198890,#198891),(#198892,#198893),(#198894,#198895),
(#198896,#198897),(#198898,#198899),(#198900,#198901),(#198902,#198903),
(#198904,#198905),(#198906,#198907),(#198908,#198909),(#198910,#198911),
(#198912,#198913),(#198914,#198915),(#198916,#198917),(#198918,#198919),
(#198920,#198921),(#198922,#198923),(#198924,#198925),(#198926,#198927),
(#198928,#198929),(#198930,#198931),(#198932,#198933),(#198934,#198935),
(#198936,#198937),(#198938,#198939),(#198940,#198941),(#198942,#198943),
(#198944,#198945),(#198946,#198947),(#198948,#198949),(#198950,#198951),
(#198952,#198953),(#198954,#198955),(#198956,#198957),(#198958,#198959),
(#198960,#198961),(#198962,#198963),(#198964,#198965),(#198966,#198967),
(#198968,#198969),(#198970,#198971),(#198972,#198973),(#198974,#198975),
(#198976,#198977),(#198978,#198979),(#198980,#198981),(#198982,#198983),
(#198984,#198985),(#198986,#198987),(#198988,#198989),(#198990,#198991),
(#198992,#198993),(#198994,#198995),(#198996,#198997),(#198998,#198999),
(#199000,#199001),(#199002,#199003),(#199004,#199005),(#199006,#199007),
(#199008,#199009),(#199010,#199011)),.UNSPECIFIED.,.F.,.F.,.F.)
B_SPLINE_SURFACE_WITH_KNOTS((6,1,1,1,1,1,1,1,1,1,1,1,1,1,1,1,1,1,1,1,1,
1,1,1,1,1,1,1,1,1,1,1,1,1,1,1,1,1,1,1,1,1,1,1,1,1,1,1,1,1,1,1,1,1,1,1,1,
1,1,1,1,1,1,1,1,1,1,1,1,1,1,1,1,1,1,1,1,1,1,1,1,1,1,1,1,1,1,1,1,1,1,1,1,
1,1,1,1,1,1,1,1,1,1,1,1,1,1,1,1,1,1,1,1,1,1,1,1,1,1,1,1,1,1,1,1,1,1,1,1,
1,1,1,1,1,1,1,1,1,1,1,1,1,1,1,1,1,1,1,1,1,1,1,1,1,1,1,1,1,1,1,1,1,1,1,1,
1,1,1,1,1,1,1,1,1,1,1,1,1,1,1,1,1,1,1,1,1,1,1,1,1,1,1,1,1,1,1,1,1,1,1,6),
(2,2),(0.,0.005,0.01,0.015,0.02,0.025,0.03,0.035,0.04,0.045,0.05,0.055,
0.06,0.065,0.07,0.075,0.08,0.085,0.09,0.095,0.1,0.105,0.11,0.115,0.12,0.125,
0.13,0.135,0.14,0.145,0.15,0.155,0.16,0.165,0.17,0.175,0.18,0.185,0.19,
0.195,0.2,0.205,0.21,0.215,0.22,0.225,0.23,0.235,0.24,0.245,0.25,0.255,
0.26,0.265,0.27,0.275,0.28,0.285,0.29,0.295,0.3,0.305,0.31,0.315,0.32,0.325,
0.33,0.335,0.34,0.345,0.35,0.355,0.36,0.365,0.37,0.375,0.38,0.385,0.39,
0.395,0.4,0.405,0.41,0.415,0.42,0.425,0.43,0.435,0.44,0.445,0.45,0.455,
0.46,0.465,0.47,0.475,0.48,0.485,0.49,0.495,0.5,0.505,0.51,0.515,0.52,0.525,
0.53,0.535,0.54,0.545,0.55,0.555,0.56,0.565,0.57,0.575,0.58,0.585,0.59,
0.595,0.6,0.605,0.61,0.615,0.62,0.625,0.63,0.635,0.64,0.645,0.65,0.655,
0.66,0.665,0.67,0.675,0.68,0.685,0.690000000000001,0.695000000000001,0.700000000000001,
0.705000000000001,0.710000000000001,0.715000000000001,0.720000000000001,
0.725000000000001,0.730000000000001,0.735000000000001,0.740000000000001,
0.745000000000001,0.750000000000001,0.755000000000001,0.760000000000001,
0.765000000000001,0.770000000000001,0.775000000000001,0.780000000000001,
0.785000000000001,0.790000000000001,0.795000000000001,0.800000000000001,
0.805000000000001,0.810000000000001,0.815000000000001,0.820000000000001,
0.825000000000001,0.830000000000001,0.835000000000001,0.840000000000001,
0.845000000000001,0.850000000000001,0.855000000000001,0.860000000000001,
0.865000000000001,0.870000000000001,0.875000000000001,0.880000000000001,
0.885000000000001,0.890000000000001,0.895000000000001,0.900000000000001,
0.905000000000001,0.910000000000001,0.915000000000001,0.920000000000001,
0.925000000000001,0.930000000000001,0.935000000000001,0.940000000000001,
0.945000000000001,0.950000000000001,0.955000000000001,0.960000000000001,
0.965000000000001,0.970000000000001,0.975000000000001,0.980000000000001,
0.985000000000001,0.990000000000001,0.995000000000001,1.),(0.,1.2),
 .UNSPECIFIED.)
GEOMETRIC_REPRESENTATION_ITEM()
RATIONAL_B_SPLINE_SURFACE(((1.,1.),(1.,1.),(1.,1.),(1.,1.),(1.,1.),(1.,
1.),(1.,1.),(1.,1.),(1.,1.),(1.,1.),(1.,1.),(1.,1.),(1.,1.),(1.,1.),(1.,
1.),(1.,1.),(1.,1.),(1.,1.),(1.,1.),(1.,1.),(1.,1.),(1.,1.),(1.,1.),(1.,
1.),(1.,1.),(1.,1.),(1.,1.),(1.,1.),(1.,1.),(1.,1.),(1.,1.),(1.,1.),(1.,
1.),(1.,1.),(1.,1.),(1.,1.),(1.,1.),(1.,1.),(1.,1.),(1.,1.),(1.,1.),(1.,
1.),(1.,1.),(1.,1.),(1.,1.),(1.,1.),(1.,1.),(1.,1.),(1.,1.),(1.,1.),(1.,
1.),(1.,1.),(1.,1.),(1.,1.),(1.,1.),(1.,1.),(1.,1.),(1.,1.),(1.,1.),(1.,
1.),(1.,1.),(1.,1.),(1.,1.),(1.,1.),(1.,1.),(1.,1.),(1.,1.),(1.,1.),(1.,
1.),(1.,1.),(1.,1.),(1.,1.),(1.,1.),(1.,1.),(1.,1.),(1.,1.),(1.,1.),(1.,
1.),(1.,1.),(1.,1.),(1.,1.),(1.,1.),(1.,1.),(1.,1.),(1.,1.),(1.,1.),(1.,
1.),(1.,1.),(1.,1.),(1.,1.),(1.,1.),(1.,1.),(1.,1.),(1.,1.),(1.,1.),(1.,
1.),(1.,1.),(1.,1.),(1.,1.),(1.,1.),(1.,1.),(1.,1.),(1.,1.),(1.,1.),(1.,
1.),(1.,1.),(1.,1.),(1.,1.),(1.,1.),(1.,1.),(1.,1.),(1.,1.),(1.,1.),(1.,
1.),(1.,1.),(1.,1.),(1.,1.),(1.,1.),(1.,1.),(1.,1.),(1.,1.),(1.,1.),(1.,
1.),(1.,1.),(1.,1.),(1.,1.),(1.,1.),(1.,1.),(1.,1.),(1.,1.),(1.,1.),(1.,
1.),(1.,1.),(1.,1.),(1.,1.),(1.,1.),(1.,1.),(1.,1.),(1.,1.),(1.,1.),(1.,
1.),(1.,1.),(1.,1.),(1.,1.),(1.,1.),(1.,1.),(1.,1.),(1.,1.),(1.,1.),(1.,
1.),(1.,1.),(1.,1.),(1.,1.),(1.,1.),(1.,1.),(1.,1.),(1.,1.),(1.,1.),(1.,
1.),(1.,1.),(1.,1.),(1.,1.),(1.,1.),(1.,1.),(1.,1.),(1.,1.),(1.,1.),(1.,
1.),(1.,1.),(1.,1.),(1.,1.),(1.,1.),(1.,1.),(1.,1.),(1.,1.),(1.,1.),(1.,
1.),(1.,1.),(1.,1.),(1.,1.),(1.,1.),(1.,1.),(1.,1.),(1.,1.),(1.,1.),(1.,
1.),(1.,1.),(1.,1.),(1.,1.),(1.,1.),(1.,1.),(1.,1.),(1.,1.),(1.,1.),(1.,
1.),(1.,1.),(1.,1.),(1.,1.),(1.,1.),(1.,1.),(1.,1.),(1.,1.),(1.,1.),(1.,
1.),(1.,1.)))
REPRESENTATION_ITEM('')
SURFACE()
);
#1049=(
BOUNDED_SURFACE()
B_SPLINE_SURFACE(5,1,((#199223,#199224),(#199225,#199226),(#199227,#199228),
(#199229,#199230),(#199231,#199232),(#199233,#199234),(#199235,#199236),
(#199237,#199238),(#199239,#199240),(#199241,#199242),(#199243,#199244),
(#199245,#199246),(#199247,#199248),(#199249,#199250),(#199251,#199252),
(#199253,#199254),(#199255,#199256),(#199257,#199258),(#199259,#199260),
(#199261,#199262),(#199263,#199264),(#199265,#199266),(#199267,#199268),
(#199269,#199270),(#199271,#199272),(#199273,#199274),(#199275,#199276),
(#199277,#199278),(#199279,#199280),(#199281,#199282),(#199283,#199284),
(#199285,#199286),(#199287,#199288),(#199289,#199290),(#199291,#199292),
(#199293,#199294),(#199295,#199296),(#199297,#199298),(#199299,#199300),
(#199301,#199302),(#199303,#199304),(#199305,#199306),(#199307,#199308),
(#199309,#199310),(#199311,#199312),(#199313,#199314),(#199315,#199316),
(#199317,#199318),(#199319,#199320),(#199321,#199322),(#199323,#199324),
(#199325,#199326),(#199327,#199328),(#199329,#199330),(#199331,#199332),
(#199333,#199334),(#199335,#199336),(#199337,#199338),(#199339,#199340),
(#199341,#199342),(#199343,#199344),(#199345,#199346),(#199347,#199348),
(#199349,#199350),(#199351,#199352),(#199353,#199354),(#199355,#199356),
(#199357,#199358),(#199359,#199360),(#199361,#199362),(#199363,#199364),
(#199365,#199366),(#199367,#199368),(#199369,#199370),(#199371,#199372),
(#199373,#199374),(#199375,#199376),(#199377,#199378),(#199379,#199380),
(#199381,#199382),(#199383,#199384),(#199385,#199386),(#199387,#199388),
(#199389,#199390),(#199391,#199392),(#199393,#199394),(#199395,#199396),
(#199397,#199398),(#199399,#199400),(#199401,#199402),(#199403,#199404),
(#199405,#199406),(#199407,#199408),(#199409,#199410),(#199411,#199412),
(#199413,#199414),(#199415,#199416),(#199417,#199418),(#199419,#199420),
(#199421,#199422),(#199423,#199424),(#199425,#199426),(#199427,#199428),
(#199429,#199430),(#199431,#199432),(#199433,#199434),(#199435,#199436),
(#199437,#199438),(#199439,#199440),(#199441,#199442),(#199443,#199444),
(#199445,#199446),(#199447,#199448),(#199449,#199450),(#199451,#199452),
(#199453,#199454),(#199455,#199456),(#199457,#199458),(#199459,#199460),
(#199461,#199462),(#199463,#199464),(#199465,#199466),(#199467,#199468),
(#199469,#199470),(#199471,#199472),(#199473,#199474),(#199475,#199476),
(#199477,#199478),(#199479,#199480),(#199481,#199482),(#199483,#199484),
(#199485,#199486),(#199487,#199488),(#199489,#199490),(#199491,#199492),
(#199493,#199494),(#199495,#199496),(#199497,#199498),(#199499,#199500),
(#199501,#199502),(#199503,#199504),(#199505,#199506),(#199507,#199508),
(#199509,#199510),(#199511,#199512),(#199513,#199514),(#199515,#199516),
(#199517,#199518),(#199519,#199520),(#199521,#199522),(#199523,#199524),
(#199525,#199526),(#199527,#199528),(#199529,#199530),(#199531,#199532),
(#199533,#199534),(#199535,#199536),(#199537,#199538),(#199539,#199540),
(#199541,#199542),(#199543,#199544),(#199545,#199546),(#199547,#199548),
(#199549,#199550),(#199551,#199552),(#199553,#199554),(#199555,#199556),
(#199557,#199558),(#199559,#199560),(#199561,#199562),(#199563,#199564),
(#199565,#199566),(#199567,#199568),(#199569,#199570),(#199571,#199572),
(#199573,#199574),(#199575,#199576),(#199577,#199578),(#199579,#199580),
(#199581,#199582),(#199583,#199584),(#199585,#199586),(#199587,#199588),
(#199589,#199590),(#199591,#199592),(#199593,#199594),(#199595,#199596),
(#199597,#199598),(#199599,#199600),(#199601,#199602),(#199603,#199604),
(#199605,#199606),(#199607,#199608),(#199609,#199610),(#199611,#199612),
(#199613,#199614),(#199615,#199616),(#199617,#199618),(#199619,#199620),
(#199621,#199622),(#199623,#199624),(#199625,#199626),(#199627,#199628),
(#199629,#199630),(#199631,#199632)),.UNSPECIFIED.,.F.,.F.,.F.)
B_SPLINE_SURFACE_WITH_KNOTS((6,1,1,1,1,1,1,1,1,1,1,1,1,1,1,1,1,1,1,1,1,
1,1,1,1,1,1,1,1,1,1,1,1,1,1,1,1,1,1,1,1,1,1,1,1,1,1,1,1,1,1,1,1,1,1,1,1,
1,1,1,1,1,1,1,1,1,1,1,1,1,1,1,1,1,1,1,1,1,1,1,1,1,1,1,1,1,1,1,1,1,1,1,1,
1,1,1,1,1,1,1,1,1,1,1,1,1,1,1,1,1,1,1,1,1,1,1,1,1,1,1,1,1,1,1,1,1,1,1,1,
1,1,1,1,1,1,1,1,1,1,1,1,1,1,1,1,1,1,1,1,1,1,1,1,1,1,1,1,1,1,1,1,1,1,1,1,
1,1,1,1,1,1,1,1,1,1,1,1,1,1,1,1,1,1,1,1,1,1,1,1,1,1,1,1,1,1,1,1,1,1,1,6),
(2,2),(-1.,-0.995000000000001,-0.990000000000001,-0.985000000000001,-0.980000000000001,
-0.975000000000001,-0.970000000000001,-0.965000000000001,-0.960000000000001,
-0.955000000000001,-0.950000000000001,-0.945000000000001,-0.940000000000001,
-0.935000000000001,-0.930000000000001,-0.925000000000001,-0.920000000000001,
-0.915000000000001,-0.910000000000001,-0.905000000000001,-0.900000000000001,
-0.895000000000001,-0.890000000000001,-0.885000000000001,-0.880000000000001,
-0.875000000000001,-0.870000000000001,-0.865000000000001,-0.860000000000001,
-0.855000000000001,-0.850000000000001,-0.845000000000001,-0.840000000000001,
-0.835000000000001,-0.830000000000001,-0.825000000000001,-0.820000000000001,
-0.815000000000001,-0.810000000000001,-0.805000000000001,-0.800000000000001,
-0.795000000000001,-0.790000000000001,-0.785000000000001,-0.780000000000001,
-0.775000000000001,-0.770000000000001,-0.765000000000001,-0.760000000000001,
-0.755000000000001,-0.750000000000001,-0.745000000000001,-0.740000000000001,
-0.735000000000001,-0.730000000000001,-0.725000000000001,-0.720000000000001,
-0.715000000000001,-0.710000000000001,-0.705000000000001,-0.700000000000001,
-0.695000000000001,-0.690000000000001,-0.685,-0.68,-0.675,-0.67,-0.665,
-0.66,-0.655,-0.65,-0.645,-0.64,-0.635,-0.63,-0.625,-0.62,-0.615,-0.61,
-0.605,-0.6,-0.595,-0.59,-0.585,-0.58,-0.575,-0.57,-0.565,-0.56,-0.555,
-0.55,-0.545,-0.54,-0.535,-0.53,-0.525,-0.52,-0.515,-0.51,-0.505,-0.5,-0.495,
-0.49,-0.485,-0.48,-0.475,-0.47,-0.465,-0.46,-0.455,-0.45,-0.445,-0.44,
-0.435,-0.43,-0.425,-0.42,-0.415,-0.41,-0.405,-0.4,-0.395,-0.39,-0.385,
-0.38,-0.375,-0.37,-0.365,-0.36,-0.355,-0.35,-0.345,-0.34,-0.335,-0.33,
-0.325,-0.32,-0.315,-0.31,-0.305,-0.3,-0.295,-0.29,-0.285,-0.28,-0.275,
-0.27,-0.265,-0.26,-0.255,-0.25,-0.245,-0.24,-0.235,-0.23,-0.225,-0.22,
-0.215,-0.21,-0.205,-0.2,-0.195,-0.19,-0.185,-0.18,-0.175,-0.17,-0.165,
-0.16,-0.155,-0.15,-0.145,-0.14,-0.135,-0.13,-0.125,-0.12,-0.115,-0.11,
-0.105,-0.1,-0.095,-0.09,-0.085,-0.08,-0.075,-0.07,-0.065,-0.06,-0.055,
-0.05,-0.045,-0.04,-0.035,-0.03,-0.025,-0.02,-0.015,-0.01,-0.005,0.),(0.,
1.2),.UNSPECIFIED.)
GEOMETRIC_REPRESENTATION_ITEM()
RATIONAL_B_SPLINE_SURFACE(((1.,1.),(1.,1.),(1.,1.),(1.,1.),(1.,1.),(1.,
1.),(1.,1.),(1.,1.),(1.,1.),(1.,1.),(1.,1.),(1.,1.),(1.,1.),(1.,1.),(1.,
1.),(1.,1.),(1.,1.),(1.,1.),(1.,1.),(1.,1.),(1.,1.),(1.,1.),(1.,1.),(1.,
1.),(1.,1.),(1.,1.),(1.,1.),(1.,1.),(1.,1.),(1.,1.),(1.,1.),(1.,1.),(1.,
1.),(1.,1.),(1.,1.),(1.,1.),(1.,1.),(1.,1.),(1.,1.),(1.,1.),(1.,1.),(1.,
1.),(1.,1.),(1.,1.),(1.,1.),(1.,1.),(1.,1.),(1.,1.),(1.,1.),(1.,1.),(1.,
1.),(1.,1.),(1.,1.),(1.,1.),(1.,1.),(1.,1.),(1.,1.),(1.,1.),(1.,1.),(1.,
1.),(1.,1.),(1.,1.),(1.,1.),(1.,1.),(1.,1.),(1.,1.),(1.,1.),(1.,1.),(1.,
1.),(1.,1.),(1.,1.),(1.,1.),(1.,1.),(1.,1.),(1.,1.),(1.,1.),(1.,1.),(1.,
1.),(1.,1.),(1.,1.),(1.,1.),(1.,1.),(1.,1.),(1.,1.),(1.,1.),(1.,1.),(1.,
1.),(1.,1.),(1.,1.),(1.,1.),(1.,1.),(1.,1.),(1.,1.),(1.,1.),(1.,1.),(1.,
1.),(1.,1.),(1.,1.),(1.,1.),(1.,1.),(1.,1.),(1.,1.),(1.,1.),(1.,1.),(1.,
1.),(1.,1.),(1.,1.),(1.,1.),(1.,1.),(1.,1.),(1.,1.),(1.,1.),(1.,1.),(1.,
1.),(1.,1.),(1.,1.),(1.,1.),(1.,1.),(1.,1.),(1.,1.),(1.,1.),(1.,1.),(1.,
1.),(1.,1.),(1.,1.),(1.,1.),(1.,1.),(1.,1.),(1.,1.),(1.,1.),(1.,1.),(1.,
1.),(1.,1.),(1.,1.),(1.,1.),(1.,1.),(1.,1.),(1.,1.),(1.,1.),(1.,1.),(1.,
1.),(1.,1.),(1.,1.),(1.,1.),(1.,1.),(1.,1.),(1.,1.),(1.,1.),(1.,1.),(1.,
1.),(1.,1.),(1.,1.),(1.,1.),(1.,1.),(1.,1.),(1.,1.),(1.,1.),(1.,1.),(1.,
1.),(1.,1.),(1.,1.),(1.,1.),(1.,1.),(1.,1.),(1.,1.),(1.,1.),(1.,1.),(1.,
1.),(1.,1.),(1.,1.),(1.,1.),(1.,1.),(1.,1.),(1.,1.),(1.,1.),(1.,1.),(1.,
1.),(1.,1.),(1.,1.),(1.,1.),(1.,1.),(1.,1.),(1.,1.),(1.,1.),(1.,1.),(1.,
1.),(1.,1.),(1.,1.),(1.,1.),(1.,1.),(1.,1.),(1.,1.),(1.,1.),(1.,1.),(1.,
1.),(1.,1.),(1.,1.),(1.,1.),(1.,1.),(1.,1.),(1.,1.),(1.,1.),(1.,1.),(1.,
1.),(1.,1.)))
REPRESENTATION_ITEM('')
SURFACE()
);
#1050=(
BOUNDED_SURFACE()
B_SPLINE_SURFACE(5,1,((#199840,#199841),(#199842,#199843),(#199844,#199845),
(#199846,#199847),(#199848,#199849),(#199850,#199851),(#199852,#199853),
(#199854,#199855),(#199856,#199857),(#199858,#199859),(#199860,#199861),
(#199862,#199863),(#199864,#199865),(#199866,#199867),(#199868,#199869),
(#199870,#199871),(#199872,#199873),(#199874,#199875),(#199876,#199877),
(#199878,#199879),(#199880,#199881),(#199882,#199883),(#199884,#199885),
(#199886,#199887),(#199888,#199889),(#199890,#199891),(#199892,#199893),
(#199894,#199895),(#199896,#199897),(#199898,#199899),(#199900,#199901),
(#199902,#199903),(#199904,#199905),(#199906,#199907),(#199908,#199909),
(#199910,#199911),(#199912,#199913),(#199914,#199915),(#199916,#199917),
(#199918,#199919),(#199920,#199921),(#199922,#199923),(#199924,#199925),
(#199926,#199927),(#199928,#199929),(#199930,#199931),(#199932,#199933),
(#199934,#199935),(#199936,#199937),(#199938,#199939),(#199940,#199941),
(#199942,#199943),(#199944,#199945),(#199946,#199947),(#199948,#199949),
(#199950,#199951),(#199952,#199953),(#199954,#199955),(#199956,#199957),
(#199958,#199959),(#199960,#199961),(#199962,#199963),(#199964,#199965),
(#199966,#199967),(#199968,#199969),(#199970,#199971),(#199972,#199973),
(#199974,#199975),(#199976,#199977),(#199978,#199979),(#199980,#199981),
(#199982,#199983),(#199984,#199985),(#199986,#199987),(#199988,#199989),
(#199990,#199991),(#199992,#199993),(#199994,#199995),(#199996,#199997),
(#199998,#199999),(#200000,#200001),(#200002,#200003),(#200004,#200005),
(#200006,#200007),(#200008,#200009),(#200010,#200011),(#200012,#200013),
(#200014,#200015),(#200016,#200017),(#200018,#200019),(#200020,#200021),
(#200022,#200023),(#200024,#200025),(#200026,#200027),(#200028,#200029),
(#200030,#200031),(#200032,#200033),(#200034,#200035),(#200036,#200037),
(#200038,#200039),(#200040,#200041),(#200042,#200043),(#200044,#200045),
(#200046,#200047),(#200048,#200049),(#200050,#200051),(#200052,#200053),
(#200054,#200055),(#200056,#200057),(#200058,#200059),(#200060,#200061),
(#200062,#200063),(#200064,#200065),(#200066,#200067),(#200068,#200069),
(#200070,#200071),(#200072,#200073),(#200074,#200075),(#200076,#200077),
(#200078,#200079),(#200080,#200081),(#200082,#200083),(#200084,#200085),
(#200086,#200087),(#200088,#200089),(#200090,#200091),(#200092,#200093),
(#200094,#200095),(#200096,#200097),(#200098,#200099),(#200100,#200101),
(#200102,#200103),(#200104,#200105),(#200106,#200107),(#200108,#200109),
(#200110,#200111),(#200112,#200113),(#200114,#200115),(#200116,#200117),
(#200118,#200119),(#200120,#200121),(#200122,#200123),(#200124,#200125),
(#200126,#200127),(#200128,#200129),(#200130,#200131),(#200132,#200133),
(#200134,#200135),(#200136,#200137),(#200138,#200139),(#200140,#200141),
(#200142,#200143),(#200144,#200145),(#200146,#200147),(#200148,#200149),
(#200150,#200151),(#200152,#200153),(#200154,#200155),(#200156,#200157),
(#200158,#200159),(#200160,#200161),(#200162,#200163),(#200164,#200165),
(#200166,#200167),(#200168,#200169),(#200170,#200171),(#200172,#200173),
(#200174,#200175),(#200176,#200177),(#200178,#200179),(#200180,#200181),
(#200182,#200183),(#200184,#200185),(#200186,#200187),(#200188,#200189),
(#200190,#200191),(#200192,#200193),(#200194,#200195),(#200196,#200197),
(#200198,#200199),(#200200,#200201),(#200202,#200203),(#200204,#200205),
(#200206,#200207),(#200208,#200209),(#200210,#200211),(#200212,#200213),
(#200214,#200215),(#200216,#200217),(#200218,#200219),(#200220,#200221),
(#200222,#200223),(#200224,#200225),(#200226,#200227),(#200228,#200229),
(#200230,#200231),(#200232,#200233),(#200234,#200235),(#200236,#200237),
(#200238,#200239),(#200240,#200241),(#200242,#200243),(#200244,#200245),
(#200246,#200247),(#200248,#200249)),.UNSPECIFIED.,.F.,.F.,.F.)
B_SPLINE_SURFACE_WITH_KNOTS((6,1,1,1,1,1,1,1,1,1,1,1,1,1,1,1,1,1,1,1,1,
1,1,1,1,1,1,1,1,1,1,1,1,1,1,1,1,1,1,1,1,1,1,1,1,1,1,1,1,1,1,1,1,1,1,1,1,
1,1,1,1,1,1,1,1,1,1,1,1,1,1,1,1,1,1,1,1,1,1,1,1,1,1,1,1,1,1,1,1,1,1,1,1,
1,1,1,1,1,1,1,1,1,1,1,1,1,1,1,1,1,1,1,1,1,1,1,1,1,1,1,1,1,1,1,1,1,1,1,1,
1,1,1,1,1,1,1,1,1,1,1,1,1,1,1,1,1,1,1,1,1,1,1,1,1,1,1,1,1,1,1,1,1,1,1,1,
1,1,1,1,1,1,1,1,1,1,1,1,1,1,1,1,1,1,1,1,1,1,1,1,1,1,1,1,1,1,1,1,1,1,1,6),
(2,2),(0.,0.005,0.01,0.015,0.02,0.025,0.03,0.035,0.04,0.045,0.05,0.055,
0.06,0.065,0.07,0.075,0.08,0.085,0.09,0.095,0.1,0.105,0.11,0.115,0.12,0.125,
0.13,0.135,0.14,0.145,0.15,0.155,0.16,0.165,0.17,0.175,0.18,0.185,0.19,
0.195,0.2,0.205,0.21,0.215,0.22,0.225,0.23,0.235,0.24,0.245,0.25,0.255,
0.26,0.265,0.27,0.275,0.28,0.285,0.29,0.295,0.3,0.305,0.31,0.315,0.32,0.325,
0.33,0.335,0.34,0.345,0.35,0.355,0.36,0.365,0.37,0.375,0.38,0.385,0.39,
0.395,0.4,0.405,0.41,0.415,0.42,0.425,0.43,0.435,0.44,0.445,0.45,0.455,
0.46,0.465,0.47,0.475,0.48,0.485,0.49,0.495,0.5,0.505,0.51,0.515,0.52,0.525,
0.53,0.535,0.54,0.545,0.55,0.555,0.56,0.565,0.57,0.575,0.58,0.585,0.59,
0.595,0.6,0.605,0.61,0.615,0.62,0.625,0.63,0.635,0.64,0.645,0.65,0.655,
0.66,0.665,0.67,0.675,0.68,0.685,0.690000000000001,0.695000000000001,0.700000000000001,
0.705000000000001,0.710000000000001,0.715000000000001,0.720000000000001,
0.725000000000001,0.730000000000001,0.735000000000001,0.740000000000001,
0.745000000000001,0.750000000000001,0.755000000000001,0.760000000000001,
0.765000000000001,0.770000000000001,0.775000000000001,0.780000000000001,
0.785000000000001,0.790000000000001,0.795000000000001,0.800000000000001,
0.805000000000001,0.810000000000001,0.815000000000001,0.820000000000001,
0.825000000000001,0.830000000000001,0.835000000000001,0.840000000000001,
0.845000000000001,0.850000000000001,0.855000000000001,0.860000000000001,
0.865000000000001,0.870000000000001,0.875000000000001,0.880000000000001,
0.885000000000001,0.890000000000001,0.895000000000001,0.900000000000001,
0.905000000000001,0.910000000000001,0.915000000000001,0.920000000000001,
0.925000000000001,0.930000000000001,0.935000000000001,0.940000000000001,
0.945000000000001,0.950000000000001,0.955000000000001,0.960000000000001,
0.965000000000001,0.970000000000001,0.975000000000001,0.980000000000001,
0.985000000000001,0.990000000000001,0.995000000000001,1.),(0.,1.2),
 .UNSPECIFIED.)
GEOMETRIC_REPRESENTATION_ITEM()
RATIONAL_B_SPLINE_SURFACE(((1.,1.),(1.,1.),(1.,1.),(1.,1.),(1.,1.),(1.,
1.),(1.,1.),(1.,1.),(1.,1.),(1.,1.),(1.,1.),(1.,1.),(1.,1.),(1.,1.),(1.,
1.),(1.,1.),(1.,1.),(1.,1.),(1.,1.),(1.,1.),(1.,1.),(1.,1.),(1.,1.),(1.,
1.),(1.,1.),(1.,1.),(1.,1.),(1.,1.),(1.,1.),(1.,1.),(1.,1.),(1.,1.),(1.,
1.),(1.,1.),(1.,1.),(1.,1.),(1.,1.),(1.,1.),(1.,1.),(1.,1.),(1.,1.),(1.,
1.),(1.,1.),(1.,1.),(1.,1.),(1.,1.),(1.,1.),(1.,1.),(1.,1.),(1.,1.),(1.,
1.),(1.,1.),(1.,1.),(1.,1.),(1.,1.),(1.,1.),(1.,1.),(1.,1.),(1.,1.),(1.,
1.),(1.,1.),(1.,1.),(1.,1.),(1.,1.),(1.,1.),(1.,1.),(1.,1.),(1.,1.),(1.,
1.),(1.,1.),(1.,1.),(1.,1.),(1.,1.),(1.,1.),(1.,1.),(1.,1.),(1.,1.),(1.,
1.),(1.,1.),(1.,1.),(1.,1.),(1.,1.),(1.,1.),(1.,1.),(1.,1.),(1.,1.),(1.,
1.),(1.,1.),(1.,1.),(1.,1.),(1.,1.),(1.,1.),(1.,1.),(1.,1.),(1.,1.),(1.,
1.),(1.,1.),(1.,1.),(1.,1.),(1.,1.),(1.,1.),(1.,1.),(1.,1.),(1.,1.),(1.,
1.),(1.,1.),(1.,1.),(1.,1.),(1.,1.),(1.,1.),(1.,1.),(1.,1.),(1.,1.),(1.,
1.),(1.,1.),(1.,1.),(1.,1.),(1.,1.),(1.,1.),(1.,1.),(1.,1.),(1.,1.),(1.,
1.),(1.,1.),(1.,1.),(1.,1.),(1.,1.),(1.,1.),(1.,1.),(1.,1.),(1.,1.),(1.,
1.),(1.,1.),(1.,1.),(1.,1.),(1.,1.),(1.,1.),(1.,1.),(1.,1.),(1.,1.),(1.,
1.),(1.,1.),(1.,1.),(1.,1.),(1.,1.),(1.,1.),(1.,1.),(1.,1.),(1.,1.),(1.,
1.),(1.,1.),(1.,1.),(1.,1.),(1.,1.),(1.,1.),(1.,1.),(1.,1.),(1.,1.),(1.,
1.),(1.,1.),(1.,1.),(1.,1.),(1.,1.),(1.,1.),(1.,1.),(1.,1.),(1.,1.),(1.,
1.),(1.,1.),(1.,1.),(1.,1.),(1.,1.),(1.,1.),(1.,1.),(1.,1.),(1.,1.),(1.,
1.),(1.,1.),(1.,1.),(1.,1.),(1.,1.),(1.,1.),(1.,1.),(1.,1.),(1.,1.),(1.,
1.),(1.,1.),(1.,1.),(1.,1.),(1.,1.),(1.,1.),(1.,1.),(1.,1.),(1.,1.),(1.,
1.),(1.,1.),(1.,1.),(1.,1.),(1.,1.),(1.,1.),(1.,1.),(1.,1.),(1.,1.),(1.,
1.),(1.,1.)))
REPRESENTATION_ITEM('')
SURFACE()
);
#1051=(
BOUNDED_SURFACE()
B_SPLINE_SURFACE(5,1,((#200461,#200462),(#200463,#200464),(#200465,#200466),
(#200467,#200468),(#200469,#200470),(#200471,#200472),(#200473,#200474),
(#200475,#200476),(#200477,#200478),(#200479,#200480),(#200481,#200482),
(#200483,#200484),(#200485,#200486),(#200487,#200488),(#200489,#200490),
(#200491,#200492),(#200493,#200494),(#200495,#200496),(#200497,#200498),
(#200499,#200500),(#200501,#200502),(#200503,#200504),(#200505,#200506),
(#200507,#200508),(#200509,#200510),(#200511,#200512),(#200513,#200514),
(#200515,#200516),(#200517,#200518),(#200519,#200520),(#200521,#200522),
(#200523,#200524),(#200525,#200526),(#200527,#200528),(#200529,#200530),
(#200531,#200532),(#200533,#200534),(#200535,#200536),(#200537,#200538),
(#200539,#200540),(#200541,#200542),(#200543,#200544),(#200545,#200546),
(#200547,#200548),(#200549,#200550),(#200551,#200552),(#200553,#200554),
(#200555,#200556),(#200557,#200558),(#200559,#200560),(#200561,#200562),
(#200563,#200564),(#200565,#200566),(#200567,#200568),(#200569,#200570),
(#200571,#200572),(#200573,#200574),(#200575,#200576),(#200577,#200578),
(#200579,#200580),(#200581,#200582),(#200583,#200584),(#200585,#200586),
(#200587,#200588),(#200589,#200590),(#200591,#200592),(#200593,#200594),
(#200595,#200596),(#200597,#200598),(#200599,#200600),(#200601,#200602),
(#200603,#200604),(#200605,#200606),(#200607,#200608),(#200609,#200610),
(#200611,#200612),(#200613,#200614),(#200615,#200616),(#200617,#200618),
(#200619,#200620),(#200621,#200622),(#200623,#200624),(#200625,#200626),
(#200627,#200628),(#200629,#200630),(#200631,#200632),(#200633,#200634),
(#200635,#200636),(#200637,#200638),(#200639,#200640),(#200641,#200642),
(#200643,#200644),(#200645,#200646),(#200647,#200648),(#200649,#200650),
(#200651,#200652),(#200653,#200654),(#200655,#200656),(#200657,#200658),
(#200659,#200660),(#200661,#200662),(#200663,#200664),(#200665,#200666),
(#200667,#200668),(#200669,#200670),(#200671,#200672),(#200673,#200674),
(#200675,#200676),(#200677,#200678),(#200679,#200680),(#200681,#200682),
(#200683,#200684),(#200685,#200686),(#200687,#200688),(#200689,#200690),
(#200691,#200692),(#200693,#200694),(#200695,#200696),(#200697,#200698),
(#200699,#200700),(#200701,#200702),(#200703,#200704),(#200705,#200706),
(#200707,#200708),(#200709,#200710),(#200711,#200712),(#200713,#200714),
(#200715,#200716),(#200717,#200718),(#200719,#200720),(#200721,#200722),
(#200723,#200724),(#200725,#200726),(#200727,#200728),(#200729,#200730),
(#200731,#200732),(#200733,#200734),(#200735,#200736),(#200737,#200738),
(#200739,#200740),(#200741,#200742),(#200743,#200744),(#200745,#200746),
(#200747,#200748),(#200749,#200750),(#200751,#200752),(#200753,#200754),
(#200755,#200756),(#200757,#200758),(#200759,#200760),(#200761,#200762),
(#200763,#200764),(#200765,#200766),(#200767,#200768),(#200769,#200770),
(#200771,#200772),(#200773,#200774),(#200775,#200776),(#200777,#200778),
(#200779,#200780),(#200781,#200782),(#200783,#200784),(#200785,#200786),
(#200787,#200788),(#200789,#200790),(#200791,#200792),(#200793,#200794),
(#200795,#200796),(#200797,#200798),(#200799,#200800),(#200801,#200802),
(#200803,#200804),(#200805,#200806),(#200807,#200808),(#200809,#200810),
(#200811,#200812),(#200813,#200814),(#200815,#200816),(#200817,#200818),
(#200819,#200820),(#200821,#200822),(#200823,#200824),(#200825,#200826),
(#200827,#200828),(#200829,#200830),(#200831,#200832),(#200833,#200834),
(#200835,#200836),(#200837,#200838),(#200839,#200840),(#200841,#200842),
(#200843,#200844),(#200845,#200846),(#200847,#200848),(#200849,#200850),
(#200851,#200852),(#200853,#200854),(#200855,#200856),(#200857,#200858),
(#200859,#200860),(#200861,#200862),(#200863,#200864),(#200865,#200866),
(#200867,#200868),(#200869,#200870)),.UNSPECIFIED.,.F.,.F.,.F.)
B_SPLINE_SURFACE_WITH_KNOTS((6,1,1,1,1,1,1,1,1,1,1,1,1,1,1,1,1,1,1,1,1,
1,1,1,1,1,1,1,1,1,1,1,1,1,1,1,1,1,1,1,1,1,1,1,1,1,1,1,1,1,1,1,1,1,1,1,1,
1,1,1,1,1,1,1,1,1,1,1,1,1,1,1,1,1,1,1,1,1,1,1,1,1,1,1,1,1,1,1,1,1,1,1,1,
1,1,1,1,1,1,1,1,1,1,1,1,1,1,1,1,1,1,1,1,1,1,1,1,1,1,1,1,1,1,1,1,1,1,1,1,
1,1,1,1,1,1,1,1,1,1,1,1,1,1,1,1,1,1,1,1,1,1,1,1,1,1,1,1,1,1,1,1,1,1,1,1,
1,1,1,1,1,1,1,1,1,1,1,1,1,1,1,1,1,1,1,1,1,1,1,1,1,1,1,1,1,1,1,1,1,1,1,6),
(2,2),(-1.,-0.995000000000001,-0.990000000000001,-0.985000000000001,-0.980000000000001,
-0.975000000000001,-0.970000000000001,-0.965000000000001,-0.960000000000001,
-0.955000000000001,-0.950000000000001,-0.945000000000001,-0.940000000000001,
-0.935000000000001,-0.930000000000001,-0.925000000000001,-0.920000000000001,
-0.915000000000001,-0.910000000000001,-0.905000000000001,-0.900000000000001,
-0.895000000000001,-0.890000000000001,-0.885000000000001,-0.880000000000001,
-0.875000000000001,-0.870000000000001,-0.865000000000001,-0.860000000000001,
-0.855000000000001,-0.850000000000001,-0.845000000000001,-0.840000000000001,
-0.835000000000001,-0.830000000000001,-0.825000000000001,-0.820000000000001,
-0.815000000000001,-0.810000000000001,-0.805000000000001,-0.800000000000001,
-0.795000000000001,-0.790000000000001,-0.785000000000001,-0.780000000000001,
-0.775000000000001,-0.770000000000001,-0.765000000000001,-0.760000000000001,
-0.755000000000001,-0.750000000000001,-0.745000000000001,-0.740000000000001,
-0.735000000000001,-0.730000000000001,-0.725000000000001,-0.720000000000001,
-0.715000000000001,-0.710000000000001,-0.705000000000001,-0.700000000000001,
-0.695000000000001,-0.690000000000001,-0.685,-0.68,-0.675,-0.67,-0.665,
-0.66,-0.655,-0.65,-0.645,-0.64,-0.635,-0.63,-0.625,-0.62,-0.615,-0.61,
-0.605,-0.6,-0.595,-0.59,-0.585,-0.58,-0.575,-0.57,-0.565,-0.56,-0.555,
-0.55,-0.545,-0.54,-0.535,-0.53,-0.525,-0.52,-0.515,-0.51,-0.505,-0.5,-0.495,
-0.49,-0.485,-0.48,-0.475,-0.47,-0.465,-0.46,-0.455,-0.45,-0.445,-0.44,
-0.435,-0.43,-0.425,-0.42,-0.415,-0.41,-0.405,-0.4,-0.395,-0.39,-0.385,
-0.38,-0.375,-0.37,-0.365,-0.36,-0.355,-0.35,-0.345,-0.34,-0.335,-0.33,
-0.325,-0.32,-0.315,-0.31,-0.305,-0.3,-0.295,-0.29,-0.285,-0.28,-0.275,
-0.27,-0.265,-0.26,-0.255,-0.25,-0.245,-0.24,-0.235,-0.23,-0.225,-0.22,
-0.215,-0.21,-0.205,-0.2,-0.195,-0.19,-0.185,-0.18,-0.175,-0.17,-0.165,
-0.16,-0.155,-0.15,-0.145,-0.14,-0.135,-0.13,-0.125,-0.12,-0.115,-0.11,
-0.105,-0.1,-0.095,-0.09,-0.085,-0.08,-0.075,-0.07,-0.065,-0.06,-0.055,
-0.05,-0.045,-0.04,-0.035,-0.03,-0.025,-0.02,-0.015,-0.01,-0.005,0.),(0.,
1.2),.UNSPECIFIED.)
GEOMETRIC_REPRESENTATION_ITEM()
RATIONAL_B_SPLINE_SURFACE(((1.,1.),(1.,1.),(1.,1.),(1.,1.),(1.,1.),(1.,
1.),(1.,1.),(1.,1.),(1.,1.),(1.,1.),(1.,1.),(1.,1.),(1.,1.),(1.,1.),(1.,
1.),(1.,1.),(1.,1.),(1.,1.),(1.,1.),(1.,1.),(1.,1.),(1.,1.),(1.,1.),(1.,
1.),(1.,1.),(1.,1.),(1.,1.),(1.,1.),(1.,1.),(1.,1.),(1.,1.),(1.,1.),(1.,
1.),(1.,1.),(1.,1.),(1.,1.),(1.,1.),(1.,1.),(1.,1.),(1.,1.),(1.,1.),(1.,
1.),(1.,1.),(1.,1.),(1.,1.),(1.,1.),(1.,1.),(1.,1.),(1.,1.),(1.,1.),(1.,
1.),(1.,1.),(1.,1.),(1.,1.),(1.,1.),(1.,1.),(1.,1.),(1.,1.),(1.,1.),(1.,
1.),(1.,1.),(1.,1.),(1.,1.),(1.,1.),(1.,1.),(1.,1.),(1.,1.),(1.,1.),(1.,
1.),(1.,1.),(1.,1.),(1.,1.),(1.,1.),(1.,1.),(1.,1.),(1.,1.),(1.,1.),(1.,
1.),(1.,1.),(1.,1.),(1.,1.),(1.,1.),(1.,1.),(1.,1.),(1.,1.),(1.,1.),(1.,
1.),(1.,1.),(1.,1.),(1.,1.),(1.,1.),(1.,1.),(1.,1.),(1.,1.),(1.,1.),(1.,
1.),(1.,1.),(1.,1.),(1.,1.),(1.,1.),(1.,1.),(1.,1.),(1.,1.),(1.,1.),(1.,
1.),(1.,1.),(1.,1.),(1.,1.),(1.,1.),(1.,1.),(1.,1.),(1.,1.),(1.,1.),(1.,
1.),(1.,1.),(1.,1.),(1.,1.),(1.,1.),(1.,1.),(1.,1.),(1.,1.),(1.,1.),(1.,
1.),(1.,1.),(1.,1.),(1.,1.),(1.,1.),(1.,1.),(1.,1.),(1.,1.),(1.,1.),(1.,
1.),(1.,1.),(1.,1.),(1.,1.),(1.,1.),(1.,1.),(1.,1.),(1.,1.),(1.,1.),(1.,
1.),(1.,1.),(1.,1.),(1.,1.),(1.,1.),(1.,1.),(1.,1.),(1.,1.),(1.,1.),(1.,
1.),(1.,1.),(1.,1.),(1.,1.),(1.,1.),(1.,1.),(1.,1.),(1.,1.),(1.,1.),(1.,
1.),(1.,1.),(1.,1.),(1.,1.),(1.,1.),(1.,1.),(1.,1.),(1.,1.),(1.,1.),(1.,
1.),(1.,1.),(1.,1.),(1.,1.),(1.,1.),(1.,1.),(1.,1.),(1.,1.),(1.,1.),(1.,
1.),(1.,1.),(1.,1.),(1.,1.),(1.,1.),(1.,1.),(1.,1.),(1.,1.),(1.,1.),(1.,
1.),(1.,1.),(1.,1.),(1.,1.),(1.,1.),(1.,1.),(1.,1.),(1.,1.),(1.,1.),(1.,
1.),(1.,1.),(1.,1.),(1.,1.),(1.,1.),(1.,1.),(1.,1.),(1.,1.),(1.,1.),(1.,
1.),(1.,1.)))
REPRESENTATION_ITEM('')
SURFACE()
);
#1052=(
BOUNDED_SURFACE()
B_SPLINE_SURFACE(5,1,((#201078,#201079),(#201080,#201081),(#201082,#201083),
(#201084,#201085),(#201086,#201087),(#201088,#201089),(#201090,#201091),
(#201092,#201093),(#201094,#201095),(#201096,#201097),(#201098,#201099),
(#201100,#201101),(#201102,#201103),(#201104,#201105),(#201106,#201107),
(#201108,#201109),(#201110,#201111),(#201112,#201113),(#201114,#201115),
(#201116,#201117),(#201118,#201119),(#201120,#201121),(#201122,#201123),
(#201124,#201125),(#201126,#201127),(#201128,#201129),(#201130,#201131),
(#201132,#201133),(#201134,#201135),(#201136,#201137),(#201138,#201139),
(#201140,#201141),(#201142,#201143),(#201144,#201145),(#201146,#201147),
(#201148,#201149),(#201150,#201151),(#201152,#201153),(#201154,#201155),
(#201156,#201157),(#201158,#201159),(#201160,#201161),(#201162,#201163),
(#201164,#201165),(#201166,#201167),(#201168,#201169),(#201170,#201171),
(#201172,#201173),(#201174,#201175),(#201176,#201177),(#201178,#201179),
(#201180,#201181),(#201182,#201183),(#201184,#201185),(#201186,#201187),
(#201188,#201189),(#201190,#201191),(#201192,#201193),(#201194,#201195),
(#201196,#201197),(#201198,#201199),(#201200,#201201),(#201202,#201203),
(#201204,#201205),(#201206,#201207),(#201208,#201209),(#201210,#201211),
(#201212,#201213),(#201214,#201215),(#201216,#201217),(#201218,#201219),
(#201220,#201221),(#201222,#201223),(#201224,#201225),(#201226,#201227),
(#201228,#201229),(#201230,#201231),(#201232,#201233),(#201234,#201235),
(#201236,#201237),(#201238,#201239),(#201240,#201241),(#201242,#201243),
(#201244,#201245),(#201246,#201247),(#201248,#201249),(#201250,#201251),
(#201252,#201253),(#201254,#201255),(#201256,#201257),(#201258,#201259),
(#201260,#201261),(#201262,#201263),(#201264,#201265),(#201266,#201267),
(#201268,#201269),(#201270,#201271),(#201272,#201273),(#201274,#201275),
(#201276,#201277),(#201278,#201279),(#201280,#201281),(#201282,#201283),
(#201284,#201285),(#201286,#201287),(#201288,#201289),(#201290,#201291),
(#201292,#201293),(#201294,#201295),(#201296,#201297),(#201298,#201299),
(#201300,#201301),(#201302,#201303),(#201304,#201305),(#201306,#201307),
(#201308,#201309),(#201310,#201311),(#201312,#201313),(#201314,#201315),
(#201316,#201317),(#201318,#201319),(#201320,#201321),(#201322,#201323),
(#201324,#201325),(#201326,#201327),(#201328,#201329),(#201330,#201331),
(#201332,#201333),(#201334,#201335),(#201336,#201337),(#201338,#201339),
(#201340,#201341),(#201342,#201343),(#201344,#201345),(#201346,#201347),
(#201348,#201349),(#201350,#201351),(#201352,#201353),(#201354,#201355),
(#201356,#201357),(#201358,#201359),(#201360,#201361),(#201362,#201363),
(#201364,#201365),(#201366,#201367),(#201368,#201369),(#201370,#201371),
(#201372,#201373),(#201374,#201375),(#201376,#201377),(#201378,#201379),
(#201380,#201381),(#201382,#201383),(#201384,#201385),(#201386,#201387),
(#201388,#201389),(#201390,#201391),(#201392,#201393),(#201394,#201395),
(#201396,#201397),(#201398,#201399),(#201400,#201401),(#201402,#201403),
(#201404,#201405),(#201406,#201407),(#201408,#201409),(#201410,#201411),
(#201412,#201413),(#201414,#201415),(#201416,#201417),(#201418,#201419),
(#201420,#201421),(#201422,#201423),(#201424,#201425),(#201426,#201427),
(#201428,#201429),(#201430,#201431),(#201432,#201433),(#201434,#201435),
(#201436,#201437),(#201438,#201439),(#201440,#201441),(#201442,#201443),
(#201444,#201445),(#201446,#201447),(#201448,#201449),(#201450,#201451),
(#201452,#201453),(#201454,#201455),(#201456,#201457),(#201458,#201459),
(#201460,#201461),(#201462,#201463),(#201464,#201465),(#201466,#201467),
(#201468,#201469),(#201470,#201471),(#201472,#201473),(#201474,#201475),
(#201476,#201477),(#201478,#201479),(#201480,#201481),(#201482,#201483),
(#201484,#201485),(#201486,#201487)),.UNSPECIFIED.,.F.,.F.,.F.)
B_SPLINE_SURFACE_WITH_KNOTS((6,1,1,1,1,1,1,1,1,1,1,1,1,1,1,1,1,1,1,1,1,
1,1,1,1,1,1,1,1,1,1,1,1,1,1,1,1,1,1,1,1,1,1,1,1,1,1,1,1,1,1,1,1,1,1,1,1,
1,1,1,1,1,1,1,1,1,1,1,1,1,1,1,1,1,1,1,1,1,1,1,1,1,1,1,1,1,1,1,1,1,1,1,1,
1,1,1,1,1,1,1,1,1,1,1,1,1,1,1,1,1,1,1,1,1,1,1,1,1,1,1,1,1,1,1,1,1,1,1,1,
1,1,1,1,1,1,1,1,1,1,1,1,1,1,1,1,1,1,1,1,1,1,1,1,1,1,1,1,1,1,1,1,1,1,1,1,
1,1,1,1,1,1,1,1,1,1,1,1,1,1,1,1,1,1,1,1,1,1,1,1,1,1,1,1,1,1,1,1,1,1,1,6),
(2,2),(0.,0.005,0.01,0.015,0.02,0.025,0.03,0.035,0.04,0.045,0.05,0.055,
0.06,0.065,0.07,0.075,0.08,0.085,0.09,0.095,0.1,0.105,0.11,0.115,0.12,0.125,
0.13,0.135,0.14,0.145,0.15,0.155,0.16,0.165,0.17,0.175,0.18,0.185,0.19,
0.195,0.2,0.205,0.21,0.215,0.22,0.225,0.23,0.235,0.24,0.245,0.25,0.255,
0.26,0.265,0.27,0.275,0.28,0.285,0.29,0.295,0.3,0.305,0.31,0.315,0.32,0.325,
0.33,0.335,0.34,0.345,0.35,0.355,0.36,0.365,0.37,0.375,0.38,0.385,0.39,
0.395,0.4,0.405,0.41,0.415,0.42,0.425,0.43,0.435,0.44,0.445,0.45,0.455,
0.46,0.465,0.47,0.475,0.48,0.485,0.49,0.495,0.5,0.505,0.51,0.515,0.52,0.525,
0.53,0.535,0.54,0.545,0.55,0.555,0.56,0.565,0.57,0.575,0.58,0.585,0.59,
0.595,0.6,0.605,0.61,0.615,0.62,0.625,0.63,0.635,0.64,0.645,0.65,0.655,
0.66,0.665,0.67,0.675,0.68,0.685,0.690000000000001,0.695000000000001,0.700000000000001,
0.705000000000001,0.710000000000001,0.715000000000001,0.720000000000001,
0.725000000000001,0.730000000000001,0.735000000000001,0.740000000000001,
0.745000000000001,0.750000000000001,0.755000000000001,0.760000000000001,
0.765000000000001,0.770000000000001,0.775000000000001,0.780000000000001,
0.785000000000001,0.790000000000001,0.795000000000001,0.800000000000001,
0.805000000000001,0.810000000000001,0.815000000000001,0.820000000000001,
0.825000000000001,0.830000000000001,0.835000000000001,0.840000000000001,
0.845000000000001,0.850000000000001,0.855000000000001,0.860000000000001,
0.865000000000001,0.870000000000001,0.875000000000001,0.880000000000001,
0.885000000000001,0.890000000000001,0.895000000000001,0.900000000000001,
0.905000000000001,0.910000000000001,0.915000000000001,0.920000000000001,
0.925000000000001,0.930000000000001,0.935000000000001,0.940000000000001,
0.945000000000001,0.950000000000001,0.955000000000001,0.960000000000001,
0.965000000000001,0.970000000000001,0.975000000000001,0.980000000000001,
0.985000000000001,0.990000000000001,0.995000000000001,1.),(0.,1.2),
 .UNSPECIFIED.)
GEOMETRIC_REPRESENTATION_ITEM()
RATIONAL_B_SPLINE_SURFACE(((1.,1.),(1.,1.),(1.,1.),(1.,1.),(1.,1.),(1.,
1.),(1.,1.),(1.,1.),(1.,1.),(1.,1.),(1.,1.),(1.,1.),(1.,1.),(1.,1.),(1.,
1.),(1.,1.),(1.,1.),(1.,1.),(1.,1.),(1.,1.),(1.,1.),(1.,1.),(1.,1.),(1.,
1.),(1.,1.),(1.,1.),(1.,1.),(1.,1.),(1.,1.),(1.,1.),(1.,1.),(1.,1.),(1.,
1.),(1.,1.),(1.,1.),(1.,1.),(1.,1.),(1.,1.),(1.,1.),(1.,1.),(1.,1.),(1.,
1.),(1.,1.),(1.,1.),(1.,1.),(1.,1.),(1.,1.),(1.,1.),(1.,1.),(1.,1.),(1.,
1.),(1.,1.),(1.,1.),(1.,1.),(1.,1.),(1.,1.),(1.,1.),(1.,1.),(1.,1.),(1.,
1.),(1.,1.),(1.,1.),(1.,1.),(1.,1.),(1.,1.),(1.,1.),(1.,1.),(1.,1.),(1.,
1.),(1.,1.),(1.,1.),(1.,1.),(1.,1.),(1.,1.),(1.,1.),(1.,1.),(1.,1.),(1.,
1.),(1.,1.),(1.,1.),(1.,1.),(1.,1.),(1.,1.),(1.,1.),(1.,1.),(1.,1.),(1.,
1.),(1.,1.),(1.,1.),(1.,1.),(1.,1.),(1.,1.),(1.,1.),(1.,1.),(1.,1.),(1.,
1.),(1.,1.),(1.,1.),(1.,1.),(1.,1.),(1.,1.),(1.,1.),(1.,1.),(1.,1.),(1.,
1.),(1.,1.),(1.,1.),(1.,1.),(1.,1.),(1.,1.),(1.,1.),(1.,1.),(1.,1.),(1.,
1.),(1.,1.),(1.,1.),(1.,1.),(1.,1.),(1.,1.),(1.,1.),(1.,1.),(1.,1.),(1.,
1.),(1.,1.),(1.,1.),(1.,1.),(1.,1.),(1.,1.),(1.,1.),(1.,1.),(1.,1.),(1.,
1.),(1.,1.),(1.,1.),(1.,1.),(1.,1.),(1.,1.),(1.,1.),(1.,1.),(1.,1.),(1.,
1.),(1.,1.),(1.,1.),(1.,1.),(1.,1.),(1.,1.),(1.,1.),(1.,1.),(1.,1.),(1.,
1.),(1.,1.),(1.,1.),(1.,1.),(1.,1.),(1.,1.),(1.,1.),(1.,1.),(1.,1.),(1.,
1.),(1.,1.),(1.,1.),(1.,1.),(1.,1.),(1.,1.),(1.,1.),(1.,1.),(1.,1.),(1.,
1.),(1.,1.),(1.,1.),(1.,1.),(1.,1.),(1.,1.),(1.,1.),(1.,1.),(1.,1.),(1.,
1.),(1.,1.),(1.,1.),(1.,1.),(1.,1.),(1.,1.),(1.,1.),(1.,1.),(1.,1.),(1.,
1.),(1.,1.),(1.,1.),(1.,1.),(1.,1.),(1.,1.),(1.,1.),(1.,1.),(1.,1.),(1.,
1.),(1.,1.),(1.,1.),(1.,1.),(1.,1.),(1.,1.),(1.,1.),(1.,1.),(1.,1.),(1.,
1.),(1.,1.)))
REPRESENTATION_ITEM('')
SURFACE()
);
#1053=(
BOUNDED_SURFACE()
B_SPLINE_SURFACE(5,1,((#201699,#201700),(#201701,#201702),(#201703,#201704),
(#201705,#201706),(#201707,#201708),(#201709,#201710),(#201711,#201712),
(#201713,#201714),(#201715,#201716),(#201717,#201718),(#201719,#201720),
(#201721,#201722),(#201723,#201724),(#201725,#201726),(#201727,#201728),
(#201729,#201730),(#201731,#201732),(#201733,#201734),(#201735,#201736),
(#201737,#201738),(#201739,#201740),(#201741,#201742),(#201743,#201744),
(#201745,#201746),(#201747,#201748),(#201749,#201750),(#201751,#201752),
(#201753,#201754),(#201755,#201756),(#201757,#201758),(#201759,#201760),
(#201761,#201762),(#201763,#201764),(#201765,#201766),(#201767,#201768),
(#201769,#201770),(#201771,#201772),(#201773,#201774),(#201775,#201776),
(#201777,#201778),(#201779,#201780),(#201781,#201782),(#201783,#201784),
(#201785,#201786),(#201787,#201788),(#201789,#201790),(#201791,#201792),
(#201793,#201794),(#201795,#201796),(#201797,#201798),(#201799,#201800),
(#201801,#201802),(#201803,#201804),(#201805,#201806),(#201807,#201808),
(#201809,#201810),(#201811,#201812),(#201813,#201814),(#201815,#201816),
(#201817,#201818),(#201819,#201820),(#201821,#201822),(#201823,#201824),
(#201825,#201826),(#201827,#201828),(#201829,#201830),(#201831,#201832),
(#201833,#201834),(#201835,#201836),(#201837,#201838),(#201839,#201840),
(#201841,#201842),(#201843,#201844),(#201845,#201846),(#201847,#201848),
(#201849,#201850),(#201851,#201852),(#201853,#201854),(#201855,#201856),
(#201857,#201858),(#201859,#201860),(#201861,#201862),(#201863,#201864),
(#201865,#201866),(#201867,#201868),(#201869,#201870),(#201871,#201872),
(#201873,#201874),(#201875,#201876),(#201877,#201878),(#201879,#201880),
(#201881,#201882),(#201883,#201884),(#201885,#201886),(#201887,#201888),
(#201889,#201890),(#201891,#201892),(#201893,#201894),(#201895,#201896),
(#201897,#201898),(#201899,#201900),(#201901,#201902),(#201903,#201904),
(#201905,#201906),(#201907,#201908),(#201909,#201910),(#201911,#201912),
(#201913,#201914),(#201915,#201916),(#201917,#201918),(#201919,#201920),
(#201921,#201922),(#201923,#201924),(#201925,#201926),(#201927,#201928),
(#201929,#201930),(#201931,#201932),(#201933,#201934),(#201935,#201936),
(#201937,#201938),(#201939,#201940),(#201941,#201942),(#201943,#201944),
(#201945,#201946),(#201947,#201948),(#201949,#201950),(#201951,#201952),
(#201953,#201954),(#201955,#201956),(#201957,#201958),(#201959,#201960),
(#201961,#201962),(#201963,#201964),(#201965,#201966),(#201967,#201968),
(#201969,#201970),(#201971,#201972),(#201973,#201974),(#201975,#201976),
(#201977,#201978),(#201979,#201980),(#201981,#201982),(#201983,#201984),
(#201985,#201986),(#201987,#201988),(#201989,#201990),(#201991,#201992),
(#201993,#201994),(#201995,#201996),(#201997,#201998),(#201999,#202000),
(#202001,#202002),(#202003,#202004),(#202005,#202006),(#202007,#202008),
(#202009,#202010),(#202011,#202012),(#202013,#202014),(#202015,#202016),
(#202017,#202018),(#202019,#202020),(#202021,#202022),(#202023,#202024),
(#202025,#202026),(#202027,#202028),(#202029,#202030),(#202031,#202032),
(#202033,#202034),(#202035,#202036),(#202037,#202038),(#202039,#202040),
(#202041,#202042),(#202043,#202044),(#202045,#202046),(#202047,#202048),
(#202049,#202050),(#202051,#202052),(#202053,#202054),(#202055,#202056),
(#202057,#202058),(#202059,#202060),(#202061,#202062),(#202063,#202064),
(#202065,#202066),(#202067,#202068),(#202069,#202070),(#202071,#202072),
(#202073,#202074),(#202075,#202076),(#202077,#202078),(#202079,#202080),
(#202081,#202082),(#202083,#202084),(#202085,#202086),(#202087,#202088),
(#202089,#202090),(#202091,#202092),(#202093,#202094),(#202095,#202096),
(#202097,#202098),(#202099,#202100),(#202101,#202102),(#202103,#202104),
(#202105,#202106),(#202107,#202108)),.UNSPECIFIED.,.F.,.F.,.F.)
B_SPLINE_SURFACE_WITH_KNOTS((6,1,1,1,1,1,1,1,1,1,1,1,1,1,1,1,1,1,1,1,1,
1,1,1,1,1,1,1,1,1,1,1,1,1,1,1,1,1,1,1,1,1,1,1,1,1,1,1,1,1,1,1,1,1,1,1,1,
1,1,1,1,1,1,1,1,1,1,1,1,1,1,1,1,1,1,1,1,1,1,1,1,1,1,1,1,1,1,1,1,1,1,1,1,
1,1,1,1,1,1,1,1,1,1,1,1,1,1,1,1,1,1,1,1,1,1,1,1,1,1,1,1,1,1,1,1,1,1,1,1,
1,1,1,1,1,1,1,1,1,1,1,1,1,1,1,1,1,1,1,1,1,1,1,1,1,1,1,1,1,1,1,1,1,1,1,1,
1,1,1,1,1,1,1,1,1,1,1,1,1,1,1,1,1,1,1,1,1,1,1,1,1,1,1,1,1,1,1,1,1,1,1,6),
(2,2),(-1.,-0.995000000000001,-0.990000000000001,-0.985000000000001,-0.980000000000001,
-0.975000000000001,-0.970000000000001,-0.965000000000001,-0.960000000000001,
-0.955000000000001,-0.950000000000001,-0.945000000000001,-0.940000000000001,
-0.935000000000001,-0.930000000000001,-0.925000000000001,-0.920000000000001,
-0.915000000000001,-0.910000000000001,-0.905000000000001,-0.900000000000001,
-0.895000000000001,-0.890000000000001,-0.885000000000001,-0.880000000000001,
-0.875000000000001,-0.870000000000001,-0.865000000000001,-0.860000000000001,
-0.855000000000001,-0.850000000000001,-0.845000000000001,-0.840000000000001,
-0.835000000000001,-0.830000000000001,-0.825000000000001,-0.820000000000001,
-0.815000000000001,-0.810000000000001,-0.805000000000001,-0.800000000000001,
-0.795000000000001,-0.790000000000001,-0.785000000000001,-0.780000000000001,
-0.775000000000001,-0.770000000000001,-0.765000000000001,-0.760000000000001,
-0.755000000000001,-0.750000000000001,-0.745000000000001,-0.740000000000001,
-0.735000000000001,-0.730000000000001,-0.725000000000001,-0.720000000000001,
-0.715000000000001,-0.710000000000001,-0.705000000000001,-0.700000000000001,
-0.695000000000001,-0.690000000000001,-0.685,-0.68,-0.675,-0.67,-0.665,
-0.66,-0.655,-0.65,-0.645,-0.64,-0.635,-0.63,-0.625,-0.62,-0.615,-0.61,
-0.605,-0.6,-0.595,-0.59,-0.585,-0.58,-0.575,-0.57,-0.565,-0.56,-0.555,
-0.55,-0.545,-0.54,-0.535,-0.53,-0.525,-0.52,-0.515,-0.51,-0.505,-0.5,-0.495,
-0.49,-0.485,-0.48,-0.475,-0.47,-0.465,-0.46,-0.455,-0.45,-0.445,-0.44,
-0.435,-0.43,-0.425,-0.42,-0.415,-0.41,-0.405,-0.4,-0.395,-0.39,-0.385,
-0.38,-0.375,-0.37,-0.365,-0.36,-0.355,-0.35,-0.345,-0.34,-0.335,-0.33,
-0.325,-0.32,-0.315,-0.31,-0.305,-0.3,-0.295,-0.29,-0.285,-0.28,-0.275,
-0.27,-0.265,-0.26,-0.255,-0.25,-0.245,-0.24,-0.235,-0.23,-0.225,-0.22,
-0.215,-0.21,-0.205,-0.2,-0.195,-0.19,-0.185,-0.18,-0.175,-0.17,-0.165,
-0.16,-0.155,-0.15,-0.145,-0.14,-0.135,-0.13,-0.125,-0.12,-0.115,-0.11,
-0.105,-0.1,-0.095,-0.09,-0.085,-0.08,-0.075,-0.07,-0.065,-0.06,-0.055,
-0.05,-0.045,-0.04,-0.035,-0.03,-0.025,-0.02,-0.015,-0.01,-0.005,0.),(0.,
1.2),.UNSPECIFIED.)
GEOMETRIC_REPRESENTATION_ITEM()
RATIONAL_B_SPLINE_SURFACE(((1.,1.),(1.,1.),(1.,1.),(1.,1.),(1.,1.),(1.,
1.),(1.,1.),(1.,1.),(1.,1.),(1.,1.),(1.,1.),(1.,1.),(1.,1.),(1.,1.),(1.,
1.),(1.,1.),(1.,1.),(1.,1.),(1.,1.),(1.,1.),(1.,1.),(1.,1.),(1.,1.),(1.,
1.),(1.,1.),(1.,1.),(1.,1.),(1.,1.),(1.,1.),(1.,1.),(1.,1.),(1.,1.),(1.,
1.),(1.,1.),(1.,1.),(1.,1.),(1.,1.),(1.,1.),(1.,1.),(1.,1.),(1.,1.),(1.,
1.),(1.,1.),(1.,1.),(1.,1.),(1.,1.),(1.,1.),(1.,1.),(1.,1.),(1.,1.),(1.,
1.),(1.,1.),(1.,1.),(1.,1.),(1.,1.),(1.,1.),(1.,1.),(1.,1.),(1.,1.),(1.,
1.),(1.,1.),(1.,1.),(1.,1.),(1.,1.),(1.,1.),(1.,1.),(1.,1.),(1.,1.),(1.,
1.),(1.,1.),(1.,1.),(1.,1.),(1.,1.),(1.,1.),(1.,1.),(1.,1.),(1.,1.),(1.,
1.),(1.,1.),(1.,1.),(1.,1.),(1.,1.),(1.,1.),(1.,1.),(1.,1.),(1.,1.),(1.,
1.),(1.,1.),(1.,1.),(1.,1.),(1.,1.),(1.,1.),(1.,1.),(1.,1.),(1.,1.),(1.,
1.),(1.,1.),(1.,1.),(1.,1.),(1.,1.),(1.,1.),(1.,1.),(1.,1.),(1.,1.),(1.,
1.),(1.,1.),(1.,1.),(1.,1.),(1.,1.),(1.,1.),(1.,1.),(1.,1.),(1.,1.),(1.,
1.),(1.,1.),(1.,1.),(1.,1.),(1.,1.),(1.,1.),(1.,1.),(1.,1.),(1.,1.),(1.,
1.),(1.,1.),(1.,1.),(1.,1.),(1.,1.),(1.,1.),(1.,1.),(1.,1.),(1.,1.),(1.,
1.),(1.,1.),(1.,1.),(1.,1.),(1.,1.),(1.,1.),(1.,1.),(1.,1.),(1.,1.),(1.,
1.),(1.,1.),(1.,1.),(1.,1.),(1.,1.),(1.,1.),(1.,1.),(1.,1.),(1.,1.),(1.,
1.),(1.,1.),(1.,1.),(1.,1.),(1.,1.),(1.,1.),(1.,1.),(1.,1.),(1.,1.),(1.,
1.),(1.,1.),(1.,1.),(1.,1.),(1.,1.),(1.,1.),(1.,1.),(1.,1.),(1.,1.),(1.,
1.),(1.,1.),(1.,1.),(1.,1.),(1.,1.),(1.,1.),(1.,1.),(1.,1.),(1.,1.),(1.,
1.),(1.,1.),(1.,1.),(1.,1.),(1.,1.),(1.,1.),(1.,1.),(1.,1.),(1.,1.),(1.,
1.),(1.,1.),(1.,1.),(1.,1.),(1.,1.),(1.,1.),(1.,1.),(1.,1.),(1.,1.),(1.,
1.),(1.,1.),(1.,1.),(1.,1.),(1.,1.),(1.,1.),(1.,1.),(1.,1.),(1.,1.),(1.,
1.),(1.,1.)))
REPRESENTATION_ITEM('')
SURFACE()
);
#1054=(
BOUNDED_SURFACE()
B_SPLINE_SURFACE(5,1,((#202316,#202317),(#202318,#202319),(#202320,#202321),
(#202322,#202323),(#202324,#202325),(#202326,#202327),(#202328,#202329),
(#202330,#202331),(#202332,#202333),(#202334,#202335),(#202336,#202337),
(#202338,#202339),(#202340,#202341),(#202342,#202343),(#202344,#202345),
(#202346,#202347),(#202348,#202349),(#202350,#202351),(#202352,#202353),
(#202354,#202355),(#202356,#202357),(#202358,#202359),(#202360,#202361),
(#202362,#202363),(#202364,#202365),(#202366,#202367),(#202368,#202369),
(#202370,#202371),(#202372,#202373),(#202374,#202375),(#202376,#202377),
(#202378,#202379),(#202380,#202381),(#202382,#202383),(#202384,#202385),
(#202386,#202387),(#202388,#202389),(#202390,#202391),(#202392,#202393),
(#202394,#202395),(#202396,#202397),(#202398,#202399),(#202400,#202401),
(#202402,#202403),(#202404,#202405),(#202406,#202407),(#202408,#202409),
(#202410,#202411),(#202412,#202413),(#202414,#202415),(#202416,#202417),
(#202418,#202419),(#202420,#202421),(#202422,#202423),(#202424,#202425),
(#202426,#202427),(#202428,#202429),(#202430,#202431),(#202432,#202433),
(#202434,#202435),(#202436,#202437),(#202438,#202439),(#202440,#202441),
(#202442,#202443),(#202444,#202445),(#202446,#202447),(#202448,#202449),
(#202450,#202451),(#202452,#202453),(#202454,#202455),(#202456,#202457),
(#202458,#202459),(#202460,#202461),(#202462,#202463),(#202464,#202465),
(#202466,#202467),(#202468,#202469),(#202470,#202471),(#202472,#202473),
(#202474,#202475),(#202476,#202477),(#202478,#202479),(#202480,#202481),
(#202482,#202483),(#202484,#202485),(#202486,#202487),(#202488,#202489),
(#202490,#202491),(#202492,#202493),(#202494,#202495),(#202496,#202497),
(#202498,#202499),(#202500,#202501),(#202502,#202503),(#202504,#202505),
(#202506,#202507),(#202508,#202509),(#202510,#202511),(#202512,#202513),
(#202514,#202515),(#202516,#202517),(#202518,#202519),(#202520,#202521),
(#202522,#202523),(#202524,#202525),(#202526,#202527),(#202528,#202529),
(#202530,#202531),(#202532,#202533),(#202534,#202535),(#202536,#202537),
(#202538,#202539),(#202540,#202541),(#202542,#202543),(#202544,#202545),
(#202546,#202547),(#202548,#202549),(#202550,#202551),(#202552,#202553),
(#202554,#202555),(#202556,#202557),(#202558,#202559),(#202560,#202561),
(#202562,#202563),(#202564,#202565),(#202566,#202567),(#202568,#202569),
(#202570,#202571),(#202572,#202573),(#202574,#202575),(#202576,#202577),
(#202578,#202579),(#202580,#202581),(#202582,#202583),(#202584,#202585),
(#202586,#202587),(#202588,#202589),(#202590,#202591),(#202592,#202593),
(#202594,#202595),(#202596,#202597),(#202598,#202599),(#202600,#202601),
(#202602,#202603),(#202604,#202605),(#202606,#202607),(#202608,#202609),
(#202610,#202611),(#202612,#202613),(#202614,#202615),(#202616,#202617),
(#202618,#202619),(#202620,#202621),(#202622,#202623),(#202624,#202625),
(#202626,#202627),(#202628,#202629),(#202630,#202631),(#202632,#202633),
(#202634,#202635),(#202636,#202637),(#202638,#202639),(#202640,#202641),
(#202642,#202643),(#202644,#202645),(#202646,#202647),(#202648,#202649),
(#202650,#202651),(#202652,#202653),(#202654,#202655),(#202656,#202657),
(#202658,#202659),(#202660,#202661),(#202662,#202663),(#202664,#202665),
(#202666,#202667),(#202668,#202669),(#202670,#202671),(#202672,#202673),
(#202674,#202675),(#202676,#202677),(#202678,#202679),(#202680,#202681),
(#202682,#202683),(#202684,#202685),(#202686,#202687),(#202688,#202689),
(#202690,#202691),(#202692,#202693),(#202694,#202695),(#202696,#202697),
(#202698,#202699),(#202700,#202701),(#202702,#202703),(#202704,#202705),
(#202706,#202707),(#202708,#202709),(#202710,#202711),(#202712,#202713),
(#202714,#202715),(#202716,#202717),(#202718,#202719),(#202720,#202721),
(#202722,#202723),(#202724,#202725)),.UNSPECIFIED.,.F.,.F.,.F.)
B_SPLINE_SURFACE_WITH_KNOTS((6,1,1,1,1,1,1,1,1,1,1,1,1,1,1,1,1,1,1,1,1,
1,1,1,1,1,1,1,1,1,1,1,1,1,1,1,1,1,1,1,1,1,1,1,1,1,1,1,1,1,1,1,1,1,1,1,1,
1,1,1,1,1,1,1,1,1,1,1,1,1,1,1,1,1,1,1,1,1,1,1,1,1,1,1,1,1,1,1,1,1,1,1,1,
1,1,1,1,1,1,1,1,1,1,1,1,1,1,1,1,1,1,1,1,1,1,1,1,1,1,1,1,1,1,1,1,1,1,1,1,
1,1,1,1,1,1,1,1,1,1,1,1,1,1,1,1,1,1,1,1,1,1,1,1,1,1,1,1,1,1,1,1,1,1,1,1,
1,1,1,1,1,1,1,1,1,1,1,1,1,1,1,1,1,1,1,1,1,1,1,1,1,1,1,1,1,1,1,1,1,1,1,6),
(2,2),(0.,0.005,0.01,0.015,0.02,0.025,0.03,0.035,0.04,0.045,0.05,0.055,
0.06,0.065,0.07,0.075,0.08,0.085,0.09,0.095,0.1,0.105,0.11,0.115,0.12,0.125,
0.13,0.135,0.14,0.145,0.15,0.155,0.16,0.165,0.17,0.175,0.18,0.185,0.19,
0.195,0.2,0.205,0.21,0.215,0.22,0.225,0.23,0.235,0.24,0.245,0.25,0.255,
0.26,0.265,0.27,0.275,0.28,0.285,0.29,0.295,0.3,0.305,0.31,0.315,0.32,0.325,
0.33,0.335,0.34,0.345,0.35,0.355,0.36,0.365,0.37,0.375,0.38,0.385,0.39,
0.395,0.4,0.405,0.41,0.415,0.42,0.425,0.43,0.435,0.44,0.445,0.45,0.455,
0.46,0.465,0.47,0.475,0.48,0.485,0.49,0.495,0.5,0.505,0.51,0.515,0.52,0.525,
0.53,0.535,0.54,0.545,0.55,0.555,0.56,0.565,0.57,0.575,0.58,0.585,0.59,
0.595,0.6,0.605,0.61,0.615,0.62,0.625,0.63,0.635,0.64,0.645,0.65,0.655,
0.66,0.665,0.67,0.675,0.68,0.685,0.690000000000001,0.695000000000001,0.700000000000001,
0.705000000000001,0.710000000000001,0.715000000000001,0.720000000000001,
0.725000000000001,0.730000000000001,0.735000000000001,0.740000000000001,
0.745000000000001,0.750000000000001,0.755000000000001,0.760000000000001,
0.765000000000001,0.770000000000001,0.775000000000001,0.780000000000001,
0.785000000000001,0.790000000000001,0.795000000000001,0.800000000000001,
0.805000000000001,0.810000000000001,0.815000000000001,0.820000000000001,
0.825000000000001,0.830000000000001,0.835000000000001,0.840000000000001,
0.845000000000001,0.850000000000001,0.855000000000001,0.860000000000001,
0.865000000000001,0.870000000000001,0.875000000000001,0.880000000000001,
0.885000000000001,0.890000000000001,0.895000000000001,0.900000000000001,
0.905000000000001,0.910000000000001,0.915000000000001,0.920000000000001,
0.925000000000001,0.930000000000001,0.935000000000001,0.940000000000001,
0.945000000000001,0.950000000000001,0.955000000000001,0.960000000000001,
0.965000000000001,0.970000000000001,0.975000000000001,0.980000000000001,
0.985000000000001,0.990000000000001,0.995000000000001,1.),(0.,1.2),
 .UNSPECIFIED.)
GEOMETRIC_REPRESENTATION_ITEM()
RATIONAL_B_SPLINE_SURFACE(((1.,1.),(1.,1.),(1.,1.),(1.,1.),(1.,1.),(1.,
1.),(1.,1.),(1.,1.),(1.,1.),(1.,1.),(1.,1.),(1.,1.),(1.,1.),(1.,1.),(1.,
1.),(1.,1.),(1.,1.),(1.,1.),(1.,1.),(1.,1.),(1.,1.),(1.,1.),(1.,1.),(1.,
1.),(1.,1.),(1.,1.),(1.,1.),(1.,1.),(1.,1.),(1.,1.),(1.,1.),(1.,1.),(1.,
1.),(1.,1.),(1.,1.),(1.,1.),(1.,1.),(1.,1.),(1.,1.),(1.,1.),(1.,1.),(1.,
1.),(1.,1.),(1.,1.),(1.,1.),(1.,1.),(1.,1.),(1.,1.),(1.,1.),(1.,1.),(1.,
1.),(1.,1.),(1.,1.),(1.,1.),(1.,1.),(1.,1.),(1.,1.),(1.,1.),(1.,1.),(1.,
1.),(1.,1.),(1.,1.),(1.,1.),(1.,1.),(1.,1.),(1.,1.),(1.,1.),(1.,1.),(1.,
1.),(1.,1.),(1.,1.),(1.,1.),(1.,1.),(1.,1.),(1.,1.),(1.,1.),(1.,1.),(1.,
1.),(1.,1.),(1.,1.),(1.,1.),(1.,1.),(1.,1.),(1.,1.),(1.,1.),(1.,1.),(1.,
1.),(1.,1.),(1.,1.),(1.,1.),(1.,1.),(1.,1.),(1.,1.),(1.,1.),(1.,1.),(1.,
1.),(1.,1.),(1.,1.),(1.,1.),(1.,1.),(1.,1.),(1.,1.),(1.,1.),(1.,1.),(1.,
1.),(1.,1.),(1.,1.),(1.,1.),(1.,1.),(1.,1.),(1.,1.),(1.,1.),(1.,1.),(1.,
1.),(1.,1.),(1.,1.),(1.,1.),(1.,1.),(1.,1.),(1.,1.),(1.,1.),(1.,1.),(1.,
1.),(1.,1.),(1.,1.),(1.,1.),(1.,1.),(1.,1.),(1.,1.),(1.,1.),(1.,1.),(1.,
1.),(1.,1.),(1.,1.),(1.,1.),(1.,1.),(1.,1.),(1.,1.),(1.,1.),(1.,1.),(1.,
1.),(1.,1.),(1.,1.),(1.,1.),(1.,1.),(1.,1.),(1.,1.),(1.,1.),(1.,1.),(1.,
1.),(1.,1.),(1.,1.),(1.,1.),(1.,1.),(1.,1.),(1.,1.),(1.,1.),(1.,1.),(1.,
1.),(1.,1.),(1.,1.),(1.,1.),(1.,1.),(1.,1.),(1.,1.),(1.,1.),(1.,1.),(1.,
1.),(1.,1.),(1.,1.),(1.,1.),(1.,1.),(1.,1.),(1.,1.),(1.,1.),(1.,1.),(1.,
1.),(1.,1.),(1.,1.),(1.,1.),(1.,1.),(1.,1.),(1.,1.),(1.,1.),(1.,1.),(1.,
1.),(1.,1.),(1.,1.),(1.,1.),(1.,1.),(1.,1.),(1.,1.),(1.,1.),(1.,1.),(1.,
1.),(1.,1.),(1.,1.),(1.,1.),(1.,1.),(1.,1.),(1.,1.),(1.,1.),(1.,1.),(1.,
1.),(1.,1.)))
REPRESENTATION_ITEM('')
SURFACE()
);
#1055=(
BOUNDED_SURFACE()
B_SPLINE_SURFACE(5,1,((#202937,#202938),(#202939,#202940),(#202941,#202942),
(#202943,#202944),(#202945,#202946),(#202947,#202948),(#202949,#202950),
(#202951,#202952),(#202953,#202954),(#202955,#202956),(#202957,#202958),
(#202959,#202960),(#202961,#202962),(#202963,#202964),(#202965,#202966),
(#202967,#202968),(#202969,#202970),(#202971,#202972),(#202973,#202974),
(#202975,#202976),(#202977,#202978),(#202979,#202980),(#202981,#202982),
(#202983,#202984),(#202985,#202986),(#202987,#202988),(#202989,#202990),
(#202991,#202992),(#202993,#202994),(#202995,#202996),(#202997,#202998),
(#202999,#203000),(#203001,#203002),(#203003,#203004),(#203005,#203006),
(#203007,#203008),(#203009,#203010),(#203011,#203012),(#203013,#203014),
(#203015,#203016),(#203017,#203018),(#203019,#203020),(#203021,#203022),
(#203023,#203024),(#203025,#203026),(#203027,#203028),(#203029,#203030),
(#203031,#203032),(#203033,#203034),(#203035,#203036),(#203037,#203038),
(#203039,#203040),(#203041,#203042),(#203043,#203044),(#203045,#203046),
(#203047,#203048),(#203049,#203050),(#203051,#203052),(#203053,#203054),
(#203055,#203056),(#203057,#203058),(#203059,#203060),(#203061,#203062),
(#203063,#203064),(#203065,#203066),(#203067,#203068),(#203069,#203070),
(#203071,#203072),(#203073,#203074),(#203075,#203076),(#203077,#203078),
(#203079,#203080),(#203081,#203082),(#203083,#203084),(#203085,#203086),
(#203087,#203088),(#203089,#203090),(#203091,#203092),(#203093,#203094),
(#203095,#203096),(#203097,#203098),(#203099,#203100),(#203101,#203102),
(#203103,#203104),(#203105,#203106),(#203107,#203108),(#203109,#203110),
(#203111,#203112),(#203113,#203114),(#203115,#203116),(#203117,#203118),
(#203119,#203120),(#203121,#203122),(#203123,#203124),(#203125,#203126),
(#203127,#203128),(#203129,#203130),(#203131,#203132),(#203133,#203134),
(#203135,#203136),(#203137,#203138),(#203139,#203140),(#203141,#203142),
(#203143,#203144),(#203145,#203146),(#203147,#203148),(#203149,#203150),
(#203151,#203152),(#203153,#203154),(#203155,#203156),(#203157,#203158),
(#203159,#203160),(#203161,#203162),(#203163,#203164),(#203165,#203166),
(#203167,#203168),(#203169,#203170),(#203171,#203172),(#203173,#203174),
(#203175,#203176),(#203177,#203178),(#203179,#203180),(#203181,#203182),
(#203183,#203184),(#203185,#203186),(#203187,#203188),(#203189,#203190),
(#203191,#203192),(#203193,#203194),(#203195,#203196),(#203197,#203198),
(#203199,#203200),(#203201,#203202),(#203203,#203204),(#203205,#203206),
(#203207,#203208),(#203209,#203210),(#203211,#203212),(#203213,#203214),
(#203215,#203216),(#203217,#203218),(#203219,#203220),(#203221,#203222),
(#203223,#203224),(#203225,#203226),(#203227,#203228),(#203229,#203230),
(#203231,#203232),(#203233,#203234),(#203235,#203236),(#203237,#203238),
(#203239,#203240),(#203241,#203242),(#203243,#203244),(#203245,#203246),
(#203247,#203248),(#203249,#203250),(#203251,#203252),(#203253,#203254),
(#203255,#203256),(#203257,#203258),(#203259,#203260),(#203261,#203262),
(#203263,#203264),(#203265,#203266),(#203267,#203268),(#203269,#203270),
(#203271,#203272),(#203273,#203274),(#203275,#203276),(#203277,#203278),
(#203279,#203280),(#203281,#203282),(#203283,#203284),(#203285,#203286),
(#203287,#203288),(#203289,#203290),(#203291,#203292),(#203293,#203294),
(#203295,#203296),(#203297,#203298),(#203299,#203300),(#203301,#203302),
(#203303,#203304),(#203305,#203306),(#203307,#203308),(#203309,#203310),
(#203311,#203312),(#203313,#203314),(#203315,#203316),(#203317,#203318),
(#203319,#203320),(#203321,#203322),(#203323,#203324),(#203325,#203326),
(#203327,#203328),(#203329,#203330),(#203331,#203332),(#203333,#203334),
(#203335,#203336),(#203337,#203338),(#203339,#203340),(#203341,#203342),
(#203343,#203344),(#203345,#203346)),.UNSPECIFIED.,.F.,.F.,.F.)
B_SPLINE_SURFACE_WITH_KNOTS((6,1,1,1,1,1,1,1,1,1,1,1,1,1,1,1,1,1,1,1,1,
1,1,1,1,1,1,1,1,1,1,1,1,1,1,1,1,1,1,1,1,1,1,1,1,1,1,1,1,1,1,1,1,1,1,1,1,
1,1,1,1,1,1,1,1,1,1,1,1,1,1,1,1,1,1,1,1,1,1,1,1,1,1,1,1,1,1,1,1,1,1,1,1,
1,1,1,1,1,1,1,1,1,1,1,1,1,1,1,1,1,1,1,1,1,1,1,1,1,1,1,1,1,1,1,1,1,1,1,1,
1,1,1,1,1,1,1,1,1,1,1,1,1,1,1,1,1,1,1,1,1,1,1,1,1,1,1,1,1,1,1,1,1,1,1,1,
1,1,1,1,1,1,1,1,1,1,1,1,1,1,1,1,1,1,1,1,1,1,1,1,1,1,1,1,1,1,1,1,1,1,1,6),
(2,2),(-1.,-0.995000000000001,-0.990000000000001,-0.985000000000001,-0.980000000000001,
-0.975000000000001,-0.970000000000001,-0.965000000000001,-0.960000000000001,
-0.955000000000001,-0.950000000000001,-0.945000000000001,-0.940000000000001,
-0.935000000000001,-0.930000000000001,-0.925000000000001,-0.920000000000001,
-0.915000000000001,-0.910000000000001,-0.905000000000001,-0.900000000000001,
-0.895000000000001,-0.890000000000001,-0.885000000000001,-0.880000000000001,
-0.875000000000001,-0.870000000000001,-0.865000000000001,-0.860000000000001,
-0.855000000000001,-0.850000000000001,-0.845000000000001,-0.840000000000001,
-0.835000000000001,-0.830000000000001,-0.825000000000001,-0.820000000000001,
-0.815000000000001,-0.810000000000001,-0.805000000000001,-0.800000000000001,
-0.795000000000001,-0.790000000000001,-0.785000000000001,-0.780000000000001,
-0.775000000000001,-0.770000000000001,-0.765000000000001,-0.760000000000001,
-0.755000000000001,-0.750000000000001,-0.745000000000001,-0.740000000000001,
-0.735000000000001,-0.730000000000001,-0.725000000000001,-0.720000000000001,
-0.715000000000001,-0.710000000000001,-0.705000000000001,-0.700000000000001,
-0.695000000000001,-0.690000000000001,-0.685,-0.68,-0.675,-0.67,-0.665,
-0.66,-0.655,-0.65,-0.645,-0.64,-0.635,-0.63,-0.625,-0.62,-0.615,-0.61,
-0.605,-0.6,-0.595,-0.59,-0.585,-0.58,-0.575,-0.57,-0.565,-0.56,-0.555,
-0.55,-0.545,-0.54,-0.535,-0.53,-0.525,-0.52,-0.515,-0.51,-0.505,-0.5,-0.495,
-0.49,-0.485,-0.48,-0.475,-0.47,-0.465,-0.46,-0.455,-0.45,-0.445,-0.44,
-0.435,-0.43,-0.425,-0.42,-0.415,-0.41,-0.405,-0.4,-0.395,-0.39,-0.385,
-0.38,-0.375,-0.37,-0.365,-0.36,-0.355,-0.35,-0.345,-0.34,-0.335,-0.33,
-0.325,-0.32,-0.315,-0.31,-0.305,-0.3,-0.295,-0.29,-0.285,-0.28,-0.275,
-0.27,-0.265,-0.26,-0.255,-0.25,-0.245,-0.24,-0.235,-0.23,-0.225,-0.22,
-0.215,-0.21,-0.205,-0.2,-0.195,-0.19,-0.185,-0.18,-0.175,-0.17,-0.165,
-0.16,-0.155,-0.15,-0.145,-0.14,-0.135,-0.13,-0.125,-0.12,-0.115,-0.11,
-0.105,-0.1,-0.095,-0.09,-0.085,-0.08,-0.075,-0.07,-0.065,-0.06,-0.055,
-0.05,-0.045,-0.04,-0.035,-0.03,-0.025,-0.02,-0.015,-0.01,-0.005,0.),(0.,
1.2),.UNSPECIFIED.)
GEOMETRIC_REPRESENTATION_ITEM()
RATIONAL_B_SPLINE_SURFACE(((1.,1.),(1.,1.),(1.,1.),(1.,1.),(1.,1.),(1.,
1.),(1.,1.),(1.,1.),(1.,1.),(1.,1.),(1.,1.),(1.,1.),(1.,1.),(1.,1.),(1.,
1.),(1.,1.),(1.,1.),(1.,1.),(1.,1.),(1.,1.),(1.,1.),(1.,1.),(1.,1.),(1.,
1.),(1.,1.),(1.,1.),(1.,1.),(1.,1.),(1.,1.),(1.,1.),(1.,1.),(1.,1.),(1.,
1.),(1.,1.),(1.,1.),(1.,1.),(1.,1.),(1.,1.),(1.,1.),(1.,1.),(1.,1.),(1.,
1.),(1.,1.),(1.,1.),(1.,1.),(1.,1.),(1.,1.),(1.,1.),(1.,1.),(1.,1.),(1.,
1.),(1.,1.),(1.,1.),(1.,1.),(1.,1.),(1.,1.),(1.,1.),(1.,1.),(1.,1.),(1.,
1.),(1.,1.),(1.,1.),(1.,1.),(1.,1.),(1.,1.),(1.,1.),(1.,1.),(1.,1.),(1.,
1.),(1.,1.),(1.,1.),(1.,1.),(1.,1.),(1.,1.),(1.,1.),(1.,1.),(1.,1.),(1.,
1.),(1.,1.),(1.,1.),(1.,1.),(1.,1.),(1.,1.),(1.,1.),(1.,1.),(1.,1.),(1.,
1.),(1.,1.),(1.,1.),(1.,1.),(1.,1.),(1.,1.),(1.,1.),(1.,1.),(1.,1.),(1.,
1.),(1.,1.),(1.,1.),(1.,1.),(1.,1.),(1.,1.),(1.,1.),(1.,1.),(1.,1.),(1.,
1.),(1.,1.),(1.,1.),(1.,1.),(1.,1.),(1.,1.),(1.,1.),(1.,1.),(1.,1.),(1.,
1.),(1.,1.),(1.,1.),(1.,1.),(1.,1.),(1.,1.),(1.,1.),(1.,1.),(1.,1.),(1.,
1.),(1.,1.),(1.,1.),(1.,1.),(1.,1.),(1.,1.),(1.,1.),(1.,1.),(1.,1.),(1.,
1.),(1.,1.),(1.,1.),(1.,1.),(1.,1.),(1.,1.),(1.,1.),(1.,1.),(1.,1.),(1.,
1.),(1.,1.),(1.,1.),(1.,1.),(1.,1.),(1.,1.),(1.,1.),(1.,1.),(1.,1.),(1.,
1.),(1.,1.),(1.,1.),(1.,1.),(1.,1.),(1.,1.),(1.,1.),(1.,1.),(1.,1.),(1.,
1.),(1.,1.),(1.,1.),(1.,1.),(1.,1.),(1.,1.),(1.,1.),(1.,1.),(1.,1.),(1.,
1.),(1.,1.),(1.,1.),(1.,1.),(1.,1.),(1.,1.),(1.,1.),(1.,1.),(1.,1.),(1.,
1.),(1.,1.),(1.,1.),(1.,1.),(1.,1.),(1.,1.),(1.,1.),(1.,1.),(1.,1.),(1.,
1.),(1.,1.),(1.,1.),(1.,1.),(1.,1.),(1.,1.),(1.,1.),(1.,1.),(1.,1.),(1.,
1.),(1.,1.),(1.,1.),(1.,1.),(1.,1.),(1.,1.),(1.,1.),(1.,1.),(1.,1.),(1.,
1.),(1.,1.)))
REPRESENTATION_ITEM('')
SURFACE()
);
#1056=(
BOUNDED_SURFACE()
B_SPLINE_SURFACE(5,1,((#203554,#203555),(#203556,#203557),(#203558,#203559),
(#203560,#203561),(#203562,#203563),(#203564,#203565),(#203566,#203567),
(#203568,#203569),(#203570,#203571),(#203572,#203573),(#203574,#203575),
(#203576,#203577),(#203578,#203579),(#203580,#203581),(#203582,#203583),
(#203584,#203585),(#203586,#203587),(#203588,#203589),(#203590,#203591),
(#203592,#203593),(#203594,#203595),(#203596,#203597),(#203598,#203599),
(#203600,#203601),(#203602,#203603),(#203604,#203605),(#203606,#203607),
(#203608,#203609),(#203610,#203611),(#203612,#203613),(#203614,#203615),
(#203616,#203617),(#203618,#203619),(#203620,#203621),(#203622,#203623),
(#203624,#203625),(#203626,#203627),(#203628,#203629),(#203630,#203631),
(#203632,#203633),(#203634,#203635),(#203636,#203637),(#203638,#203639),
(#203640,#203641),(#203642,#203643),(#203644,#203645),(#203646,#203647),
(#203648,#203649),(#203650,#203651),(#203652,#203653),(#203654,#203655),
(#203656,#203657),(#203658,#203659),(#203660,#203661),(#203662,#203663),
(#203664,#203665),(#203666,#203667),(#203668,#203669),(#203670,#203671),
(#203672,#203673),(#203674,#203675),(#203676,#203677),(#203678,#203679),
(#203680,#203681),(#203682,#203683),(#203684,#203685),(#203686,#203687),
(#203688,#203689),(#203690,#203691),(#203692,#203693),(#203694,#203695),
(#203696,#203697),(#203698,#203699),(#203700,#203701),(#203702,#203703),
(#203704,#203705),(#203706,#203707),(#203708,#203709),(#203710,#203711),
(#203712,#203713),(#203714,#203715),(#203716,#203717),(#203718,#203719),
(#203720,#203721),(#203722,#203723),(#203724,#203725),(#203726,#203727),
(#203728,#203729),(#203730,#203731),(#203732,#203733),(#203734,#203735),
(#203736,#203737),(#203738,#203739),(#203740,#203741),(#203742,#203743),
(#203744,#203745),(#203746,#203747),(#203748,#203749),(#203750,#203751),
(#203752,#203753),(#203754,#203755),(#203756,#203757),(#203758,#203759),
(#203760,#203761),(#203762,#203763),(#203764,#203765),(#203766,#203767),
(#203768,#203769),(#203770,#203771),(#203772,#203773),(#203774,#203775),
(#203776,#203777),(#203778,#203779),(#203780,#203781),(#203782,#203783),
(#203784,#203785),(#203786,#203787),(#203788,#203789),(#203790,#203791),
(#203792,#203793),(#203794,#203795),(#203796,#203797),(#203798,#203799),
(#203800,#203801),(#203802,#203803),(#203804,#203805),(#203806,#203807),
(#203808,#203809),(#203810,#203811),(#203812,#203813),(#203814,#203815),
(#203816,#203817),(#203818,#203819),(#203820,#203821),(#203822,#203823),
(#203824,#203825),(#203826,#203827),(#203828,#203829),(#203830,#203831),
(#203832,#203833),(#203834,#203835),(#203836,#203837),(#203838,#203839),
(#203840,#203841),(#203842,#203843),(#203844,#203845),(#203846,#203847),
(#203848,#203849),(#203850,#203851),(#203852,#203853),(#203854,#203855),
(#203856,#203857),(#203858,#203859),(#203860,#203861),(#203862,#203863),
(#203864,#203865),(#203866,#203867),(#203868,#203869),(#203870,#203871),
(#203872,#203873),(#203874,#203875),(#203876,#203877),(#203878,#203879),
(#203880,#203881),(#203882,#203883),(#203884,#203885),(#203886,#203887),
(#203888,#203889),(#203890,#203891),(#203892,#203893),(#203894,#203895),
(#203896,#203897),(#203898,#203899),(#203900,#203901),(#203902,#203903),
(#203904,#203905),(#203906,#203907),(#203908,#203909),(#203910,#203911),
(#203912,#203913),(#203914,#203915),(#203916,#203917),(#203918,#203919),
(#203920,#203921),(#203922,#203923),(#203924,#203925),(#203926,#203927),
(#203928,#203929),(#203930,#203931),(#203932,#203933),(#203934,#203935),
(#203936,#203937),(#203938,#203939),(#203940,#203941),(#203942,#203943),
(#203944,#203945),(#203946,#203947),(#203948,#203949),(#203950,#203951),
(#203952,#203953),(#203954,#203955),(#203956,#203957),(#203958,#203959),
(#203960,#203961),(#203962,#203963)),.UNSPECIFIED.,.F.,.F.,.F.)
B_SPLINE_SURFACE_WITH_KNOTS((6,1,1,1,1,1,1,1,1,1,1,1,1,1,1,1,1,1,1,1,1,
1,1,1,1,1,1,1,1,1,1,1,1,1,1,1,1,1,1,1,1,1,1,1,1,1,1,1,1,1,1,1,1,1,1,1,1,
1,1,1,1,1,1,1,1,1,1,1,1,1,1,1,1,1,1,1,1,1,1,1,1,1,1,1,1,1,1,1,1,1,1,1,1,
1,1,1,1,1,1,1,1,1,1,1,1,1,1,1,1,1,1,1,1,1,1,1,1,1,1,1,1,1,1,1,1,1,1,1,1,
1,1,1,1,1,1,1,1,1,1,1,1,1,1,1,1,1,1,1,1,1,1,1,1,1,1,1,1,1,1,1,1,1,1,1,1,
1,1,1,1,1,1,1,1,1,1,1,1,1,1,1,1,1,1,1,1,1,1,1,1,1,1,1,1,1,1,1,1,1,1,1,6),
(2,2),(0.,0.005,0.01,0.015,0.02,0.025,0.03,0.035,0.04,0.045,0.05,0.055,
0.06,0.065,0.07,0.075,0.08,0.085,0.09,0.095,0.1,0.105,0.11,0.115,0.12,0.125,
0.13,0.135,0.14,0.145,0.15,0.155,0.16,0.165,0.17,0.175,0.18,0.185,0.19,
0.195,0.2,0.205,0.21,0.215,0.22,0.225,0.23,0.235,0.24,0.245,0.25,0.255,
0.26,0.265,0.27,0.275,0.28,0.285,0.29,0.295,0.3,0.305,0.31,0.315,0.32,0.325,
0.33,0.335,0.34,0.345,0.35,0.355,0.36,0.365,0.37,0.375,0.38,0.385,0.39,
0.395,0.4,0.405,0.41,0.415,0.42,0.425,0.43,0.435,0.44,0.445,0.45,0.455,
0.46,0.465,0.47,0.475,0.48,0.485,0.49,0.495,0.5,0.505,0.51,0.515,0.52,0.525,
0.53,0.535,0.54,0.545,0.55,0.555,0.56,0.565,0.57,0.575,0.58,0.585,0.59,
0.595,0.6,0.605,0.61,0.615,0.62,0.625,0.63,0.635,0.64,0.645,0.65,0.655,
0.66,0.665,0.67,0.675,0.68,0.685,0.690000000000001,0.695000000000001,0.700000000000001,
0.705000000000001,0.710000000000001,0.715000000000001,0.720000000000001,
0.725000000000001,0.730000000000001,0.735000000000001,0.740000000000001,
0.745000000000001,0.750000000000001,0.755000000000001,0.760000000000001,
0.765000000000001,0.770000000000001,0.775000000000001,0.780000000000001,
0.785000000000001,0.790000000000001,0.795000000000001,0.800000000000001,
0.805000000000001,0.810000000000001,0.815000000000001,0.820000000000001,
0.825000000000001,0.830000000000001,0.835000000000001,0.840000000000001,
0.845000000000001,0.850000000000001,0.855000000000001,0.860000000000001,
0.865000000000001,0.870000000000001,0.875000000000001,0.880000000000001,
0.885000000000001,0.890000000000001,0.895000000000001,0.900000000000001,
0.905000000000001,0.910000000000001,0.915000000000001,0.920000000000001,
0.925000000000001,0.930000000000001,0.935000000000001,0.940000000000001,
0.945000000000001,0.950000000000001,0.955000000000001,0.960000000000001,
0.965000000000001,0.970000000000001,0.975000000000001,0.980000000000001,
0.985000000000001,0.990000000000001,0.995000000000001,1.),(0.,1.2),
 .UNSPECIFIED.)
GEOMETRIC_REPRESENTATION_ITEM()
RATIONAL_B_SPLINE_SURFACE(((1.,1.),(1.,1.),(1.,1.),(1.,1.),(1.,1.),(1.,
1.),(1.,1.),(1.,1.),(1.,1.),(1.,1.),(1.,1.),(1.,1.),(1.,1.),(1.,1.),(1.,
1.),(1.,1.),(1.,1.),(1.,1.),(1.,1.),(1.,1.),(1.,1.),(1.,1.),(1.,1.),(1.,
1.),(1.,1.),(1.,1.),(1.,1.),(1.,1.),(1.,1.),(1.,1.),(1.,1.),(1.,1.),(1.,
1.),(1.,1.),(1.,1.),(1.,1.),(1.,1.),(1.,1.),(1.,1.),(1.,1.),(1.,1.),(1.,
1.),(1.,1.),(1.,1.),(1.,1.),(1.,1.),(1.,1.),(1.,1.),(1.,1.),(1.,1.),(1.,
1.),(1.,1.),(1.,1.),(1.,1.),(1.,1.),(1.,1.),(1.,1.),(1.,1.),(1.,1.),(1.,
1.),(1.,1.),(1.,1.),(1.,1.),(1.,1.),(1.,1.),(1.,1.),(1.,1.),(1.,1.),(1.,
1.),(1.,1.),(1.,1.),(1.,1.),(1.,1.),(1.,1.),(1.,1.),(1.,1.),(1.,1.),(1.,
1.),(1.,1.),(1.,1.),(1.,1.),(1.,1.),(1.,1.),(1.,1.),(1.,1.),(1.,1.),(1.,
1.),(1.,1.),(1.,1.),(1.,1.),(1.,1.),(1.,1.),(1.,1.),(1.,1.),(1.,1.),(1.,
1.),(1.,1.),(1.,1.),(1.,1.),(1.,1.),(1.,1.),(1.,1.),(1.,1.),(1.,1.),(1.,
1.),(1.,1.),(1.,1.),(1.,1.),(1.,1.),(1.,1.),(1.,1.),(1.,1.),(1.,1.),(1.,
1.),(1.,1.),(1.,1.),(1.,1.),(1.,1.),(1.,1.),(1.,1.),(1.,1.),(1.,1.),(1.,
1.),(1.,1.),(1.,1.),(1.,1.),(1.,1.),(1.,1.),(1.,1.),(1.,1.),(1.,1.),(1.,
1.),(1.,1.),(1.,1.),(1.,1.),(1.,1.),(1.,1.),(1.,1.),(1.,1.),(1.,1.),(1.,
1.),(1.,1.),(1.,1.),(1.,1.),(1.,1.),(1.,1.),(1.,1.),(1.,1.),(1.,1.),(1.,
1.),(1.,1.),(1.,1.),(1.,1.),(1.,1.),(1.,1.),(1.,1.),(1.,1.),(1.,1.),(1.,
1.),(1.,1.),(1.,1.),(1.,1.),(1.,1.),(1.,1.),(1.,1.),(1.,1.),(1.,1.),(1.,
1.),(1.,1.),(1.,1.),(1.,1.),(1.,1.),(1.,1.),(1.,1.),(1.,1.),(1.,1.),(1.,
1.),(1.,1.),(1.,1.),(1.,1.),(1.,1.),(1.,1.),(1.,1.),(1.,1.),(1.,1.),(1.,
1.),(1.,1.),(1.,1.),(1.,1.),(1.,1.),(1.,1.),(1.,1.),(1.,1.),(1.,1.),(1.,
1.),(1.,1.),(1.,1.),(1.,1.),(1.,1.),(1.,1.),(1.,1.),(1.,1.),(1.,1.),(1.,
1.),(1.,1.)))
REPRESENTATION_ITEM('')
SURFACE()
);
#1057=(
BOUNDED_SURFACE()
B_SPLINE_SURFACE(5,1,((#204175,#204176),(#204177,#204178),(#204179,#204180),
(#204181,#204182),(#204183,#204184),(#204185,#204186),(#204187,#204188),
(#204189,#204190),(#204191,#204192),(#204193,#204194),(#204195,#204196),
(#204197,#204198),(#204199,#204200),(#204201,#204202),(#204203,#204204),
(#204205,#204206),(#204207,#204208),(#204209,#204210),(#204211,#204212),
(#204213,#204214),(#204215,#204216),(#204217,#204218),(#204219,#204220),
(#204221,#204222),(#204223,#204224),(#204225,#204226),(#204227,#204228),
(#204229,#204230),(#204231,#204232),(#204233,#204234),(#204235,#204236),
(#204237,#204238),(#204239,#204240),(#204241,#204242),(#204243,#204244),
(#204245,#204246),(#204247,#204248),(#204249,#204250),(#204251,#204252),
(#204253,#204254),(#204255,#204256),(#204257,#204258),(#204259,#204260),
(#204261,#204262),(#204263,#204264),(#204265,#204266),(#204267,#204268),
(#204269,#204270),(#204271,#204272),(#204273,#204274),(#204275,#204276),
(#204277,#204278),(#204279,#204280),(#204281,#204282),(#204283,#204284),
(#204285,#204286),(#204287,#204288),(#204289,#204290),(#204291,#204292),
(#204293,#204294),(#204295,#204296),(#204297,#204298),(#204299,#204300),
(#204301,#204302),(#204303,#204304),(#204305,#204306),(#204307,#204308),
(#204309,#204310),(#204311,#204312),(#204313,#204314),(#204315,#204316),
(#204317,#204318),(#204319,#204320),(#204321,#204322),(#204323,#204324),
(#204325,#204326),(#204327,#204328),(#204329,#204330),(#204331,#204332),
(#204333,#204334),(#204335,#204336),(#204337,#204338),(#204339,#204340),
(#204341,#204342),(#204343,#204344),(#204345,#204346),(#204347,#204348),
(#204349,#204350),(#204351,#204352),(#204353,#204354),(#204355,#204356),
(#204357,#204358),(#204359,#204360),(#204361,#204362),(#204363,#204364),
(#204365,#204366),(#204367,#204368),(#204369,#204370),(#204371,#204372),
(#204373,#204374),(#204375,#204376),(#204377,#204378),(#204379,#204380),
(#204381,#204382),(#204383,#204384),(#204385,#204386),(#204387,#204388),
(#204389,#204390),(#204391,#204392),(#204393,#204394),(#204395,#204396),
(#204397,#204398),(#204399,#204400),(#204401,#204402),(#204403,#204404),
(#204405,#204406),(#204407,#204408),(#204409,#204410),(#204411,#204412),
(#204413,#204414),(#204415,#204416),(#204417,#204418),(#204419,#204420),
(#204421,#204422),(#204423,#204424),(#204425,#204426),(#204427,#204428),
(#204429,#204430),(#204431,#204432),(#204433,#204434),(#204435,#204436),
(#204437,#204438),(#204439,#204440),(#204441,#204442),(#204443,#204444),
(#204445,#204446),(#204447,#204448),(#204449,#204450),(#204451,#204452),
(#204453,#204454),(#204455,#204456),(#204457,#204458),(#204459,#204460),
(#204461,#204462),(#204463,#204464),(#204465,#204466),(#204467,#204468),
(#204469,#204470),(#204471,#204472),(#204473,#204474),(#204475,#204476),
(#204477,#204478),(#204479,#204480),(#204481,#204482),(#204483,#204484),
(#204485,#204486),(#204487,#204488),(#204489,#204490),(#204491,#204492),
(#204493,#204494),(#204495,#204496),(#204497,#204498),(#204499,#204500),
(#204501,#204502),(#204503,#204504),(#204505,#204506),(#204507,#204508),
(#204509,#204510),(#204511,#204512),(#204513,#204514),(#204515,#204516),
(#204517,#204518),(#204519,#204520),(#204521,#204522),(#204523,#204524),
(#204525,#204526),(#204527,#204528),(#204529,#204530),(#204531,#204532),
(#204533,#204534),(#204535,#204536),(#204537,#204538),(#204539,#204540),
(#204541,#204542),(#204543,#204544),(#204545,#204546),(#204547,#204548),
(#204549,#204550),(#204551,#204552),(#204553,#204554),(#204555,#204556),
(#204557,#204558),(#204559,#204560),(#204561,#204562),(#204563,#204564),
(#204565,#204566),(#204567,#204568),(#204569,#204570),(#204571,#204572),
(#204573,#204574),(#204575,#204576),(#204577,#204578),(#204579,#204580),
(#204581,#204582),(#204583,#204584)),.UNSPECIFIED.,.F.,.F.,.F.)
B_SPLINE_SURFACE_WITH_KNOTS((6,1,1,1,1,1,1,1,1,1,1,1,1,1,1,1,1,1,1,1,1,
1,1,1,1,1,1,1,1,1,1,1,1,1,1,1,1,1,1,1,1,1,1,1,1,1,1,1,1,1,1,1,1,1,1,1,1,
1,1,1,1,1,1,1,1,1,1,1,1,1,1,1,1,1,1,1,1,1,1,1,1,1,1,1,1,1,1,1,1,1,1,1,1,
1,1,1,1,1,1,1,1,1,1,1,1,1,1,1,1,1,1,1,1,1,1,1,1,1,1,1,1,1,1,1,1,1,1,1,1,
1,1,1,1,1,1,1,1,1,1,1,1,1,1,1,1,1,1,1,1,1,1,1,1,1,1,1,1,1,1,1,1,1,1,1,1,
1,1,1,1,1,1,1,1,1,1,1,1,1,1,1,1,1,1,1,1,1,1,1,1,1,1,1,1,1,1,1,1,1,1,1,6),
(2,2),(-1.,-0.995000000000001,-0.990000000000001,-0.985000000000001,-0.980000000000001,
-0.975000000000001,-0.970000000000001,-0.965000000000001,-0.960000000000001,
-0.955000000000001,-0.950000000000001,-0.945000000000001,-0.940000000000001,
-0.935000000000001,-0.930000000000001,-0.925000000000001,-0.920000000000001,
-0.915000000000001,-0.910000000000001,-0.905000000000001,-0.900000000000001,
-0.895000000000001,-0.890000000000001,-0.885000000000001,-0.880000000000001,
-0.875000000000001,-0.870000000000001,-0.865000000000001,-0.860000000000001,
-0.855000000000001,-0.850000000000001,-0.845000000000001,-0.840000000000001,
-0.835000000000001,-0.830000000000001,-0.825000000000001,-0.820000000000001,
-0.815000000000001,-0.810000000000001,-0.805000000000001,-0.800000000000001,
-0.795000000000001,-0.790000000000001,-0.785000000000001,-0.780000000000001,
-0.775000000000001,-0.770000000000001,-0.765000000000001,-0.760000000000001,
-0.755000000000001,-0.750000000000001,-0.745000000000001,-0.740000000000001,
-0.735000000000001,-0.730000000000001,-0.725000000000001,-0.720000000000001,
-0.715000000000001,-0.710000000000001,-0.705000000000001,-0.700000000000001,
-0.695000000000001,-0.690000000000001,-0.685,-0.68,-0.675,-0.67,-0.665,
-0.66,-0.655,-0.65,-0.645,-0.64,-0.635,-0.63,-0.625,-0.62,-0.615,-0.61,
-0.605,-0.6,-0.595,-0.59,-0.585,-0.58,-0.575,-0.57,-0.565,-0.56,-0.555,
-0.55,-0.545,-0.54,-0.535,-0.53,-0.525,-0.52,-0.515,-0.51,-0.505,-0.5,-0.495,
-0.49,-0.485,-0.48,-0.475,-0.47,-0.465,-0.46,-0.455,-0.45,-0.445,-0.44,
-0.435,-0.43,-0.425,-0.42,-0.415,-0.41,-0.405,-0.4,-0.395,-0.39,-0.385,
-0.38,-0.375,-0.37,-0.365,-0.36,-0.355,-0.35,-0.345,-0.34,-0.335,-0.33,
-0.325,-0.32,-0.315,-0.31,-0.305,-0.3,-0.295,-0.29,-0.285,-0.28,-0.275,
-0.27,-0.265,-0.26,-0.255,-0.25,-0.245,-0.24,-0.235,-0.23,-0.225,-0.22,
-0.215,-0.21,-0.205,-0.2,-0.195,-0.19,-0.185,-0.18,-0.175,-0.17,-0.165,
-0.16,-0.155,-0.15,-0.145,-0.14,-0.135,-0.13,-0.125,-0.12,-0.115,-0.11,
-0.105,-0.1,-0.095,-0.09,-0.085,-0.08,-0.075,-0.07,-0.065,-0.06,-0.055,
-0.05,-0.045,-0.04,-0.035,-0.03,-0.025,-0.02,-0.015,-0.01,-0.005,0.),(0.,
1.2),.UNSPECIFIED.)
GEOMETRIC_REPRESENTATION_ITEM()
RATIONAL_B_SPLINE_SURFACE(((1.,1.),(1.,1.),(1.,1.),(1.,1.),(1.,1.),(1.,
1.),(1.,1.),(1.,1.),(1.,1.),(1.,1.),(1.,1.),(1.,1.),(1.,1.),(1.,1.),(1.,
1.),(1.,1.),(1.,1.),(1.,1.),(1.,1.),(1.,1.),(1.,1.),(1.,1.),(1.,1.),(1.,
1.),(1.,1.),(1.,1.),(1.,1.),(1.,1.),(1.,1.),(1.,1.),(1.,1.),(1.,1.),(1.,
1.),(1.,1.),(1.,1.),(1.,1.),(1.,1.),(1.,1.),(1.,1.),(1.,1.),(1.,1.),(1.,
1.),(1.,1.),(1.,1.),(1.,1.),(1.,1.),(1.,1.),(1.,1.),(1.,1.),(1.,1.),(1.,
1.),(1.,1.),(1.,1.),(1.,1.),(1.,1.),(1.,1.),(1.,1.),(1.,1.),(1.,1.),(1.,
1.),(1.,1.),(1.,1.),(1.,1.),(1.,1.),(1.,1.),(1.,1.),(1.,1.),(1.,1.),(1.,
1.),(1.,1.),(1.,1.),(1.,1.),(1.,1.),(1.,1.),(1.,1.),(1.,1.),(1.,1.),(1.,
1.),(1.,1.),(1.,1.),(1.,1.),(1.,1.),(1.,1.),(1.,1.),(1.,1.),(1.,1.),(1.,
1.),(1.,1.),(1.,1.),(1.,1.),(1.,1.),(1.,1.),(1.,1.),(1.,1.),(1.,1.),(1.,
1.),(1.,1.),(1.,1.),(1.,1.),(1.,1.),(1.,1.),(1.,1.),(1.,1.),(1.,1.),(1.,
1.),(1.,1.),(1.,1.),(1.,1.),(1.,1.),(1.,1.),(1.,1.),(1.,1.),(1.,1.),(1.,
1.),(1.,1.),(1.,1.),(1.,1.),(1.,1.),(1.,1.),(1.,1.),(1.,1.),(1.,1.),(1.,
1.),(1.,1.),(1.,1.),(1.,1.),(1.,1.),(1.,1.),(1.,1.),(1.,1.),(1.,1.),(1.,
1.),(1.,1.),(1.,1.),(1.,1.),(1.,1.),(1.,1.),(1.,1.),(1.,1.),(1.,1.),(1.,
1.),(1.,1.),(1.,1.),(1.,1.),(1.,1.),(1.,1.),(1.,1.),(1.,1.),(1.,1.),(1.,
1.),(1.,1.),(1.,1.),(1.,1.),(1.,1.),(1.,1.),(1.,1.),(1.,1.),(1.,1.),(1.,
1.),(1.,1.),(1.,1.),(1.,1.),(1.,1.),(1.,1.),(1.,1.),(1.,1.),(1.,1.),(1.,
1.),(1.,1.),(1.,1.),(1.,1.),(1.,1.),(1.,1.),(1.,1.),(1.,1.),(1.,1.),(1.,
1.),(1.,1.),(1.,1.),(1.,1.),(1.,1.),(1.,1.),(1.,1.),(1.,1.),(1.,1.),(1.,
1.),(1.,1.),(1.,1.),(1.,1.),(1.,1.),(1.,1.),(1.,1.),(1.,1.),(1.,1.),(1.,
1.),(1.,1.),(1.,1.),(1.,1.),(1.,1.),(1.,1.),(1.,1.),(1.,1.),(1.,1.),(1.,
1.),(1.,1.)))
REPRESENTATION_ITEM('')
SURFACE()
);
#1058=(
BOUNDED_SURFACE()
B_SPLINE_SURFACE(5,1,((#204792,#204793),(#204794,#204795),(#204796,#204797),
(#204798,#204799),(#204800,#204801),(#204802,#204803),(#204804,#204805),
(#204806,#204807),(#204808,#204809),(#204810,#204811),(#204812,#204813),
(#204814,#204815),(#204816,#204817),(#204818,#204819),(#204820,#204821),
(#204822,#204823),(#204824,#204825),(#204826,#204827),(#204828,#204829),
(#204830,#204831),(#204832,#204833),(#204834,#204835),(#204836,#204837),
(#204838,#204839),(#204840,#204841),(#204842,#204843),(#204844,#204845),
(#204846,#204847),(#204848,#204849),(#204850,#204851),(#204852,#204853),
(#204854,#204855),(#204856,#204857),(#204858,#204859),(#204860,#204861),
(#204862,#204863),(#204864,#204865),(#204866,#204867),(#204868,#204869),
(#204870,#204871),(#204872,#204873),(#204874,#204875),(#204876,#204877),
(#204878,#204879),(#204880,#204881),(#204882,#204883),(#204884,#204885),
(#204886,#204887),(#204888,#204889),(#204890,#204891),(#204892,#204893),
(#204894,#204895),(#204896,#204897),(#204898,#204899),(#204900,#204901),
(#204902,#204903),(#204904,#204905),(#204906,#204907),(#204908,#204909),
(#204910,#204911),(#204912,#204913),(#204914,#204915),(#204916,#204917),
(#204918,#204919),(#204920,#204921),(#204922,#204923),(#204924,#204925),
(#204926,#204927),(#204928,#204929),(#204930,#204931),(#204932,#204933),
(#204934,#204935),(#204936,#204937),(#204938,#204939),(#204940,#204941),
(#204942,#204943),(#204944,#204945),(#204946,#204947),(#204948,#204949),
(#204950,#204951),(#204952,#204953),(#204954,#204955),(#204956,#204957),
(#204958,#204959),(#204960,#204961),(#204962,#204963),(#204964,#204965),
(#204966,#204967),(#204968,#204969),(#204970,#204971),(#204972,#204973),
(#204974,#204975),(#204976,#204977),(#204978,#204979),(#204980,#204981),
(#204982,#204983),(#204984,#204985),(#204986,#204987),(#204988,#204989),
(#204990,#204991),(#204992,#204993),(#204994,#204995),(#204996,#204997),
(#204998,#204999),(#205000,#205001),(#205002,#205003),(#205004,#205005),
(#205006,#205007),(#205008,#205009),(#205010,#205011),(#205012,#205013),
(#205014,#205015),(#205016,#205017),(#205018,#205019),(#205020,#205021),
(#205022,#205023),(#205024,#205025),(#205026,#205027),(#205028,#205029),
(#205030,#205031),(#205032,#205033),(#205034,#205035),(#205036,#205037),
(#205038,#205039),(#205040,#205041),(#205042,#205043),(#205044,#205045),
(#205046,#205047),(#205048,#205049),(#205050,#205051),(#205052,#205053),
(#205054,#205055),(#205056,#205057),(#205058,#205059),(#205060,#205061),
(#205062,#205063),(#205064,#205065),(#205066,#205067),(#205068,#205069),
(#205070,#205071),(#205072,#205073),(#205074,#205075),(#205076,#205077),
(#205078,#205079),(#205080,#205081),(#205082,#205083),(#205084,#205085),
(#205086,#205087),(#205088,#205089),(#205090,#205091),(#205092,#205093),
(#205094,#205095),(#205096,#205097),(#205098,#205099),(#205100,#205101),
(#205102,#205103),(#205104,#205105),(#205106,#205107),(#205108,#205109),
(#205110,#205111),(#205112,#205113),(#205114,#205115),(#205116,#205117),
(#205118,#205119),(#205120,#205121),(#205122,#205123),(#205124,#205125),
(#205126,#205127),(#205128,#205129),(#205130,#205131),(#205132,#205133),
(#205134,#205135),(#205136,#205137),(#205138,#205139),(#205140,#205141),
(#205142,#205143),(#205144,#205145),(#205146,#205147),(#205148,#205149),
(#205150,#205151),(#205152,#205153),(#205154,#205155),(#205156,#205157),
(#205158,#205159),(#205160,#205161),(#205162,#205163),(#205164,#205165),
(#205166,#205167),(#205168,#205169),(#205170,#205171),(#205172,#205173),
(#205174,#205175),(#205176,#205177),(#205178,#205179),(#205180,#205181),
(#205182,#205183),(#205184,#205185),(#205186,#205187),(#205188,#205189),
(#205190,#205191),(#205192,#205193),(#205194,#205195),(#205196,#205197),
(#205198,#205199),(#205200,#205201)),.UNSPECIFIED.,.F.,.F.,.F.)
B_SPLINE_SURFACE_WITH_KNOTS((6,1,1,1,1,1,1,1,1,1,1,1,1,1,1,1,1,1,1,1,1,
1,1,1,1,1,1,1,1,1,1,1,1,1,1,1,1,1,1,1,1,1,1,1,1,1,1,1,1,1,1,1,1,1,1,1,1,
1,1,1,1,1,1,1,1,1,1,1,1,1,1,1,1,1,1,1,1,1,1,1,1,1,1,1,1,1,1,1,1,1,1,1,1,
1,1,1,1,1,1,1,1,1,1,1,1,1,1,1,1,1,1,1,1,1,1,1,1,1,1,1,1,1,1,1,1,1,1,1,1,
1,1,1,1,1,1,1,1,1,1,1,1,1,1,1,1,1,1,1,1,1,1,1,1,1,1,1,1,1,1,1,1,1,1,1,1,
1,1,1,1,1,1,1,1,1,1,1,1,1,1,1,1,1,1,1,1,1,1,1,1,1,1,1,1,1,1,1,1,1,1,1,6),
(2,2),(0.,0.005,0.01,0.015,0.02,0.025,0.03,0.035,0.04,0.045,0.05,0.055,
0.06,0.065,0.07,0.075,0.08,0.085,0.09,0.095,0.1,0.105,0.11,0.115,0.12,0.125,
0.13,0.135,0.14,0.145,0.15,0.155,0.16,0.165,0.17,0.175,0.18,0.185,0.19,
0.195,0.2,0.205,0.21,0.215,0.22,0.225,0.23,0.235,0.24,0.245,0.25,0.255,
0.26,0.265,0.27,0.275,0.28,0.285,0.29,0.295,0.3,0.305,0.31,0.315,0.32,0.325,
0.33,0.335,0.34,0.345,0.35,0.355,0.36,0.365,0.37,0.375,0.38,0.385,0.39,
0.395,0.4,0.405,0.41,0.415,0.42,0.425,0.43,0.435,0.44,0.445,0.45,0.455,
0.46,0.465,0.47,0.475,0.48,0.485,0.49,0.495,0.5,0.505,0.51,0.515,0.52,0.525,
0.53,0.535,0.54,0.545,0.55,0.555,0.56,0.565,0.57,0.575,0.58,0.585,0.59,
0.595,0.6,0.605,0.61,0.615,0.62,0.625,0.63,0.635,0.64,0.645,0.65,0.655,
0.66,0.665,0.67,0.675,0.68,0.685,0.690000000000001,0.695000000000001,0.700000000000001,
0.705000000000001,0.710000000000001,0.715000000000001,0.720000000000001,
0.725000000000001,0.730000000000001,0.735000000000001,0.740000000000001,
0.745000000000001,0.750000000000001,0.755000000000001,0.760000000000001,
0.765000000000001,0.770000000000001,0.775000000000001,0.780000000000001,
0.785000000000001,0.790000000000001,0.795000000000001,0.800000000000001,
0.805000000000001,0.810000000000001,0.815000000000001,0.820000000000001,
0.825000000000001,0.830000000000001,0.835000000000001,0.840000000000001,
0.845000000000001,0.850000000000001,0.855000000000001,0.860000000000001,
0.865000000000001,0.870000000000001,0.875000000000001,0.880000000000001,
0.885000000000001,0.890000000000001,0.895000000000001,0.900000000000001,
0.905000000000001,0.910000000000001,0.915000000000001,0.920000000000001,
0.925000000000001,0.930000000000001,0.935000000000001,0.940000000000001,
0.945000000000001,0.950000000000001,0.955000000000001,0.960000000000001,
0.965000000000001,0.970000000000001,0.975000000000001,0.980000000000001,
0.985000000000001,0.990000000000001,0.995000000000001,1.),(0.,1.2),
 .UNSPECIFIED.)
GEOMETRIC_REPRESENTATION_ITEM()
RATIONAL_B_SPLINE_SURFACE(((1.,1.),(1.,1.),(1.,1.),(1.,1.),(1.,1.),(1.,
1.),(1.,1.),(1.,1.),(1.,1.),(1.,1.),(1.,1.),(1.,1.),(1.,1.),(1.,1.),(1.,
1.),(1.,1.),(1.,1.),(1.,1.),(1.,1.),(1.,1.),(1.,1.),(1.,1.),(1.,1.),(1.,
1.),(1.,1.),(1.,1.),(1.,1.),(1.,1.),(1.,1.),(1.,1.),(1.,1.),(1.,1.),(1.,
1.),(1.,1.),(1.,1.),(1.,1.),(1.,1.),(1.,1.),(1.,1.),(1.,1.),(1.,1.),(1.,
1.),(1.,1.),(1.,1.),(1.,1.),(1.,1.),(1.,1.),(1.,1.),(1.,1.),(1.,1.),(1.,
1.),(1.,1.),(1.,1.),(1.,1.),(1.,1.),(1.,1.),(1.,1.),(1.,1.),(1.,1.),(1.,
1.),(1.,1.),(1.,1.),(1.,1.),(1.,1.),(1.,1.),(1.,1.),(1.,1.),(1.,1.),(1.,
1.),(1.,1.),(1.,1.),(1.,1.),(1.,1.),(1.,1.),(1.,1.),(1.,1.),(1.,1.),(1.,
1.),(1.,1.),(1.,1.),(1.,1.),(1.,1.),(1.,1.),(1.,1.),(1.,1.),(1.,1.),(1.,
1.),(1.,1.),(1.,1.),(1.,1.),(1.,1.),(1.,1.),(1.,1.),(1.,1.),(1.,1.),(1.,
1.),(1.,1.),(1.,1.),(1.,1.),(1.,1.),(1.,1.),(1.,1.),(1.,1.),(1.,1.),(1.,
1.),(1.,1.),(1.,1.),(1.,1.),(1.,1.),(1.,1.),(1.,1.),(1.,1.),(1.,1.),(1.,
1.),(1.,1.),(1.,1.),(1.,1.),(1.,1.),(1.,1.),(1.,1.),(1.,1.),(1.,1.),(1.,
1.),(1.,1.),(1.,1.),(1.,1.),(1.,1.),(1.,1.),(1.,1.),(1.,1.),(1.,1.),(1.,
1.),(1.,1.),(1.,1.),(1.,1.),(1.,1.),(1.,1.),(1.,1.),(1.,1.),(1.,1.),(1.,
1.),(1.,1.),(1.,1.),(1.,1.),(1.,1.),(1.,1.),(1.,1.),(1.,1.),(1.,1.),(1.,
1.),(1.,1.),(1.,1.),(1.,1.),(1.,1.),(1.,1.),(1.,1.),(1.,1.),(1.,1.),(1.,
1.),(1.,1.),(1.,1.),(1.,1.),(1.,1.),(1.,1.),(1.,1.),(1.,1.),(1.,1.),(1.,
1.),(1.,1.),(1.,1.),(1.,1.),(1.,1.),(1.,1.),(1.,1.),(1.,1.),(1.,1.),(1.,
1.),(1.,1.),(1.,1.),(1.,1.),(1.,1.),(1.,1.),(1.,1.),(1.,1.),(1.,1.),(1.,
1.),(1.,1.),(1.,1.),(1.,1.),(1.,1.),(1.,1.),(1.,1.),(1.,1.),(1.,1.),(1.,
1.),(1.,1.),(1.,1.),(1.,1.),(1.,1.),(1.,1.),(1.,1.),(1.,1.),(1.,1.),(1.,
1.),(1.,1.)))
REPRESENTATION_ITEM('')
SURFACE()
);
#1059=(
BOUNDED_SURFACE()
B_SPLINE_SURFACE(5,1,((#205413,#205414),(#205415,#205416),(#205417,#205418),
(#205419,#205420),(#205421,#205422),(#205423,#205424),(#205425,#205426),
(#205427,#205428),(#205429,#205430),(#205431,#205432),(#205433,#205434),
(#205435,#205436),(#205437,#205438),(#205439,#205440),(#205441,#205442),
(#205443,#205444),(#205445,#205446),(#205447,#205448),(#205449,#205450),
(#205451,#205452),(#205453,#205454),(#205455,#205456),(#205457,#205458),
(#205459,#205460),(#205461,#205462),(#205463,#205464),(#205465,#205466),
(#205467,#205468),(#205469,#205470),(#205471,#205472),(#205473,#205474),
(#205475,#205476),(#205477,#205478),(#205479,#205480),(#205481,#205482),
(#205483,#205484),(#205485,#205486),(#205487,#205488),(#205489,#205490),
(#205491,#205492),(#205493,#205494),(#205495,#205496),(#205497,#205498),
(#205499,#205500),(#205501,#205502),(#205503,#205504),(#205505,#205506),
(#205507,#205508),(#205509,#205510),(#205511,#205512),(#205513,#205514),
(#205515,#205516),(#205517,#205518),(#205519,#205520),(#205521,#205522),
(#205523,#205524),(#205525,#205526),(#205527,#205528),(#205529,#205530),
(#205531,#205532),(#205533,#205534),(#205535,#205536),(#205537,#205538),
(#205539,#205540),(#205541,#205542),(#205543,#205544),(#205545,#205546),
(#205547,#205548),(#205549,#205550),(#205551,#205552),(#205553,#205554),
(#205555,#205556),(#205557,#205558),(#205559,#205560),(#205561,#205562),
(#205563,#205564),(#205565,#205566),(#205567,#205568),(#205569,#205570),
(#205571,#205572),(#205573,#205574),(#205575,#205576),(#205577,#205578),
(#205579,#205580),(#205581,#205582),(#205583,#205584),(#205585,#205586),
(#205587,#205588),(#205589,#205590),(#205591,#205592),(#205593,#205594),
(#205595,#205596),(#205597,#205598),(#205599,#205600),(#205601,#205602),
(#205603,#205604),(#205605,#205606),(#205607,#205608),(#205609,#205610),
(#205611,#205612),(#205613,#205614),(#205615,#205616),(#205617,#205618),
(#205619,#205620),(#205621,#205622),(#205623,#205624),(#205625,#205626),
(#205627,#205628),(#205629,#205630),(#205631,#205632),(#205633,#205634),
(#205635,#205636),(#205637,#205638),(#205639,#205640),(#205641,#205642),
(#205643,#205644),(#205645,#205646),(#205647,#205648),(#205649,#205650),
(#205651,#205652),(#205653,#205654),(#205655,#205656),(#205657,#205658),
(#205659,#205660),(#205661,#205662),(#205663,#205664),(#205665,#205666),
(#205667,#205668),(#205669,#205670),(#205671,#205672),(#205673,#205674),
(#205675,#205676),(#205677,#205678),(#205679,#205680),(#205681,#205682),
(#205683,#205684),(#205685,#205686),(#205687,#205688),(#205689,#205690),
(#205691,#205692),(#205693,#205694),(#205695,#205696),(#205697,#205698),
(#205699,#205700),(#205701,#205702),(#205703,#205704),(#205705,#205706),
(#205707,#205708),(#205709,#205710),(#205711,#205712),(#205713,#205714),
(#205715,#205716),(#205717,#205718),(#205719,#205720),(#205721,#205722),
(#205723,#205724),(#205725,#205726),(#205727,#205728),(#205729,#205730),
(#205731,#205732),(#205733,#205734),(#205735,#205736),(#205737,#205738),
(#205739,#205740),(#205741,#205742),(#205743,#205744),(#205745,#205746),
(#205747,#205748),(#205749,#205750),(#205751,#205752),(#205753,#205754),
(#205755,#205756),(#205757,#205758),(#205759,#205760),(#205761,#205762),
(#205763,#205764),(#205765,#205766),(#205767,#205768),(#205769,#205770),
(#205771,#205772),(#205773,#205774),(#205775,#205776),(#205777,#205778),
(#205779,#205780),(#205781,#205782),(#205783,#205784),(#205785,#205786),
(#205787,#205788),(#205789,#205790),(#205791,#205792),(#205793,#205794),
(#205795,#205796),(#205797,#205798),(#205799,#205800),(#205801,#205802),
(#205803,#205804),(#205805,#205806),(#205807,#205808),(#205809,#205810),
(#205811,#205812),(#205813,#205814),(#205815,#205816),(#205817,#205818),
(#205819,#205820),(#205821,#205822)),.UNSPECIFIED.,.F.,.F.,.F.)
B_SPLINE_SURFACE_WITH_KNOTS((6,1,1,1,1,1,1,1,1,1,1,1,1,1,1,1,1,1,1,1,1,
1,1,1,1,1,1,1,1,1,1,1,1,1,1,1,1,1,1,1,1,1,1,1,1,1,1,1,1,1,1,1,1,1,1,1,1,
1,1,1,1,1,1,1,1,1,1,1,1,1,1,1,1,1,1,1,1,1,1,1,1,1,1,1,1,1,1,1,1,1,1,1,1,
1,1,1,1,1,1,1,1,1,1,1,1,1,1,1,1,1,1,1,1,1,1,1,1,1,1,1,1,1,1,1,1,1,1,1,1,
1,1,1,1,1,1,1,1,1,1,1,1,1,1,1,1,1,1,1,1,1,1,1,1,1,1,1,1,1,1,1,1,1,1,1,1,
1,1,1,1,1,1,1,1,1,1,1,1,1,1,1,1,1,1,1,1,1,1,1,1,1,1,1,1,1,1,1,1,1,1,1,6),
(2,2),(-1.,-0.995000000000001,-0.990000000000001,-0.985000000000001,-0.980000000000001,
-0.975000000000001,-0.970000000000001,-0.965000000000001,-0.960000000000001,
-0.955000000000001,-0.950000000000001,-0.945000000000001,-0.940000000000001,
-0.935000000000001,-0.930000000000001,-0.925000000000001,-0.920000000000001,
-0.915000000000001,-0.910000000000001,-0.905000000000001,-0.900000000000001,
-0.895000000000001,-0.890000000000001,-0.885000000000001,-0.880000000000001,
-0.875000000000001,-0.870000000000001,-0.865000000000001,-0.860000000000001,
-0.855000000000001,-0.850000000000001,-0.845000000000001,-0.840000000000001,
-0.835000000000001,-0.830000000000001,-0.825000000000001,-0.820000000000001,
-0.815000000000001,-0.810000000000001,-0.805000000000001,-0.800000000000001,
-0.795000000000001,-0.790000000000001,-0.785000000000001,-0.780000000000001,
-0.775000000000001,-0.770000000000001,-0.765000000000001,-0.760000000000001,
-0.755000000000001,-0.750000000000001,-0.745000000000001,-0.740000000000001,
-0.735000000000001,-0.730000000000001,-0.725000000000001,-0.720000000000001,
-0.715000000000001,-0.710000000000001,-0.705000000000001,-0.700000000000001,
-0.695000000000001,-0.690000000000001,-0.685,-0.68,-0.675,-0.67,-0.665,
-0.66,-0.655,-0.65,-0.645,-0.64,-0.635,-0.63,-0.625,-0.62,-0.615,-0.61,
-0.605,-0.6,-0.595,-0.59,-0.585,-0.58,-0.575,-0.57,-0.565,-0.56,-0.555,
-0.55,-0.545,-0.54,-0.535,-0.53,-0.525,-0.52,-0.515,-0.51,-0.505,-0.5,-0.495,
-0.49,-0.485,-0.48,-0.475,-0.47,-0.465,-0.46,-0.455,-0.45,-0.445,-0.44,
-0.435,-0.43,-0.425,-0.42,-0.415,-0.41,-0.405,-0.4,-0.395,-0.39,-0.385,
-0.38,-0.375,-0.37,-0.365,-0.36,-0.355,-0.35,-0.345,-0.34,-0.335,-0.33,
-0.325,-0.32,-0.315,-0.31,-0.305,-0.3,-0.295,-0.29,-0.285,-0.28,-0.275,
-0.27,-0.265,-0.26,-0.255,-0.25,-0.245,-0.24,-0.235,-0.23,-0.225,-0.22,
-0.215,-0.21,-0.205,-0.2,-0.195,-0.19,-0.185,-0.18,-0.175,-0.17,-0.165,
-0.16,-0.155,-0.15,-0.145,-0.14,-0.135,-0.13,-0.125,-0.12,-0.115,-0.11,
-0.105,-0.1,-0.095,-0.09,-0.085,-0.08,-0.075,-0.07,-0.065,-0.06,-0.055,
-0.05,-0.045,-0.04,-0.035,-0.03,-0.025,-0.02,-0.015,-0.01,-0.005,0.),(0.,
1.2),.UNSPECIFIED.)
GEOMETRIC_REPRESENTATION_ITEM()
RATIONAL_B_SPLINE_SURFACE(((1.,1.),(1.,1.),(1.,1.),(1.,1.),(1.,1.),(1.,
1.),(1.,1.),(1.,1.),(1.,1.),(1.,1.),(1.,1.),(1.,1.),(1.,1.),(1.,1.),(1.,
1.),(1.,1.),(1.,1.),(1.,1.),(1.,1.),(1.,1.),(1.,1.),(1.,1.),(1.,1.),(1.,
1.),(1.,1.),(1.,1.),(1.,1.),(1.,1.),(1.,1.),(1.,1.),(1.,1.),(1.,1.),(1.,
1.),(1.,1.),(1.,1.),(1.,1.),(1.,1.),(1.,1.),(1.,1.),(1.,1.),(1.,1.),(1.,
1.),(1.,1.),(1.,1.),(1.,1.),(1.,1.),(1.,1.),(1.,1.),(1.,1.),(1.,1.),(1.,
1.),(1.,1.),(1.,1.),(1.,1.),(1.,1.),(1.,1.),(1.,1.),(1.,1.),(1.,1.),(1.,
1.),(1.,1.),(1.,1.),(1.,1.),(1.,1.),(1.,1.),(1.,1.),(1.,1.),(1.,1.),(1.,
1.),(1.,1.),(1.,1.),(1.,1.),(1.,1.),(1.,1.),(1.,1.),(1.,1.),(1.,1.),(1.,
1.),(1.,1.),(1.,1.),(1.,1.),(1.,1.),(1.,1.),(1.,1.),(1.,1.),(1.,1.),(1.,
1.),(1.,1.),(1.,1.),(1.,1.),(1.,1.),(1.,1.),(1.,1.),(1.,1.),(1.,1.),(1.,
1.),(1.,1.),(1.,1.),(1.,1.),(1.,1.),(1.,1.),(1.,1.),(1.,1.),(1.,1.),(1.,
1.),(1.,1.),(1.,1.),(1.,1.),(1.,1.),(1.,1.),(1.,1.),(1.,1.),(1.,1.),(1.,
1.),(1.,1.),(1.,1.),(1.,1.),(1.,1.),(1.,1.),(1.,1.),(1.,1.),(1.,1.),(1.,
1.),(1.,1.),(1.,1.),(1.,1.),(1.,1.),(1.,1.),(1.,1.),(1.,1.),(1.,1.),(1.,
1.),(1.,1.),(1.,1.),(1.,1.),(1.,1.),(1.,1.),(1.,1.),(1.,1.),(1.,1.),(1.,
1.),(1.,1.),(1.,1.),(1.,1.),(1.,1.),(1.,1.),(1.,1.),(1.,1.),(1.,1.),(1.,
1.),(1.,1.),(1.,1.),(1.,1.),(1.,1.),(1.,1.),(1.,1.),(1.,1.),(1.,1.),(1.,
1.),(1.,1.),(1.,1.),(1.,1.),(1.,1.),(1.,1.),(1.,1.),(1.,1.),(1.,1.),(1.,
1.),(1.,1.),(1.,1.),(1.,1.),(1.,1.),(1.,1.),(1.,1.),(1.,1.),(1.,1.),(1.,
1.),(1.,1.),(1.,1.),(1.,1.),(1.,1.),(1.,1.),(1.,1.),(1.,1.),(1.,1.),(1.,
1.),(1.,1.),(1.,1.),(1.,1.),(1.,1.),(1.,1.),(1.,1.),(1.,1.),(1.,1.),(1.,
1.),(1.,1.),(1.,1.),(1.,1.),(1.,1.),(1.,1.),(1.,1.),(1.,1.),(1.,1.),(1.,
1.),(1.,1.)))
REPRESENTATION_ITEM('')
SURFACE()
);
#1060=(
BOUNDED_SURFACE()
B_SPLINE_SURFACE(5,1,((#206030,#206031),(#206032,#206033),(#206034,#206035),
(#206036,#206037),(#206038,#206039),(#206040,#206041),(#206042,#206043),
(#206044,#206045),(#206046,#206047),(#206048,#206049),(#206050,#206051),
(#206052,#206053),(#206054,#206055),(#206056,#206057),(#206058,#206059),
(#206060,#206061),(#206062,#206063),(#206064,#206065),(#206066,#206067),
(#206068,#206069),(#206070,#206071),(#206072,#206073),(#206074,#206075),
(#206076,#206077),(#206078,#206079),(#206080,#206081),(#206082,#206083),
(#206084,#206085),(#206086,#206087),(#206088,#206089),(#206090,#206091),
(#206092,#206093),(#206094,#206095),(#206096,#206097),(#206098,#206099),
(#206100,#206101),(#206102,#206103),(#206104,#206105),(#206106,#206107),
(#206108,#206109),(#206110,#206111),(#206112,#206113),(#206114,#206115),
(#206116,#206117),(#206118,#206119),(#206120,#206121),(#206122,#206123),
(#206124,#206125),(#206126,#206127),(#206128,#206129),(#206130,#206131),
(#206132,#206133),(#206134,#206135),(#206136,#206137),(#206138,#206139),
(#206140,#206141),(#206142,#206143),(#206144,#206145),(#206146,#206147),
(#206148,#206149),(#206150,#206151),(#206152,#206153),(#206154,#206155),
(#206156,#206157),(#206158,#206159),(#206160,#206161),(#206162,#206163),
(#206164,#206165),(#206166,#206167),(#206168,#206169),(#206170,#206171),
(#206172,#206173),(#206174,#206175),(#206176,#206177),(#206178,#206179),
(#206180,#206181),(#206182,#206183),(#206184,#206185),(#206186,#206187),
(#206188,#206189),(#206190,#206191),(#206192,#206193),(#206194,#206195),
(#206196,#206197),(#206198,#206199),(#206200,#206201),(#206202,#206203),
(#206204,#206205),(#206206,#206207),(#206208,#206209),(#206210,#206211),
(#206212,#206213),(#206214,#206215),(#206216,#206217),(#206218,#206219),
(#206220,#206221),(#206222,#206223),(#206224,#206225),(#206226,#206227),
(#206228,#206229),(#206230,#206231),(#206232,#206233),(#206234,#206235),
(#206236,#206237),(#206238,#206239),(#206240,#206241),(#206242,#206243),
(#206244,#206245),(#206246,#206247),(#206248,#206249),(#206250,#206251),
(#206252,#206253),(#206254,#206255),(#206256,#206257),(#206258,#206259),
(#206260,#206261),(#206262,#206263),(#206264,#206265),(#206266,#206267),
(#206268,#206269),(#206270,#206271),(#206272,#206273),(#206274,#206275),
(#206276,#206277),(#206278,#206279),(#206280,#206281),(#206282,#206283),
(#206284,#206285),(#206286,#206287),(#206288,#206289),(#206290,#206291),
(#206292,#206293),(#206294,#206295),(#206296,#206297),(#206298,#206299),
(#206300,#206301),(#206302,#206303),(#206304,#206305),(#206306,#206307),
(#206308,#206309),(#206310,#206311),(#206312,#206313),(#206314,#206315),
(#206316,#206317),(#206318,#206319),(#206320,#206321),(#206322,#206323),
(#206324,#206325),(#206326,#206327),(#206328,#206329),(#206330,#206331),
(#206332,#206333),(#206334,#206335),(#206336,#206337),(#206338,#206339),
(#206340,#206341),(#206342,#206343),(#206344,#206345),(#206346,#206347),
(#206348,#206349),(#206350,#206351),(#206352,#206353),(#206354,#206355),
(#206356,#206357),(#206358,#206359),(#206360,#206361),(#206362,#206363),
(#206364,#206365),(#206366,#206367),(#206368,#206369),(#206370,#206371),
(#206372,#206373),(#206374,#206375),(#206376,#206377),(#206378,#206379),
(#206380,#206381),(#206382,#206383),(#206384,#206385),(#206386,#206387),
(#206388,#206389),(#206390,#206391),(#206392,#206393),(#206394,#206395),
(#206396,#206397),(#206398,#206399),(#206400,#206401),(#206402,#206403),
(#206404,#206405),(#206406,#206407),(#206408,#206409),(#206410,#206411),
(#206412,#206413),(#206414,#206415),(#206416,#206417),(#206418,#206419),
(#206420,#206421),(#206422,#206423),(#206424,#206425),(#206426,#206427),
(#206428,#206429),(#206430,#206431),(#206432,#206433),(#206434,#206435),
(#206436,#206437),(#206438,#206439)),.UNSPECIFIED.,.F.,.F.,.F.)
B_SPLINE_SURFACE_WITH_KNOTS((6,1,1,1,1,1,1,1,1,1,1,1,1,1,1,1,1,1,1,1,1,
1,1,1,1,1,1,1,1,1,1,1,1,1,1,1,1,1,1,1,1,1,1,1,1,1,1,1,1,1,1,1,1,1,1,1,1,
1,1,1,1,1,1,1,1,1,1,1,1,1,1,1,1,1,1,1,1,1,1,1,1,1,1,1,1,1,1,1,1,1,1,1,1,
1,1,1,1,1,1,1,1,1,1,1,1,1,1,1,1,1,1,1,1,1,1,1,1,1,1,1,1,1,1,1,1,1,1,1,1,
1,1,1,1,1,1,1,1,1,1,1,1,1,1,1,1,1,1,1,1,1,1,1,1,1,1,1,1,1,1,1,1,1,1,1,1,
1,1,1,1,1,1,1,1,1,1,1,1,1,1,1,1,1,1,1,1,1,1,1,1,1,1,1,1,1,1,1,1,1,1,1,6),
(2,2),(0.,0.005,0.01,0.015,0.02,0.025,0.03,0.035,0.04,0.045,0.05,0.055,
0.06,0.065,0.07,0.075,0.08,0.085,0.09,0.095,0.1,0.105,0.11,0.115,0.12,0.125,
0.13,0.135,0.14,0.145,0.15,0.155,0.16,0.165,0.17,0.175,0.18,0.185,0.19,
0.195,0.2,0.205,0.21,0.215,0.22,0.225,0.23,0.235,0.24,0.245,0.25,0.255,
0.26,0.265,0.27,0.275,0.28,0.285,0.29,0.295,0.3,0.305,0.31,0.315,0.32,0.325,
0.33,0.335,0.34,0.345,0.35,0.355,0.36,0.365,0.37,0.375,0.38,0.385,0.39,
0.395,0.4,0.405,0.41,0.415,0.42,0.425,0.43,0.435,0.44,0.445,0.45,0.455,
0.46,0.465,0.47,0.475,0.48,0.485,0.49,0.495,0.5,0.505,0.51,0.515,0.52,0.525,
0.53,0.535,0.54,0.545,0.55,0.555,0.56,0.565,0.57,0.575,0.58,0.585,0.59,
0.595,0.6,0.605,0.61,0.615,0.62,0.625,0.63,0.635,0.64,0.645,0.65,0.655,
0.66,0.665,0.67,0.675,0.68,0.685,0.690000000000001,0.695000000000001,0.700000000000001,
0.705000000000001,0.710000000000001,0.715000000000001,0.720000000000001,
0.725000000000001,0.730000000000001,0.735000000000001,0.740000000000001,
0.745000000000001,0.750000000000001,0.755000000000001,0.760000000000001,
0.765000000000001,0.770000000000001,0.775000000000001,0.780000000000001,
0.785000000000001,0.790000000000001,0.795000000000001,0.800000000000001,
0.805000000000001,0.810000000000001,0.815000000000001,0.820000000000001,
0.825000000000001,0.830000000000001,0.835000000000001,0.840000000000001,
0.845000000000001,0.850000000000001,0.855000000000001,0.860000000000001,
0.865000000000001,0.870000000000001,0.875000000000001,0.880000000000001,
0.885000000000001,0.890000000000001,0.895000000000001,0.900000000000001,
0.905000000000001,0.910000000000001,0.915000000000001,0.920000000000001,
0.925000000000001,0.930000000000001,0.935000000000001,0.940000000000001,
0.945000000000001,0.950000000000001,0.955000000000001,0.960000000000001,
0.965000000000001,0.970000000000001,0.975000000000001,0.980000000000001,
0.985000000000001,0.990000000000001,0.995000000000001,1.),(0.,1.2),
 .UNSPECIFIED.)
GEOMETRIC_REPRESENTATION_ITEM()
RATIONAL_B_SPLINE_SURFACE(((1.,1.),(1.,1.),(1.,1.),(1.,1.),(1.,1.),(1.,
1.),(1.,1.),(1.,1.),(1.,1.),(1.,1.),(1.,1.),(1.,1.),(1.,1.),(1.,1.),(1.,
1.),(1.,1.),(1.,1.),(1.,1.),(1.,1.),(1.,1.),(1.,1.),(1.,1.),(1.,1.),(1.,
1.),(1.,1.),(1.,1.),(1.,1.),(1.,1.),(1.,1.),(1.,1.),(1.,1.),(1.,1.),(1.,
1.),(1.,1.),(1.,1.),(1.,1.),(1.,1.),(1.,1.),(1.,1.),(1.,1.),(1.,1.),(1.,
1.),(1.,1.),(1.,1.),(1.,1.),(1.,1.),(1.,1.),(1.,1.),(1.,1.),(1.,1.),(1.,
1.),(1.,1.),(1.,1.),(1.,1.),(1.,1.),(1.,1.),(1.,1.),(1.,1.),(1.,1.),(1.,
1.),(1.,1.),(1.,1.),(1.,1.),(1.,1.),(1.,1.),(1.,1.),(1.,1.),(1.,1.),(1.,
1.),(1.,1.),(1.,1.),(1.,1.),(1.,1.),(1.,1.),(1.,1.),(1.,1.),(1.,1.),(1.,
1.),(1.,1.),(1.,1.),(1.,1.),(1.,1.),(1.,1.),(1.,1.),(1.,1.),(1.,1.),(1.,
1.),(1.,1.),(1.,1.),(1.,1.),(1.,1.),(1.,1.),(1.,1.),(1.,1.),(1.,1.),(1.,
1.),(1.,1.),(1.,1.),(1.,1.),(1.,1.),(1.,1.),(1.,1.),(1.,1.),(1.,1.),(1.,
1.),(1.,1.),(1.,1.),(1.,1.),(1.,1.),(1.,1.),(1.,1.),(1.,1.),(1.,1.),(1.,
1.),(1.,1.),(1.,1.),(1.,1.),(1.,1.),(1.,1.),(1.,1.),(1.,1.),(1.,1.),(1.,
1.),(1.,1.),(1.,1.),(1.,1.),(1.,1.),(1.,1.),(1.,1.),(1.,1.),(1.,1.),(1.,
1.),(1.,1.),(1.,1.),(1.,1.),(1.,1.),(1.,1.),(1.,1.),(1.,1.),(1.,1.),(1.,
1.),(1.,1.),(1.,1.),(1.,1.),(1.,1.),(1.,1.),(1.,1.),(1.,1.),(1.,1.),(1.,
1.),(1.,1.),(1.,1.),(1.,1.),(1.,1.),(1.,1.),(1.,1.),(1.,1.),(1.,1.),(1.,
1.),(1.,1.),(1.,1.),(1.,1.),(1.,1.),(1.,1.),(1.,1.),(1.,1.),(1.,1.),(1.,
1.),(1.,1.),(1.,1.),(1.,1.),(1.,1.),(1.,1.),(1.,1.),(1.,1.),(1.,1.),(1.,
1.),(1.,1.),(1.,1.),(1.,1.),(1.,1.),(1.,1.),(1.,1.),(1.,1.),(1.,1.),(1.,
1.),(1.,1.),(1.,1.),(1.,1.),(1.,1.),(1.,1.),(1.,1.),(1.,1.),(1.,1.),(1.,
1.),(1.,1.),(1.,1.),(1.,1.),(1.,1.),(1.,1.),(1.,1.),(1.,1.),(1.,1.),(1.,
1.),(1.,1.)))
REPRESENTATION_ITEM('')
SURFACE()
);
#1061=(
BOUNDED_SURFACE()
B_SPLINE_SURFACE(5,1,((#206651,#206652),(#206653,#206654),(#206655,#206656),
(#206657,#206658),(#206659,#206660),(#206661,#206662),(#206663,#206664),
(#206665,#206666),(#206667,#206668),(#206669,#206670),(#206671,#206672),
(#206673,#206674),(#206675,#206676),(#206677,#206678),(#206679,#206680),
(#206681,#206682),(#206683,#206684),(#206685,#206686),(#206687,#206688),
(#206689,#206690),(#206691,#206692),(#206693,#206694),(#206695,#206696),
(#206697,#206698),(#206699,#206700),(#206701,#206702),(#206703,#206704),
(#206705,#206706),(#206707,#206708),(#206709,#206710),(#206711,#206712),
(#206713,#206714),(#206715,#206716),(#206717,#206718),(#206719,#206720),
(#206721,#206722),(#206723,#206724),(#206725,#206726),(#206727,#206728),
(#206729,#206730),(#206731,#206732),(#206733,#206734),(#206735,#206736),
(#206737,#206738),(#206739,#206740),(#206741,#206742),(#206743,#206744),
(#206745,#206746),(#206747,#206748),(#206749,#206750),(#206751,#206752),
(#206753,#206754),(#206755,#206756),(#206757,#206758),(#206759,#206760),
(#206761,#206762),(#206763,#206764),(#206765,#206766),(#206767,#206768),
(#206769,#206770),(#206771,#206772),(#206773,#206774),(#206775,#206776),
(#206777,#206778),(#206779,#206780),(#206781,#206782),(#206783,#206784),
(#206785,#206786),(#206787,#206788),(#206789,#206790),(#206791,#206792),
(#206793,#206794),(#206795,#206796),(#206797,#206798),(#206799,#206800),
(#206801,#206802),(#206803,#206804),(#206805,#206806),(#206807,#206808),
(#206809,#206810),(#206811,#206812),(#206813,#206814),(#206815,#206816),
(#206817,#206818),(#206819,#206820),(#206821,#206822),(#206823,#206824),
(#206825,#206826),(#206827,#206828),(#206829,#206830),(#206831,#206832),
(#206833,#206834),(#206835,#206836),(#206837,#206838),(#206839,#206840),
(#206841,#206842),(#206843,#206844),(#206845,#206846),(#206847,#206848),
(#206849,#206850),(#206851,#206852),(#206853,#206854),(#206855,#206856),
(#206857,#206858),(#206859,#206860),(#206861,#206862),(#206863,#206864),
(#206865,#206866),(#206867,#206868),(#206869,#206870),(#206871,#206872),
(#206873,#206874),(#206875,#206876),(#206877,#206878),(#206879,#206880),
(#206881,#206882),(#206883,#206884),(#206885,#206886),(#206887,#206888),
(#206889,#206890),(#206891,#206892),(#206893,#206894),(#206895,#206896),
(#206897,#206898),(#206899,#206900),(#206901,#206902),(#206903,#206904),
(#206905,#206906),(#206907,#206908),(#206909,#206910),(#206911,#206912),
(#206913,#206914),(#206915,#206916),(#206917,#206918),(#206919,#206920),
(#206921,#206922),(#206923,#206924),(#206925,#206926),(#206927,#206928),
(#206929,#206930),(#206931,#206932),(#206933,#206934),(#206935,#206936),
(#206937,#206938),(#206939,#206940),(#206941,#206942),(#206943,#206944),
(#206945,#206946),(#206947,#206948),(#206949,#206950),(#206951,#206952),
(#206953,#206954),(#206955,#206956),(#206957,#206958),(#206959,#206960),
(#206961,#206962),(#206963,#206964),(#206965,#206966),(#206967,#206968),
(#206969,#206970),(#206971,#206972),(#206973,#206974),(#206975,#206976),
(#206977,#206978),(#206979,#206980),(#206981,#206982),(#206983,#206984),
(#206985,#206986),(#206987,#206988),(#206989,#206990),(#206991,#206992),
(#206993,#206994),(#206995,#206996),(#206997,#206998),(#206999,#207000),
(#207001,#207002),(#207003,#207004),(#207005,#207006),(#207007,#207008),
(#207009,#207010),(#207011,#207012),(#207013,#207014),(#207015,#207016),
(#207017,#207018),(#207019,#207020),(#207021,#207022),(#207023,#207024),
(#207025,#207026),(#207027,#207028),(#207029,#207030),(#207031,#207032),
(#207033,#207034),(#207035,#207036),(#207037,#207038),(#207039,#207040),
(#207041,#207042),(#207043,#207044),(#207045,#207046),(#207047,#207048),
(#207049,#207050),(#207051,#207052),(#207053,#207054),(#207055,#207056),
(#207057,#207058),(#207059,#207060)),.UNSPECIFIED.,.F.,.F.,.F.)
B_SPLINE_SURFACE_WITH_KNOTS((6,1,1,1,1,1,1,1,1,1,1,1,1,1,1,1,1,1,1,1,1,
1,1,1,1,1,1,1,1,1,1,1,1,1,1,1,1,1,1,1,1,1,1,1,1,1,1,1,1,1,1,1,1,1,1,1,1,
1,1,1,1,1,1,1,1,1,1,1,1,1,1,1,1,1,1,1,1,1,1,1,1,1,1,1,1,1,1,1,1,1,1,1,1,
1,1,1,1,1,1,1,1,1,1,1,1,1,1,1,1,1,1,1,1,1,1,1,1,1,1,1,1,1,1,1,1,1,1,1,1,
1,1,1,1,1,1,1,1,1,1,1,1,1,1,1,1,1,1,1,1,1,1,1,1,1,1,1,1,1,1,1,1,1,1,1,1,
1,1,1,1,1,1,1,1,1,1,1,1,1,1,1,1,1,1,1,1,1,1,1,1,1,1,1,1,1,1,1,1,1,1,1,6),
(2,2),(-1.,-0.995000000000001,-0.990000000000001,-0.985000000000001,-0.980000000000001,
-0.975000000000001,-0.970000000000001,-0.965000000000001,-0.960000000000001,
-0.955000000000001,-0.950000000000001,-0.945000000000001,-0.940000000000001,
-0.935000000000001,-0.930000000000001,-0.925000000000001,-0.920000000000001,
-0.915000000000001,-0.910000000000001,-0.905000000000001,-0.900000000000001,
-0.895000000000001,-0.890000000000001,-0.885000000000001,-0.880000000000001,
-0.875000000000001,-0.870000000000001,-0.865000000000001,-0.860000000000001,
-0.855000000000001,-0.850000000000001,-0.845000000000001,-0.840000000000001,
-0.835000000000001,-0.830000000000001,-0.825000000000001,-0.820000000000001,
-0.815000000000001,-0.810000000000001,-0.805000000000001,-0.800000000000001,
-0.795000000000001,-0.790000000000001,-0.785000000000001,-0.780000000000001,
-0.775000000000001,-0.770000000000001,-0.765000000000001,-0.760000000000001,
-0.755000000000001,-0.750000000000001,-0.745000000000001,-0.740000000000001,
-0.735000000000001,-0.730000000000001,-0.725000000000001,-0.720000000000001,
-0.715000000000001,-0.710000000000001,-0.705000000000001,-0.700000000000001,
-0.695000000000001,-0.690000000000001,-0.685,-0.68,-0.675,-0.67,-0.665,
-0.66,-0.655,-0.65,-0.645,-0.64,-0.635,-0.63,-0.625,-0.62,-0.615,-0.61,
-0.605,-0.6,-0.595,-0.59,-0.585,-0.58,-0.575,-0.57,-0.565,-0.56,-0.555,
-0.55,-0.545,-0.54,-0.535,-0.53,-0.525,-0.52,-0.515,-0.51,-0.505,-0.5,-0.495,
-0.49,-0.485,-0.48,-0.475,-0.47,-0.465,-0.46,-0.455,-0.45,-0.445,-0.44,
-0.435,-0.43,-0.425,-0.42,-0.415,-0.41,-0.405,-0.4,-0.395,-0.39,-0.385,
-0.38,-0.375,-0.37,-0.365,-0.36,-0.355,-0.35,-0.345,-0.34,-0.335,-0.33,
-0.325,-0.32,-0.315,-0.31,-0.305,-0.3,-0.295,-0.29,-0.285,-0.28,-0.275,
-0.27,-0.265,-0.26,-0.255,-0.25,-0.245,-0.24,-0.235,-0.23,-0.225,-0.22,
-0.215,-0.21,-0.205,-0.2,-0.195,-0.19,-0.185,-0.18,-0.175,-0.17,-0.165,
-0.16,-0.155,-0.15,-0.145,-0.14,-0.135,-0.13,-0.125,-0.12,-0.115,-0.11,
-0.105,-0.1,-0.095,-0.09,-0.085,-0.08,-0.075,-0.07,-0.065,-0.06,-0.055,
-0.05,-0.045,-0.04,-0.035,-0.03,-0.025,-0.02,-0.015,-0.01,-0.005,0.),(0.,
1.2),.UNSPECIFIED.)
GEOMETRIC_REPRESENTATION_ITEM()
RATIONAL_B_SPLINE_SURFACE(((1.,1.),(1.,1.),(1.,1.),(1.,1.),(1.,1.),(1.,
1.),(1.,1.),(1.,1.),(1.,1.),(1.,1.),(1.,1.),(1.,1.),(1.,1.),(1.,1.),(1.,
1.),(1.,1.),(1.,1.),(1.,1.),(1.,1.),(1.,1.),(1.,1.),(1.,1.),(1.,1.),(1.,
1.),(1.,1.),(1.,1.),(1.,1.),(1.,1.),(1.,1.),(1.,1.),(1.,1.),(1.,1.),(1.,
1.),(1.,1.),(1.,1.),(1.,1.),(1.,1.),(1.,1.),(1.,1.),(1.,1.),(1.,1.),(1.,
1.),(1.,1.),(1.,1.),(1.,1.),(1.,1.),(1.,1.),(1.,1.),(1.,1.),(1.,1.),(1.,
1.),(1.,1.),(1.,1.),(1.,1.),(1.,1.),(1.,1.),(1.,1.),(1.,1.),(1.,1.),(1.,
1.),(1.,1.),(1.,1.),(1.,1.),(1.,1.),(1.,1.),(1.,1.),(1.,1.),(1.,1.),(1.,
1.),(1.,1.),(1.,1.),(1.,1.),(1.,1.),(1.,1.),(1.,1.),(1.,1.),(1.,1.),(1.,
1.),(1.,1.),(1.,1.),(1.,1.),(1.,1.),(1.,1.),(1.,1.),(1.,1.),(1.,1.),(1.,
1.),(1.,1.),(1.,1.),(1.,1.),(1.,1.),(1.,1.),(1.,1.),(1.,1.),(1.,1.),(1.,
1.),(1.,1.),(1.,1.),(1.,1.),(1.,1.),(1.,1.),(1.,1.),(1.,1.),(1.,1.),(1.,
1.),(1.,1.),(1.,1.),(1.,1.),(1.,1.),(1.,1.),(1.,1.),(1.,1.),(1.,1.),(1.,
1.),(1.,1.),(1.,1.),(1.,1.),(1.,1.),(1.,1.),(1.,1.),(1.,1.),(1.,1.),(1.,
1.),(1.,1.),(1.,1.),(1.,1.),(1.,1.),(1.,1.),(1.,1.),(1.,1.),(1.,1.),(1.,
1.),(1.,1.),(1.,1.),(1.,1.),(1.,1.),(1.,1.),(1.,1.),(1.,1.),(1.,1.),(1.,
1.),(1.,1.),(1.,1.),(1.,1.),(1.,1.),(1.,1.),(1.,1.),(1.,1.),(1.,1.),(1.,
1.),(1.,1.),(1.,1.),(1.,1.),(1.,1.),(1.,1.),(1.,1.),(1.,1.),(1.,1.),(1.,
1.),(1.,1.),(1.,1.),(1.,1.),(1.,1.),(1.,1.),(1.,1.),(1.,1.),(1.,1.),(1.,
1.),(1.,1.),(1.,1.),(1.,1.),(1.,1.),(1.,1.),(1.,1.),(1.,1.),(1.,1.),(1.,
1.),(1.,1.),(1.,1.),(1.,1.),(1.,1.),(1.,1.),(1.,1.),(1.,1.),(1.,1.),(1.,
1.),(1.,1.),(1.,1.),(1.,1.),(1.,1.),(1.,1.),(1.,1.),(1.,1.),(1.,1.),(1.,
1.),(1.,1.),(1.,1.),(1.,1.),(1.,1.),(1.,1.),(1.,1.),(1.,1.),(1.,1.),(1.,
1.),(1.,1.)))
REPRESENTATION_ITEM('')
SURFACE()
);
#1062=(
BOUNDED_SURFACE()
B_SPLINE_SURFACE(5,1,((#207268,#207269),(#207270,#207271),(#207272,#207273),
(#207274,#207275),(#207276,#207277),(#207278,#207279),(#207280,#207281),
(#207282,#207283),(#207284,#207285),(#207286,#207287),(#207288,#207289),
(#207290,#207291),(#207292,#207293),(#207294,#207295),(#207296,#207297),
(#207298,#207299),(#207300,#207301),(#207302,#207303),(#207304,#207305),
(#207306,#207307),(#207308,#207309),(#207310,#207311),(#207312,#207313),
(#207314,#207315),(#207316,#207317),(#207318,#207319),(#207320,#207321),
(#207322,#207323),(#207324,#207325),(#207326,#207327),(#207328,#207329),
(#207330,#207331),(#207332,#207333),(#207334,#207335),(#207336,#207337),
(#207338,#207339),(#207340,#207341),(#207342,#207343),(#207344,#207345),
(#207346,#207347),(#207348,#207349),(#207350,#207351),(#207352,#207353),
(#207354,#207355),(#207356,#207357),(#207358,#207359),(#207360,#207361),
(#207362,#207363),(#207364,#207365),(#207366,#207367),(#207368,#207369),
(#207370,#207371),(#207372,#207373),(#207374,#207375),(#207376,#207377),
(#207378,#207379),(#207380,#207381),(#207382,#207383),(#207384,#207385),
(#207386,#207387),(#207388,#207389),(#207390,#207391),(#207392,#207393),
(#207394,#207395),(#207396,#207397),(#207398,#207399),(#207400,#207401),
(#207402,#207403),(#207404,#207405),(#207406,#207407),(#207408,#207409),
(#207410,#207411),(#207412,#207413),(#207414,#207415),(#207416,#207417),
(#207418,#207419),(#207420,#207421),(#207422,#207423),(#207424,#207425),
(#207426,#207427),(#207428,#207429),(#207430,#207431),(#207432,#207433),
(#207434,#207435),(#207436,#207437),(#207438,#207439),(#207440,#207441),
(#207442,#207443),(#207444,#207445),(#207446,#207447),(#207448,#207449),
(#207450,#207451),(#207452,#207453),(#207454,#207455),(#207456,#207457),
(#207458,#207459),(#207460,#207461),(#207462,#207463),(#207464,#207465),
(#207466,#207467),(#207468,#207469),(#207470,#207471),(#207472,#207473),
(#207474,#207475),(#207476,#207477),(#207478,#207479),(#207480,#207481),
(#207482,#207483),(#207484,#207485),(#207486,#207487),(#207488,#207489),
(#207490,#207491),(#207492,#207493),(#207494,#207495),(#207496,#207497),
(#207498,#207499),(#207500,#207501),(#207502,#207503),(#207504,#207505),
(#207506,#207507),(#207508,#207509),(#207510,#207511),(#207512,#207513),
(#207514,#207515),(#207516,#207517),(#207518,#207519),(#207520,#207521),
(#207522,#207523),(#207524,#207525),(#207526,#207527),(#207528,#207529),
(#207530,#207531),(#207532,#207533),(#207534,#207535),(#207536,#207537),
(#207538,#207539),(#207540,#207541),(#207542,#207543),(#207544,#207545),
(#207546,#207547),(#207548,#207549),(#207550,#207551),(#207552,#207553),
(#207554,#207555),(#207556,#207557),(#207558,#207559),(#207560,#207561),
(#207562,#207563),(#207564,#207565),(#207566,#207567),(#207568,#207569),
(#207570,#207571),(#207572,#207573),(#207574,#207575),(#207576,#207577),
(#207578,#207579),(#207580,#207581),(#207582,#207583),(#207584,#207585),
(#207586,#207587),(#207588,#207589),(#207590,#207591),(#207592,#207593),
(#207594,#207595),(#207596,#207597),(#207598,#207599),(#207600,#207601),
(#207602,#207603),(#207604,#207605),(#207606,#207607),(#207608,#207609),
(#207610,#207611),(#207612,#207613),(#207614,#207615),(#207616,#207617),
(#207618,#207619),(#207620,#207621),(#207622,#207623),(#207624,#207625),
(#207626,#207627),(#207628,#207629),(#207630,#207631),(#207632,#207633),
(#207634,#207635),(#207636,#207637),(#207638,#207639),(#207640,#207641),
(#207642,#207643),(#207644,#207645),(#207646,#207647),(#207648,#207649),
(#207650,#207651),(#207652,#207653),(#207654,#207655),(#207656,#207657),
(#207658,#207659),(#207660,#207661),(#207662,#207663),(#207664,#207665),
(#207666,#207667),(#207668,#207669),(#207670,#207671),(#207672,#207673),
(#207674,#207675),(#207676,#207677)),.UNSPECIFIED.,.F.,.F.,.F.)
B_SPLINE_SURFACE_WITH_KNOTS((6,1,1,1,1,1,1,1,1,1,1,1,1,1,1,1,1,1,1,1,1,
1,1,1,1,1,1,1,1,1,1,1,1,1,1,1,1,1,1,1,1,1,1,1,1,1,1,1,1,1,1,1,1,1,1,1,1,
1,1,1,1,1,1,1,1,1,1,1,1,1,1,1,1,1,1,1,1,1,1,1,1,1,1,1,1,1,1,1,1,1,1,1,1,
1,1,1,1,1,1,1,1,1,1,1,1,1,1,1,1,1,1,1,1,1,1,1,1,1,1,1,1,1,1,1,1,1,1,1,1,
1,1,1,1,1,1,1,1,1,1,1,1,1,1,1,1,1,1,1,1,1,1,1,1,1,1,1,1,1,1,1,1,1,1,1,1,
1,1,1,1,1,1,1,1,1,1,1,1,1,1,1,1,1,1,1,1,1,1,1,1,1,1,1,1,1,1,1,1,1,1,1,6),
(2,2),(0.,0.005,0.01,0.015,0.02,0.025,0.03,0.035,0.04,0.045,0.05,0.055,
0.06,0.065,0.07,0.075,0.08,0.085,0.09,0.095,0.1,0.105,0.11,0.115,0.12,0.125,
0.13,0.135,0.14,0.145,0.15,0.155,0.16,0.165,0.17,0.175,0.18,0.185,0.19,
0.195,0.2,0.205,0.21,0.215,0.22,0.225,0.23,0.235,0.24,0.245,0.25,0.255,
0.26,0.265,0.27,0.275,0.28,0.285,0.29,0.295,0.3,0.305,0.31,0.315,0.32,0.325,
0.33,0.335,0.34,0.345,0.35,0.355,0.36,0.365,0.37,0.375,0.38,0.385,0.39,
0.395,0.4,0.405,0.41,0.415,0.42,0.425,0.43,0.435,0.44,0.445,0.45,0.455,
0.46,0.465,0.47,0.475,0.48,0.485,0.49,0.495,0.5,0.505,0.51,0.515,0.52,0.525,
0.53,0.535,0.54,0.545,0.55,0.555,0.56,0.565,0.57,0.575,0.58,0.585,0.59,
0.595,0.6,0.605,0.61,0.615,0.62,0.625,0.63,0.635,0.64,0.645,0.65,0.655,
0.66,0.665,0.67,0.675,0.68,0.685,0.690000000000001,0.695000000000001,0.700000000000001,
0.705000000000001,0.710000000000001,0.715000000000001,0.720000000000001,
0.725000000000001,0.730000000000001,0.735000000000001,0.740000000000001,
0.745000000000001,0.750000000000001,0.755000000000001,0.760000000000001,
0.765000000000001,0.770000000000001,0.775000000000001,0.780000000000001,
0.785000000000001,0.790000000000001,0.795000000000001,0.800000000000001,
0.805000000000001,0.810000000000001,0.815000000000001,0.820000000000001,
0.825000000000001,0.830000000000001,0.835000000000001,0.840000000000001,
0.845000000000001,0.850000000000001,0.855000000000001,0.860000000000001,
0.865000000000001,0.870000000000001,0.875000000000001,0.880000000000001,
0.885000000000001,0.890000000000001,0.895000000000001,0.900000000000001,
0.905000000000001,0.910000000000001,0.915000000000001,0.920000000000001,
0.925000000000001,0.930000000000001,0.935000000000001,0.940000000000001,
0.945000000000001,0.950000000000001,0.955000000000001,0.960000000000001,
0.965000000000001,0.970000000000001,0.975000000000001,0.980000000000001,
0.985000000000001,0.990000000000001,0.995000000000001,1.),(0.,1.2),
 .UNSPECIFIED.)
GEOMETRIC_REPRESENTATION_ITEM()
RATIONAL_B_SPLINE_SURFACE(((1.,1.),(1.,1.),(1.,1.),(1.,1.),(1.,1.),(1.,
1.),(1.,1.),(1.,1.),(1.,1.),(1.,1.),(1.,1.),(1.,1.),(1.,1.),(1.,1.),(1.,
1.),(1.,1.),(1.,1.),(1.,1.),(1.,1.),(1.,1.),(1.,1.),(1.,1.),(1.,1.),(1.,
1.),(1.,1.),(1.,1.),(1.,1.),(1.,1.),(1.,1.),(1.,1.),(1.,1.),(1.,1.),(1.,
1.),(1.,1.),(1.,1.),(1.,1.),(1.,1.),(1.,1.),(1.,1.),(1.,1.),(1.,1.),(1.,
1.),(1.,1.),(1.,1.),(1.,1.),(1.,1.),(1.,1.),(1.,1.),(1.,1.),(1.,1.),(1.,
1.),(1.,1.),(1.,1.),(1.,1.),(1.,1.),(1.,1.),(1.,1.),(1.,1.),(1.,1.),(1.,
1.),(1.,1.),(1.,1.),(1.,1.),(1.,1.),(1.,1.),(1.,1.),(1.,1.),(1.,1.),(1.,
1.),(1.,1.),(1.,1.),(1.,1.),(1.,1.),(1.,1.),(1.,1.),(1.,1.),(1.,1.),(1.,
1.),(1.,1.),(1.,1.),(1.,1.),(1.,1.),(1.,1.),(1.,1.),(1.,1.),(1.,1.),(1.,
1.),(1.,1.),(1.,1.),(1.,1.),(1.,1.),(1.,1.),(1.,1.),(1.,1.),(1.,1.),(1.,
1.),(1.,1.),(1.,1.),(1.,1.),(1.,1.),(1.,1.),(1.,1.),(1.,1.),(1.,1.),(1.,
1.),(1.,1.),(1.,1.),(1.,1.),(1.,1.),(1.,1.),(1.,1.),(1.,1.),(1.,1.),(1.,
1.),(1.,1.),(1.,1.),(1.,1.),(1.,1.),(1.,1.),(1.,1.),(1.,1.),(1.,1.),(1.,
1.),(1.,1.),(1.,1.),(1.,1.),(1.,1.),(1.,1.),(1.,1.),(1.,1.),(1.,1.),(1.,
1.),(1.,1.),(1.,1.),(1.,1.),(1.,1.),(1.,1.),(1.,1.),(1.,1.),(1.,1.),(1.,
1.),(1.,1.),(1.,1.),(1.,1.),(1.,1.),(1.,1.),(1.,1.),(1.,1.),(1.,1.),(1.,
1.),(1.,1.),(1.,1.),(1.,1.),(1.,1.),(1.,1.),(1.,1.),(1.,1.),(1.,1.),(1.,
1.),(1.,1.),(1.,1.),(1.,1.),(1.,1.),(1.,1.),(1.,1.),(1.,1.),(1.,1.),(1.,
1.),(1.,1.),(1.,1.),(1.,1.),(1.,1.),(1.,1.),(1.,1.),(1.,1.),(1.,1.),(1.,
1.),(1.,1.),(1.,1.),(1.,1.),(1.,1.),(1.,1.),(1.,1.),(1.,1.),(1.,1.),(1.,
1.),(1.,1.),(1.,1.),(1.,1.),(1.,1.),(1.,1.),(1.,1.),(1.,1.),(1.,1.),(1.,
1.),(1.,1.),(1.,1.),(1.,1.),(1.,1.),(1.,1.),(1.,1.),(1.,1.),(1.,1.),(1.,
1.),(1.,1.)))
REPRESENTATION_ITEM('')
SURFACE()
);
#1063=(
BOUNDED_SURFACE()
B_SPLINE_SURFACE(5,1,((#207889,#207890),(#207891,#207892),(#207893,#207894),
(#207895,#207896),(#207897,#207898),(#207899,#207900),(#207901,#207902),
(#207903,#207904),(#207905,#207906),(#207907,#207908),(#207909,#207910),
(#207911,#207912),(#207913,#207914),(#207915,#207916),(#207917,#207918),
(#207919,#207920),(#207921,#207922),(#207923,#207924),(#207925,#207926),
(#207927,#207928),(#207929,#207930),(#207931,#207932),(#207933,#207934),
(#207935,#207936),(#207937,#207938),(#207939,#207940),(#207941,#207942),
(#207943,#207944),(#207945,#207946),(#207947,#207948),(#207949,#207950),
(#207951,#207952),(#207953,#207954),(#207955,#207956),(#207957,#207958),
(#207959,#207960),(#207961,#207962),(#207963,#207964),(#207965,#207966),
(#207967,#207968),(#207969,#207970),(#207971,#207972),(#207973,#207974),
(#207975,#207976),(#207977,#207978),(#207979,#207980),(#207981,#207982),
(#207983,#207984),(#207985,#207986),(#207987,#207988),(#207989,#207990),
(#207991,#207992),(#207993,#207994),(#207995,#207996),(#207997,#207998),
(#207999,#208000),(#208001,#208002),(#208003,#208004),(#208005,#208006),
(#208007,#208008),(#208009,#208010),(#208011,#208012),(#208013,#208014),
(#208015,#208016),(#208017,#208018),(#208019,#208020),(#208021,#208022),
(#208023,#208024),(#208025,#208026),(#208027,#208028),(#208029,#208030),
(#208031,#208032),(#208033,#208034),(#208035,#208036),(#208037,#208038),
(#208039,#208040),(#208041,#208042),(#208043,#208044),(#208045,#208046),
(#208047,#208048),(#208049,#208050),(#208051,#208052),(#208053,#208054),
(#208055,#208056),(#208057,#208058),(#208059,#208060),(#208061,#208062),
(#208063,#208064),(#208065,#208066),(#208067,#208068),(#208069,#208070),
(#208071,#208072),(#208073,#208074),(#208075,#208076),(#208077,#208078),
(#208079,#208080),(#208081,#208082),(#208083,#208084),(#208085,#208086),
(#208087,#208088),(#208089,#208090),(#208091,#208092),(#208093,#208094),
(#208095,#208096),(#208097,#208098),(#208099,#208100),(#208101,#208102),
(#208103,#208104),(#208105,#208106),(#208107,#208108),(#208109,#208110),
(#208111,#208112),(#208113,#208114),(#208115,#208116),(#208117,#208118),
(#208119,#208120),(#208121,#208122),(#208123,#208124),(#208125,#208126),
(#208127,#208128),(#208129,#208130),(#208131,#208132),(#208133,#208134),
(#208135,#208136),(#208137,#208138),(#208139,#208140),(#208141,#208142),
(#208143,#208144),(#208145,#208146),(#208147,#208148),(#208149,#208150),
(#208151,#208152),(#208153,#208154),(#208155,#208156),(#208157,#208158),
(#208159,#208160),(#208161,#208162),(#208163,#208164),(#208165,#208166),
(#208167,#208168),(#208169,#208170),(#208171,#208172),(#208173,#208174),
(#208175,#208176),(#208177,#208178),(#208179,#208180),(#208181,#208182),
(#208183,#208184),(#208185,#208186),(#208187,#208188),(#208189,#208190),
(#208191,#208192),(#208193,#208194),(#208195,#208196),(#208197,#208198),
(#208199,#208200),(#208201,#208202),(#208203,#208204),(#208205,#208206),
(#208207,#208208),(#208209,#208210),(#208211,#208212),(#208213,#208214),
(#208215,#208216),(#208217,#208218),(#208219,#208220),(#208221,#208222),
(#208223,#208224),(#208225,#208226),(#208227,#208228),(#208229,#208230),
(#208231,#208232),(#208233,#208234),(#208235,#208236),(#208237,#208238),
(#208239,#208240),(#208241,#208242),(#208243,#208244),(#208245,#208246),
(#208247,#208248),(#208249,#208250),(#208251,#208252),(#208253,#208254),
(#208255,#208256),(#208257,#208258),(#208259,#208260),(#208261,#208262),
(#208263,#208264),(#208265,#208266),(#208267,#208268),(#208269,#208270),
(#208271,#208272),(#208273,#208274),(#208275,#208276),(#208277,#208278),
(#208279,#208280),(#208281,#208282),(#208283,#208284),(#208285,#208286),
(#208287,#208288),(#208289,#208290),(#208291,#208292),(#208293,#208294),
(#208295,#208296),(#208297,#208298)),.UNSPECIFIED.,.F.,.F.,.F.)
B_SPLINE_SURFACE_WITH_KNOTS((6,1,1,1,1,1,1,1,1,1,1,1,1,1,1,1,1,1,1,1,1,
1,1,1,1,1,1,1,1,1,1,1,1,1,1,1,1,1,1,1,1,1,1,1,1,1,1,1,1,1,1,1,1,1,1,1,1,
1,1,1,1,1,1,1,1,1,1,1,1,1,1,1,1,1,1,1,1,1,1,1,1,1,1,1,1,1,1,1,1,1,1,1,1,
1,1,1,1,1,1,1,1,1,1,1,1,1,1,1,1,1,1,1,1,1,1,1,1,1,1,1,1,1,1,1,1,1,1,1,1,
1,1,1,1,1,1,1,1,1,1,1,1,1,1,1,1,1,1,1,1,1,1,1,1,1,1,1,1,1,1,1,1,1,1,1,1,
1,1,1,1,1,1,1,1,1,1,1,1,1,1,1,1,1,1,1,1,1,1,1,1,1,1,1,1,1,1,1,1,1,1,1,6),
(2,2),(-1.,-0.995000000000001,-0.990000000000001,-0.985000000000001,-0.980000000000001,
-0.975000000000001,-0.970000000000001,-0.965000000000001,-0.960000000000001,
-0.955000000000001,-0.950000000000001,-0.945000000000001,-0.940000000000001,
-0.935000000000001,-0.930000000000001,-0.925000000000001,-0.920000000000001,
-0.915000000000001,-0.910000000000001,-0.905000000000001,-0.900000000000001,
-0.895000000000001,-0.890000000000001,-0.885000000000001,-0.880000000000001,
-0.875000000000001,-0.870000000000001,-0.865000000000001,-0.860000000000001,
-0.855000000000001,-0.850000000000001,-0.845000000000001,-0.840000000000001,
-0.835000000000001,-0.830000000000001,-0.825000000000001,-0.820000000000001,
-0.815000000000001,-0.810000000000001,-0.805000000000001,-0.800000000000001,
-0.795000000000001,-0.790000000000001,-0.785000000000001,-0.780000000000001,
-0.775000000000001,-0.770000000000001,-0.765000000000001,-0.760000000000001,
-0.755000000000001,-0.750000000000001,-0.745000000000001,-0.740000000000001,
-0.735000000000001,-0.730000000000001,-0.725000000000001,-0.720000000000001,
-0.715000000000001,-0.710000000000001,-0.705000000000001,-0.700000000000001,
-0.695000000000001,-0.690000000000001,-0.685,-0.68,-0.675,-0.67,-0.665,
-0.66,-0.655,-0.65,-0.645,-0.64,-0.635,-0.63,-0.625,-0.62,-0.615,-0.61,
-0.605,-0.6,-0.595,-0.59,-0.585,-0.58,-0.575,-0.57,-0.565,-0.56,-0.555,
-0.55,-0.545,-0.54,-0.535,-0.53,-0.525,-0.52,-0.515,-0.51,-0.505,-0.5,-0.495,
-0.49,-0.485,-0.48,-0.475,-0.47,-0.465,-0.46,-0.455,-0.45,-0.445,-0.44,
-0.435,-0.43,-0.425,-0.42,-0.415,-0.41,-0.405,-0.4,-0.395,-0.39,-0.385,
-0.38,-0.375,-0.37,-0.365,-0.36,-0.355,-0.35,-0.345,-0.34,-0.335,-0.33,
-0.325,-0.32,-0.315,-0.31,-0.305,-0.3,-0.295,-0.29,-0.285,-0.28,-0.275,
-0.27,-0.265,-0.26,-0.255,-0.25,-0.245,-0.24,-0.235,-0.23,-0.225,-0.22,
-0.215,-0.21,-0.205,-0.2,-0.195,-0.19,-0.185,-0.18,-0.175,-0.17,-0.165,
-0.16,-0.155,-0.15,-0.145,-0.14,-0.135,-0.13,-0.125,-0.12,-0.115,-0.11,
-0.105,-0.1,-0.095,-0.09,-0.085,-0.08,-0.075,-0.07,-0.065,-0.06,-0.055,
-0.05,-0.045,-0.04,-0.035,-0.03,-0.025,-0.02,-0.015,-0.01,-0.005,0.),(0.,
1.2),.UNSPECIFIED.)
GEOMETRIC_REPRESENTATION_ITEM()
RATIONAL_B_SPLINE_SURFACE(((1.,1.),(1.,1.),(1.,1.),(1.,1.),(1.,1.),(1.,
1.),(1.,1.),(1.,1.),(1.,1.),(1.,1.),(1.,1.),(1.,1.),(1.,1.),(1.,1.),(1.,
1.),(1.,1.),(1.,1.),(1.,1.),(1.,1.),(1.,1.),(1.,1.),(1.,1.),(1.,1.),(1.,
1.),(1.,1.),(1.,1.),(1.,1.),(1.,1.),(1.,1.),(1.,1.),(1.,1.),(1.,1.),(1.,
1.),(1.,1.),(1.,1.),(1.,1.),(1.,1.),(1.,1.),(1.,1.),(1.,1.),(1.,1.),(1.,
1.),(1.,1.),(1.,1.),(1.,1.),(1.,1.),(1.,1.),(1.,1.),(1.,1.),(1.,1.),(1.,
1.),(1.,1.),(1.,1.),(1.,1.),(1.,1.),(1.,1.),(1.,1.),(1.,1.),(1.,1.),(1.,
1.),(1.,1.),(1.,1.),(1.,1.),(1.,1.),(1.,1.),(1.,1.),(1.,1.),(1.,1.),(1.,
1.),(1.,1.),(1.,1.),(1.,1.),(1.,1.),(1.,1.),(1.,1.),(1.,1.),(1.,1.),(1.,
1.),(1.,1.),(1.,1.),(1.,1.),(1.,1.),(1.,1.),(1.,1.),(1.,1.),(1.,1.),(1.,
1.),(1.,1.),(1.,1.),(1.,1.),(1.,1.),(1.,1.),(1.,1.),(1.,1.),(1.,1.),(1.,
1.),(1.,1.),(1.,1.),(1.,1.),(1.,1.),(1.,1.),(1.,1.),(1.,1.),(1.,1.),(1.,
1.),(1.,1.),(1.,1.),(1.,1.),(1.,1.),(1.,1.),(1.,1.),(1.,1.),(1.,1.),(1.,
1.),(1.,1.),(1.,1.),(1.,1.),(1.,1.),(1.,1.),(1.,1.),(1.,1.),(1.,1.),(1.,
1.),(1.,1.),(1.,1.),(1.,1.),(1.,1.),(1.,1.),(1.,1.),(1.,1.),(1.,1.),(1.,
1.),(1.,1.),(1.,1.),(1.,1.),(1.,1.),(1.,1.),(1.,1.),(1.,1.),(1.,1.),(1.,
1.),(1.,1.),(1.,1.),(1.,1.),(1.,1.),(1.,1.),(1.,1.),(1.,1.),(1.,1.),(1.,
1.),(1.,1.),(1.,1.),(1.,1.),(1.,1.),(1.,1.),(1.,1.),(1.,1.),(1.,1.),(1.,
1.),(1.,1.),(1.,1.),(1.,1.),(1.,1.),(1.,1.),(1.,1.),(1.,1.),(1.,1.),(1.,
1.),(1.,1.),(1.,1.),(1.,1.),(1.,1.),(1.,1.),(1.,1.),(1.,1.),(1.,1.),(1.,
1.),(1.,1.),(1.,1.),(1.,1.),(1.,1.),(1.,1.),(1.,1.),(1.,1.),(1.,1.),(1.,
1.),(1.,1.),(1.,1.),(1.,1.),(1.,1.),(1.,1.),(1.,1.),(1.,1.),(1.,1.),(1.,
1.),(1.,1.),(1.,1.),(1.,1.),(1.,1.),(1.,1.),(1.,1.),(1.,1.),(1.,1.),(1.,
1.),(1.,1.)))
REPRESENTATION_ITEM('')
SURFACE()
);
#1064=(
BOUNDED_SURFACE()
B_SPLINE_SURFACE(5,1,((#208506,#208507),(#208508,#208509),(#208510,#208511),
(#208512,#208513),(#208514,#208515),(#208516,#208517),(#208518,#208519),
(#208520,#208521),(#208522,#208523),(#208524,#208525),(#208526,#208527),
(#208528,#208529),(#208530,#208531),(#208532,#208533),(#208534,#208535),
(#208536,#208537),(#208538,#208539),(#208540,#208541),(#208542,#208543),
(#208544,#208545),(#208546,#208547),(#208548,#208549),(#208550,#208551),
(#208552,#208553),(#208554,#208555),(#208556,#208557),(#208558,#208559),
(#208560,#208561),(#208562,#208563),(#208564,#208565),(#208566,#208567),
(#208568,#208569),(#208570,#208571),(#208572,#208573),(#208574,#208575),
(#208576,#208577),(#208578,#208579),(#208580,#208581),(#208582,#208583),
(#208584,#208585),(#208586,#208587),(#208588,#208589),(#208590,#208591),
(#208592,#208593),(#208594,#208595),(#208596,#208597),(#208598,#208599),
(#208600,#208601),(#208602,#208603),(#208604,#208605),(#208606,#208607),
(#208608,#208609),(#208610,#208611),(#208612,#208613),(#208614,#208615),
(#208616,#208617),(#208618,#208619),(#208620,#208621),(#208622,#208623),
(#208624,#208625),(#208626,#208627),(#208628,#208629),(#208630,#208631),
(#208632,#208633),(#208634,#208635),(#208636,#208637),(#208638,#208639),
(#208640,#208641),(#208642,#208643),(#208644,#208645),(#208646,#208647),
(#208648,#208649),(#208650,#208651),(#208652,#208653),(#208654,#208655),
(#208656,#208657),(#208658,#208659),(#208660,#208661),(#208662,#208663),
(#208664,#208665),(#208666,#208667),(#208668,#208669),(#208670,#208671),
(#208672,#208673),(#208674,#208675),(#208676,#208677),(#208678,#208679),
(#208680,#208681),(#208682,#208683),(#208684,#208685),(#208686,#208687),
(#208688,#208689),(#208690,#208691),(#208692,#208693),(#208694,#208695),
(#208696,#208697),(#208698,#208699),(#208700,#208701),(#208702,#208703),
(#208704,#208705),(#208706,#208707),(#208708,#208709),(#208710,#208711),
(#208712,#208713),(#208714,#208715),(#208716,#208717),(#208718,#208719),
(#208720,#208721),(#208722,#208723),(#208724,#208725),(#208726,#208727),
(#208728,#208729),(#208730,#208731),(#208732,#208733),(#208734,#208735),
(#208736,#208737),(#208738,#208739),(#208740,#208741),(#208742,#208743),
(#208744,#208745),(#208746,#208747),(#208748,#208749),(#208750,#208751),
(#208752,#208753),(#208754,#208755),(#208756,#208757),(#208758,#208759),
(#208760,#208761),(#208762,#208763),(#208764,#208765),(#208766,#208767),
(#208768,#208769),(#208770,#208771),(#208772,#208773),(#208774,#208775),
(#208776,#208777),(#208778,#208779),(#208780,#208781),(#208782,#208783),
(#208784,#208785),(#208786,#208787),(#208788,#208789),(#208790,#208791),
(#208792,#208793),(#208794,#208795),(#208796,#208797),(#208798,#208799),
(#208800,#208801),(#208802,#208803),(#208804,#208805),(#208806,#208807),
(#208808,#208809),(#208810,#208811),(#208812,#208813),(#208814,#208815),
(#208816,#208817),(#208818,#208819),(#208820,#208821),(#208822,#208823),
(#208824,#208825),(#208826,#208827),(#208828,#208829),(#208830,#208831),
(#208832,#208833),(#208834,#208835),(#208836,#208837),(#208838,#208839),
(#208840,#208841),(#208842,#208843),(#208844,#208845),(#208846,#208847),
(#208848,#208849),(#208850,#208851),(#208852,#208853),(#208854,#208855),
(#208856,#208857),(#208858,#208859),(#208860,#208861),(#208862,#208863),
(#208864,#208865),(#208866,#208867),(#208868,#208869),(#208870,#208871),
(#208872,#208873),(#208874,#208875),(#208876,#208877),(#208878,#208879),
(#208880,#208881),(#208882,#208883),(#208884,#208885),(#208886,#208887),
(#208888,#208889),(#208890,#208891),(#208892,#208893),(#208894,#208895),
(#208896,#208897),(#208898,#208899),(#208900,#208901),(#208902,#208903),
(#208904,#208905),(#208906,#208907),(#208908,#208909),(#208910,#208911),
(#208912,#208913),(#208914,#208915)),.UNSPECIFIED.,.F.,.F.,.F.)
B_SPLINE_SURFACE_WITH_KNOTS((6,1,1,1,1,1,1,1,1,1,1,1,1,1,1,1,1,1,1,1,1,
1,1,1,1,1,1,1,1,1,1,1,1,1,1,1,1,1,1,1,1,1,1,1,1,1,1,1,1,1,1,1,1,1,1,1,1,
1,1,1,1,1,1,1,1,1,1,1,1,1,1,1,1,1,1,1,1,1,1,1,1,1,1,1,1,1,1,1,1,1,1,1,1,
1,1,1,1,1,1,1,1,1,1,1,1,1,1,1,1,1,1,1,1,1,1,1,1,1,1,1,1,1,1,1,1,1,1,1,1,
1,1,1,1,1,1,1,1,1,1,1,1,1,1,1,1,1,1,1,1,1,1,1,1,1,1,1,1,1,1,1,1,1,1,1,1,
1,1,1,1,1,1,1,1,1,1,1,1,1,1,1,1,1,1,1,1,1,1,1,1,1,1,1,1,1,1,1,1,1,1,1,6),
(2,2),(0.,0.005,0.01,0.015,0.02,0.025,0.03,0.035,0.04,0.045,0.05,0.055,
0.06,0.065,0.07,0.075,0.08,0.085,0.09,0.095,0.1,0.105,0.11,0.115,0.12,0.125,
0.13,0.135,0.14,0.145,0.15,0.155,0.16,0.165,0.17,0.175,0.18,0.185,0.19,
0.195,0.2,0.205,0.21,0.215,0.22,0.225,0.23,0.235,0.24,0.245,0.25,0.255,
0.26,0.265,0.27,0.275,0.28,0.285,0.29,0.295,0.3,0.305,0.31,0.315,0.32,0.325,
0.33,0.335,0.34,0.345,0.35,0.355,0.36,0.365,0.37,0.375,0.38,0.385,0.39,
0.395,0.4,0.405,0.41,0.415,0.42,0.425,0.43,0.435,0.44,0.445,0.45,0.455,
0.46,0.465,0.47,0.475,0.48,0.485,0.49,0.495,0.5,0.505,0.51,0.515,0.52,0.525,
0.53,0.535,0.54,0.545,0.55,0.555,0.56,0.565,0.57,0.575,0.58,0.585,0.59,
0.595,0.6,0.605,0.61,0.615,0.62,0.625,0.63,0.635,0.64,0.645,0.65,0.655,
0.66,0.665,0.67,0.675,0.68,0.685,0.690000000000001,0.695000000000001,0.700000000000001,
0.705000000000001,0.710000000000001,0.715000000000001,0.720000000000001,
0.725000000000001,0.730000000000001,0.735000000000001,0.740000000000001,
0.745000000000001,0.750000000000001,0.755000000000001,0.760000000000001,
0.765000000000001,0.770000000000001,0.775000000000001,0.780000000000001,
0.785000000000001,0.790000000000001,0.795000000000001,0.800000000000001,
0.805000000000001,0.810000000000001,0.815000000000001,0.820000000000001,
0.825000000000001,0.830000000000001,0.835000000000001,0.840000000000001,
0.845000000000001,0.850000000000001,0.855000000000001,0.860000000000001,
0.865000000000001,0.870000000000001,0.875000000000001,0.880000000000001,
0.885000000000001,0.890000000000001,0.895000000000001,0.900000000000001,
0.905000000000001,0.910000000000001,0.915000000000001,0.920000000000001,
0.925000000000001,0.930000000000001,0.935000000000001,0.940000000000001,
0.945000000000001,0.950000000000001,0.955000000000001,0.960000000000001,
0.965000000000001,0.970000000000001,0.975000000000001,0.980000000000001,
0.985000000000001,0.990000000000001,0.995000000000001,1.),(0.,1.2),
 .UNSPECIFIED.)
GEOMETRIC_REPRESENTATION_ITEM()
RATIONAL_B_SPLINE_SURFACE(((1.,1.),(1.,1.),(1.,1.),(1.,1.),(1.,1.),(1.,
1.),(1.,1.),(1.,1.),(1.,1.),(1.,1.),(1.,1.),(1.,1.),(1.,1.),(1.,1.),(1.,
1.),(1.,1.),(1.,1.),(1.,1.),(1.,1.),(1.,1.),(1.,1.),(1.,1.),(1.,1.),(1.,
1.),(1.,1.),(1.,1.),(1.,1.),(1.,1.),(1.,1.),(1.,1.),(1.,1.),(1.,1.),(1.,
1.),(1.,1.),(1.,1.),(1.,1.),(1.,1.),(1.,1.),(1.,1.),(1.,1.),(1.,1.),(1.,
1.),(1.,1.),(1.,1.),(1.,1.),(1.,1.),(1.,1.),(1.,1.),(1.,1.),(1.,1.),(1.,
1.),(1.,1.),(1.,1.),(1.,1.),(1.,1.),(1.,1.),(1.,1.),(1.,1.),(1.,1.),(1.,
1.),(1.,1.),(1.,1.),(1.,1.),(1.,1.),(1.,1.),(1.,1.),(1.,1.),(1.,1.),(1.,
1.),(1.,1.),(1.,1.),(1.,1.),(1.,1.),(1.,1.),(1.,1.),(1.,1.),(1.,1.),(1.,
1.),(1.,1.),(1.,1.),(1.,1.),(1.,1.),(1.,1.),(1.,1.),(1.,1.),(1.,1.),(1.,
1.),(1.,1.),(1.,1.),(1.,1.),(1.,1.),(1.,1.),(1.,1.),(1.,1.),(1.,1.),(1.,
1.),(1.,1.),(1.,1.),(1.,1.),(1.,1.),(1.,1.),(1.,1.),(1.,1.),(1.,1.),(1.,
1.),(1.,1.),(1.,1.),(1.,1.),(1.,1.),(1.,1.),(1.,1.),(1.,1.),(1.,1.),(1.,
1.),(1.,1.),(1.,1.),(1.,1.),(1.,1.),(1.,1.),(1.,1.),(1.,1.),(1.,1.),(1.,
1.),(1.,1.),(1.,1.),(1.,1.),(1.,1.),(1.,1.),(1.,1.),(1.,1.),(1.,1.),(1.,
1.),(1.,1.),(1.,1.),(1.,1.),(1.,1.),(1.,1.),(1.,1.),(1.,1.),(1.,1.),(1.,
1.),(1.,1.),(1.,1.),(1.,1.),(1.,1.),(1.,1.),(1.,1.),(1.,1.),(1.,1.),(1.,
1.),(1.,1.),(1.,1.),(1.,1.),(1.,1.),(1.,1.),(1.,1.),(1.,1.),(1.,1.),(1.,
1.),(1.,1.),(1.,1.),(1.,1.),(1.,1.),(1.,1.),(1.,1.),(1.,1.),(1.,1.),(1.,
1.),(1.,1.),(1.,1.),(1.,1.),(1.,1.),(1.,1.),(1.,1.),(1.,1.),(1.,1.),(1.,
1.),(1.,1.),(1.,1.),(1.,1.),(1.,1.),(1.,1.),(1.,1.),(1.,1.),(1.,1.),(1.,
1.),(1.,1.),(1.,1.),(1.,1.),(1.,1.),(1.,1.),(1.,1.),(1.,1.),(1.,1.),(1.,
1.),(1.,1.),(1.,1.),(1.,1.),(1.,1.),(1.,1.),(1.,1.),(1.,1.),(1.,1.),(1.,
1.),(1.,1.)))
REPRESENTATION_ITEM('')
SURFACE()
);
#1065=(
BOUNDED_SURFACE()
B_SPLINE_SURFACE(5,1,((#209127,#209128),(#209129,#209130),(#209131,#209132),
(#209133,#209134),(#209135,#209136),(#209137,#209138),(#209139,#209140),
(#209141,#209142),(#209143,#209144),(#209145,#209146),(#209147,#209148),
(#209149,#209150),(#209151,#209152),(#209153,#209154),(#209155,#209156),
(#209157,#209158),(#209159,#209160),(#209161,#209162),(#209163,#209164),
(#209165,#209166),(#209167,#209168),(#209169,#209170),(#209171,#209172),
(#209173,#209174),(#209175,#209176),(#209177,#209178),(#209179,#209180),
(#209181,#209182),(#209183,#209184),(#209185,#209186),(#209187,#209188),
(#209189,#209190),(#209191,#209192),(#209193,#209194),(#209195,#209196),
(#209197,#209198),(#209199,#209200),(#209201,#209202),(#209203,#209204),
(#209205,#209206),(#209207,#209208),(#209209,#209210),(#209211,#209212),
(#209213,#209214),(#209215,#209216),(#209217,#209218),(#209219,#209220),
(#209221,#209222),(#209223,#209224),(#209225,#209226),(#209227,#209228),
(#209229,#209230),(#209231,#209232),(#209233,#209234),(#209235,#209236),
(#209237,#209238),(#209239,#209240),(#209241,#209242),(#209243,#209244),
(#209245,#209246),(#209247,#209248),(#209249,#209250),(#209251,#209252),
(#209253,#209254),(#209255,#209256),(#209257,#209258),(#209259,#209260),
(#209261,#209262),(#209263,#209264),(#209265,#209266),(#209267,#209268),
(#209269,#209270),(#209271,#209272),(#209273,#209274),(#209275,#209276),
(#209277,#209278),(#209279,#209280),(#209281,#209282),(#209283,#209284),
(#209285,#209286),(#209287,#209288),(#209289,#209290),(#209291,#209292),
(#209293,#209294),(#209295,#209296),(#209297,#209298),(#209299,#209300),
(#209301,#209302),(#209303,#209304),(#209305,#209306),(#209307,#209308),
(#209309,#209310),(#209311,#209312),(#209313,#209314),(#209315,#209316),
(#209317,#209318),(#209319,#209320),(#209321,#209322),(#209323,#209324),
(#209325,#209326),(#209327,#209328),(#209329,#209330),(#209331,#209332),
(#209333,#209334),(#209335,#209336),(#209337,#209338),(#209339,#209340),
(#209341,#209342),(#209343,#209344),(#209345,#209346),(#209347,#209348),
(#209349,#209350),(#209351,#209352),(#209353,#209354),(#209355,#209356),
(#209357,#209358),(#209359,#209360),(#209361,#209362),(#209363,#209364),
(#209365,#209366),(#209367,#209368),(#209369,#209370),(#209371,#209372),
(#209373,#209374),(#209375,#209376),(#209377,#209378),(#209379,#209380),
(#209381,#209382),(#209383,#209384),(#209385,#209386),(#209387,#209388),
(#209389,#209390),(#209391,#209392),(#209393,#209394),(#209395,#209396),
(#209397,#209398),(#209399,#209400),(#209401,#209402),(#209403,#209404),
(#209405,#209406),(#209407,#209408),(#209409,#209410),(#209411,#209412),
(#209413,#209414),(#209415,#209416),(#209417,#209418),(#209419,#209420),
(#209421,#209422),(#209423,#209424),(#209425,#209426),(#209427,#209428),
(#209429,#209430),(#209431,#209432),(#209433,#209434),(#209435,#209436),
(#209437,#209438),(#209439,#209440),(#209441,#209442),(#209443,#209444),
(#209445,#209446),(#209447,#209448),(#209449,#209450),(#209451,#209452),
(#209453,#209454),(#209455,#209456),(#209457,#209458),(#209459,#209460),
(#209461,#209462),(#209463,#209464),(#209465,#209466),(#209467,#209468),
(#209469,#209470),(#209471,#209472),(#209473,#209474),(#209475,#209476),
(#209477,#209478),(#209479,#209480),(#209481,#209482),(#209483,#209484),
(#209485,#209486),(#209487,#209488),(#209489,#209490),(#209491,#209492),
(#209493,#209494),(#209495,#209496),(#209497,#209498),(#209499,#209500),
(#209501,#209502),(#209503,#209504),(#209505,#209506),(#209507,#209508),
(#209509,#209510),(#209511,#209512),(#209513,#209514),(#209515,#209516),
(#209517,#209518),(#209519,#209520),(#209521,#209522),(#209523,#209524),
(#209525,#209526),(#209527,#209528),(#209529,#209530),(#209531,#209532),
(#209533,#209534),(#209535,#209536)),.UNSPECIFIED.,.F.,.F.,.F.)
B_SPLINE_SURFACE_WITH_KNOTS((6,1,1,1,1,1,1,1,1,1,1,1,1,1,1,1,1,1,1,1,1,
1,1,1,1,1,1,1,1,1,1,1,1,1,1,1,1,1,1,1,1,1,1,1,1,1,1,1,1,1,1,1,1,1,1,1,1,
1,1,1,1,1,1,1,1,1,1,1,1,1,1,1,1,1,1,1,1,1,1,1,1,1,1,1,1,1,1,1,1,1,1,1,1,
1,1,1,1,1,1,1,1,1,1,1,1,1,1,1,1,1,1,1,1,1,1,1,1,1,1,1,1,1,1,1,1,1,1,1,1,
1,1,1,1,1,1,1,1,1,1,1,1,1,1,1,1,1,1,1,1,1,1,1,1,1,1,1,1,1,1,1,1,1,1,1,1,
1,1,1,1,1,1,1,1,1,1,1,1,1,1,1,1,1,1,1,1,1,1,1,1,1,1,1,1,1,1,1,1,1,1,1,6),
(2,2),(-1.,-0.995000000000001,-0.990000000000001,-0.985000000000001,-0.980000000000001,
-0.975000000000001,-0.970000000000001,-0.965000000000001,-0.960000000000001,
-0.955000000000001,-0.950000000000001,-0.945000000000001,-0.940000000000001,
-0.935000000000001,-0.930000000000001,-0.925000000000001,-0.920000000000001,
-0.915000000000001,-0.910000000000001,-0.905000000000001,-0.900000000000001,
-0.895000000000001,-0.890000000000001,-0.885000000000001,-0.880000000000001,
-0.875000000000001,-0.870000000000001,-0.865000000000001,-0.860000000000001,
-0.855000000000001,-0.850000000000001,-0.845000000000001,-0.840000000000001,
-0.835000000000001,-0.830000000000001,-0.825000000000001,-0.820000000000001,
-0.815000000000001,-0.810000000000001,-0.805000000000001,-0.800000000000001,
-0.795000000000001,-0.790000000000001,-0.785000000000001,-0.780000000000001,
-0.775000000000001,-0.770000000000001,-0.765000000000001,-0.760000000000001,
-0.755000000000001,-0.750000000000001,-0.745000000000001,-0.740000000000001,
-0.735000000000001,-0.730000000000001,-0.725000000000001,-0.720000000000001,
-0.715000000000001,-0.710000000000001,-0.705000000000001,-0.700000000000001,
-0.695000000000001,-0.690000000000001,-0.685,-0.68,-0.675,-0.67,-0.665,
-0.66,-0.655,-0.65,-0.645,-0.64,-0.635,-0.63,-0.625,-0.62,-0.615,-0.61,
-0.605,-0.6,-0.595,-0.59,-0.585,-0.58,-0.575,-0.57,-0.565,-0.56,-0.555,
-0.55,-0.545,-0.54,-0.535,-0.53,-0.525,-0.52,-0.515,-0.51,-0.505,-0.5,-0.495,
-0.49,-0.485,-0.48,-0.475,-0.47,-0.465,-0.46,-0.455,-0.45,-0.445,-0.44,
-0.435,-0.43,-0.425,-0.42,-0.415,-0.41,-0.405,-0.4,-0.395,-0.39,-0.385,
-0.38,-0.375,-0.37,-0.365,-0.36,-0.355,-0.35,-0.345,-0.34,-0.335,-0.33,
-0.325,-0.32,-0.315,-0.31,-0.305,-0.3,-0.295,-0.29,-0.285,-0.28,-0.275,
-0.27,-0.265,-0.26,-0.255,-0.25,-0.245,-0.24,-0.235,-0.23,-0.225,-0.22,
-0.215,-0.21,-0.205,-0.2,-0.195,-0.19,-0.185,-0.18,-0.175,-0.17,-0.165,
-0.16,-0.155,-0.15,-0.145,-0.14,-0.135,-0.13,-0.125,-0.12,-0.115,-0.11,
-0.105,-0.1,-0.095,-0.09,-0.085,-0.08,-0.075,-0.07,-0.065,-0.06,-0.055,
-0.05,-0.045,-0.04,-0.035,-0.03,-0.025,-0.02,-0.015,-0.01,-0.005,0.),(0.,
1.2),.UNSPECIFIED.)
GEOMETRIC_REPRESENTATION_ITEM()
RATIONAL_B_SPLINE_SURFACE(((1.,1.),(1.,1.),(1.,1.),(1.,1.),(1.,1.),(1.,
1.),(1.,1.),(1.,1.),(1.,1.),(1.,1.),(1.,1.),(1.,1.),(1.,1.),(1.,1.),(1.,
1.),(1.,1.),(1.,1.),(1.,1.),(1.,1.),(1.,1.),(1.,1.),(1.,1.),(1.,1.),(1.,
1.),(1.,1.),(1.,1.),(1.,1.),(1.,1.),(1.,1.),(1.,1.),(1.,1.),(1.,1.),(1.,
1.),(1.,1.),(1.,1.),(1.,1.),(1.,1.),(1.,1.),(1.,1.),(1.,1.),(1.,1.),(1.,
1.),(1.,1.),(1.,1.),(1.,1.),(1.,1.),(1.,1.),(1.,1.),(1.,1.),(1.,1.),(1.,
1.),(1.,1.),(1.,1.),(1.,1.),(1.,1.),(1.,1.),(1.,1.),(1.,1.),(1.,1.),(1.,
1.),(1.,1.),(1.,1.),(1.,1.),(1.,1.),(1.,1.),(1.,1.),(1.,1.),(1.,1.),(1.,
1.),(1.,1.),(1.,1.),(1.,1.),(1.,1.),(1.,1.),(1.,1.),(1.,1.),(1.,1.),(1.,
1.),(1.,1.),(1.,1.),(1.,1.),(1.,1.),(1.,1.),(1.,1.),(1.,1.),(1.,1.),(1.,
1.),(1.,1.),(1.,1.),(1.,1.),(1.,1.),(1.,1.),(1.,1.),(1.,1.),(1.,1.),(1.,
1.),(1.,1.),(1.,1.),(1.,1.),(1.,1.),(1.,1.),(1.,1.),(1.,1.),(1.,1.),(1.,
1.),(1.,1.),(1.,1.),(1.,1.),(1.,1.),(1.,1.),(1.,1.),(1.,1.),(1.,1.),(1.,
1.),(1.,1.),(1.,1.),(1.,1.),(1.,1.),(1.,1.),(1.,1.),(1.,1.),(1.,1.),(1.,
1.),(1.,1.),(1.,1.),(1.,1.),(1.,1.),(1.,1.),(1.,1.),(1.,1.),(1.,1.),(1.,
1.),(1.,1.),(1.,1.),(1.,1.),(1.,1.),(1.,1.),(1.,1.),(1.,1.),(1.,1.),(1.,
1.),(1.,1.),(1.,1.),(1.,1.),(1.,1.),(1.,1.),(1.,1.),(1.,1.),(1.,1.),(1.,
1.),(1.,1.),(1.,1.),(1.,1.),(1.,1.),(1.,1.),(1.,1.),(1.,1.),(1.,1.),(1.,
1.),(1.,1.),(1.,1.),(1.,1.),(1.,1.),(1.,1.),(1.,1.),(1.,1.),(1.,1.),(1.,
1.),(1.,1.),(1.,1.),(1.,1.),(1.,1.),(1.,1.),(1.,1.),(1.,1.),(1.,1.),(1.,
1.),(1.,1.),(1.,1.),(1.,1.),(1.,1.),(1.,1.),(1.,1.),(1.,1.),(1.,1.),(1.,
1.),(1.,1.),(1.,1.),(1.,1.),(1.,1.),(1.,1.),(1.,1.),(1.,1.),(1.,1.),(1.,
1.),(1.,1.),(1.,1.),(1.,1.),(1.,1.),(1.,1.),(1.,1.),(1.,1.),(1.,1.),(1.,
1.),(1.,1.)))
REPRESENTATION_ITEM('')
SURFACE()
);
#1066=(
BOUNDED_SURFACE()
B_SPLINE_SURFACE(5,1,((#209744,#209745),(#209746,#209747),(#209748,#209749),
(#209750,#209751),(#209752,#209753),(#209754,#209755),(#209756,#209757),
(#209758,#209759),(#209760,#209761),(#209762,#209763),(#209764,#209765),
(#209766,#209767),(#209768,#209769),(#209770,#209771),(#209772,#209773),
(#209774,#209775),(#209776,#209777),(#209778,#209779),(#209780,#209781),
(#209782,#209783),(#209784,#209785),(#209786,#209787),(#209788,#209789),
(#209790,#209791),(#209792,#209793),(#209794,#209795),(#209796,#209797),
(#209798,#209799),(#209800,#209801),(#209802,#209803),(#209804,#209805),
(#209806,#209807),(#209808,#209809),(#209810,#209811),(#209812,#209813),
(#209814,#209815),(#209816,#209817),(#209818,#209819),(#209820,#209821),
(#209822,#209823),(#209824,#209825),(#209826,#209827),(#209828,#209829),
(#209830,#209831),(#209832,#209833),(#209834,#209835),(#209836,#209837),
(#209838,#209839),(#209840,#209841),(#209842,#209843),(#209844,#209845),
(#209846,#209847),(#209848,#209849),(#209850,#209851),(#209852,#209853),
(#209854,#209855),(#209856,#209857),(#209858,#209859),(#209860,#209861),
(#209862,#209863),(#209864,#209865),(#209866,#209867),(#209868,#209869),
(#209870,#209871),(#209872,#209873),(#209874,#209875),(#209876,#209877),
(#209878,#209879),(#209880,#209881),(#209882,#209883),(#209884,#209885),
(#209886,#209887),(#209888,#209889),(#209890,#209891),(#209892,#209893),
(#209894,#209895),(#209896,#209897),(#209898,#209899),(#209900,#209901),
(#209902,#209903),(#209904,#209905),(#209906,#209907),(#209908,#209909),
(#209910,#209911),(#209912,#209913),(#209914,#209915),(#209916,#209917),
(#209918,#209919),(#209920,#209921),(#209922,#209923),(#209924,#209925),
(#209926,#209927),(#209928,#209929),(#209930,#209931),(#209932,#209933),
(#209934,#209935),(#209936,#209937),(#209938,#209939),(#209940,#209941),
(#209942,#209943),(#209944,#209945),(#209946,#209947),(#209948,#209949),
(#209950,#209951),(#209952,#209953),(#209954,#209955),(#209956,#209957),
(#209958,#209959),(#209960,#209961),(#209962,#209963),(#209964,#209965),
(#209966,#209967),(#209968,#209969),(#209970,#209971),(#209972,#209973),
(#209974,#209975),(#209976,#209977),(#209978,#209979),(#209980,#209981),
(#209982,#209983),(#209984,#209985),(#209986,#209987),(#209988,#209989),
(#209990,#209991),(#209992,#209993),(#209994,#209995),(#209996,#209997),
(#209998,#209999),(#210000,#210001),(#210002,#210003),(#210004,#210005),
(#210006,#210007),(#210008,#210009),(#210010,#210011),(#210012,#210013),
(#210014,#210015),(#210016,#210017),(#210018,#210019),(#210020,#210021),
(#210022,#210023),(#210024,#210025),(#210026,#210027),(#210028,#210029),
(#210030,#210031),(#210032,#210033),(#210034,#210035),(#210036,#210037),
(#210038,#210039),(#210040,#210041),(#210042,#210043),(#210044,#210045),
(#210046,#210047),(#210048,#210049),(#210050,#210051),(#210052,#210053),
(#210054,#210055),(#210056,#210057),(#210058,#210059),(#210060,#210061),
(#210062,#210063),(#210064,#210065),(#210066,#210067),(#210068,#210069),
(#210070,#210071),(#210072,#210073),(#210074,#210075),(#210076,#210077),
(#210078,#210079),(#210080,#210081),(#210082,#210083),(#210084,#210085),
(#210086,#210087),(#210088,#210089),(#210090,#210091),(#210092,#210093),
(#210094,#210095),(#210096,#210097),(#210098,#210099),(#210100,#210101),
(#210102,#210103),(#210104,#210105),(#210106,#210107),(#210108,#210109),
(#210110,#210111),(#210112,#210113),(#210114,#210115),(#210116,#210117),
(#210118,#210119),(#210120,#210121),(#210122,#210123),(#210124,#210125),
(#210126,#210127),(#210128,#210129),(#210130,#210131),(#210132,#210133),
(#210134,#210135),(#210136,#210137),(#210138,#210139),(#210140,#210141),
(#210142,#210143),(#210144,#210145),(#210146,#210147),(#210148,#210149),
(#210150,#210151),(#210152,#210153)),.UNSPECIFIED.,.F.,.F.,.F.)
B_SPLINE_SURFACE_WITH_KNOTS((6,1,1,1,1,1,1,1,1,1,1,1,1,1,1,1,1,1,1,1,1,
1,1,1,1,1,1,1,1,1,1,1,1,1,1,1,1,1,1,1,1,1,1,1,1,1,1,1,1,1,1,1,1,1,1,1,1,
1,1,1,1,1,1,1,1,1,1,1,1,1,1,1,1,1,1,1,1,1,1,1,1,1,1,1,1,1,1,1,1,1,1,1,1,
1,1,1,1,1,1,1,1,1,1,1,1,1,1,1,1,1,1,1,1,1,1,1,1,1,1,1,1,1,1,1,1,1,1,1,1,
1,1,1,1,1,1,1,1,1,1,1,1,1,1,1,1,1,1,1,1,1,1,1,1,1,1,1,1,1,1,1,1,1,1,1,1,
1,1,1,1,1,1,1,1,1,1,1,1,1,1,1,1,1,1,1,1,1,1,1,1,1,1,1,1,1,1,1,1,1,1,1,6),
(2,2),(0.,0.005,0.01,0.015,0.02,0.025,0.03,0.035,0.04,0.045,0.05,0.055,
0.06,0.065,0.07,0.075,0.08,0.085,0.09,0.095,0.1,0.105,0.11,0.115,0.12,0.125,
0.13,0.135,0.14,0.145,0.15,0.155,0.16,0.165,0.17,0.175,0.18,0.185,0.19,
0.195,0.2,0.205,0.21,0.215,0.22,0.225,0.23,0.235,0.24,0.245,0.25,0.255,
0.26,0.265,0.27,0.275,0.28,0.285,0.29,0.295,0.3,0.305,0.31,0.315,0.32,0.325,
0.33,0.335,0.34,0.345,0.35,0.355,0.36,0.365,0.37,0.375,0.38,0.385,0.39,
0.395,0.4,0.405,0.41,0.415,0.42,0.425,0.43,0.435,0.44,0.445,0.45,0.455,
0.46,0.465,0.47,0.475,0.48,0.485,0.49,0.495,0.5,0.505,0.51,0.515,0.52,0.525,
0.53,0.535,0.54,0.545,0.55,0.555,0.56,0.565,0.57,0.575,0.58,0.585,0.59,
0.595,0.6,0.605,0.61,0.615,0.62,0.625,0.63,0.635,0.64,0.645,0.65,0.655,
0.66,0.665,0.67,0.675,0.68,0.685,0.690000000000001,0.695000000000001,0.700000000000001,
0.705000000000001,0.710000000000001,0.715000000000001,0.720000000000001,
0.725000000000001,0.730000000000001,0.735000000000001,0.740000000000001,
0.745000000000001,0.750000000000001,0.755000000000001,0.760000000000001,
0.765000000000001,0.770000000000001,0.775000000000001,0.780000000000001,
0.785000000000001,0.790000000000001,0.795000000000001,0.800000000000001,
0.805000000000001,0.810000000000001,0.815000000000001,0.820000000000001,
0.825000000000001,0.830000000000001,0.835000000000001,0.840000000000001,
0.845000000000001,0.850000000000001,0.855000000000001,0.860000000000001,
0.865000000000001,0.870000000000001,0.875000000000001,0.880000000000001,
0.885000000000001,0.890000000000001,0.895000000000001,0.900000000000001,
0.905000000000001,0.910000000000001,0.915000000000001,0.920000000000001,
0.925000000000001,0.930000000000001,0.935000000000001,0.940000000000001,
0.945000000000001,0.950000000000001,0.955000000000001,0.960000000000001,
0.965000000000001,0.970000000000001,0.975000000000001,0.980000000000001,
0.985000000000001,0.990000000000001,0.995000000000001,1.),(0.,1.2),
 .UNSPECIFIED.)
GEOMETRIC_REPRESENTATION_ITEM()
RATIONAL_B_SPLINE_SURFACE(((1.,1.),(1.,1.),(1.,1.),(1.,1.),(1.,1.),(1.,
1.),(1.,1.),(1.,1.),(1.,1.),(1.,1.),(1.,1.),(1.,1.),(1.,1.),(1.,1.),(1.,
1.),(1.,1.),(1.,1.),(1.,1.),(1.,1.),(1.,1.),(1.,1.),(1.,1.),(1.,1.),(1.,
1.),(1.,1.),(1.,1.),(1.,1.),(1.,1.),(1.,1.),(1.,1.),(1.,1.),(1.,1.),(1.,
1.),(1.,1.),(1.,1.),(1.,1.),(1.,1.),(1.,1.),(1.,1.),(1.,1.),(1.,1.),(1.,
1.),(1.,1.),(1.,1.),(1.,1.),(1.,1.),(1.,1.),(1.,1.),(1.,1.),(1.,1.),(1.,
1.),(1.,1.),(1.,1.),(1.,1.),(1.,1.),(1.,1.),(1.,1.),(1.,1.),(1.,1.),(1.,
1.),(1.,1.),(1.,1.),(1.,1.),(1.,1.),(1.,1.),(1.,1.),(1.,1.),(1.,1.),(1.,
1.),(1.,1.),(1.,1.),(1.,1.),(1.,1.),(1.,1.),(1.,1.),(1.,1.),(1.,1.),(1.,
1.),(1.,1.),(1.,1.),(1.,1.),(1.,1.),(1.,1.),(1.,1.),(1.,1.),(1.,1.),(1.,
1.),(1.,1.),(1.,1.),(1.,1.),(1.,1.),(1.,1.),(1.,1.),(1.,1.),(1.,1.),(1.,
1.),(1.,1.),(1.,1.),(1.,1.),(1.,1.),(1.,1.),(1.,1.),(1.,1.),(1.,1.),(1.,
1.),(1.,1.),(1.,1.),(1.,1.),(1.,1.),(1.,1.),(1.,1.),(1.,1.),(1.,1.),(1.,
1.),(1.,1.),(1.,1.),(1.,1.),(1.,1.),(1.,1.),(1.,1.),(1.,1.),(1.,1.),(1.,
1.),(1.,1.),(1.,1.),(1.,1.),(1.,1.),(1.,1.),(1.,1.),(1.,1.),(1.,1.),(1.,
1.),(1.,1.),(1.,1.),(1.,1.),(1.,1.),(1.,1.),(1.,1.),(1.,1.),(1.,1.),(1.,
1.),(1.,1.),(1.,1.),(1.,1.),(1.,1.),(1.,1.),(1.,1.),(1.,1.),(1.,1.),(1.,
1.),(1.,1.),(1.,1.),(1.,1.),(1.,1.),(1.,1.),(1.,1.),(1.,1.),(1.,1.),(1.,
1.),(1.,1.),(1.,1.),(1.,1.),(1.,1.),(1.,1.),(1.,1.),(1.,1.),(1.,1.),(1.,
1.),(1.,1.),(1.,1.),(1.,1.),(1.,1.),(1.,1.),(1.,1.),(1.,1.),(1.,1.),(1.,
1.),(1.,1.),(1.,1.),(1.,1.),(1.,1.),(1.,1.),(1.,1.),(1.,1.),(1.,1.),(1.,
1.),(1.,1.),(1.,1.),(1.,1.),(1.,1.),(1.,1.),(1.,1.),(1.,1.),(1.,1.),(1.,
1.),(1.,1.),(1.,1.),(1.,1.),(1.,1.),(1.,1.),(1.,1.),(1.,1.),(1.,1.),(1.,
1.),(1.,1.)))
REPRESENTATION_ITEM('')
SURFACE()
);
#1067=(
BOUNDED_SURFACE()
B_SPLINE_SURFACE(5,1,((#210365,#210366),(#210367,#210368),(#210369,#210370),
(#210371,#210372),(#210373,#210374),(#210375,#210376),(#210377,#210378),
(#210379,#210380),(#210381,#210382),(#210383,#210384),(#210385,#210386),
(#210387,#210388),(#210389,#210390),(#210391,#210392),(#210393,#210394),
(#210395,#210396),(#210397,#210398),(#210399,#210400),(#210401,#210402),
(#210403,#210404),(#210405,#210406),(#210407,#210408),(#210409,#210410),
(#210411,#210412),(#210413,#210414),(#210415,#210416),(#210417,#210418),
(#210419,#210420),(#210421,#210422),(#210423,#210424),(#210425,#210426),
(#210427,#210428),(#210429,#210430),(#210431,#210432),(#210433,#210434),
(#210435,#210436),(#210437,#210438),(#210439,#210440),(#210441,#210442),
(#210443,#210444),(#210445,#210446),(#210447,#210448),(#210449,#210450),
(#210451,#210452),(#210453,#210454),(#210455,#210456),(#210457,#210458),
(#210459,#210460),(#210461,#210462),(#210463,#210464),(#210465,#210466),
(#210467,#210468),(#210469,#210470),(#210471,#210472),(#210473,#210474),
(#210475,#210476),(#210477,#210478),(#210479,#210480),(#210481,#210482),
(#210483,#210484),(#210485,#210486),(#210487,#210488),(#210489,#210490),
(#210491,#210492),(#210493,#210494),(#210495,#210496),(#210497,#210498),
(#210499,#210500),(#210501,#210502),(#210503,#210504),(#210505,#210506),
(#210507,#210508),(#210509,#210510),(#210511,#210512),(#210513,#210514),
(#210515,#210516),(#210517,#210518),(#210519,#210520),(#210521,#210522),
(#210523,#210524),(#210525,#210526),(#210527,#210528),(#210529,#210530),
(#210531,#210532),(#210533,#210534),(#210535,#210536),(#210537,#210538),
(#210539,#210540),(#210541,#210542),(#210543,#210544),(#210545,#210546),
(#210547,#210548),(#210549,#210550),(#210551,#210552),(#210553,#210554),
(#210555,#210556),(#210557,#210558),(#210559,#210560),(#210561,#210562),
(#210563,#210564),(#210565,#210566),(#210567,#210568),(#210569,#210570),
(#210571,#210572),(#210573,#210574),(#210575,#210576),(#210577,#210578),
(#210579,#210580),(#210581,#210582),(#210583,#210584),(#210585,#210586),
(#210587,#210588),(#210589,#210590),(#210591,#210592),(#210593,#210594),
(#210595,#210596),(#210597,#210598),(#210599,#210600),(#210601,#210602),
(#210603,#210604),(#210605,#210606),(#210607,#210608),(#210609,#210610),
(#210611,#210612),(#210613,#210614),(#210615,#210616),(#210617,#210618),
(#210619,#210620),(#210621,#210622),(#210623,#210624),(#210625,#210626),
(#210627,#210628),(#210629,#210630),(#210631,#210632),(#210633,#210634),
(#210635,#210636),(#210637,#210638),(#210639,#210640),(#210641,#210642),
(#210643,#210644),(#210645,#210646),(#210647,#210648),(#210649,#210650),
(#210651,#210652),(#210653,#210654),(#210655,#210656),(#210657,#210658),
(#210659,#210660),(#210661,#210662),(#210663,#210664),(#210665,#210666),
(#210667,#210668),(#210669,#210670),(#210671,#210672),(#210673,#210674),
(#210675,#210676),(#210677,#210678),(#210679,#210680),(#210681,#210682),
(#210683,#210684),(#210685,#210686),(#210687,#210688),(#210689,#210690),
(#210691,#210692),(#210693,#210694),(#210695,#210696),(#210697,#210698),
(#210699,#210700),(#210701,#210702),(#210703,#210704),(#210705,#210706),
(#210707,#210708),(#210709,#210710),(#210711,#210712),(#210713,#210714),
(#210715,#210716),(#210717,#210718),(#210719,#210720),(#210721,#210722),
(#210723,#210724),(#210725,#210726),(#210727,#210728),(#210729,#210730),
(#210731,#210732),(#210733,#210734),(#210735,#210736),(#210737,#210738),
(#210739,#210740),(#210741,#210742),(#210743,#210744),(#210745,#210746),
(#210747,#210748),(#210749,#210750),(#210751,#210752),(#210753,#210754),
(#210755,#210756),(#210757,#210758),(#210759,#210760),(#210761,#210762),
(#210763,#210764),(#210765,#210766),(#210767,#210768),(#210769,#210770),
(#210771,#210772),(#210773,#210774)),.UNSPECIFIED.,.F.,.F.,.F.)
B_SPLINE_SURFACE_WITH_KNOTS((6,1,1,1,1,1,1,1,1,1,1,1,1,1,1,1,1,1,1,1,1,
1,1,1,1,1,1,1,1,1,1,1,1,1,1,1,1,1,1,1,1,1,1,1,1,1,1,1,1,1,1,1,1,1,1,1,1,
1,1,1,1,1,1,1,1,1,1,1,1,1,1,1,1,1,1,1,1,1,1,1,1,1,1,1,1,1,1,1,1,1,1,1,1,
1,1,1,1,1,1,1,1,1,1,1,1,1,1,1,1,1,1,1,1,1,1,1,1,1,1,1,1,1,1,1,1,1,1,1,1,
1,1,1,1,1,1,1,1,1,1,1,1,1,1,1,1,1,1,1,1,1,1,1,1,1,1,1,1,1,1,1,1,1,1,1,1,
1,1,1,1,1,1,1,1,1,1,1,1,1,1,1,1,1,1,1,1,1,1,1,1,1,1,1,1,1,1,1,1,1,1,1,6),
(2,2),(-1.,-0.995000000000001,-0.990000000000001,-0.985000000000001,-0.980000000000001,
-0.975000000000001,-0.970000000000001,-0.965000000000001,-0.960000000000001,
-0.955000000000001,-0.950000000000001,-0.945000000000001,-0.940000000000001,
-0.935000000000001,-0.930000000000001,-0.925000000000001,-0.920000000000001,
-0.915000000000001,-0.910000000000001,-0.905000000000001,-0.900000000000001,
-0.895000000000001,-0.890000000000001,-0.885000000000001,-0.880000000000001,
-0.875000000000001,-0.870000000000001,-0.865000000000001,-0.860000000000001,
-0.855000000000001,-0.850000000000001,-0.845000000000001,-0.840000000000001,
-0.835000000000001,-0.830000000000001,-0.825000000000001,-0.820000000000001,
-0.815000000000001,-0.810000000000001,-0.805000000000001,-0.800000000000001,
-0.795000000000001,-0.790000000000001,-0.785000000000001,-0.780000000000001,
-0.775000000000001,-0.770000000000001,-0.765000000000001,-0.760000000000001,
-0.755000000000001,-0.750000000000001,-0.745000000000001,-0.740000000000001,
-0.735000000000001,-0.730000000000001,-0.725000000000001,-0.720000000000001,
-0.715000000000001,-0.710000000000001,-0.705000000000001,-0.700000000000001,
-0.695000000000001,-0.690000000000001,-0.685,-0.68,-0.675,-0.67,-0.665,
-0.66,-0.655,-0.65,-0.645,-0.64,-0.635,-0.63,-0.625,-0.62,-0.615,-0.61,
-0.605,-0.6,-0.595,-0.59,-0.585,-0.58,-0.575,-0.57,-0.565,-0.56,-0.555,
-0.55,-0.545,-0.54,-0.535,-0.53,-0.525,-0.52,-0.515,-0.51,-0.505,-0.5,-0.495,
-0.49,-0.485,-0.48,-0.475,-0.47,-0.465,-0.46,-0.455,-0.45,-0.445,-0.44,
-0.435,-0.43,-0.425,-0.42,-0.415,-0.41,-0.405,-0.4,-0.395,-0.39,-0.385,
-0.38,-0.375,-0.37,-0.365,-0.36,-0.355,-0.35,-0.345,-0.34,-0.335,-0.33,
-0.325,-0.32,-0.315,-0.31,-0.305,-0.3,-0.295,-0.29,-0.285,-0.28,-0.275,
-0.27,-0.265,-0.26,-0.255,-0.25,-0.245,-0.24,-0.235,-0.23,-0.225,-0.22,
-0.215,-0.21,-0.205,-0.2,-0.195,-0.19,-0.185,-0.18,-0.175,-0.17,-0.165,
-0.16,-0.155,-0.15,-0.145,-0.14,-0.135,-0.13,-0.125,-0.12,-0.115,-0.11,
-0.105,-0.1,-0.095,-0.09,-0.085,-0.08,-0.075,-0.07,-0.065,-0.06,-0.055,
-0.05,-0.045,-0.04,-0.035,-0.03,-0.025,-0.02,-0.015,-0.01,-0.005,0.),(0.,
1.2),.UNSPECIFIED.)
GEOMETRIC_REPRESENTATION_ITEM()
RATIONAL_B_SPLINE_SURFACE(((1.,1.),(1.,1.),(1.,1.),(1.,1.),(1.,1.),(1.,
1.),(1.,1.),(1.,1.),(1.,1.),(1.,1.),(1.,1.),(1.,1.),(1.,1.),(1.,1.),(1.,
1.),(1.,1.),(1.,1.),(1.,1.),(1.,1.),(1.,1.),(1.,1.),(1.,1.),(1.,1.),(1.,
1.),(1.,1.),(1.,1.),(1.,1.),(1.,1.),(1.,1.),(1.,1.),(1.,1.),(1.,1.),(1.,
1.),(1.,1.),(1.,1.),(1.,1.),(1.,1.),(1.,1.),(1.,1.),(1.,1.),(1.,1.),(1.,
1.),(1.,1.),(1.,1.),(1.,1.),(1.,1.),(1.,1.),(1.,1.),(1.,1.),(1.,1.),(1.,
1.),(1.,1.),(1.,1.),(1.,1.),(1.,1.),(1.,1.),(1.,1.),(1.,1.),(1.,1.),(1.,
1.),(1.,1.),(1.,1.),(1.,1.),(1.,1.),(1.,1.),(1.,1.),(1.,1.),(1.,1.),(1.,
1.),(1.,1.),(1.,1.),(1.,1.),(1.,1.),(1.,1.),(1.,1.),(1.,1.),(1.,1.),(1.,
1.),(1.,1.),(1.,1.),(1.,1.),(1.,1.),(1.,1.),(1.,1.),(1.,1.),(1.,1.),(1.,
1.),(1.,1.),(1.,1.),(1.,1.),(1.,1.),(1.,1.),(1.,1.),(1.,1.),(1.,1.),(1.,
1.),(1.,1.),(1.,1.),(1.,1.),(1.,1.),(1.,1.),(1.,1.),(1.,1.),(1.,1.),(1.,
1.),(1.,1.),(1.,1.),(1.,1.),(1.,1.),(1.,1.),(1.,1.),(1.,1.),(1.,1.),(1.,
1.),(1.,1.),(1.,1.),(1.,1.),(1.,1.),(1.,1.),(1.,1.),(1.,1.),(1.,1.),(1.,
1.),(1.,1.),(1.,1.),(1.,1.),(1.,1.),(1.,1.),(1.,1.),(1.,1.),(1.,1.),(1.,
1.),(1.,1.),(1.,1.),(1.,1.),(1.,1.),(1.,1.),(1.,1.),(1.,1.),(1.,1.),(1.,
1.),(1.,1.),(1.,1.),(1.,1.),(1.,1.),(1.,1.),(1.,1.),(1.,1.),(1.,1.),(1.,
1.),(1.,1.),(1.,1.),(1.,1.),(1.,1.),(1.,1.),(1.,1.),(1.,1.),(1.,1.),(1.,
1.),(1.,1.),(1.,1.),(1.,1.),(1.,1.),(1.,1.),(1.,1.),(1.,1.),(1.,1.),(1.,
1.),(1.,1.),(1.,1.),(1.,1.),(1.,1.),(1.,1.),(1.,1.),(1.,1.),(1.,1.),(1.,
1.),(1.,1.),(1.,1.),(1.,1.),(1.,1.),(1.,1.),(1.,1.),(1.,1.),(1.,1.),(1.,
1.),(1.,1.),(1.,1.),(1.,1.),(1.,1.),(1.,1.),(1.,1.),(1.,1.),(1.,1.),(1.,
1.),(1.,1.),(1.,1.),(1.,1.),(1.,1.),(1.,1.),(1.,1.),(1.,1.),(1.,1.),(1.,
1.),(1.,1.)))
REPRESENTATION_ITEM('')
SURFACE()
);
#1068=(
BOUNDED_SURFACE()
B_SPLINE_SURFACE(5,1,((#210982,#210983),(#210984,#210985),(#210986,#210987),
(#210988,#210989),(#210990,#210991),(#210992,#210993),(#210994,#210995),
(#210996,#210997),(#210998,#210999),(#211000,#211001),(#211002,#211003),
(#211004,#211005),(#211006,#211007),(#211008,#211009),(#211010,#211011),
(#211012,#211013),(#211014,#211015),(#211016,#211017),(#211018,#211019),
(#211020,#211021),(#211022,#211023),(#211024,#211025),(#211026,#211027),
(#211028,#211029),(#211030,#211031),(#211032,#211033),(#211034,#211035),
(#211036,#211037),(#211038,#211039),(#211040,#211041),(#211042,#211043),
(#211044,#211045),(#211046,#211047),(#211048,#211049),(#211050,#211051),
(#211052,#211053),(#211054,#211055),(#211056,#211057),(#211058,#211059),
(#211060,#211061),(#211062,#211063),(#211064,#211065),(#211066,#211067),
(#211068,#211069),(#211070,#211071),(#211072,#211073),(#211074,#211075),
(#211076,#211077),(#211078,#211079),(#211080,#211081),(#211082,#211083),
(#211084,#211085),(#211086,#211087),(#211088,#211089),(#211090,#211091),
(#211092,#211093),(#211094,#211095),(#211096,#211097),(#211098,#211099),
(#211100,#211101),(#211102,#211103),(#211104,#211105),(#211106,#211107),
(#211108,#211109),(#211110,#211111),(#211112,#211113),(#211114,#211115),
(#211116,#211117),(#211118,#211119),(#211120,#211121),(#211122,#211123),
(#211124,#211125),(#211126,#211127),(#211128,#211129),(#211130,#211131),
(#211132,#211133),(#211134,#211135),(#211136,#211137),(#211138,#211139),
(#211140,#211141),(#211142,#211143),(#211144,#211145),(#211146,#211147),
(#211148,#211149),(#211150,#211151),(#211152,#211153),(#211154,#211155),
(#211156,#211157),(#211158,#211159),(#211160,#211161),(#211162,#211163),
(#211164,#211165),(#211166,#211167),(#211168,#211169),(#211170,#211171),
(#211172,#211173),(#211174,#211175),(#211176,#211177),(#211178,#211179),
(#211180,#211181),(#211182,#211183),(#211184,#211185),(#211186,#211187),
(#211188,#211189),(#211190,#211191),(#211192,#211193),(#211194,#211195),
(#211196,#211197),(#211198,#211199),(#211200,#211201),(#211202,#211203),
(#211204,#211205),(#211206,#211207),(#211208,#211209),(#211210,#211211),
(#211212,#211213),(#211214,#211215),(#211216,#211217),(#211218,#211219),
(#211220,#211221),(#211222,#211223),(#211224,#211225),(#211226,#211227),
(#211228,#211229),(#211230,#211231),(#211232,#211233),(#211234,#211235),
(#211236,#211237),(#211238,#211239),(#211240,#211241),(#211242,#211243),
(#211244,#211245),(#211246,#211247),(#211248,#211249),(#211250,#211251),
(#211252,#211253),(#211254,#211255),(#211256,#211257),(#211258,#211259),
(#211260,#211261),(#211262,#211263),(#211264,#211265),(#211266,#211267),
(#211268,#211269),(#211270,#211271),(#211272,#211273),(#211274,#211275),
(#211276,#211277),(#211278,#211279),(#211280,#211281),(#211282,#211283),
(#211284,#211285),(#211286,#211287),(#211288,#211289),(#211290,#211291),
(#211292,#211293),(#211294,#211295),(#211296,#211297),(#211298,#211299),
(#211300,#211301),(#211302,#211303),(#211304,#211305),(#211306,#211307),
(#211308,#211309),(#211310,#211311),(#211312,#211313),(#211314,#211315),
(#211316,#211317),(#211318,#211319),(#211320,#211321),(#211322,#211323),
(#211324,#211325),(#211326,#211327),(#211328,#211329),(#211330,#211331),
(#211332,#211333),(#211334,#211335),(#211336,#211337),(#211338,#211339),
(#211340,#211341),(#211342,#211343),(#211344,#211345),(#211346,#211347),
(#211348,#211349),(#211350,#211351),(#211352,#211353),(#211354,#211355),
(#211356,#211357),(#211358,#211359),(#211360,#211361),(#211362,#211363),
(#211364,#211365),(#211366,#211367),(#211368,#211369),(#211370,#211371),
(#211372,#211373),(#211374,#211375),(#211376,#211377),(#211378,#211379),
(#211380,#211381),(#211382,#211383),(#211384,#211385),(#211386,#211387),
(#211388,#211389),(#211390,#211391)),.UNSPECIFIED.,.F.,.F.,.F.)
B_SPLINE_SURFACE_WITH_KNOTS((6,1,1,1,1,1,1,1,1,1,1,1,1,1,1,1,1,1,1,1,1,
1,1,1,1,1,1,1,1,1,1,1,1,1,1,1,1,1,1,1,1,1,1,1,1,1,1,1,1,1,1,1,1,1,1,1,1,
1,1,1,1,1,1,1,1,1,1,1,1,1,1,1,1,1,1,1,1,1,1,1,1,1,1,1,1,1,1,1,1,1,1,1,1,
1,1,1,1,1,1,1,1,1,1,1,1,1,1,1,1,1,1,1,1,1,1,1,1,1,1,1,1,1,1,1,1,1,1,1,1,
1,1,1,1,1,1,1,1,1,1,1,1,1,1,1,1,1,1,1,1,1,1,1,1,1,1,1,1,1,1,1,1,1,1,1,1,
1,1,1,1,1,1,1,1,1,1,1,1,1,1,1,1,1,1,1,1,1,1,1,1,1,1,1,1,1,1,1,1,1,1,1,6),
(2,2),(0.,0.005,0.01,0.015,0.02,0.025,0.03,0.035,0.04,0.045,0.05,0.055,
0.06,0.065,0.07,0.075,0.08,0.085,0.09,0.095,0.1,0.105,0.11,0.115,0.12,0.125,
0.13,0.135,0.14,0.145,0.15,0.155,0.16,0.165,0.17,0.175,0.18,0.185,0.19,
0.195,0.2,0.205,0.21,0.215,0.22,0.225,0.23,0.235,0.24,0.245,0.25,0.255,
0.26,0.265,0.27,0.275,0.28,0.285,0.29,0.295,0.3,0.305,0.31,0.315,0.32,0.325,
0.33,0.335,0.34,0.345,0.35,0.355,0.36,0.365,0.37,0.375,0.38,0.385,0.39,
0.395,0.4,0.405,0.41,0.415,0.42,0.425,0.43,0.435,0.44,0.445,0.45,0.455,
0.46,0.465,0.47,0.475,0.48,0.485,0.49,0.495,0.5,0.505,0.51,0.515,0.52,0.525,
0.53,0.535,0.54,0.545,0.55,0.555,0.56,0.565,0.57,0.575,0.58,0.585,0.59,
0.595,0.6,0.605,0.61,0.615,0.62,0.625,0.63,0.635,0.64,0.645,0.65,0.655,
0.66,0.665,0.67,0.675,0.68,0.685,0.690000000000001,0.695000000000001,0.700000000000001,
0.705000000000001,0.710000000000001,0.715000000000001,0.720000000000001,
0.725000000000001,0.730000000000001,0.735000000000001,0.740000000000001,
0.745000000000001,0.750000000000001,0.755000000000001,0.760000000000001,
0.765000000000001,0.770000000000001,0.775000000000001,0.780000000000001,
0.785000000000001,0.790000000000001,0.795000000000001,0.800000000000001,
0.805000000000001,0.810000000000001,0.815000000000001,0.820000000000001,
0.825000000000001,0.830000000000001,0.835000000000001,0.840000000000001,
0.845000000000001,0.850000000000001,0.855000000000001,0.860000000000001,
0.865000000000001,0.870000000000001,0.875000000000001,0.880000000000001,
0.885000000000001,0.890000000000001,0.895000000000001,0.900000000000001,
0.905000000000001,0.910000000000001,0.915000000000001,0.920000000000001,
0.925000000000001,0.930000000000001,0.935000000000001,0.940000000000001,
0.945000000000001,0.950000000000001,0.955000000000001,0.960000000000001,
0.965000000000001,0.970000000000001,0.975000000000001,0.980000000000001,
0.985000000000001,0.990000000000001,0.995000000000001,1.),(0.,1.2),
 .UNSPECIFIED.)
GEOMETRIC_REPRESENTATION_ITEM()
RATIONAL_B_SPLINE_SURFACE(((1.,1.),(1.,1.),(1.,1.),(1.,1.),(1.,1.),(1.,
1.),(1.,1.),(1.,1.),(1.,1.),(1.,1.),(1.,1.),(1.,1.),(1.,1.),(1.,1.),(1.,
1.),(1.,1.),(1.,1.),(1.,1.),(1.,1.),(1.,1.),(1.,1.),(1.,1.),(1.,1.),(1.,
1.),(1.,1.),(1.,1.),(1.,1.),(1.,1.),(1.,1.),(1.,1.),(1.,1.),(1.,1.),(1.,
1.),(1.,1.),(1.,1.),(1.,1.),(1.,1.),(1.,1.),(1.,1.),(1.,1.),(1.,1.),(1.,
1.),(1.,1.),(1.,1.),(1.,1.),(1.,1.),(1.,1.),(1.,1.),(1.,1.),(1.,1.),(1.,
1.),(1.,1.),(1.,1.),(1.,1.),(1.,1.),(1.,1.),(1.,1.),(1.,1.),(1.,1.),(1.,
1.),(1.,1.),(1.,1.),(1.,1.),(1.,1.),(1.,1.),(1.,1.),(1.,1.),(1.,1.),(1.,
1.),(1.,1.),(1.,1.),(1.,1.),(1.,1.),(1.,1.),(1.,1.),(1.,1.),(1.,1.),(1.,
1.),(1.,1.),(1.,1.),(1.,1.),(1.,1.),(1.,1.),(1.,1.),(1.,1.),(1.,1.),(1.,
1.),(1.,1.),(1.,1.),(1.,1.),(1.,1.),(1.,1.),(1.,1.),(1.,1.),(1.,1.),(1.,
1.),(1.,1.),(1.,1.),(1.,1.),(1.,1.),(1.,1.),(1.,1.),(1.,1.),(1.,1.),(1.,
1.),(1.,1.),(1.,1.),(1.,1.),(1.,1.),(1.,1.),(1.,1.),(1.,1.),(1.,1.),(1.,
1.),(1.,1.),(1.,1.),(1.,1.),(1.,1.),(1.,1.),(1.,1.),(1.,1.),(1.,1.),(1.,
1.),(1.,1.),(1.,1.),(1.,1.),(1.,1.),(1.,1.),(1.,1.),(1.,1.),(1.,1.),(1.,
1.),(1.,1.),(1.,1.),(1.,1.),(1.,1.),(1.,1.),(1.,1.),(1.,1.),(1.,1.),(1.,
1.),(1.,1.),(1.,1.),(1.,1.),(1.,1.),(1.,1.),(1.,1.),(1.,1.),(1.,1.),(1.,
1.),(1.,1.),(1.,1.),(1.,1.),(1.,1.),(1.,1.),(1.,1.),(1.,1.),(1.,1.),(1.,
1.),(1.,1.),(1.,1.),(1.,1.),(1.,1.),(1.,1.),(1.,1.),(1.,1.),(1.,1.),(1.,
1.),(1.,1.),(1.,1.),(1.,1.),(1.,1.),(1.,1.),(1.,1.),(1.,1.),(1.,1.),(1.,
1.),(1.,1.),(1.,1.),(1.,1.),(1.,1.),(1.,1.),(1.,1.),(1.,1.),(1.,1.),(1.,
1.),(1.,1.),(1.,1.),(1.,1.),(1.,1.),(1.,1.),(1.,1.),(1.,1.),(1.,1.),(1.,
1.),(1.,1.),(1.,1.),(1.,1.),(1.,1.),(1.,1.),(1.,1.),(1.,1.),(1.,1.),(1.,
1.),(1.,1.)))
REPRESENTATION_ITEM('')
SURFACE()
);
#1069=(
BOUNDED_SURFACE()
B_SPLINE_SURFACE(5,1,((#211603,#211604),(#211605,#211606),(#211607,#211608),
(#211609,#211610),(#211611,#211612),(#211613,#211614),(#211615,#211616),
(#211617,#211618),(#211619,#211620),(#211621,#211622),(#211623,#211624),
(#211625,#211626),(#211627,#211628),(#211629,#211630),(#211631,#211632),
(#211633,#211634),(#211635,#211636),(#211637,#211638),(#211639,#211640),
(#211641,#211642),(#211643,#211644),(#211645,#211646),(#211647,#211648),
(#211649,#211650),(#211651,#211652),(#211653,#211654),(#211655,#211656),
(#211657,#211658),(#211659,#211660),(#211661,#211662),(#211663,#211664),
(#211665,#211666),(#211667,#211668),(#211669,#211670),(#211671,#211672),
(#211673,#211674),(#211675,#211676),(#211677,#211678),(#211679,#211680),
(#211681,#211682),(#211683,#211684),(#211685,#211686),(#211687,#211688),
(#211689,#211690),(#211691,#211692),(#211693,#211694),(#211695,#211696),
(#211697,#211698),(#211699,#211700),(#211701,#211702),(#211703,#211704),
(#211705,#211706),(#211707,#211708),(#211709,#211710),(#211711,#211712),
(#211713,#211714),(#211715,#211716),(#211717,#211718),(#211719,#211720),
(#211721,#211722),(#211723,#211724),(#211725,#211726),(#211727,#211728),
(#211729,#211730),(#211731,#211732),(#211733,#211734),(#211735,#211736),
(#211737,#211738),(#211739,#211740),(#211741,#211742),(#211743,#211744),
(#211745,#211746),(#211747,#211748),(#211749,#211750),(#211751,#211752),
(#211753,#211754),(#211755,#211756),(#211757,#211758),(#211759,#211760),
(#211761,#211762),(#211763,#211764),(#211765,#211766),(#211767,#211768),
(#211769,#211770),(#211771,#211772),(#211773,#211774),(#211775,#211776),
(#211777,#211778),(#211779,#211780),(#211781,#211782),(#211783,#211784),
(#211785,#211786),(#211787,#211788),(#211789,#211790),(#211791,#211792),
(#211793,#211794),(#211795,#211796),(#211797,#211798),(#211799,#211800),
(#211801,#211802),(#211803,#211804),(#211805,#211806),(#211807,#211808),
(#211809,#211810),(#211811,#211812),(#211813,#211814),(#211815,#211816),
(#211817,#211818),(#211819,#211820),(#211821,#211822),(#211823,#211824),
(#211825,#211826),(#211827,#211828),(#211829,#211830),(#211831,#211832),
(#211833,#211834),(#211835,#211836),(#211837,#211838),(#211839,#211840),
(#211841,#211842),(#211843,#211844),(#211845,#211846),(#211847,#211848),
(#211849,#211850),(#211851,#211852),(#211853,#211854),(#211855,#211856),
(#211857,#211858),(#211859,#211860),(#211861,#211862),(#211863,#211864),
(#211865,#211866),(#211867,#211868),(#211869,#211870),(#211871,#211872),
(#211873,#211874),(#211875,#211876),(#211877,#211878),(#211879,#211880),
(#211881,#211882),(#211883,#211884),(#211885,#211886),(#211887,#211888),
(#211889,#211890),(#211891,#211892),(#211893,#211894),(#211895,#211896),
(#211897,#211898),(#211899,#211900),(#211901,#211902),(#211903,#211904),
(#211905,#211906),(#211907,#211908),(#211909,#211910),(#211911,#211912),
(#211913,#211914),(#211915,#211916),(#211917,#211918),(#211919,#211920),
(#211921,#211922),(#211923,#211924),(#211925,#211926),(#211927,#211928),
(#211929,#211930),(#211931,#211932),(#211933,#211934),(#211935,#211936),
(#211937,#211938),(#211939,#211940),(#211941,#211942),(#211943,#211944),
(#211945,#211946),(#211947,#211948),(#211949,#211950),(#211951,#211952),
(#211953,#211954),(#211955,#211956),(#211957,#211958),(#211959,#211960),
(#211961,#211962),(#211963,#211964),(#211965,#211966),(#211967,#211968),
(#211969,#211970),(#211971,#211972),(#211973,#211974),(#211975,#211976),
(#211977,#211978),(#211979,#211980),(#211981,#211982),(#211983,#211984),
(#211985,#211986),(#211987,#211988),(#211989,#211990),(#211991,#211992),
(#211993,#211994),(#211995,#211996),(#211997,#211998),(#211999,#212000),
(#212001,#212002),(#212003,#212004),(#212005,#212006),(#212007,#212008),
(#212009,#212010),(#212011,#212012)),.UNSPECIFIED.,.F.,.F.,.F.)
B_SPLINE_SURFACE_WITH_KNOTS((6,1,1,1,1,1,1,1,1,1,1,1,1,1,1,1,1,1,1,1,1,
1,1,1,1,1,1,1,1,1,1,1,1,1,1,1,1,1,1,1,1,1,1,1,1,1,1,1,1,1,1,1,1,1,1,1,1,
1,1,1,1,1,1,1,1,1,1,1,1,1,1,1,1,1,1,1,1,1,1,1,1,1,1,1,1,1,1,1,1,1,1,1,1,
1,1,1,1,1,1,1,1,1,1,1,1,1,1,1,1,1,1,1,1,1,1,1,1,1,1,1,1,1,1,1,1,1,1,1,1,
1,1,1,1,1,1,1,1,1,1,1,1,1,1,1,1,1,1,1,1,1,1,1,1,1,1,1,1,1,1,1,1,1,1,1,1,
1,1,1,1,1,1,1,1,1,1,1,1,1,1,1,1,1,1,1,1,1,1,1,1,1,1,1,1,1,1,1,1,1,1,1,6),
(2,2),(-1.,-0.995000000000001,-0.990000000000001,-0.985000000000001,-0.980000000000001,
-0.975000000000001,-0.970000000000001,-0.965000000000001,-0.960000000000001,
-0.955000000000001,-0.950000000000001,-0.945000000000001,-0.940000000000001,
-0.935000000000001,-0.930000000000001,-0.925000000000001,-0.920000000000001,
-0.915000000000001,-0.910000000000001,-0.905000000000001,-0.900000000000001,
-0.895000000000001,-0.890000000000001,-0.885000000000001,-0.880000000000001,
-0.875000000000001,-0.870000000000001,-0.865000000000001,-0.860000000000001,
-0.855000000000001,-0.850000000000001,-0.845000000000001,-0.840000000000001,
-0.835000000000001,-0.830000000000001,-0.825000000000001,-0.820000000000001,
-0.815000000000001,-0.810000000000001,-0.805000000000001,-0.800000000000001,
-0.795000000000001,-0.790000000000001,-0.785000000000001,-0.780000000000001,
-0.775000000000001,-0.770000000000001,-0.765000000000001,-0.760000000000001,
-0.755000000000001,-0.750000000000001,-0.745000000000001,-0.740000000000001,
-0.735000000000001,-0.730000000000001,-0.725000000000001,-0.720000000000001,
-0.715000000000001,-0.710000000000001,-0.705000000000001,-0.700000000000001,
-0.695000000000001,-0.690000000000001,-0.685,-0.68,-0.675,-0.67,-0.665,
-0.66,-0.655,-0.65,-0.645,-0.64,-0.635,-0.63,-0.625,-0.62,-0.615,-0.61,
-0.605,-0.6,-0.595,-0.59,-0.585,-0.58,-0.575,-0.57,-0.565,-0.56,-0.555,
-0.55,-0.545,-0.54,-0.535,-0.53,-0.525,-0.52,-0.515,-0.51,-0.505,-0.5,-0.495,
-0.49,-0.485,-0.48,-0.475,-0.47,-0.465,-0.46,-0.455,-0.45,-0.445,-0.44,
-0.435,-0.43,-0.425,-0.42,-0.415,-0.41,-0.405,-0.4,-0.395,-0.39,-0.385,
-0.38,-0.375,-0.37,-0.365,-0.36,-0.355,-0.35,-0.345,-0.34,-0.335,-0.33,
-0.325,-0.32,-0.315,-0.31,-0.305,-0.3,-0.295,-0.29,-0.285,-0.28,-0.275,
-0.27,-0.265,-0.26,-0.255,-0.25,-0.245,-0.24,-0.235,-0.23,-0.225,-0.22,
-0.215,-0.21,-0.205,-0.2,-0.195,-0.19,-0.185,-0.18,-0.175,-0.17,-0.165,
-0.16,-0.155,-0.15,-0.145,-0.14,-0.135,-0.13,-0.125,-0.12,-0.115,-0.11,
-0.105,-0.1,-0.095,-0.09,-0.085,-0.08,-0.075,-0.07,-0.065,-0.06,-0.055,
-0.05,-0.045,-0.04,-0.035,-0.03,-0.025,-0.02,-0.015,-0.01,-0.005,0.),(0.,
1.2),.UNSPECIFIED.)
GEOMETRIC_REPRESENTATION_ITEM()
RATIONAL_B_SPLINE_SURFACE(((1.,1.),(1.,1.),(1.,1.),(1.,1.),(1.,1.),(1.,
1.),(1.,1.),(1.,1.),(1.,1.),(1.,1.),(1.,1.),(1.,1.),(1.,1.),(1.,1.),(1.,
1.),(1.,1.),(1.,1.),(1.,1.),(1.,1.),(1.,1.),(1.,1.),(1.,1.),(1.,1.),(1.,
1.),(1.,1.),(1.,1.),(1.,1.),(1.,1.),(1.,1.),(1.,1.),(1.,1.),(1.,1.),(1.,
1.),(1.,1.),(1.,1.),(1.,1.),(1.,1.),(1.,1.),(1.,1.),(1.,1.),(1.,1.),(1.,
1.),(1.,1.),(1.,1.),(1.,1.),(1.,1.),(1.,1.),(1.,1.),(1.,1.),(1.,1.),(1.,
1.),(1.,1.),(1.,1.),(1.,1.),(1.,1.),(1.,1.),(1.,1.),(1.,1.),(1.,1.),(1.,
1.),(1.,1.),(1.,1.),(1.,1.),(1.,1.),(1.,1.),(1.,1.),(1.,1.),(1.,1.),(1.,
1.),(1.,1.),(1.,1.),(1.,1.),(1.,1.),(1.,1.),(1.,1.),(1.,1.),(1.,1.),(1.,
1.),(1.,1.),(1.,1.),(1.,1.),(1.,1.),(1.,1.),(1.,1.),(1.,1.),(1.,1.),(1.,
1.),(1.,1.),(1.,1.),(1.,1.),(1.,1.),(1.,1.),(1.,1.),(1.,1.),(1.,1.),(1.,
1.),(1.,1.),(1.,1.),(1.,1.),(1.,1.),(1.,1.),(1.,1.),(1.,1.),(1.,1.),(1.,
1.),(1.,1.),(1.,1.),(1.,1.),(1.,1.),(1.,1.),(1.,1.),(1.,1.),(1.,1.),(1.,
1.),(1.,1.),(1.,1.),(1.,1.),(1.,1.),(1.,1.),(1.,1.),(1.,1.),(1.,1.),(1.,
1.),(1.,1.),(1.,1.),(1.,1.),(1.,1.),(1.,1.),(1.,1.),(1.,1.),(1.,1.),(1.,
1.),(1.,1.),(1.,1.),(1.,1.),(1.,1.),(1.,1.),(1.,1.),(1.,1.),(1.,1.),(1.,
1.),(1.,1.),(1.,1.),(1.,1.),(1.,1.),(1.,1.),(1.,1.),(1.,1.),(1.,1.),(1.,
1.),(1.,1.),(1.,1.),(1.,1.),(1.,1.),(1.,1.),(1.,1.),(1.,1.),(1.,1.),(1.,
1.),(1.,1.),(1.,1.),(1.,1.),(1.,1.),(1.,1.),(1.,1.),(1.,1.),(1.,1.),(1.,
1.),(1.,1.),(1.,1.),(1.,1.),(1.,1.),(1.,1.),(1.,1.),(1.,1.),(1.,1.),(1.,
1.),(1.,1.),(1.,1.),(1.,1.),(1.,1.),(1.,1.),(1.,1.),(1.,1.),(1.,1.),(1.,
1.),(1.,1.),(1.,1.),(1.,1.),(1.,1.),(1.,1.),(1.,1.),(1.,1.),(1.,1.),(1.,
1.),(1.,1.),(1.,1.),(1.,1.),(1.,1.),(1.,1.),(1.,1.),(1.,1.),(1.,1.),(1.,
1.),(1.,1.)))
REPRESENTATION_ITEM('')
SURFACE()
);
#1070=(
BOUNDED_SURFACE()
B_SPLINE_SURFACE(5,1,((#212220,#212221),(#212222,#212223),(#212224,#212225),
(#212226,#212227),(#212228,#212229),(#212230,#212231),(#212232,#212233),
(#212234,#212235),(#212236,#212237),(#212238,#212239),(#212240,#212241),
(#212242,#212243),(#212244,#212245),(#212246,#212247),(#212248,#212249),
(#212250,#212251),(#212252,#212253),(#212254,#212255),(#212256,#212257),
(#212258,#212259),(#212260,#212261),(#212262,#212263),(#212264,#212265),
(#212266,#212267),(#212268,#212269),(#212270,#212271),(#212272,#212273),
(#212274,#212275),(#212276,#212277),(#212278,#212279),(#212280,#212281),
(#212282,#212283),(#212284,#212285),(#212286,#212287),(#212288,#212289),
(#212290,#212291),(#212292,#212293),(#212294,#212295),(#212296,#212297),
(#212298,#212299),(#212300,#212301),(#212302,#212303),(#212304,#212305),
(#212306,#212307),(#212308,#212309),(#212310,#212311),(#212312,#212313),
(#212314,#212315),(#212316,#212317),(#212318,#212319),(#212320,#212321),
(#212322,#212323),(#212324,#212325),(#212326,#212327),(#212328,#212329),
(#212330,#212331),(#212332,#212333),(#212334,#212335),(#212336,#212337),
(#212338,#212339),(#212340,#212341),(#212342,#212343),(#212344,#212345),
(#212346,#212347),(#212348,#212349),(#212350,#212351),(#212352,#212353),
(#212354,#212355),(#212356,#212357),(#212358,#212359),(#212360,#212361),
(#212362,#212363),(#212364,#212365),(#212366,#212367),(#212368,#212369),
(#212370,#212371),(#212372,#212373),(#212374,#212375),(#212376,#212377),
(#212378,#212379),(#212380,#212381),(#212382,#212383),(#212384,#212385),
(#212386,#212387),(#212388,#212389),(#212390,#212391),(#212392,#212393),
(#212394,#212395),(#212396,#212397),(#212398,#212399),(#212400,#212401),
(#212402,#212403),(#212404,#212405),(#212406,#212407),(#212408,#212409),
(#212410,#212411),(#212412,#212413),(#212414,#212415),(#212416,#212417),
(#212418,#212419),(#212420,#212421),(#212422,#212423),(#212424,#212425),
(#212426,#212427),(#212428,#212429),(#212430,#212431),(#212432,#212433),
(#212434,#212435),(#212436,#212437),(#212438,#212439),(#212440,#212441),
(#212442,#212443),(#212444,#212445),(#212446,#212447),(#212448,#212449),
(#212450,#212451),(#212452,#212453),(#212454,#212455),(#212456,#212457),
(#212458,#212459),(#212460,#212461),(#212462,#212463),(#212464,#212465),
(#212466,#212467),(#212468,#212469),(#212470,#212471),(#212472,#212473),
(#212474,#212475),(#212476,#212477),(#212478,#212479),(#212480,#212481),
(#212482,#212483),(#212484,#212485),(#212486,#212487),(#212488,#212489),
(#212490,#212491),(#212492,#212493),(#212494,#212495),(#212496,#212497),
(#212498,#212499),(#212500,#212501),(#212502,#212503),(#212504,#212505),
(#212506,#212507),(#212508,#212509),(#212510,#212511),(#212512,#212513),
(#212514,#212515),(#212516,#212517),(#212518,#212519),(#212520,#212521),
(#212522,#212523),(#212524,#212525),(#212526,#212527),(#212528,#212529),
(#212530,#212531),(#212532,#212533),(#212534,#212535),(#212536,#212537),
(#212538,#212539),(#212540,#212541),(#212542,#212543),(#212544,#212545),
(#212546,#212547),(#212548,#212549),(#212550,#212551),(#212552,#212553),
(#212554,#212555),(#212556,#212557),(#212558,#212559),(#212560,#212561),
(#212562,#212563),(#212564,#212565),(#212566,#212567),(#212568,#212569),
(#212570,#212571),(#212572,#212573),(#212574,#212575),(#212576,#212577),
(#212578,#212579),(#212580,#212581),(#212582,#212583),(#212584,#212585),
(#212586,#212587),(#212588,#212589),(#212590,#212591),(#212592,#212593),
(#212594,#212595),(#212596,#212597),(#212598,#212599),(#212600,#212601),
(#212602,#212603),(#212604,#212605),(#212606,#212607),(#212608,#212609),
(#212610,#212611),(#212612,#212613),(#212614,#212615),(#212616,#212617),
(#212618,#212619),(#212620,#212621),(#212622,#212623),(#212624,#212625),
(#212626,#212627),(#212628,#212629)),.UNSPECIFIED.,.F.,.F.,.F.)
B_SPLINE_SURFACE_WITH_KNOTS((6,1,1,1,1,1,1,1,1,1,1,1,1,1,1,1,1,1,1,1,1,
1,1,1,1,1,1,1,1,1,1,1,1,1,1,1,1,1,1,1,1,1,1,1,1,1,1,1,1,1,1,1,1,1,1,1,1,
1,1,1,1,1,1,1,1,1,1,1,1,1,1,1,1,1,1,1,1,1,1,1,1,1,1,1,1,1,1,1,1,1,1,1,1,
1,1,1,1,1,1,1,1,1,1,1,1,1,1,1,1,1,1,1,1,1,1,1,1,1,1,1,1,1,1,1,1,1,1,1,1,
1,1,1,1,1,1,1,1,1,1,1,1,1,1,1,1,1,1,1,1,1,1,1,1,1,1,1,1,1,1,1,1,1,1,1,1,
1,1,1,1,1,1,1,1,1,1,1,1,1,1,1,1,1,1,1,1,1,1,1,1,1,1,1,1,1,1,1,1,1,1,1,6),
(2,2),(0.,0.005,0.01,0.015,0.02,0.025,0.03,0.035,0.04,0.045,0.05,0.055,
0.06,0.065,0.07,0.075,0.08,0.085,0.09,0.095,0.1,0.105,0.11,0.115,0.12,0.125,
0.13,0.135,0.14,0.145,0.15,0.155,0.16,0.165,0.17,0.175,0.18,0.185,0.19,
0.195,0.2,0.205,0.21,0.215,0.22,0.225,0.23,0.235,0.24,0.245,0.25,0.255,
0.26,0.265,0.27,0.275,0.28,0.285,0.29,0.295,0.3,0.305,0.31,0.315,0.32,0.325,
0.33,0.335,0.34,0.345,0.35,0.355,0.36,0.365,0.37,0.375,0.38,0.385,0.39,
0.395,0.4,0.405,0.41,0.415,0.42,0.425,0.43,0.435,0.44,0.445,0.45,0.455,
0.46,0.465,0.47,0.475,0.48,0.485,0.49,0.495,0.5,0.505,0.51,0.515,0.52,0.525,
0.53,0.535,0.54,0.545,0.55,0.555,0.56,0.565,0.57,0.575,0.58,0.585,0.59,
0.595,0.6,0.605,0.61,0.615,0.62,0.625,0.63,0.635,0.64,0.645,0.65,0.655,
0.66,0.665,0.67,0.675,0.68,0.685,0.690000000000001,0.695000000000001,0.700000000000001,
0.705000000000001,0.710000000000001,0.715000000000001,0.720000000000001,
0.725000000000001,0.730000000000001,0.735000000000001,0.740000000000001,
0.745000000000001,0.750000000000001,0.755000000000001,0.760000000000001,
0.765000000000001,0.770000000000001,0.775000000000001,0.780000000000001,
0.785000000000001,0.790000000000001,0.795000000000001,0.800000000000001,
0.805000000000001,0.810000000000001,0.815000000000001,0.820000000000001,
0.825000000000001,0.830000000000001,0.835000000000001,0.840000000000001,
0.845000000000001,0.850000000000001,0.855000000000001,0.860000000000001,
0.865000000000001,0.870000000000001,0.875000000000001,0.880000000000001,
0.885000000000001,0.890000000000001,0.895000000000001,0.900000000000001,
0.905000000000001,0.910000000000001,0.915000000000001,0.920000000000001,
0.925000000000001,0.930000000000001,0.935000000000001,0.940000000000001,
0.945000000000001,0.950000000000001,0.955000000000001,0.960000000000001,
0.965000000000001,0.970000000000001,0.975000000000001,0.980000000000001,
0.985000000000001,0.990000000000001,0.995000000000001,1.),(0.,1.2),
 .UNSPECIFIED.)
GEOMETRIC_REPRESENTATION_ITEM()
RATIONAL_B_SPLINE_SURFACE(((1.,1.),(1.,1.),(1.,1.),(1.,1.),(1.,1.),(1.,
1.),(1.,1.),(1.,1.),(1.,1.),(1.,1.),(1.,1.),(1.,1.),(1.,1.),(1.,1.),(1.,
1.),(1.,1.),(1.,1.),(1.,1.),(1.,1.),(1.,1.),(1.,1.),(1.,1.),(1.,1.),(1.,
1.),(1.,1.),(1.,1.),(1.,1.),(1.,1.),(1.,1.),(1.,1.),(1.,1.),(1.,1.),(1.,
1.),(1.,1.),(1.,1.),(1.,1.),(1.,1.),(1.,1.),(1.,1.),(1.,1.),(1.,1.),(1.,
1.),(1.,1.),(1.,1.),(1.,1.),(1.,1.),(1.,1.),(1.,1.),(1.,1.),(1.,1.),(1.,
1.),(1.,1.),(1.,1.),(1.,1.),(1.,1.),(1.,1.),(1.,1.),(1.,1.),(1.,1.),(1.,
1.),(1.,1.),(1.,1.),(1.,1.),(1.,1.),(1.,1.),(1.,1.),(1.,1.),(1.,1.),(1.,
1.),(1.,1.),(1.,1.),(1.,1.),(1.,1.),(1.,1.),(1.,1.),(1.,1.),(1.,1.),(1.,
1.),(1.,1.),(1.,1.),(1.,1.),(1.,1.),(1.,1.),(1.,1.),(1.,1.),(1.,1.),(1.,
1.),(1.,1.),(1.,1.),(1.,1.),(1.,1.),(1.,1.),(1.,1.),(1.,1.),(1.,1.),(1.,
1.),(1.,1.),(1.,1.),(1.,1.),(1.,1.),(1.,1.),(1.,1.),(1.,1.),(1.,1.),(1.,
1.),(1.,1.),(1.,1.),(1.,1.),(1.,1.),(1.,1.),(1.,1.),(1.,1.),(1.,1.),(1.,
1.),(1.,1.),(1.,1.),(1.,1.),(1.,1.),(1.,1.),(1.,1.),(1.,1.),(1.,1.),(1.,
1.),(1.,1.),(1.,1.),(1.,1.),(1.,1.),(1.,1.),(1.,1.),(1.,1.),(1.,1.),(1.,
1.),(1.,1.),(1.,1.),(1.,1.),(1.,1.),(1.,1.),(1.,1.),(1.,1.),(1.,1.),(1.,
1.),(1.,1.),(1.,1.),(1.,1.),(1.,1.),(1.,1.),(1.,1.),(1.,1.),(1.,1.),(1.,
1.),(1.,1.),(1.,1.),(1.,1.),(1.,1.),(1.,1.),(1.,1.),(1.,1.),(1.,1.),(1.,
1.),(1.,1.),(1.,1.),(1.,1.),(1.,1.),(1.,1.),(1.,1.),(1.,1.),(1.,1.),(1.,
1.),(1.,1.),(1.,1.),(1.,1.),(1.,1.),(1.,1.),(1.,1.),(1.,1.),(1.,1.),(1.,
1.),(1.,1.),(1.,1.),(1.,1.),(1.,1.),(1.,1.),(1.,1.),(1.,1.),(1.,1.),(1.,
1.),(1.,1.),(1.,1.),(1.,1.),(1.,1.),(1.,1.),(1.,1.),(1.,1.),(1.,1.),(1.,
1.),(1.,1.),(1.,1.),(1.,1.),(1.,1.),(1.,1.),(1.,1.),(1.,1.),(1.,1.),(1.,
1.),(1.,1.)))
REPRESENTATION_ITEM('')
SURFACE()
);
#1071=(
BOUNDED_SURFACE()
B_SPLINE_SURFACE(5,1,((#212841,#212842),(#212843,#212844),(#212845,#212846),
(#212847,#212848),(#212849,#212850),(#212851,#212852),(#212853,#212854),
(#212855,#212856),(#212857,#212858),(#212859,#212860),(#212861,#212862),
(#212863,#212864),(#212865,#212866),(#212867,#212868),(#212869,#212870),
(#212871,#212872),(#212873,#212874),(#212875,#212876),(#212877,#212878),
(#212879,#212880),(#212881,#212882),(#212883,#212884),(#212885,#212886),
(#212887,#212888),(#212889,#212890),(#212891,#212892),(#212893,#212894),
(#212895,#212896),(#212897,#212898),(#212899,#212900),(#212901,#212902),
(#212903,#212904),(#212905,#212906),(#212907,#212908),(#212909,#212910),
(#212911,#212912),(#212913,#212914),(#212915,#212916),(#212917,#212918),
(#212919,#212920),(#212921,#212922),(#212923,#212924),(#212925,#212926),
(#212927,#212928),(#212929,#212930),(#212931,#212932),(#212933,#212934),
(#212935,#212936),(#212937,#212938),(#212939,#212940),(#212941,#212942),
(#212943,#212944),(#212945,#212946),(#212947,#212948),(#212949,#212950),
(#212951,#212952),(#212953,#212954),(#212955,#212956),(#212957,#212958),
(#212959,#212960),(#212961,#212962),(#212963,#212964),(#212965,#212966),
(#212967,#212968),(#212969,#212970),(#212971,#212972),(#212973,#212974),
(#212975,#212976),(#212977,#212978),(#212979,#212980),(#212981,#212982),
(#212983,#212984),(#212985,#212986),(#212987,#212988),(#212989,#212990),
(#212991,#212992),(#212993,#212994),(#212995,#212996),(#212997,#212998),
(#212999,#213000),(#213001,#213002),(#213003,#213004),(#213005,#213006),
(#213007,#213008),(#213009,#213010),(#213011,#213012),(#213013,#213014),
(#213015,#213016),(#213017,#213018),(#213019,#213020),(#213021,#213022),
(#213023,#213024),(#213025,#213026),(#213027,#213028),(#213029,#213030),
(#213031,#213032),(#213033,#213034),(#213035,#213036),(#213037,#213038),
(#213039,#213040),(#213041,#213042),(#213043,#213044),(#213045,#213046),
(#213047,#213048),(#213049,#213050),(#213051,#213052),(#213053,#213054),
(#213055,#213056),(#213057,#213058),(#213059,#213060),(#213061,#213062),
(#213063,#213064),(#213065,#213066),(#213067,#213068),(#213069,#213070),
(#213071,#213072),(#213073,#213074),(#213075,#213076),(#213077,#213078),
(#213079,#213080),(#213081,#213082),(#213083,#213084),(#213085,#213086),
(#213087,#213088),(#213089,#213090),(#213091,#213092),(#213093,#213094),
(#213095,#213096),(#213097,#213098),(#213099,#213100),(#213101,#213102),
(#213103,#213104),(#213105,#213106),(#213107,#213108),(#213109,#213110),
(#213111,#213112),(#213113,#213114),(#213115,#213116),(#213117,#213118),
(#213119,#213120),(#213121,#213122),(#213123,#213124),(#213125,#213126),
(#213127,#213128),(#213129,#213130),(#213131,#213132),(#213133,#213134),
(#213135,#213136),(#213137,#213138),(#213139,#213140),(#213141,#213142),
(#213143,#213144),(#213145,#213146),(#213147,#213148),(#213149,#213150),
(#213151,#213152),(#213153,#213154),(#213155,#213156),(#213157,#213158),
(#213159,#213160),(#213161,#213162),(#213163,#213164),(#213165,#213166),
(#213167,#213168),(#213169,#213170),(#213171,#213172),(#213173,#213174),
(#213175,#213176),(#213177,#213178),(#213179,#213180),(#213181,#213182),
(#213183,#213184),(#213185,#213186),(#213187,#213188),(#213189,#213190),
(#213191,#213192),(#213193,#213194),(#213195,#213196),(#213197,#213198),
(#213199,#213200),(#213201,#213202),(#213203,#213204),(#213205,#213206),
(#213207,#213208),(#213209,#213210),(#213211,#213212),(#213213,#213214),
(#213215,#213216),(#213217,#213218),(#213219,#213220),(#213221,#213222),
(#213223,#213224),(#213225,#213226),(#213227,#213228),(#213229,#213230),
(#213231,#213232),(#213233,#213234),(#213235,#213236),(#213237,#213238),
(#213239,#213240),(#213241,#213242),(#213243,#213244),(#213245,#213246),
(#213247,#213248),(#213249,#213250)),.UNSPECIFIED.,.F.,.F.,.F.)
B_SPLINE_SURFACE_WITH_KNOTS((6,1,1,1,1,1,1,1,1,1,1,1,1,1,1,1,1,1,1,1,1,
1,1,1,1,1,1,1,1,1,1,1,1,1,1,1,1,1,1,1,1,1,1,1,1,1,1,1,1,1,1,1,1,1,1,1,1,
1,1,1,1,1,1,1,1,1,1,1,1,1,1,1,1,1,1,1,1,1,1,1,1,1,1,1,1,1,1,1,1,1,1,1,1,
1,1,1,1,1,1,1,1,1,1,1,1,1,1,1,1,1,1,1,1,1,1,1,1,1,1,1,1,1,1,1,1,1,1,1,1,
1,1,1,1,1,1,1,1,1,1,1,1,1,1,1,1,1,1,1,1,1,1,1,1,1,1,1,1,1,1,1,1,1,1,1,1,
1,1,1,1,1,1,1,1,1,1,1,1,1,1,1,1,1,1,1,1,1,1,1,1,1,1,1,1,1,1,1,1,1,1,1,6),
(2,2),(-1.,-0.995000000000001,-0.990000000000001,-0.985000000000001,-0.980000000000001,
-0.975000000000001,-0.970000000000001,-0.965000000000001,-0.960000000000001,
-0.955000000000001,-0.950000000000001,-0.945000000000001,-0.940000000000001,
-0.935000000000001,-0.930000000000001,-0.925000000000001,-0.920000000000001,
-0.915000000000001,-0.910000000000001,-0.905000000000001,-0.900000000000001,
-0.895000000000001,-0.890000000000001,-0.885000000000001,-0.880000000000001,
-0.875000000000001,-0.870000000000001,-0.865000000000001,-0.860000000000001,
-0.855000000000001,-0.850000000000001,-0.845000000000001,-0.840000000000001,
-0.835000000000001,-0.830000000000001,-0.825000000000001,-0.820000000000001,
-0.815000000000001,-0.810000000000001,-0.805000000000001,-0.800000000000001,
-0.795000000000001,-0.790000000000001,-0.785000000000001,-0.780000000000001,
-0.775000000000001,-0.770000000000001,-0.765000000000001,-0.760000000000001,
-0.755000000000001,-0.750000000000001,-0.745000000000001,-0.740000000000001,
-0.735000000000001,-0.730000000000001,-0.725000000000001,-0.720000000000001,
-0.715000000000001,-0.710000000000001,-0.705000000000001,-0.700000000000001,
-0.695000000000001,-0.690000000000001,-0.685,-0.68,-0.675,-0.67,-0.665,
-0.66,-0.655,-0.65,-0.645,-0.64,-0.635,-0.63,-0.625,-0.62,-0.615,-0.61,
-0.605,-0.6,-0.595,-0.59,-0.585,-0.58,-0.575,-0.57,-0.565,-0.56,-0.555,
-0.55,-0.545,-0.54,-0.535,-0.53,-0.525,-0.52,-0.515,-0.51,-0.505,-0.5,-0.495,
-0.49,-0.485,-0.48,-0.475,-0.47,-0.465,-0.46,-0.455,-0.45,-0.445,-0.44,
-0.435,-0.43,-0.425,-0.42,-0.415,-0.41,-0.405,-0.4,-0.395,-0.39,-0.385,
-0.38,-0.375,-0.37,-0.365,-0.36,-0.355,-0.35,-0.345,-0.34,-0.335,-0.33,
-0.325,-0.32,-0.315,-0.31,-0.305,-0.3,-0.295,-0.29,-0.285,-0.28,-0.275,
-0.27,-0.265,-0.26,-0.255,-0.25,-0.245,-0.24,-0.235,-0.23,-0.225,-0.22,
-0.215,-0.21,-0.205,-0.2,-0.195,-0.19,-0.185,-0.18,-0.175,-0.17,-0.165,
-0.16,-0.155,-0.15,-0.145,-0.14,-0.135,-0.13,-0.125,-0.12,-0.115,-0.11,
-0.105,-0.1,-0.095,-0.09,-0.085,-0.08,-0.075,-0.07,-0.065,-0.06,-0.055,
-0.05,-0.045,-0.04,-0.035,-0.03,-0.025,-0.02,-0.015,-0.01,-0.005,0.),(0.,
1.2),.UNSPECIFIED.)
GEOMETRIC_REPRESENTATION_ITEM()
RATIONAL_B_SPLINE_SURFACE(((1.,1.),(1.,1.),(1.,1.),(1.,1.),(1.,1.),(1.,
1.),(1.,1.),(1.,1.),(1.,1.),(1.,1.),(1.,1.),(1.,1.),(1.,1.),(1.,1.),(1.,
1.),(1.,1.),(1.,1.),(1.,1.),(1.,1.),(1.,1.),(1.,1.),(1.,1.),(1.,1.),(1.,
1.),(1.,1.),(1.,1.),(1.,1.),(1.,1.),(1.,1.),(1.,1.),(1.,1.),(1.,1.),(1.,
1.),(1.,1.),(1.,1.),(1.,1.),(1.,1.),(1.,1.),(1.,1.),(1.,1.),(1.,1.),(1.,
1.),(1.,1.),(1.,1.),(1.,1.),(1.,1.),(1.,1.),(1.,1.),(1.,1.),(1.,1.),(1.,
1.),(1.,1.),(1.,1.),(1.,1.),(1.,1.),(1.,1.),(1.,1.),(1.,1.),(1.,1.),(1.,
1.),(1.,1.),(1.,1.),(1.,1.),(1.,1.),(1.,1.),(1.,1.),(1.,1.),(1.,1.),(1.,
1.),(1.,1.),(1.,1.),(1.,1.),(1.,1.),(1.,1.),(1.,1.),(1.,1.),(1.,1.),(1.,
1.),(1.,1.),(1.,1.),(1.,1.),(1.,1.),(1.,1.),(1.,1.),(1.,1.),(1.,1.),(1.,
1.),(1.,1.),(1.,1.),(1.,1.),(1.,1.),(1.,1.),(1.,1.),(1.,1.),(1.,1.),(1.,
1.),(1.,1.),(1.,1.),(1.,1.),(1.,1.),(1.,1.),(1.,1.),(1.,1.),(1.,1.),(1.,
1.),(1.,1.),(1.,1.),(1.,1.),(1.,1.),(1.,1.),(1.,1.),(1.,1.),(1.,1.),(1.,
1.),(1.,1.),(1.,1.),(1.,1.),(1.,1.),(1.,1.),(1.,1.),(1.,1.),(1.,1.),(1.,
1.),(1.,1.),(1.,1.),(1.,1.),(1.,1.),(1.,1.),(1.,1.),(1.,1.),(1.,1.),(1.,
1.),(1.,1.),(1.,1.),(1.,1.),(1.,1.),(1.,1.),(1.,1.),(1.,1.),(1.,1.),(1.,
1.),(1.,1.),(1.,1.),(1.,1.),(1.,1.),(1.,1.),(1.,1.),(1.,1.),(1.,1.),(1.,
1.),(1.,1.),(1.,1.),(1.,1.),(1.,1.),(1.,1.),(1.,1.),(1.,1.),(1.,1.),(1.,
1.),(1.,1.),(1.,1.),(1.,1.),(1.,1.),(1.,1.),(1.,1.),(1.,1.),(1.,1.),(1.,
1.),(1.,1.),(1.,1.),(1.,1.),(1.,1.),(1.,1.),(1.,1.),(1.,1.),(1.,1.),(1.,
1.),(1.,1.),(1.,1.),(1.,1.),(1.,1.),(1.,1.),(1.,1.),(1.,1.),(1.,1.),(1.,
1.),(1.,1.),(1.,1.),(1.,1.),(1.,1.),(1.,1.),(1.,1.),(1.,1.),(1.,1.),(1.,
1.),(1.,1.),(1.,1.),(1.,1.),(1.,1.),(1.,1.),(1.,1.),(1.,1.),(1.,1.),(1.,
1.),(1.,1.)))
REPRESENTATION_ITEM('')
SURFACE()
);
#1072=(
BOUNDED_SURFACE()
B_SPLINE_SURFACE(5,1,((#213458,#213459),(#213460,#213461),(#213462,#213463),
(#213464,#213465),(#213466,#213467),(#213468,#213469),(#213470,#213471),
(#213472,#213473),(#213474,#213475),(#213476,#213477),(#213478,#213479),
(#213480,#213481),(#213482,#213483),(#213484,#213485),(#213486,#213487),
(#213488,#213489),(#213490,#213491),(#213492,#213493),(#213494,#213495),
(#213496,#213497),(#213498,#213499),(#213500,#213501),(#213502,#213503),
(#213504,#213505),(#213506,#213507),(#213508,#213509),(#213510,#213511),
(#213512,#213513),(#213514,#213515),(#213516,#213517),(#213518,#213519),
(#213520,#213521),(#213522,#213523),(#213524,#213525),(#213526,#213527),
(#213528,#213529),(#213530,#213531),(#213532,#213533),(#213534,#213535),
(#213536,#213537),(#213538,#213539),(#213540,#213541),(#213542,#213543),
(#213544,#213545),(#213546,#213547),(#213548,#213549),(#213550,#213551),
(#213552,#213553),(#213554,#213555),(#213556,#213557),(#213558,#213559),
(#213560,#213561),(#213562,#213563),(#213564,#213565),(#213566,#213567),
(#213568,#213569),(#213570,#213571),(#213572,#213573),(#213574,#213575),
(#213576,#213577),(#213578,#213579),(#213580,#213581),(#213582,#213583),
(#213584,#213585),(#213586,#213587),(#213588,#213589),(#213590,#213591),
(#213592,#213593),(#213594,#213595),(#213596,#213597),(#213598,#213599),
(#213600,#213601),(#213602,#213603),(#213604,#213605),(#213606,#213607),
(#213608,#213609),(#213610,#213611),(#213612,#213613),(#213614,#213615),
(#213616,#213617),(#213618,#213619),(#213620,#213621),(#213622,#213623),
(#213624,#213625),(#213626,#213627),(#213628,#213629),(#213630,#213631),
(#213632,#213633),(#213634,#213635),(#213636,#213637),(#213638,#213639),
(#213640,#213641),(#213642,#213643),(#213644,#213645),(#213646,#213647),
(#213648,#213649),(#213650,#213651),(#213652,#213653),(#213654,#213655),
(#213656,#213657),(#213658,#213659),(#213660,#213661),(#213662,#213663),
(#213664,#213665),(#213666,#213667),(#213668,#213669),(#213670,#213671),
(#213672,#213673),(#213674,#213675),(#213676,#213677),(#213678,#213679),
(#213680,#213681),(#213682,#213683),(#213684,#213685),(#213686,#213687),
(#213688,#213689),(#213690,#213691),(#213692,#213693),(#213694,#213695),
(#213696,#213697),(#213698,#213699),(#213700,#213701),(#213702,#213703),
(#213704,#213705),(#213706,#213707),(#213708,#213709),(#213710,#213711),
(#213712,#213713),(#213714,#213715),(#213716,#213717),(#213718,#213719),
(#213720,#213721),(#213722,#213723),(#213724,#213725),(#213726,#213727),
(#213728,#213729),(#213730,#213731),(#213732,#213733),(#213734,#213735),
(#213736,#213737),(#213738,#213739),(#213740,#213741),(#213742,#213743),
(#213744,#213745),(#213746,#213747),(#213748,#213749),(#213750,#213751),
(#213752,#213753),(#213754,#213755),(#213756,#213757),(#213758,#213759),
(#213760,#213761),(#213762,#213763),(#213764,#213765),(#213766,#213767),
(#213768,#213769),(#213770,#213771),(#213772,#213773),(#213774,#213775),
(#213776,#213777),(#213778,#213779),(#213780,#213781),(#213782,#213783),
(#213784,#213785),(#213786,#213787),(#213788,#213789),(#213790,#213791),
(#213792,#213793),(#213794,#213795),(#213796,#213797),(#213798,#213799),
(#213800,#213801),(#213802,#213803),(#213804,#213805),(#213806,#213807),
(#213808,#213809),(#213810,#213811),(#213812,#213813),(#213814,#213815),
(#213816,#213817),(#213818,#213819),(#213820,#213821),(#213822,#213823),
(#213824,#213825),(#213826,#213827),(#213828,#213829),(#213830,#213831),
(#213832,#213833),(#213834,#213835),(#213836,#213837),(#213838,#213839),
(#213840,#213841),(#213842,#213843),(#213844,#213845),(#213846,#213847),
(#213848,#213849),(#213850,#213851),(#213852,#213853),(#213854,#213855),
(#213856,#213857),(#213858,#213859),(#213860,#213861),(#213862,#213863),
(#213864,#213865),(#213866,#213867)),.UNSPECIFIED.,.F.,.F.,.F.)
B_SPLINE_SURFACE_WITH_KNOTS((6,1,1,1,1,1,1,1,1,1,1,1,1,1,1,1,1,1,1,1,1,
1,1,1,1,1,1,1,1,1,1,1,1,1,1,1,1,1,1,1,1,1,1,1,1,1,1,1,1,1,1,1,1,1,1,1,1,
1,1,1,1,1,1,1,1,1,1,1,1,1,1,1,1,1,1,1,1,1,1,1,1,1,1,1,1,1,1,1,1,1,1,1,1,
1,1,1,1,1,1,1,1,1,1,1,1,1,1,1,1,1,1,1,1,1,1,1,1,1,1,1,1,1,1,1,1,1,1,1,1,
1,1,1,1,1,1,1,1,1,1,1,1,1,1,1,1,1,1,1,1,1,1,1,1,1,1,1,1,1,1,1,1,1,1,1,1,
1,1,1,1,1,1,1,1,1,1,1,1,1,1,1,1,1,1,1,1,1,1,1,1,1,1,1,1,1,1,1,1,1,1,1,6),
(2,2),(0.,0.005,0.01,0.015,0.02,0.025,0.03,0.035,0.04,0.045,0.05,0.055,
0.06,0.065,0.07,0.075,0.08,0.085,0.09,0.095,0.1,0.105,0.11,0.115,0.12,0.125,
0.13,0.135,0.14,0.145,0.15,0.155,0.16,0.165,0.17,0.175,0.18,0.185,0.19,
0.195,0.2,0.205,0.21,0.215,0.22,0.225,0.23,0.235,0.24,0.245,0.25,0.255,
0.26,0.265,0.27,0.275,0.28,0.285,0.29,0.295,0.3,0.305,0.31,0.315,0.32,0.325,
0.33,0.335,0.34,0.345,0.35,0.355,0.36,0.365,0.37,0.375,0.38,0.385,0.39,
0.395,0.4,0.405,0.41,0.415,0.42,0.425,0.43,0.435,0.44,0.445,0.45,0.455,
0.46,0.465,0.47,0.475,0.48,0.485,0.49,0.495,0.5,0.505,0.51,0.515,0.52,0.525,
0.53,0.535,0.54,0.545,0.55,0.555,0.56,0.565,0.57,0.575,0.58,0.585,0.59,
0.595,0.6,0.605,0.61,0.615,0.62,0.625,0.63,0.635,0.64,0.645,0.65,0.655,
0.66,0.665,0.67,0.675,0.68,0.685,0.690000000000001,0.695000000000001,0.700000000000001,
0.705000000000001,0.710000000000001,0.715000000000001,0.720000000000001,
0.725000000000001,0.730000000000001,0.735000000000001,0.740000000000001,
0.745000000000001,0.750000000000001,0.755000000000001,0.760000000000001,
0.765000000000001,0.770000000000001,0.775000000000001,0.780000000000001,
0.785000000000001,0.790000000000001,0.795000000000001,0.800000000000001,
0.805000000000001,0.810000000000001,0.815000000000001,0.820000000000001,
0.825000000000001,0.830000000000001,0.835000000000001,0.840000000000001,
0.845000000000001,0.850000000000001,0.855000000000001,0.860000000000001,
0.865000000000001,0.870000000000001,0.875000000000001,0.880000000000001,
0.885000000000001,0.890000000000001,0.895000000000001,0.900000000000001,
0.905000000000001,0.910000000000001,0.915000000000001,0.920000000000001,
0.925000000000001,0.930000000000001,0.935000000000001,0.940000000000001,
0.945000000000001,0.950000000000001,0.955000000000001,0.960000000000001,
0.965000000000001,0.970000000000001,0.975000000000001,0.980000000000001,
0.985000000000001,0.990000000000001,0.995000000000001,1.),(0.,1.2),
 .UNSPECIFIED.)
GEOMETRIC_REPRESENTATION_ITEM()
RATIONAL_B_SPLINE_SURFACE(((1.,1.),(1.,1.),(1.,1.),(1.,1.),(1.,1.),(1.,
1.),(1.,1.),(1.,1.),(1.,1.),(1.,1.),(1.,1.),(1.,1.),(1.,1.),(1.,1.),(1.,
1.),(1.,1.),(1.,1.),(1.,1.),(1.,1.),(1.,1.),(1.,1.),(1.,1.),(1.,1.),(1.,
1.),(1.,1.),(1.,1.),(1.,1.),(1.,1.),(1.,1.),(1.,1.),(1.,1.),(1.,1.),(1.,
1.),(1.,1.),(1.,1.),(1.,1.),(1.,1.),(1.,1.),(1.,1.),(1.,1.),(1.,1.),(1.,
1.),(1.,1.),(1.,1.),(1.,1.),(1.,1.),(1.,1.),(1.,1.),(1.,1.),(1.,1.),(1.,
1.),(1.,1.),(1.,1.),(1.,1.),(1.,1.),(1.,1.),(1.,1.),(1.,1.),(1.,1.),(1.,
1.),(1.,1.),(1.,1.),(1.,1.),(1.,1.),(1.,1.),(1.,1.),(1.,1.),(1.,1.),(1.,
1.),(1.,1.),(1.,1.),(1.,1.),(1.,1.),(1.,1.),(1.,1.),(1.,1.),(1.,1.),(1.,
1.),(1.,1.),(1.,1.),(1.,1.),(1.,1.),(1.,1.),(1.,1.),(1.,1.),(1.,1.),(1.,
1.),(1.,1.),(1.,1.),(1.,1.),(1.,1.),(1.,1.),(1.,1.),(1.,1.),(1.,1.),(1.,
1.),(1.,1.),(1.,1.),(1.,1.),(1.,1.),(1.,1.),(1.,1.),(1.,1.),(1.,1.),(1.,
1.),(1.,1.),(1.,1.),(1.,1.),(1.,1.),(1.,1.),(1.,1.),(1.,1.),(1.,1.),(1.,
1.),(1.,1.),(1.,1.),(1.,1.),(1.,1.),(1.,1.),(1.,1.),(1.,1.),(1.,1.),(1.,
1.),(1.,1.),(1.,1.),(1.,1.),(1.,1.),(1.,1.),(1.,1.),(1.,1.),(1.,1.),(1.,
1.),(1.,1.),(1.,1.),(1.,1.),(1.,1.),(1.,1.),(1.,1.),(1.,1.),(1.,1.),(1.,
1.),(1.,1.),(1.,1.),(1.,1.),(1.,1.),(1.,1.),(1.,1.),(1.,1.),(1.,1.),(1.,
1.),(1.,1.),(1.,1.),(1.,1.),(1.,1.),(1.,1.),(1.,1.),(1.,1.),(1.,1.),(1.,
1.),(1.,1.),(1.,1.),(1.,1.),(1.,1.),(1.,1.),(1.,1.),(1.,1.),(1.,1.),(1.,
1.),(1.,1.),(1.,1.),(1.,1.),(1.,1.),(1.,1.),(1.,1.),(1.,1.),(1.,1.),(1.,
1.),(1.,1.),(1.,1.),(1.,1.),(1.,1.),(1.,1.),(1.,1.),(1.,1.),(1.,1.),(1.,
1.),(1.,1.),(1.,1.),(1.,1.),(1.,1.),(1.,1.),(1.,1.),(1.,1.),(1.,1.),(1.,
1.),(1.,1.),(1.,1.),(1.,1.),(1.,1.),(1.,1.),(1.,1.),(1.,1.),(1.,1.),(1.,
1.),(1.,1.)))
REPRESENTATION_ITEM('')
SURFACE()
);
#1073=(
BOUNDED_SURFACE()
B_SPLINE_SURFACE(5,1,((#214558,#214559),(#214560,#214561),(#214562,#214563),
(#214564,#214565),(#214566,#214567),(#214568,#214569),(#214570,#214571),
(#214572,#214573),(#214574,#214575),(#214576,#214577),(#214578,#214579),
(#214580,#214581),(#214582,#214583),(#214584,#214585),(#214586,#214587),
(#214588,#214589),(#214590,#214591),(#214592,#214593),(#214594,#214595),
(#214596,#214597),(#214598,#214599),(#214600,#214601),(#214602,#214603),
(#214604,#214605),(#214606,#214607),(#214608,#214609),(#214610,#214611),
(#214612,#214613),(#214614,#214615),(#214616,#214617),(#214618,#214619),
(#214620,#214621),(#214622,#214623),(#214624,#214625),(#214626,#214627),
(#214628,#214629),(#214630,#214631),(#214632,#214633),(#214634,#214635),
(#214636,#214637),(#214638,#214639),(#214640,#214641),(#214642,#214643),
(#214644,#214645),(#214646,#214647),(#214648,#214649),(#214650,#214651),
(#214652,#214653),(#214654,#214655),(#214656,#214657),(#214658,#214659),
(#214660,#214661),(#214662,#214663),(#214664,#214665),(#214666,#214667),
(#214668,#214669),(#214670,#214671),(#214672,#214673),(#214674,#214675),
(#214676,#214677),(#214678,#214679),(#214680,#214681),(#214682,#214683),
(#214684,#214685),(#214686,#214687),(#214688,#214689),(#214690,#214691),
(#214692,#214693),(#214694,#214695),(#214696,#214697),(#214698,#214699),
(#214700,#214701),(#214702,#214703),(#214704,#214705),(#214706,#214707),
(#214708,#214709),(#214710,#214711),(#214712,#214713),(#214714,#214715),
(#214716,#214717),(#214718,#214719),(#214720,#214721),(#214722,#214723),
(#214724,#214725),(#214726,#214727),(#214728,#214729),(#214730,#214731),
(#214732,#214733),(#214734,#214735),(#214736,#214737),(#214738,#214739),
(#214740,#214741),(#214742,#214743),(#214744,#214745),(#214746,#214747),
(#214748,#214749),(#214750,#214751),(#214752,#214753),(#214754,#214755),
(#214756,#214757),(#214758,#214759),(#214760,#214761),(#214762,#214763),
(#214764,#214765),(#214766,#214767),(#214768,#214769),(#214770,#214771),
(#214772,#214773),(#214774,#214775),(#214776,#214777),(#214778,#214779),
(#214780,#214781),(#214782,#214783),(#214784,#214785),(#214786,#214787),
(#214788,#214789),(#214790,#214791),(#214792,#214793),(#214794,#214795),
(#214796,#214797),(#214798,#214799),(#214800,#214801),(#214802,#214803),
(#214804,#214805),(#214806,#214807),(#214808,#214809),(#214810,#214811),
(#214812,#214813),(#214814,#214815),(#214816,#214817),(#214818,#214819),
(#214820,#214821),(#214822,#214823),(#214824,#214825),(#214826,#214827),
(#214828,#214829),(#214830,#214831),(#214832,#214833),(#214834,#214835),
(#214836,#214837),(#214838,#214839),(#214840,#214841),(#214842,#214843),
(#214844,#214845),(#214846,#214847),(#214848,#214849),(#214850,#214851),
(#214852,#214853),(#214854,#214855),(#214856,#214857),(#214858,#214859),
(#214860,#214861),(#214862,#214863),(#214864,#214865),(#214866,#214867),
(#214868,#214869),(#214870,#214871),(#214872,#214873),(#214874,#214875),
(#214876,#214877),(#214878,#214879),(#214880,#214881),(#214882,#214883),
(#214884,#214885),(#214886,#214887),(#214888,#214889),(#214890,#214891),
(#214892,#214893),(#214894,#214895),(#214896,#214897),(#214898,#214899),
(#214900,#214901),(#214902,#214903),(#214904,#214905),(#214906,#214907),
(#214908,#214909),(#214910,#214911),(#214912,#214913),(#214914,#214915),
(#214916,#214917),(#214918,#214919),(#214920,#214921),(#214922,#214923),
(#214924,#214925),(#214926,#214927),(#214928,#214929),(#214930,#214931),
(#214932,#214933),(#214934,#214935),(#214936,#214937),(#214938,#214939),
(#214940,#214941),(#214942,#214943),(#214944,#214945),(#214946,#214947),
(#214948,#214949),(#214950,#214951),(#214952,#214953),(#214954,#214955),
(#214956,#214957),(#214958,#214959),(#214960,#214961),(#214962,#214963),
(#214964,#214965),(#214966,#214967)),.UNSPECIFIED.,.F.,.F.,.F.)
B_SPLINE_SURFACE_WITH_KNOTS((6,1,1,1,1,1,1,1,1,1,1,1,1,1,1,1,1,1,1,1,1,
1,1,1,1,1,1,1,1,1,1,1,1,1,1,1,1,1,1,1,1,1,1,1,1,1,1,1,1,1,1,1,1,1,1,1,1,
1,1,1,1,1,1,1,1,1,1,1,1,1,1,1,1,1,1,1,1,1,1,1,1,1,1,1,1,1,1,1,1,1,1,1,1,
1,1,1,1,1,1,1,1,1,1,1,1,1,1,1,1,1,1,1,1,1,1,1,1,1,1,1,1,1,1,1,1,1,1,1,1,
1,1,1,1,1,1,1,1,1,1,1,1,1,1,1,1,1,1,1,1,1,1,1,1,1,1,1,1,1,1,1,1,1,1,1,1,
1,1,1,1,1,1,1,1,1,1,1,1,1,1,1,1,1,1,1,1,1,1,1,1,1,1,1,1,1,1,1,1,1,1,1,6),
(2,2),(-1.,-0.995000000000001,-0.990000000000001,-0.985000000000001,-0.980000000000001,
-0.975000000000001,-0.970000000000001,-0.965000000000001,-0.960000000000001,
-0.955000000000001,-0.950000000000001,-0.945000000000001,-0.940000000000001,
-0.935000000000001,-0.930000000000001,-0.925000000000001,-0.920000000000001,
-0.915000000000001,-0.910000000000001,-0.905000000000001,-0.900000000000001,
-0.895000000000001,-0.890000000000001,-0.885000000000001,-0.880000000000001,
-0.875000000000001,-0.870000000000001,-0.865000000000001,-0.860000000000001,
-0.855000000000001,-0.850000000000001,-0.845000000000001,-0.840000000000001,
-0.835000000000001,-0.830000000000001,-0.825000000000001,-0.820000000000001,
-0.815000000000001,-0.810000000000001,-0.805000000000001,-0.800000000000001,
-0.795000000000001,-0.790000000000001,-0.785000000000001,-0.780000000000001,
-0.775000000000001,-0.770000000000001,-0.765000000000001,-0.760000000000001,
-0.755000000000001,-0.750000000000001,-0.745000000000001,-0.740000000000001,
-0.735000000000001,-0.730000000000001,-0.725000000000001,-0.720000000000001,
-0.715000000000001,-0.710000000000001,-0.705000000000001,-0.700000000000001,
-0.695000000000001,-0.690000000000001,-0.685,-0.68,-0.675,-0.67,-0.665,
-0.66,-0.655,-0.65,-0.645,-0.64,-0.635,-0.63,-0.625,-0.62,-0.615,-0.61,
-0.605,-0.6,-0.595,-0.59,-0.585,-0.58,-0.575,-0.57,-0.565,-0.56,-0.555,
-0.55,-0.545,-0.54,-0.535,-0.53,-0.525,-0.52,-0.515,-0.51,-0.505,-0.5,-0.495,
-0.49,-0.485,-0.48,-0.475,-0.47,-0.465,-0.46,-0.455,-0.45,-0.445,-0.44,
-0.435,-0.43,-0.425,-0.42,-0.415,-0.41,-0.405,-0.4,-0.395,-0.39,-0.385,
-0.38,-0.375,-0.37,-0.365,-0.36,-0.355,-0.35,-0.345,-0.34,-0.335,-0.33,
-0.325,-0.32,-0.315,-0.31,-0.305,-0.3,-0.295,-0.29,-0.285,-0.28,-0.275,
-0.27,-0.265,-0.26,-0.255,-0.25,-0.245,-0.24,-0.235,-0.23,-0.225,-0.22,
-0.215,-0.21,-0.205,-0.2,-0.195,-0.19,-0.185,-0.18,-0.175,-0.17,-0.165,
-0.16,-0.155,-0.15,-0.145,-0.14,-0.135,-0.13,-0.125,-0.12,-0.115,-0.11,
-0.105,-0.1,-0.095,-0.09,-0.085,-0.08,-0.075,-0.07,-0.065,-0.06,-0.055,
-0.05,-0.045,-0.04,-0.035,-0.03,-0.025,-0.02,-0.015,-0.01,-0.005,0.),(0.,
1.2),.UNSPECIFIED.)
GEOMETRIC_REPRESENTATION_ITEM()
RATIONAL_B_SPLINE_SURFACE(((1.,1.),(1.,1.),(1.,1.),(1.,1.),(1.,1.),(1.,
1.),(1.,1.),(1.,1.),(1.,1.),(1.,1.),(1.,1.),(1.,1.),(1.,1.),(1.,1.),(1.,
1.),(1.,1.),(1.,1.),(1.,1.),(1.,1.),(1.,1.),(1.,1.),(1.,1.),(1.,1.),(1.,
1.),(1.,1.),(1.,1.),(1.,1.),(1.,1.),(1.,1.),(1.,1.),(1.,1.),(1.,1.),(1.,
1.),(1.,1.),(1.,1.),(1.,1.),(1.,1.),(1.,1.),(1.,1.),(1.,1.),(1.,1.),(1.,
1.),(1.,1.),(1.,1.),(1.,1.),(1.,1.),(1.,1.),(1.,1.),(1.,1.),(1.,1.),(1.,
1.),(1.,1.),(1.,1.),(1.,1.),(1.,1.),(1.,1.),(1.,1.),(1.,1.),(1.,1.),(1.,
1.),(1.,1.),(1.,1.),(1.,1.),(1.,1.),(1.,1.),(1.,1.),(1.,1.),(1.,1.),(1.,
1.),(1.,1.),(1.,1.),(1.,1.),(1.,1.),(1.,1.),(1.,1.),(1.,1.),(1.,1.),(1.,
1.),(1.,1.),(1.,1.),(1.,1.),(1.,1.),(1.,1.),(1.,1.),(1.,1.),(1.,1.),(1.,
1.),(1.,1.),(1.,1.),(1.,1.),(1.,1.),(1.,1.),(1.,1.),(1.,1.),(1.,1.),(1.,
1.),(1.,1.),(1.,1.),(1.,1.),(1.,1.),(1.,1.),(1.,1.),(1.,1.),(1.,1.),(1.,
1.),(1.,1.),(1.,1.),(1.,1.),(1.,1.),(1.,1.),(1.,1.),(1.,1.),(1.,1.),(1.,
1.),(1.,1.),(1.,1.),(1.,1.),(1.,1.),(1.,1.),(1.,1.),(1.,1.),(1.,1.),(1.,
1.),(1.,1.),(1.,1.),(1.,1.),(1.,1.),(1.,1.),(1.,1.),(1.,1.),(1.,1.),(1.,
1.),(1.,1.),(1.,1.),(1.,1.),(1.,1.),(1.,1.),(1.,1.),(1.,1.),(1.,1.),(1.,
1.),(1.,1.),(1.,1.),(1.,1.),(1.,1.),(1.,1.),(1.,1.),(1.,1.),(1.,1.),(1.,
1.),(1.,1.),(1.,1.),(1.,1.),(1.,1.),(1.,1.),(1.,1.),(1.,1.),(1.,1.),(1.,
1.),(1.,1.),(1.,1.),(1.,1.),(1.,1.),(1.,1.),(1.,1.),(1.,1.),(1.,1.),(1.,
1.),(1.,1.),(1.,1.),(1.,1.),(1.,1.),(1.,1.),(1.,1.),(1.,1.),(1.,1.),(1.,
1.),(1.,1.),(1.,1.),(1.,1.),(1.,1.),(1.,1.),(1.,1.),(1.,1.),(1.,1.),(1.,
1.),(1.,1.),(1.,1.),(1.,1.),(1.,1.),(1.,1.),(1.,1.),(1.,1.),(1.,1.),(1.,
1.),(1.,1.),(1.,1.),(1.,1.),(1.,1.),(1.,1.),(1.,1.),(1.,1.),(1.,1.),(1.,
1.),(1.,1.)))
REPRESENTATION_ITEM('')
SURFACE()
);
#1074=(
BOUNDED_SURFACE()
B_SPLINE_SURFACE(5,1,((#214968,#214969),(#214970,#214971),(#214972,#214973),
(#214974,#214975),(#214976,#214977),(#214978,#214979),(#214980,#214981),
(#214982,#214983),(#214984,#214985),(#214986,#214987),(#214988,#214989),
(#214990,#214991),(#214992,#214993),(#214994,#214995),(#214996,#214997),
(#214998,#214999),(#215000,#215001),(#215002,#215003),(#215004,#215005),
(#215006,#215007),(#215008,#215009),(#215010,#215011),(#215012,#215013),
(#215014,#215015),(#215016,#215017),(#215018,#215019),(#215020,#215021),
(#215022,#215023),(#215024,#215025),(#215026,#215027),(#215028,#215029),
(#215030,#215031),(#215032,#215033),(#215034,#215035),(#215036,#215037),
(#215038,#215039),(#215040,#215041),(#215042,#215043),(#215044,#215045),
(#215046,#215047),(#215048,#215049),(#215050,#215051),(#215052,#215053),
(#215054,#215055),(#215056,#215057),(#215058,#215059),(#215060,#215061),
(#215062,#215063),(#215064,#215065),(#215066,#215067),(#215068,#215069),
(#215070,#215071),(#215072,#215073),(#215074,#215075),(#215076,#215077),
(#215078,#215079),(#215080,#215081),(#215082,#215083),(#215084,#215085),
(#215086,#215087),(#215088,#215089),(#215090,#215091),(#215092,#215093),
(#215094,#215095),(#215096,#215097),(#215098,#215099),(#215100,#215101),
(#215102,#215103),(#215104,#215105),(#215106,#215107),(#215108,#215109),
(#215110,#215111),(#215112,#215113),(#215114,#215115),(#215116,#215117),
(#215118,#215119),(#215120,#215121),(#215122,#215123),(#215124,#215125),
(#215126,#215127),(#215128,#215129),(#215130,#215131),(#215132,#215133),
(#215134,#215135),(#215136,#215137),(#215138,#215139),(#215140,#215141),
(#215142,#215143),(#215144,#215145),(#215146,#215147),(#215148,#215149),
(#215150,#215151),(#215152,#215153),(#215154,#215155),(#215156,#215157),
(#215158,#215159),(#215160,#215161),(#215162,#215163),(#215164,#215165),
(#215166,#215167),(#215168,#215169),(#215170,#215171),(#215172,#215173),
(#215174,#215175),(#215176,#215177),(#215178,#215179),(#215180,#215181),
(#215182,#215183),(#215184,#215185),(#215186,#215187),(#215188,#215189),
(#215190,#215191),(#215192,#215193),(#215194,#215195),(#215196,#215197),
(#215198,#215199),(#215200,#215201),(#215202,#215203),(#215204,#215205),
(#215206,#215207),(#215208,#215209),(#215210,#215211),(#215212,#215213),
(#215214,#215215),(#215216,#215217),(#215218,#215219),(#215220,#215221),
(#215222,#215223),(#215224,#215225),(#215226,#215227),(#215228,#215229),
(#215230,#215231),(#215232,#215233),(#215234,#215235),(#215236,#215237),
(#215238,#215239),(#215240,#215241),(#215242,#215243),(#215244,#215245),
(#215246,#215247),(#215248,#215249),(#215250,#215251),(#215252,#215253),
(#215254,#215255),(#215256,#215257),(#215258,#215259),(#215260,#215261),
(#215262,#215263),(#215264,#215265),(#215266,#215267),(#215268,#215269),
(#215270,#215271),(#215272,#215273),(#215274,#215275),(#215276,#215277),
(#215278,#215279),(#215280,#215281),(#215282,#215283),(#215284,#215285),
(#215286,#215287),(#215288,#215289),(#215290,#215291),(#215292,#215293),
(#215294,#215295),(#215296,#215297),(#215298,#215299),(#215300,#215301),
(#215302,#215303),(#215304,#215305),(#215306,#215307),(#215308,#215309),
(#215310,#215311),(#215312,#215313),(#215314,#215315),(#215316,#215317),
(#215318,#215319),(#215320,#215321),(#215322,#215323),(#215324,#215325),
(#215326,#215327),(#215328,#215329),(#215330,#215331),(#215332,#215333),
(#215334,#215335),(#215336,#215337),(#215338,#215339),(#215340,#215341),
(#215342,#215343),(#215344,#215345),(#215346,#215347),(#215348,#215349),
(#215350,#215351),(#215352,#215353),(#215354,#215355),(#215356,#215357),
(#215358,#215359),(#215360,#215361),(#215362,#215363),(#215364,#215365),
(#215366,#215367),(#215368,#215369),(#215370,#215371),(#215372,#215373),
(#215374,#215375),(#215376,#215377)),.UNSPECIFIED.,.F.,.F.,.F.)
B_SPLINE_SURFACE_WITH_KNOTS((6,1,1,1,1,1,1,1,1,1,1,1,1,1,1,1,1,1,1,1,1,
1,1,1,1,1,1,1,1,1,1,1,1,1,1,1,1,1,1,1,1,1,1,1,1,1,1,1,1,1,1,1,1,1,1,1,1,
1,1,1,1,1,1,1,1,1,1,1,1,1,1,1,1,1,1,1,1,1,1,1,1,1,1,1,1,1,1,1,1,1,1,1,1,
1,1,1,1,1,1,1,1,1,1,1,1,1,1,1,1,1,1,1,1,1,1,1,1,1,1,1,1,1,1,1,1,1,1,1,1,
1,1,1,1,1,1,1,1,1,1,1,1,1,1,1,1,1,1,1,1,1,1,1,1,1,1,1,1,1,1,1,1,1,1,1,1,
1,1,1,1,1,1,1,1,1,1,1,1,1,1,1,1,1,1,1,1,1,1,1,1,1,1,1,1,1,1,1,1,1,1,1,6),
(2,2),(0.,0.005,0.01,0.015,0.02,0.025,0.03,0.035,0.04,0.045,0.05,0.055,
0.06,0.065,0.07,0.075,0.08,0.085,0.09,0.095,0.1,0.105,0.11,0.115,0.12,0.125,
0.13,0.135,0.14,0.145,0.15,0.155,0.16,0.165,0.17,0.175,0.18,0.185,0.19,
0.195,0.2,0.205,0.21,0.215,0.22,0.225,0.23,0.235,0.24,0.245,0.25,0.255,
0.26,0.265,0.27,0.275,0.28,0.285,0.29,0.295,0.3,0.305,0.31,0.315,0.32,0.325,
0.33,0.335,0.34,0.345,0.35,0.355,0.36,0.365,0.37,0.375,0.38,0.385,0.39,
0.395,0.4,0.405,0.41,0.415,0.42,0.425,0.43,0.435,0.44,0.445,0.45,0.455,
0.46,0.465,0.47,0.475,0.48,0.485,0.49,0.495,0.5,0.505,0.51,0.515,0.52,0.525,
0.53,0.535,0.54,0.545,0.55,0.555,0.56,0.565,0.57,0.575,0.58,0.585,0.59,
0.595,0.6,0.605,0.61,0.615,0.62,0.625,0.63,0.635,0.64,0.645,0.65,0.655,
0.66,0.665,0.67,0.675,0.68,0.685,0.690000000000001,0.695000000000001,0.700000000000001,
0.705000000000001,0.710000000000001,0.715000000000001,0.720000000000001,
0.725000000000001,0.730000000000001,0.735000000000001,0.740000000000001,
0.745000000000001,0.750000000000001,0.755000000000001,0.760000000000001,
0.765000000000001,0.770000000000001,0.775000000000001,0.780000000000001,
0.785000000000001,0.790000000000001,0.795000000000001,0.800000000000001,
0.805000000000001,0.810000000000001,0.815000000000001,0.820000000000001,
0.825000000000001,0.830000000000001,0.835000000000001,0.840000000000001,
0.845000000000001,0.850000000000001,0.855000000000001,0.860000000000001,
0.865000000000001,0.870000000000001,0.875000000000001,0.880000000000001,
0.885000000000001,0.890000000000001,0.895000000000001,0.900000000000001,
0.905000000000001,0.910000000000001,0.915000000000001,0.920000000000001,
0.925000000000001,0.930000000000001,0.935000000000001,0.940000000000001,
0.945000000000001,0.950000000000001,0.955000000000001,0.960000000000001,
0.965000000000001,0.970000000000001,0.975000000000001,0.980000000000001,
0.985000000000001,0.990000000000001,0.995000000000001,1.),(0.,1.2),
 .UNSPECIFIED.)
GEOMETRIC_REPRESENTATION_ITEM()
RATIONAL_B_SPLINE_SURFACE(((1.,1.),(1.,1.),(1.,1.),(1.,1.),(1.,1.),(1.,
1.),(1.,1.),(1.,1.),(1.,1.),(1.,1.),(1.,1.),(1.,1.),(1.,1.),(1.,1.),(1.,
1.),(1.,1.),(1.,1.),(1.,1.),(1.,1.),(1.,1.),(1.,1.),(1.,1.),(1.,1.),(1.,
1.),(1.,1.),(1.,1.),(1.,1.),(1.,1.),(1.,1.),(1.,1.),(1.,1.),(1.,1.),(1.,
1.),(1.,1.),(1.,1.),(1.,1.),(1.,1.),(1.,1.),(1.,1.),(1.,1.),(1.,1.),(1.,
1.),(1.,1.),(1.,1.),(1.,1.),(1.,1.),(1.,1.),(1.,1.),(1.,1.),(1.,1.),(1.,
1.),(1.,1.),(1.,1.),(1.,1.),(1.,1.),(1.,1.),(1.,1.),(1.,1.),(1.,1.),(1.,
1.),(1.,1.),(1.,1.),(1.,1.),(1.,1.),(1.,1.),(1.,1.),(1.,1.),(1.,1.),(1.,
1.),(1.,1.),(1.,1.),(1.,1.),(1.,1.),(1.,1.),(1.,1.),(1.,1.),(1.,1.),(1.,
1.),(1.,1.),(1.,1.),(1.,1.),(1.,1.),(1.,1.),(1.,1.),(1.,1.),(1.,1.),(1.,
1.),(1.,1.),(1.,1.),(1.,1.),(1.,1.),(1.,1.),(1.,1.),(1.,1.),(1.,1.),(1.,
1.),(1.,1.),(1.,1.),(1.,1.),(1.,1.),(1.,1.),(1.,1.),(1.,1.),(1.,1.),(1.,
1.),(1.,1.),(1.,1.),(1.,1.),(1.,1.),(1.,1.),(1.,1.),(1.,1.),(1.,1.),(1.,
1.),(1.,1.),(1.,1.),(1.,1.),(1.,1.),(1.,1.),(1.,1.),(1.,1.),(1.,1.),(1.,
1.),(1.,1.),(1.,1.),(1.,1.),(1.,1.),(1.,1.),(1.,1.),(1.,1.),(1.,1.),(1.,
1.),(1.,1.),(1.,1.),(1.,1.),(1.,1.),(1.,1.),(1.,1.),(1.,1.),(1.,1.),(1.,
1.),(1.,1.),(1.,1.),(1.,1.),(1.,1.),(1.,1.),(1.,1.),(1.,1.),(1.,1.),(1.,
1.),(1.,1.),(1.,1.),(1.,1.),(1.,1.),(1.,1.),(1.,1.),(1.,1.),(1.,1.),(1.,
1.),(1.,1.),(1.,1.),(1.,1.),(1.,1.),(1.,1.),(1.,1.),(1.,1.),(1.,1.),(1.,
1.),(1.,1.),(1.,1.),(1.,1.),(1.,1.),(1.,1.),(1.,1.),(1.,1.),(1.,1.),(1.,
1.),(1.,1.),(1.,1.),(1.,1.),(1.,1.),(1.,1.),(1.,1.),(1.,1.),(1.,1.),(1.,
1.),(1.,1.),(1.,1.),(1.,1.),(1.,1.),(1.,1.),(1.,1.),(1.,1.),(1.,1.),(1.,
1.),(1.,1.),(1.,1.),(1.,1.),(1.,1.),(1.,1.),(1.,1.),(1.,1.),(1.,1.),(1.,
1.),(1.,1.)))
REPRESENTATION_ITEM('')
SURFACE()
);
#1128=SHAPE_REPRESENTATION_RELATIONSHIP('SRR','None',#259375,#1148);
#1148=ADVANCED_BREP_SHAPE_REPRESENTATION('',(#1188),#259209);
#1168=STYLED_ITEM('',(#259484),#1188);
#1188=MANIFOLD_SOLID_BREP('Gear blank',#25155);
#1281=FACE_BOUND('',#3936,.T.);
#1282=FACE_BOUND('',#4099,.T.);
#1532=PLANE('',#26315);
#1533=PLANE('',#26316);
#1534=PLANE('',#26317);
#1535=PLANE('',#26321);
#1536=PLANE('',#26420);
#1537=PLANE('',#26427);
#1538=PLANE('',#26434);
#1539=PLANE('',#26441);
#1540=PLANE('',#26448);
#1541=PLANE('',#26455);
#1542=PLANE('',#26462);
#1543=PLANE('',#26469);
#1544=PLANE('',#26476);
#1545=PLANE('',#26483);
#1546=PLANE('',#26490);
#1547=PLANE('',#26497);
#1548=PLANE('',#26504);
#1549=PLANE('',#26511);
#1550=PLANE('',#26518);
#1551=PLANE('',#26525);
#1552=PLANE('',#26532);
#1553=PLANE('',#26539);
#1554=PLANE('',#26546);
#1555=PLANE('',#26553);
#1556=PLANE('',#26560);
#1557=PLANE('',#26567);
#1558=PLANE('',#26574);
#1559=PLANE('',#26579);
#1560=PLANE('',#26580);
#1561=PLANE('',#26581);
#1562=PLANE('',#26582);
#1563=PLANE('',#26583);
#1564=PLANE('',#26584);
#1565=PLANE('',#26585);
#1566=PLANE('',#26586);
#1567=PLANE('',#26587);
#1568=PLANE('',#26588);
#1569=PLANE('',#26589);
#1570=PLANE('',#26590);
#1571=PLANE('',#26591);
#1572=PLANE('',#26592);
#1573=PLANE('',#26593);
#1574=PLANE('',#26594);
#1575=PLANE('',#26595);
#1576=PLANE('',#26596);
#1577=PLANE('',#26597);
#1578=PLANE('',#26598);
#1579=PLANE('',#26599);
#1580=PLANE('',#26600);
#1581=PLANE('',#26601);
#1582=PLANE('',#26602);
#1583=PLANE('',#26654);
#1584=PLANE('',#26657);
#2507=FACE_OUTER_BOUND('',#3931,.T.);
#2508=FACE_OUTER_BOUND('',#3932,.T.);
#2509=FACE_OUTER_BOUND('',#3933,.T.);
#2510=FACE_OUTER_BOUND('',#3934,.T.);
#2511=FACE_OUTER_BOUND('',#3935,.T.);
#2512=FACE_OUTER_BOUND('',#3937,.T.);
#2513=FACE_OUTER_BOUND('',#3938,.T.);
#2514=FACE_OUTER_BOUND('',#3939,.T.);
#2515=FACE_OUTER_BOUND('',#3940,.T.);
#2516=FACE_OUTER_BOUND('',#3941,.T.);
#2517=FACE_OUTER_BOUND('',#3942,.T.);
#2518=FACE_OUTER_BOUND('',#3943,.T.);
#2519=FACE_OUTER_BOUND('',#3944,.T.);
#2520=FACE_OUTER_BOUND('',#3945,.T.);
#2521=FACE_OUTER_BOUND('',#3946,.T.);
#2522=FACE_OUTER_BOUND('',#3947,.T.);
#2523=FACE_OUTER_BOUND('',#3948,.T.);
#2524=FACE_OUTER_BOUND('',#3949,.T.);
#2525=FACE_OUTER_BOUND('',#3950,.T.);
#2526=FACE_OUTER_BOUND('',#3951,.T.);
#2527=FACE_OUTER_BOUND('',#3952,.T.);
#2528=FACE_OUTER_BOUND('',#3953,.T.);
#2529=FACE_OUTER_BOUND('',#3954,.T.);
#2530=FACE_OUTER_BOUND('',#3955,.T.);
#2531=FACE_OUTER_BOUND('',#3956,.T.);
#2532=FACE_OUTER_BOUND('',#3957,.T.);
#2533=FACE_OUTER_BOUND('',#3958,.T.);
#2534=FACE_OUTER_BOUND('',#3959,.T.);
#2535=FACE_OUTER_BOUND('',#3960,.T.);
#2536=FACE_OUTER_BOUND('',#3961,.T.);
#2537=FACE_OUTER_BOUND('',#3962,.T.);
#2538=FACE_OUTER_BOUND('',#3963,.T.);
#2539=FACE_OUTER_BOUND('',#3964,.T.);
#2540=FACE_OUTER_BOUND('',#3965,.T.);
#2541=FACE_OUTER_BOUND('',#3966,.T.);
#2542=FACE_OUTER_BOUND('',#3967,.T.);
#2543=FACE_OUTER_BOUND('',#3968,.T.);
#2544=FACE_OUTER_BOUND('',#3969,.T.);
#2545=FACE_OUTER_BOUND('',#3970,.T.);
#2546=FACE_OUTER_BOUND('',#3971,.T.);
#2547=FACE_OUTER_BOUND('',#3972,.T.);
#2548=FACE_OUTER_BOUND('',#3973,.T.);
#2549=FACE_OUTER_BOUND('',#3974,.T.);
#2550=FACE_OUTER_BOUND('',#3975,.T.);
#2551=FACE_OUTER_BOUND('',#3976,.T.);
#2552=FACE_OUTER_BOUND('',#3977,.T.);
#2553=FACE_OUTER_BOUND('',#3978,.T.);
#2554=FACE_OUTER_BOUND('',#3979,.T.);
#2555=FACE_OUTER_BOUND('',#3980,.T.);
#2556=FACE_OUTER_BOUND('',#3981,.T.);
#2557=FACE_OUTER_BOUND('',#3982,.T.);
#2558=FACE_OUTER_BOUND('',#3983,.T.);
#2559=FACE_OUTER_BOUND('',#3984,.T.);
#2560=FACE_OUTER_BOUND('',#3985,.T.);
#2561=FACE_OUTER_BOUND('',#3986,.T.);
#2562=FACE_OUTER_BOUND('',#3987,.T.);
#2563=FACE_OUTER_BOUND('',#3988,.T.);
#2564=FACE_OUTER_BOUND('',#3989,.T.);
#2565=FACE_OUTER_BOUND('',#3990,.T.);
#2566=FACE_OUTER_BOUND('',#3991,.T.);
#2567=FACE_OUTER_BOUND('',#3992,.T.);
#2568=FACE_OUTER_BOUND('',#3993,.T.);
#2569=FACE_OUTER_BOUND('',#3994,.T.);
#2570=FACE_OUTER_BOUND('',#3995,.T.);
#2571=FACE_OUTER_BOUND('',#3996,.T.);
#2572=FACE_OUTER_BOUND('',#3997,.T.);
#2573=FACE_OUTER_BOUND('',#3998,.T.);
#2574=FACE_OUTER_BOUND('',#3999,.T.);
#2575=FACE_OUTER_BOUND('',#4000,.T.);
#2576=FACE_OUTER_BOUND('',#4001,.T.);
#2577=FACE_OUTER_BOUND('',#4002,.T.);
#2578=FACE_OUTER_BOUND('',#4003,.T.);
#2579=FACE_OUTER_BOUND('',#4004,.T.);
#2580=FACE_OUTER_BOUND('',#4005,.T.);
#2581=FACE_OUTER_BOUND('',#4006,.T.);
#2582=FACE_OUTER_BOUND('',#4007,.T.);
#2583=FACE_OUTER_BOUND('',#4008,.T.);
#2584=FACE_OUTER_BOUND('',#4009,.T.);
#2585=FACE_OUTER_BOUND('',#4010,.T.);
#2586=FACE_OUTER_BOUND('',#4011,.T.);
#2587=FACE_OUTER_BOUND('',#4012,.T.);
#2588=FACE_OUTER_BOUND('',#4013,.T.);
#2589=FACE_OUTER_BOUND('',#4014,.T.);
#2590=FACE_OUTER_BOUND('',#4015,.T.);
#2591=FACE_OUTER_BOUND('',#4016,.T.);
#2592=FACE_OUTER_BOUND('',#4017,.T.);
#2593=FACE_OUTER_BOUND('',#4018,.T.);
#2594=FACE_OUTER_BOUND('',#4019,.T.);
#2595=FACE_OUTER_BOUND('',#4020,.T.);
#2596=FACE_OUTER_BOUND('',#4021,.T.);
#2597=FACE_OUTER_BOUND('',#4022,.T.);
#2598=FACE_OUTER_BOUND('',#4023,.T.);
#2599=FACE_OUTER_BOUND('',#4024,.T.);
#2600=FACE_OUTER_BOUND('',#4025,.T.);
#2601=FACE_OUTER_BOUND('',#4026,.T.);
#2602=FACE_OUTER_BOUND('',#4027,.T.);
#2603=FACE_OUTER_BOUND('',#4028,.T.);
#2604=FACE_OUTER_BOUND('',#4029,.T.);
#2605=FACE_OUTER_BOUND('',#4030,.T.);
#2606=FACE_OUTER_BOUND('',#4031,.T.);
#2607=FACE_OUTER_BOUND('',#4032,.T.);
#2608=FACE_OUTER_BOUND('',#4033,.T.);
#2609=FACE_OUTER_BOUND('',#4034,.T.);
#2610=FACE_OUTER_BOUND('',#4035,.T.);
#2611=FACE_OUTER_BOUND('',#4036,.T.);
#2612=FACE_OUTER_BOUND('',#4037,.T.);
#2613=FACE_OUTER_BOUND('',#4038,.T.);
#2614=FACE_OUTER_BOUND('',#4039,.T.);
#2615=FACE_OUTER_BOUND('',#4040,.T.);
#2616=FACE_OUTER_BOUND('',#4041,.T.);
#2617=FACE_OUTER_BOUND('',#4042,.T.);
#2618=FACE_OUTER_BOUND('',#4043,.T.);
#2619=FACE_OUTER_BOUND('',#4044,.T.);
#2620=FACE_OUTER_BOUND('',#4045,.T.);
#2621=FACE_OUTER_BOUND('',#4046,.T.);
#2622=FACE_OUTER_BOUND('',#4047,.T.);
#2623=FACE_OUTER_BOUND('',#4048,.T.);
#2624=FACE_OUTER_BOUND('',#4049,.T.);
#2625=FACE_OUTER_BOUND('',#4050,.T.);
#2626=FACE_OUTER_BOUND('',#4051,.T.);
#2627=FACE_OUTER_BOUND('',#4052,.T.);
#2628=FACE_OUTER_BOUND('',#4053,.T.);
#2629=FACE_OUTER_BOUND('',#4054,.T.);
#2630=FACE_OUTER_BOUND('',#4055,.T.);
#2631=FACE_OUTER_BOUND('',#4056,.T.);
#2632=FACE_OUTER_BOUND('',#4057,.T.);
#2633=FACE_OUTER_BOUND('',#4058,.T.);
#2634=FACE_OUTER_BOUND('',#4059,.T.);
#2635=FACE_OUTER_BOUND('',#4060,.T.);
#2636=FACE_OUTER_BOUND('',#4061,.T.);
#2637=FACE_OUTER_BOUND('',#4062,.T.);
#2638=FACE_OUTER_BOUND('',#4063,.T.);
#2639=FACE_OUTER_BOUND('',#4064,.T.);
#2640=FACE_OUTER_BOUND('',#4065,.T.);
#2641=FACE_OUTER_BOUND('',#4066,.T.);
#2642=FACE_OUTER_BOUND('',#4067,.T.);
#2643=FACE_OUTER_BOUND('',#4068,.T.);
#2644=FACE_OUTER_BOUND('',#4069,.T.);
#2645=FACE_OUTER_BOUND('',#4070,.T.);
#2646=FACE_OUTER_BOUND('',#4071,.T.);
#2647=FACE_OUTER_BOUND('',#4072,.T.);
#2648=FACE_OUTER_BOUND('',#4073,.T.);
#2649=FACE_OUTER_BOUND('',#4074,.T.);
#2650=FACE_OUTER_BOUND('',#4075,.T.);
#2651=FACE_OUTER_BOUND('',#4076,.T.);
#2652=FACE_OUTER_BOUND('',#4077,.T.);
#2653=FACE_OUTER_BOUND('',#4078,.T.);
#2654=FACE_OUTER_BOUND('',#4079,.T.);
#2655=FACE_OUTER_BOUND('',#4080,.T.);
#2656=FACE_OUTER_BOUND('',#4081,.T.);
#2657=FACE_OUTER_BOUND('',#4082,.T.);
#2658=FACE_OUTER_BOUND('',#4083,.T.);
#2659=FACE_OUTER_BOUND('',#4084,.T.);
#2660=FACE_OUTER_BOUND('',#4085,.T.);
#2661=FACE_OUTER_BOUND('',#4086,.T.);
#2662=FACE_OUTER_BOUND('',#4087,.T.);
#2663=FACE_OUTER_BOUND('',#4088,.T.);
#2664=FACE_OUTER_BOUND('',#4089,.T.);
#2665=FACE_OUTER_BOUND('',#4090,.T.);
#2666=FACE_OUTER_BOUND('',#4091,.T.);
#2667=FACE_OUTER_BOUND('',#4092,.T.);
#2668=FACE_OUTER_BOUND('',#4093,.T.);
#2669=FACE_OUTER_BOUND('',#4094,.T.);
#2670=FACE_OUTER_BOUND('',#4095,.T.);
#2671=FACE_OUTER_BOUND('',#4096,.T.);
#2672=FACE_OUTER_BOUND('',#4097,.T.);
#2673=FACE_OUTER_BOUND('',#4098,.T.);
#2674=FACE_OUTER_BOUND('',#4100,.T.);
#2675=FACE_OUTER_BOUND('',#4101,.T.);
#2676=FACE_OUTER_BOUND('',#4102,.T.);
#2677=FACE_OUTER_BOUND('',#4103,.T.);
#2678=FACE_OUTER_BOUND('',#4104,.T.);
#2679=FACE_OUTER_BOUND('',#4105,.T.);
#2680=FACE_OUTER_BOUND('',#4106,.T.);
#2681=FACE_OUTER_BOUND('',#4107,.T.);
#2682=FACE_OUTER_BOUND('',#4108,.T.);
#2683=FACE_OUTER_BOUND('',#4109,.T.);
#2684=FACE_OUTER_BOUND('',#4110,.T.);
#2685=FACE_OUTER_BOUND('',#4111,.T.);
#2686=FACE_OUTER_BOUND('',#4112,.T.);
#2687=FACE_OUTER_BOUND('',#4113,.T.);
#2688=FACE_OUTER_BOUND('',#4114,.T.);
#2689=FACE_OUTER_BOUND('',#4115,.T.);
#2690=FACE_OUTER_BOUND('',#4116,.T.);
#2691=FACE_OUTER_BOUND('',#4117,.T.);
#2692=FACE_OUTER_BOUND('',#4118,.T.);
#2693=FACE_OUTER_BOUND('',#4119,.T.);
#2694=FACE_OUTER_BOUND('',#4120,.T.);
#2695=FACE_OUTER_BOUND('',#4121,.T.);
#2696=FACE_OUTER_BOUND('',#4122,.T.);
#2697=FACE_OUTER_BOUND('',#4123,.T.);
#2698=FACE_OUTER_BOUND('',#4124,.T.);
#2699=FACE_OUTER_BOUND('',#4125,.T.);
#2700=FACE_OUTER_BOUND('',#4126,.T.);
#2701=FACE_OUTER_BOUND('',#4127,.T.);
#2702=FACE_OUTER_BOUND('',#4128,.T.);
#2703=FACE_OUTER_BOUND('',#4129,.T.);
#2704=FACE_OUTER_BOUND('',#4130,.T.);
#3931=EDGE_LOOP('',(#20138,#20139,#20140,#20141));
#3932=EDGE_LOOP('',(#20142,#20143,#20144,#20145));
#3933=EDGE_LOOP('',(#20146,#20147,#20148,#20149));
#3934=EDGE_LOOP('',(#20150,#20151,#20152,#20153));
#3935=EDGE_LOOP('',(#20154,#20155,#20156,#20157,#20158,#20159,#20160,#20161,
#20162,#20163,#20164,#20165,#20166,#20167,#20168,#20169,#20170,#20171,#20172,
#20173,#20174,#20175,#20176,#20177,#20178,#20179,#20180,#20181,#20182,#20183,
#20184,#20185,#20186,#20187,#20188,#20189,#20190,#20191,#20192,#20193,#20194,
#20195,#20196,#20197,#20198,#20199,#20200,#20201,#20202,#20203,#20204,#20205,
#20206,#20207,#20208,#20209,#20210,#20211,#20212,#20213,#20214,#20215,#20216,
#20217,#20218,#20219,#20220,#20221,#20222,#20223,#20224,#20225,#20226,#20227,
#20228,#20229,#20230,#20231,#20232,#20233,#20234,#20235,#20236,#20237,#20238,
#20239,#20240,#20241,#20242,#20243,#20244,#20245,#20246,#20247,#20248,#20249,
#20250,#20251,#20252,#20253,#20254,#20255,#20256,#20257,#20258,#20259,#20260,
#20261,#20262,#20263,#20264,#20265,#20266,#20267,#20268,#20269,#20270,#20271,
#20272,#20273,#20274,#20275,#20276,#20277,#20278,#20279,#20280,#20281,#20282,
#20283,#20284,#20285,#20286,#20287,#20288,#20289,#20290,#20291,#20292,#20293,
#20294,#20295,#20296,#20297,#20298,#20299,#20300,#20301,#20302,#20303,#20304,
#20305,#20306,#20307,#20308,#20309,#20310,#20311,#20312,#20313,#20314,#20315,
#20316,#20317,#20318,#20319,#20320,#20321,#20322,#20323,#20324,#20325,#20326,
#20327,#20328,#20329,#20330,#20331,#20332,#20333,#20334,#20335,#20336,#20337,
#20338,#20339,#20340,#20341,#20342,#20343,#20344,#20345));
#3936=EDGE_LOOP('',(#20346,#20347,#20348,#20349));
#3937=EDGE_LOOP('',(#20350,#20351,#20352,#20353));
#3938=EDGE_LOOP('',(#20354,#20355,#20356,#20357));
#3939=EDGE_LOOP('',(#20358,#20359,#20360,#20361));
#3940=EDGE_LOOP('',(#20362,#20363,#20364,#20365));
#3941=EDGE_LOOP('',(#20366,#20367,#20368,#20369));
#3942=EDGE_LOOP('',(#20370,#20371,#20372,#20373));
#3943=EDGE_LOOP('',(#20374,#20375,#20376,#20377));
#3944=EDGE_LOOP('',(#20378,#20379,#20380,#20381));
#3945=EDGE_LOOP('',(#20382,#20383,#20384,#20385));
#3946=EDGE_LOOP('',(#20386,#20387,#20388,#20389));
#3947=EDGE_LOOP('',(#20390,#20391,#20392,#20393));
#3948=EDGE_LOOP('',(#20394,#20395,#20396,#20397));
#3949=EDGE_LOOP('',(#20398,#20399,#20400,#20401));
#3950=EDGE_LOOP('',(#20402,#20403,#20404,#20405));
#3951=EDGE_LOOP('',(#20406,#20407,#20408,#20409));
#3952=EDGE_LOOP('',(#20410,#20411,#20412,#20413));
#3953=EDGE_LOOP('',(#20414,#20415,#20416,#20417));
#3954=EDGE_LOOP('',(#20418,#20419,#20420,#20421));
#3955=EDGE_LOOP('',(#20422,#20423,#20424,#20425));
#3956=EDGE_LOOP('',(#20426,#20427,#20428,#20429));
#3957=EDGE_LOOP('',(#20430,#20431,#20432,#20433));
#3958=EDGE_LOOP('',(#20434,#20435,#20436,#20437));
#3959=EDGE_LOOP('',(#20438,#20439,#20440,#20441));
#3960=EDGE_LOOP('',(#20442,#20443,#20444,#20445));
#3961=EDGE_LOOP('',(#20446,#20447,#20448,#20449));
#3962=EDGE_LOOP('',(#20450,#20451,#20452,#20453));
#3963=EDGE_LOOP('',(#20454,#20455,#20456,#20457));
#3964=EDGE_LOOP('',(#20458,#20459,#20460,#20461));
#3965=EDGE_LOOP('',(#20462,#20463,#20464,#20465));
#3966=EDGE_LOOP('',(#20466,#20467,#20468,#20469));
#3967=EDGE_LOOP('',(#20470,#20471,#20472,#20473));
#3968=EDGE_LOOP('',(#20474,#20475,#20476,#20477));
#3969=EDGE_LOOP('',(#20478,#20479,#20480,#20481));
#3970=EDGE_LOOP('',(#20482,#20483,#20484,#20485));
#3971=EDGE_LOOP('',(#20486,#20487,#20488,#20489));
#3972=EDGE_LOOP('',(#20490,#20491,#20492,#20493));
#3973=EDGE_LOOP('',(#20494,#20495,#20496,#20497));
#3974=EDGE_LOOP('',(#20498,#20499,#20500,#20501));
#3975=EDGE_LOOP('',(#20502,#20503,#20504,#20505));
#3976=EDGE_LOOP('',(#20506,#20507,#20508,#20509));
#3977=EDGE_LOOP('',(#20510,#20511,#20512,#20513));
#3978=EDGE_LOOP('',(#20514,#20515,#20516,#20517));
#3979=EDGE_LOOP('',(#20518,#20519,#20520,#20521));
#3980=EDGE_LOOP('',(#20522,#20523,#20524,#20525));
#3981=EDGE_LOOP('',(#20526,#20527,#20528,#20529));
#3982=EDGE_LOOP('',(#20530,#20531,#20532,#20533));
#3983=EDGE_LOOP('',(#20534,#20535,#20536,#20537));
#3984=EDGE_LOOP('',(#20538,#20539,#20540,#20541));
#3985=EDGE_LOOP('',(#20542,#20543,#20544,#20545));
#3986=EDGE_LOOP('',(#20546,#20547,#20548,#20549));
#3987=EDGE_LOOP('',(#20550,#20551,#20552,#20553));
#3988=EDGE_LOOP('',(#20554,#20555,#20556,#20557));
#3989=EDGE_LOOP('',(#20558,#20559,#20560,#20561));
#3990=EDGE_LOOP('',(#20562,#20563,#20564,#20565));
#3991=EDGE_LOOP('',(#20566,#20567,#20568,#20569));
#3992=EDGE_LOOP('',(#20570,#20571,#20572,#20573));
#3993=EDGE_LOOP('',(#20574,#20575,#20576,#20577));
#3994=EDGE_LOOP('',(#20578,#20579,#20580,#20581));
#3995=EDGE_LOOP('',(#20582,#20583,#20584,#20585));
#3996=EDGE_LOOP('',(#20586,#20587,#20588,#20589));
#3997=EDGE_LOOP('',(#20590,#20591,#20592,#20593));
#3998=EDGE_LOOP('',(#20594,#20595,#20596,#20597));
#3999=EDGE_LOOP('',(#20598,#20599,#20600,#20601));
#4000=EDGE_LOOP('',(#20602,#20603,#20604,#20605));
#4001=EDGE_LOOP('',(#20606,#20607,#20608,#20609));
#4002=EDGE_LOOP('',(#20610,#20611,#20612,#20613));
#4003=EDGE_LOOP('',(#20614,#20615,#20616,#20617));
#4004=EDGE_LOOP('',(#20618,#20619,#20620,#20621));
#4005=EDGE_LOOP('',(#20622,#20623,#20624,#20625));
#4006=EDGE_LOOP('',(#20626,#20627,#20628,#20629));
#4007=EDGE_LOOP('',(#20630,#20631,#20632,#20633));
#4008=EDGE_LOOP('',(#20634,#20635,#20636,#20637));
#4009=EDGE_LOOP('',(#20638,#20639,#20640,#20641));
#4010=EDGE_LOOP('',(#20642,#20643,#20644,#20645));
#4011=EDGE_LOOP('',(#20646,#20647,#20648,#20649));
#4012=EDGE_LOOP('',(#20650,#20651,#20652,#20653));
#4013=EDGE_LOOP('',(#20654,#20655,#20656,#20657));
#4014=EDGE_LOOP('',(#20658,#20659,#20660,#20661));
#4015=EDGE_LOOP('',(#20662,#20663,#20664,#20665));
#4016=EDGE_LOOP('',(#20666,#20667,#20668,#20669));
#4017=EDGE_LOOP('',(#20670,#20671,#20672,#20673));
#4018=EDGE_LOOP('',(#20674,#20675,#20676,#20677));
#4019=EDGE_LOOP('',(#20678,#20679,#20680,#20681));
#4020=EDGE_LOOP('',(#20682,#20683,#20684,#20685));
#4021=EDGE_LOOP('',(#20686,#20687,#20688,#20689));
#4022=EDGE_LOOP('',(#20690,#20691,#20692,#20693));
#4023=EDGE_LOOP('',(#20694,#20695,#20696,#20697));
#4024=EDGE_LOOP('',(#20698,#20699,#20700,#20701));
#4025=EDGE_LOOP('',(#20702,#20703,#20704,#20705));
#4026=EDGE_LOOP('',(#20706,#20707,#20708,#20709));
#4027=EDGE_LOOP('',(#20710,#20711,#20712,#20713));
#4028=EDGE_LOOP('',(#20714,#20715,#20716,#20717));
#4029=EDGE_LOOP('',(#20718,#20719,#20720,#20721));
#4030=EDGE_LOOP('',(#20722,#20723,#20724,#20725));
#4031=EDGE_LOOP('',(#20726,#20727,#20728,#20729));
#4032=EDGE_LOOP('',(#20730,#20731,#20732,#20733));
#4033=EDGE_LOOP('',(#20734,#20735,#20736,#20737));
#4034=EDGE_LOOP('',(#20738,#20739,#20740,#20741));
#4035=EDGE_LOOP('',(#20742,#20743,#20744,#20745));
#4036=EDGE_LOOP('',(#20746,#20747,#20748,#20749));
#4037=EDGE_LOOP('',(#20750,#20751,#20752,#20753));
#4038=EDGE_LOOP('',(#20754,#20755,#20756,#20757));
#4039=EDGE_LOOP('',(#20758,#20759,#20760,#20761));
#4040=EDGE_LOOP('',(#20762,#20763,#20764,#20765));
#4041=EDGE_LOOP('',(#20766,#20767,#20768,#20769));
#4042=EDGE_LOOP('',(#20770,#20771,#20772,#20773));
#4043=EDGE_LOOP('',(#20774,#20775,#20776,#20777));
#4044=EDGE_LOOP('',(#20778,#20779,#20780,#20781));
#4045=EDGE_LOOP('',(#20782,#20783,#20784,#20785));
#4046=EDGE_LOOP('',(#20786,#20787,#20788,#20789));
#4047=EDGE_LOOP('',(#20790,#20791,#20792,#20793));
#4048=EDGE_LOOP('',(#20794,#20795,#20796,#20797));
#4049=EDGE_LOOP('',(#20798,#20799,#20800,#20801));
#4050=EDGE_LOOP('',(#20802,#20803,#20804,#20805));
#4051=EDGE_LOOP('',(#20806,#20807,#20808,#20809));
#4052=EDGE_LOOP('',(#20810,#20811,#20812,#20813));
#4053=EDGE_LOOP('',(#20814,#20815,#20816,#20817));
#4054=EDGE_LOOP('',(#20818,#20819,#20820,#20821));
#4055=EDGE_LOOP('',(#20822,#20823,#20824,#20825));
#4056=EDGE_LOOP('',(#20826,#20827,#20828,#20829));
#4057=EDGE_LOOP('',(#20830,#20831,#20832,#20833));
#4058=EDGE_LOOP('',(#20834,#20835,#20836,#20837));
#4059=EDGE_LOOP('',(#20838,#20839,#20840,#20841));
#4060=EDGE_LOOP('',(#20842,#20843,#20844,#20845));
#4061=EDGE_LOOP('',(#20846,#20847,#20848,#20849));
#4062=EDGE_LOOP('',(#20850,#20851,#20852,#20853));
#4063=EDGE_LOOP('',(#20854,#20855,#20856,#20857));
#4064=EDGE_LOOP('',(#20858,#20859,#20860,#20861));
#4065=EDGE_LOOP('',(#20862,#20863,#20864,#20865));
#4066=EDGE_LOOP('',(#20866,#20867,#20868,#20869));
#4067=EDGE_LOOP('',(#20870,#20871,#20872,#20873));
#4068=EDGE_LOOP('',(#20874,#20875,#20876,#20877));
#4069=EDGE_LOOP('',(#20878,#20879,#20880,#20881));
#4070=EDGE_LOOP('',(#20882,#20883,#20884,#20885));
#4071=EDGE_LOOP('',(#20886,#20887,#20888,#20889));
#4072=EDGE_LOOP('',(#20890,#20891,#20892,#20893));
#4073=EDGE_LOOP('',(#20894,#20895,#20896,#20897));
#4074=EDGE_LOOP('',(#20898,#20899,#20900,#20901));
#4075=EDGE_LOOP('',(#20902,#20903,#20904,#20905));
#4076=EDGE_LOOP('',(#20906,#20907,#20908,#20909));
#4077=EDGE_LOOP('',(#20910,#20911,#20912,#20913));
#4078=EDGE_LOOP('',(#20914,#20915,#20916,#20917));
#4079=EDGE_LOOP('',(#20918,#20919,#20920,#20921));
#4080=EDGE_LOOP('',(#20922,#20923,#20924,#20925));
#4081=EDGE_LOOP('',(#20926,#20927,#20928,#20929));
#4082=EDGE_LOOP('',(#20930,#20931,#20932,#20933));
#4083=EDGE_LOOP('',(#20934,#20935,#20936,#20937));
#4084=EDGE_LOOP('',(#20938,#20939,#20940,#20941));
#4085=EDGE_LOOP('',(#20942,#20943,#20944,#20945));
#4086=EDGE_LOOP('',(#20946,#20947,#20948,#20949));
#4087=EDGE_LOOP('',(#20950,#20951,#20952,#20953));
#4088=EDGE_LOOP('',(#20954,#20955,#20956,#20957));
#4089=EDGE_LOOP('',(#20958,#20959,#20960,#20961));
#4090=EDGE_LOOP('',(#20962,#20963,#20964,#20965));
#4091=EDGE_LOOP('',(#20966,#20967,#20968,#20969));
#4092=EDGE_LOOP('',(#20970,#20971,#20972,#20973));
#4093=EDGE_LOOP('',(#20974,#20975,#20976,#20977));
#4094=EDGE_LOOP('',(#20978,#20979,#20980,#20981));
#4095=EDGE_LOOP('',(#20982,#20983,#20984,#20985));
#4096=EDGE_LOOP('',(#20986,#20987,#20988,#20989));
#4097=EDGE_LOOP('',(#20990,#20991,#20992,#20993));
#4098=EDGE_LOOP('',(#20994,#20995,#20996,#20997,#20998,#20999,#21000,#21001,
#21002,#21003,#21004,#21005,#21006,#21007,#21008,#21009,#21010,#21011,#21012,
#21013,#21014,#21015,#21016,#21017,#21018,#21019,#21020,#21021,#21022,#21023,
#21024,#21025,#21026,#21027,#21028,#21029,#21030,#21031,#21032,#21033,#21034,
#21035,#21036,#21037,#21038,#21039,#21040,#21041,#21042,#21043,#21044,#21045,
#21046,#21047,#21048,#21049,#21050,#21051,#21052,#21053,#21054,#21055,#21056,
#21057,#21058,#21059,#21060,#21061,#21062,#21063,#21064,#21065,#21066,#21067,
#21068,#21069,#21070,#21071,#21072,#21073,#21074,#21075,#21076,#21077,#21078,
#21079,#21080,#21081,#21082,#21083,#21084,#21085,#21086,#21087,#21088,#21089,
#21090,#21091,#21092,#21093,#21094,#21095,#21096,#21097,#21098,#21099,#21100,
#21101,#21102,#21103,#21104,#21105,#21106,#21107,#21108,#21109,#21110,#21111,
#21112,#21113,#21114,#21115,#21116,#21117,#21118,#21119,#21120,#21121,#21122,
#21123,#21124,#21125,#21126,#21127,#21128,#21129,#21130,#21131,#21132,#21133,
#21134,#21135,#21136,#21137,#21138,#21139,#21140,#21141,#21142,#21143,#21144,
#21145,#21146,#21147,#21148,#21149,#21150,#21151,#21152,#21153,#21154,#21155,
#21156,#21157,#21158,#21159,#21160,#21161,#21162,#21163,#21164,#21165,#21166,
#21167,#21168,#21169,#21170,#21171,#21172,#21173,#21174,#21175,#21176,#21177,
#21178,#21179,#21180,#21181,#21182,#21183,#21184,#21185));
#4099=EDGE_LOOP('',(#21186,#21187,#21188,#21189));
#4100=EDGE_LOOP('',(#21190,#21191,#21192,#21193));
#4101=EDGE_LOOP('',(#21194,#21195,#21196,#21197));
#4102=EDGE_LOOP('',(#21198,#21199,#21200,#21201));
#4103=EDGE_LOOP('',(#21202,#21203,#21204,#21205));
#4104=EDGE_LOOP('',(#21206,#21207,#21208,#21209));
#4105=EDGE_LOOP('',(#21210,#21211,#21212,#21213));
#4106=EDGE_LOOP('',(#21214,#21215,#21216,#21217));
#4107=EDGE_LOOP('',(#21218,#21219,#21220,#21221));
#4108=EDGE_LOOP('',(#21222,#21223,#21224,#21225));
#4109=EDGE_LOOP('',(#21226,#21227,#21228,#21229));
#4110=EDGE_LOOP('',(#21230,#21231,#21232,#21233));
#4111=EDGE_LOOP('',(#21234,#21235,#21236,#21237));
#4112=EDGE_LOOP('',(#21238,#21239,#21240,#21241));
#4113=EDGE_LOOP('',(#21242,#21243,#21244,#21245));
#4114=EDGE_LOOP('',(#21246,#21247,#21248,#21249));
#4115=EDGE_LOOP('',(#21250,#21251,#21252,#21253));
#4116=EDGE_LOOP('',(#21254,#21255,#21256,#21257));
#4117=EDGE_LOOP('',(#21258,#21259,#21260,#21261));
#4118=EDGE_LOOP('',(#21262,#21263,#21264,#21265));
#4119=EDGE_LOOP('',(#21266,#21267,#21268,#21269));
#4120=EDGE_LOOP('',(#21270,#21271,#21272,#21273));
#4121=EDGE_LOOP('',(#21274,#21275,#21276,#21277));
#4122=EDGE_LOOP('',(#21278,#21279,#21280,#21281));
#4123=EDGE_LOOP('',(#21282,#21283,#21284,#21285));
#4124=EDGE_LOOP('',(#21286,#21287,#21288,#21289));
#4125=EDGE_LOOP('',(#21290,#21291,#21292,#21293));
#4126=EDGE_LOOP('',(#21294,#21295,#21296,#21297));
#4127=EDGE_LOOP('',(#21298,#21299,#21300,#21301));
#4128=EDGE_LOOP('',(#21302,#21303,#21304,#21305));
#4129=EDGE_LOOP('',(#21306,#21307,#21308,#21309));
#4130=EDGE_LOOP('',(#21310,#21311,#21312,#21313));
#4917=CIRCLE('',#26319,8.);
#4918=CIRCLE('',#26320,8.);
#4919=CIRCLE('',#26322,26.);
#4920=CIRCLE('',#26323,0.5);
#4921=CIRCLE('',#26324,21.4999999999992);
#4922=CIRCLE('',#26325,0.5);
#4923=CIRCLE('',#26326,26.);
#4924=CIRCLE('',#26327,0.5);
#4925=CIRCLE('',#26328,21.4999999999992);
#4926=CIRCLE('',#26329,0.5);
#4927=CIRCLE('',#26330,26.);
#4928=CIRCLE('',#26331,0.5);
#4929=CIRCLE('',#26332,21.4999999999992);
#4930=CIRCLE('',#26333,0.5);
#4931=CIRCLE('',#26334,26.);
#4932=CIRCLE('',#26335,0.5);
#4933=CIRCLE('',#26336,21.4999999999992);
#4934=CIRCLE('',#26337,0.5);
#4935=CIRCLE('',#26338,26.);
#4936=CIRCLE('',#26339,0.5);
#4937=CIRCLE('',#26340,21.4999999999992);
#4938=CIRCLE('',#26341,0.5);
#4939=CIRCLE('',#26342,26.);
#4940=CIRCLE('',#26343,0.5);
#4941=CIRCLE('',#26344,21.4999999999992);
#4942=CIRCLE('',#26345,0.5);
#4943=CIRCLE('',#26346,26.);
#4944=CIRCLE('',#26347,0.5);
#4945=CIRCLE('',#26348,21.4999999999992);
#4946=CIRCLE('',#26349,0.5);
#4947=CIRCLE('',#26350,26.);
#4948=CIRCLE('',#26351,0.5);
#4949=CIRCLE('',#26352,21.4999999999992);
#4950=CIRCLE('',#26353,0.5);
#4951=CIRCLE('',#26354,26.);
#4952=CIRCLE('',#26355,0.5);
#4953=CIRCLE('',#26356,21.4999999999992);
#4954=CIRCLE('',#26357,0.5);
#4955=CIRCLE('',#26358,26.);
#4956=CIRCLE('',#26359,0.5);
#4957=CIRCLE('',#26360,21.4999999999992);
#4958=CIRCLE('',#26361,0.5);
#4959=CIRCLE('',#26362,26.);
#4960=CIRCLE('',#26363,0.5);
#4961=CIRCLE('',#26364,21.4999999999992);
#4962=CIRCLE('',#26365,0.5);
#4963=CIRCLE('',#26366,26.);
#4964=CIRCLE('',#26367,0.5);
#4965=CIRCLE('',#26368,21.4999999999992);
#4966=CIRCLE('',#26369,0.5);
#4967=CIRCLE('',#26370,26.);
#4968=CIRCLE('',#26371,0.5);
#4969=CIRCLE('',#26372,21.4999999999992);
#4970=CIRCLE('',#26373,0.5);
#4971=CIRCLE('',#26374,26.);
#4972=CIRCLE('',#26375,0.5);
#4973=CIRCLE('',#26376,21.4999999999992);
#4974=CIRCLE('',#26377,0.5);
#4975=CIRCLE('',#26378,26.);
#4976=CIRCLE('',#26379,0.5);
#4977=CIRCLE('',#26380,21.4999999999992);
#4978=CIRCLE('',#26381,0.5);
#4979=CIRCLE('',#26382,26.);
#4980=CIRCLE('',#26383,0.5);
#4981=CIRCLE('',#26384,21.4999999999992);
#4982=CIRCLE('',#26385,0.5);
#4983=CIRCLE('',#26386,26.);
#4984=CIRCLE('',#26387,0.5);
#4985=CIRCLE('',#26388,21.4999999999992);
#4986=CIRCLE('',#26389,0.5);
#4987=CIRCLE('',#26390,26.);
#4988=CIRCLE('',#26391,0.5);
#4989=CIRCLE('',#26392,21.4999999999992);
#4990=CIRCLE('',#26393,0.5);
#4991=CIRCLE('',#26394,26.);
#4992=CIRCLE('',#26395,0.5);
#4993=CIRCLE('',#26396,21.4999999999992);
#4994=CIRCLE('',#26397,0.5);
#4995=CIRCLE('',#26398,26.);
#4996=CIRCLE('',#26399,0.5);
#4997=CIRCLE('',#26400,21.4999999999992);
#4998=CIRCLE('',#26401,0.5);
#4999=CIRCLE('',#26402,26.);
#5000=CIRCLE('',#26403,0.5);
#5001=CIRCLE('',#26404,21.4999999999992);
#5002=CIRCLE('',#26405,0.5);
#5003=CIRCLE('',#26406,26.);
#5004=CIRCLE('',#26407,0.5);
#5005=CIRCLE('',#26408,21.4999999999992);
#5006=CIRCLE('',#26409,0.5);
#5007=CIRCLE('',#26410,26.);
#5008=CIRCLE('',#26411,0.5);
#5009=CIRCLE('',#26412,21.4999999999992);
#5010=CIRCLE('',#26413,0.5);
#5011=CIRCLE('',#26414,26.);
#5012=CIRCLE('',#26415,0.5);
#5013=CIRCLE('',#26416,21.4999999999992);
#5014=CIRCLE('',#26417,0.5);
#5015=CIRCLE('',#26419,0.5);
#5016=CIRCLE('',#26422,0.5);
#5017=CIRCLE('',#26424,21.4999999999992);
#5018=CIRCLE('',#26426,0.5);
#5019=CIRCLE('',#26429,0.5);
#5020=CIRCLE('',#26431,21.4999999999992);
#5021=CIRCLE('',#26433,0.5);
#5022=CIRCLE('',#26436,0.5);
#5023=CIRCLE('',#26438,21.4999999999992);
#5024=CIRCLE('',#26440,0.5);
#5025=CIRCLE('',#26443,0.5);
#5026=CIRCLE('',#26445,21.4999999999992);
#5027=CIRCLE('',#26447,0.5);
#5028=CIRCLE('',#26450,0.5);
#5029=CIRCLE('',#26452,21.4999999999992);
#5030=CIRCLE('',#26454,0.5);
#5031=CIRCLE('',#26457,0.5);
#5032=CIRCLE('',#26459,21.4999999999992);
#5033=CIRCLE('',#26461,0.5);
#5034=CIRCLE('',#26464,0.5);
#5035=CIRCLE('',#26466,21.4999999999992);
#5036=CIRCLE('',#26468,0.5);
#5037=CIRCLE('',#26471,0.5);
#5038=CIRCLE('',#26473,21.4999999999992);
#5039=CIRCLE('',#26475,0.5);
#5040=CIRCLE('',#26478,0.5);
#5041=CIRCLE('',#26480,21.4999999999992);
#5042=CIRCLE('',#26482,0.5);
#5043=CIRCLE('',#26485,0.5);
#5044=CIRCLE('',#26487,21.4999999999992);
#5045=CIRCLE('',#26489,0.5);
#5046=CIRCLE('',#26492,0.5);
#5047=CIRCLE('',#26494,21.4999999999992);
#5048=CIRCLE('',#26496,0.5);
#5049=CIRCLE('',#26499,0.5);
#5050=CIRCLE('',#26501,21.4999999999992);
#5051=CIRCLE('',#26503,0.5);
#5052=CIRCLE('',#26506,0.5);
#5053=CIRCLE('',#26508,21.4999999999992);
#5054=CIRCLE('',#26510,0.5);
#5055=CIRCLE('',#26513,0.5);
#5056=CIRCLE('',#26515,21.4999999999992);
#5057=CIRCLE('',#26517,0.5);
#5058=CIRCLE('',#26520,0.5);
#5059=CIRCLE('',#26522,21.4999999999992);
#5060=CIRCLE('',#26524,0.5);
#5061=CIRCLE('',#26527,0.5);
#5062=CIRCLE('',#26529,21.4999999999992);
#5063=CIRCLE('',#26531,0.5);
#5064=CIRCLE('',#26534,0.5);
#5065=CIRCLE('',#26536,21.4999999999992);
#5066=CIRCLE('',#26538,0.5);
#5067=CIRCLE('',#26541,0.5);
#5068=CIRCLE('',#26543,21.4999999999992);
#5069=CIRCLE('',#26545,0.5);
#5070=CIRCLE('',#26548,0.5);
#5071=CIRCLE('',#26550,21.4999999999992);
#5072=CIRCLE('',#26552,0.5);
#5073=CIRCLE('',#26555,0.5);
#5074=CIRCLE('',#26557,21.4999999999992);
#5075=CIRCLE('',#26559,0.5);
#5076=CIRCLE('',#26562,0.5);
#5077=CIRCLE('',#26564,21.4999999999992);
#5078=CIRCLE('',#26566,0.5);
#5079=CIRCLE('',#26569,0.5);
#5080=CIRCLE('',#26571,21.4999999999992);
#5081=CIRCLE('',#26573,0.5);
#5082=CIRCLE('',#26576,0.5);
#5083=CIRCLE('',#26578,21.4999999999992);
#5084=CIRCLE('',#26603,26.);
#5085=CIRCLE('',#26604,26.);
#5086=CIRCLE('',#26605,26.);
#5087=CIRCLE('',#26606,26.);
#5088=CIRCLE('',#26607,26.);
#5089=CIRCLE('',#26608,26.);
#5090=CIRCLE('',#26609,26.);
#5091=CIRCLE('',#26610,26.);
#5092=CIRCLE('',#26611,26.);
#5093=CIRCLE('',#26612,26.);
#5094=CIRCLE('',#26613,26.);
#5095=CIRCLE('',#26614,26.);
#5096=CIRCLE('',#26615,26.);
#5097=CIRCLE('',#26616,26.);
#5098=CIRCLE('',#26617,26.);
#5099=CIRCLE('',#26618,26.);
#5100=CIRCLE('',#26619,26.);
#5101=CIRCLE('',#26620,26.);
#5102=CIRCLE('',#26621,26.);
#5103=CIRCLE('',#26622,26.);
#5104=CIRCLE('',#26623,26.);
#5105=CIRCLE('',#26624,26.);
#5106=CIRCLE('',#26625,26.);
#5107=CIRCLE('',#26626,0.5);
#5108=CIRCLE('',#26627,21.4999999999992);
#5109=CIRCLE('',#26628,0.5);
#5110=CIRCLE('',#26629,26.);
#7130=LINE('',#174989,#8315);
#7131=LINE('',#174991,#8316);
#7132=LINE('',#174993,#8317);
#7133=LINE('',#174994,#8318);
#7134=LINE('',#174998,#8319);
#7135=LINE('',#175000,#8320);
#7136=LINE('',#175002,#8321);
#7137=LINE('',#175003,#8322);
#7138=LINE('',#175005,#8323);
#7139=LINE('',#175006,#8324);
#7140=LINE('',#175427,#8325);
#7141=LINE('',#175435,#8326);
#7142=LINE('',#175851,#8327);
#7143=LINE('',#175859,#8328);
#7144=LINE('',#176275,#8329);
#7145=LINE('',#176283,#8330);
#7146=LINE('',#176699,#8331);
#7147=LINE('',#176707,#8332);
#7148=LINE('',#177123,#8333);
#7149=LINE('',#177131,#8334);
#7150=LINE('',#177547,#8335);
#7151=LINE('',#177555,#8336);
#7152=LINE('',#177971,#8337);
#7153=LINE('',#177979,#8338);
#7154=LINE('',#178395,#8339);
#7155=LINE('',#178403,#8340);
#7156=LINE('',#178819,#8341);
#7157=LINE('',#178827,#8342);
#7158=LINE('',#179243,#8343);
#7159=LINE('',#179251,#8344);
#7160=LINE('',#179667,#8345);
#7161=LINE('',#179675,#8346);
#7162=LINE('',#180091,#8347);
#7163=LINE('',#180099,#8348);
#7164=LINE('',#180515,#8349);
#7165=LINE('',#180523,#8350);
#7166=LINE('',#180939,#8351);
#7167=LINE('',#180947,#8352);
#7168=LINE('',#181363,#8353);
#7169=LINE('',#181371,#8354);
#7170=LINE('',#181787,#8355);
#7171=LINE('',#181795,#8356);
#7172=LINE('',#182211,#8357);
#7173=LINE('',#182219,#8358);
#7174=LINE('',#182635,#8359);
#7175=LINE('',#182643,#8360);
#7176=LINE('',#183059,#8361);
#7177=LINE('',#183067,#8362);
#7178=LINE('',#183483,#8363);
#7179=LINE('',#183491,#8364);
#7180=LINE('',#183907,#8365);
#7181=LINE('',#183915,#8366);
#7182=LINE('',#184331,#8367);
#7183=LINE('',#184339,#8368);
#7184=LINE('',#184755,#8369);
#7185=LINE('',#184763,#8370);
#7186=LINE('',#185179,#8371);
#7187=LINE('',#185186,#8372);
#7188=LINE('',#185191,#8373);
#7189=LINE('',#185192,#8374);
#7190=LINE('',#185195,#8375);
#7191=LINE('',#185196,#8376);
#7192=LINE('',#185201,#8377);
#7193=LINE('',#185202,#8378);
#7194=LINE('',#185209,#8379);
#7195=LINE('',#185210,#8380);
#7196=LINE('',#185213,#8381);
#7197=LINE('',#185214,#8382);
#7198=LINE('',#185219,#8383);
#7199=LINE('',#185220,#8384);
#7200=LINE('',#185227,#8385);
#7201=LINE('',#185228,#8386);
#7202=LINE('',#185231,#8387);
#7203=LINE('',#185232,#8388);
#7204=LINE('',#185237,#8389);
#7205=LINE('',#185238,#8390);
#7206=LINE('',#185245,#8391);
#7207=LINE('',#185246,#8392);
#7208=LINE('',#185249,#8393);
#7209=LINE('',#185250,#8394);
#7210=LINE('',#185255,#8395);
#7211=LINE('',#185256,#8396);
#7212=LINE('',#185263,#8397);
#7213=LINE('',#185264,#8398);
#7214=LINE('',#185267,#8399);
#7215=LINE('',#185268,#8400);
#7216=LINE('',#185273,#8401);
#7217=LINE('',#185274,#8402);
#7218=LINE('',#185281,#8403);
#7219=LINE('',#185282,#8404);
#7220=LINE('',#185285,#8405);
#7221=LINE('',#185286,#8406);
#7222=LINE('',#185291,#8407);
#7223=LINE('',#185292,#8408);
#7224=LINE('',#185299,#8409);
#7225=LINE('',#185300,#8410);
#7226=LINE('',#185303,#8411);
#7227=LINE('',#185304,#8412);
#7228=LINE('',#185309,#8413);
#7229=LINE('',#185310,#8414);
#7230=LINE('',#185317,#8415);
#7231=LINE('',#185318,#8416);
#7232=LINE('',#185321,#8417);
#7233=LINE('',#185322,#8418);
#7234=LINE('',#185327,#8419);
#7235=LINE('',#185328,#8420);
#7236=LINE('',#185335,#8421);
#7237=LINE('',#185336,#8422);
#7238=LINE('',#185339,#8423);
#7239=LINE('',#185340,#8424);
#7240=LINE('',#185345,#8425);
#7241=LINE('',#185346,#8426);
#7242=LINE('',#185353,#8427);
#7243=LINE('',#185354,#8428);
#7244=LINE('',#185357,#8429);
#7245=LINE('',#185358,#8430);
#7246=LINE('',#185363,#8431);
#7247=LINE('',#185364,#8432);
#7248=LINE('',#185371,#8433);
#7249=LINE('',#185372,#8434);
#7250=LINE('',#185375,#8435);
#7251=LINE('',#185376,#8436);
#7252=LINE('',#185381,#8437);
#7253=LINE('',#185382,#8438);
#7254=LINE('',#185389,#8439);
#7255=LINE('',#185390,#8440);
#7256=LINE('',#185393,#8441);
#7257=LINE('',#185394,#8442);
#7258=LINE('',#185399,#8443);
#7259=LINE('',#185400,#8444);
#7260=LINE('',#185407,#8445);
#7261=LINE('',#185408,#8446);
#7262=LINE('',#185411,#8447);
#7263=LINE('',#185412,#8448);
#7264=LINE('',#185417,#8449);
#7265=LINE('',#185418,#8450);
#7266=LINE('',#185425,#8451);
#7267=LINE('',#185426,#8452);
#7268=LINE('',#185429,#8453);
#7269=LINE('',#185430,#8454);
#7270=LINE('',#185435,#8455);
#7271=LINE('',#185436,#8456);
#7272=LINE('',#185443,#8457);
#7273=LINE('',#185444,#8458);
#7274=LINE('',#185447,#8459);
#7275=LINE('',#185448,#8460);
#7276=LINE('',#185453,#8461);
#7277=LINE('',#185454,#8462);
#7278=LINE('',#185461,#8463);
#7279=LINE('',#185462,#8464);
#7280=LINE('',#185465,#8465);
#7281=LINE('',#185466,#8466);
#7282=LINE('',#185471,#8467);
#7283=LINE('',#185472,#8468);
#7284=LINE('',#185479,#8469);
#7285=LINE('',#185480,#8470);
#7286=LINE('',#185483,#8471);
#7287=LINE('',#185484,#8472);
#7288=LINE('',#185489,#8473);
#7289=LINE('',#185490,#8474);
#7290=LINE('',#185497,#8475);
#7291=LINE('',#185498,#8476);
#7292=LINE('',#185501,#8477);
#7293=LINE('',#185502,#8478);
#7294=LINE('',#185507,#8479);
#7295=LINE('',#185508,#8480);
#7296=LINE('',#185515,#8481);
#7297=LINE('',#185516,#8482);
#7298=LINE('',#185519,#8483);
#7299=LINE('',#185520,#8484);
#7300=LINE('',#185525,#8485);
#7301=LINE('',#185526,#8486);
#7302=LINE('',#185533,#8487);
#7303=LINE('',#185534,#8488);
#7304=LINE('',#185537,#8489);
#7305=LINE('',#185538,#8490);
#7306=LINE('',#185543,#8491);
#7307=LINE('',#185544,#8492);
#7308=LINE('',#185551,#8493);
#7309=LINE('',#185552,#8494);
#7310=LINE('',#185555,#8495);
#7311=LINE('',#185556,#8496);
#7312=LINE('',#185561,#8497);
#7313=LINE('',#185562,#8498);
#7314=LINE('',#185569,#8499);
#7315=LINE('',#185570,#8500);
#7316=LINE('',#185573,#8501);
#7317=LINE('',#185574,#8502);
#7318=LINE('',#185579,#8503);
#7319=LINE('',#185580,#8504);
#7320=LINE('',#185587,#8505);
#7321=LINE('',#185588,#8506);
#7322=LINE('',#185591,#8507);
#7323=LINE('',#185592,#8508);
#7324=LINE('',#185597,#8509);
#7325=LINE('',#185598,#8510);
#7326=LINE('',#185603,#8511);
#7327=LINE('',#185604,#8512);
#7328=LINE('',#186221,#8513);
#7329=LINE('',#186838,#8514);
#7330=LINE('',#186841,#8515);
#7331=LINE('',#186842,#8516);
#7332=LINE('',#187459,#8517);
#7333=LINE('',#188076,#8518);
#7334=LINE('',#188079,#8519);
#7335=LINE('',#188080,#8520);
#7336=LINE('',#188697,#8521);
#7337=LINE('',#189314,#8522);
#7338=LINE('',#189317,#8523);
#7339=LINE('',#189318,#8524);
#7340=LINE('',#189935,#8525);
#7341=LINE('',#190552,#8526);
#7342=LINE('',#190555,#8527);
#7343=LINE('',#190556,#8528);
#7344=LINE('',#191173,#8529);
#7345=LINE('',#191790,#8530);
#7346=LINE('',#191793,#8531);
#7347=LINE('',#191794,#8532);
#7348=LINE('',#192411,#8533);
#7349=LINE('',#193028,#8534);
#7350=LINE('',#193031,#8535);
#7351=LINE('',#193032,#8536);
#7352=LINE('',#193649,#8537);
#7353=LINE('',#194266,#8538);
#7354=LINE('',#194269,#8539);
#7355=LINE('',#194270,#8540);
#7356=LINE('',#194887,#8541);
#7357=LINE('',#195504,#8542);
#7358=LINE('',#195507,#8543);
#7359=LINE('',#195508,#8544);
#7360=LINE('',#196125,#8545);
#7361=LINE('',#196742,#8546);
#7362=LINE('',#196745,#8547);
#7363=LINE('',#196746,#8548);
#7364=LINE('',#197363,#8549);
#7365=LINE('',#197980,#8550);
#7366=LINE('',#197983,#8551);
#7367=LINE('',#197984,#8552);
#7368=LINE('',#198601,#8553);
#7369=LINE('',#199218,#8554);
#7370=LINE('',#199221,#8555);
#7371=LINE('',#199222,#8556);
#7372=LINE('',#199839,#8557);
#7373=LINE('',#200456,#8558);
#7374=LINE('',#200459,#8559);
#7375=LINE('',#200460,#8560);
#7376=LINE('',#201077,#8561);
#7377=LINE('',#201694,#8562);
#7378=LINE('',#201697,#8563);
#7379=LINE('',#201698,#8564);
#7380=LINE('',#202315,#8565);
#7381=LINE('',#202932,#8566);
#7382=LINE('',#202935,#8567);
#7383=LINE('',#202936,#8568);
#7384=LINE('',#203553,#8569);
#7385=LINE('',#204170,#8570);
#7386=LINE('',#204173,#8571);
#7387=LINE('',#204174,#8572);
#7388=LINE('',#204791,#8573);
#7389=LINE('',#205408,#8574);
#7390=LINE('',#205411,#8575);
#7391=LINE('',#205412,#8576);
#7392=LINE('',#206029,#8577);
#7393=LINE('',#206646,#8578);
#7394=LINE('',#206649,#8579);
#7395=LINE('',#206650,#8580);
#7396=LINE('',#207267,#8581);
#7397=LINE('',#207884,#8582);
#7398=LINE('',#207887,#8583);
#7399=LINE('',#207888,#8584);
#7400=LINE('',#208505,#8585);
#7401=LINE('',#209122,#8586);
#7402=LINE('',#209125,#8587);
#7403=LINE('',#209126,#8588);
#7404=LINE('',#209743,#8589);
#7405=LINE('',#210360,#8590);
#7406=LINE('',#210363,#8591);
#7407=LINE('',#210364,#8592);
#7408=LINE('',#210981,#8593);
#7409=LINE('',#211598,#8594);
#7410=LINE('',#211601,#8595);
#7411=LINE('',#211602,#8596);
#7412=LINE('',#212219,#8597);
#7413=LINE('',#212836,#8598);
#7414=LINE('',#212839,#8599);
#7415=LINE('',#212840,#8600);
#7416=LINE('',#213457,#8601);
#7417=LINE('',#214074,#8602);
#7418=LINE('',#214307,#8603);
#7419=LINE('',#214315,#8604);
#7420=LINE('',#214524,#8605);
#7421=LINE('',#214548,#8606);
#7422=LINE('',#214549,#8607);
#7423=LINE('',#214551,#8608);
#7424=LINE('',#214553,#8609);
#7425=LINE('',#214554,#8610);
#7426=LINE('',#214557,#8611);
#7427=LINE('',#215378,#8612);
#8315=VECTOR('',#29647,10.);
#8316=VECTOR('',#29648,10.);
#8317=VECTOR('',#29649,10.);
#8318=VECTOR('',#29650,10.);
#8319=VECTOR('',#29653,10.);
#8320=VECTOR('',#29654,10.);
#8321=VECTOR('',#29655,10.);
#8322=VECTOR('',#29656,10.);
#8323=VECTOR('',#29659,10.);
#8324=VECTOR('',#29660,10.);
#8325=VECTOR('',#29671,10.);
#8326=VECTOR('',#29678,10.);
#8327=VECTOR('',#29681,10.);
#8328=VECTOR('',#29688,10.);
#8329=VECTOR('',#29691,10.);
#8330=VECTOR('',#29698,10.);
#8331=VECTOR('',#29701,10.);
#8332=VECTOR('',#29708,10.);
#8333=VECTOR('',#29711,10.);
#8334=VECTOR('',#29718,10.);
#8335=VECTOR('',#29721,10.);
#8336=VECTOR('',#29728,10.);
#8337=VECTOR('',#29731,10.);
#8338=VECTOR('',#29738,10.);
#8339=VECTOR('',#29741,10.);
#8340=VECTOR('',#29748,10.);
#8341=VECTOR('',#29751,10.);
#8342=VECTOR('',#29758,10.);
#8343=VECTOR('',#29761,10.);
#8344=VECTOR('',#29768,10.);
#8345=VECTOR('',#29771,10.);
#8346=VECTOR('',#29778,10.);
#8347=VECTOR('',#29781,10.);
#8348=VECTOR('',#29788,10.);
#8349=VECTOR('',#29791,10.);
#8350=VECTOR('',#29798,10.);
#8351=VECTOR('',#29801,10.);
#8352=VECTOR('',#29808,10.);
#8353=VECTOR('',#29811,10.);
#8354=VECTOR('',#29818,10.);
#8355=VECTOR('',#29821,10.);
#8356=VECTOR('',#29828,10.);
#8357=VECTOR('',#29831,10.);
#8358=VECTOR('',#29838,10.);
#8359=VECTOR('',#29841,10.);
#8360=VECTOR('',#29848,10.);
#8361=VECTOR('',#29851,10.);
#8362=VECTOR('',#29858,10.);
#8363=VECTOR('',#29861,10.);
#8364=VECTOR('',#29868,10.);
#8365=VECTOR('',#29871,10.);
#8366=VECTOR('',#29878,10.);
#8367=VECTOR('',#29881,10.);
#8368=VECTOR('',#29888,10.);
#8369=VECTOR('',#29891,10.);
#8370=VECTOR('',#29898,10.);
#8371=VECTOR('',#29901,10.);
#8372=VECTOR('',#29908,10.);
#8373=VECTOR('',#29913,10.);
#8374=VECTOR('',#29914,10.);
#8375=VECTOR('',#29917,10.);
#8376=VECTOR('',#29918,10.);
#8377=VECTOR('',#29923,10.);
#8378=VECTOR('',#29924,10.);
#8379=VECTOR('',#29933,10.);
#8380=VECTOR('',#29934,10.);
#8381=VECTOR('',#29937,10.);
#8382=VECTOR('',#29938,10.);
#8383=VECTOR('',#29943,10.);
#8384=VECTOR('',#29944,10.);
#8385=VECTOR('',#29953,10.);
#8386=VECTOR('',#29954,10.);
#8387=VECTOR('',#29957,10.);
#8388=VECTOR('',#29958,10.);
#8389=VECTOR('',#29963,10.);
#8390=VECTOR('',#29964,10.);
#8391=VECTOR('',#29973,10.);
#8392=VECTOR('',#29974,10.);
#8393=VECTOR('',#29977,10.);
#8394=VECTOR('',#29978,10.);
#8395=VECTOR('',#29983,10.);
#8396=VECTOR('',#29984,10.);
#8397=VECTOR('',#29993,10.);
#8398=VECTOR('',#29994,10.);
#8399=VECTOR('',#29997,10.);
#8400=VECTOR('',#29998,10.);
#8401=VECTOR('',#30003,10.);
#8402=VECTOR('',#30004,10.);
#8403=VECTOR('',#30013,10.);
#8404=VECTOR('',#30014,10.);
#8405=VECTOR('',#30017,10.);
#8406=VECTOR('',#30018,10.);
#8407=VECTOR('',#30023,10.);
#8408=VECTOR('',#30024,10.);
#8409=VECTOR('',#30033,10.);
#8410=VECTOR('',#30034,10.);
#8411=VECTOR('',#30037,10.);
#8412=VECTOR('',#30038,10.);
#8413=VECTOR('',#30043,10.);
#8414=VECTOR('',#30044,10.);
#8415=VECTOR('',#30053,10.);
#8416=VECTOR('',#30054,10.);
#8417=VECTOR('',#30057,10.);
#8418=VECTOR('',#30058,10.);
#8419=VECTOR('',#30063,10.);
#8420=VECTOR('',#30064,10.);
#8421=VECTOR('',#30073,10.);
#8422=VECTOR('',#30074,10.);
#8423=VECTOR('',#30077,10.);
#8424=VECTOR('',#30078,10.);
#8425=VECTOR('',#30083,10.);
#8426=VECTOR('',#30084,10.);
#8427=VECTOR('',#30093,10.);
#8428=VECTOR('',#30094,10.);
#8429=VECTOR('',#30097,10.);
#8430=VECTOR('',#30098,10.);
#8431=VECTOR('',#30103,10.);
#8432=VECTOR('',#30104,10.);
#8433=VECTOR('',#30113,10.);
#8434=VECTOR('',#30114,10.);
#8435=VECTOR('',#30117,10.);
#8436=VECTOR('',#30118,10.);
#8437=VECTOR('',#30123,10.);
#8438=VECTOR('',#30124,10.);
#8439=VECTOR('',#30133,10.);
#8440=VECTOR('',#30134,10.);
#8441=VECTOR('',#30137,10.);
#8442=VECTOR('',#30138,10.);
#8443=VECTOR('',#30143,10.);
#8444=VECTOR('',#30144,10.);
#8445=VECTOR('',#30153,10.);
#8446=VECTOR('',#30154,10.);
#8447=VECTOR('',#30157,10.);
#8448=VECTOR('',#30158,10.);
#8449=VECTOR('',#30163,10.);
#8450=VECTOR('',#30164,10.);
#8451=VECTOR('',#30173,10.);
#8452=VECTOR('',#30174,10.);
#8453=VECTOR('',#30177,10.);
#8454=VECTOR('',#30178,10.);
#8455=VECTOR('',#30183,10.);
#8456=VECTOR('',#30184,10.);
#8457=VECTOR('',#30193,10.);
#8458=VECTOR('',#30194,10.);
#8459=VECTOR('',#30197,10.);
#8460=VECTOR('',#30198,10.);
#8461=VECTOR('',#30203,10.);
#8462=VECTOR('',#30204,10.);
#8463=VECTOR('',#30213,10.);
#8464=VECTOR('',#30214,10.);
#8465=VECTOR('',#30217,10.);
#8466=VECTOR('',#30218,10.);
#8467=VECTOR('',#30223,10.);
#8468=VECTOR('',#30224,10.);
#8469=VECTOR('',#30233,10.);
#8470=VECTOR('',#30234,10.);
#8471=VECTOR('',#30237,10.);
#8472=VECTOR('',#30238,10.);
#8473=VECTOR('',#30243,10.);
#8474=VECTOR('',#30244,10.);
#8475=VECTOR('',#30253,10.);
#8476=VECTOR('',#30254,10.);
#8477=VECTOR('',#30257,10.);
#8478=VECTOR('',#30258,10.);
#8479=VECTOR('',#30263,10.);
#8480=VECTOR('',#30264,10.);
#8481=VECTOR('',#30273,10.);
#8482=VECTOR('',#30274,10.);
#8483=VECTOR('',#30277,10.);
#8484=VECTOR('',#30278,10.);
#8485=VECTOR('',#30283,10.);
#8486=VECTOR('',#30284,10.);
#8487=VECTOR('',#30293,10.);
#8488=VECTOR('',#30294,10.);
#8489=VECTOR('',#30297,10.);
#8490=VECTOR('',#30298,10.);
#8491=VECTOR('',#30303,10.);
#8492=VECTOR('',#30304,10.);
#8493=VECTOR('',#30313,10.);
#8494=VECTOR('',#30314,10.);
#8495=VECTOR('',#30317,10.);
#8496=VECTOR('',#30318,10.);
#8497=VECTOR('',#30323,10.);
#8498=VECTOR('',#30324,10.);
#8499=VECTOR('',#30333,10.);
#8500=VECTOR('',#30334,10.);
#8501=VECTOR('',#30337,10.);
#8502=VECTOR('',#30338,10.);
#8503=VECTOR('',#30343,10.);
#8504=VECTOR('',#30344,10.);
#8505=VECTOR('',#30353,10.);
#8506=VECTOR('',#30354,10.);
#8507=VECTOR('',#30357,10.);
#8508=VECTOR('',#30358,10.);
#8509=VECTOR('',#30363,10.);
#8510=VECTOR('',#30364,10.);
#8511=VECTOR('',#30371,10.);
#8512=VECTOR('',#30372,10.);
#8513=VECTOR('',#30373,10.);
#8514=VECTOR('',#30374,10.);
#8515=VECTOR('',#30377,10.);
#8516=VECTOR('',#30378,10.);
#8517=VECTOR('',#30379,10.);
#8518=VECTOR('',#30380,10.);
#8519=VECTOR('',#30383,10.);
#8520=VECTOR('',#30384,10.);
#8521=VECTOR('',#30385,10.);
#8522=VECTOR('',#30386,10.);
#8523=VECTOR('',#30389,10.);
#8524=VECTOR('',#30390,10.);
#8525=VECTOR('',#30391,10.);
#8526=VECTOR('',#30392,10.);
#8527=VECTOR('',#30395,10.);
#8528=VECTOR('',#30396,10.);
#8529=VECTOR('',#30397,10.);
#8530=VECTOR('',#30398,10.);
#8531=VECTOR('',#30401,10.);
#8532=VECTOR('',#30402,10.);
#8533=VECTOR('',#30403,10.);
#8534=VECTOR('',#30404,10.);
#8535=VECTOR('',#30407,10.);
#8536=VECTOR('',#30408,10.);
#8537=VECTOR('',#30409,10.);
#8538=VECTOR('',#30410,10.);
#8539=VECTOR('',#30413,10.);
#8540=VECTOR('',#30414,10.);
#8541=VECTOR('',#30415,10.);
#8542=VECTOR('',#30416,10.);
#8543=VECTOR('',#30419,10.);
#8544=VECTOR('',#30420,10.);
#8545=VECTOR('',#30421,10.);
#8546=VECTOR('',#30422,10.);
#8547=VECTOR('',#30425,10.);
#8548=VECTOR('',#30426,10.);
#8549=VECTOR('',#30427,10.);
#8550=VECTOR('',#30428,10.);
#8551=VECTOR('',#30431,10.);
#8552=VECTOR('',#30432,10.);
#8553=VECTOR('',#30433,10.);
#8554=VECTOR('',#30434,10.);
#8555=VECTOR('',#30437,10.);
#8556=VECTOR('',#30438,10.);
#8557=VECTOR('',#30439,10.);
#8558=VECTOR('',#30440,10.);
#8559=VECTOR('',#30443,10.);
#8560=VECTOR('',#30444,10.);
#8561=VECTOR('',#30445,10.);
#8562=VECTOR('',#30446,10.);
#8563=VECTOR('',#30449,10.);
#8564=VECTOR('',#30450,10.);
#8565=VECTOR('',#30451,10.);
#8566=VECTOR('',#30452,10.);
#8567=VECTOR('',#30455,10.);
#8568=VECTOR('',#30456,10.);
#8569=VECTOR('',#30457,10.);
#8570=VECTOR('',#30458,10.);
#8571=VECTOR('',#30461,10.);
#8572=VECTOR('',#30462,10.);
#8573=VECTOR('',#30463,10.);
#8574=VECTOR('',#30464,10.);
#8575=VECTOR('',#30467,10.);
#8576=VECTOR('',#30468,10.);
#8577=VECTOR('',#30469,10.);
#8578=VECTOR('',#30470,10.);
#8579=VECTOR('',#30473,10.);
#8580=VECTOR('',#30474,10.);
#8581=VECTOR('',#30475,10.);
#8582=VECTOR('',#30476,10.);
#8583=VECTOR('',#30479,10.);
#8584=VECTOR('',#30480,10.);
#8585=VECTOR('',#30481,10.);
#8586=VECTOR('',#30482,10.);
#8587=VECTOR('',#30485,10.);
#8588=VECTOR('',#30486,10.);
#8589=VECTOR('',#30487,10.);
#8590=VECTOR('',#30488,10.);
#8591=VECTOR('',#30491,10.);
#8592=VECTOR('',#30492,10.);
#8593=VECTOR('',#30493,10.);
#8594=VECTOR('',#30494,10.);
#8595=VECTOR('',#30497,10.);
#8596=VECTOR('',#30498,10.);
#8597=VECTOR('',#30499,10.);
#8598=VECTOR('',#30500,10.);
#8599=VECTOR('',#30503,10.);
#8600=VECTOR('',#30504,10.);
#8601=VECTOR('',#30505,10.);
#8602=VECTOR('',#30506,10.);
#8603=VECTOR('',#30555,10.);
#8604=VECTOR('',#30562,10.);
#8605=VECTOR('',#30567,10.);
#8606=VECTOR('',#30614,10.);
#8607=VECTOR('',#30615,10.);
#8608=VECTOR('',#30618,10.);
#8609=VECTOR('',#30621,10.);
#8610=VECTOR('',#30622,10.);
#8611=VECTOR('',#30627,10.);
#8612=VECTOR('',#30628,10.);
#10617=VERTEX_POINT('',#174987);
#10618=VERTEX_POINT('',#174988);
#10619=VERTEX_POINT('',#174990);
#10620=VERTEX_POINT('',#174992);
#10621=VERTEX_POINT('',#174996);
#10622=VERTEX_POINT('',#174997);
#10623=VERTEX_POINT('',#174999);
#10624=VERTEX_POINT('',#175001);
#10625=VERTEX_POINT('',#175011);
#10626=VERTEX_POINT('',#175012);
#10627=VERTEX_POINT('',#175218);
#10628=VERTEX_POINT('',#175220);
#10629=VERTEX_POINT('',#175426);
#10630=VERTEX_POINT('',#175428);
#10631=VERTEX_POINT('',#175430);
#10632=VERTEX_POINT('',#175432);
#10633=VERTEX_POINT('',#175434);
#10634=VERTEX_POINT('',#175436);
#10635=VERTEX_POINT('',#175642);
#10636=VERTEX_POINT('',#175644);
#10637=VERTEX_POINT('',#175850);
#10638=VERTEX_POINT('',#175852);
#10639=VERTEX_POINT('',#175854);
#10640=VERTEX_POINT('',#175856);
#10641=VERTEX_POINT('',#175858);
#10642=VERTEX_POINT('',#175860);
#10643=VERTEX_POINT('',#176066);
#10644=VERTEX_POINT('',#176068);
#10645=VERTEX_POINT('',#176274);
#10646=VERTEX_POINT('',#176276);
#10647=VERTEX_POINT('',#176278);
#10648=VERTEX_POINT('',#176280);
#10649=VERTEX_POINT('',#176282);
#10650=VERTEX_POINT('',#176284);
#10651=VERTEX_POINT('',#176490);
#10652=VERTEX_POINT('',#176492);
#10653=VERTEX_POINT('',#176698);
#10654=VERTEX_POINT('',#176700);
#10655=VERTEX_POINT('',#176702);
#10656=VERTEX_POINT('',#176704);
#10657=VERTEX_POINT('',#176706);
#10658=VERTEX_POINT('',#176708);
#10659=VERTEX_POINT('',#176914);
#10660=VERTEX_POINT('',#176916);
#10661=VERTEX_POINT('',#177122);
#10662=VERTEX_POINT('',#177124);
#10663=VERTEX_POINT('',#177126);
#10664=VERTEX_POINT('',#177128);
#10665=VERTEX_POINT('',#177130);
#10666=VERTEX_POINT('',#177132);
#10667=VERTEX_POINT('',#177338);
#10668=VERTEX_POINT('',#177340);
#10669=VERTEX_POINT('',#177546);
#10670=VERTEX_POINT('',#177548);
#10671=VERTEX_POINT('',#177550);
#10672=VERTEX_POINT('',#177552);
#10673=VERTEX_POINT('',#177554);
#10674=VERTEX_POINT('',#177556);
#10675=VERTEX_POINT('',#177762);
#10676=VERTEX_POINT('',#177764);
#10677=VERTEX_POINT('',#177970);
#10678=VERTEX_POINT('',#177972);
#10679=VERTEX_POINT('',#177974);
#10680=VERTEX_POINT('',#177976);
#10681=VERTEX_POINT('',#177978);
#10682=VERTEX_POINT('',#177980);
#10683=VERTEX_POINT('',#178186);
#10684=VERTEX_POINT('',#178188);
#10685=VERTEX_POINT('',#178394);
#10686=VERTEX_POINT('',#178396);
#10687=VERTEX_POINT('',#178398);
#10688=VERTEX_POINT('',#178400);
#10689=VERTEX_POINT('',#178402);
#10690=VERTEX_POINT('',#178404);
#10691=VERTEX_POINT('',#178610);
#10692=VERTEX_POINT('',#178612);
#10693=VERTEX_POINT('',#178818);
#10694=VERTEX_POINT('',#178820);
#10695=VERTEX_POINT('',#178822);
#10696=VERTEX_POINT('',#178824);
#10697=VERTEX_POINT('',#178826);
#10698=VERTEX_POINT('',#178828);
#10699=VERTEX_POINT('',#179034);
#10700=VERTEX_POINT('',#179036);
#10701=VERTEX_POINT('',#179242);
#10702=VERTEX_POINT('',#179244);
#10703=VERTEX_POINT('',#179246);
#10704=VERTEX_POINT('',#179248);
#10705=VERTEX_POINT('',#179250);
#10706=VERTEX_POINT('',#179252);
#10707=VERTEX_POINT('',#179458);
#10708=VERTEX_POINT('',#179460);
#10709=VERTEX_POINT('',#179666);
#10710=VERTEX_POINT('',#179668);
#10711=VERTEX_POINT('',#179670);
#10712=VERTEX_POINT('',#179672);
#10713=VERTEX_POINT('',#179674);
#10714=VERTEX_POINT('',#179676);
#10715=VERTEX_POINT('',#179882);
#10716=VERTEX_POINT('',#179884);
#10717=VERTEX_POINT('',#180090);
#10718=VERTEX_POINT('',#180092);
#10719=VERTEX_POINT('',#180094);
#10720=VERTEX_POINT('',#180096);
#10721=VERTEX_POINT('',#180098);
#10722=VERTEX_POINT('',#180100);
#10723=VERTEX_POINT('',#180306);
#10724=VERTEX_POINT('',#180308);
#10725=VERTEX_POINT('',#180514);
#10726=VERTEX_POINT('',#180516);
#10727=VERTEX_POINT('',#180518);
#10728=VERTEX_POINT('',#180520);
#10729=VERTEX_POINT('',#180522);
#10730=VERTEX_POINT('',#180524);
#10731=VERTEX_POINT('',#180730);
#10732=VERTEX_POINT('',#180732);
#10733=VERTEX_POINT('',#180938);
#10734=VERTEX_POINT('',#180940);
#10735=VERTEX_POINT('',#180942);
#10736=VERTEX_POINT('',#180944);
#10737=VERTEX_POINT('',#180946);
#10738=VERTEX_POINT('',#180948);
#10739=VERTEX_POINT('',#181154);
#10740=VERTEX_POINT('',#181156);
#10741=VERTEX_POINT('',#181362);
#10742=VERTEX_POINT('',#181364);
#10743=VERTEX_POINT('',#181366);
#10744=VERTEX_POINT('',#181368);
#10745=VERTEX_POINT('',#181370);
#10746=VERTEX_POINT('',#181372);
#10747=VERTEX_POINT('',#181578);
#10748=VERTEX_POINT('',#181580);
#10749=VERTEX_POINT('',#181786);
#10750=VERTEX_POINT('',#181788);
#10751=VERTEX_POINT('',#181790);
#10752=VERTEX_POINT('',#181792);
#10753=VERTEX_POINT('',#181794);
#10754=VERTEX_POINT('',#181796);
#10755=VERTEX_POINT('',#182002);
#10756=VERTEX_POINT('',#182004);
#10757=VERTEX_POINT('',#182210);
#10758=VERTEX_POINT('',#182212);
#10759=VERTEX_POINT('',#182214);
#10760=VERTEX_POINT('',#182216);
#10761=VERTEX_POINT('',#182218);
#10762=VERTEX_POINT('',#182220);
#10763=VERTEX_POINT('',#182426);
#10764=VERTEX_POINT('',#182428);
#10765=VERTEX_POINT('',#182634);
#10766=VERTEX_POINT('',#182636);
#10767=VERTEX_POINT('',#182638);
#10768=VERTEX_POINT('',#182640);
#10769=VERTEX_POINT('',#182642);
#10770=VERTEX_POINT('',#182644);
#10771=VERTEX_POINT('',#182850);
#10772=VERTEX_POINT('',#182852);
#10773=VERTEX_POINT('',#183058);
#10774=VERTEX_POINT('',#183060);
#10775=VERTEX_POINT('',#183062);
#10776=VERTEX_POINT('',#183064);
#10777=VERTEX_POINT('',#183066);
#10778=VERTEX_POINT('',#183068);
#10779=VERTEX_POINT('',#183274);
#10780=VERTEX_POINT('',#183276);
#10781=VERTEX_POINT('',#183482);
#10782=VERTEX_POINT('',#183484);
#10783=VERTEX_POINT('',#183486);
#10784=VERTEX_POINT('',#183488);
#10785=VERTEX_POINT('',#183490);
#10786=VERTEX_POINT('',#183492);
#10787=VERTEX_POINT('',#183698);
#10788=VERTEX_POINT('',#183700);
#10789=VERTEX_POINT('',#183906);
#10790=VERTEX_POINT('',#183908);
#10791=VERTEX_POINT('',#183910);
#10792=VERTEX_POINT('',#183912);
#10793=VERTEX_POINT('',#183914);
#10794=VERTEX_POINT('',#183916);
#10795=VERTEX_POINT('',#184122);
#10796=VERTEX_POINT('',#184124);
#10797=VERTEX_POINT('',#184330);
#10798=VERTEX_POINT('',#184332);
#10799=VERTEX_POINT('',#184334);
#10800=VERTEX_POINT('',#184336);
#10801=VERTEX_POINT('',#184338);
#10802=VERTEX_POINT('',#184340);
#10803=VERTEX_POINT('',#184546);
#10804=VERTEX_POINT('',#184548);
#10805=VERTEX_POINT('',#184754);
#10806=VERTEX_POINT('',#184756);
#10807=VERTEX_POINT('',#184758);
#10808=VERTEX_POINT('',#184760);
#10809=VERTEX_POINT('',#184762);
#10810=VERTEX_POINT('',#184764);
#10811=VERTEX_POINT('',#184970);
#10812=VERTEX_POINT('',#184972);
#10813=VERTEX_POINT('',#185178);
#10814=VERTEX_POINT('',#185180);
#10815=VERTEX_POINT('',#185182);
#10816=VERTEX_POINT('',#185184);
#10817=VERTEX_POINT('',#185188);
#10818=VERTEX_POINT('',#185189);
#10819=VERTEX_POINT('',#185194);
#10820=VERTEX_POINT('',#185198);
#10821=VERTEX_POINT('',#185199);
#10822=VERTEX_POINT('',#185206);
#10823=VERTEX_POINT('',#185207);
#10824=VERTEX_POINT('',#185212);
#10825=VERTEX_POINT('',#185216);
#10826=VERTEX_POINT('',#185217);
#10827=VERTEX_POINT('',#185224);
#10828=VERTEX_POINT('',#185225);
#10829=VERTEX_POINT('',#185230);
#10830=VERTEX_POINT('',#185234);
#10831=VERTEX_POINT('',#185235);
#10832=VERTEX_POINT('',#185242);
#10833=VERTEX_POINT('',#185243);
#10834=VERTEX_POINT('',#185248);
#10835=VERTEX_POINT('',#185252);
#10836=VERTEX_POINT('',#185253);
#10837=VERTEX_POINT('',#185260);
#10838=VERTEX_POINT('',#185261);
#10839=VERTEX_POINT('',#185266);
#10840=VERTEX_POINT('',#185270);
#10841=VERTEX_POINT('',#185271);
#10842=VERTEX_POINT('',#185278);
#10843=VERTEX_POINT('',#185279);
#10844=VERTEX_POINT('',#185284);
#10845=VERTEX_POINT('',#185288);
#10846=VERTEX_POINT('',#185289);
#10847=VERTEX_POINT('',#185296);
#10848=VERTEX_POINT('',#185297);
#10849=VERTEX_POINT('',#185302);
#10850=VERTEX_POINT('',#185306);
#10851=VERTEX_POINT('',#185307);
#10852=VERTEX_POINT('',#185314);
#10853=VERTEX_POINT('',#185315);
#10854=VERTEX_POINT('',#185320);
#10855=VERTEX_POINT('',#185324);
#10856=VERTEX_POINT('',#185325);
#10857=VERTEX_POINT('',#185332);
#10858=VERTEX_POINT('',#185333);
#10859=VERTEX_POINT('',#185338);
#10860=VERTEX_POINT('',#185342);
#10861=VERTEX_POINT('',#185343);
#10862=VERTEX_POINT('',#185350);
#10863=VERTEX_POINT('',#185351);
#10864=VERTEX_POINT('',#185356);
#10865=VERTEX_POINT('',#185360);
#10866=VERTEX_POINT('',#185361);
#10867=VERTEX_POINT('',#185368);
#10868=VERTEX_POINT('',#185369);
#10869=VERTEX_POINT('',#185374);
#10870=VERTEX_POINT('',#185378);
#10871=VERTEX_POINT('',#185379);
#10872=VERTEX_POINT('',#185386);
#10873=VERTEX_POINT('',#185387);
#10874=VERTEX_POINT('',#185392);
#10875=VERTEX_POINT('',#185396);
#10876=VERTEX_POINT('',#185397);
#10877=VERTEX_POINT('',#185404);
#10878=VERTEX_POINT('',#185405);
#10879=VERTEX_POINT('',#185410);
#10880=VERTEX_POINT('',#185414);
#10881=VERTEX_POINT('',#185415);
#10882=VERTEX_POINT('',#185422);
#10883=VERTEX_POINT('',#185423);
#10884=VERTEX_POINT('',#185428);
#10885=VERTEX_POINT('',#185432);
#10886=VERTEX_POINT('',#185433);
#10887=VERTEX_POINT('',#185440);
#10888=VERTEX_POINT('',#185441);
#10889=VERTEX_POINT('',#185446);
#10890=VERTEX_POINT('',#185450);
#10891=VERTEX_POINT('',#185451);
#10892=VERTEX_POINT('',#185458);
#10893=VERTEX_POINT('',#185459);
#10894=VERTEX_POINT('',#185464);
#10895=VERTEX_POINT('',#185468);
#10896=VERTEX_POINT('',#185469);
#10897=VERTEX_POINT('',#185476);
#10898=VERTEX_POINT('',#185477);
#10899=VERTEX_POINT('',#185482);
#10900=VERTEX_POINT('',#185486);
#10901=VERTEX_POINT('',#185487);
#10902=VERTEX_POINT('',#185494);
#10903=VERTEX_POINT('',#185495);
#10904=VERTEX_POINT('',#185500);
#10905=VERTEX_POINT('',#185504);
#10906=VERTEX_POINT('',#185505);
#10907=VERTEX_POINT('',#185512);
#10908=VERTEX_POINT('',#185513);
#10909=VERTEX_POINT('',#185518);
#10910=VERTEX_POINT('',#185522);
#10911=VERTEX_POINT('',#185523);
#10912=VERTEX_POINT('',#185530);
#10913=VERTEX_POINT('',#185531);
#10914=VERTEX_POINT('',#185536);
#10915=VERTEX_POINT('',#185540);
#10916=VERTEX_POINT('',#185541);
#10917=VERTEX_POINT('',#185548);
#10918=VERTEX_POINT('',#185549);
#10919=VERTEX_POINT('',#185554);
#10920=VERTEX_POINT('',#185558);
#10921=VERTEX_POINT('',#185559);
#10922=VERTEX_POINT('',#185566);
#10923=VERTEX_POINT('',#185567);
#10924=VERTEX_POINT('',#185572);
#10925=VERTEX_POINT('',#185576);
#10926=VERTEX_POINT('',#185577);
#10927=VERTEX_POINT('',#185584);
#10928=VERTEX_POINT('',#185585);
#10929=VERTEX_POINT('',#185590);
#10930=VERTEX_POINT('',#185594);
#10931=VERTEX_POINT('',#185595);
#10932=VERTEX_POINT('',#185602);
#10933=VERTEX_POINT('',#186015);
#10934=VERTEX_POINT('',#186632);
#10935=VERTEX_POINT('',#186840);
#10936=VERTEX_POINT('',#187253);
#10937=VERTEX_POINT('',#187870);
#10938=VERTEX_POINT('',#188078);
#10939=VERTEX_POINT('',#188491);
#10940=VERTEX_POINT('',#189108);
#10941=VERTEX_POINT('',#189316);
#10942=VERTEX_POINT('',#189729);
#10943=VERTEX_POINT('',#190346);
#10944=VERTEX_POINT('',#190554);
#10945=VERTEX_POINT('',#190967);
#10946=VERTEX_POINT('',#191584);
#10947=VERTEX_POINT('',#191792);
#10948=VERTEX_POINT('',#192205);
#10949=VERTEX_POINT('',#192822);
#10950=VERTEX_POINT('',#193030);
#10951=VERTEX_POINT('',#193443);
#10952=VERTEX_POINT('',#194060);
#10953=VERTEX_POINT('',#194268);
#10954=VERTEX_POINT('',#194681);
#10955=VERTEX_POINT('',#195298);
#10956=VERTEX_POINT('',#195506);
#10957=VERTEX_POINT('',#195919);
#10958=VERTEX_POINT('',#196536);
#10959=VERTEX_POINT('',#196744);
#10960=VERTEX_POINT('',#197157);
#10961=VERTEX_POINT('',#197774);
#10962=VERTEX_POINT('',#197982);
#10963=VERTEX_POINT('',#198395);
#10964=VERTEX_POINT('',#199012);
#10965=VERTEX_POINT('',#199220);
#10966=VERTEX_POINT('',#199633);
#10967=VERTEX_POINT('',#200250);
#10968=VERTEX_POINT('',#200458);
#10969=VERTEX_POINT('',#200871);
#10970=VERTEX_POINT('',#201488);
#10971=VERTEX_POINT('',#201696);
#10972=VERTEX_POINT('',#202109);
#10973=VERTEX_POINT('',#202726);
#10974=VERTEX_POINT('',#202934);
#10975=VERTEX_POINT('',#203347);
#10976=VERTEX_POINT('',#203964);
#10977=VERTEX_POINT('',#204172);
#10978=VERTEX_POINT('',#204585);
#10979=VERTEX_POINT('',#205202);
#10980=VERTEX_POINT('',#205410);
#10981=VERTEX_POINT('',#205823);
#10982=VERTEX_POINT('',#206440);
#10983=VERTEX_POINT('',#206648);
#10984=VERTEX_POINT('',#207061);
#10985=VERTEX_POINT('',#207678);
#10986=VERTEX_POINT('',#207886);
#10987=VERTEX_POINT('',#208299);
#10988=VERTEX_POINT('',#208916);
#10989=VERTEX_POINT('',#209124);
#10990=VERTEX_POINT('',#209537);
#10991=VERTEX_POINT('',#210154);
#10992=VERTEX_POINT('',#210362);
#10993=VERTEX_POINT('',#210775);
#10994=VERTEX_POINT('',#211392);
#10995=VERTEX_POINT('',#211600);
#10996=VERTEX_POINT('',#212013);
#10997=VERTEX_POINT('',#212630);
#10998=VERTEX_POINT('',#212838);
#10999=VERTEX_POINT('',#213251);
#11000=VERTEX_POINT('',#213868);
#11001=VERTEX_POINT('',#214098);
#11002=VERTEX_POINT('',#214100);
#11003=VERTEX_POINT('',#214306);
#11004=VERTEX_POINT('',#214308);
#11005=VERTEX_POINT('',#214310);
#11006=VERTEX_POINT('',#214312);
#11007=VERTEX_POINT('',#214314);
#11008=VERTEX_POINT('',#214316);
#13954=EDGE_CURVE('',#10617,#10618,#7130,.T.);
#13955=EDGE_CURVE('',#10619,#10617,#7131,.T.);
#13956=EDGE_CURVE('',#10620,#10619,#7132,.T.);
#13957=EDGE_CURVE('',#10618,#10620,#7133,.T.);
#13958=EDGE_CURVE('',#10621,#10622,#7134,.T.);
#13959=EDGE_CURVE('',#10623,#10621,#7135,.T.);
#13960=EDGE_CURVE('',#10623,#10624,#7136,.T.);
#13961=EDGE_CURVE('',#10622,#10624,#7137,.T.);
#13962=EDGE_CURVE('',#10620,#10623,#7138,.T.);
#13963=EDGE_CURVE('',#10624,#10619,#7139,.T.);
#13964=EDGE_CURVE('',#10621,#10618,#4917,.T.);
#13965=EDGE_CURVE('',#10622,#10617,#4918,.T.);
#13966=EDGE_CURVE('',#10625,#10626,#691,.T.);
#13967=EDGE_CURVE('',#10626,#10627,#4919,.T.);
#13968=EDGE_CURVE('',#10627,#10628,#692,.T.);
#13969=EDGE_CURVE('',#10628,#10629,#7140,.T.);
#13970=EDGE_CURVE('',#10630,#10629,#4920,.T.);
#13971=EDGE_CURVE('',#10630,#10631,#4921,.T.);
#13972=EDGE_CURVE('',#10632,#10631,#4922,.T.);
#13973=EDGE_CURVE('',#10632,#10633,#7141,.T.);
#13974=EDGE_CURVE('',#10633,#10634,#693,.T.);
#13975=EDGE_CURVE('',#10634,#10635,#4923,.T.);
#13976=EDGE_CURVE('',#10635,#10636,#694,.T.);
#13977=EDGE_CURVE('',#10636,#10637,#7142,.T.);
#13978=EDGE_CURVE('',#10638,#10637,#4924,.T.);
#13979=EDGE_CURVE('',#10638,#10639,#4925,.T.);
#13980=EDGE_CURVE('',#10640,#10639,#4926,.T.);
#13981=EDGE_CURVE('',#10640,#10641,#7143,.T.);
#13982=EDGE_CURVE('',#10641,#10642,#695,.T.);
#13983=EDGE_CURVE('',#10642,#10643,#4927,.T.);
#13984=EDGE_CURVE('',#10643,#10644,#696,.T.);
#13985=EDGE_CURVE('',#10644,#10645,#7144,.T.);
#13986=EDGE_CURVE('',#10646,#10645,#4928,.T.);
#13987=EDGE_CURVE('',#10646,#10647,#4929,.T.);
#13988=EDGE_CURVE('',#10648,#10647,#4930,.T.);
#13989=EDGE_CURVE('',#10648,#10649,#7145,.T.);
#13990=EDGE_CURVE('',#10649,#10650,#697,.T.);
#13991=EDGE_CURVE('',#10650,#10651,#4931,.T.);
#13992=EDGE_CURVE('',#10651,#10652,#698,.T.);
#13993=EDGE_CURVE('',#10652,#10653,#7146,.T.);
#13994=EDGE_CURVE('',#10654,#10653,#4932,.T.);
#13995=EDGE_CURVE('',#10654,#10655,#4933,.T.);
#13996=EDGE_CURVE('',#10656,#10655,#4934,.T.);
#13997=EDGE_CURVE('',#10656,#10657,#7147,.T.);
#13998=EDGE_CURVE('',#10657,#10658,#699,.T.);
#13999=EDGE_CURVE('',#10658,#10659,#4935,.T.);
#14000=EDGE_CURVE('',#10659,#10660,#700,.T.);
#14001=EDGE_CURVE('',#10660,#10661,#7148,.T.);
#14002=EDGE_CURVE('',#10662,#10661,#4936,.T.);
#14003=EDGE_CURVE('',#10662,#10663,#4937,.T.);
#14004=EDGE_CURVE('',#10664,#10663,#4938,.T.);
#14005=EDGE_CURVE('',#10664,#10665,#7149,.T.);
#14006=EDGE_CURVE('',#10665,#10666,#701,.T.);
#14007=EDGE_CURVE('',#10666,#10667,#4939,.T.);
#14008=EDGE_CURVE('',#10667,#10668,#702,.T.);
#14009=EDGE_CURVE('',#10668,#10669,#7150,.T.);
#14010=EDGE_CURVE('',#10670,#10669,#4940,.T.);
#14011=EDGE_CURVE('',#10670,#10671,#4941,.T.);
#14012=EDGE_CURVE('',#10672,#10671,#4942,.T.);
#14013=EDGE_CURVE('',#10672,#10673,#7151,.T.);
#14014=EDGE_CURVE('',#10673,#10674,#703,.T.);
#14015=EDGE_CURVE('',#10674,#10675,#4943,.T.);
#14016=EDGE_CURVE('',#10675,#10676,#704,.T.);
#14017=EDGE_CURVE('',#10676,#10677,#7152,.T.);
#14018=EDGE_CURVE('',#10678,#10677,#4944,.T.);
#14019=EDGE_CURVE('',#10678,#10679,#4945,.T.);
#14020=EDGE_CURVE('',#10680,#10679,#4946,.T.);
#14021=EDGE_CURVE('',#10680,#10681,#7153,.T.);
#14022=EDGE_CURVE('',#10681,#10682,#705,.T.);
#14023=EDGE_CURVE('',#10682,#10683,#4947,.T.);
#14024=EDGE_CURVE('',#10683,#10684,#706,.T.);
#14025=EDGE_CURVE('',#10684,#10685,#7154,.T.);
#14026=EDGE_CURVE('',#10686,#10685,#4948,.T.);
#14027=EDGE_CURVE('',#10686,#10687,#4949,.T.);
#14028=EDGE_CURVE('',#10688,#10687,#4950,.T.);
#14029=EDGE_CURVE('',#10688,#10689,#7155,.T.);
#14030=EDGE_CURVE('',#10689,#10690,#707,.T.);
#14031=EDGE_CURVE('',#10690,#10691,#4951,.T.);
#14032=EDGE_CURVE('',#10691,#10692,#708,.T.);
#14033=EDGE_CURVE('',#10692,#10693,#7156,.T.);
#14034=EDGE_CURVE('',#10694,#10693,#4952,.T.);
#14035=EDGE_CURVE('',#10694,#10695,#4953,.T.);
#14036=EDGE_CURVE('',#10696,#10695,#4954,.T.);
#14037=EDGE_CURVE('',#10696,#10697,#7157,.T.);
#14038=EDGE_CURVE('',#10697,#10698,#709,.T.);
#14039=EDGE_CURVE('',#10698,#10699,#4955,.T.);
#14040=EDGE_CURVE('',#10699,#10700,#710,.T.);
#14041=EDGE_CURVE('',#10700,#10701,#7158,.T.);
#14042=EDGE_CURVE('',#10702,#10701,#4956,.T.);
#14043=EDGE_CURVE('',#10702,#10703,#4957,.T.);
#14044=EDGE_CURVE('',#10704,#10703,#4958,.T.);
#14045=EDGE_CURVE('',#10704,#10705,#7159,.T.);
#14046=EDGE_CURVE('',#10705,#10706,#711,.T.);
#14047=EDGE_CURVE('',#10706,#10707,#4959,.T.);
#14048=EDGE_CURVE('',#10707,#10708,#712,.T.);
#14049=EDGE_CURVE('',#10708,#10709,#7160,.T.);
#14050=EDGE_CURVE('',#10710,#10709,#4960,.T.);
#14051=EDGE_CURVE('',#10710,#10711,#4961,.T.);
#14052=EDGE_CURVE('',#10712,#10711,#4962,.T.);
#14053=EDGE_CURVE('',#10712,#10713,#7161,.T.);
#14054=EDGE_CURVE('',#10713,#10714,#713,.T.);
#14055=EDGE_CURVE('',#10714,#10715,#4963,.T.);
#14056=EDGE_CURVE('',#10715,#10716,#714,.T.);
#14057=EDGE_CURVE('',#10716,#10717,#7162,.T.);
#14058=EDGE_CURVE('',#10718,#10717,#4964,.T.);
#14059=EDGE_CURVE('',#10718,#10719,#4965,.T.);
#14060=EDGE_CURVE('',#10720,#10719,#4966,.T.);
#14061=EDGE_CURVE('',#10720,#10721,#7163,.T.);
#14062=EDGE_CURVE('',#10721,#10722,#715,.T.);
#14063=EDGE_CURVE('',#10722,#10723,#4967,.T.);
#14064=EDGE_CURVE('',#10723,#10724,#716,.T.);
#14065=EDGE_CURVE('',#10724,#10725,#7164,.T.);
#14066=EDGE_CURVE('',#10726,#10725,#4968,.T.);
#14067=EDGE_CURVE('',#10726,#10727,#4969,.T.);
#14068=EDGE_CURVE('',#10728,#10727,#4970,.T.);
#14069=EDGE_CURVE('',#10728,#10729,#7165,.T.);
#14070=EDGE_CURVE('',#10729,#10730,#717,.T.);
#14071=EDGE_CURVE('',#10730,#10731,#4971,.T.);
#14072=EDGE_CURVE('',#10731,#10732,#718,.T.);
#14073=EDGE_CURVE('',#10732,#10733,#7166,.T.);
#14074=EDGE_CURVE('',#10734,#10733,#4972,.T.);
#14075=EDGE_CURVE('',#10734,#10735,#4973,.T.);
#14076=EDGE_CURVE('',#10736,#10735,#4974,.T.);
#14077=EDGE_CURVE('',#10736,#10737,#7167,.T.);
#14078=EDGE_CURVE('',#10737,#10738,#719,.T.);
#14079=EDGE_CURVE('',#10738,#10739,#4975,.T.);
#14080=EDGE_CURVE('',#10739,#10740,#720,.T.);
#14081=EDGE_CURVE('',#10740,#10741,#7168,.T.);
#14082=EDGE_CURVE('',#10742,#10741,#4976,.T.);
#14083=EDGE_CURVE('',#10742,#10743,#4977,.T.);
#14084=EDGE_CURVE('',#10744,#10743,#4978,.T.);
#14085=EDGE_CURVE('',#10744,#10745,#7169,.T.);
#14086=EDGE_CURVE('',#10745,#10746,#721,.T.);
#14087=EDGE_CURVE('',#10746,#10747,#4979,.T.);
#14088=EDGE_CURVE('',#10747,#10748,#722,.T.);
#14089=EDGE_CURVE('',#10748,#10749,#7170,.T.);
#14090=EDGE_CURVE('',#10750,#10749,#4980,.T.);
#14091=EDGE_CURVE('',#10750,#10751,#4981,.T.);
#14092=EDGE_CURVE('',#10752,#10751,#4982,.T.);
#14093=EDGE_CURVE('',#10752,#10753,#7171,.T.);
#14094=EDGE_CURVE('',#10753,#10754,#723,.T.);
#14095=EDGE_CURVE('',#10754,#10755,#4983,.T.);
#14096=EDGE_CURVE('',#10755,#10756,#724,.T.);
#14097=EDGE_CURVE('',#10756,#10757,#7172,.T.);
#14098=EDGE_CURVE('',#10758,#10757,#4984,.T.);
#14099=EDGE_CURVE('',#10758,#10759,#4985,.T.);
#14100=EDGE_CURVE('',#10760,#10759,#4986,.T.);
#14101=EDGE_CURVE('',#10760,#10761,#7173,.T.);
#14102=EDGE_CURVE('',#10761,#10762,#725,.T.);
#14103=EDGE_CURVE('',#10762,#10763,#4987,.T.);
#14104=EDGE_CURVE('',#10763,#10764,#726,.T.);
#14105=EDGE_CURVE('',#10764,#10765,#7174,.T.);
#14106=EDGE_CURVE('',#10766,#10765,#4988,.T.);
#14107=EDGE_CURVE('',#10766,#10767,#4989,.T.);
#14108=EDGE_CURVE('',#10768,#10767,#4990,.T.);
#14109=EDGE_CURVE('',#10768,#10769,#7175,.T.);
#14110=EDGE_CURVE('',#10769,#10770,#727,.T.);
#14111=EDGE_CURVE('',#10770,#10771,#4991,.T.);
#14112=EDGE_CURVE('',#10771,#10772,#728,.T.);
#14113=EDGE_CURVE('',#10772,#10773,#7176,.T.);
#14114=EDGE_CURVE('',#10774,#10773,#4992,.T.);
#14115=EDGE_CURVE('',#10774,#10775,#4993,.T.);
#14116=EDGE_CURVE('',#10776,#10775,#4994,.T.);
#14117=EDGE_CURVE('',#10776,#10777,#7177,.T.);
#14118=EDGE_CURVE('',#10777,#10778,#729,.T.);
#14119=EDGE_CURVE('',#10778,#10779,#4995,.T.);
#14120=EDGE_CURVE('',#10779,#10780,#730,.T.);
#14121=EDGE_CURVE('',#10780,#10781,#7178,.T.);
#14122=EDGE_CURVE('',#10782,#10781,#4996,.T.);
#14123=EDGE_CURVE('',#10782,#10783,#4997,.T.);
#14124=EDGE_CURVE('',#10784,#10783,#4998,.T.);
#14125=EDGE_CURVE('',#10784,#10785,#7179,.T.);
#14126=EDGE_CURVE('',#10785,#10786,#731,.T.);
#14127=EDGE_CURVE('',#10786,#10787,#4999,.T.);
#14128=EDGE_CURVE('',#10787,#10788,#732,.T.);
#14129=EDGE_CURVE('',#10788,#10789,#7180,.T.);
#14130=EDGE_CURVE('',#10790,#10789,#5000,.T.);
#14131=EDGE_CURVE('',#10790,#10791,#5001,.T.);
#14132=EDGE_CURVE('',#10792,#10791,#5002,.T.);
#14133=EDGE_CURVE('',#10792,#10793,#7181,.T.);
#14134=EDGE_CURVE('',#10793,#10794,#733,.T.);
#14135=EDGE_CURVE('',#10794,#10795,#5003,.T.);
#14136=EDGE_CURVE('',#10795,#10796,#734,.T.);
#14137=EDGE_CURVE('',#10796,#10797,#7182,.T.);
#14138=EDGE_CURVE('',#10798,#10797,#5004,.T.);
#14139=EDGE_CURVE('',#10798,#10799,#5005,.T.);
#14140=EDGE_CURVE('',#10800,#10799,#5006,.T.);
#14141=EDGE_CURVE('',#10800,#10801,#7183,.T.);
#14142=EDGE_CURVE('',#10801,#10802,#735,.T.);
#14143=EDGE_CURVE('',#10802,#10803,#5007,.T.);
#14144=EDGE_CURVE('',#10803,#10804,#736,.T.);
#14145=EDGE_CURVE('',#10804,#10805,#7184,.T.);
#14146=EDGE_CURVE('',#10806,#10805,#5008,.T.);
#14147=EDGE_CURVE('',#10806,#10807,#5009,.T.);
#14148=EDGE_CURVE('',#10808,#10807,#5010,.T.);
#14149=EDGE_CURVE('',#10808,#10809,#7185,.T.);
#14150=EDGE_CURVE('',#10809,#10810,#737,.T.);
#14151=EDGE_CURVE('',#10810,#10811,#5011,.T.);
#14152=EDGE_CURVE('',#10811,#10812,#738,.T.);
#14153=EDGE_CURVE('',#10812,#10813,#7186,.T.);
#14154=EDGE_CURVE('',#10814,#10813,#5012,.T.);
#14155=EDGE_CURVE('',#10814,#10815,#5013,.T.);
#14156=EDGE_CURVE('',#10816,#10815,#5014,.T.);
#14157=EDGE_CURVE('',#10816,#10625,#7187,.T.);
#14158=EDGE_CURVE('',#10817,#10818,#5015,.T.);
#14159=EDGE_CURVE('',#10818,#10816,#7188,.T.);
#14160=EDGE_CURVE('',#10815,#10817,#7189,.T.);
#14161=EDGE_CURVE('',#10819,#10818,#7190,.T.);
#14162=EDGE_CURVE('',#10819,#10625,#7191,.T.);
#14163=EDGE_CURVE('',#10820,#10821,#5016,.T.);
#14164=EDGE_CURVE('',#10821,#10814,#7192,.T.);
#14165=EDGE_CURVE('',#10813,#10820,#7193,.T.);
#14166=EDGE_CURVE('',#10817,#10821,#5017,.T.);
#14167=EDGE_CURVE('',#10822,#10823,#5018,.T.);
#14168=EDGE_CURVE('',#10823,#10808,#7194,.T.);
#14169=EDGE_CURVE('',#10807,#10822,#7195,.T.);
#14170=EDGE_CURVE('',#10824,#10823,#7196,.T.);
#14171=EDGE_CURVE('',#10824,#10809,#7197,.T.);
#14172=EDGE_CURVE('',#10825,#10826,#5019,.T.);
#14173=EDGE_CURVE('',#10826,#10806,#7198,.T.);
#14174=EDGE_CURVE('',#10805,#10825,#7199,.T.);
#14175=EDGE_CURVE('',#10822,#10826,#5020,.T.);
#14176=EDGE_CURVE('',#10827,#10828,#5021,.T.);
#14177=EDGE_CURVE('',#10828,#10800,#7200,.T.);
#14178=EDGE_CURVE('',#10799,#10827,#7201,.T.);
#14179=EDGE_CURVE('',#10829,#10828,#7202,.T.);
#14180=EDGE_CURVE('',#10829,#10801,#7203,.T.);
#14181=EDGE_CURVE('',#10830,#10831,#5022,.T.);
#14182=EDGE_CURVE('',#10831,#10798,#7204,.T.);
#14183=EDGE_CURVE('',#10797,#10830,#7205,.T.);
#14184=EDGE_CURVE('',#10827,#10831,#5023,.T.);
#14185=EDGE_CURVE('',#10832,#10833,#5024,.T.);
#14186=EDGE_CURVE('',#10833,#10792,#7206,.T.);
#14187=EDGE_CURVE('',#10791,#10832,#7207,.T.);
#14188=EDGE_CURVE('',#10834,#10833,#7208,.T.);
#14189=EDGE_CURVE('',#10834,#10793,#7209,.T.);
#14190=EDGE_CURVE('',#10835,#10836,#5025,.T.);
#14191=EDGE_CURVE('',#10836,#10790,#7210,.T.);
#14192=EDGE_CURVE('',#10789,#10835,#7211,.T.);
#14193=EDGE_CURVE('',#10832,#10836,#5026,.T.);
#14194=EDGE_CURVE('',#10837,#10838,#5027,.T.);
#14195=EDGE_CURVE('',#10838,#10784,#7212,.T.);
#14196=EDGE_CURVE('',#10783,#10837,#7213,.T.);
#14197=EDGE_CURVE('',#10839,#10838,#7214,.T.);
#14198=EDGE_CURVE('',#10839,#10785,#7215,.T.);
#14199=EDGE_CURVE('',#10840,#10841,#5028,.T.);
#14200=EDGE_CURVE('',#10841,#10782,#7216,.T.);
#14201=EDGE_CURVE('',#10781,#10840,#7217,.T.);
#14202=EDGE_CURVE('',#10837,#10841,#5029,.T.);
#14203=EDGE_CURVE('',#10842,#10843,#5030,.T.);
#14204=EDGE_CURVE('',#10843,#10776,#7218,.T.);
#14205=EDGE_CURVE('',#10775,#10842,#7219,.T.);
#14206=EDGE_CURVE('',#10844,#10843,#7220,.T.);
#14207=EDGE_CURVE('',#10844,#10777,#7221,.T.);
#14208=EDGE_CURVE('',#10845,#10846,#5031,.T.);
#14209=EDGE_CURVE('',#10846,#10774,#7222,.T.);
#14210=EDGE_CURVE('',#10773,#10845,#7223,.T.);
#14211=EDGE_CURVE('',#10842,#10846,#5032,.T.);
#14212=EDGE_CURVE('',#10847,#10848,#5033,.T.);
#14213=EDGE_CURVE('',#10848,#10768,#7224,.T.);
#14214=EDGE_CURVE('',#10767,#10847,#7225,.T.);
#14215=EDGE_CURVE('',#10849,#10848,#7226,.T.);
#14216=EDGE_CURVE('',#10849,#10769,#7227,.T.);
#14217=EDGE_CURVE('',#10850,#10851,#5034,.T.);
#14218=EDGE_CURVE('',#10851,#10766,#7228,.T.);
#14219=EDGE_CURVE('',#10765,#10850,#7229,.T.);
#14220=EDGE_CURVE('',#10847,#10851,#5035,.T.);
#14221=EDGE_CURVE('',#10852,#10853,#5036,.T.);
#14222=EDGE_CURVE('',#10853,#10760,#7230,.T.);
#14223=EDGE_CURVE('',#10759,#10852,#7231,.T.);
#14224=EDGE_CURVE('',#10854,#10853,#7232,.T.);
#14225=EDGE_CURVE('',#10854,#10761,#7233,.T.);
#14226=EDGE_CURVE('',#10855,#10856,#5037,.T.);
#14227=EDGE_CURVE('',#10856,#10758,#7234,.T.);
#14228=EDGE_CURVE('',#10757,#10855,#7235,.T.);
#14229=EDGE_CURVE('',#10852,#10856,#5038,.T.);
#14230=EDGE_CURVE('',#10857,#10858,#5039,.T.);
#14231=EDGE_CURVE('',#10858,#10752,#7236,.T.);
#14232=EDGE_CURVE('',#10751,#10857,#7237,.T.);
#14233=EDGE_CURVE('',#10859,#10858,#7238,.T.);
#14234=EDGE_CURVE('',#10859,#10753,#7239,.T.);
#14235=EDGE_CURVE('',#10860,#10861,#5040,.T.);
#14236=EDGE_CURVE('',#10861,#10750,#7240,.T.);
#14237=EDGE_CURVE('',#10749,#10860,#7241,.T.);
#14238=EDGE_CURVE('',#10857,#10861,#5041,.T.);
#14239=EDGE_CURVE('',#10862,#10863,#5042,.T.);
#14240=EDGE_CURVE('',#10863,#10744,#7242,.T.);
#14241=EDGE_CURVE('',#10743,#10862,#7243,.T.);
#14242=EDGE_CURVE('',#10864,#10863,#7244,.T.);
#14243=EDGE_CURVE('',#10864,#10745,#7245,.T.);
#14244=EDGE_CURVE('',#10865,#10866,#5043,.T.);
#14245=EDGE_CURVE('',#10866,#10742,#7246,.T.);
#14246=EDGE_CURVE('',#10741,#10865,#7247,.T.);
#14247=EDGE_CURVE('',#10862,#10866,#5044,.T.);
#14248=EDGE_CURVE('',#10867,#10868,#5045,.T.);
#14249=EDGE_CURVE('',#10868,#10736,#7248,.T.);
#14250=EDGE_CURVE('',#10735,#10867,#7249,.T.);
#14251=EDGE_CURVE('',#10869,#10868,#7250,.T.);
#14252=EDGE_CURVE('',#10869,#10737,#7251,.T.);
#14253=EDGE_CURVE('',#10870,#10871,#5046,.T.);
#14254=EDGE_CURVE('',#10871,#10734,#7252,.T.);
#14255=EDGE_CURVE('',#10733,#10870,#7253,.T.);
#14256=EDGE_CURVE('',#10867,#10871,#5047,.T.);
#14257=EDGE_CURVE('',#10872,#10873,#5048,.T.);
#14258=EDGE_CURVE('',#10873,#10728,#7254,.T.);
#14259=EDGE_CURVE('',#10727,#10872,#7255,.T.);
#14260=EDGE_CURVE('',#10874,#10873,#7256,.T.);
#14261=EDGE_CURVE('',#10874,#10729,#7257,.T.);
#14262=EDGE_CURVE('',#10875,#10876,#5049,.T.);
#14263=EDGE_CURVE('',#10876,#10726,#7258,.T.);
#14264=EDGE_CURVE('',#10725,#10875,#7259,.T.);
#14265=EDGE_CURVE('',#10872,#10876,#5050,.T.);
#14266=EDGE_CURVE('',#10877,#10878,#5051,.T.);
#14267=EDGE_CURVE('',#10878,#10720,#7260,.T.);
#14268=EDGE_CURVE('',#10719,#10877,#7261,.T.);
#14269=EDGE_CURVE('',#10879,#10878,#7262,.T.);
#14270=EDGE_CURVE('',#10879,#10721,#7263,.T.);
#14271=EDGE_CURVE('',#10880,#10881,#5052,.T.);
#14272=EDGE_CURVE('',#10881,#10718,#7264,.T.);
#14273=EDGE_CURVE('',#10717,#10880,#7265,.T.);
#14274=EDGE_CURVE('',#10877,#10881,#5053,.T.);
#14275=EDGE_CURVE('',#10882,#10883,#5054,.T.);
#14276=EDGE_CURVE('',#10883,#10712,#7266,.T.);
#14277=EDGE_CURVE('',#10711,#10882,#7267,.T.);
#14278=EDGE_CURVE('',#10884,#10883,#7268,.T.);
#14279=EDGE_CURVE('',#10884,#10713,#7269,.T.);
#14280=EDGE_CURVE('',#10885,#10886,#5055,.T.);
#14281=EDGE_CURVE('',#10886,#10710,#7270,.T.);
#14282=EDGE_CURVE('',#10709,#10885,#7271,.T.);
#14283=EDGE_CURVE('',#10882,#10886,#5056,.T.);
#14284=EDGE_CURVE('',#10887,#10888,#5057,.T.);
#14285=EDGE_CURVE('',#10888,#10704,#7272,.T.);
#14286=EDGE_CURVE('',#10703,#10887,#7273,.T.);
#14287=EDGE_CURVE('',#10889,#10888,#7274,.T.);
#14288=EDGE_CURVE('',#10889,#10705,#7275,.T.);
#14289=EDGE_CURVE('',#10890,#10891,#5058,.T.);
#14290=EDGE_CURVE('',#10891,#10702,#7276,.T.);
#14291=EDGE_CURVE('',#10701,#10890,#7277,.T.);
#14292=EDGE_CURVE('',#10887,#10891,#5059,.T.);
#14293=EDGE_CURVE('',#10892,#10893,#5060,.T.);
#14294=EDGE_CURVE('',#10893,#10696,#7278,.T.);
#14295=EDGE_CURVE('',#10695,#10892,#7279,.T.);
#14296=EDGE_CURVE('',#10894,#10893,#7280,.T.);
#14297=EDGE_CURVE('',#10894,#10697,#7281,.T.);
#14298=EDGE_CURVE('',#10895,#10896,#5061,.T.);
#14299=EDGE_CURVE('',#10896,#10694,#7282,.T.);
#14300=EDGE_CURVE('',#10693,#10895,#7283,.T.);
#14301=EDGE_CURVE('',#10892,#10896,#5062,.T.);
#14302=EDGE_CURVE('',#10897,#10898,#5063,.T.);
#14303=EDGE_CURVE('',#10898,#10688,#7284,.T.);
#14304=EDGE_CURVE('',#10687,#10897,#7285,.T.);
#14305=EDGE_CURVE('',#10899,#10898,#7286,.T.);
#14306=EDGE_CURVE('',#10899,#10689,#7287,.T.);
#14307=EDGE_CURVE('',#10900,#10901,#5064,.T.);
#14308=EDGE_CURVE('',#10901,#10686,#7288,.T.);
#14309=EDGE_CURVE('',#10685,#10900,#7289,.T.);
#14310=EDGE_CURVE('',#10897,#10901,#5065,.T.);
#14311=EDGE_CURVE('',#10902,#10903,#5066,.T.);
#14312=EDGE_CURVE('',#10903,#10680,#7290,.T.);
#14313=EDGE_CURVE('',#10679,#10902,#7291,.T.);
#14314=EDGE_CURVE('',#10904,#10903,#7292,.T.);
#14315=EDGE_CURVE('',#10904,#10681,#7293,.T.);
#14316=EDGE_CURVE('',#10905,#10906,#5067,.T.);
#14317=EDGE_CURVE('',#10906,#10678,#7294,.T.);
#14318=EDGE_CURVE('',#10677,#10905,#7295,.T.);
#14319=EDGE_CURVE('',#10902,#10906,#5068,.T.);
#14320=EDGE_CURVE('',#10907,#10908,#5069,.T.);
#14321=EDGE_CURVE('',#10908,#10672,#7296,.T.);
#14322=EDGE_CURVE('',#10671,#10907,#7297,.T.);
#14323=EDGE_CURVE('',#10909,#10908,#7298,.T.);
#14324=EDGE_CURVE('',#10909,#10673,#7299,.T.);
#14325=EDGE_CURVE('',#10910,#10911,#5070,.T.);
#14326=EDGE_CURVE('',#10911,#10670,#7300,.T.);
#14327=EDGE_CURVE('',#10669,#10910,#7301,.T.);
#14328=EDGE_CURVE('',#10907,#10911,#5071,.T.);
#14329=EDGE_CURVE('',#10912,#10913,#5072,.T.);
#14330=EDGE_CURVE('',#10913,#10664,#7302,.T.);
#14331=EDGE_CURVE('',#10663,#10912,#7303,.T.);
#14332=EDGE_CURVE('',#10914,#10913,#7304,.T.);
#14333=EDGE_CURVE('',#10914,#10665,#7305,.T.);
#14334=EDGE_CURVE('',#10915,#10916,#5073,.T.);
#14335=EDGE_CURVE('',#10916,#10662,#7306,.T.);
#14336=EDGE_CURVE('',#10661,#10915,#7307,.T.);
#14337=EDGE_CURVE('',#10912,#10916,#5074,.T.);
#14338=EDGE_CURVE('',#10917,#10918,#5075,.T.);
#14339=EDGE_CURVE('',#10918,#10656,#7308,.T.);
#14340=EDGE_CURVE('',#10655,#10917,#7309,.T.);
#14341=EDGE_CURVE('',#10919,#10918,#7310,.T.);
#14342=EDGE_CURVE('',#10919,#10657,#7311,.T.);
#14343=EDGE_CURVE('',#10920,#10921,#5076,.T.);
#14344=EDGE_CURVE('',#10921,#10654,#7312,.T.);
#14345=EDGE_CURVE('',#10653,#10920,#7313,.T.);
#14346=EDGE_CURVE('',#10917,#10921,#5077,.T.);
#14347=EDGE_CURVE('',#10922,#10923,#5078,.T.);
#14348=EDGE_CURVE('',#10923,#10648,#7314,.T.);
#14349=EDGE_CURVE('',#10647,#10922,#7315,.T.);
#14350=EDGE_CURVE('',#10924,#10923,#7316,.T.);
#14351=EDGE_CURVE('',#10924,#10649,#7317,.T.);
#14352=EDGE_CURVE('',#10925,#10926,#5079,.T.);
#14353=EDGE_CURVE('',#10926,#10646,#7318,.T.);
#14354=EDGE_CURVE('',#10645,#10925,#7319,.T.);
#14355=EDGE_CURVE('',#10922,#10926,#5080,.T.);
#14356=EDGE_CURVE('',#10927,#10928,#5081,.T.);
#14357=EDGE_CURVE('',#10928,#10640,#7320,.T.);
#14358=EDGE_CURVE('',#10639,#10927,#7321,.T.);
#14359=EDGE_CURVE('',#10929,#10928,#7322,.T.);
#14360=EDGE_CURVE('',#10929,#10641,#7323,.T.);
#14361=EDGE_CURVE('',#10930,#10931,#5082,.T.);
#14362=EDGE_CURVE('',#10931,#10638,#7324,.T.);
#14363=EDGE_CURVE('',#10637,#10930,#7325,.T.);
#14364=EDGE_CURVE('',#10927,#10931,#5083,.T.);
#14365=EDGE_CURVE('',#10932,#10812,#7326,.T.);
#14366=EDGE_CURVE('',#10820,#10932,#7327,.T.);
#14367=EDGE_CURVE('',#10933,#10819,#739,.T.);
#14368=EDGE_CURVE('',#10626,#10933,#7328,.T.);
#14369=EDGE_CURVE('',#10932,#10934,#740,.T.);
#14370=EDGE_CURVE('',#10934,#10811,#7329,.T.);
#14371=EDGE_CURVE('',#10935,#10804,#7330,.T.);
#14372=EDGE_CURVE('',#10825,#10935,#7331,.T.);
#14373=EDGE_CURVE('',#10936,#10824,#741,.T.);
#14374=EDGE_CURVE('',#10810,#10936,#7332,.T.);
#14375=EDGE_CURVE('',#10935,#10937,#742,.T.);
#14376=EDGE_CURVE('',#10937,#10803,#7333,.T.);
#14377=EDGE_CURVE('',#10938,#10796,#7334,.T.);
#14378=EDGE_CURVE('',#10830,#10938,#7335,.T.);
#14379=EDGE_CURVE('',#10939,#10829,#743,.T.);
#14380=EDGE_CURVE('',#10802,#10939,#7336,.T.);
#14381=EDGE_CURVE('',#10938,#10940,#744,.T.);
#14382=EDGE_CURVE('',#10940,#10795,#7337,.T.);
#14383=EDGE_CURVE('',#10941,#10788,#7338,.T.);
#14384=EDGE_CURVE('',#10835,#10941,#7339,.T.);
#14385=EDGE_CURVE('',#10942,#10834,#745,.T.);
#14386=EDGE_CURVE('',#10794,#10942,#7340,.T.);
#14387=EDGE_CURVE('',#10941,#10943,#746,.T.);
#14388=EDGE_CURVE('',#10943,#10787,#7341,.T.);
#14389=EDGE_CURVE('',#10944,#10780,#7342,.T.);
#14390=EDGE_CURVE('',#10840,#10944,#7343,.T.);
#14391=EDGE_CURVE('',#10945,#10839,#747,.T.);
#14392=EDGE_CURVE('',#10786,#10945,#7344,.T.);
#14393=EDGE_CURVE('',#10944,#10946,#748,.T.);
#14394=EDGE_CURVE('',#10946,#10779,#7345,.T.);
#14395=EDGE_CURVE('',#10947,#10772,#7346,.T.);
#14396=EDGE_CURVE('',#10845,#10947,#7347,.T.);
#14397=EDGE_CURVE('',#10948,#10844,#749,.T.);
#14398=EDGE_CURVE('',#10778,#10948,#7348,.T.);
#14399=EDGE_CURVE('',#10947,#10949,#750,.T.);
#14400=EDGE_CURVE('',#10949,#10771,#7349,.T.);
#14401=EDGE_CURVE('',#10950,#10764,#7350,.T.);
#14402=EDGE_CURVE('',#10850,#10950,#7351,.T.);
#14403=EDGE_CURVE('',#10951,#10849,#751,.T.);
#14404=EDGE_CURVE('',#10770,#10951,#7352,.T.);
#14405=EDGE_CURVE('',#10950,#10952,#752,.T.);
#14406=EDGE_CURVE('',#10952,#10763,#7353,.T.);
#14407=EDGE_CURVE('',#10953,#10756,#7354,.T.);
#14408=EDGE_CURVE('',#10855,#10953,#7355,.T.);
#14409=EDGE_CURVE('',#10954,#10854,#753,.T.);
#14410=EDGE_CURVE('',#10762,#10954,#7356,.T.);
#14411=EDGE_CURVE('',#10953,#10955,#754,.T.);
#14412=EDGE_CURVE('',#10955,#10755,#7357,.T.);
#14413=EDGE_CURVE('',#10956,#10748,#7358,.T.);
#14414=EDGE_CURVE('',#10860,#10956,#7359,.T.);
#14415=EDGE_CURVE('',#10957,#10859,#755,.T.);
#14416=EDGE_CURVE('',#10754,#10957,#7360,.T.);
#14417=EDGE_CURVE('',#10956,#10958,#756,.T.);
#14418=EDGE_CURVE('',#10958,#10747,#7361,.T.);
#14419=EDGE_CURVE('',#10959,#10740,#7362,.T.);
#14420=EDGE_CURVE('',#10865,#10959,#7363,.T.);
#14421=EDGE_CURVE('',#10960,#10864,#757,.T.);
#14422=EDGE_CURVE('',#10746,#10960,#7364,.T.);
#14423=EDGE_CURVE('',#10959,#10961,#758,.T.);
#14424=EDGE_CURVE('',#10961,#10739,#7365,.T.);
#14425=EDGE_CURVE('',#10962,#10732,#7366,.T.);
#14426=EDGE_CURVE('',#10870,#10962,#7367,.T.);
#14427=EDGE_CURVE('',#10963,#10869,#759,.T.);
#14428=EDGE_CURVE('',#10738,#10963,#7368,.T.);
#14429=EDGE_CURVE('',#10962,#10964,#760,.T.);
#14430=EDGE_CURVE('',#10964,#10731,#7369,.T.);
#14431=EDGE_CURVE('',#10965,#10724,#7370,.T.);
#14432=EDGE_CURVE('',#10875,#10965,#7371,.T.);
#14433=EDGE_CURVE('',#10966,#10874,#761,.T.);
#14434=EDGE_CURVE('',#10730,#10966,#7372,.T.);
#14435=EDGE_CURVE('',#10965,#10967,#762,.T.);
#14436=EDGE_CURVE('',#10967,#10723,#7373,.T.);
#14437=EDGE_CURVE('',#10968,#10716,#7374,.T.);
#14438=EDGE_CURVE('',#10880,#10968,#7375,.T.);
#14439=EDGE_CURVE('',#10969,#10879,#763,.T.);
#14440=EDGE_CURVE('',#10722,#10969,#7376,.T.);
#14441=EDGE_CURVE('',#10968,#10970,#764,.T.);
#14442=EDGE_CURVE('',#10970,#10715,#7377,.T.);
#14443=EDGE_CURVE('',#10971,#10708,#7378,.T.);
#14444=EDGE_CURVE('',#10885,#10971,#7379,.T.);
#14445=EDGE_CURVE('',#10972,#10884,#765,.T.);
#14446=EDGE_CURVE('',#10714,#10972,#7380,.T.);
#14447=EDGE_CURVE('',#10971,#10973,#766,.T.);
#14448=EDGE_CURVE('',#10973,#10707,#7381,.T.);
#14449=EDGE_CURVE('',#10974,#10700,#7382,.T.);
#14450=EDGE_CURVE('',#10890,#10974,#7383,.T.);
#14451=EDGE_CURVE('',#10975,#10889,#767,.T.);
#14452=EDGE_CURVE('',#10706,#10975,#7384,.T.);
#14453=EDGE_CURVE('',#10974,#10976,#768,.T.);
#14454=EDGE_CURVE('',#10976,#10699,#7385,.T.);
#14455=EDGE_CURVE('',#10977,#10692,#7386,.T.);
#14456=EDGE_CURVE('',#10895,#10977,#7387,.T.);
#14457=EDGE_CURVE('',#10978,#10894,#769,.T.);
#14458=EDGE_CURVE('',#10698,#10978,#7388,.T.);
#14459=EDGE_CURVE('',#10977,#10979,#770,.T.);
#14460=EDGE_CURVE('',#10979,#10691,#7389,.T.);
#14461=EDGE_CURVE('',#10980,#10684,#7390,.T.);
#14462=EDGE_CURVE('',#10900,#10980,#7391,.T.);
#14463=EDGE_CURVE('',#10981,#10899,#771,.T.);
#14464=EDGE_CURVE('',#10690,#10981,#7392,.T.);
#14465=EDGE_CURVE('',#10980,#10982,#772,.T.);
#14466=EDGE_CURVE('',#10982,#10683,#7393,.T.);
#14467=EDGE_CURVE('',#10983,#10676,#7394,.T.);
#14468=EDGE_CURVE('',#10905,#10983,#7395,.T.);
#14469=EDGE_CURVE('',#10984,#10904,#773,.T.);
#14470=EDGE_CURVE('',#10682,#10984,#7396,.T.);
#14471=EDGE_CURVE('',#10983,#10985,#774,.T.);
#14472=EDGE_CURVE('',#10985,#10675,#7397,.T.);
#14473=EDGE_CURVE('',#10986,#10668,#7398,.T.);
#14474=EDGE_CURVE('',#10910,#10986,#7399,.T.);
#14475=EDGE_CURVE('',#10987,#10909,#775,.T.);
#14476=EDGE_CURVE('',#10674,#10987,#7400,.T.);
#14477=EDGE_CURVE('',#10986,#10988,#776,.T.);
#14478=EDGE_CURVE('',#10988,#10667,#7401,.T.);
#14479=EDGE_CURVE('',#10989,#10660,#7402,.T.);
#14480=EDGE_CURVE('',#10915,#10989,#7403,.T.);
#14481=EDGE_CURVE('',#10990,#10914,#777,.T.);
#14482=EDGE_CURVE('',#10666,#10990,#7404,.T.);
#14483=EDGE_CURVE('',#10989,#10991,#778,.T.);
#14484=EDGE_CURVE('',#10991,#10659,#7405,.T.);
#14485=EDGE_CURVE('',#10992,#10652,#7406,.T.);
#14486=EDGE_CURVE('',#10920,#10992,#7407,.T.);
#14487=EDGE_CURVE('',#10993,#10919,#779,.T.);
#14488=EDGE_CURVE('',#10658,#10993,#7408,.T.);
#14489=EDGE_CURVE('',#10992,#10994,#780,.T.);
#14490=EDGE_CURVE('',#10994,#10651,#7409,.T.);
#14491=EDGE_CURVE('',#10995,#10644,#7410,.T.);
#14492=EDGE_CURVE('',#10925,#10995,#7411,.T.);
#14493=EDGE_CURVE('',#10996,#10924,#781,.T.);
#14494=EDGE_CURVE('',#10650,#10996,#7412,.T.);
#14495=EDGE_CURVE('',#10995,#10997,#782,.T.);
#14496=EDGE_CURVE('',#10997,#10643,#7413,.T.);
#14497=EDGE_CURVE('',#10998,#10636,#7414,.T.);
#14498=EDGE_CURVE('',#10930,#10998,#7415,.T.);
#14499=EDGE_CURVE('',#10999,#10929,#783,.T.);
#14500=EDGE_CURVE('',#10642,#10999,#7416,.T.);
#14501=EDGE_CURVE('',#10998,#11000,#784,.T.);
#14502=EDGE_CURVE('',#11000,#10635,#7417,.T.);
#14503=EDGE_CURVE('',#10936,#10934,#5084,.T.);
#14504=EDGE_CURVE('',#10939,#10937,#5085,.T.);
#14505=EDGE_CURVE('',#10942,#10940,#5086,.T.);
#14506=EDGE_CURVE('',#10945,#10943,#5087,.T.);
#14507=EDGE_CURVE('',#10948,#10946,#5088,.T.);
#14508=EDGE_CURVE('',#10951,#10949,#5089,.T.);
#14509=EDGE_CURVE('',#10954,#10952,#5090,.T.);
#14510=EDGE_CURVE('',#10957,#10955,#5091,.T.);
#14511=EDGE_CURVE('',#10960,#10958,#5092,.T.);
#14512=EDGE_CURVE('',#10963,#10961,#5093,.T.);
#14513=EDGE_CURVE('',#10966,#10964,#5094,.T.);
#14514=EDGE_CURVE('',#10969,#10967,#5095,.T.);
#14515=EDGE_CURVE('',#10972,#10970,#5096,.T.);
#14516=EDGE_CURVE('',#10975,#10973,#5097,.T.);
#14517=EDGE_CURVE('',#10978,#10976,#5098,.T.);
#14518=EDGE_CURVE('',#10981,#10979,#5099,.T.);
#14519=EDGE_CURVE('',#10984,#10982,#5100,.T.);
#14520=EDGE_CURVE('',#10987,#10985,#5101,.T.);
#14521=EDGE_CURVE('',#10990,#10988,#5102,.T.);
#14522=EDGE_CURVE('',#10993,#10991,#5103,.T.);
#14523=EDGE_CURVE('',#10996,#10994,#5104,.T.);
#14524=EDGE_CURVE('',#10999,#10997,#5105,.T.);
#14525=EDGE_CURVE('',#11001,#11000,#5106,.T.);
#14526=EDGE_CURVE('',#11001,#11002,#785,.T.);
#14527=EDGE_CURVE('',#11002,#11003,#7418,.T.);
#14528=EDGE_CURVE('',#11004,#11003,#5107,.T.);
#14529=EDGE_CURVE('',#11004,#11005,#5108,.T.);
#14530=EDGE_CURVE('',#11006,#11005,#5109,.T.);
#14531=EDGE_CURVE('',#11006,#11007,#7419,.T.);
#14532=EDGE_CURVE('',#11007,#11008,#786,.T.);
#14533=EDGE_CURVE('',#10933,#11008,#5110,.T.);
#14534=EDGE_CURVE('',#10634,#11001,#7420,.T.);
#14535=EDGE_CURVE('',#11003,#10632,#7421,.T.);
#14536=EDGE_CURVE('',#10631,#11004,#7422,.T.);
#14537=EDGE_CURVE('',#11002,#10633,#7423,.T.);
#14538=EDGE_CURVE('',#11005,#10630,#7424,.T.);
#14539=EDGE_CURVE('',#10629,#11006,#7425,.T.);
#14540=EDGE_CURVE('',#11007,#10628,#7426,.T.);
#14541=EDGE_CURVE('',#11008,#10627,#7427,.T.);
#20138=ORIENTED_EDGE('',*,*,#13954,.F.);
#20139=ORIENTED_EDGE('',*,*,#13955,.F.);
#20140=ORIENTED_EDGE('',*,*,#13956,.F.);
#20141=ORIENTED_EDGE('',*,*,#13957,.F.);
#20142=ORIENTED_EDGE('',*,*,#13958,.F.);
#20143=ORIENTED_EDGE('',*,*,#13959,.F.);
#20144=ORIENTED_EDGE('',*,*,#13960,.T.);
#20145=ORIENTED_EDGE('',*,*,#13961,.F.);
#20146=ORIENTED_EDGE('',*,*,#13962,.F.);
#20147=ORIENTED_EDGE('',*,*,#13956,.T.);
#20148=ORIENTED_EDGE('',*,*,#13963,.F.);
#20149=ORIENTED_EDGE('',*,*,#13960,.F.);
#20150=ORIENTED_EDGE('',*,*,#13954,.T.);
#20151=ORIENTED_EDGE('',*,*,#13964,.F.);
#20152=ORIENTED_EDGE('',*,*,#13958,.T.);
#20153=ORIENTED_EDGE('',*,*,#13965,.T.);
#20154=ORIENTED_EDGE('',*,*,#13966,.T.);
#20155=ORIENTED_EDGE('',*,*,#13967,.T.);
#20156=ORIENTED_EDGE('',*,*,#13968,.T.);
#20157=ORIENTED_EDGE('',*,*,#13969,.T.);
#20158=ORIENTED_EDGE('',*,*,#13970,.F.);
#20159=ORIENTED_EDGE('',*,*,#13971,.T.);
#20160=ORIENTED_EDGE('',*,*,#13972,.F.);
#20161=ORIENTED_EDGE('',*,*,#13973,.T.);
#20162=ORIENTED_EDGE('',*,*,#13974,.T.);
#20163=ORIENTED_EDGE('',*,*,#13975,.T.);
#20164=ORIENTED_EDGE('',*,*,#13976,.T.);
#20165=ORIENTED_EDGE('',*,*,#13977,.T.);
#20166=ORIENTED_EDGE('',*,*,#13978,.F.);
#20167=ORIENTED_EDGE('',*,*,#13979,.T.);
#20168=ORIENTED_EDGE('',*,*,#13980,.F.);
#20169=ORIENTED_EDGE('',*,*,#13981,.T.);
#20170=ORIENTED_EDGE('',*,*,#13982,.T.);
#20171=ORIENTED_EDGE('',*,*,#13983,.T.);
#20172=ORIENTED_EDGE('',*,*,#13984,.T.);
#20173=ORIENTED_EDGE('',*,*,#13985,.T.);
#20174=ORIENTED_EDGE('',*,*,#13986,.F.);
#20175=ORIENTED_EDGE('',*,*,#13987,.T.);
#20176=ORIENTED_EDGE('',*,*,#13988,.F.);
#20177=ORIENTED_EDGE('',*,*,#13989,.T.);
#20178=ORIENTED_EDGE('',*,*,#13990,.T.);
#20179=ORIENTED_EDGE('',*,*,#13991,.T.);
#20180=ORIENTED_EDGE('',*,*,#13992,.T.);
#20181=ORIENTED_EDGE('',*,*,#13993,.T.);
#20182=ORIENTED_EDGE('',*,*,#13994,.F.);
#20183=ORIENTED_EDGE('',*,*,#13995,.T.);
#20184=ORIENTED_EDGE('',*,*,#13996,.F.);
#20185=ORIENTED_EDGE('',*,*,#13997,.T.);
#20186=ORIENTED_EDGE('',*,*,#13998,.T.);
#20187=ORIENTED_EDGE('',*,*,#13999,.T.);
#20188=ORIENTED_EDGE('',*,*,#14000,.T.);
#20189=ORIENTED_EDGE('',*,*,#14001,.T.);
#20190=ORIENTED_EDGE('',*,*,#14002,.F.);
#20191=ORIENTED_EDGE('',*,*,#14003,.T.);
#20192=ORIENTED_EDGE('',*,*,#14004,.F.);
#20193=ORIENTED_EDGE('',*,*,#14005,.T.);
#20194=ORIENTED_EDGE('',*,*,#14006,.T.);
#20195=ORIENTED_EDGE('',*,*,#14007,.T.);
#20196=ORIENTED_EDGE('',*,*,#14008,.T.);
#20197=ORIENTED_EDGE('',*,*,#14009,.T.);
#20198=ORIENTED_EDGE('',*,*,#14010,.F.);
#20199=ORIENTED_EDGE('',*,*,#14011,.T.);
#20200=ORIENTED_EDGE('',*,*,#14012,.F.);
#20201=ORIENTED_EDGE('',*,*,#14013,.T.);
#20202=ORIENTED_EDGE('',*,*,#14014,.T.);
#20203=ORIENTED_EDGE('',*,*,#14015,.T.);
#20204=ORIENTED_EDGE('',*,*,#14016,.T.);
#20205=ORIENTED_EDGE('',*,*,#14017,.T.);
#20206=ORIENTED_EDGE('',*,*,#14018,.F.);
#20207=ORIENTED_EDGE('',*,*,#14019,.T.);
#20208=ORIENTED_EDGE('',*,*,#14020,.F.);
#20209=ORIENTED_EDGE('',*,*,#14021,.T.);
#20210=ORIENTED_EDGE('',*,*,#14022,.T.);
#20211=ORIENTED_EDGE('',*,*,#14023,.T.);
#20212=ORIENTED_EDGE('',*,*,#14024,.T.);
#20213=ORIENTED_EDGE('',*,*,#14025,.T.);
#20214=ORIENTED_EDGE('',*,*,#14026,.F.);
#20215=ORIENTED_EDGE('',*,*,#14027,.T.);
#20216=ORIENTED_EDGE('',*,*,#14028,.F.);
#20217=ORIENTED_EDGE('',*,*,#14029,.T.);
#20218=ORIENTED_EDGE('',*,*,#14030,.T.);
#20219=ORIENTED_EDGE('',*,*,#14031,.T.);
#20220=ORIENTED_EDGE('',*,*,#14032,.T.);
#20221=ORIENTED_EDGE('',*,*,#14033,.T.);
#20222=ORIENTED_EDGE('',*,*,#14034,.F.);
#20223=ORIENTED_EDGE('',*,*,#14035,.T.);
#20224=ORIENTED_EDGE('',*,*,#14036,.F.);
#20225=ORIENTED_EDGE('',*,*,#14037,.T.);
#20226=ORIENTED_EDGE('',*,*,#14038,.T.);
#20227=ORIENTED_EDGE('',*,*,#14039,.T.);
#20228=ORIENTED_EDGE('',*,*,#14040,.T.);
#20229=ORIENTED_EDGE('',*,*,#14041,.T.);
#20230=ORIENTED_EDGE('',*,*,#14042,.F.);
#20231=ORIENTED_EDGE('',*,*,#14043,.T.);
#20232=ORIENTED_EDGE('',*,*,#14044,.F.);
#20233=ORIENTED_EDGE('',*,*,#14045,.T.);
#20234=ORIENTED_EDGE('',*,*,#14046,.T.);
#20235=ORIENTED_EDGE('',*,*,#14047,.T.);
#20236=ORIENTED_EDGE('',*,*,#14048,.T.);
#20237=ORIENTED_EDGE('',*,*,#14049,.T.);
#20238=ORIENTED_EDGE('',*,*,#14050,.F.);
#20239=ORIENTED_EDGE('',*,*,#14051,.T.);
#20240=ORIENTED_EDGE('',*,*,#14052,.F.);
#20241=ORIENTED_EDGE('',*,*,#14053,.T.);
#20242=ORIENTED_EDGE('',*,*,#14054,.T.);
#20243=ORIENTED_EDGE('',*,*,#14055,.T.);
#20244=ORIENTED_EDGE('',*,*,#14056,.T.);
#20245=ORIENTED_EDGE('',*,*,#14057,.T.);
#20246=ORIENTED_EDGE('',*,*,#14058,.F.);
#20247=ORIENTED_EDGE('',*,*,#14059,.T.);
#20248=ORIENTED_EDGE('',*,*,#14060,.F.);
#20249=ORIENTED_EDGE('',*,*,#14061,.T.);
#20250=ORIENTED_EDGE('',*,*,#14062,.T.);
#20251=ORIENTED_EDGE('',*,*,#14063,.T.);
#20252=ORIENTED_EDGE('',*,*,#14064,.T.);
#20253=ORIENTED_EDGE('',*,*,#14065,.T.);
#20254=ORIENTED_EDGE('',*,*,#14066,.F.);
#20255=ORIENTED_EDGE('',*,*,#14067,.T.);
#20256=ORIENTED_EDGE('',*,*,#14068,.F.);
#20257=ORIENTED_EDGE('',*,*,#14069,.T.);
#20258=ORIENTED_EDGE('',*,*,#14070,.T.);
#20259=ORIENTED_EDGE('',*,*,#14071,.T.);
#20260=ORIENTED_EDGE('',*,*,#14072,.T.);
#20261=ORIENTED_EDGE('',*,*,#14073,.T.);
#20262=ORIENTED_EDGE('',*,*,#14074,.F.);
#20263=ORIENTED_EDGE('',*,*,#14075,.T.);
#20264=ORIENTED_EDGE('',*,*,#14076,.F.);
#20265=ORIENTED_EDGE('',*,*,#14077,.T.);
#20266=ORIENTED_EDGE('',*,*,#14078,.T.);
#20267=ORIENTED_EDGE('',*,*,#14079,.T.);
#20268=ORIENTED_EDGE('',*,*,#14080,.T.);
#20269=ORIENTED_EDGE('',*,*,#14081,.T.);
#20270=ORIENTED_EDGE('',*,*,#14082,.F.);
#20271=ORIENTED_EDGE('',*,*,#14083,.T.);
#20272=ORIENTED_EDGE('',*,*,#14084,.F.);
#20273=ORIENTED_EDGE('',*,*,#14085,.T.);
#20274=ORIENTED_EDGE('',*,*,#14086,.T.);
#20275=ORIENTED_EDGE('',*,*,#14087,.T.);
#20276=ORIENTED_EDGE('',*,*,#14088,.T.);
#20277=ORIENTED_EDGE('',*,*,#14089,.T.);
#20278=ORIENTED_EDGE('',*,*,#14090,.F.);
#20279=ORIENTED_EDGE('',*,*,#14091,.T.);
#20280=ORIENTED_EDGE('',*,*,#14092,.F.);
#20281=ORIENTED_EDGE('',*,*,#14093,.T.);
#20282=ORIENTED_EDGE('',*,*,#14094,.T.);
#20283=ORIENTED_EDGE('',*,*,#14095,.T.);
#20284=ORIENTED_EDGE('',*,*,#14096,.T.);
#20285=ORIENTED_EDGE('',*,*,#14097,.T.);
#20286=ORIENTED_EDGE('',*,*,#14098,.F.);
#20287=ORIENTED_EDGE('',*,*,#14099,.T.);
#20288=ORIENTED_EDGE('',*,*,#14100,.F.);
#20289=ORIENTED_EDGE('',*,*,#14101,.T.);
#20290=ORIENTED_EDGE('',*,*,#14102,.T.);
#20291=ORIENTED_EDGE('',*,*,#14103,.T.);
#20292=ORIENTED_EDGE('',*,*,#14104,.T.);
#20293=ORIENTED_EDGE('',*,*,#14105,.T.);
#20294=ORIENTED_EDGE('',*,*,#14106,.F.);
#20295=ORIENTED_EDGE('',*,*,#14107,.T.);
#20296=ORIENTED_EDGE('',*,*,#14108,.F.);
#20297=ORIENTED_EDGE('',*,*,#14109,.T.);
#20298=ORIENTED_EDGE('',*,*,#14110,.T.);
#20299=ORIENTED_EDGE('',*,*,#14111,.T.);
#20300=ORIENTED_EDGE('',*,*,#14112,.T.);
#20301=ORIENTED_EDGE('',*,*,#14113,.T.);
#20302=ORIENTED_EDGE('',*,*,#14114,.F.);
#20303=ORIENTED_EDGE('',*,*,#14115,.T.);
#20304=ORIENTED_EDGE('',*,*,#14116,.F.);
#20305=ORIENTED_EDGE('',*,*,#14117,.T.);
#20306=ORIENTED_EDGE('',*,*,#14118,.T.);
#20307=ORIENTED_EDGE('',*,*,#14119,.T.);
#20308=ORIENTED_EDGE('',*,*,#14120,.T.);
#20309=ORIENTED_EDGE('',*,*,#14121,.T.);
#20310=ORIENTED_EDGE('',*,*,#14122,.F.);
#20311=ORIENTED_EDGE('',*,*,#14123,.T.);
#20312=ORIENTED_EDGE('',*,*,#14124,.F.);
#20313=ORIENTED_EDGE('',*,*,#14125,.T.);
#20314=ORIENTED_EDGE('',*,*,#14126,.T.);
#20315=ORIENTED_EDGE('',*,*,#14127,.T.);
#20316=ORIENTED_EDGE('',*,*,#14128,.T.);
#20317=ORIENTED_EDGE('',*,*,#14129,.T.);
#20318=ORIENTED_EDGE('',*,*,#14130,.F.);
#20319=ORIENTED_EDGE('',*,*,#14131,.T.);
#20320=ORIENTED_EDGE('',*,*,#14132,.F.);
#20321=ORIENTED_EDGE('',*,*,#14133,.T.);
#20322=ORIENTED_EDGE('',*,*,#14134,.T.);
#20323=ORIENTED_EDGE('',*,*,#14135,.T.);
#20324=ORIENTED_EDGE('',*,*,#14136,.T.);
#20325=ORIENTED_EDGE('',*,*,#14137,.T.);
#20326=ORIENTED_EDGE('',*,*,#14138,.F.);
#20327=ORIENTED_EDGE('',*,*,#14139,.T.);
#20328=ORIENTED_EDGE('',*,*,#14140,.F.);
#20329=ORIENTED_EDGE('',*,*,#14141,.T.);
#20330=ORIENTED_EDGE('',*,*,#14142,.T.);
#20331=ORIENTED_EDGE('',*,*,#14143,.T.);
#20332=ORIENTED_EDGE('',*,*,#14144,.T.);
#20333=ORIENTED_EDGE('',*,*,#14145,.T.);
#20334=ORIENTED_EDGE('',*,*,#14146,.F.);
#20335=ORIENTED_EDGE('',*,*,#14147,.T.);
#20336=ORIENTED_EDGE('',*,*,#14148,.F.);
#20337=ORIENTED_EDGE('',*,*,#14149,.T.);
#20338=ORIENTED_EDGE('',*,*,#14150,.T.);
#20339=ORIENTED_EDGE('',*,*,#14151,.T.);
#20340=ORIENTED_EDGE('',*,*,#14152,.T.);
#20341=ORIENTED_EDGE('',*,*,#14153,.T.);
#20342=ORIENTED_EDGE('',*,*,#14154,.F.);
#20343=ORIENTED_EDGE('',*,*,#14155,.T.);
#20344=ORIENTED_EDGE('',*,*,#14156,.F.);
#20345=ORIENTED_EDGE('',*,*,#14157,.T.);
#20346=ORIENTED_EDGE('',*,*,#13957,.T.);
#20347=ORIENTED_EDGE('',*,*,#13962,.T.);
#20348=ORIENTED_EDGE('',*,*,#13959,.T.);
#20349=ORIENTED_EDGE('',*,*,#13964,.T.);
#20350=ORIENTED_EDGE('',*,*,#14158,.T.);
#20351=ORIENTED_EDGE('',*,*,#14159,.T.);
#20352=ORIENTED_EDGE('',*,*,#14156,.T.);
#20353=ORIENTED_EDGE('',*,*,#14160,.T.);
#20354=ORIENTED_EDGE('',*,*,#14159,.F.);
#20355=ORIENTED_EDGE('',*,*,#14161,.F.);
#20356=ORIENTED_EDGE('',*,*,#14162,.T.);
#20357=ORIENTED_EDGE('',*,*,#14157,.F.);
#20358=ORIENTED_EDGE('',*,*,#14163,.T.);
#20359=ORIENTED_EDGE('',*,*,#14164,.T.);
#20360=ORIENTED_EDGE('',*,*,#14154,.T.);
#20361=ORIENTED_EDGE('',*,*,#14165,.T.);
#20362=ORIENTED_EDGE('',*,*,#14160,.F.);
#20363=ORIENTED_EDGE('',*,*,#14155,.F.);
#20364=ORIENTED_EDGE('',*,*,#14164,.F.);
#20365=ORIENTED_EDGE('',*,*,#14166,.F.);
#20366=ORIENTED_EDGE('',*,*,#14167,.T.);
#20367=ORIENTED_EDGE('',*,*,#14168,.T.);
#20368=ORIENTED_EDGE('',*,*,#14148,.T.);
#20369=ORIENTED_EDGE('',*,*,#14169,.T.);
#20370=ORIENTED_EDGE('',*,*,#14168,.F.);
#20371=ORIENTED_EDGE('',*,*,#14170,.F.);
#20372=ORIENTED_EDGE('',*,*,#14171,.T.);
#20373=ORIENTED_EDGE('',*,*,#14149,.F.);
#20374=ORIENTED_EDGE('',*,*,#14172,.T.);
#20375=ORIENTED_EDGE('',*,*,#14173,.T.);
#20376=ORIENTED_EDGE('',*,*,#14146,.T.);
#20377=ORIENTED_EDGE('',*,*,#14174,.T.);
#20378=ORIENTED_EDGE('',*,*,#14169,.F.);
#20379=ORIENTED_EDGE('',*,*,#14147,.F.);
#20380=ORIENTED_EDGE('',*,*,#14173,.F.);
#20381=ORIENTED_EDGE('',*,*,#14175,.F.);
#20382=ORIENTED_EDGE('',*,*,#14176,.T.);
#20383=ORIENTED_EDGE('',*,*,#14177,.T.);
#20384=ORIENTED_EDGE('',*,*,#14140,.T.);
#20385=ORIENTED_EDGE('',*,*,#14178,.T.);
#20386=ORIENTED_EDGE('',*,*,#14177,.F.);
#20387=ORIENTED_EDGE('',*,*,#14179,.F.);
#20388=ORIENTED_EDGE('',*,*,#14180,.T.);
#20389=ORIENTED_EDGE('',*,*,#14141,.F.);
#20390=ORIENTED_EDGE('',*,*,#14181,.T.);
#20391=ORIENTED_EDGE('',*,*,#14182,.T.);
#20392=ORIENTED_EDGE('',*,*,#14138,.T.);
#20393=ORIENTED_EDGE('',*,*,#14183,.T.);
#20394=ORIENTED_EDGE('',*,*,#14178,.F.);
#20395=ORIENTED_EDGE('',*,*,#14139,.F.);
#20396=ORIENTED_EDGE('',*,*,#14182,.F.);
#20397=ORIENTED_EDGE('',*,*,#14184,.F.);
#20398=ORIENTED_EDGE('',*,*,#14185,.T.);
#20399=ORIENTED_EDGE('',*,*,#14186,.T.);
#20400=ORIENTED_EDGE('',*,*,#14132,.T.);
#20401=ORIENTED_EDGE('',*,*,#14187,.T.);
#20402=ORIENTED_EDGE('',*,*,#14186,.F.);
#20403=ORIENTED_EDGE('',*,*,#14188,.F.);
#20404=ORIENTED_EDGE('',*,*,#14189,.T.);
#20405=ORIENTED_EDGE('',*,*,#14133,.F.);
#20406=ORIENTED_EDGE('',*,*,#14190,.T.);
#20407=ORIENTED_EDGE('',*,*,#14191,.T.);
#20408=ORIENTED_EDGE('',*,*,#14130,.T.);
#20409=ORIENTED_EDGE('',*,*,#14192,.T.);
#20410=ORIENTED_EDGE('',*,*,#14187,.F.);
#20411=ORIENTED_EDGE('',*,*,#14131,.F.);
#20412=ORIENTED_EDGE('',*,*,#14191,.F.);
#20413=ORIENTED_EDGE('',*,*,#14193,.F.);
#20414=ORIENTED_EDGE('',*,*,#14194,.T.);
#20415=ORIENTED_EDGE('',*,*,#14195,.T.);
#20416=ORIENTED_EDGE('',*,*,#14124,.T.);
#20417=ORIENTED_EDGE('',*,*,#14196,.T.);
#20418=ORIENTED_EDGE('',*,*,#14195,.F.);
#20419=ORIENTED_EDGE('',*,*,#14197,.F.);
#20420=ORIENTED_EDGE('',*,*,#14198,.T.);
#20421=ORIENTED_EDGE('',*,*,#14125,.F.);
#20422=ORIENTED_EDGE('',*,*,#14199,.T.);
#20423=ORIENTED_EDGE('',*,*,#14200,.T.);
#20424=ORIENTED_EDGE('',*,*,#14122,.T.);
#20425=ORIENTED_EDGE('',*,*,#14201,.T.);
#20426=ORIENTED_EDGE('',*,*,#14196,.F.);
#20427=ORIENTED_EDGE('',*,*,#14123,.F.);
#20428=ORIENTED_EDGE('',*,*,#14200,.F.);
#20429=ORIENTED_EDGE('',*,*,#14202,.F.);
#20430=ORIENTED_EDGE('',*,*,#14203,.T.);
#20431=ORIENTED_EDGE('',*,*,#14204,.T.);
#20432=ORIENTED_EDGE('',*,*,#14116,.T.);
#20433=ORIENTED_EDGE('',*,*,#14205,.T.);
#20434=ORIENTED_EDGE('',*,*,#14204,.F.);
#20435=ORIENTED_EDGE('',*,*,#14206,.F.);
#20436=ORIENTED_EDGE('',*,*,#14207,.T.);
#20437=ORIENTED_EDGE('',*,*,#14117,.F.);
#20438=ORIENTED_EDGE('',*,*,#14208,.T.);
#20439=ORIENTED_EDGE('',*,*,#14209,.T.);
#20440=ORIENTED_EDGE('',*,*,#14114,.T.);
#20441=ORIENTED_EDGE('',*,*,#14210,.T.);
#20442=ORIENTED_EDGE('',*,*,#14205,.F.);
#20443=ORIENTED_EDGE('',*,*,#14115,.F.);
#20444=ORIENTED_EDGE('',*,*,#14209,.F.);
#20445=ORIENTED_EDGE('',*,*,#14211,.F.);
#20446=ORIENTED_EDGE('',*,*,#14212,.T.);
#20447=ORIENTED_EDGE('',*,*,#14213,.T.);
#20448=ORIENTED_EDGE('',*,*,#14108,.T.);
#20449=ORIENTED_EDGE('',*,*,#14214,.T.);
#20450=ORIENTED_EDGE('',*,*,#14213,.F.);
#20451=ORIENTED_EDGE('',*,*,#14215,.F.);
#20452=ORIENTED_EDGE('',*,*,#14216,.T.);
#20453=ORIENTED_EDGE('',*,*,#14109,.F.);
#20454=ORIENTED_EDGE('',*,*,#14217,.T.);
#20455=ORIENTED_EDGE('',*,*,#14218,.T.);
#20456=ORIENTED_EDGE('',*,*,#14106,.T.);
#20457=ORIENTED_EDGE('',*,*,#14219,.T.);
#20458=ORIENTED_EDGE('',*,*,#14214,.F.);
#20459=ORIENTED_EDGE('',*,*,#14107,.F.);
#20460=ORIENTED_EDGE('',*,*,#14218,.F.);
#20461=ORIENTED_EDGE('',*,*,#14220,.F.);
#20462=ORIENTED_EDGE('',*,*,#14221,.T.);
#20463=ORIENTED_EDGE('',*,*,#14222,.T.);
#20464=ORIENTED_EDGE('',*,*,#14100,.T.);
#20465=ORIENTED_EDGE('',*,*,#14223,.T.);
#20466=ORIENTED_EDGE('',*,*,#14222,.F.);
#20467=ORIENTED_EDGE('',*,*,#14224,.F.);
#20468=ORIENTED_EDGE('',*,*,#14225,.T.);
#20469=ORIENTED_EDGE('',*,*,#14101,.F.);
#20470=ORIENTED_EDGE('',*,*,#14226,.T.);
#20471=ORIENTED_EDGE('',*,*,#14227,.T.);
#20472=ORIENTED_EDGE('',*,*,#14098,.T.);
#20473=ORIENTED_EDGE('',*,*,#14228,.T.);
#20474=ORIENTED_EDGE('',*,*,#14223,.F.);
#20475=ORIENTED_EDGE('',*,*,#14099,.F.);
#20476=ORIENTED_EDGE('',*,*,#14227,.F.);
#20477=ORIENTED_EDGE('',*,*,#14229,.F.);
#20478=ORIENTED_EDGE('',*,*,#14230,.T.);
#20479=ORIENTED_EDGE('',*,*,#14231,.T.);
#20480=ORIENTED_EDGE('',*,*,#14092,.T.);
#20481=ORIENTED_EDGE('',*,*,#14232,.T.);
#20482=ORIENTED_EDGE('',*,*,#14231,.F.);
#20483=ORIENTED_EDGE('',*,*,#14233,.F.);
#20484=ORIENTED_EDGE('',*,*,#14234,.T.);
#20485=ORIENTED_EDGE('',*,*,#14093,.F.);
#20486=ORIENTED_EDGE('',*,*,#14235,.T.);
#20487=ORIENTED_EDGE('',*,*,#14236,.T.);
#20488=ORIENTED_EDGE('',*,*,#14090,.T.);
#20489=ORIENTED_EDGE('',*,*,#14237,.T.);
#20490=ORIENTED_EDGE('',*,*,#14232,.F.);
#20491=ORIENTED_EDGE('',*,*,#14091,.F.);
#20492=ORIENTED_EDGE('',*,*,#14236,.F.);
#20493=ORIENTED_EDGE('',*,*,#14238,.F.);
#20494=ORIENTED_EDGE('',*,*,#14239,.T.);
#20495=ORIENTED_EDGE('',*,*,#14240,.T.);
#20496=ORIENTED_EDGE('',*,*,#14084,.T.);
#20497=ORIENTED_EDGE('',*,*,#14241,.T.);
#20498=ORIENTED_EDGE('',*,*,#14240,.F.);
#20499=ORIENTED_EDGE('',*,*,#14242,.F.);
#20500=ORIENTED_EDGE('',*,*,#14243,.T.);
#20501=ORIENTED_EDGE('',*,*,#14085,.F.);
#20502=ORIENTED_EDGE('',*,*,#14244,.T.);
#20503=ORIENTED_EDGE('',*,*,#14245,.T.);
#20504=ORIENTED_EDGE('',*,*,#14082,.T.);
#20505=ORIENTED_EDGE('',*,*,#14246,.T.);
#20506=ORIENTED_EDGE('',*,*,#14241,.F.);
#20507=ORIENTED_EDGE('',*,*,#14083,.F.);
#20508=ORIENTED_EDGE('',*,*,#14245,.F.);
#20509=ORIENTED_EDGE('',*,*,#14247,.F.);
#20510=ORIENTED_EDGE('',*,*,#14248,.T.);
#20511=ORIENTED_EDGE('',*,*,#14249,.T.);
#20512=ORIENTED_EDGE('',*,*,#14076,.T.);
#20513=ORIENTED_EDGE('',*,*,#14250,.T.);
#20514=ORIENTED_EDGE('',*,*,#14249,.F.);
#20515=ORIENTED_EDGE('',*,*,#14251,.F.);
#20516=ORIENTED_EDGE('',*,*,#14252,.T.);
#20517=ORIENTED_EDGE('',*,*,#14077,.F.);
#20518=ORIENTED_EDGE('',*,*,#14253,.T.);
#20519=ORIENTED_EDGE('',*,*,#14254,.T.);
#20520=ORIENTED_EDGE('',*,*,#14074,.T.);
#20521=ORIENTED_EDGE('',*,*,#14255,.T.);
#20522=ORIENTED_EDGE('',*,*,#14250,.F.);
#20523=ORIENTED_EDGE('',*,*,#14075,.F.);
#20524=ORIENTED_EDGE('',*,*,#14254,.F.);
#20525=ORIENTED_EDGE('',*,*,#14256,.F.);
#20526=ORIENTED_EDGE('',*,*,#14257,.T.);
#20527=ORIENTED_EDGE('',*,*,#14258,.T.);
#20528=ORIENTED_EDGE('',*,*,#14068,.T.);
#20529=ORIENTED_EDGE('',*,*,#14259,.T.);
#20530=ORIENTED_EDGE('',*,*,#14258,.F.);
#20531=ORIENTED_EDGE('',*,*,#14260,.F.);
#20532=ORIENTED_EDGE('',*,*,#14261,.T.);
#20533=ORIENTED_EDGE('',*,*,#14069,.F.);
#20534=ORIENTED_EDGE('',*,*,#14262,.T.);
#20535=ORIENTED_EDGE('',*,*,#14263,.T.);
#20536=ORIENTED_EDGE('',*,*,#14066,.T.);
#20537=ORIENTED_EDGE('',*,*,#14264,.T.);
#20538=ORIENTED_EDGE('',*,*,#14259,.F.);
#20539=ORIENTED_EDGE('',*,*,#14067,.F.);
#20540=ORIENTED_EDGE('',*,*,#14263,.F.);
#20541=ORIENTED_EDGE('',*,*,#14265,.F.);
#20542=ORIENTED_EDGE('',*,*,#14266,.T.);
#20543=ORIENTED_EDGE('',*,*,#14267,.T.);
#20544=ORIENTED_EDGE('',*,*,#14060,.T.);
#20545=ORIENTED_EDGE('',*,*,#14268,.T.);
#20546=ORIENTED_EDGE('',*,*,#14267,.F.);
#20547=ORIENTED_EDGE('',*,*,#14269,.F.);
#20548=ORIENTED_EDGE('',*,*,#14270,.T.);
#20549=ORIENTED_EDGE('',*,*,#14061,.F.);
#20550=ORIENTED_EDGE('',*,*,#14271,.T.);
#20551=ORIENTED_EDGE('',*,*,#14272,.T.);
#20552=ORIENTED_EDGE('',*,*,#14058,.T.);
#20553=ORIENTED_EDGE('',*,*,#14273,.T.);
#20554=ORIENTED_EDGE('',*,*,#14268,.F.);
#20555=ORIENTED_EDGE('',*,*,#14059,.F.);
#20556=ORIENTED_EDGE('',*,*,#14272,.F.);
#20557=ORIENTED_EDGE('',*,*,#14274,.F.);
#20558=ORIENTED_EDGE('',*,*,#14275,.T.);
#20559=ORIENTED_EDGE('',*,*,#14276,.T.);
#20560=ORIENTED_EDGE('',*,*,#14052,.T.);
#20561=ORIENTED_EDGE('',*,*,#14277,.T.);
#20562=ORIENTED_EDGE('',*,*,#14276,.F.);
#20563=ORIENTED_EDGE('',*,*,#14278,.F.);
#20564=ORIENTED_EDGE('',*,*,#14279,.T.);
#20565=ORIENTED_EDGE('',*,*,#14053,.F.);
#20566=ORIENTED_EDGE('',*,*,#14280,.T.);
#20567=ORIENTED_EDGE('',*,*,#14281,.T.);
#20568=ORIENTED_EDGE('',*,*,#14050,.T.);
#20569=ORIENTED_EDGE('',*,*,#14282,.T.);
#20570=ORIENTED_EDGE('',*,*,#14277,.F.);
#20571=ORIENTED_EDGE('',*,*,#14051,.F.);
#20572=ORIENTED_EDGE('',*,*,#14281,.F.);
#20573=ORIENTED_EDGE('',*,*,#14283,.F.);
#20574=ORIENTED_EDGE('',*,*,#14284,.T.);
#20575=ORIENTED_EDGE('',*,*,#14285,.T.);
#20576=ORIENTED_EDGE('',*,*,#14044,.T.);
#20577=ORIENTED_EDGE('',*,*,#14286,.T.);
#20578=ORIENTED_EDGE('',*,*,#14285,.F.);
#20579=ORIENTED_EDGE('',*,*,#14287,.F.);
#20580=ORIENTED_EDGE('',*,*,#14288,.T.);
#20581=ORIENTED_EDGE('',*,*,#14045,.F.);
#20582=ORIENTED_EDGE('',*,*,#14289,.T.);
#20583=ORIENTED_EDGE('',*,*,#14290,.T.);
#20584=ORIENTED_EDGE('',*,*,#14042,.T.);
#20585=ORIENTED_EDGE('',*,*,#14291,.T.);
#20586=ORIENTED_EDGE('',*,*,#14286,.F.);
#20587=ORIENTED_EDGE('',*,*,#14043,.F.);
#20588=ORIENTED_EDGE('',*,*,#14290,.F.);
#20589=ORIENTED_EDGE('',*,*,#14292,.F.);
#20590=ORIENTED_EDGE('',*,*,#14293,.T.);
#20591=ORIENTED_EDGE('',*,*,#14294,.T.);
#20592=ORIENTED_EDGE('',*,*,#14036,.T.);
#20593=ORIENTED_EDGE('',*,*,#14295,.T.);
#20594=ORIENTED_EDGE('',*,*,#14294,.F.);
#20595=ORIENTED_EDGE('',*,*,#14296,.F.);
#20596=ORIENTED_EDGE('',*,*,#14297,.T.);
#20597=ORIENTED_EDGE('',*,*,#14037,.F.);
#20598=ORIENTED_EDGE('',*,*,#14298,.T.);
#20599=ORIENTED_EDGE('',*,*,#14299,.T.);
#20600=ORIENTED_EDGE('',*,*,#14034,.T.);
#20601=ORIENTED_EDGE('',*,*,#14300,.T.);
#20602=ORIENTED_EDGE('',*,*,#14295,.F.);
#20603=ORIENTED_EDGE('',*,*,#14035,.F.);
#20604=ORIENTED_EDGE('',*,*,#14299,.F.);
#20605=ORIENTED_EDGE('',*,*,#14301,.F.);
#20606=ORIENTED_EDGE('',*,*,#14302,.T.);
#20607=ORIENTED_EDGE('',*,*,#14303,.T.);
#20608=ORIENTED_EDGE('',*,*,#14028,.T.);
#20609=ORIENTED_EDGE('',*,*,#14304,.T.);
#20610=ORIENTED_EDGE('',*,*,#14303,.F.);
#20611=ORIENTED_EDGE('',*,*,#14305,.F.);
#20612=ORIENTED_EDGE('',*,*,#14306,.T.);
#20613=ORIENTED_EDGE('',*,*,#14029,.F.);
#20614=ORIENTED_EDGE('',*,*,#14307,.T.);
#20615=ORIENTED_EDGE('',*,*,#14308,.T.);
#20616=ORIENTED_EDGE('',*,*,#14026,.T.);
#20617=ORIENTED_EDGE('',*,*,#14309,.T.);
#20618=ORIENTED_EDGE('',*,*,#14304,.F.);
#20619=ORIENTED_EDGE('',*,*,#14027,.F.);
#20620=ORIENTED_EDGE('',*,*,#14308,.F.);
#20621=ORIENTED_EDGE('',*,*,#14310,.F.);
#20622=ORIENTED_EDGE('',*,*,#14311,.T.);
#20623=ORIENTED_EDGE('',*,*,#14312,.T.);
#20624=ORIENTED_EDGE('',*,*,#14020,.T.);
#20625=ORIENTED_EDGE('',*,*,#14313,.T.);
#20626=ORIENTED_EDGE('',*,*,#14312,.F.);
#20627=ORIENTED_EDGE('',*,*,#14314,.F.);
#20628=ORIENTED_EDGE('',*,*,#14315,.T.);
#20629=ORIENTED_EDGE('',*,*,#14021,.F.);
#20630=ORIENTED_EDGE('',*,*,#14316,.T.);
#20631=ORIENTED_EDGE('',*,*,#14317,.T.);
#20632=ORIENTED_EDGE('',*,*,#14018,.T.);
#20633=ORIENTED_EDGE('',*,*,#14318,.T.);
#20634=ORIENTED_EDGE('',*,*,#14313,.F.);
#20635=ORIENTED_EDGE('',*,*,#14019,.F.);
#20636=ORIENTED_EDGE('',*,*,#14317,.F.);
#20637=ORIENTED_EDGE('',*,*,#14319,.F.);
#20638=ORIENTED_EDGE('',*,*,#14320,.T.);
#20639=ORIENTED_EDGE('',*,*,#14321,.T.);
#20640=ORIENTED_EDGE('',*,*,#14012,.T.);
#20641=ORIENTED_EDGE('',*,*,#14322,.T.);
#20642=ORIENTED_EDGE('',*,*,#14321,.F.);
#20643=ORIENTED_EDGE('',*,*,#14323,.F.);
#20644=ORIENTED_EDGE('',*,*,#14324,.T.);
#20645=ORIENTED_EDGE('',*,*,#14013,.F.);
#20646=ORIENTED_EDGE('',*,*,#14325,.T.);
#20647=ORIENTED_EDGE('',*,*,#14326,.T.);
#20648=ORIENTED_EDGE('',*,*,#14010,.T.);
#20649=ORIENTED_EDGE('',*,*,#14327,.T.);
#20650=ORIENTED_EDGE('',*,*,#14322,.F.);
#20651=ORIENTED_EDGE('',*,*,#14011,.F.);
#20652=ORIENTED_EDGE('',*,*,#14326,.F.);
#20653=ORIENTED_EDGE('',*,*,#14328,.F.);
#20654=ORIENTED_EDGE('',*,*,#14329,.T.);
#20655=ORIENTED_EDGE('',*,*,#14330,.T.);
#20656=ORIENTED_EDGE('',*,*,#14004,.T.);
#20657=ORIENTED_EDGE('',*,*,#14331,.T.);
#20658=ORIENTED_EDGE('',*,*,#14330,.F.);
#20659=ORIENTED_EDGE('',*,*,#14332,.F.);
#20660=ORIENTED_EDGE('',*,*,#14333,.T.);
#20661=ORIENTED_EDGE('',*,*,#14005,.F.);
#20662=ORIENTED_EDGE('',*,*,#14334,.T.);
#20663=ORIENTED_EDGE('',*,*,#14335,.T.);
#20664=ORIENTED_EDGE('',*,*,#14002,.T.);
#20665=ORIENTED_EDGE('',*,*,#14336,.T.);
#20666=ORIENTED_EDGE('',*,*,#14331,.F.);
#20667=ORIENTED_EDGE('',*,*,#14003,.F.);
#20668=ORIENTED_EDGE('',*,*,#14335,.F.);
#20669=ORIENTED_EDGE('',*,*,#14337,.F.);
#20670=ORIENTED_EDGE('',*,*,#14338,.T.);
#20671=ORIENTED_EDGE('',*,*,#14339,.T.);
#20672=ORIENTED_EDGE('',*,*,#13996,.T.);
#20673=ORIENTED_EDGE('',*,*,#14340,.T.);
#20674=ORIENTED_EDGE('',*,*,#14339,.F.);
#20675=ORIENTED_EDGE('',*,*,#14341,.F.);
#20676=ORIENTED_EDGE('',*,*,#14342,.T.);
#20677=ORIENTED_EDGE('',*,*,#13997,.F.);
#20678=ORIENTED_EDGE('',*,*,#14343,.T.);
#20679=ORIENTED_EDGE('',*,*,#14344,.T.);
#20680=ORIENTED_EDGE('',*,*,#13994,.T.);
#20681=ORIENTED_EDGE('',*,*,#14345,.T.);
#20682=ORIENTED_EDGE('',*,*,#14340,.F.);
#20683=ORIENTED_EDGE('',*,*,#13995,.F.);
#20684=ORIENTED_EDGE('',*,*,#14344,.F.);
#20685=ORIENTED_EDGE('',*,*,#14346,.F.);
#20686=ORIENTED_EDGE('',*,*,#14347,.T.);
#20687=ORIENTED_EDGE('',*,*,#14348,.T.);
#20688=ORIENTED_EDGE('',*,*,#13988,.T.);
#20689=ORIENTED_EDGE('',*,*,#14349,.T.);
#20690=ORIENTED_EDGE('',*,*,#14348,.F.);
#20691=ORIENTED_EDGE('',*,*,#14350,.F.);
#20692=ORIENTED_EDGE('',*,*,#14351,.T.);
#20693=ORIENTED_EDGE('',*,*,#13989,.F.);
#20694=ORIENTED_EDGE('',*,*,#14352,.T.);
#20695=ORIENTED_EDGE('',*,*,#14353,.T.);
#20696=ORIENTED_EDGE('',*,*,#13986,.T.);
#20697=ORIENTED_EDGE('',*,*,#14354,.T.);
#20698=ORIENTED_EDGE('',*,*,#14349,.F.);
#20699=ORIENTED_EDGE('',*,*,#13987,.F.);
#20700=ORIENTED_EDGE('',*,*,#14353,.F.);
#20701=ORIENTED_EDGE('',*,*,#14355,.F.);
#20702=ORIENTED_EDGE('',*,*,#14356,.T.);
#20703=ORIENTED_EDGE('',*,*,#14357,.T.);
#20704=ORIENTED_EDGE('',*,*,#13980,.T.);
#20705=ORIENTED_EDGE('',*,*,#14358,.T.);
#20706=ORIENTED_EDGE('',*,*,#14357,.F.);
#20707=ORIENTED_EDGE('',*,*,#14359,.F.);
#20708=ORIENTED_EDGE('',*,*,#14360,.T.);
#20709=ORIENTED_EDGE('',*,*,#13981,.F.);
#20710=ORIENTED_EDGE('',*,*,#14361,.T.);
#20711=ORIENTED_EDGE('',*,*,#14362,.T.);
#20712=ORIENTED_EDGE('',*,*,#13978,.T.);
#20713=ORIENTED_EDGE('',*,*,#14363,.T.);
#20714=ORIENTED_EDGE('',*,*,#14358,.F.);
#20715=ORIENTED_EDGE('',*,*,#13979,.F.);
#20716=ORIENTED_EDGE('',*,*,#14362,.F.);
#20717=ORIENTED_EDGE('',*,*,#14364,.F.);
#20718=ORIENTED_EDGE('',*,*,#14165,.F.);
#20719=ORIENTED_EDGE('',*,*,#14153,.F.);
#20720=ORIENTED_EDGE('',*,*,#14365,.F.);
#20721=ORIENTED_EDGE('',*,*,#14366,.F.);
#20722=ORIENTED_EDGE('',*,*,#14367,.F.);
#20723=ORIENTED_EDGE('',*,*,#14368,.F.);
#20724=ORIENTED_EDGE('',*,*,#13966,.F.);
#20725=ORIENTED_EDGE('',*,*,#14162,.F.);
#20726=ORIENTED_EDGE('',*,*,#14369,.F.);
#20727=ORIENTED_EDGE('',*,*,#14365,.T.);
#20728=ORIENTED_EDGE('',*,*,#14152,.F.);
#20729=ORIENTED_EDGE('',*,*,#14370,.F.);
#20730=ORIENTED_EDGE('',*,*,#14174,.F.);
#20731=ORIENTED_EDGE('',*,*,#14145,.F.);
#20732=ORIENTED_EDGE('',*,*,#14371,.F.);
#20733=ORIENTED_EDGE('',*,*,#14372,.F.);
#20734=ORIENTED_EDGE('',*,*,#14373,.F.);
#20735=ORIENTED_EDGE('',*,*,#14374,.F.);
#20736=ORIENTED_EDGE('',*,*,#14150,.F.);
#20737=ORIENTED_EDGE('',*,*,#14171,.F.);
#20738=ORIENTED_EDGE('',*,*,#14375,.F.);
#20739=ORIENTED_EDGE('',*,*,#14371,.T.);
#20740=ORIENTED_EDGE('',*,*,#14144,.F.);
#20741=ORIENTED_EDGE('',*,*,#14376,.F.);
#20742=ORIENTED_EDGE('',*,*,#14183,.F.);
#20743=ORIENTED_EDGE('',*,*,#14137,.F.);
#20744=ORIENTED_EDGE('',*,*,#14377,.F.);
#20745=ORIENTED_EDGE('',*,*,#14378,.F.);
#20746=ORIENTED_EDGE('',*,*,#14379,.F.);
#20747=ORIENTED_EDGE('',*,*,#14380,.F.);
#20748=ORIENTED_EDGE('',*,*,#14142,.F.);
#20749=ORIENTED_EDGE('',*,*,#14180,.F.);
#20750=ORIENTED_EDGE('',*,*,#14381,.F.);
#20751=ORIENTED_EDGE('',*,*,#14377,.T.);
#20752=ORIENTED_EDGE('',*,*,#14136,.F.);
#20753=ORIENTED_EDGE('',*,*,#14382,.F.);
#20754=ORIENTED_EDGE('',*,*,#14192,.F.);
#20755=ORIENTED_EDGE('',*,*,#14129,.F.);
#20756=ORIENTED_EDGE('',*,*,#14383,.F.);
#20757=ORIENTED_EDGE('',*,*,#14384,.F.);
#20758=ORIENTED_EDGE('',*,*,#14385,.F.);
#20759=ORIENTED_EDGE('',*,*,#14386,.F.);
#20760=ORIENTED_EDGE('',*,*,#14134,.F.);
#20761=ORIENTED_EDGE('',*,*,#14189,.F.);
#20762=ORIENTED_EDGE('',*,*,#14387,.F.);
#20763=ORIENTED_EDGE('',*,*,#14383,.T.);
#20764=ORIENTED_EDGE('',*,*,#14128,.F.);
#20765=ORIENTED_EDGE('',*,*,#14388,.F.);
#20766=ORIENTED_EDGE('',*,*,#14201,.F.);
#20767=ORIENTED_EDGE('',*,*,#14121,.F.);
#20768=ORIENTED_EDGE('',*,*,#14389,.F.);
#20769=ORIENTED_EDGE('',*,*,#14390,.F.);
#20770=ORIENTED_EDGE('',*,*,#14391,.F.);
#20771=ORIENTED_EDGE('',*,*,#14392,.F.);
#20772=ORIENTED_EDGE('',*,*,#14126,.F.);
#20773=ORIENTED_EDGE('',*,*,#14198,.F.);
#20774=ORIENTED_EDGE('',*,*,#14393,.F.);
#20775=ORIENTED_EDGE('',*,*,#14389,.T.);
#20776=ORIENTED_EDGE('',*,*,#14120,.F.);
#20777=ORIENTED_EDGE('',*,*,#14394,.F.);
#20778=ORIENTED_EDGE('',*,*,#14210,.F.);
#20779=ORIENTED_EDGE('',*,*,#14113,.F.);
#20780=ORIENTED_EDGE('',*,*,#14395,.F.);
#20781=ORIENTED_EDGE('',*,*,#14396,.F.);
#20782=ORIENTED_EDGE('',*,*,#14397,.F.);
#20783=ORIENTED_EDGE('',*,*,#14398,.F.);
#20784=ORIENTED_EDGE('',*,*,#14118,.F.);
#20785=ORIENTED_EDGE('',*,*,#14207,.F.);
#20786=ORIENTED_EDGE('',*,*,#14399,.F.);
#20787=ORIENTED_EDGE('',*,*,#14395,.T.);
#20788=ORIENTED_EDGE('',*,*,#14112,.F.);
#20789=ORIENTED_EDGE('',*,*,#14400,.F.);
#20790=ORIENTED_EDGE('',*,*,#14219,.F.);
#20791=ORIENTED_EDGE('',*,*,#14105,.F.);
#20792=ORIENTED_EDGE('',*,*,#14401,.F.);
#20793=ORIENTED_EDGE('',*,*,#14402,.F.);
#20794=ORIENTED_EDGE('',*,*,#14403,.F.);
#20795=ORIENTED_EDGE('',*,*,#14404,.F.);
#20796=ORIENTED_EDGE('',*,*,#14110,.F.);
#20797=ORIENTED_EDGE('',*,*,#14216,.F.);
#20798=ORIENTED_EDGE('',*,*,#14405,.F.);
#20799=ORIENTED_EDGE('',*,*,#14401,.T.);
#20800=ORIENTED_EDGE('',*,*,#14104,.F.);
#20801=ORIENTED_EDGE('',*,*,#14406,.F.);
#20802=ORIENTED_EDGE('',*,*,#14228,.F.);
#20803=ORIENTED_EDGE('',*,*,#14097,.F.);
#20804=ORIENTED_EDGE('',*,*,#14407,.F.);
#20805=ORIENTED_EDGE('',*,*,#14408,.F.);
#20806=ORIENTED_EDGE('',*,*,#14409,.F.);
#20807=ORIENTED_EDGE('',*,*,#14410,.F.);
#20808=ORIENTED_EDGE('',*,*,#14102,.F.);
#20809=ORIENTED_EDGE('',*,*,#14225,.F.);
#20810=ORIENTED_EDGE('',*,*,#14411,.F.);
#20811=ORIENTED_EDGE('',*,*,#14407,.T.);
#20812=ORIENTED_EDGE('',*,*,#14096,.F.);
#20813=ORIENTED_EDGE('',*,*,#14412,.F.);
#20814=ORIENTED_EDGE('',*,*,#14237,.F.);
#20815=ORIENTED_EDGE('',*,*,#14089,.F.);
#20816=ORIENTED_EDGE('',*,*,#14413,.F.);
#20817=ORIENTED_EDGE('',*,*,#14414,.F.);
#20818=ORIENTED_EDGE('',*,*,#14415,.F.);
#20819=ORIENTED_EDGE('',*,*,#14416,.F.);
#20820=ORIENTED_EDGE('',*,*,#14094,.F.);
#20821=ORIENTED_EDGE('',*,*,#14234,.F.);
#20822=ORIENTED_EDGE('',*,*,#14417,.F.);
#20823=ORIENTED_EDGE('',*,*,#14413,.T.);
#20824=ORIENTED_EDGE('',*,*,#14088,.F.);
#20825=ORIENTED_EDGE('',*,*,#14418,.F.);
#20826=ORIENTED_EDGE('',*,*,#14246,.F.);
#20827=ORIENTED_EDGE('',*,*,#14081,.F.);
#20828=ORIENTED_EDGE('',*,*,#14419,.F.);
#20829=ORIENTED_EDGE('',*,*,#14420,.F.);
#20830=ORIENTED_EDGE('',*,*,#14421,.F.);
#20831=ORIENTED_EDGE('',*,*,#14422,.F.);
#20832=ORIENTED_EDGE('',*,*,#14086,.F.);
#20833=ORIENTED_EDGE('',*,*,#14243,.F.);
#20834=ORIENTED_EDGE('',*,*,#14423,.F.);
#20835=ORIENTED_EDGE('',*,*,#14419,.T.);
#20836=ORIENTED_EDGE('',*,*,#14080,.F.);
#20837=ORIENTED_EDGE('',*,*,#14424,.F.);
#20838=ORIENTED_EDGE('',*,*,#14255,.F.);
#20839=ORIENTED_EDGE('',*,*,#14073,.F.);
#20840=ORIENTED_EDGE('',*,*,#14425,.F.);
#20841=ORIENTED_EDGE('',*,*,#14426,.F.);
#20842=ORIENTED_EDGE('',*,*,#14427,.F.);
#20843=ORIENTED_EDGE('',*,*,#14428,.F.);
#20844=ORIENTED_EDGE('',*,*,#14078,.F.);
#20845=ORIENTED_EDGE('',*,*,#14252,.F.);
#20846=ORIENTED_EDGE('',*,*,#14429,.F.);
#20847=ORIENTED_EDGE('',*,*,#14425,.T.);
#20848=ORIENTED_EDGE('',*,*,#14072,.F.);
#20849=ORIENTED_EDGE('',*,*,#14430,.F.);
#20850=ORIENTED_EDGE('',*,*,#14264,.F.);
#20851=ORIENTED_EDGE('',*,*,#14065,.F.);
#20852=ORIENTED_EDGE('',*,*,#14431,.F.);
#20853=ORIENTED_EDGE('',*,*,#14432,.F.);
#20854=ORIENTED_EDGE('',*,*,#14433,.F.);
#20855=ORIENTED_EDGE('',*,*,#14434,.F.);
#20856=ORIENTED_EDGE('',*,*,#14070,.F.);
#20857=ORIENTED_EDGE('',*,*,#14261,.F.);
#20858=ORIENTED_EDGE('',*,*,#14435,.F.);
#20859=ORIENTED_EDGE('',*,*,#14431,.T.);
#20860=ORIENTED_EDGE('',*,*,#14064,.F.);
#20861=ORIENTED_EDGE('',*,*,#14436,.F.);
#20862=ORIENTED_EDGE('',*,*,#14273,.F.);
#20863=ORIENTED_EDGE('',*,*,#14057,.F.);
#20864=ORIENTED_EDGE('',*,*,#14437,.F.);
#20865=ORIENTED_EDGE('',*,*,#14438,.F.);
#20866=ORIENTED_EDGE('',*,*,#14439,.F.);
#20867=ORIENTED_EDGE('',*,*,#14440,.F.);
#20868=ORIENTED_EDGE('',*,*,#14062,.F.);
#20869=ORIENTED_EDGE('',*,*,#14270,.F.);
#20870=ORIENTED_EDGE('',*,*,#14441,.F.);
#20871=ORIENTED_EDGE('',*,*,#14437,.T.);
#20872=ORIENTED_EDGE('',*,*,#14056,.F.);
#20873=ORIENTED_EDGE('',*,*,#14442,.F.);
#20874=ORIENTED_EDGE('',*,*,#14282,.F.);
#20875=ORIENTED_EDGE('',*,*,#14049,.F.);
#20876=ORIENTED_EDGE('',*,*,#14443,.F.);
#20877=ORIENTED_EDGE('',*,*,#14444,.F.);
#20878=ORIENTED_EDGE('',*,*,#14445,.F.);
#20879=ORIENTED_EDGE('',*,*,#14446,.F.);
#20880=ORIENTED_EDGE('',*,*,#14054,.F.);
#20881=ORIENTED_EDGE('',*,*,#14279,.F.);
#20882=ORIENTED_EDGE('',*,*,#14447,.F.);
#20883=ORIENTED_EDGE('',*,*,#14443,.T.);
#20884=ORIENTED_EDGE('',*,*,#14048,.F.);
#20885=ORIENTED_EDGE('',*,*,#14448,.F.);
#20886=ORIENTED_EDGE('',*,*,#14291,.F.);
#20887=ORIENTED_EDGE('',*,*,#14041,.F.);
#20888=ORIENTED_EDGE('',*,*,#14449,.F.);
#20889=ORIENTED_EDGE('',*,*,#14450,.F.);
#20890=ORIENTED_EDGE('',*,*,#14451,.F.);
#20891=ORIENTED_EDGE('',*,*,#14452,.F.);
#20892=ORIENTED_EDGE('',*,*,#14046,.F.);
#20893=ORIENTED_EDGE('',*,*,#14288,.F.);
#20894=ORIENTED_EDGE('',*,*,#14453,.F.);
#20895=ORIENTED_EDGE('',*,*,#14449,.T.);
#20896=ORIENTED_EDGE('',*,*,#14040,.F.);
#20897=ORIENTED_EDGE('',*,*,#14454,.F.);
#20898=ORIENTED_EDGE('',*,*,#14300,.F.);
#20899=ORIENTED_EDGE('',*,*,#14033,.F.);
#20900=ORIENTED_EDGE('',*,*,#14455,.F.);
#20901=ORIENTED_EDGE('',*,*,#14456,.F.);
#20902=ORIENTED_EDGE('',*,*,#14457,.F.);
#20903=ORIENTED_EDGE('',*,*,#14458,.F.);
#20904=ORIENTED_EDGE('',*,*,#14038,.F.);
#20905=ORIENTED_EDGE('',*,*,#14297,.F.);
#20906=ORIENTED_EDGE('',*,*,#14459,.F.);
#20907=ORIENTED_EDGE('',*,*,#14455,.T.);
#20908=ORIENTED_EDGE('',*,*,#14032,.F.);
#20909=ORIENTED_EDGE('',*,*,#14460,.F.);
#20910=ORIENTED_EDGE('',*,*,#14309,.F.);
#20911=ORIENTED_EDGE('',*,*,#14025,.F.);
#20912=ORIENTED_EDGE('',*,*,#14461,.F.);
#20913=ORIENTED_EDGE('',*,*,#14462,.F.);
#20914=ORIENTED_EDGE('',*,*,#14463,.F.);
#20915=ORIENTED_EDGE('',*,*,#14464,.F.);
#20916=ORIENTED_EDGE('',*,*,#14030,.F.);
#20917=ORIENTED_EDGE('',*,*,#14306,.F.);
#20918=ORIENTED_EDGE('',*,*,#14465,.F.);
#20919=ORIENTED_EDGE('',*,*,#14461,.T.);
#20920=ORIENTED_EDGE('',*,*,#14024,.F.);
#20921=ORIENTED_EDGE('',*,*,#14466,.F.);
#20922=ORIENTED_EDGE('',*,*,#14318,.F.);
#20923=ORIENTED_EDGE('',*,*,#14017,.F.);
#20924=ORIENTED_EDGE('',*,*,#14467,.F.);
#20925=ORIENTED_EDGE('',*,*,#14468,.F.);
#20926=ORIENTED_EDGE('',*,*,#14469,.F.);
#20927=ORIENTED_EDGE('',*,*,#14470,.F.);
#20928=ORIENTED_EDGE('',*,*,#14022,.F.);
#20929=ORIENTED_EDGE('',*,*,#14315,.F.);
#20930=ORIENTED_EDGE('',*,*,#14471,.F.);
#20931=ORIENTED_EDGE('',*,*,#14467,.T.);
#20932=ORIENTED_EDGE('',*,*,#14016,.F.);
#20933=ORIENTED_EDGE('',*,*,#14472,.F.);
#20934=ORIENTED_EDGE('',*,*,#14327,.F.);
#20935=ORIENTED_EDGE('',*,*,#14009,.F.);
#20936=ORIENTED_EDGE('',*,*,#14473,.F.);
#20937=ORIENTED_EDGE('',*,*,#14474,.F.);
#20938=ORIENTED_EDGE('',*,*,#14475,.F.);
#20939=ORIENTED_EDGE('',*,*,#14476,.F.);
#20940=ORIENTED_EDGE('',*,*,#14014,.F.);
#20941=ORIENTED_EDGE('',*,*,#14324,.F.);
#20942=ORIENTED_EDGE('',*,*,#14477,.F.);
#20943=ORIENTED_EDGE('',*,*,#14473,.T.);
#20944=ORIENTED_EDGE('',*,*,#14008,.F.);
#20945=ORIENTED_EDGE('',*,*,#14478,.F.);
#20946=ORIENTED_EDGE('',*,*,#14336,.F.);
#20947=ORIENTED_EDGE('',*,*,#14001,.F.);
#20948=ORIENTED_EDGE('',*,*,#14479,.F.);
#20949=ORIENTED_EDGE('',*,*,#14480,.F.);
#20950=ORIENTED_EDGE('',*,*,#14481,.F.);
#20951=ORIENTED_EDGE('',*,*,#14482,.F.);
#20952=ORIENTED_EDGE('',*,*,#14006,.F.);
#20953=ORIENTED_EDGE('',*,*,#14333,.F.);
#20954=ORIENTED_EDGE('',*,*,#14483,.F.);
#20955=ORIENTED_EDGE('',*,*,#14479,.T.);
#20956=ORIENTED_EDGE('',*,*,#14000,.F.);
#20957=ORIENTED_EDGE('',*,*,#14484,.F.);
#20958=ORIENTED_EDGE('',*,*,#14345,.F.);
#20959=ORIENTED_EDGE('',*,*,#13993,.F.);
#20960=ORIENTED_EDGE('',*,*,#14485,.F.);
#20961=ORIENTED_EDGE('',*,*,#14486,.F.);
#20962=ORIENTED_EDGE('',*,*,#14487,.F.);
#20963=ORIENTED_EDGE('',*,*,#14488,.F.);
#20964=ORIENTED_EDGE('',*,*,#13998,.F.);
#20965=ORIENTED_EDGE('',*,*,#14342,.F.);
#20966=ORIENTED_EDGE('',*,*,#14489,.F.);
#20967=ORIENTED_EDGE('',*,*,#14485,.T.);
#20968=ORIENTED_EDGE('',*,*,#13992,.F.);
#20969=ORIENTED_EDGE('',*,*,#14490,.F.);
#20970=ORIENTED_EDGE('',*,*,#14354,.F.);
#20971=ORIENTED_EDGE('',*,*,#13985,.F.);
#20972=ORIENTED_EDGE('',*,*,#14491,.F.);
#20973=ORIENTED_EDGE('',*,*,#14492,.F.);
#20974=ORIENTED_EDGE('',*,*,#14493,.F.);
#20975=ORIENTED_EDGE('',*,*,#14494,.F.);
#20976=ORIENTED_EDGE('',*,*,#13990,.F.);
#20977=ORIENTED_EDGE('',*,*,#14351,.F.);
#20978=ORIENTED_EDGE('',*,*,#14495,.F.);
#20979=ORIENTED_EDGE('',*,*,#14491,.T.);
#20980=ORIENTED_EDGE('',*,*,#13984,.F.);
#20981=ORIENTED_EDGE('',*,*,#14496,.F.);
#20982=ORIENTED_EDGE('',*,*,#14363,.F.);
#20983=ORIENTED_EDGE('',*,*,#13977,.F.);
#20984=ORIENTED_EDGE('',*,*,#14497,.F.);
#20985=ORIENTED_EDGE('',*,*,#14498,.F.);
#20986=ORIENTED_EDGE('',*,*,#14499,.F.);
#20987=ORIENTED_EDGE('',*,*,#14500,.F.);
#20988=ORIENTED_EDGE('',*,*,#13982,.F.);
#20989=ORIENTED_EDGE('',*,*,#14360,.F.);
#20990=ORIENTED_EDGE('',*,*,#14501,.F.);
#20991=ORIENTED_EDGE('',*,*,#14497,.T.);
#20992=ORIENTED_EDGE('',*,*,#13976,.F.);
#20993=ORIENTED_EDGE('',*,*,#14502,.F.);
#20994=ORIENTED_EDGE('',*,*,#14367,.T.);
#20995=ORIENTED_EDGE('',*,*,#14161,.T.);
#20996=ORIENTED_EDGE('',*,*,#14158,.F.);
#20997=ORIENTED_EDGE('',*,*,#14166,.T.);
#20998=ORIENTED_EDGE('',*,*,#14163,.F.);
#20999=ORIENTED_EDGE('',*,*,#14366,.T.);
#21000=ORIENTED_EDGE('',*,*,#14369,.T.);
#21001=ORIENTED_EDGE('',*,*,#14503,.F.);
#21002=ORIENTED_EDGE('',*,*,#14373,.T.);
#21003=ORIENTED_EDGE('',*,*,#14170,.T.);
#21004=ORIENTED_EDGE('',*,*,#14167,.F.);
#21005=ORIENTED_EDGE('',*,*,#14175,.T.);
#21006=ORIENTED_EDGE('',*,*,#14172,.F.);
#21007=ORIENTED_EDGE('',*,*,#14372,.T.);
#21008=ORIENTED_EDGE('',*,*,#14375,.T.);
#21009=ORIENTED_EDGE('',*,*,#14504,.F.);
#21010=ORIENTED_EDGE('',*,*,#14379,.T.);
#21011=ORIENTED_EDGE('',*,*,#14179,.T.);
#21012=ORIENTED_EDGE('',*,*,#14176,.F.);
#21013=ORIENTED_EDGE('',*,*,#14184,.T.);
#21014=ORIENTED_EDGE('',*,*,#14181,.F.);
#21015=ORIENTED_EDGE('',*,*,#14378,.T.);
#21016=ORIENTED_EDGE('',*,*,#14381,.T.);
#21017=ORIENTED_EDGE('',*,*,#14505,.F.);
#21018=ORIENTED_EDGE('',*,*,#14385,.T.);
#21019=ORIENTED_EDGE('',*,*,#14188,.T.);
#21020=ORIENTED_EDGE('',*,*,#14185,.F.);
#21021=ORIENTED_EDGE('',*,*,#14193,.T.);
#21022=ORIENTED_EDGE('',*,*,#14190,.F.);
#21023=ORIENTED_EDGE('',*,*,#14384,.T.);
#21024=ORIENTED_EDGE('',*,*,#14387,.T.);
#21025=ORIENTED_EDGE('',*,*,#14506,.F.);
#21026=ORIENTED_EDGE('',*,*,#14391,.T.);
#21027=ORIENTED_EDGE('',*,*,#14197,.T.);
#21028=ORIENTED_EDGE('',*,*,#14194,.F.);
#21029=ORIENTED_EDGE('',*,*,#14202,.T.);
#21030=ORIENTED_EDGE('',*,*,#14199,.F.);
#21031=ORIENTED_EDGE('',*,*,#14390,.T.);
#21032=ORIENTED_EDGE('',*,*,#14393,.T.);
#21033=ORIENTED_EDGE('',*,*,#14507,.F.);
#21034=ORIENTED_EDGE('',*,*,#14397,.T.);
#21035=ORIENTED_EDGE('',*,*,#14206,.T.);
#21036=ORIENTED_EDGE('',*,*,#14203,.F.);
#21037=ORIENTED_EDGE('',*,*,#14211,.T.);
#21038=ORIENTED_EDGE('',*,*,#14208,.F.);
#21039=ORIENTED_EDGE('',*,*,#14396,.T.);
#21040=ORIENTED_EDGE('',*,*,#14399,.T.);
#21041=ORIENTED_EDGE('',*,*,#14508,.F.);
#21042=ORIENTED_EDGE('',*,*,#14403,.T.);
#21043=ORIENTED_EDGE('',*,*,#14215,.T.);
#21044=ORIENTED_EDGE('',*,*,#14212,.F.);
#21045=ORIENTED_EDGE('',*,*,#14220,.T.);
#21046=ORIENTED_EDGE('',*,*,#14217,.F.);
#21047=ORIENTED_EDGE('',*,*,#14402,.T.);
#21048=ORIENTED_EDGE('',*,*,#14405,.T.);
#21049=ORIENTED_EDGE('',*,*,#14509,.F.);
#21050=ORIENTED_EDGE('',*,*,#14409,.T.);
#21051=ORIENTED_EDGE('',*,*,#14224,.T.);
#21052=ORIENTED_EDGE('',*,*,#14221,.F.);
#21053=ORIENTED_EDGE('',*,*,#14229,.T.);
#21054=ORIENTED_EDGE('',*,*,#14226,.F.);
#21055=ORIENTED_EDGE('',*,*,#14408,.T.);
#21056=ORIENTED_EDGE('',*,*,#14411,.T.);
#21057=ORIENTED_EDGE('',*,*,#14510,.F.);
#21058=ORIENTED_EDGE('',*,*,#14415,.T.);
#21059=ORIENTED_EDGE('',*,*,#14233,.T.);
#21060=ORIENTED_EDGE('',*,*,#14230,.F.);
#21061=ORIENTED_EDGE('',*,*,#14238,.T.);
#21062=ORIENTED_EDGE('',*,*,#14235,.F.);
#21063=ORIENTED_EDGE('',*,*,#14414,.T.);
#21064=ORIENTED_EDGE('',*,*,#14417,.T.);
#21065=ORIENTED_EDGE('',*,*,#14511,.F.);
#21066=ORIENTED_EDGE('',*,*,#14421,.T.);
#21067=ORIENTED_EDGE('',*,*,#14242,.T.);
#21068=ORIENTED_EDGE('',*,*,#14239,.F.);
#21069=ORIENTED_EDGE('',*,*,#14247,.T.);
#21070=ORIENTED_EDGE('',*,*,#14244,.F.);
#21071=ORIENTED_EDGE('',*,*,#14420,.T.);
#21072=ORIENTED_EDGE('',*,*,#14423,.T.);
#21073=ORIENTED_EDGE('',*,*,#14512,.F.);
#21074=ORIENTED_EDGE('',*,*,#14427,.T.);
#21075=ORIENTED_EDGE('',*,*,#14251,.T.);
#21076=ORIENTED_EDGE('',*,*,#14248,.F.);
#21077=ORIENTED_EDGE('',*,*,#14256,.T.);
#21078=ORIENTED_EDGE('',*,*,#14253,.F.);
#21079=ORIENTED_EDGE('',*,*,#14426,.T.);
#21080=ORIENTED_EDGE('',*,*,#14429,.T.);
#21081=ORIENTED_EDGE('',*,*,#14513,.F.);
#21082=ORIENTED_EDGE('',*,*,#14433,.T.);
#21083=ORIENTED_EDGE('',*,*,#14260,.T.);
#21084=ORIENTED_EDGE('',*,*,#14257,.F.);
#21085=ORIENTED_EDGE('',*,*,#14265,.T.);
#21086=ORIENTED_EDGE('',*,*,#14262,.F.);
#21087=ORIENTED_EDGE('',*,*,#14432,.T.);
#21088=ORIENTED_EDGE('',*,*,#14435,.T.);
#21089=ORIENTED_EDGE('',*,*,#14514,.F.);
#21090=ORIENTED_EDGE('',*,*,#14439,.T.);
#21091=ORIENTED_EDGE('',*,*,#14269,.T.);
#21092=ORIENTED_EDGE('',*,*,#14266,.F.);
#21093=ORIENTED_EDGE('',*,*,#14274,.T.);
#21094=ORIENTED_EDGE('',*,*,#14271,.F.);
#21095=ORIENTED_EDGE('',*,*,#14438,.T.);
#21096=ORIENTED_EDGE('',*,*,#14441,.T.);
#21097=ORIENTED_EDGE('',*,*,#14515,.F.);
#21098=ORIENTED_EDGE('',*,*,#14445,.T.);
#21099=ORIENTED_EDGE('',*,*,#14278,.T.);
#21100=ORIENTED_EDGE('',*,*,#14275,.F.);
#21101=ORIENTED_EDGE('',*,*,#14283,.T.);
#21102=ORIENTED_EDGE('',*,*,#14280,.F.);
#21103=ORIENTED_EDGE('',*,*,#14444,.T.);
#21104=ORIENTED_EDGE('',*,*,#14447,.T.);
#21105=ORIENTED_EDGE('',*,*,#14516,.F.);
#21106=ORIENTED_EDGE('',*,*,#14451,.T.);
#21107=ORIENTED_EDGE('',*,*,#14287,.T.);
#21108=ORIENTED_EDGE('',*,*,#14284,.F.);
#21109=ORIENTED_EDGE('',*,*,#14292,.T.);
#21110=ORIENTED_EDGE('',*,*,#14289,.F.);
#21111=ORIENTED_EDGE('',*,*,#14450,.T.);
#21112=ORIENTED_EDGE('',*,*,#14453,.T.);
#21113=ORIENTED_EDGE('',*,*,#14517,.F.);
#21114=ORIENTED_EDGE('',*,*,#14457,.T.);
#21115=ORIENTED_EDGE('',*,*,#14296,.T.);
#21116=ORIENTED_EDGE('',*,*,#14293,.F.);
#21117=ORIENTED_EDGE('',*,*,#14301,.T.);
#21118=ORIENTED_EDGE('',*,*,#14298,.F.);
#21119=ORIENTED_EDGE('',*,*,#14456,.T.);
#21120=ORIENTED_EDGE('',*,*,#14459,.T.);
#21121=ORIENTED_EDGE('',*,*,#14518,.F.);
#21122=ORIENTED_EDGE('',*,*,#14463,.T.);
#21123=ORIENTED_EDGE('',*,*,#14305,.T.);
#21124=ORIENTED_EDGE('',*,*,#14302,.F.);
#21125=ORIENTED_EDGE('',*,*,#14310,.T.);
#21126=ORIENTED_EDGE('',*,*,#14307,.F.);
#21127=ORIENTED_EDGE('',*,*,#14462,.T.);
#21128=ORIENTED_EDGE('',*,*,#14465,.T.);
#21129=ORIENTED_EDGE('',*,*,#14519,.F.);
#21130=ORIENTED_EDGE('',*,*,#14469,.T.);
#21131=ORIENTED_EDGE('',*,*,#14314,.T.);
#21132=ORIENTED_EDGE('',*,*,#14311,.F.);
#21133=ORIENTED_EDGE('',*,*,#14319,.T.);
#21134=ORIENTED_EDGE('',*,*,#14316,.F.);
#21135=ORIENTED_EDGE('',*,*,#14468,.T.);
#21136=ORIENTED_EDGE('',*,*,#14471,.T.);
#21137=ORIENTED_EDGE('',*,*,#14520,.F.);
#21138=ORIENTED_EDGE('',*,*,#14475,.T.);
#21139=ORIENTED_EDGE('',*,*,#14323,.T.);
#21140=ORIENTED_EDGE('',*,*,#14320,.F.);
#21141=ORIENTED_EDGE('',*,*,#14328,.T.);
#21142=ORIENTED_EDGE('',*,*,#14325,.F.);
#21143=ORIENTED_EDGE('',*,*,#14474,.T.);
#21144=ORIENTED_EDGE('',*,*,#14477,.T.);
#21145=ORIENTED_EDGE('',*,*,#14521,.F.);
#21146=ORIENTED_EDGE('',*,*,#14481,.T.);
#21147=ORIENTED_EDGE('',*,*,#14332,.T.);
#21148=ORIENTED_EDGE('',*,*,#14329,.F.);
#21149=ORIENTED_EDGE('',*,*,#14337,.T.);
#21150=ORIENTED_EDGE('',*,*,#14334,.F.);
#21151=ORIENTED_EDGE('',*,*,#14480,.T.);
#21152=ORIENTED_EDGE('',*,*,#14483,.T.);
#21153=ORIENTED_EDGE('',*,*,#14522,.F.);
#21154=ORIENTED_EDGE('',*,*,#14487,.T.);
#21155=ORIENTED_EDGE('',*,*,#14341,.T.);
#21156=ORIENTED_EDGE('',*,*,#14338,.F.);
#21157=ORIENTED_EDGE('',*,*,#14346,.T.);
#21158=ORIENTED_EDGE('',*,*,#14343,.F.);
#21159=ORIENTED_EDGE('',*,*,#14486,.T.);
#21160=ORIENTED_EDGE('',*,*,#14489,.T.);
#21161=ORIENTED_EDGE('',*,*,#14523,.F.);
#21162=ORIENTED_EDGE('',*,*,#14493,.T.);
#21163=ORIENTED_EDGE('',*,*,#14350,.T.);
#21164=ORIENTED_EDGE('',*,*,#14347,.F.);
#21165=ORIENTED_EDGE('',*,*,#14355,.T.);
#21166=ORIENTED_EDGE('',*,*,#14352,.F.);
#21167=ORIENTED_EDGE('',*,*,#14492,.T.);
#21168=ORIENTED_EDGE('',*,*,#14495,.T.);
#21169=ORIENTED_EDGE('',*,*,#14524,.F.);
#21170=ORIENTED_EDGE('',*,*,#14499,.T.);
#21171=ORIENTED_EDGE('',*,*,#14359,.T.);
#21172=ORIENTED_EDGE('',*,*,#14356,.F.);
#21173=ORIENTED_EDGE('',*,*,#14364,.T.);
#21174=ORIENTED_EDGE('',*,*,#14361,.F.);
#21175=ORIENTED_EDGE('',*,*,#14498,.T.);
#21176=ORIENTED_EDGE('',*,*,#14501,.T.);
#21177=ORIENTED_EDGE('',*,*,#14525,.F.);
#21178=ORIENTED_EDGE('',*,*,#14526,.T.);
#21179=ORIENTED_EDGE('',*,*,#14527,.T.);
#21180=ORIENTED_EDGE('',*,*,#14528,.F.);
#21181=ORIENTED_EDGE('',*,*,#14529,.T.);
#21182=ORIENTED_EDGE('',*,*,#14530,.F.);
#21183=ORIENTED_EDGE('',*,*,#14531,.T.);
#21184=ORIENTED_EDGE('',*,*,#14532,.T.);
#21185=ORIENTED_EDGE('',*,*,#14533,.F.);
#21186=ORIENTED_EDGE('',*,*,#13955,.T.);
#21187=ORIENTED_EDGE('',*,*,#13965,.F.);
#21188=ORIENTED_EDGE('',*,*,#13961,.T.);
#21189=ORIENTED_EDGE('',*,*,#13963,.T.);
#21190=ORIENTED_EDGE('',*,*,#14502,.T.);
#21191=ORIENTED_EDGE('',*,*,#13975,.F.);
#21192=ORIENTED_EDGE('',*,*,#14534,.T.);
#21193=ORIENTED_EDGE('',*,*,#14525,.T.);
#21194=ORIENTED_EDGE('',*,*,#14496,.T.);
#21195=ORIENTED_EDGE('',*,*,#13983,.F.);
#21196=ORIENTED_EDGE('',*,*,#14500,.T.);
#21197=ORIENTED_EDGE('',*,*,#14524,.T.);
#21198=ORIENTED_EDGE('',*,*,#14490,.T.);
#21199=ORIENTED_EDGE('',*,*,#13991,.F.);
#21200=ORIENTED_EDGE('',*,*,#14494,.T.);
#21201=ORIENTED_EDGE('',*,*,#14523,.T.);
#21202=ORIENTED_EDGE('',*,*,#14484,.T.);
#21203=ORIENTED_EDGE('',*,*,#13999,.F.);
#21204=ORIENTED_EDGE('',*,*,#14488,.T.);
#21205=ORIENTED_EDGE('',*,*,#14522,.T.);
#21206=ORIENTED_EDGE('',*,*,#14478,.T.);
#21207=ORIENTED_EDGE('',*,*,#14007,.F.);
#21208=ORIENTED_EDGE('',*,*,#14482,.T.);
#21209=ORIENTED_EDGE('',*,*,#14521,.T.);
#21210=ORIENTED_EDGE('',*,*,#14472,.T.);
#21211=ORIENTED_EDGE('',*,*,#14015,.F.);
#21212=ORIENTED_EDGE('',*,*,#14476,.T.);
#21213=ORIENTED_EDGE('',*,*,#14520,.T.);
#21214=ORIENTED_EDGE('',*,*,#14466,.T.);
#21215=ORIENTED_EDGE('',*,*,#14023,.F.);
#21216=ORIENTED_EDGE('',*,*,#14470,.T.);
#21217=ORIENTED_EDGE('',*,*,#14519,.T.);
#21218=ORIENTED_EDGE('',*,*,#14460,.T.);
#21219=ORIENTED_EDGE('',*,*,#14031,.F.);
#21220=ORIENTED_EDGE('',*,*,#14464,.T.);
#21221=ORIENTED_EDGE('',*,*,#14518,.T.);
#21222=ORIENTED_EDGE('',*,*,#14454,.T.);
#21223=ORIENTED_EDGE('',*,*,#14039,.F.);
#21224=ORIENTED_EDGE('',*,*,#14458,.T.);
#21225=ORIENTED_EDGE('',*,*,#14517,.T.);
#21226=ORIENTED_EDGE('',*,*,#14448,.T.);
#21227=ORIENTED_EDGE('',*,*,#14047,.F.);
#21228=ORIENTED_EDGE('',*,*,#14452,.T.);
#21229=ORIENTED_EDGE('',*,*,#14516,.T.);
#21230=ORIENTED_EDGE('',*,*,#14442,.T.);
#21231=ORIENTED_EDGE('',*,*,#14055,.F.);
#21232=ORIENTED_EDGE('',*,*,#14446,.T.);
#21233=ORIENTED_EDGE('',*,*,#14515,.T.);
#21234=ORIENTED_EDGE('',*,*,#14436,.T.);
#21235=ORIENTED_EDGE('',*,*,#14063,.F.);
#21236=ORIENTED_EDGE('',*,*,#14440,.T.);
#21237=ORIENTED_EDGE('',*,*,#14514,.T.);
#21238=ORIENTED_EDGE('',*,*,#14430,.T.);
#21239=ORIENTED_EDGE('',*,*,#14071,.F.);
#21240=ORIENTED_EDGE('',*,*,#14434,.T.);
#21241=ORIENTED_EDGE('',*,*,#14513,.T.);
#21242=ORIENTED_EDGE('',*,*,#14424,.T.);
#21243=ORIENTED_EDGE('',*,*,#14079,.F.);
#21244=ORIENTED_EDGE('',*,*,#14428,.T.);
#21245=ORIENTED_EDGE('',*,*,#14512,.T.);
#21246=ORIENTED_EDGE('',*,*,#14418,.T.);
#21247=ORIENTED_EDGE('',*,*,#14087,.F.);
#21248=ORIENTED_EDGE('',*,*,#14422,.T.);
#21249=ORIENTED_EDGE('',*,*,#14511,.T.);
#21250=ORIENTED_EDGE('',*,*,#14412,.T.);
#21251=ORIENTED_EDGE('',*,*,#14095,.F.);
#21252=ORIENTED_EDGE('',*,*,#14416,.T.);
#21253=ORIENTED_EDGE('',*,*,#14510,.T.);
#21254=ORIENTED_EDGE('',*,*,#14406,.T.);
#21255=ORIENTED_EDGE('',*,*,#14103,.F.);
#21256=ORIENTED_EDGE('',*,*,#14410,.T.);
#21257=ORIENTED_EDGE('',*,*,#14509,.T.);
#21258=ORIENTED_EDGE('',*,*,#14400,.T.);
#21259=ORIENTED_EDGE('',*,*,#14111,.F.);
#21260=ORIENTED_EDGE('',*,*,#14404,.T.);
#21261=ORIENTED_EDGE('',*,*,#14508,.T.);
#21262=ORIENTED_EDGE('',*,*,#14394,.T.);
#21263=ORIENTED_EDGE('',*,*,#14119,.F.);
#21264=ORIENTED_EDGE('',*,*,#14398,.T.);
#21265=ORIENTED_EDGE('',*,*,#14507,.T.);
#21266=ORIENTED_EDGE('',*,*,#14388,.T.);
#21267=ORIENTED_EDGE('',*,*,#14127,.F.);
#21268=ORIENTED_EDGE('',*,*,#14392,.T.);
#21269=ORIENTED_EDGE('',*,*,#14506,.T.);
#21270=ORIENTED_EDGE('',*,*,#14382,.T.);
#21271=ORIENTED_EDGE('',*,*,#14135,.F.);
#21272=ORIENTED_EDGE('',*,*,#14386,.T.);
#21273=ORIENTED_EDGE('',*,*,#14505,.T.);
#21274=ORIENTED_EDGE('',*,*,#14376,.T.);
#21275=ORIENTED_EDGE('',*,*,#14143,.F.);
#21276=ORIENTED_EDGE('',*,*,#14380,.T.);
#21277=ORIENTED_EDGE('',*,*,#14504,.T.);
#21278=ORIENTED_EDGE('',*,*,#14370,.T.);
#21279=ORIENTED_EDGE('',*,*,#14151,.F.);
#21280=ORIENTED_EDGE('',*,*,#14374,.T.);
#21281=ORIENTED_EDGE('',*,*,#14503,.T.);
#21282=ORIENTED_EDGE('',*,*,#14528,.T.);
#21283=ORIENTED_EDGE('',*,*,#14535,.T.);
#21284=ORIENTED_EDGE('',*,*,#13972,.T.);
#21285=ORIENTED_EDGE('',*,*,#14536,.T.);
#21286=ORIENTED_EDGE('',*,*,#14535,.F.);
#21287=ORIENTED_EDGE('',*,*,#14527,.F.);
#21288=ORIENTED_EDGE('',*,*,#14537,.T.);
#21289=ORIENTED_EDGE('',*,*,#13973,.F.);
#21290=ORIENTED_EDGE('',*,*,#14530,.T.);
#21291=ORIENTED_EDGE('',*,*,#14538,.T.);
#21292=ORIENTED_EDGE('',*,*,#13970,.T.);
#21293=ORIENTED_EDGE('',*,*,#14539,.T.);
#21294=ORIENTED_EDGE('',*,*,#14536,.F.);
#21295=ORIENTED_EDGE('',*,*,#13971,.F.);
#21296=ORIENTED_EDGE('',*,*,#14538,.F.);
#21297=ORIENTED_EDGE('',*,*,#14529,.F.);
#21298=ORIENTED_EDGE('',*,*,#14539,.F.);
#21299=ORIENTED_EDGE('',*,*,#13969,.F.);
#21300=ORIENTED_EDGE('',*,*,#14540,.F.);
#21301=ORIENTED_EDGE('',*,*,#14531,.F.);
#21302=ORIENTED_EDGE('',*,*,#14526,.F.);
#21303=ORIENTED_EDGE('',*,*,#14534,.F.);
#21304=ORIENTED_EDGE('',*,*,#13974,.F.);
#21305=ORIENTED_EDGE('',*,*,#14537,.F.);
#21306=ORIENTED_EDGE('',*,*,#14532,.F.);
#21307=ORIENTED_EDGE('',*,*,#14540,.T.);
#21308=ORIENTED_EDGE('',*,*,#13968,.F.);
#21309=ORIENTED_EDGE('',*,*,#14541,.F.);
#21310=ORIENTED_EDGE('',*,*,#14368,.T.);
#21311=ORIENTED_EDGE('',*,*,#14533,.T.);
#21312=ORIENTED_EDGE('',*,*,#14541,.T.);
#21313=ORIENTED_EDGE('',*,*,#13967,.F.);
#23531=CYLINDRICAL_SURFACE('',#26318,8.);
#23532=CYLINDRICAL_SURFACE('',#26418,0.5);
#23533=CYLINDRICAL_SURFACE('',#26421,0.5);
#23534=CYLINDRICAL_SURFACE('',#26423,21.4999999999992);
#23535=CYLINDRICAL_SURFACE('',#26425,0.5);
#23536=CYLINDRICAL_SURFACE('',#26428,0.5);
#23537=CYLINDRICAL_SURFACE('',#26430,21.4999999999992);
#23538=CYLINDRICAL_SURFACE('',#26432,0.5);
#23539=CYLINDRICAL_SURFACE('',#26435,0.5);
#23540=CYLINDRICAL_SURFACE('',#26437,21.4999999999992);
#23541=CYLINDRICAL_SURFACE('',#26439,0.5);
#23542=CYLINDRICAL_SURFACE('',#26442,0.5);
#23543=CYLINDRICAL_SURFACE('',#26444,21.4999999999992);
#23544=CYLINDRICAL_SURFACE('',#26446,0.5);
#23545=CYLINDRICAL_SURFACE('',#26449,0.5);
#23546=CYLINDRICAL_SURFACE('',#26451,21.4999999999992);
#23547=CYLINDRICAL_SURFACE('',#26453,0.5);
#23548=CYLINDRICAL_SURFACE('',#26456,0.5);
#23549=CYLINDRICAL_SURFACE('',#26458,21.4999999999992);
#23550=CYLINDRICAL_SURFACE('',#26460,0.5);
#23551=CYLINDRICAL_SURFACE('',#26463,0.5);
#23552=CYLINDRICAL_SURFACE('',#26465,21.4999999999992);
#23553=CYLINDRICAL_SURFACE('',#26467,0.5);
#23554=CYLINDRICAL_SURFACE('',#26470,0.5);
#23555=CYLINDRICAL_SURFACE('',#26472,21.4999999999992);
#23556=CYLINDRICAL_SURFACE('',#26474,0.5);
#23557=CYLINDRICAL_SURFACE('',#26477,0.5);
#23558=CYLINDRICAL_SURFACE('',#26479,21.4999999999992);
#23559=CYLINDRICAL_SURFACE('',#26481,0.5);
#23560=CYLINDRICAL_SURFACE('',#26484,0.5);
#23561=CYLINDRICAL_SURFACE('',#26486,21.4999999999992);
#23562=CYLINDRICAL_SURFACE('',#26488,0.5);
#23563=CYLINDRICAL_SURFACE('',#26491,0.5);
#23564=CYLINDRICAL_SURFACE('',#26493,21.4999999999992);
#23565=CYLINDRICAL_SURFACE('',#26495,0.5);
#23566=CYLINDRICAL_SURFACE('',#26498,0.5);
#23567=CYLINDRICAL_SURFACE('',#26500,21.4999999999992);
#23568=CYLINDRICAL_SURFACE('',#26502,0.5);
#23569=CYLINDRICAL_SURFACE('',#26505,0.5);
#23570=CYLINDRICAL_SURFACE('',#26507,21.4999999999992);
#23571=CYLINDRICAL_SURFACE('',#26509,0.5);
#23572=CYLINDRICAL_SURFACE('',#26512,0.5);
#23573=CYLINDRICAL_SURFACE('',#26514,21.4999999999992);
#23574=CYLINDRICAL_SURFACE('',#26516,0.5);
#23575=CYLINDRICAL_SURFACE('',#26519,0.5);
#23576=CYLINDRICAL_SURFACE('',#26521,21.4999999999992);
#23577=CYLINDRICAL_SURFACE('',#26523,0.5);
#23578=CYLINDRICAL_SURFACE('',#26526,0.5);
#23579=CYLINDRICAL_SURFACE('',#26528,21.4999999999992);
#23580=CYLINDRICAL_SURFACE('',#26530,0.5);
#23581=CYLINDRICAL_SURFACE('',#26533,0.5);
#23582=CYLINDRICAL_SURFACE('',#26535,21.4999999999992);
#23583=CYLINDRICAL_SURFACE('',#26537,0.5);
#23584=CYLINDRICAL_SURFACE('',#26540,0.5);
#23585=CYLINDRICAL_SURFACE('',#26542,21.4999999999992);
#23586=CYLINDRICAL_SURFACE('',#26544,0.5);
#23587=CYLINDRICAL_SURFACE('',#26547,0.5);
#23588=CYLINDRICAL_SURFACE('',#26549,21.4999999999992);
#23589=CYLINDRICAL_SURFACE('',#26551,0.5);
#23590=CYLINDRICAL_SURFACE('',#26554,0.5);
#23591=CYLINDRICAL_SURFACE('',#26556,21.4999999999992);
#23592=CYLINDRICAL_SURFACE('',#26558,0.5);
#23593=CYLINDRICAL_SURFACE('',#26561,0.5);
#23594=CYLINDRICAL_SURFACE('',#26563,21.4999999999992);
#23595=CYLINDRICAL_SURFACE('',#26565,0.5);
#23596=CYLINDRICAL_SURFACE('',#26568,0.5);
#23597=CYLINDRICAL_SURFACE('',#26570,21.4999999999992);
#23598=CYLINDRICAL_SURFACE('',#26572,0.5);
#23599=CYLINDRICAL_SURFACE('',#26575,0.5);
#23600=CYLINDRICAL_SURFACE('',#26577,21.4999999999992);
#23601=CYLINDRICAL_SURFACE('',#26630,26.);
#23602=CYLINDRICAL_SURFACE('',#26631,26.);
#23603=CYLINDRICAL_SURFACE('',#26632,26.);
#23604=CYLINDRICAL_SURFACE('',#26633,26.);
#23605=CYLINDRICAL_SURFACE('',#26634,26.);
#23606=CYLINDRICAL_SURFACE('',#26635,26.);
#23607=CYLINDRICAL_SURFACE('',#26636,26.);
#23608=CYLINDRICAL_SURFACE('',#26637,26.);
#23609=CYLINDRICAL_SURFACE('',#26638,26.);
#23610=CYLINDRICAL_SURFACE('',#26639,26.);
#23611=CYLINDRICAL_SURFACE('',#26640,26.);
#23612=CYLINDRICAL_SURFACE('',#26641,26.);
#23613=CYLINDRICAL_SURFACE('',#26642,26.);
#23614=CYLINDRICAL_SURFACE('',#26643,26.);
#23615=CYLINDRICAL_SURFACE('',#26644,26.);
#23616=CYLINDRICAL_SURFACE('',#26645,26.);
#23617=CYLINDRICAL_SURFACE('',#26646,26.);
#23618=CYLINDRICAL_SURFACE('',#26647,26.);
#23619=CYLINDRICAL_SURFACE('',#26648,26.);
#23620=CYLINDRICAL_SURFACE('',#26649,26.);
#23621=CYLINDRICAL_SURFACE('',#26650,26.);
#23622=CYLINDRICAL_SURFACE('',#26651,26.);
#23623=CYLINDRICAL_SURFACE('',#26652,26.);
#23624=CYLINDRICAL_SURFACE('',#26653,0.5);
#23625=CYLINDRICAL_SURFACE('',#26655,0.5);
#23626=CYLINDRICAL_SURFACE('',#26656,21.4999999999992);
#23627=CYLINDRICAL_SURFACE('',#26658,26.);
#24613=ADVANCED_FACE('',(#2507),#1532,.F.);
#24614=ADVANCED_FACE('',(#2508),#1533,.F.);
#24615=ADVANCED_FACE('',(#2509),#1534,.F.);
#24616=ADVANCED_FACE('',(#2510),#23531,.F.);
#24617=ADVANCED_FACE('',(#2511,#1281),#1535,.T.);
#24618=ADVANCED_FACE('',(#2512),#23532,.F.);
#24619=ADVANCED_FACE('',(#2513),#1536,.F.);
#24620=ADVANCED_FACE('',(#2514),#23533,.F.);
#24621=ADVANCED_FACE('',(#2515),#23534,.T.);
#24622=ADVANCED_FACE('',(#2516),#23535,.F.);
#24623=ADVANCED_FACE('',(#2517),#1537,.F.);
#24624=ADVANCED_FACE('',(#2518),#23536,.F.);
#24625=ADVANCED_FACE('',(#2519),#23537,.T.);
#24626=ADVANCED_FACE('',(#2520),#23538,.F.);
#24627=ADVANCED_FACE('',(#2521),#1538,.F.);
#24628=ADVANCED_FACE('',(#2522),#23539,.F.);
#24629=ADVANCED_FACE('',(#2523),#23540,.T.);
#24630=ADVANCED_FACE('',(#2524),#23541,.F.);
#24631=ADVANCED_FACE('',(#2525),#1539,.F.);
#24632=ADVANCED_FACE('',(#2526),#23542,.F.);
#24633=ADVANCED_FACE('',(#2527),#23543,.T.);
#24634=ADVANCED_FACE('',(#2528),#23544,.F.);
#24635=ADVANCED_FACE('',(#2529),#1540,.F.);
#24636=ADVANCED_FACE('',(#2530),#23545,.F.);
#24637=ADVANCED_FACE('',(#2531),#23546,.T.);
#24638=ADVANCED_FACE('',(#2532),#23547,.F.);
#24639=ADVANCED_FACE('',(#2533),#1541,.F.);
#24640=ADVANCED_FACE('',(#2534),#23548,.F.);
#24641=ADVANCED_FACE('',(#2535),#23549,.T.);
#24642=ADVANCED_FACE('',(#2536),#23550,.F.);
#24643=ADVANCED_FACE('',(#2537),#1542,.F.);
#24644=ADVANCED_FACE('',(#2538),#23551,.F.);
#24645=ADVANCED_FACE('',(#2539),#23552,.T.);
#24646=ADVANCED_FACE('',(#2540),#23553,.F.);
#24647=ADVANCED_FACE('',(#2541),#1543,.F.);
#24648=ADVANCED_FACE('',(#2542),#23554,.F.);
#24649=ADVANCED_FACE('',(#2543),#23555,.T.);
#24650=ADVANCED_FACE('',(#2544),#23556,.F.);
#24651=ADVANCED_FACE('',(#2545),#1544,.F.);
#24652=ADVANCED_FACE('',(#2546),#23557,.F.);
#24653=ADVANCED_FACE('',(#2547),#23558,.T.);
#24654=ADVANCED_FACE('',(#2548),#23559,.F.);
#24655=ADVANCED_FACE('',(#2549),#1545,.F.);
#24656=ADVANCED_FACE('',(#2550),#23560,.F.);
#24657=ADVANCED_FACE('',(#2551),#23561,.T.);
#24658=ADVANCED_FACE('',(#2552),#23562,.F.);
#24659=ADVANCED_FACE('',(#2553),#1546,.F.);
#24660=ADVANCED_FACE('',(#2554),#23563,.F.);
#24661=ADVANCED_FACE('',(#2555),#23564,.T.);
#24662=ADVANCED_FACE('',(#2556),#23565,.F.);
#24663=ADVANCED_FACE('',(#2557),#1547,.F.);
#24664=ADVANCED_FACE('',(#2558),#23566,.F.);
#24665=ADVANCED_FACE('',(#2559),#23567,.T.);
#24666=ADVANCED_FACE('',(#2560),#23568,.F.);
#24667=ADVANCED_FACE('',(#2561),#1548,.F.);
#24668=ADVANCED_FACE('',(#2562),#23569,.F.);
#24669=ADVANCED_FACE('',(#2563),#23570,.T.);
#24670=ADVANCED_FACE('',(#2564),#23571,.F.);
#24671=ADVANCED_FACE('',(#2565),#1549,.F.);
#24672=ADVANCED_FACE('',(#2566),#23572,.F.);
#24673=ADVANCED_FACE('',(#2567),#23573,.T.);
#24674=ADVANCED_FACE('',(#2568),#23574,.F.);
#24675=ADVANCED_FACE('',(#2569),#1550,.F.);
#24676=ADVANCED_FACE('',(#2570),#23575,.F.);
#24677=ADVANCED_FACE('',(#2571),#23576,.T.);
#24678=ADVANCED_FACE('',(#2572),#23577,.F.);
#24679=ADVANCED_FACE('',(#2573),#1551,.F.);
#24680=ADVANCED_FACE('',(#2574),#23578,.F.);
#24681=ADVANCED_FACE('',(#2575),#23579,.T.);
#24682=ADVANCED_FACE('',(#2576),#23580,.F.);
#24683=ADVANCED_FACE('',(#2577),#1552,.F.);
#24684=ADVANCED_FACE('',(#2578),#23581,.F.);
#24685=ADVANCED_FACE('',(#2579),#23582,.T.);
#24686=ADVANCED_FACE('',(#2580),#23583,.F.);
#24687=ADVANCED_FACE('',(#2581),#1553,.F.);
#24688=ADVANCED_FACE('',(#2582),#23584,.F.);
#24689=ADVANCED_FACE('',(#2583),#23585,.T.);
#24690=ADVANCED_FACE('',(#2584),#23586,.F.);
#24691=ADVANCED_FACE('',(#2585),#1554,.F.);
#24692=ADVANCED_FACE('',(#2586),#23587,.F.);
#24693=ADVANCED_FACE('',(#2587),#23588,.T.);
#24694=ADVANCED_FACE('',(#2588),#23589,.F.);
#24695=ADVANCED_FACE('',(#2589),#1555,.F.);
#24696=ADVANCED_FACE('',(#2590),#23590,.F.);
#24697=ADVANCED_FACE('',(#2591),#23591,.T.);
#24698=ADVANCED_FACE('',(#2592),#23592,.F.);
#24699=ADVANCED_FACE('',(#2593),#1556,.F.);
#24700=ADVANCED_FACE('',(#2594),#23593,.F.);
#24701=ADVANCED_FACE('',(#2595),#23594,.T.);
#24702=ADVANCED_FACE('',(#2596),#23595,.F.);
#24703=ADVANCED_FACE('',(#2597),#1557,.F.);
#24704=ADVANCED_FACE('',(#2598),#23596,.F.);
#24705=ADVANCED_FACE('',(#2599),#23597,.T.);
#24706=ADVANCED_FACE('',(#2600),#23598,.F.);
#24707=ADVANCED_FACE('',(#2601),#1558,.F.);
#24708=ADVANCED_FACE('',(#2602),#23599,.F.);
#24709=ADVANCED_FACE('',(#2603),#23600,.T.);
#24710=ADVANCED_FACE('',(#2604),#1559,.F.);
#24711=ADVANCED_FACE('',(#2605),#1027,.F.);
#24712=ADVANCED_FACE('',(#2606),#1028,.F.);
#24713=ADVANCED_FACE('',(#2607),#1560,.F.);
#24714=ADVANCED_FACE('',(#2608),#1029,.F.);
#24715=ADVANCED_FACE('',(#2609),#1030,.F.);
#24716=ADVANCED_FACE('',(#2610),#1561,.F.);
#24717=ADVANCED_FACE('',(#2611),#1031,.F.);
#24718=ADVANCED_FACE('',(#2612),#1032,.F.);
#24719=ADVANCED_FACE('',(#2613),#1562,.F.);
#24720=ADVANCED_FACE('',(#2614),#1033,.F.);
#24721=ADVANCED_FACE('',(#2615),#1034,.F.);
#24722=ADVANCED_FACE('',(#2616),#1563,.F.);
#24723=ADVANCED_FACE('',(#2617),#1035,.F.);
#24724=ADVANCED_FACE('',(#2618),#1036,.F.);
#24725=ADVANCED_FACE('',(#2619),#1564,.F.);
#24726=ADVANCED_FACE('',(#2620),#1037,.F.);
#24727=ADVANCED_FACE('',(#2621),#1038,.F.);
#24728=ADVANCED_FACE('',(#2622),#1565,.F.);
#24729=ADVANCED_FACE('',(#2623),#1039,.F.);
#24730=ADVANCED_FACE('',(#2624),#1040,.F.);
#24731=ADVANCED_FACE('',(#2625),#1566,.F.);
#24732=ADVANCED_FACE('',(#2626),#1041,.F.);
#24733=ADVANCED_FACE('',(#2627),#1042,.F.);
#24734=ADVANCED_FACE('',(#2628),#1567,.F.);
#24735=ADVANCED_FACE('',(#2629),#1043,.F.);
#24736=ADVANCED_FACE('',(#2630),#1044,.F.);
#24737=ADVANCED_FACE('',(#2631),#1568,.F.);
#24738=ADVANCED_FACE('',(#2632),#1045,.F.);
#24739=ADVANCED_FACE('',(#2633),#1046,.F.);
#24740=ADVANCED_FACE('',(#2634),#1569,.F.);
#24741=ADVANCED_FACE('',(#2635),#1047,.F.);
#24742=ADVANCED_FACE('',(#2636),#1048,.F.);
#24743=ADVANCED_FACE('',(#2637),#1570,.F.);
#24744=ADVANCED_FACE('',(#2638),#1049,.F.);
#24745=ADVANCED_FACE('',(#2639),#1050,.F.);
#24746=ADVANCED_FACE('',(#2640),#1571,.F.);
#24747=ADVANCED_FACE('',(#2641),#1051,.F.);
#24748=ADVANCED_FACE('',(#2642),#1052,.F.);
#24749=ADVANCED_FACE('',(#2643),#1572,.F.);
#24750=ADVANCED_FACE('',(#2644),#1053,.F.);
#24751=ADVANCED_FACE('',(#2645),#1054,.F.);
#24752=ADVANCED_FACE('',(#2646),#1573,.F.);
#24753=ADVANCED_FACE('',(#2647),#1055,.F.);
#24754=ADVANCED_FACE('',(#2648),#1056,.F.);
#24755=ADVANCED_FACE('',(#2649),#1574,.F.);
#24756=ADVANCED_FACE('',(#2650),#1057,.F.);
#24757=ADVANCED_FACE('',(#2651),#1058,.F.);
#24758=ADVANCED_FACE('',(#2652),#1575,.F.);
#24759=ADVANCED_FACE('',(#2653),#1059,.F.);
#24760=ADVANCED_FACE('',(#2654),#1060,.F.);
#24761=ADVANCED_FACE('',(#2655),#1576,.F.);
#24762=ADVANCED_FACE('',(#2656),#1061,.F.);
#24763=ADVANCED_FACE('',(#2657),#1062,.F.);
#24764=ADVANCED_FACE('',(#2658),#1577,.F.);
#24765=ADVANCED_FACE('',(#2659),#1063,.F.);
#24766=ADVANCED_FACE('',(#2660),#1064,.F.);
#24767=ADVANCED_FACE('',(#2661),#1578,.F.);
#24768=ADVANCED_FACE('',(#2662),#1065,.F.);
#24769=ADVANCED_FACE('',(#2663),#1066,.F.);
#24770=ADVANCED_FACE('',(#2664),#1579,.F.);
#24771=ADVANCED_FACE('',(#2665),#1067,.F.);
#24772=ADVANCED_FACE('',(#2666),#1068,.F.);
#24773=ADVANCED_FACE('',(#2667),#1580,.F.);
#24774=ADVANCED_FACE('',(#2668),#1069,.F.);
#24775=ADVANCED_FACE('',(#2669),#1070,.F.);
#24776=ADVANCED_FACE('',(#2670),#1581,.F.);
#24777=ADVANCED_FACE('',(#2671),#1071,.F.);
#24778=ADVANCED_FACE('',(#2672),#1072,.F.);
#24779=ADVANCED_FACE('',(#2673,#1282),#1582,.F.);
#24780=ADVANCED_FACE('',(#2674),#23601,.T.);
#24781=ADVANCED_FACE('',(#2675),#23602,.T.);
#24782=ADVANCED_FACE('',(#2676),#23603,.T.);
#24783=ADVANCED_FACE('',(#2677),#23604,.T.);
#24784=ADVANCED_FACE('',(#2678),#23605,.T.);
#24785=ADVANCED_FACE('',(#2679),#23606,.T.);
#24786=ADVANCED_FACE('',(#2680),#23607,.T.);
#24787=ADVANCED_FACE('',(#2681),#23608,.T.);
#24788=ADVANCED_FACE('',(#2682),#23609,.T.);
#24789=ADVANCED_FACE('',(#2683),#23610,.T.);
#24790=ADVANCED_FACE('',(#2684),#23611,.T.);
#24791=ADVANCED_FACE('',(#2685),#23612,.T.);
#24792=ADVANCED_FACE('',(#2686),#23613,.T.);
#24793=ADVANCED_FACE('',(#2687),#23614,.T.);
#24794=ADVANCED_FACE('',(#2688),#23615,.T.);
#24795=ADVANCED_FACE('',(#2689),#23616,.T.);
#24796=ADVANCED_FACE('',(#2690),#23617,.T.);
#24797=ADVANCED_FACE('',(#2691),#23618,.T.);
#24798=ADVANCED_FACE('',(#2692),#23619,.T.);
#24799=ADVANCED_FACE('',(#2693),#23620,.T.);
#24800=ADVANCED_FACE('',(#2694),#23621,.T.);
#24801=ADVANCED_FACE('',(#2695),#23622,.T.);
#24802=ADVANCED_FACE('',(#2696),#23623,.T.);
#24803=ADVANCED_FACE('',(#2697),#23624,.F.);
#24804=ADVANCED_FACE('',(#2698),#1583,.F.);
#24805=ADVANCED_FACE('',(#2699),#23625,.F.);
#24806=ADVANCED_FACE('',(#2700),#23626,.T.);
#24807=ADVANCED_FACE('',(#2701),#1584,.F.);
#24808=ADVANCED_FACE('',(#2702),#1073,.F.);
#24809=ADVANCED_FACE('',(#2703),#1074,.F.);
#24810=ADVANCED_FACE('',(#2704),#23627,.T.);
#25155=CLOSED_SHELL('',(#24613,#24614,#24615,#24616,#24617,#24618,#24619,
#24620,#24621,#24622,#24623,#24624,#24625,#24626,#24627,#24628,#24629,#24630,
#24631,#24632,#24633,#24634,#24635,#24636,#24637,#24638,#24639,#24640,#24641,
#24642,#24643,#24644,#24645,#24646,#24647,#24648,#24649,#24650,#24651,#24652,
#24653,#24654,#24655,#24656,#24657,#24658,#24659,#24660,#24661,#24662,#24663,
#24664,#24665,#24666,#24667,#24668,#24669,#24670,#24671,#24672,#24673,#24674,
#24675,#24676,#24677,#24678,#24679,#24680,#24681,#24682,#24683,#24684,#24685,
#24686,#24687,#24688,#24689,#24690,#24691,#24692,#24693,#24694,#24695,#24696,
#24697,#24698,#24699,#24700,#24701,#24702,#24703,#24704,#24705,#24706,#24707,
#24708,#24709,#24710,#24711,#24712,#24713,#24714,#24715,#24716,#24717,#24718,
#24719,#24720,#24721,#24722,#24723,#24724,#24725,#24726,#24727,#24728,#24729,
#24730,#24731,#24732,#24733,#24734,#24735,#24736,#24737,#24738,#24739,#24740,
#24741,#24742,#24743,#24744,#24745,#24746,#24747,#24748,#24749,#24750,#24751,
#24752,#24753,#24754,#24755,#24756,#24757,#24758,#24759,#24760,#24761,#24762,
#24763,#24764,#24765,#24766,#24767,#24768,#24769,#24770,#24771,#24772,#24773,
#24774,#24775,#24776,#24777,#24778,#24779,#24780,#24781,#24782,#24783,#24784,
#24785,#24786,#24787,#24788,#24789,#24790,#24791,#24792,#24793,#24794,#24795,
#24796,#24797,#24798,#24799,#24800,#24801,#24802,#24803,#24804,#24805,#24806,
#24807,#24808,#24809,#24810));
#26314=AXIS2_PLACEMENT_3D('',#174985,#29643,#29644);
#26315=AXIS2_PLACEMENT_3D('',#174986,#29645,#29646);
#26316=AXIS2_PLACEMENT_3D('',#174995,#29651,#29652);
#26317=AXIS2_PLACEMENT_3D('',#175004,#29657,#29658);
#26318=AXIS2_PLACEMENT_3D('',#175007,#29661,#29662);
#26319=AXIS2_PLACEMENT_3D('',#175008,#29663,#29664);
#26320=AXIS2_PLACEMENT_3D('',#175009,#29665,#29666);
#26321=AXIS2_PLACEMENT_3D('',#175010,#29667,#29668);
#26322=AXIS2_PLACEMENT_3D('',#175219,#29669,#29670);
#26323=AXIS2_PLACEMENT_3D('',#175429,#29672,#29673);
#26324=AXIS2_PLACEMENT_3D('',#175431,#29674,#29675);
#26325=AXIS2_PLACEMENT_3D('',#175433,#29676,#29677);
#26326=AXIS2_PLACEMENT_3D('',#175643,#29679,#29680);
#26327=AXIS2_PLACEMENT_3D('',#175853,#29682,#29683);
#26328=AXIS2_PLACEMENT_3D('',#175855,#29684,#29685);
#26329=AXIS2_PLACEMENT_3D('',#175857,#29686,#29687);
#26330=AXIS2_PLACEMENT_3D('',#176067,#29689,#29690);
#26331=AXIS2_PLACEMENT_3D('',#176277,#29692,#29693);
#26332=AXIS2_PLACEMENT_3D('',#176279,#29694,#29695);
#26333=AXIS2_PLACEMENT_3D('',#176281,#29696,#29697);
#26334=AXIS2_PLACEMENT_3D('',#176491,#29699,#29700);
#26335=AXIS2_PLACEMENT_3D('',#176701,#29702,#29703);
#26336=AXIS2_PLACEMENT_3D('',#176703,#29704,#29705);
#26337=AXIS2_PLACEMENT_3D('',#176705,#29706,#29707);
#26338=AXIS2_PLACEMENT_3D('',#176915,#29709,#29710);
#26339=AXIS2_PLACEMENT_3D('',#177125,#29712,#29713);
#26340=AXIS2_PLACEMENT_3D('',#177127,#29714,#29715);
#26341=AXIS2_PLACEMENT_3D('',#177129,#29716,#29717);
#26342=AXIS2_PLACEMENT_3D('',#177339,#29719,#29720);
#26343=AXIS2_PLACEMENT_3D('',#177549,#29722,#29723);
#26344=AXIS2_PLACEMENT_3D('',#177551,#29724,#29725);
#26345=AXIS2_PLACEMENT_3D('',#177553,#29726,#29727);
#26346=AXIS2_PLACEMENT_3D('',#177763,#29729,#29730);
#26347=AXIS2_PLACEMENT_3D('',#177973,#29732,#29733);
#26348=AXIS2_PLACEMENT_3D('',#177975,#29734,#29735);
#26349=AXIS2_PLACEMENT_3D('',#177977,#29736,#29737);
#26350=AXIS2_PLACEMENT_3D('',#178187,#29739,#29740);
#26351=AXIS2_PLACEMENT_3D('',#178397,#29742,#29743);
#26352=AXIS2_PLACEMENT_3D('',#178399,#29744,#29745);
#26353=AXIS2_PLACEMENT_3D('',#178401,#29746,#29747);
#26354=AXIS2_PLACEMENT_3D('',#178611,#29749,#29750);
#26355=AXIS2_PLACEMENT_3D('',#178821,#29752,#29753);
#26356=AXIS2_PLACEMENT_3D('',#178823,#29754,#29755);
#26357=AXIS2_PLACEMENT_3D('',#178825,#29756,#29757);
#26358=AXIS2_PLACEMENT_3D('',#179035,#29759,#29760);
#26359=AXIS2_PLACEMENT_3D('',#179245,#29762,#29763);
#26360=AXIS2_PLACEMENT_3D('',#179247,#29764,#29765);
#26361=AXIS2_PLACEMENT_3D('',#179249,#29766,#29767);
#26362=AXIS2_PLACEMENT_3D('',#179459,#29769,#29770);
#26363=AXIS2_PLACEMENT_3D('',#179669,#29772,#29773);
#26364=AXIS2_PLACEMENT_3D('',#179671,#29774,#29775);
#26365=AXIS2_PLACEMENT_3D('',#179673,#29776,#29777);
#26366=AXIS2_PLACEMENT_3D('',#179883,#29779,#29780);
#26367=AXIS2_PLACEMENT_3D('',#180093,#29782,#29783);
#26368=AXIS2_PLACEMENT_3D('',#180095,#29784,#29785);
#26369=AXIS2_PLACEMENT_3D('',#180097,#29786,#29787);
#26370=AXIS2_PLACEMENT_3D('',#180307,#29789,#29790);
#26371=AXIS2_PLACEMENT_3D('',#180517,#29792,#29793);
#26372=AXIS2_PLACEMENT_3D('',#180519,#29794,#29795);
#26373=AXIS2_PLACEMENT_3D('',#180521,#29796,#29797);
#26374=AXIS2_PLACEMENT_3D('',#180731,#29799,#29800);
#26375=AXIS2_PLACEMENT_3D('',#180941,#29802,#29803);
#26376=AXIS2_PLACEMENT_3D('',#180943,#29804,#29805);
#26377=AXIS2_PLACEMENT_3D('',#180945,#29806,#29807);
#26378=AXIS2_PLACEMENT_3D('',#181155,#29809,#29810);
#26379=AXIS2_PLACEMENT_3D('',#181365,#29812,#29813);
#26380=AXIS2_PLACEMENT_3D('',#181367,#29814,#29815);
#26381=AXIS2_PLACEMENT_3D('',#181369,#29816,#29817);
#26382=AXIS2_PLACEMENT_3D('',#181579,#29819,#29820);
#26383=AXIS2_PLACEMENT_3D('',#181789,#29822,#29823);
#26384=AXIS2_PLACEMENT_3D('',#181791,#29824,#29825);
#26385=AXIS2_PLACEMENT_3D('',#181793,#29826,#29827);
#26386=AXIS2_PLACEMENT_3D('',#182003,#29829,#29830);
#26387=AXIS2_PLACEMENT_3D('',#182213,#29832,#29833);
#26388=AXIS2_PLACEMENT_3D('',#182215,#29834,#29835);
#26389=AXIS2_PLACEMENT_3D('',#182217,#29836,#29837);
#26390=AXIS2_PLACEMENT_3D('',#182427,#29839,#29840);
#26391=AXIS2_PLACEMENT_3D('',#182637,#29842,#29843);
#26392=AXIS2_PLACEMENT_3D('',#182639,#29844,#29845);
#26393=AXIS2_PLACEMENT_3D('',#182641,#29846,#29847);
#26394=AXIS2_PLACEMENT_3D('',#182851,#29849,#29850);
#26395=AXIS2_PLACEMENT_3D('',#183061,#29852,#29853);
#26396=AXIS2_PLACEMENT_3D('',#183063,#29854,#29855);
#26397=AXIS2_PLACEMENT_3D('',#183065,#29856,#29857);
#26398=AXIS2_PLACEMENT_3D('',#183275,#29859,#29860);
#26399=AXIS2_PLACEMENT_3D('',#183485,#29862,#29863);
#26400=AXIS2_PLACEMENT_3D('',#183487,#29864,#29865);
#26401=AXIS2_PLACEMENT_3D('',#183489,#29866,#29867);
#26402=AXIS2_PLACEMENT_3D('',#183699,#29869,#29870);
#26403=AXIS2_PLACEMENT_3D('',#183909,#29872,#29873);
#26404=AXIS2_PLACEMENT_3D('',#183911,#29874,#29875);
#26405=AXIS2_PLACEMENT_3D('',#183913,#29876,#29877);
#26406=AXIS2_PLACEMENT_3D('',#184123,#29879,#29880);
#26407=AXIS2_PLACEMENT_3D('',#184333,#29882,#29883);
#26408=AXIS2_PLACEMENT_3D('',#184335,#29884,#29885);
#26409=AXIS2_PLACEMENT_3D('',#184337,#29886,#29887);
#26410=AXIS2_PLACEMENT_3D('',#184547,#29889,#29890);
#26411=AXIS2_PLACEMENT_3D('',#184757,#29892,#29893);
#26412=AXIS2_PLACEMENT_3D('',#184759,#29894,#29895);
#26413=AXIS2_PLACEMENT_3D('',#184761,#29896,#29897);
#26414=AXIS2_PLACEMENT_3D('',#184971,#29899,#29900);
#26415=AXIS2_PLACEMENT_3D('',#185181,#29902,#29903);
#26416=AXIS2_PLACEMENT_3D('',#185183,#29904,#29905);
#26417=AXIS2_PLACEMENT_3D('',#185185,#29906,#29907);
#26418=AXIS2_PLACEMENT_3D('',#185187,#29909,#29910);
#26419=AXIS2_PLACEMENT_3D('',#185190,#29911,#29912);
#26420=AXIS2_PLACEMENT_3D('',#185193,#29915,#29916);
#26421=AXIS2_PLACEMENT_3D('',#185197,#29919,#29920);
#26422=AXIS2_PLACEMENT_3D('',#185200,#29921,#29922);
#26423=AXIS2_PLACEMENT_3D('',#185203,#29925,#29926);
#26424=AXIS2_PLACEMENT_3D('',#185204,#29927,#29928);
#26425=AXIS2_PLACEMENT_3D('',#185205,#29929,#29930);
#26426=AXIS2_PLACEMENT_3D('',#185208,#29931,#29932);
#26427=AXIS2_PLACEMENT_3D('',#185211,#29935,#29936);
#26428=AXIS2_PLACEMENT_3D('',#185215,#29939,#29940);
#26429=AXIS2_PLACEMENT_3D('',#185218,#29941,#29942);
#26430=AXIS2_PLACEMENT_3D('',#185221,#29945,#29946);
#26431=AXIS2_PLACEMENT_3D('',#185222,#29947,#29948);
#26432=AXIS2_PLACEMENT_3D('',#185223,#29949,#29950);
#26433=AXIS2_PLACEMENT_3D('',#185226,#29951,#29952);
#26434=AXIS2_PLACEMENT_3D('',#185229,#29955,#29956);
#26435=AXIS2_PLACEMENT_3D('',#185233,#29959,#29960);
#26436=AXIS2_PLACEMENT_3D('',#185236,#29961,#29962);
#26437=AXIS2_PLACEMENT_3D('',#185239,#29965,#29966);
#26438=AXIS2_PLACEMENT_3D('',#185240,#29967,#29968);
#26439=AXIS2_PLACEMENT_3D('',#185241,#29969,#29970);
#26440=AXIS2_PLACEMENT_3D('',#185244,#29971,#29972);
#26441=AXIS2_PLACEMENT_3D('',#185247,#29975,#29976);
#26442=AXIS2_PLACEMENT_3D('',#185251,#29979,#29980);
#26443=AXIS2_PLACEMENT_3D('',#185254,#29981,#29982);
#26444=AXIS2_PLACEMENT_3D('',#185257,#29985,#29986);
#26445=AXIS2_PLACEMENT_3D('',#185258,#29987,#29988);
#26446=AXIS2_PLACEMENT_3D('',#185259,#29989,#29990);
#26447=AXIS2_PLACEMENT_3D('',#185262,#29991,#29992);
#26448=AXIS2_PLACEMENT_3D('',#185265,#29995,#29996);
#26449=AXIS2_PLACEMENT_3D('',#185269,#29999,#30000);
#26450=AXIS2_PLACEMENT_3D('',#185272,#30001,#30002);
#26451=AXIS2_PLACEMENT_3D('',#185275,#30005,#30006);
#26452=AXIS2_PLACEMENT_3D('',#185276,#30007,#30008);
#26453=AXIS2_PLACEMENT_3D('',#185277,#30009,#30010);
#26454=AXIS2_PLACEMENT_3D('',#185280,#30011,#30012);
#26455=AXIS2_PLACEMENT_3D('',#185283,#30015,#30016);
#26456=AXIS2_PLACEMENT_3D('',#185287,#30019,#30020);
#26457=AXIS2_PLACEMENT_3D('',#185290,#30021,#30022);
#26458=AXIS2_PLACEMENT_3D('',#185293,#30025,#30026);
#26459=AXIS2_PLACEMENT_3D('',#185294,#30027,#30028);
#26460=AXIS2_PLACEMENT_3D('',#185295,#30029,#30030);
#26461=AXIS2_PLACEMENT_3D('',#185298,#30031,#30032);
#26462=AXIS2_PLACEMENT_3D('',#185301,#30035,#30036);
#26463=AXIS2_PLACEMENT_3D('',#185305,#30039,#30040);
#26464=AXIS2_PLACEMENT_3D('',#185308,#30041,#30042);
#26465=AXIS2_PLACEMENT_3D('',#185311,#30045,#30046);
#26466=AXIS2_PLACEMENT_3D('',#185312,#30047,#30048);
#26467=AXIS2_PLACEMENT_3D('',#185313,#30049,#30050);
#26468=AXIS2_PLACEMENT_3D('',#185316,#30051,#30052);
#26469=AXIS2_PLACEMENT_3D('',#185319,#30055,#30056);
#26470=AXIS2_PLACEMENT_3D('',#185323,#30059,#30060);
#26471=AXIS2_PLACEMENT_3D('',#185326,#30061,#30062);
#26472=AXIS2_PLACEMENT_3D('',#185329,#30065,#30066);
#26473=AXIS2_PLACEMENT_3D('',#185330,#30067,#30068);
#26474=AXIS2_PLACEMENT_3D('',#185331,#30069,#30070);
#26475=AXIS2_PLACEMENT_3D('',#185334,#30071,#30072);
#26476=AXIS2_PLACEMENT_3D('',#185337,#30075,#30076);
#26477=AXIS2_PLACEMENT_3D('',#185341,#30079,#30080);
#26478=AXIS2_PLACEMENT_3D('',#185344,#30081,#30082);
#26479=AXIS2_PLACEMENT_3D('',#185347,#30085,#30086);
#26480=AXIS2_PLACEMENT_3D('',#185348,#30087,#30088);
#26481=AXIS2_PLACEMENT_3D('',#185349,#30089,#30090);
#26482=AXIS2_PLACEMENT_3D('',#185352,#30091,#30092);
#26483=AXIS2_PLACEMENT_3D('',#185355,#30095,#30096);
#26484=AXIS2_PLACEMENT_3D('',#185359,#30099,#30100);
#26485=AXIS2_PLACEMENT_3D('',#185362,#30101,#30102);
#26486=AXIS2_PLACEMENT_3D('',#185365,#30105,#30106);
#26487=AXIS2_PLACEMENT_3D('',#185366,#30107,#30108);
#26488=AXIS2_PLACEMENT_3D('',#185367,#30109,#30110);
#26489=AXIS2_PLACEMENT_3D('',#185370,#30111,#30112);
#26490=AXIS2_PLACEMENT_3D('',#185373,#30115,#30116);
#26491=AXIS2_PLACEMENT_3D('',#185377,#30119,#30120);
#26492=AXIS2_PLACEMENT_3D('',#185380,#30121,#30122);
#26493=AXIS2_PLACEMENT_3D('',#185383,#30125,#30126);
#26494=AXIS2_PLACEMENT_3D('',#185384,#30127,#30128);
#26495=AXIS2_PLACEMENT_3D('',#185385,#30129,#30130);
#26496=AXIS2_PLACEMENT_3D('',#185388,#30131,#30132);
#26497=AXIS2_PLACEMENT_3D('',#185391,#30135,#30136);
#26498=AXIS2_PLACEMENT_3D('',#185395,#30139,#30140);
#26499=AXIS2_PLACEMENT_3D('',#185398,#30141,#30142);
#26500=AXIS2_PLACEMENT_3D('',#185401,#30145,#30146);
#26501=AXIS2_PLACEMENT_3D('',#185402,#30147,#30148);
#26502=AXIS2_PLACEMENT_3D('',#185403,#30149,#30150);
#26503=AXIS2_PLACEMENT_3D('',#185406,#30151,#30152);
#26504=AXIS2_PLACEMENT_3D('',#185409,#30155,#30156);
#26505=AXIS2_PLACEMENT_3D('',#185413,#30159,#30160);
#26506=AXIS2_PLACEMENT_3D('',#185416,#30161,#30162);
#26507=AXIS2_PLACEMENT_3D('',#185419,#30165,#30166);
#26508=AXIS2_PLACEMENT_3D('',#185420,#30167,#30168);
#26509=AXIS2_PLACEMENT_3D('',#185421,#30169,#30170);
#26510=AXIS2_PLACEMENT_3D('',#185424,#30171,#30172);
#26511=AXIS2_PLACEMENT_3D('',#185427,#30175,#30176);
#26512=AXIS2_PLACEMENT_3D('',#185431,#30179,#30180);
#26513=AXIS2_PLACEMENT_3D('',#185434,#30181,#30182);
#26514=AXIS2_PLACEMENT_3D('',#185437,#30185,#30186);
#26515=AXIS2_PLACEMENT_3D('',#185438,#30187,#30188);
#26516=AXIS2_PLACEMENT_3D('',#185439,#30189,#30190);
#26517=AXIS2_PLACEMENT_3D('',#185442,#30191,#30192);
#26518=AXIS2_PLACEMENT_3D('',#185445,#30195,#30196);
#26519=AXIS2_PLACEMENT_3D('',#185449,#30199,#30200);
#26520=AXIS2_PLACEMENT_3D('',#185452,#30201,#30202);
#26521=AXIS2_PLACEMENT_3D('',#185455,#30205,#30206);
#26522=AXIS2_PLACEMENT_3D('',#185456,#30207,#30208);
#26523=AXIS2_PLACEMENT_3D('',#185457,#30209,#30210);
#26524=AXIS2_PLACEMENT_3D('',#185460,#30211,#30212);
#26525=AXIS2_PLACEMENT_3D('',#185463,#30215,#30216);
#26526=AXIS2_PLACEMENT_3D('',#185467,#30219,#30220);
#26527=AXIS2_PLACEMENT_3D('',#185470,#30221,#30222);
#26528=AXIS2_PLACEMENT_3D('',#185473,#30225,#30226);
#26529=AXIS2_PLACEMENT_3D('',#185474,#30227,#30228);
#26530=AXIS2_PLACEMENT_3D('',#185475,#30229,#30230);
#26531=AXIS2_PLACEMENT_3D('',#185478,#30231,#30232);
#26532=AXIS2_PLACEMENT_3D('',#185481,#30235,#30236);
#26533=AXIS2_PLACEMENT_3D('',#185485,#30239,#30240);
#26534=AXIS2_PLACEMENT_3D('',#185488,#30241,#30242);
#26535=AXIS2_PLACEMENT_3D('',#185491,#30245,#30246);
#26536=AXIS2_PLACEMENT_3D('',#185492,#30247,#30248);
#26537=AXIS2_PLACEMENT_3D('',#185493,#30249,#30250);
#26538=AXIS2_PLACEMENT_3D('',#185496,#30251,#30252);
#26539=AXIS2_PLACEMENT_3D('',#185499,#30255,#30256);
#26540=AXIS2_PLACEMENT_3D('',#185503,#30259,#30260);
#26541=AXIS2_PLACEMENT_3D('',#185506,#30261,#30262);
#26542=AXIS2_PLACEMENT_3D('',#185509,#30265,#30266);
#26543=AXIS2_PLACEMENT_3D('',#185510,#30267,#30268);
#26544=AXIS2_PLACEMENT_3D('',#185511,#30269,#30270);
#26545=AXIS2_PLACEMENT_3D('',#185514,#30271,#30272);
#26546=AXIS2_PLACEMENT_3D('',#185517,#30275,#30276);
#26547=AXIS2_PLACEMENT_3D('',#185521,#30279,#30280);
#26548=AXIS2_PLACEMENT_3D('',#185524,#30281,#30282);
#26549=AXIS2_PLACEMENT_3D('',#185527,#30285,#30286);
#26550=AXIS2_PLACEMENT_3D('',#185528,#30287,#30288);
#26551=AXIS2_PLACEMENT_3D('',#185529,#30289,#30290);
#26552=AXIS2_PLACEMENT_3D('',#185532,#30291,#30292);
#26553=AXIS2_PLACEMENT_3D('',#185535,#30295,#30296);
#26554=AXIS2_PLACEMENT_3D('',#185539,#30299,#30300);
#26555=AXIS2_PLACEMENT_3D('',#185542,#30301,#30302);
#26556=AXIS2_PLACEMENT_3D('',#185545,#30305,#30306);
#26557=AXIS2_PLACEMENT_3D('',#185546,#30307,#30308);
#26558=AXIS2_PLACEMENT_3D('',#185547,#30309,#30310);
#26559=AXIS2_PLACEMENT_3D('',#185550,#30311,#30312);
#26560=AXIS2_PLACEMENT_3D('',#185553,#30315,#30316);
#26561=AXIS2_PLACEMENT_3D('',#185557,#30319,#30320);
#26562=AXIS2_PLACEMENT_3D('',#185560,#30321,#30322);
#26563=AXIS2_PLACEMENT_3D('',#185563,#30325,#30326);
#26564=AXIS2_PLACEMENT_3D('',#185564,#30327,#30328);
#26565=AXIS2_PLACEMENT_3D('',#185565,#30329,#30330);
#26566=AXIS2_PLACEMENT_3D('',#185568,#30331,#30332);
#26567=AXIS2_PLACEMENT_3D('',#185571,#30335,#30336);
#26568=AXIS2_PLACEMENT_3D('',#185575,#30339,#30340);
#26569=AXIS2_PLACEMENT_3D('',#185578,#30341,#30342);
#26570=AXIS2_PLACEMENT_3D('',#185581,#30345,#30346);
#26571=AXIS2_PLACEMENT_3D('',#185582,#30347,#30348);
#26572=AXIS2_PLACEMENT_3D('',#185583,#30349,#30350);
#26573=AXIS2_PLACEMENT_3D('',#185586,#30351,#30352);
#26574=AXIS2_PLACEMENT_3D('',#185589,#30355,#30356);
#26575=AXIS2_PLACEMENT_3D('',#185593,#30359,#30360);
#26576=AXIS2_PLACEMENT_3D('',#185596,#30361,#30362);
#26577=AXIS2_PLACEMENT_3D('',#185599,#30365,#30366);
#26578=AXIS2_PLACEMENT_3D('',#185600,#30367,#30368);
#26579=AXIS2_PLACEMENT_3D('',#185601,#30369,#30370);
#26580=AXIS2_PLACEMENT_3D('',#186839,#30375,#30376);
#26581=AXIS2_PLACEMENT_3D('',#188077,#30381,#30382);
#26582=AXIS2_PLACEMENT_3D('',#189315,#30387,#30388);
#26583=AXIS2_PLACEMENT_3D('',#190553,#30393,#30394);
#26584=AXIS2_PLACEMENT_3D('',#191791,#30399,#30400);
#26585=AXIS2_PLACEMENT_3D('',#193029,#30405,#30406);
#26586=AXIS2_PLACEMENT_3D('',#194267,#30411,#30412);
#26587=AXIS2_PLACEMENT_3D('',#195505,#30417,#30418);
#26588=AXIS2_PLACEMENT_3D('',#196743,#30423,#30424);
#26589=AXIS2_PLACEMENT_3D('',#197981,#30429,#30430);
#26590=AXIS2_PLACEMENT_3D('',#199219,#30435,#30436);
#26591=AXIS2_PLACEMENT_3D('',#200457,#30441,#30442);
#26592=AXIS2_PLACEMENT_3D('',#201695,#30447,#30448);
#26593=AXIS2_PLACEMENT_3D('',#202933,#30453,#30454);
#26594=AXIS2_PLACEMENT_3D('',#204171,#30459,#30460);
#26595=AXIS2_PLACEMENT_3D('',#205409,#30465,#30466);
#26596=AXIS2_PLACEMENT_3D('',#206647,#30471,#30472);
#26597=AXIS2_PLACEMENT_3D('',#207885,#30477,#30478);
#26598=AXIS2_PLACEMENT_3D('',#209123,#30483,#30484);
#26599=AXIS2_PLACEMENT_3D('',#210361,#30489,#30490);
#26600=AXIS2_PLACEMENT_3D('',#211599,#30495,#30496);
#26601=AXIS2_PLACEMENT_3D('',#212837,#30501,#30502);
#26602=AXIS2_PLACEMENT_3D('',#214075,#30507,#30508);
#26603=AXIS2_PLACEMENT_3D('',#214076,#30509,#30510);
#26604=AXIS2_PLACEMENT_3D('',#214077,#30511,#30512);
#26605=AXIS2_PLACEMENT_3D('',#214078,#30513,#30514);
#26606=AXIS2_PLACEMENT_3D('',#214079,#30515,#30516);
#26607=AXIS2_PLACEMENT_3D('',#214080,#30517,#30518);
#26608=AXIS2_PLACEMENT_3D('',#214081,#30519,#30520);
#26609=AXIS2_PLACEMENT_3D('',#214082,#30521,#30522);
#26610=AXIS2_PLACEMENT_3D('',#214083,#30523,#30524);
#26611=AXIS2_PLACEMENT_3D('',#214084,#30525,#30526);
#26612=AXIS2_PLACEMENT_3D('',#214085,#30527,#30528);
#26613=AXIS2_PLACEMENT_3D('',#214086,#30529,#30530);
#26614=AXIS2_PLACEMENT_3D('',#214087,#30531,#30532);
#26615=AXIS2_PLACEMENT_3D('',#214088,#30533,#30534);
#26616=AXIS2_PLACEMENT_3D('',#214089,#30535,#30536);
#26617=AXIS2_PLACEMENT_3D('',#214090,#30537,#30538);
#26618=AXIS2_PLACEMENT_3D('',#214091,#30539,#30540);
#26619=AXIS2_PLACEMENT_3D('',#214092,#30541,#30542);
#26620=AXIS2_PLACEMENT_3D('',#214093,#30543,#30544);
#26621=AXIS2_PLACEMENT_3D('',#214094,#30545,#30546);
#26622=AXIS2_PLACEMENT_3D('',#214095,#30547,#30548);
#26623=AXIS2_PLACEMENT_3D('',#214096,#30549,#30550);
#26624=AXIS2_PLACEMENT_3D('',#214097,#30551,#30552);
#26625=AXIS2_PLACEMENT_3D('',#214099,#30553,#30554);
#26626=AXIS2_PLACEMENT_3D('',#214309,#30556,#30557);
#26627=AXIS2_PLACEMENT_3D('',#214311,#30558,#30559);
#26628=AXIS2_PLACEMENT_3D('',#214313,#30560,#30561);
#26629=AXIS2_PLACEMENT_3D('',#214522,#30563,#30564);
#26630=AXIS2_PLACEMENT_3D('',#214523,#30565,#30566);
#26631=AXIS2_PLACEMENT_3D('',#214525,#30568,#30569);
#26632=AXIS2_PLACEMENT_3D('',#214526,#30570,#30571);
#26633=AXIS2_PLACEMENT_3D('',#214527,#30572,#30573);
#26634=AXIS2_PLACEMENT_3D('',#214528,#30574,#30575);
#26635=AXIS2_PLACEMENT_3D('',#214529,#30576,#30577);
#26636=AXIS2_PLACEMENT_3D('',#214530,#30578,#30579);
#26637=AXIS2_PLACEMENT_3D('',#214531,#30580,#30581);
#26638=AXIS2_PLACEMENT_3D('',#214532,#30582,#30583);
#26639=AXIS2_PLACEMENT_3D('',#214533,#30584,#30585);
#26640=AXIS2_PLACEMENT_3D('',#214534,#30586,#30587);
#26641=AXIS2_PLACEMENT_3D('',#214535,#30588,#30589);
#26642=AXIS2_PLACEMENT_3D('',#214536,#30590,#30591);
#26643=AXIS2_PLACEMENT_3D('',#214537,#30592,#30593);
#26644=AXIS2_PLACEMENT_3D('',#214538,#30594,#30595);
#26645=AXIS2_PLACEMENT_3D('',#214539,#30596,#30597);
#26646=AXIS2_PLACEMENT_3D('',#214540,#30598,#30599);
#26647=AXIS2_PLACEMENT_3D('',#214541,#30600,#30601);
#26648=AXIS2_PLACEMENT_3D('',#214542,#30602,#30603);
#26649=AXIS2_PLACEMENT_3D('',#214543,#30604,#30605);
#26650=AXIS2_PLACEMENT_3D('',#214544,#30606,#30607);
#26651=AXIS2_PLACEMENT_3D('',#214545,#30608,#30609);
#26652=AXIS2_PLACEMENT_3D('',#214546,#30610,#30611);
#26653=AXIS2_PLACEMENT_3D('',#214547,#30612,#30613);
#26654=AXIS2_PLACEMENT_3D('',#214550,#30616,#30617);
#26655=AXIS2_PLACEMENT_3D('',#214552,#30619,#30620);
#26656=AXIS2_PLACEMENT_3D('',#214555,#30623,#30624);
#26657=AXIS2_PLACEMENT_3D('',#214556,#30625,#30626);
#26658=AXIS2_PLACEMENT_3D('',#215379,#30629,#30630);
#29643=DIRECTION('axis',(0.,0.,1.));
#29644=DIRECTION('refdir',(1.,0.,0.));
#29645=DIRECTION('center_axis',(0.,1.,0.));
#29646=DIRECTION('ref_axis',(1.,0.,0.));
#29647=DIRECTION('',(0.,0.,1.));
#29648=DIRECTION('',(-1.,0.,0.));
#29649=DIRECTION('',(0.,0.,-1.));
#29650=DIRECTION('',(1.,0.,0.));
#29651=DIRECTION('center_axis',(0.,-1.,0.));
#29652=DIRECTION('ref_axis',(-1.,0.,0.));
#29653=DIRECTION('',(0.,0.,-1.));
#29654=DIRECTION('',(-1.,0.,0.));
#29655=DIRECTION('',(0.,0.,-1.));
#29656=DIRECTION('',(1.,0.,0.));
#29657=DIRECTION('center_axis',(1.,0.,0.));
#29658=DIRECTION('ref_axis',(0.,-1.,0.));
#29659=DIRECTION('',(0.,-1.,0.));
#29660=DIRECTION('',(0.,1.,0.));
#29661=DIRECTION('center_axis',(0.,0.,1.));
#29662=DIRECTION('ref_axis',(-1.,1.22464679914735E-16,0.));
#29663=DIRECTION('center_axis',(0.,0.,-1.));
#29664=DIRECTION('ref_axis',(1.,0.,0.));
#29665=DIRECTION('center_axis',(0.,0.,-1.));
#29666=DIRECTION('ref_axis',(1.,0.,0.));
#29667=DIRECTION('center_axis',(0.,0.,1.));
#29668=DIRECTION('ref_axis',(1.,0.,0.));
#29669=DIRECTION('center_axis',(0.,0.,1.));
#29670=DIRECTION('ref_axis',(1.,0.,0.));
#29671=DIRECTION('',(-0.996938396815926,-0.0781910030252308,0.));
#29672=DIRECTION('center_axis',(0.,0.,1.));
#29673=DIRECTION('ref_axis',(-0.640971010199219,-0.767565087848707,0.));
#29674=DIRECTION('center_axis',(0.,0.,1.));
#29675=DIRECTION('ref_axis',(0.996938396815926,0.0781910030252301,0.));
#29676=DIRECTION('center_axis',(0.,0.,1.));
#29677=DIRECTION('ref_axis',(-0.817790915745051,0.575515436912748,0.));
#29678=DIRECTION('',(0.983205865442321,0.182499934684418,0.));
#29679=DIRECTION('center_axis',(0.,0.,1.));
#29680=DIRECTION('ref_axis',(1.,0.,0.));
#29681=DIRECTION('',(-0.942731223965124,-0.333553353095453,0.));
#29682=DIRECTION('center_axis',(0.,0.,1.));
#29683=DIRECTION('ref_axis',(-0.420469989562974,-0.907306446509068,0.));
#29684=DIRECTION('center_axis',(0.,0.,1.));
#29685=DIRECTION('ref_axis',(0.942731223965124,0.333553353095452,0.));
#29686=DIRECTION('center_axis',(0.,0.,1.));
#29687=DIRECTION('ref_axis',(-0.93887972184625,0.34424536003541,0.));
#29688=DIRECTION('',(0.902469479163339,0.430753803440726,0.));
#29689=DIRECTION('center_axis',(0.,0.,1.));
#29690=DIRECTION('ref_axis',(1.,0.,0.));
#29691=DIRECTION('',(-0.824278476138108,-0.566184593375199,0.));
#29692=DIRECTION('center_axis',(0.,0.,1.));
#29693=DIRECTION('ref_axis',(-0.171314633997547,-0.985216370234623,0.));
#29694=DIRECTION('center_axis',(0.,0.,1.));
#29695=DIRECTION('ref_axis',(0.824278476138108,0.566184593375198,0.));
#29696=DIRECTION('center_axis',(0.,0.,1.));
#29697=DIRECTION('ref_axis',(-0.995985426475728,0.0895155307640127,0.));
#29698=DIRECTION('',(0.760231289280706,0.649652512346867,0.));
#29699=DIRECTION('center_axis',(0.,0.,1.));
#29700=DIRECTION('ref_axis',(1.,0.,0.));
#29701=DIRECTION('',(-0.649652512346868,-0.760231289280705,0.));
#29702=DIRECTION('center_axis',(0.,0.,1.));
#29703=DIRECTION('ref_axis',(0.0895155307640121,-0.995985426475728,0.));
#29704=DIRECTION('center_axis',(0.,0.,1.));
#29705=DIRECTION('ref_axis',(0.649652512346868,0.760231289280704,0.));
#29706=DIRECTION('center_axis',(0.,0.,1.));
#29707=DIRECTION('ref_axis',(-0.985216370234624,-0.171314633997546,0.));
#29708=DIRECTION('',(0.5661845933752,0.824278476138107,0.));
#29709=DIRECTION('center_axis',(0.,0.,1.));
#29710=DIRECTION('ref_axis',(1.,0.,0.));
#29711=DIRECTION('',(-0.430753803440727,-0.902469479163338,0.));
#29712=DIRECTION('center_axis',(0.,0.,1.));
#29713=DIRECTION('ref_axis',(0.344245360035413,-0.938879721846248,0.));
#29714=DIRECTION('center_axis',(0.,0.,1.));
#29715=DIRECTION('ref_axis',(0.430753803440728,0.902469479163338,0.));
#29716=DIRECTION('center_axis',(0.,0.,1.));
#29717=DIRECTION('ref_axis',(-0.907306446509064,-0.420469989562983,0.));
#29718=DIRECTION('',(0.333553353095454,0.942731223965123,0.));
#29719=DIRECTION('center_axis',(0.,0.,1.));
#29720=DIRECTION('ref_axis',(1.,0.,0.));
#29721=DIRECTION('',(-0.182499934684419,-0.983205865442321,0.));
#29722=DIRECTION('center_axis',(0.,0.,1.));
#29723=DIRECTION('ref_axis',(0.57551543691275,-0.817790915745049,0.));
#29724=DIRECTION('center_axis',(0.,0.,1.));
#29725=DIRECTION('ref_axis',(0.18249993468442,0.983205865442321,0.));
#29726=DIRECTION('center_axis',(0.,0.,1.));
#29727=DIRECTION('ref_axis',(-0.767565087848706,-0.640971010199219,0.));
#29728=DIRECTION('',(0.0781910030252323,0.996938396815926,0.));
#29729=DIRECTION('center_axis',(0.,0.,1.));
#29730=DIRECTION('ref_axis',(1.,0.,0.));
#29731=DIRECTION('',(0.0781910030252308,-0.996938396815926,0.));
#29732=DIRECTION('center_axis',(0.,0.,1.));
#29733=DIRECTION('ref_axis',(0.767565087848708,-0.640971010199218,0.));
#29734=DIRECTION('center_axis',(0.,0.,1.));
#29735=DIRECTION('ref_axis',(-0.0781910030252301,0.996938396815926,0.));
#29736=DIRECTION('center_axis',(0.,0.,1.));
#29737=DIRECTION('ref_axis',(-0.575515436912748,-0.817790915745051,0.));
#29738=DIRECTION('',(-0.182499934684418,0.983205865442321,0.));
#29739=DIRECTION('center_axis',(0.,0.,1.));
#29740=DIRECTION('ref_axis',(1.,0.,0.));
#29741=DIRECTION('',(0.333553353095453,-0.942731223965124,0.));
#29742=DIRECTION('center_axis',(0.,0.,1.));
#29743=DIRECTION('ref_axis',(0.907306446509069,-0.420469989562973,0.));
#29744=DIRECTION('center_axis',(0.,0.,1.));
#29745=DIRECTION('ref_axis',(-0.333553353095452,0.942731223965124,0.));
#29746=DIRECTION('center_axis',(0.,0.,1.));
#29747=DIRECTION('ref_axis',(-0.34424536003541,-0.93887972184625,0.));
#29748=DIRECTION('',(-0.430753803440726,0.902469479163339,0.));
#29749=DIRECTION('center_axis',(0.,0.,1.));
#29750=DIRECTION('ref_axis',(1.,0.,0.));
#29751=DIRECTION('',(0.566184593375199,-0.824278476138108,0.));
#29752=DIRECTION('center_axis',(0.,0.,1.));
#29753=DIRECTION('ref_axis',(0.985216370234623,-0.171314633997547,0.));
#29754=DIRECTION('center_axis',(0.,0.,1.));
#29755=DIRECTION('ref_axis',(-0.566184593375198,0.824278476138108,0.));
#29756=DIRECTION('center_axis',(0.,0.,1.));
#29757=DIRECTION('ref_axis',(-0.0895155307640188,-0.995985426475727,0.));
#29758=DIRECTION('',(-0.649652512346867,0.760231289280706,0.));
#29759=DIRECTION('center_axis',(0.,0.,1.));
#29760=DIRECTION('ref_axis',(1.,0.,0.));
#29761=DIRECTION('',(0.760231289280705,-0.649652512346868,0.));
#29762=DIRECTION('center_axis',(0.,0.,1.));
#29763=DIRECTION('ref_axis',(0.995985426475728,0.0895155307640127,0.));
#29764=DIRECTION('center_axis',(0.,0.,1.));
#29765=DIRECTION('ref_axis',(-0.760231289280704,0.649652512346868,0.));
#29766=DIRECTION('center_axis',(0.,0.,1.));
#29767=DIRECTION('ref_axis',(0.171314633997546,-0.985216370234624,0.));
#29768=DIRECTION('',(-0.824278476138107,0.5661845933752,0.));
#29769=DIRECTION('center_axis',(0.,0.,1.));
#29770=DIRECTION('ref_axis',(1.,0.,0.));
#29771=DIRECTION('',(0.902469479163338,-0.430753803440727,0.));
#29772=DIRECTION('center_axis',(0.,0.,1.));
#29773=DIRECTION('ref_axis',(0.93887972184625,0.344245360035408,0.));
#29774=DIRECTION('center_axis',(0.,0.,1.));
#29775=DIRECTION('ref_axis',(-0.902469479163338,0.430753803440728,0.));
#29776=DIRECTION('center_axis',(0.,0.,1.));
#29777=DIRECTION('ref_axis',(0.420469989562984,-0.907306446509064,0.));
#29778=DIRECTION('',(-0.942731223965123,0.333553353095454,0.));
#29779=DIRECTION('center_axis',(0.,0.,1.));
#29780=DIRECTION('ref_axis',(1.,0.,0.));
#29781=DIRECTION('',(0.983205865442321,-0.182499934684419,0.));
#29782=DIRECTION('center_axis',(0.,0.,1.));
#29783=DIRECTION('ref_axis',(0.817790915745049,0.57551543691275,0.));
#29784=DIRECTION('center_axis',(0.,0.,1.));
#29785=DIRECTION('ref_axis',(-0.983205865442321,0.18249993468442,0.));
#29786=DIRECTION('center_axis',(0.,0.,1.));
#29787=DIRECTION('ref_axis',(0.640971010199219,-0.767565087848706,0.));
#29788=DIRECTION('',(-0.996938396815926,0.0781910030252323,0.));
#29789=DIRECTION('center_axis',(0.,0.,1.));
#29790=DIRECTION('ref_axis',(1.,0.,0.));
#29791=DIRECTION('',(0.996938396815926,0.0781910030252307,0.));
#29792=DIRECTION('center_axis',(0.,0.,1.));
#29793=DIRECTION('ref_axis',(0.64097101019921,0.767565087848714,0.));
#29794=DIRECTION('center_axis',(0.,0.,1.));
#29795=DIRECTION('ref_axis',(-0.996938396815926,-0.07819100302523,0.));
#29796=DIRECTION('center_axis',(0.,0.,1.));
#29797=DIRECTION('ref_axis',(0.817790915745051,-0.575515436912747,0.));
#29798=DIRECTION('',(-0.983205865442321,-0.182499934684417,0.));
#29799=DIRECTION('center_axis',(0.,0.,1.));
#29800=DIRECTION('ref_axis',(1.,0.,0.));
#29801=DIRECTION('',(0.942731223965124,0.333553353095453,0.));
#29802=DIRECTION('center_axis',(0.,0.,1.));
#29803=DIRECTION('ref_axis',(0.420469989562982,0.907306446509065,0.));
#29804=DIRECTION('center_axis',(0.,0.,1.));
#29805=DIRECTION('ref_axis',(-0.942731223965124,-0.333553353095452,0.));
#29806=DIRECTION('center_axis',(0.,0.,1.));
#29807=DIRECTION('ref_axis',(0.93887972184625,-0.344245360035407,0.));
#29808=DIRECTION('',(-0.902469479163339,-0.430753803440726,0.));
#29809=DIRECTION('center_axis',(0.,0.,1.));
#29810=DIRECTION('ref_axis',(1.,0.,0.));
#29811=DIRECTION('',(0.824278476138108,0.566184593375198,0.));
#29812=DIRECTION('center_axis',(0.,0.,1.));
#29813=DIRECTION('ref_axis',(0.17131463399754,0.985216370234625,0.));
#29814=DIRECTION('center_axis',(0.,0.,1.));
#29815=DIRECTION('ref_axis',(-0.824278476138108,-0.566184593375198,0.));
#29816=DIRECTION('center_axis',(0.,0.,1.));
#29817=DIRECTION('ref_axis',(0.995985426475728,-0.0895155307640127,0.));
#29818=DIRECTION('',(-0.760231289280706,-0.649652512346867,0.));
#29819=DIRECTION('center_axis',(0.,0.,1.));
#29820=DIRECTION('ref_axis',(1.,0.,0.));
#29821=DIRECTION('',(0.649652512346868,0.760231289280705,0.));
#29822=DIRECTION('center_axis',(0.,0.,1.));
#29823=DIRECTION('ref_axis',(-0.0895155307640188,0.995985426475727,0.));
#29824=DIRECTION('center_axis',(0.,0.,1.));
#29825=DIRECTION('ref_axis',(-0.649652512346869,-0.760231289280704,0.));
#29826=DIRECTION('center_axis',(0.,0.,1.));
#29827=DIRECTION('ref_axis',(0.985216370234623,0.171314633997547,0.));
#29828=DIRECTION('',(-0.5661845933752,-0.824278476138107,0.));
#29829=DIRECTION('center_axis',(0.,0.,1.));
#29830=DIRECTION('ref_axis',(1.,0.,0.));
#29831=DIRECTION('',(0.430753803440728,0.902469479163338,0.));
#29832=DIRECTION('center_axis',(0.,0.,1.));
#29833=DIRECTION('ref_axis',(-0.344245360035407,0.93887972184625,0.));
#29834=DIRECTION('center_axis',(0.,0.,1.));
#29835=DIRECTION('ref_axis',(-0.430753803440728,-0.902469479163338,0.));
#29836=DIRECTION('center_axis',(0.,0.,1.));
#29837=DIRECTION('ref_axis',(0.907306446509064,0.420469989562984,0.));
#29838=DIRECTION('',(-0.333553353095455,-0.942731223965123,0.));
#29839=DIRECTION('center_axis',(0.,0.,1.));
#29840=DIRECTION('ref_axis',(1.,0.,0.));
#29841=DIRECTION('',(0.182499934684419,0.983205865442321,0.));
#29842=DIRECTION('center_axis',(0.,0.,1.));
#29843=DIRECTION('ref_axis',(-0.575515436912756,0.817790915745045,0.));
#29844=DIRECTION('center_axis',(0.,0.,1.));
#29845=DIRECTION('ref_axis',(-0.18249993468442,-0.983205865442321,0.));
#29846=DIRECTION('center_axis',(0.,0.,1.));
#29847=DIRECTION('ref_axis',(0.767565087848712,0.640971010199212,0.));
#29848=DIRECTION('',(-0.0781910030252327,-0.996938396815926,0.));
#29849=DIRECTION('center_axis',(0.,0.,1.));
#29850=DIRECTION('ref_axis',(1.,0.,0.));
#29851=DIRECTION('',(-0.0781910030252307,0.996938396815926,0.));
#29852=DIRECTION('center_axis',(0.,0.,1.));
#29853=DIRECTION('ref_axis',(-0.767565087848714,0.64097101019921,0.));
#29854=DIRECTION('center_axis',(0.,0.,1.));
#29855=DIRECTION('ref_axis',(0.07819100302523,-0.996938396815926,0.));
#29856=DIRECTION('center_axis',(0.,0.,1.));
#29857=DIRECTION('ref_axis',(0.575515436912747,0.817790915745051,0.));
#29858=DIRECTION('',(0.182499934684417,-0.983205865442321,0.));
#29859=DIRECTION('center_axis',(0.,0.,1.));
#29860=DIRECTION('ref_axis',(1.,0.,0.));
#29861=DIRECTION('',(-0.333553353095453,0.942731223965124,0.));
#29862=DIRECTION('center_axis',(0.,0.,1.));
#29863=DIRECTION('ref_axis',(-0.907306446509064,0.420469989562983,0.));
#29864=DIRECTION('center_axis',(0.,0.,1.));
#29865=DIRECTION('ref_axis',(0.333553353095452,-0.942731223965124,0.));
#29866=DIRECTION('center_axis',(0.,0.,1.));
#29867=DIRECTION('ref_axis',(0.344245360035407,0.938879721846251,0.));
#29868=DIRECTION('',(0.430753803440726,-0.902469479163339,0.));
#29869=DIRECTION('center_axis',(0.,0.,1.));
#29870=DIRECTION('ref_axis',(1.,0.,0.));
#29871=DIRECTION('',(-0.566184593375198,0.824278476138108,0.));
#29872=DIRECTION('center_axis',(0.,0.,1.));
#29873=DIRECTION('ref_axis',(-0.985216370234624,0.171314633997541,0.));
#29874=DIRECTION('center_axis',(0.,0.,1.));
#29875=DIRECTION('ref_axis',(0.566184593375197,-0.824278476138108,0.));
#29876=DIRECTION('center_axis',(0.,0.,1.));
#29877=DIRECTION('ref_axis',(0.0895155307640188,0.995985426475727,0.));
#29878=DIRECTION('',(0.649652512346866,-0.760231289280706,0.));
#29879=DIRECTION('center_axis',(0.,0.,1.));
#29880=DIRECTION('ref_axis',(1.,0.,0.));
#29881=DIRECTION('',(-0.760231289280705,0.649652512346868,0.));
#29882=DIRECTION('center_axis',(0.,0.,1.));
#29883=DIRECTION('ref_axis',(-0.995985426475728,-0.0895155307640121,0.));
#29884=DIRECTION('center_axis',(0.,0.,1.));
#29885=DIRECTION('ref_axis',(0.760231289280704,-0.649652512346868,0.));
#29886=DIRECTION('center_axis',(0.,0.,1.));
#29887=DIRECTION('ref_axis',(-0.171314633997541,0.985216370234624,0.));
#29888=DIRECTION('',(0.824278476138107,-0.5661845933752,0.));
#29889=DIRECTION('center_axis',(0.,0.,1.));
#29890=DIRECTION('ref_axis',(1.,0.,0.));
#29891=DIRECTION('',(-0.902469479163338,0.430753803440728,0.));
#29892=DIRECTION('center_axis',(0.,0.,1.));
#29893=DIRECTION('ref_axis',(-0.93887972184625,-0.344245360035407,0.));
#29894=DIRECTION('center_axis',(0.,0.,1.));
#29895=DIRECTION('ref_axis',(0.902469479163338,-0.430753803440728,0.));
#29896=DIRECTION('center_axis',(0.,0.,1.));
#29897=DIRECTION('ref_axis',(-0.420469989562984,0.907306446509064,0.));
#29898=DIRECTION('',(0.942731223965123,-0.333553353095455,0.));
#29899=DIRECTION('center_axis',(0.,0.,1.));
#29900=DIRECTION('ref_axis',(1.,0.,0.));
#29901=DIRECTION('',(-0.983205865442321,0.182499934684419,0.));
#29902=DIRECTION('center_axis',(0.,0.,1.));
#29903=DIRECTION('ref_axis',(-0.817790915745045,-0.575515436912756,0.));
#29904=DIRECTION('center_axis',(0.,0.,1.));
#29905=DIRECTION('ref_axis',(0.983205865442321,-0.18249993468442,0.));
#29906=DIRECTION('center_axis',(0.,0.,1.));
#29907=DIRECTION('ref_axis',(-0.640971010199212,0.767565087848712,0.));
#29908=DIRECTION('',(0.996938396815926,-0.0781910030252328,0.));
#29909=DIRECTION('center_axis',(0.,0.,1.));
#29910=DIRECTION('ref_axis',(-0.640971010199212,0.767565087848712,0.));
#29911=DIRECTION('center_axis',(0.,0.,-1.));
#29912=DIRECTION('ref_axis',(-0.640971010199212,0.767565087848712,0.));
#29913=DIRECTION('',(0.,0.,1.));
#29914=DIRECTION('',(0.,0.,-1.));
#29915=DIRECTION('center_axis',(0.0781910030252328,0.996938396815926,0.));
#29916=DIRECTION('ref_axis',(-0.996938396815926,0.0781910030252328,0.));
#29917=DIRECTION('',(-0.996938396815926,0.0781910030252328,0.));
#29918=DIRECTION('',(0.,0.,1.));
#29919=DIRECTION('center_axis',(0.,0.,1.));
#29920=DIRECTION('ref_axis',(-0.817790915745045,-0.575515436912756,0.));
#29921=DIRECTION('center_axis',(0.,0.,-1.));
#29922=DIRECTION('ref_axis',(-0.817790915745045,-0.575515436912756,0.));
#29923=DIRECTION('',(0.,0.,1.));
#29924=DIRECTION('',(0.,0.,-1.));
#29925=DIRECTION('center_axis',(0.,0.,1.));
#29926=DIRECTION('ref_axis',(0.983205865442321,-0.18249993468442,0.));
#29927=DIRECTION('center_axis',(0.,0.,-1.));
#29928=DIRECTION('ref_axis',(0.983205865442321,-0.18249993468442,0.));
#29929=DIRECTION('center_axis',(0.,0.,1.));
#29930=DIRECTION('ref_axis',(-0.420469989562984,0.907306446509064,0.));
#29931=DIRECTION('center_axis',(0.,0.,-1.));
#29932=DIRECTION('ref_axis',(-0.420469989562984,0.907306446509064,0.));
#29933=DIRECTION('',(0.,0.,1.));
#29934=DIRECTION('',(0.,0.,-1.));
#29935=DIRECTION('center_axis',(0.333553353095455,0.942731223965123,0.));
#29936=DIRECTION('ref_axis',(-0.942731223965123,0.333553353095455,0.));
#29937=DIRECTION('',(-0.942731223965123,0.333553353095455,0.));
#29938=DIRECTION('',(0.,0.,1.));
#29939=DIRECTION('center_axis',(0.,0.,1.));
#29940=DIRECTION('ref_axis',(-0.93887972184625,-0.344245360035407,0.));
#29941=DIRECTION('center_axis',(0.,0.,-1.));
#29942=DIRECTION('ref_axis',(-0.93887972184625,-0.344245360035407,0.));
#29943=DIRECTION('',(0.,0.,1.));
#29944=DIRECTION('',(0.,0.,-1.));
#29945=DIRECTION('center_axis',(0.,0.,1.));
#29946=DIRECTION('ref_axis',(0.902469479163338,-0.430753803440728,0.));
#29947=DIRECTION('center_axis',(0.,0.,-1.));
#29948=DIRECTION('ref_axis',(0.902469479163338,-0.430753803440728,0.));
#29949=DIRECTION('center_axis',(0.,0.,1.));
#29950=DIRECTION('ref_axis',(-0.171314633997541,0.985216370234624,0.));
#29951=DIRECTION('center_axis',(0.,0.,-1.));
#29952=DIRECTION('ref_axis',(-0.171314633997541,0.985216370234624,0.));
#29953=DIRECTION('',(0.,0.,1.));
#29954=DIRECTION('',(0.,0.,-1.));
#29955=DIRECTION('center_axis',(0.5661845933752,0.824278476138107,0.));
#29956=DIRECTION('ref_axis',(-0.824278476138107,0.5661845933752,0.));
#29957=DIRECTION('',(-0.824278476138107,0.5661845933752,0.));
#29958=DIRECTION('',(0.,0.,1.));
#29959=DIRECTION('center_axis',(0.,0.,1.));
#29960=DIRECTION('ref_axis',(-0.995985426475728,-0.0895155307640121,0.));
#29961=DIRECTION('center_axis',(0.,0.,-1.));
#29962=DIRECTION('ref_axis',(-0.995985426475728,-0.0895155307640121,0.));
#29963=DIRECTION('',(0.,0.,1.));
#29964=DIRECTION('',(0.,0.,-1.));
#29965=DIRECTION('center_axis',(0.,0.,1.));
#29966=DIRECTION('ref_axis',(0.760231289280704,-0.649652512346868,0.));
#29967=DIRECTION('center_axis',(0.,0.,-1.));
#29968=DIRECTION('ref_axis',(0.760231289280704,-0.649652512346868,0.));
#29969=DIRECTION('center_axis',(0.,0.,1.));
#29970=DIRECTION('ref_axis',(0.0895155307640188,0.995985426475727,0.));
#29971=DIRECTION('center_axis',(0.,0.,-1.));
#29972=DIRECTION('ref_axis',(0.0895155307640188,0.995985426475727,0.));
#29973=DIRECTION('',(0.,0.,1.));
#29974=DIRECTION('',(0.,0.,-1.));
#29975=DIRECTION('center_axis',(0.760231289280706,0.649652512346866,0.));
#29976=DIRECTION('ref_axis',(-0.649652512346866,0.760231289280706,0.));
#29977=DIRECTION('',(-0.649652512346866,0.760231289280706,0.));
#29978=DIRECTION('',(0.,0.,1.));
#29979=DIRECTION('center_axis',(0.,0.,1.));
#29980=DIRECTION('ref_axis',(-0.985216370234624,0.171314633997541,0.));
#29981=DIRECTION('center_axis',(0.,0.,-1.));
#29982=DIRECTION('ref_axis',(-0.985216370234624,0.171314633997541,0.));
#29983=DIRECTION('',(0.,0.,1.));
#29984=DIRECTION('',(0.,0.,-1.));
#29985=DIRECTION('center_axis',(0.,0.,1.));
#29986=DIRECTION('ref_axis',(0.566184593375197,-0.824278476138108,0.));
#29987=DIRECTION('center_axis',(0.,0.,-1.));
#29988=DIRECTION('ref_axis',(0.566184593375197,-0.824278476138108,0.));
#29989=DIRECTION('center_axis',(0.,0.,1.));
#29990=DIRECTION('ref_axis',(0.344245360035407,0.938879721846251,0.));
#29991=DIRECTION('center_axis',(0.,0.,-1.));
#29992=DIRECTION('ref_axis',(0.344245360035407,0.938879721846251,0.));
#29993=DIRECTION('',(0.,0.,1.));
#29994=DIRECTION('',(0.,0.,-1.));
#29995=DIRECTION('center_axis',(0.902469479163339,0.430753803440726,0.));
#29996=DIRECTION('ref_axis',(-0.430753803440726,0.902469479163339,0.));
#29997=DIRECTION('',(-0.430753803440726,0.902469479163339,0.));
#29998=DIRECTION('',(0.,0.,1.));
#29999=DIRECTION('center_axis',(0.,0.,1.));
#30000=DIRECTION('ref_axis',(-0.907306446509064,0.420469989562983,0.));
#30001=DIRECTION('center_axis',(0.,0.,-1.));
#30002=DIRECTION('ref_axis',(-0.907306446509064,0.420469989562983,0.));
#30003=DIRECTION('',(0.,0.,1.));
#30004=DIRECTION('',(0.,0.,-1.));
#30005=DIRECTION('center_axis',(0.,0.,1.));
#30006=DIRECTION('ref_axis',(0.333553353095452,-0.942731223965124,0.));
#30007=DIRECTION('center_axis',(0.,0.,-1.));
#30008=DIRECTION('ref_axis',(0.333553353095452,-0.942731223965124,0.));
#30009=DIRECTION('center_axis',(0.,0.,1.));
#30010=DIRECTION('ref_axis',(0.575515436912747,0.817790915745051,0.));
#30011=DIRECTION('center_axis',(0.,0.,-1.));
#30012=DIRECTION('ref_axis',(0.575515436912747,0.817790915745051,0.));
#30013=DIRECTION('',(0.,0.,1.));
#30014=DIRECTION('',(0.,0.,-1.));
#30015=DIRECTION('center_axis',(0.983205865442321,0.182499934684417,0.));
#30016=DIRECTION('ref_axis',(-0.182499934684417,0.983205865442321,0.));
#30017=DIRECTION('',(-0.182499934684417,0.983205865442321,0.));
#30018=DIRECTION('',(0.,0.,1.));
#30019=DIRECTION('center_axis',(0.,0.,1.));
#30020=DIRECTION('ref_axis',(-0.767565087848714,0.64097101019921,0.));
#30021=DIRECTION('center_axis',(0.,0.,-1.));
#30022=DIRECTION('ref_axis',(-0.767565087848714,0.64097101019921,0.));
#30023=DIRECTION('',(0.,0.,1.));
#30024=DIRECTION('',(0.,0.,-1.));
#30025=DIRECTION('center_axis',(0.,0.,1.));
#30026=DIRECTION('ref_axis',(0.07819100302523,-0.996938396815926,0.));
#30027=DIRECTION('center_axis',(0.,0.,-1.));
#30028=DIRECTION('ref_axis',(0.07819100302523,-0.996938396815926,0.));
#30029=DIRECTION('center_axis',(0.,0.,1.));
#30030=DIRECTION('ref_axis',(0.767565087848712,0.640971010199212,0.));
#30031=DIRECTION('center_axis',(0.,0.,-1.));
#30032=DIRECTION('ref_axis',(0.767565087848712,0.640971010199212,0.));
#30033=DIRECTION('',(0.,0.,1.));
#30034=DIRECTION('',(0.,0.,-1.));
#30035=DIRECTION('center_axis',(0.996938396815926,-0.0781910030252327,0.));
#30036=DIRECTION('ref_axis',(0.0781910030252327,0.996938396815926,0.));
#30037=DIRECTION('',(0.0781910030252327,0.996938396815926,0.));
#30038=DIRECTION('',(0.,0.,1.));
#30039=DIRECTION('center_axis',(0.,0.,1.));
#30040=DIRECTION('ref_axis',(-0.575515436912756,0.817790915745045,0.));
#30041=DIRECTION('center_axis',(0.,0.,-1.));
#30042=DIRECTION('ref_axis',(-0.575515436912756,0.817790915745045,0.));
#30043=DIRECTION('',(0.,0.,1.));
#30044=DIRECTION('',(0.,0.,-1.));
#30045=DIRECTION('center_axis',(0.,0.,1.));
#30046=DIRECTION('ref_axis',(-0.18249993468442,-0.983205865442321,0.));
#30047=DIRECTION('center_axis',(0.,0.,-1.));
#30048=DIRECTION('ref_axis',(-0.18249993468442,-0.983205865442321,0.));
#30049=DIRECTION('center_axis',(0.,0.,1.));
#30050=DIRECTION('ref_axis',(0.907306446509064,0.420469989562984,0.));
#30051=DIRECTION('center_axis',(0.,0.,-1.));
#30052=DIRECTION('ref_axis',(0.907306446509064,0.420469989562984,0.));
#30053=DIRECTION('',(0.,0.,1.));
#30054=DIRECTION('',(0.,0.,-1.));
#30055=DIRECTION('center_axis',(0.942731223965123,-0.333553353095455,0.));
#30056=DIRECTION('ref_axis',(0.333553353095455,0.942731223965123,0.));
#30057=DIRECTION('',(0.333553353095455,0.942731223965123,0.));
#30058=DIRECTION('',(0.,0.,1.));
#30059=DIRECTION('center_axis',(0.,0.,1.));
#30060=DIRECTION('ref_axis',(-0.344245360035407,0.93887972184625,0.));
#30061=DIRECTION('center_axis',(0.,0.,-1.));
#30062=DIRECTION('ref_axis',(-0.344245360035407,0.93887972184625,0.));
#30063=DIRECTION('',(0.,0.,1.));
#30064=DIRECTION('',(0.,0.,-1.));
#30065=DIRECTION('center_axis',(0.,0.,1.));
#30066=DIRECTION('ref_axis',(-0.430753803440728,-0.902469479163338,0.));
#30067=DIRECTION('center_axis',(0.,0.,-1.));
#30068=DIRECTION('ref_axis',(-0.430753803440728,-0.902469479163338,0.));
#30069=DIRECTION('center_axis',(0.,0.,1.));
#30070=DIRECTION('ref_axis',(0.985216370234623,0.171314633997547,0.));
#30071=DIRECTION('center_axis',(0.,0.,-1.));
#30072=DIRECTION('ref_axis',(0.985216370234623,0.171314633997547,0.));
#30073=DIRECTION('',(0.,0.,1.));
#30074=DIRECTION('',(0.,0.,-1.));
#30075=DIRECTION('center_axis',(0.824278476138107,-0.5661845933752,0.));
#30076=DIRECTION('ref_axis',(0.5661845933752,0.824278476138107,0.));
#30077=DIRECTION('',(0.5661845933752,0.824278476138107,0.));
#30078=DIRECTION('',(0.,0.,1.));
#30079=DIRECTION('center_axis',(0.,0.,1.));
#30080=DIRECTION('ref_axis',(-0.0895155307640188,0.995985426475727,0.));
#30081=DIRECTION('center_axis',(0.,0.,-1.));
#30082=DIRECTION('ref_axis',(-0.0895155307640188,0.995985426475727,0.));
#30083=DIRECTION('',(0.,0.,1.));
#30084=DIRECTION('',(0.,0.,-1.));
#30085=DIRECTION('center_axis',(0.,0.,1.));
#30086=DIRECTION('ref_axis',(-0.649652512346869,-0.760231289280704,0.));
#30087=DIRECTION('center_axis',(0.,0.,-1.));
#30088=DIRECTION('ref_axis',(-0.649652512346869,-0.760231289280704,0.));
#30089=DIRECTION('center_axis',(0.,0.,1.));
#30090=DIRECTION('ref_axis',(0.995985426475728,-0.0895155307640127,0.));
#30091=DIRECTION('center_axis',(0.,0.,-1.));
#30092=DIRECTION('ref_axis',(0.995985426475728,-0.0895155307640127,0.));
#30093=DIRECTION('',(0.,0.,1.));
#30094=DIRECTION('',(0.,0.,-1.));
#30095=DIRECTION('center_axis',(0.649652512346867,-0.760231289280706,0.));
#30096=DIRECTION('ref_axis',(0.760231289280706,0.649652512346867,0.));
#30097=DIRECTION('',(0.760231289280706,0.649652512346867,0.));
#30098=DIRECTION('',(0.,0.,1.));
#30099=DIRECTION('center_axis',(0.,0.,1.));
#30100=DIRECTION('ref_axis',(0.17131463399754,0.985216370234625,0.));
#30101=DIRECTION('center_axis',(0.,0.,-1.));
#30102=DIRECTION('ref_axis',(0.17131463399754,0.985216370234625,0.));
#30103=DIRECTION('',(0.,0.,1.));
#30104=DIRECTION('',(0.,0.,-1.));
#30105=DIRECTION('center_axis',(0.,0.,1.));
#30106=DIRECTION('ref_axis',(-0.824278476138108,-0.566184593375198,0.));
#30107=DIRECTION('center_axis',(0.,0.,-1.));
#30108=DIRECTION('ref_axis',(-0.824278476138108,-0.566184593375198,0.));
#30109=DIRECTION('center_axis',(0.,0.,1.));
#30110=DIRECTION('ref_axis',(0.93887972184625,-0.344245360035407,0.));
#30111=DIRECTION('center_axis',(0.,0.,-1.));
#30112=DIRECTION('ref_axis',(0.93887972184625,-0.344245360035407,0.));
#30113=DIRECTION('',(0.,0.,1.));
#30114=DIRECTION('',(0.,0.,-1.));
#30115=DIRECTION('center_axis',(0.430753803440726,-0.902469479163339,0.));
#30116=DIRECTION('ref_axis',(0.902469479163339,0.430753803440726,0.));
#30117=DIRECTION('',(0.902469479163339,0.430753803440726,0.));
#30118=DIRECTION('',(0.,0.,1.));
#30119=DIRECTION('center_axis',(0.,0.,1.));
#30120=DIRECTION('ref_axis',(0.420469989562982,0.907306446509065,0.));
#30121=DIRECTION('center_axis',(0.,0.,-1.));
#30122=DIRECTION('ref_axis',(0.420469989562982,0.907306446509065,0.));
#30123=DIRECTION('',(0.,0.,1.));
#30124=DIRECTION('',(0.,0.,-1.));
#30125=DIRECTION('center_axis',(0.,0.,1.));
#30126=DIRECTION('ref_axis',(-0.942731223965124,-0.333553353095452,0.));
#30127=DIRECTION('center_axis',(0.,0.,-1.));
#30128=DIRECTION('ref_axis',(-0.942731223965124,-0.333553353095452,0.));
#30129=DIRECTION('center_axis',(0.,0.,1.));
#30130=DIRECTION('ref_axis',(0.817790915745051,-0.575515436912747,0.));
#30131=DIRECTION('center_axis',(0.,0.,-1.));
#30132=DIRECTION('ref_axis',(0.817790915745051,-0.575515436912747,0.));
#30133=DIRECTION('',(0.,0.,1.));
#30134=DIRECTION('',(0.,0.,-1.));
#30135=DIRECTION('center_axis',(0.182499934684417,-0.983205865442321,0.));
#30136=DIRECTION('ref_axis',(0.983205865442321,0.182499934684417,0.));
#30137=DIRECTION('',(0.983205865442321,0.182499934684417,0.));
#30138=DIRECTION('',(0.,0.,1.));
#30139=DIRECTION('center_axis',(0.,0.,1.));
#30140=DIRECTION('ref_axis',(0.64097101019921,0.767565087848714,0.));
#30141=DIRECTION('center_axis',(0.,0.,-1.));
#30142=DIRECTION('ref_axis',(0.64097101019921,0.767565087848714,0.));
#30143=DIRECTION('',(0.,0.,1.));
#30144=DIRECTION('',(0.,0.,-1.));
#30145=DIRECTION('center_axis',(0.,0.,1.));
#30146=DIRECTION('ref_axis',(-0.996938396815926,-0.07819100302523,0.));
#30147=DIRECTION('center_axis',(0.,0.,-1.));
#30148=DIRECTION('ref_axis',(-0.996938396815926,-0.07819100302523,0.));
#30149=DIRECTION('center_axis',(0.,0.,1.));
#30150=DIRECTION('ref_axis',(0.640971010199219,-0.767565087848706,0.));
#30151=DIRECTION('center_axis',(0.,0.,-1.));
#30152=DIRECTION('ref_axis',(0.640971010199219,-0.767565087848706,0.));
#30153=DIRECTION('',(0.,0.,1.));
#30154=DIRECTION('',(0.,0.,-1.));
#30155=DIRECTION('center_axis',(-0.0781910030252323,-0.996938396815926,
0.));
#30156=DIRECTION('ref_axis',(0.996938396815926,-0.0781910030252323,0.));
#30157=DIRECTION('',(0.996938396815926,-0.0781910030252323,0.));
#30158=DIRECTION('',(0.,0.,1.));
#30159=DIRECTION('center_axis',(0.,0.,1.));
#30160=DIRECTION('ref_axis',(0.817790915745049,0.57551543691275,0.));
#30161=DIRECTION('center_axis',(0.,0.,-1.));
#30162=DIRECTION('ref_axis',(0.817790915745049,0.57551543691275,0.));
#30163=DIRECTION('',(0.,0.,1.));
#30164=DIRECTION('',(0.,0.,-1.));
#30165=DIRECTION('center_axis',(0.,0.,1.));
#30166=DIRECTION('ref_axis',(-0.983205865442321,0.18249993468442,0.));
#30167=DIRECTION('center_axis',(0.,0.,-1.));
#30168=DIRECTION('ref_axis',(-0.983205865442321,0.18249993468442,0.));
#30169=DIRECTION('center_axis',(0.,0.,1.));
#30170=DIRECTION('ref_axis',(0.420469989562984,-0.907306446509064,0.));
#30171=DIRECTION('center_axis',(0.,0.,-1.));
#30172=DIRECTION('ref_axis',(0.420469989562984,-0.907306446509064,0.));
#30173=DIRECTION('',(0.,0.,1.));
#30174=DIRECTION('',(0.,0.,-1.));
#30175=DIRECTION('center_axis',(-0.333553353095454,-0.942731223965123,0.));
#30176=DIRECTION('ref_axis',(0.942731223965123,-0.333553353095454,0.));
#30177=DIRECTION('',(0.942731223965123,-0.333553353095454,0.));
#30178=DIRECTION('',(0.,0.,1.));
#30179=DIRECTION('center_axis',(0.,0.,1.));
#30180=DIRECTION('ref_axis',(0.93887972184625,0.344245360035408,0.));
#30181=DIRECTION('center_axis',(0.,0.,-1.));
#30182=DIRECTION('ref_axis',(0.93887972184625,0.344245360035408,0.));
#30183=DIRECTION('',(0.,0.,1.));
#30184=DIRECTION('',(0.,0.,-1.));
#30185=DIRECTION('center_axis',(0.,0.,1.));
#30186=DIRECTION('ref_axis',(-0.902469479163338,0.430753803440728,0.));
#30187=DIRECTION('center_axis',(0.,0.,-1.));
#30188=DIRECTION('ref_axis',(-0.902469479163338,0.430753803440728,0.));
#30189=DIRECTION('center_axis',(0.,0.,1.));
#30190=DIRECTION('ref_axis',(0.171314633997546,-0.985216370234624,0.));
#30191=DIRECTION('center_axis',(0.,0.,-1.));
#30192=DIRECTION('ref_axis',(0.171314633997546,-0.985216370234624,0.));
#30193=DIRECTION('',(0.,0.,1.));
#30194=DIRECTION('',(0.,0.,-1.));
#30195=DIRECTION('center_axis',(-0.5661845933752,-0.824278476138107,0.));
#30196=DIRECTION('ref_axis',(0.824278476138107,-0.5661845933752,0.));
#30197=DIRECTION('',(0.824278476138107,-0.5661845933752,0.));
#30198=DIRECTION('',(0.,0.,1.));
#30199=DIRECTION('center_axis',(0.,0.,1.));
#30200=DIRECTION('ref_axis',(0.995985426475728,0.0895155307640127,0.));
#30201=DIRECTION('center_axis',(0.,0.,-1.));
#30202=DIRECTION('ref_axis',(0.995985426475728,0.0895155307640127,0.));
#30203=DIRECTION('',(0.,0.,1.));
#30204=DIRECTION('',(0.,0.,-1.));
#30205=DIRECTION('center_axis',(0.,0.,1.));
#30206=DIRECTION('ref_axis',(-0.760231289280704,0.649652512346868,0.));
#30207=DIRECTION('center_axis',(0.,0.,-1.));
#30208=DIRECTION('ref_axis',(-0.760231289280704,0.649652512346868,0.));
#30209=DIRECTION('center_axis',(0.,0.,1.));
#30210=DIRECTION('ref_axis',(-0.0895155307640188,-0.995985426475727,0.));
#30211=DIRECTION('center_axis',(0.,0.,-1.));
#30212=DIRECTION('ref_axis',(-0.0895155307640188,-0.995985426475727,0.));
#30213=DIRECTION('',(0.,0.,1.));
#30214=DIRECTION('',(0.,0.,-1.));
#30215=DIRECTION('center_axis',(-0.760231289280706,-0.649652512346867,0.));
#30216=DIRECTION('ref_axis',(0.649652512346867,-0.760231289280706,0.));
#30217=DIRECTION('',(0.649652512346867,-0.760231289280706,0.));
#30218=DIRECTION('',(0.,0.,1.));
#30219=DIRECTION('center_axis',(0.,0.,1.));
#30220=DIRECTION('ref_axis',(0.985216370234623,-0.171314633997547,0.));
#30221=DIRECTION('center_axis',(0.,0.,-1.));
#30222=DIRECTION('ref_axis',(0.985216370234623,-0.171314633997547,0.));
#30223=DIRECTION('',(0.,0.,1.));
#30224=DIRECTION('',(0.,0.,-1.));
#30225=DIRECTION('center_axis',(0.,0.,1.));
#30226=DIRECTION('ref_axis',(-0.566184593375198,0.824278476138108,0.));
#30227=DIRECTION('center_axis',(0.,0.,-1.));
#30228=DIRECTION('ref_axis',(-0.566184593375198,0.824278476138108,0.));
#30229=DIRECTION('center_axis',(0.,0.,1.));
#30230=DIRECTION('ref_axis',(-0.34424536003541,-0.93887972184625,0.));
#30231=DIRECTION('center_axis',(0.,0.,-1.));
#30232=DIRECTION('ref_axis',(-0.34424536003541,-0.93887972184625,0.));
#30233=DIRECTION('',(0.,0.,1.));
#30234=DIRECTION('',(0.,0.,-1.));
#30235=DIRECTION('center_axis',(-0.902469479163339,-0.430753803440726,0.));
#30236=DIRECTION('ref_axis',(0.430753803440726,-0.902469479163339,0.));
#30237=DIRECTION('',(0.430753803440726,-0.902469479163339,0.));
#30238=DIRECTION('',(0.,0.,1.));
#30239=DIRECTION('center_axis',(0.,0.,1.));
#30240=DIRECTION('ref_axis',(0.907306446509069,-0.420469989562973,0.));
#30241=DIRECTION('center_axis',(0.,0.,-1.));
#30242=DIRECTION('ref_axis',(0.907306446509069,-0.420469989562973,0.));
#30243=DIRECTION('',(0.,0.,1.));
#30244=DIRECTION('',(0.,0.,-1.));
#30245=DIRECTION('center_axis',(0.,0.,1.));
#30246=DIRECTION('ref_axis',(-0.333553353095452,0.942731223965124,0.));
#30247=DIRECTION('center_axis',(0.,0.,-1.));
#30248=DIRECTION('ref_axis',(-0.333553353095452,0.942731223965124,0.));
#30249=DIRECTION('center_axis',(0.,0.,1.));
#30250=DIRECTION('ref_axis',(-0.575515436912748,-0.817790915745051,0.));
#30251=DIRECTION('center_axis',(0.,0.,-1.));
#30252=DIRECTION('ref_axis',(-0.575515436912748,-0.817790915745051,0.));
#30253=DIRECTION('',(0.,0.,1.));
#30254=DIRECTION('',(0.,0.,-1.));
#30255=DIRECTION('center_axis',(-0.983205865442321,-0.182499934684418,0.));
#30256=DIRECTION('ref_axis',(0.182499934684418,-0.983205865442321,0.));
#30257=DIRECTION('',(0.182499934684418,-0.983205865442321,0.));
#30258=DIRECTION('',(0.,0.,1.));
#30259=DIRECTION('center_axis',(0.,0.,1.));
#30260=DIRECTION('ref_axis',(0.767565087848708,-0.640971010199218,0.));
#30261=DIRECTION('center_axis',(0.,0.,-1.));
#30262=DIRECTION('ref_axis',(0.767565087848708,-0.640971010199218,0.));
#30263=DIRECTION('',(0.,0.,1.));
#30264=DIRECTION('',(0.,0.,-1.));
#30265=DIRECTION('center_axis',(0.,0.,1.));
#30266=DIRECTION('ref_axis',(-0.0781910030252301,0.996938396815926,0.));
#30267=DIRECTION('center_axis',(0.,0.,-1.));
#30268=DIRECTION('ref_axis',(-0.0781910030252301,0.996938396815926,0.));
#30269=DIRECTION('center_axis',(0.,0.,1.));
#30270=DIRECTION('ref_axis',(-0.767565087848706,-0.640971010199219,0.));
#30271=DIRECTION('center_axis',(0.,0.,-1.));
#30272=DIRECTION('ref_axis',(-0.767565087848706,-0.640971010199219,0.));
#30273=DIRECTION('',(0.,0.,1.));
#30274=DIRECTION('',(0.,0.,-1.));
#30275=DIRECTION('center_axis',(-0.996938396815926,0.0781910030252323,0.));
#30276=DIRECTION('ref_axis',(-0.0781910030252323,-0.996938396815926,0.));
#30277=DIRECTION('',(-0.0781910030252323,-0.996938396815926,0.));
#30278=DIRECTION('',(0.,0.,1.));
#30279=DIRECTION('center_axis',(0.,0.,1.));
#30280=DIRECTION('ref_axis',(0.57551543691275,-0.817790915745049,0.));
#30281=DIRECTION('center_axis',(0.,0.,-1.));
#30282=DIRECTION('ref_axis',(0.57551543691275,-0.817790915745049,0.));
#30283=DIRECTION('',(0.,0.,1.));
#30284=DIRECTION('',(0.,0.,-1.));
#30285=DIRECTION('center_axis',(0.,0.,1.));
#30286=DIRECTION('ref_axis',(0.18249993468442,0.983205865442321,0.));
#30287=DIRECTION('center_axis',(0.,0.,-1.));
#30288=DIRECTION('ref_axis',(0.18249993468442,0.983205865442321,0.));
#30289=DIRECTION('center_axis',(0.,0.,1.));
#30290=DIRECTION('ref_axis',(-0.907306446509064,-0.420469989562983,0.));
#30291=DIRECTION('center_axis',(0.,0.,-1.));
#30292=DIRECTION('ref_axis',(-0.907306446509064,-0.420469989562983,0.));
#30293=DIRECTION('',(0.,0.,1.));
#30294=DIRECTION('',(0.,0.,-1.));
#30295=DIRECTION('center_axis',(-0.942731223965123,0.333553353095454,0.));
#30296=DIRECTION('ref_axis',(-0.333553353095454,-0.942731223965123,0.));
#30297=DIRECTION('',(-0.333553353095454,-0.942731223965123,0.));
#30298=DIRECTION('',(0.,0.,1.));
#30299=DIRECTION('center_axis',(0.,0.,1.));
#30300=DIRECTION('ref_axis',(0.344245360035413,-0.938879721846248,0.));
#30301=DIRECTION('center_axis',(0.,0.,-1.));
#30302=DIRECTION('ref_axis',(0.344245360035413,-0.938879721846248,0.));
#30303=DIRECTION('',(0.,0.,1.));
#30304=DIRECTION('',(0.,0.,-1.));
#30305=DIRECTION('center_axis',(0.,0.,1.));
#30306=DIRECTION('ref_axis',(0.430753803440728,0.902469479163338,0.));
#30307=DIRECTION('center_axis',(0.,0.,-1.));
#30308=DIRECTION('ref_axis',(0.430753803440728,0.902469479163338,0.));
#30309=DIRECTION('center_axis',(0.,0.,1.));
#30310=DIRECTION('ref_axis',(-0.985216370234624,-0.171314633997546,0.));
#30311=DIRECTION('center_axis',(0.,0.,-1.));
#30312=DIRECTION('ref_axis',(-0.985216370234624,-0.171314633997546,0.));
#30313=DIRECTION('',(0.,0.,1.));
#30314=DIRECTION('',(0.,0.,-1.));
#30315=DIRECTION('center_axis',(-0.824278476138107,0.5661845933752,0.));
#30316=DIRECTION('ref_axis',(-0.5661845933752,-0.824278476138107,0.));
#30317=DIRECTION('',(-0.5661845933752,-0.824278476138107,0.));
#30318=DIRECTION('',(0.,0.,1.));
#30319=DIRECTION('center_axis',(0.,0.,1.));
#30320=DIRECTION('ref_axis',(0.0895155307640121,-0.995985426475728,0.));
#30321=DIRECTION('center_axis',(0.,0.,-1.));
#30322=DIRECTION('ref_axis',(0.0895155307640121,-0.995985426475728,0.));
#30323=DIRECTION('',(0.,0.,1.));
#30324=DIRECTION('',(0.,0.,-1.));
#30325=DIRECTION('center_axis',(0.,0.,1.));
#30326=DIRECTION('ref_axis',(0.649652512346868,0.760231289280704,0.));
#30327=DIRECTION('center_axis',(0.,0.,-1.));
#30328=DIRECTION('ref_axis',(0.649652512346868,0.760231289280704,0.));
#30329=DIRECTION('center_axis',(0.,0.,1.));
#30330=DIRECTION('ref_axis',(-0.995985426475728,0.0895155307640127,0.));
#30331=DIRECTION('center_axis',(0.,0.,-1.));
#30332=DIRECTION('ref_axis',(-0.995985426475728,0.0895155307640127,0.));
#30333=DIRECTION('',(0.,0.,1.));
#30334=DIRECTION('',(0.,0.,-1.));
#30335=DIRECTION('center_axis',(-0.649652512346867,0.760231289280706,0.));
#30336=DIRECTION('ref_axis',(-0.760231289280706,-0.649652512346867,0.));
#30337=DIRECTION('',(-0.760231289280706,-0.649652512346867,0.));
#30338=DIRECTION('',(0.,0.,1.));
#30339=DIRECTION('center_axis',(0.,0.,1.));
#30340=DIRECTION('ref_axis',(-0.171314633997547,-0.985216370234623,0.));
#30341=DIRECTION('center_axis',(0.,0.,-1.));
#30342=DIRECTION('ref_axis',(-0.171314633997547,-0.985216370234623,0.));
#30343=DIRECTION('',(0.,0.,1.));
#30344=DIRECTION('',(0.,0.,-1.));
#30345=DIRECTION('center_axis',(0.,0.,1.));
#30346=DIRECTION('ref_axis',(0.824278476138108,0.566184593375198,0.));
#30347=DIRECTION('center_axis',(0.,0.,-1.));
#30348=DIRECTION('ref_axis',(0.824278476138108,0.566184593375198,0.));
#30349=DIRECTION('center_axis',(0.,0.,1.));
#30350=DIRECTION('ref_axis',(-0.93887972184625,0.34424536003541,0.));
#30351=DIRECTION('center_axis',(0.,0.,-1.));
#30352=DIRECTION('ref_axis',(-0.93887972184625,0.34424536003541,0.));
#30353=DIRECTION('',(0.,0.,1.));
#30354=DIRECTION('',(0.,0.,-1.));
#30355=DIRECTION('center_axis',(-0.430753803440726,0.902469479163339,0.));
#30356=DIRECTION('ref_axis',(-0.902469479163339,-0.430753803440726,0.));
#30357=DIRECTION('',(-0.902469479163339,-0.430753803440726,0.));
#30358=DIRECTION('',(0.,0.,1.));
#30359=DIRECTION('center_axis',(0.,0.,1.));
#30360=DIRECTION('ref_axis',(-0.420469989562974,-0.907306446509068,0.));
#30361=DIRECTION('center_axis',(0.,0.,-1.));
#30362=DIRECTION('ref_axis',(-0.420469989562974,-0.907306446509068,0.));
#30363=DIRECTION('',(0.,0.,1.));
#30364=DIRECTION('',(0.,0.,-1.));
#30365=DIRECTION('center_axis',(0.,0.,1.));
#30366=DIRECTION('ref_axis',(0.942731223965124,0.333553353095452,0.));
#30367=DIRECTION('center_axis',(0.,0.,-1.));
#30368=DIRECTION('ref_axis',(0.942731223965124,0.333553353095452,0.));
#30369=DIRECTION('center_axis',(-0.18249993468442,-0.983205865442321,0.));
#30370=DIRECTION('ref_axis',(0.983205865442321,-0.182499934684419,0.));
#30371=DIRECTION('',(0.,0.,1.));
#30372=DIRECTION('',(0.983205865442321,-0.182499934684419,0.));
#30373=DIRECTION('',(0.,0.,-1.));
#30374=DIRECTION('',(0.,0.,1.));
#30375=DIRECTION('center_axis',(-0.430753803440728,-0.902469479163338,0.));
#30376=DIRECTION('ref_axis',(0.902469479163338,-0.430753803440728,0.));
#30377=DIRECTION('',(0.,0.,1.));
#30378=DIRECTION('',(0.902469479163338,-0.430753803440728,0.));
#30379=DIRECTION('',(0.,0.,-1.));
#30380=DIRECTION('',(0.,0.,1.));
#30381=DIRECTION('center_axis',(-0.649652512346868,-0.760231289280705,0.));
#30382=DIRECTION('ref_axis',(0.760231289280705,-0.649652512346868,0.));
#30383=DIRECTION('',(0.,0.,1.));
#30384=DIRECTION('',(0.760231289280705,-0.649652512346868,0.));
#30385=DIRECTION('',(0.,0.,-1.));
#30386=DIRECTION('',(0.,0.,1.));
#30387=DIRECTION('center_axis',(-0.824278476138108,-0.566184593375198,0.));
#30388=DIRECTION('ref_axis',(0.566184593375198,-0.824278476138108,0.));
#30389=DIRECTION('',(0.,0.,1.));
#30390=DIRECTION('',(0.566184593375198,-0.824278476138108,0.));
#30391=DIRECTION('',(0.,0.,-1.));
#30392=DIRECTION('',(0.,0.,1.));
#30393=DIRECTION('center_axis',(-0.942731223965124,-0.333553353095453,0.));
#30394=DIRECTION('ref_axis',(0.333553353095453,-0.942731223965124,0.));
#30395=DIRECTION('',(0.,0.,1.));
#30396=DIRECTION('',(0.333553353095453,-0.942731223965124,0.));
#30397=DIRECTION('',(0.,0.,-1.));
#30398=DIRECTION('',(0.,0.,1.));
#30399=DIRECTION('center_axis',(-0.996938396815926,-0.0781910030252307,
0.));
#30400=DIRECTION('ref_axis',(0.0781910030252307,-0.996938396815926,0.));
#30401=DIRECTION('',(0.,0.,1.));
#30402=DIRECTION('',(0.0781910030252307,-0.996938396815926,0.));
#30403=DIRECTION('',(0.,0.,-1.));
#30404=DIRECTION('',(0.,0.,1.));
#30405=DIRECTION('center_axis',(-0.983205865442321,0.182499934684419,0.));
#30406=DIRECTION('ref_axis',(-0.182499934684419,-0.983205865442321,0.));
#30407=DIRECTION('',(0.,0.,1.));
#30408=DIRECTION('',(-0.182499934684419,-0.983205865442321,0.));
#30409=DIRECTION('',(0.,0.,-1.));
#30410=DIRECTION('',(0.,0.,1.));
#30411=DIRECTION('center_axis',(-0.902469479163338,0.430753803440728,0.));
#30412=DIRECTION('ref_axis',(-0.430753803440728,-0.902469479163338,0.));
#30413=DIRECTION('',(0.,0.,1.));
#30414=DIRECTION('',(-0.430753803440728,-0.902469479163338,0.));
#30415=DIRECTION('',(0.,0.,-1.));
#30416=DIRECTION('',(0.,0.,1.));
#30417=DIRECTION('center_axis',(-0.760231289280705,0.649652512346868,0.));
#30418=DIRECTION('ref_axis',(-0.649652512346868,-0.760231289280705,0.));
#30419=DIRECTION('',(0.,0.,1.));
#30420=DIRECTION('',(-0.649652512346868,-0.760231289280705,0.));
#30421=DIRECTION('',(0.,0.,-1.));
#30422=DIRECTION('',(0.,0.,1.));
#30423=DIRECTION('center_axis',(-0.566184593375199,0.824278476138108,0.));
#30424=DIRECTION('ref_axis',(-0.824278476138108,-0.566184593375198,0.));
#30425=DIRECTION('',(0.,0.,1.));
#30426=DIRECTION('',(-0.824278476138108,-0.566184593375198,0.));
#30427=DIRECTION('',(0.,0.,-1.));
#30428=DIRECTION('',(0.,0.,1.));
#30429=DIRECTION('center_axis',(-0.333553353095453,0.942731223965124,0.));
#30430=DIRECTION('ref_axis',(-0.942731223965124,-0.333553353095453,0.));
#30431=DIRECTION('',(0.,0.,1.));
#30432=DIRECTION('',(-0.942731223965124,-0.333553353095453,0.));
#30433=DIRECTION('',(0.,0.,-1.));
#30434=DIRECTION('',(0.,0.,1.));
#30435=DIRECTION('center_axis',(-0.0781910030252307,0.996938396815926,0.));
#30436=DIRECTION('ref_axis',(-0.996938396815926,-0.0781910030252307,0.));
#30437=DIRECTION('',(0.,0.,1.));
#30438=DIRECTION('',(-0.996938396815926,-0.0781910030252307,0.));
#30439=DIRECTION('',(0.,0.,-1.));
#30440=DIRECTION('',(0.,0.,1.));
#30441=DIRECTION('center_axis',(0.182499934684419,0.983205865442321,0.));
#30442=DIRECTION('ref_axis',(-0.983205865442321,0.182499934684419,0.));
#30443=DIRECTION('',(0.,0.,1.));
#30444=DIRECTION('',(-0.983205865442321,0.182499934684419,0.));
#30445=DIRECTION('',(0.,0.,-1.));
#30446=DIRECTION('',(0.,0.,1.));
#30447=DIRECTION('center_axis',(0.430753803440728,0.902469479163338,0.));
#30448=DIRECTION('ref_axis',(-0.902469479163338,0.430753803440727,0.));
#30449=DIRECTION('',(0.,0.,1.));
#30450=DIRECTION('',(-0.902469479163338,0.430753803440727,0.));
#30451=DIRECTION('',(0.,0.,-1.));
#30452=DIRECTION('',(0.,0.,1.));
#30453=DIRECTION('center_axis',(0.649652512346868,0.760231289280705,0.));
#30454=DIRECTION('ref_axis',(-0.760231289280705,0.649652512346868,0.));
#30455=DIRECTION('',(0.,0.,1.));
#30456=DIRECTION('',(-0.760231289280705,0.649652512346868,0.));
#30457=DIRECTION('',(0.,0.,-1.));
#30458=DIRECTION('',(0.,0.,1.));
#30459=DIRECTION('center_axis',(0.824278476138108,0.566184593375199,0.));
#30460=DIRECTION('ref_axis',(-0.566184593375199,0.824278476138108,0.));
#30461=DIRECTION('',(0.,0.,1.));
#30462=DIRECTION('',(-0.566184593375199,0.824278476138108,0.));
#30463=DIRECTION('',(0.,0.,-1.));
#30464=DIRECTION('',(0.,0.,1.));
#30465=DIRECTION('center_axis',(0.942731223965124,0.333553353095453,0.));
#30466=DIRECTION('ref_axis',(-0.333553353095453,0.942731223965124,0.));
#30467=DIRECTION('',(0.,0.,1.));
#30468=DIRECTION('',(-0.333553353095453,0.942731223965124,0.));
#30469=DIRECTION('',(0.,0.,-1.));
#30470=DIRECTION('',(0.,0.,1.));
#30471=DIRECTION('center_axis',(0.996938396815926,0.0781910030252308,0.));
#30472=DIRECTION('ref_axis',(-0.0781910030252308,0.996938396815926,0.));
#30473=DIRECTION('',(0.,0.,1.));
#30474=DIRECTION('',(-0.0781910030252308,0.996938396815926,0.));
#30475=DIRECTION('',(0.,0.,-1.));
#30476=DIRECTION('',(0.,0.,1.));
#30477=DIRECTION('center_axis',(0.983205865442321,-0.182499934684419,0.));
#30478=DIRECTION('ref_axis',(0.182499934684419,0.983205865442321,0.));
#30479=DIRECTION('',(0.,0.,1.));
#30480=DIRECTION('',(0.182499934684419,0.983205865442321,0.));
#30481=DIRECTION('',(0.,0.,-1.));
#30482=DIRECTION('',(0.,0.,1.));
#30483=DIRECTION('center_axis',(0.902469479163338,-0.430753803440727,0.));
#30484=DIRECTION('ref_axis',(0.430753803440727,0.902469479163338,0.));
#30485=DIRECTION('',(0.,0.,1.));
#30486=DIRECTION('',(0.430753803440727,0.902469479163338,0.));
#30487=DIRECTION('',(0.,0.,-1.));
#30488=DIRECTION('',(0.,0.,1.));
#30489=DIRECTION('center_axis',(0.760231289280705,-0.649652512346868,0.));
#30490=DIRECTION('ref_axis',(0.649652512346868,0.760231289280705,0.));
#30491=DIRECTION('',(0.,0.,1.));
#30492=DIRECTION('',(0.649652512346868,0.760231289280705,0.));
#30493=DIRECTION('',(0.,0.,-1.));
#30494=DIRECTION('',(0.,0.,1.));
#30495=DIRECTION('center_axis',(0.566184593375199,-0.824278476138108,0.));
#30496=DIRECTION('ref_axis',(0.824278476138108,0.566184593375199,0.));
#30497=DIRECTION('',(0.,0.,1.));
#30498=DIRECTION('',(0.824278476138108,0.566184593375199,0.));
#30499=DIRECTION('',(0.,0.,-1.));
#30500=DIRECTION('',(0.,0.,1.));
#30501=DIRECTION('center_axis',(0.333553353095453,-0.942731223965124,0.));
#30502=DIRECTION('ref_axis',(0.942731223965124,0.333553353095453,0.));
#30503=DIRECTION('',(0.,0.,1.));
#30504=DIRECTION('',(0.942731223965124,0.333553353095453,0.));
#30505=DIRECTION('',(0.,0.,-1.));
#30506=DIRECTION('',(0.,0.,1.));
#30507=DIRECTION('center_axis',(0.,0.,1.));
#30508=DIRECTION('ref_axis',(1.,0.,0.));
#30509=DIRECTION('center_axis',(0.,0.,1.));
#30510=DIRECTION('ref_axis',(1.,0.,0.));
#30511=DIRECTION('center_axis',(0.,0.,1.));
#30512=DIRECTION('ref_axis',(1.,0.,0.));
#30513=DIRECTION('center_axis',(0.,0.,1.));
#30514=DIRECTION('ref_axis',(1.,0.,0.));
#30515=DIRECTION('center_axis',(0.,0.,1.));
#30516=DIRECTION('ref_axis',(1.,0.,0.));
#30517=DIRECTION('center_axis',(0.,0.,1.));
#30518=DIRECTION('ref_axis',(1.,0.,0.));
#30519=DIRECTION('center_axis',(0.,0.,1.));
#30520=DIRECTION('ref_axis',(1.,0.,0.));
#30521=DIRECTION('center_axis',(0.,0.,1.));
#30522=DIRECTION('ref_axis',(1.,0.,0.));
#30523=DIRECTION('center_axis',(0.,0.,1.));
#30524=DIRECTION('ref_axis',(1.,0.,0.));
#30525=DIRECTION('center_axis',(0.,0.,1.));
#30526=DIRECTION('ref_axis',(1.,0.,0.));
#30527=DIRECTION('center_axis',(0.,0.,1.));
#30528=DIRECTION('ref_axis',(1.,0.,0.));
#30529=DIRECTION('center_axis',(0.,0.,1.));
#30530=DIRECTION('ref_axis',(1.,0.,0.));
#30531=DIRECTION('center_axis',(0.,0.,1.));
#30532=DIRECTION('ref_axis',(1.,0.,0.));
#30533=DIRECTION('center_axis',(0.,0.,1.));
#30534=DIRECTION('ref_axis',(1.,0.,0.));
#30535=DIRECTION('center_axis',(0.,0.,1.));
#30536=DIRECTION('ref_axis',(1.,0.,0.));
#30537=DIRECTION('center_axis',(0.,0.,1.));
#30538=DIRECTION('ref_axis',(1.,0.,0.));
#30539=DIRECTION('center_axis',(0.,0.,1.));
#30540=DIRECTION('ref_axis',(1.,0.,0.));
#30541=DIRECTION('center_axis',(0.,0.,1.));
#30542=DIRECTION('ref_axis',(1.,0.,0.));
#30543=DIRECTION('center_axis',(0.,0.,1.));
#30544=DIRECTION('ref_axis',(1.,0.,0.));
#30545=DIRECTION('center_axis',(0.,0.,1.));
#30546=DIRECTION('ref_axis',(1.,0.,0.));
#30547=DIRECTION('center_axis',(0.,0.,1.));
#30548=DIRECTION('ref_axis',(1.,0.,0.));
#30549=DIRECTION('center_axis',(0.,0.,1.));
#30550=DIRECTION('ref_axis',(1.,0.,0.));
#30551=DIRECTION('center_axis',(0.,0.,1.));
#30552=DIRECTION('ref_axis',(1.,0.,0.));
#30553=DIRECTION('center_axis',(0.,0.,1.));
#30554=DIRECTION('ref_axis',(1.,0.,0.));
#30555=DIRECTION('',(-0.983205865442321,-0.182499934684418,0.));
#30556=DIRECTION('center_axis',(0.,0.,-1.));
#30557=DIRECTION('ref_axis',(-0.817790915745051,0.575515436912748,0.));
#30558=DIRECTION('center_axis',(0.,0.,-1.));
#30559=DIRECTION('ref_axis',(0.996938396815926,0.0781910030252301,0.));
#30560=DIRECTION('center_axis',(0.,0.,-1.));
#30561=DIRECTION('ref_axis',(-0.640971010199219,-0.767565087848707,0.));
#30562=DIRECTION('',(0.996938396815926,0.0781910030252308,0.));
#30563=DIRECTION('center_axis',(0.,0.,1.));
#30564=DIRECTION('ref_axis',(1.,0.,0.));
#30565=DIRECTION('center_axis',(0.,0.,1.));
#30566=DIRECTION('ref_axis',(1.,0.,0.));
#30567=DIRECTION('',(0.,0.,-1.));
#30568=DIRECTION('center_axis',(0.,0.,1.));
#30569=DIRECTION('ref_axis',(1.,0.,0.));
#30570=DIRECTION('center_axis',(0.,0.,1.));
#30571=DIRECTION('ref_axis',(1.,0.,0.));
#30572=DIRECTION('center_axis',(0.,0.,1.));
#30573=DIRECTION('ref_axis',(1.,0.,0.));
#30574=DIRECTION('center_axis',(0.,0.,1.));
#30575=DIRECTION('ref_axis',(1.,0.,0.));
#30576=DIRECTION('center_axis',(0.,0.,1.));
#30577=DIRECTION('ref_axis',(1.,0.,0.));
#30578=DIRECTION('center_axis',(0.,0.,1.));
#30579=DIRECTION('ref_axis',(1.,0.,0.));
#30580=DIRECTION('center_axis',(0.,0.,1.));
#30581=DIRECTION('ref_axis',(1.,0.,0.));
#30582=DIRECTION('center_axis',(0.,0.,1.));
#30583=DIRECTION('ref_axis',(1.,0.,0.));
#30584=DIRECTION('center_axis',(0.,0.,1.));
#30585=DIRECTION('ref_axis',(1.,0.,0.));
#30586=DIRECTION('center_axis',(0.,0.,1.));
#30587=DIRECTION('ref_axis',(1.,0.,0.));
#30588=DIRECTION('center_axis',(0.,0.,1.));
#30589=DIRECTION('ref_axis',(-1.,-1.22464679914735E-16,0.));
#30590=DIRECTION('center_axis',(0.,0.,1.));
#30591=DIRECTION('ref_axis',(1.,0.,0.));
#30592=DIRECTION('center_axis',(0.,0.,1.));
#30593=DIRECTION('ref_axis',(1.,0.,0.));
#30594=DIRECTION('center_axis',(0.,0.,1.));
#30595=DIRECTION('ref_axis',(1.,0.,0.));
#30596=DIRECTION('center_axis',(0.,0.,1.));
#30597=DIRECTION('ref_axis',(1.,0.,0.));
#30598=DIRECTION('center_axis',(0.,0.,1.));
#30599=DIRECTION('ref_axis',(1.,0.,0.));
#30600=DIRECTION('center_axis',(0.,0.,1.));
#30601=DIRECTION('ref_axis',(1.,0.,0.));
#30602=DIRECTION('center_axis',(0.,0.,1.));
#30603=DIRECTION('ref_axis',(1.,0.,0.));
#30604=DIRECTION('center_axis',(0.,0.,1.));
#30605=DIRECTION('ref_axis',(1.,0.,0.));
#30606=DIRECTION('center_axis',(0.,0.,1.));
#30607=DIRECTION('ref_axis',(1.,0.,0.));
#30608=DIRECTION('center_axis',(0.,0.,1.));
#30609=DIRECTION('ref_axis',(1.,0.,0.));
#30610=DIRECTION('center_axis',(0.,0.,1.));
#30611=DIRECTION('ref_axis',(1.,0.,0.));
#30612=DIRECTION('center_axis',(0.,0.,1.));
#30613=DIRECTION('ref_axis',(-0.817790915745051,0.575515436912748,0.));
#30614=DIRECTION('',(0.,0.,1.));
#30615=DIRECTION('',(0.,0.,-1.));
#30616=DIRECTION('center_axis',(-0.182499934684418,0.983205865442321,0.));
#30617=DIRECTION('ref_axis',(-0.983205865442321,-0.182499934684418,0.));
#30618=DIRECTION('',(0.,0.,1.));
#30619=DIRECTION('center_axis',(0.,0.,1.));
#30620=DIRECTION('ref_axis',(-0.640971010199219,-0.767565087848707,0.));
#30621=DIRECTION('',(0.,0.,1.));
#30622=DIRECTION('',(0.,0.,-1.));
#30623=DIRECTION('center_axis',(0.,0.,1.));
#30624=DIRECTION('ref_axis',(0.996938396815926,0.0781910030252301,0.));
#30625=DIRECTION('center_axis',(0.0781910030252308,-0.996938396815926,0.));
#30626=DIRECTION('ref_axis',(0.996938396815926,0.0781910030252308,0.));
#30627=DIRECTION('',(0.,0.,1.));
#30628=DIRECTION('',(0.,0.,1.));
#30629=DIRECTION('center_axis',(0.,0.,1.));
#30630=DIRECTION('ref_axis',(1.,0.,0.));
#174985=CARTESIAN_POINT('',(0.,0.,0.));
#174986=CARTESIAN_POINT('Origin',(5.,3.,12.));
#174987=CARTESIAN_POINT('',(7.41619848709566,3.,0.));
#174988=CARTESIAN_POINT('',(7.41619848709566,3.,12.));
#174989=CARTESIAN_POINT('',(7.41619848709566,3.,0.));
#174990=CARTESIAN_POINT('',(11.,3.,0.));
#174991=CARTESIAN_POINT('',(2.5,3.,0.));
#174992=CARTESIAN_POINT('',(11.,3.,12.));
#174993=CARTESIAN_POINT('',(11.,3.,12.));
#174994=CARTESIAN_POINT('',(2.5,3.,12.));
#174995=CARTESIAN_POINT('Origin',(11.,-3.,12.));
#174996=CARTESIAN_POINT('',(7.41619848709566,-3.,12.));
#174997=CARTESIAN_POINT('',(7.41619848709566,-3.,0.));
#174998=CARTESIAN_POINT('',(7.41619848709566,-3.,0.));
#174999=CARTESIAN_POINT('',(11.,-3.,12.));
#175000=CARTESIAN_POINT('',(5.5,-3.,12.));
#175001=CARTESIAN_POINT('',(11.,-3.,0.));
#175002=CARTESIAN_POINT('',(11.,-3.,12.));
#175003=CARTESIAN_POINT('',(5.5,-3.,0.));
#175004=CARTESIAN_POINT('Origin',(11.,3.,12.));
#175005=CARTESIAN_POINT('',(11.,1.5,12.));
#175006=CARTESIAN_POINT('',(11.,1.5,0.));
#175007=CARTESIAN_POINT('Origin',(0.,0.,0.));
#175008=CARTESIAN_POINT('Origin',(0.,0.,12.));
#175009=CARTESIAN_POINT('Origin',(0.,0.,0.));
#175010=CARTESIAN_POINT('Origin',(0.,0.,12.));
#175011=CARTESIAN_POINT('',(22.4835757167854,-1.76341220531181,12.));
#175012=CARTESIAN_POINT('',(25.991588367311,-0.661312440730916,12.));
#175013=CARTESIAN_POINT('Ctrl Pts',(22.4835757167854,-1.76341220531181,
12.));
#175014=CARTESIAN_POINT('Ctrl Pts',(22.4835819929788,-1.76341415538792,
12.));
#175015=CARTESIAN_POINT('Ctrl Pts',(22.4836387052228,-1.76342064263638,
12.));
#175016=CARTESIAN_POINT('Ctrl Pts',(22.4838562517064,-1.7634381343466,12.));
#175017=CARTESIAN_POINT('Ctrl Pts',(22.4844112933125,-1.76347698284863,
12.));
#175018=CARTESIAN_POINT('Ctrl Pts',(22.4855446605991,-1.7635507604555,12.));
#175019=CARTESIAN_POINT('Ctrl Pts',(22.4871115206572,-1.76364784232927,
12.));
#175020=CARTESIAN_POINT('Ctrl Pts',(22.4890991659479,-1.76376424879469,
12.));
#175021=CARTESIAN_POINT('Ctrl Pts',(22.4914909094908,-1.76389475965715,
12.));
#175022=CARTESIAN_POINT('Ctrl Pts',(22.4942693792449,-1.76403393880317,
12.));
#175023=CARTESIAN_POINT('Ctrl Pts',(22.4974203063191,-1.76417731243484,
12.));
#175024=CARTESIAN_POINT('Ctrl Pts',(22.5009332677316,-1.76432160068739,
12.));
#175025=CARTESIAN_POINT('Ctrl Pts',(22.5047996391978,-1.76446408210366,
12.));
#175026=CARTESIAN_POINT('Ctrl Pts',(22.5090112700212,-1.76460218257314,
12.));
#175027=CARTESIAN_POINT('Ctrl Pts',(22.5135590569554,-1.7647330328115,12.));
#175028=CARTESIAN_POINT('Ctrl Pts',(22.5184336670207,-1.76485369319896,
12.));
#175029=CARTESIAN_POINT('Ctrl Pts',(22.5236259635515,-1.76496128643376,
12.));
#175030=CARTESIAN_POINT('Ctrl Pts',(22.529127665298,-1.7650532026276,12.));
#175031=CARTESIAN_POINT('Ctrl Pts',(22.5349313983571,-1.76512711563255,
12.));
#175032=CARTESIAN_POINT('Ctrl Pts',(22.5410303590892,-1.76518087841494,
12.));
#175033=CARTESIAN_POINT('Ctrl Pts',(22.5474180954006,-1.76521245524048,
12.));
#175034=CARTESIAN_POINT('Ctrl Pts',(22.5540882235837,-1.76521983384064,
12.));
#175035=CARTESIAN_POINT('Ctrl Pts',(22.5610344912501,-1.76520104500451,
12.));
#175036=CARTESIAN_POINT('Ctrl Pts',(22.5682508499873,-1.76515418518832,
12.));
#175037=CARTESIAN_POINT('Ctrl Pts',(22.5757315316353,-1.76507744026747,
12.));
#175038=CARTESIAN_POINT('Ctrl Pts',(22.5834711038022,-1.76496910283089,
12.));
#175039=CARTESIAN_POINT('Ctrl Pts',(22.5914644078105,-1.76482755288412,
12.));
#175040=CARTESIAN_POINT('Ctrl Pts',(22.5997065145638,-1.76465124413558,
12.));
#175041=CARTESIAN_POINT('Ctrl Pts',(22.6081926681343,-1.76443868648017,
12.));
#175042=CARTESIAN_POINT('Ctrl Pts',(22.6169182517694,-1.76418843543741,
12.));
#175043=CARTESIAN_POINT('Ctrl Pts',(22.6258787994848,-1.76389909571404,
12.));
#175044=CARTESIAN_POINT('Ctrl Pts',(22.6350699979359,-1.76356932176274,
12.));
#175045=CARTESIAN_POINT('Ctrl Pts',(22.6444876940423,-1.76319782013917,
12.));
#175046=CARTESIAN_POINT('Ctrl Pts',(22.6541278938409,-1.76278334912562,
12.));
#175047=CARTESIAN_POINT('Ctrl Pts',(22.6639867471753,-1.7623247139257,12.));
#175048=CARTESIAN_POINT('Ctrl Pts',(22.67406053567,-1.76182076289527,12.));
#175049=CARTESIAN_POINT('Ctrl Pts',(22.684345658525,-1.76127038310615,12.));
#175050=CARTESIAN_POINT('Ctrl Pts',(22.6948386219851,-1.76067249704888,
12.));
#175051=CARTESIAN_POINT('Ctrl Pts',(22.7055360375485,-1.76002606202402,
12.));
#175052=CARTESIAN_POINT('Ctrl Pts',(22.7164346186006,-1.75933006905926,
12.));
#175053=CARTESIAN_POINT('Ctrl Pts',(22.72753117773,-1.75858354204634,12.));
#175054=CARTESIAN_POINT('Ctrl Pts',(22.7388226235559,-1.75778553673245,
12.));
#175055=CARTESIAN_POINT('Ctrl Pts',(22.750305955645,-1.75693513908908,12.));
#175056=CARTESIAN_POINT('Ctrl Pts',(22.7619782595013,-1.75603146371642,
12.));
#175057=CARTESIAN_POINT('Ctrl Pts',(22.7738367016118,-1.75507365227133,
12.));
#175058=CARTESIAN_POINT('Ctrl Pts',(22.7858785242361,-1.75406087182937,
12.));
#175059=CARTESIAN_POINT('Ctrl Pts',(22.7981010424314,-1.75299231391468,
12.));
#175060=CARTESIAN_POINT('Ctrl Pts',(22.8105016414713,-1.75186719365593,
12.));
#175061=CARTESIAN_POINT('Ctrl Pts',(22.8230777741284,-1.75068474890884,
12.));
#175062=CARTESIAN_POINT('Ctrl Pts',(22.8358269579853,-1.74944423940117,
12.));
#175063=CARTESIAN_POINT('Ctrl Pts',(22.8487467728076,-1.74814494588494,
12.));
#175064=CARTESIAN_POINT('Ctrl Pts',(22.8618348580235,-1.74678616930666,
12.));
#175065=CARTESIAN_POINT('Ctrl Pts',(22.8750889101696,-1.74536722998202,
12.));
#175066=CARTESIAN_POINT('Ctrl Pts',(22.888506680335,-1.74388746677704,12.));
#175067=CARTESIAN_POINT('Ctrl Pts',(22.9020859716141,-1.74234623630081,
12.));
#175068=CARTESIAN_POINT('Ctrl Pts',(22.9158246373363,-1.7407429123106,12.));
#175069=CARTESIAN_POINT('Ctrl Pts',(22.9297205792586,-1.73907688511667,
12.));
#175070=CARTESIAN_POINT('Ctrl Pts',(22.9437717457826,-1.7373475610004,12.));
#175071=CARTESIAN_POINT('Ctrl Pts',(22.9579761301063,-1.73555436162771,
12.));
#175072=CARTESIAN_POINT('Ctrl Pts',(22.9723317685688,-1.73369672350816,
12.));
#175073=CARTESIAN_POINT('Ctrl Pts',(22.9868367391978,-1.73177409750192,
12.));
#175074=CARTESIAN_POINT('Ctrl Pts',(23.001489160189,-1.72978594832137,12.));
#175075=CARTESIAN_POINT('Ctrl Pts',(23.0162871884168,-1.7277317540471,12.));
#175076=CARTESIAN_POINT('Ctrl Pts',(23.0312290178883,-1.72561100564047,
12.));
#175077=CARTESIAN_POINT('Ctrl Pts',(23.0463128785531,-1.72342320653748,
12.));
#175078=CARTESIAN_POINT('Ctrl Pts',(23.0615370351562,-1.72116787225993,
12.));
#175079=CARTESIAN_POINT('Ctrl Pts',(23.0768997860708,-1.71884453003028,
12.));
#175080=CARTESIAN_POINT('Ctrl Pts',(23.0923994621213,-1.71645271839298,
12.));
#175081=CARTESIAN_POINT('Ctrl Pts',(23.1080344254286,-1.71399198684705,
12.));
#175082=CARTESIAN_POINT('Ctrl Pts',(23.1238030684925,-1.71146189552175,
12.));
#175083=CARTESIAN_POINT('Ctrl Pts',(23.1397038132356,-1.70886201485453,
12.));
#175084=CARTESIAN_POINT('Ctrl Pts',(23.1557351100614,-1.70619192527853,
12.));
#175085=CARTESIAN_POINT('Ctrl Pts',(23.1718954368751,-1.70345121691278,
12.));
#175086=CARTESIAN_POINT('Ctrl Pts',(23.1881832981851,-1.70063948927011,
12.));
#175087=CARTESIAN_POINT('Ctrl Pts',(23.2045972243767,-1.69775635099444,
12.));
#175088=CARTESIAN_POINT('Ctrl Pts',(23.2211357709374,-1.69480141959954,
12.));
#175089=CARTESIAN_POINT('Ctrl Pts',(23.2377975177013,-1.69177432121712,
12.));
#175090=CARTESIAN_POINT('Ctrl Pts',(23.2545810680537,-1.68867469034897,
12.));
#175091=CARTESIAN_POINT('Ctrl Pts',(23.2714850482246,-1.68550216963259,
12.));
#175092=CARTESIAN_POINT('Ctrl Pts',(23.2885081066951,-1.68225640962169,
12.));
#175093=CARTESIAN_POINT('Ctrl Pts',(23.3056489135611,-1.67893706857118,
12.));
#175094=CARTESIAN_POINT('Ctrl Pts',(23.3229061599144,-1.67554381222995,
12.));
#175095=CARTESIAN_POINT('Ctrl Pts',(23.3402785571865,-1.67207631363923,
12.));
#175096=CARTESIAN_POINT('Ctrl Pts',(23.3577648365744,-1.66853425293997,
12.));
#175097=CARTESIAN_POINT('Ctrl Pts',(23.3753637485545,-1.66491731718878,
12.));
#175098=CARTESIAN_POINT('Ctrl Pts',(23.3930740623619,-1.66122520018012,
12.));
#175099=CARTESIAN_POINT('Ctrl Pts',(23.4108945654805,-1.65745760227506,
12.));
#175100=CARTESIAN_POINT('Ctrl Pts',(23.4288240631043,-1.6536142302373,12.));
#175101=CARTESIAN_POINT('Ctrl Pts',(23.4468613776574,-1.64969479707341,
12.));
#175102=CARTESIAN_POINT('Ctrl Pts',(23.4650053483932,-1.64569902187612,
12.));
#175103=CARTESIAN_POINT('Ctrl Pts',(23.4832548309645,-1.64162662967529,
12.));
#175104=CARTESIAN_POINT('Ctrl Pts',(23.5016086970003,-1.63747735129475,
12.));
#175105=CARTESIAN_POINT('Ctrl Pts',(23.5200658336612,-1.63325092321727,
12.));
#175106=CARTESIAN_POINT('Ctrl Pts',(23.538625143226,-1.62894708745224,12.));
#175107=CARTESIAN_POINT('Ctrl Pts',(23.5572855427601,-1.62456559140066,
12.));
#175108=CARTESIAN_POINT('Ctrl Pts',(23.57604596376,-1.62010618772867,12.));
#175109=CARTESIAN_POINT('Ctrl Pts',(23.5949053517997,-1.61556863424699,
12.));
#175110=CARTESIAN_POINT('Ctrl Pts',(23.6138626661653,-1.61095269379779,
12.));
#175111=CARTESIAN_POINT('Ctrl Pts',(23.6329168794929,-1.60625813414674,
12.));
#175112=CARTESIAN_POINT('Ctrl Pts',(23.6520669774876,-1.60148472786596,
12.));
#175113=CARTESIAN_POINT('Ctrl Pts',(23.671311958631,-1.59663225222464,12.));
#175114=CARTESIAN_POINT('Ctrl Pts',(23.6906508338833,-1.59170048908634,
12.));
#175115=CARTESIAN_POINT('Ctrl Pts',(23.710082626383,-1.58668922481222,12.));
#175116=CARTESIAN_POINT('Ctrl Pts',(23.72960637113,-1.58159825017359,12.));
#175117=CARTESIAN_POINT('Ctrl Pts',(23.749221114736,-1.57642736025247,12.));
#175118=CARTESIAN_POINT('Ctrl Pts',(23.7689259151862,-1.57117635434409,
12.));
#175119=CARTESIAN_POINT('Ctrl Pts',(23.7887198415878,-1.56584503586844,
12.));
#175120=CARTESIAN_POINT('Ctrl Pts',(23.8086019739194,-1.56043321228635,
12.));
#175121=CARTESIAN_POINT('Ctrl Pts',(23.8285714027636,-1.55494069502636,
12.));
#175122=CARTESIAN_POINT('Ctrl Pts',(23.8486272290705,-1.54936729940542,
12.));
#175123=CARTESIAN_POINT('Ctrl Pts',(23.8687685639642,-1.54371284453992,
12.));
#175124=CARTESIAN_POINT('Ctrl Pts',(23.8889945285318,-1.53797715326759,
12.));
#175125=CARTESIAN_POINT('Ctrl Pts',(23.9093042536119,-1.53216005207464,
12.));
#175126=CARTESIAN_POINT('Ctrl Pts',(23.9296968795757,-1.52626137103033,
12.));
#175127=CARTESIAN_POINT('Ctrl Pts',(23.9501715561033,-1.52028094372793,
12.));
#175128=CARTESIAN_POINT('Ctrl Pts',(23.970727442014,-1.51421860720616,12.));
#175129=CARTESIAN_POINT('Ctrl Pts',(23.9913637050927,-1.50807420187695,
12.));
#175130=CARTESIAN_POINT('Ctrl Pts',(24.0120795219086,-1.501847571461,12.));
#175131=CARTESIAN_POINT('Ctrl Pts',(24.0328740776331,-1.49553856292802,
12.));
#175132=CARTESIAN_POINT('Ctrl Pts',(24.0537465658429,-1.48914702644889,
12.));
#175133=CARTESIAN_POINT('Ctrl Pts',(24.0746961883528,-1.48267281533684,
12.));
#175134=CARTESIAN_POINT('Ctrl Pts',(24.0957221550778,-1.47611578597743,
12.));
#175135=CARTESIAN_POINT('Ctrl Pts',(24.1168236838824,-1.46947579776993,
12.));
#175136=CARTESIAN_POINT('Ctrl Pts',(24.1380000004272,-1.46275271307399,
12.));
#175137=CARTESIAN_POINT('Ctrl Pts',(24.1592503380107,-1.45594639716319,
12.));
#175138=CARTESIAN_POINT('Ctrl Pts',(24.1805739374038,-1.44905671818729,
12.));
#175139=CARTESIAN_POINT('Ctrl Pts',(24.201970046722,-1.44208354711083,12.));
#175140=CARTESIAN_POINT('Ctrl Pts',(24.2234379212984,-1.4350267576551,12.));
#175141=CARTESIAN_POINT('Ctrl Pts',(24.2449768235488,-1.42788622624855,
12.));
#175142=CARTESIAN_POINT('Ctrl Pts',(24.2665860228356,-1.42066183198254,
12.));
#175143=CARTESIAN_POINT('Ctrl Pts',(24.288264795321,-1.41335345657684,12.));
#175144=CARTESIAN_POINT('Ctrl Pts',(24.3100124238311,-1.40596098434339,
12.));
#175145=CARTESIAN_POINT('Ctrl Pts',(24.3318281977643,-1.39848430212808,
12.));
#175146=CARTESIAN_POINT('Ctrl Pts',(24.3537114129875,-1.3909232992639,12.));
#175147=CARTESIAN_POINT('Ctrl Pts',(24.3756613717299,-1.38327786753,12.));
#175148=CARTESIAN_POINT('Ctrl Pts',(24.3976773824732,-1.37554790111611,
12.));
#175149=CARTESIAN_POINT('Ctrl Pts',(24.4197587598337,-1.36773329659958,
12.));
#175150=CARTESIAN_POINT('Ctrl Pts',(24.4419048244523,-1.35983395290629,
12.));
#175151=CARTESIAN_POINT('Ctrl Pts',(24.4641149028892,-1.35184977125649,
12.));
#175152=CARTESIAN_POINT('Ctrl Pts',(24.4863883275134,-1.34378065512339,
12.));
#175153=CARTESIAN_POINT('Ctrl Pts',(24.5087244363856,-1.33562651019687,
12.));
#175154=CARTESIAN_POINT('Ctrl Pts',(24.5311225731435,-1.32738724435327,
12.));
#175155=CARTESIAN_POINT('Ctrl Pts',(24.5535820868674,-1.31906276763669,
12.));
#175156=CARTESIAN_POINT('Ctrl Pts',(24.5761023320183,-1.31065299222023,
12.));
#175157=CARTESIAN_POINT('Ctrl Pts',(24.5986826684027,-1.30215783236363,
12.));
#175158=CARTESIAN_POINT('Ctrl Pts',(24.6213224611229,-1.29357720438108,
12.));
#175159=CARTESIAN_POINT('Ctrl Pts',(24.6440210805278,-1.28491102661515,
12.));
#175160=CARTESIAN_POINT('Ctrl Pts',(24.6667779021559,-1.27615921941643,
12.));
#175161=CARTESIAN_POINT('Ctrl Pts',(24.6895923066836,-1.26732170513501,
12.));
#175162=CARTESIAN_POINT('Ctrl Pts',(24.7124636797894,-1.25839840807419,
12.));
#175163=CARTESIAN_POINT('Ctrl Pts',(24.7353914120011,-1.24938925444327,
12.));
#175164=CARTESIAN_POINT('Ctrl Pts',(24.7583748985438,-1.2402941723199,12.));
#175165=CARTESIAN_POINT('Ctrl Pts',(24.7814135391799,-1.23111309161845,
12.));
#175166=CARTESIAN_POINT('Ctrl Pts',(24.8045067380536,-1.22184594406529,
12.));
#175167=CARTESIAN_POINT('Ctrl Pts',(24.8276539035092,-1.21249266318209,
12.));
#175168=CARTESIAN_POINT('Ctrl Pts',(24.8508544481974,-1.20305318426021,
12.));
#175169=CARTESIAN_POINT('Ctrl Pts',(24.8741077892075,-1.19352744434066,
12.));
#175170=CARTESIAN_POINT('Ctrl Pts',(24.8974133481829,-1.18391538220104,
12.));
#175171=CARTESIAN_POINT('Ctrl Pts',(24.9207705514448,-1.17421693835042,
12.));
#175172=CARTESIAN_POINT('Ctrl Pts',(24.9441788300932,-1.16443205502851,
12.));
#175173=CARTESIAN_POINT('Ctrl Pts',(24.9676376201502,-1.15456067621891,
12.));
#175174=CARTESIAN_POINT('Ctrl Pts',(24.9911463621433,-1.14460274758202,
12.));
#175175=CARTESIAN_POINT('Ctrl Pts',(25.0147045006195,-1.13455821638531,
12.));
#175176=CARTESIAN_POINT('Ctrl Pts',(25.0383114836899,-1.12442703144453,
12.));
#175177=CARTESIAN_POINT('Ctrl Pts',(25.0619667625336,-1.11420914306891,
12.));
#175178=CARTESIAN_POINT('Ctrl Pts',(25.0856697909679,-1.10390450301747,
12.));
#175179=CARTESIAN_POINT('Ctrl Pts',(25.1094200248446,-1.09351306445309,
12.));
#175180=CARTESIAN_POINT('Ctrl Pts',(25.1332169227413,-1.08303478197189,
12.));
#175181=CARTESIAN_POINT('Ctrl Pts',(25.157059946931,-1.07246961165477,12.));
#175182=CARTESIAN_POINT('Ctrl Pts',(25.1809485642192,-1.06181751111769,
12.));
#175183=CARTESIAN_POINT('Ctrl Pts',(25.2048822469028,-1.05107843957933,
12.));
#175184=CARTESIAN_POINT('Ctrl Pts',(25.2288604735086,-1.04025235791508,
12.));
#175185=CARTESIAN_POINT('Ctrl Pts',(25.2528827300422,-1.02933922876807,
12.));
#175186=CARTESIAN_POINT('Ctrl Pts',(25.276948508726,-1.01833901642238,12.));
#175187=CARTESIAN_POINT('Ctrl Pts',(25.3010573055547,-1.00725168656897,
12.));
#175188=CARTESIAN_POINT('Ctrl Pts',(25.3252086182968,-0.996077206120637,
12.));
#175189=CARTESIAN_POINT('Ctrl Pts',(25.3494019441441,-0.984815543003986,
12.));
#175190=CARTESIAN_POINT('Ctrl Pts',(25.3736367778845,-0.973466666000178,
12.));
#175191=CARTESIAN_POINT('Ctrl Pts',(25.3979126089163,-0.962030544503156,
12.));
#175192=CARTESIAN_POINT('Ctrl Pts',(25.4222289223167,-0.950507148597483,
12.));
#175193=CARTESIAN_POINT('Ctrl Pts',(25.4465852044849,-0.938896449496205,
12.));
#175194=CARTESIAN_POINT('Ctrl Pts',(25.4709809475009,-0.927198419886108,
12.));
#175195=CARTESIAN_POINT('Ctrl Pts',(25.4954156541795,-0.915413034335626,
12.));
#175196=CARTESIAN_POINT('Ctrl Pts',(25.5198888424194,-0.903540269651121,
12.));
#175197=CARTESIAN_POINT('Ctrl Pts',(25.5444000508211,-0.891580105349052,
12.));
#175198=CARTESIAN_POINT('Ctrl Pts',(25.5689488408156,-0.879532523834308,
12.));
#175199=CARTESIAN_POINT('Ctrl Pts',(25.5935347843585,-0.867397509338443,
12.));
#175200=CARTESIAN_POINT('Ctrl Pts',(25.6181574536049,-0.855175047036563,
12.));
#175201=CARTESIAN_POINT('Ctrl Pts',(25.6428164100055,-0.842865122120773,
12.));
#175202=CARTESIAN_POINT('Ctrl Pts',(25.6675111931952,-0.830467718864221,
12.));
#175203=CARTESIAN_POINT('Ctrl Pts',(25.6922413110194,-0.817982819787478,
12.));
#175204=CARTESIAN_POINT('Ctrl Pts',(25.7170062262525,-0.805410404554366,
12.));
#175205=CARTESIAN_POINT('Ctrl Pts',(25.7418053757746,-0.79275045161614,
12.));
#175206=CARTESIAN_POINT('Ctrl Pts',(25.7666381946955,-0.780002940291977,
12.));
#175207=CARTESIAN_POINT('Ctrl Pts',(25.7915041383376,-0.767167852651183,
12.));
#175208=CARTESIAN_POINT('Ctrl Pts',(25.8164027059984,-0.754245175609537,
12.));
#175209=CARTESIAN_POINT('Ctrl Pts',(25.8413334619054,-0.74123490266382,
12.));
#175210=CARTESIAN_POINT('Ctrl Pts',(25.8662960624185,-0.728137036482349,
12.));
#175211=CARTESIAN_POINT('Ctrl Pts',(25.8912902614969,-0.714951588527653,
12.));
#175212=CARTESIAN_POINT('Ctrl Pts',(25.9163158909426,-0.701678575228769,
12.));
#175213=CARTESIAN_POINT('Ctrl Pts',(25.9413728471909,-0.688318015057744,
12.));
#175214=CARTESIAN_POINT('Ctrl Pts',(25.9614434297919,-0.67755954320974,
12.));
#175215=CARTESIAN_POINT('Ctrl Pts',(25.9765104298071,-0.669451306780839,
12.));
#175216=CARTESIAN_POINT('Ctrl Pts',(25.9865613464773,-0.66402831318764,
12.));
#175217=CARTESIAN_POINT('Ctrl Pts',(25.991588367311,-0.661312440730916,
12.));
#175218=CARTESIAN_POINT('',(25.991588367311,0.661312440730894,12.));
#175219=CARTESIAN_POINT('Origin',(0.,0.,12.));
#175220=CARTESIAN_POINT('',(22.4835757167854,1.76341220531179,12.));
#175221=CARTESIAN_POINT('Ctrl Pts',(25.991588367311,0.661312440730894,12.));
#175222=CARTESIAN_POINT('Ctrl Pts',(25.9865613464809,0.664028313188916,
12.));
#175223=CARTESIAN_POINT('Ctrl Pts',(25.9765104298171,0.669451306784419,
12.));
#175224=CARTESIAN_POINT('Ctrl Pts',(25.9614434298092,0.677559543215907,
12.));
#175225=CARTESIAN_POINT('Ctrl Pts',(25.941372847213,0.68831801506568,12.));
#175226=CARTESIAN_POINT('Ctrl Pts',(25.9163158909645,0.701678575236605,
12.));
#175227=CARTESIAN_POINT('Ctrl Pts',(25.8912902615141,0.714951588533756,
12.));
#175228=CARTESIAN_POINT('Ctrl Pts',(25.8662960624285,0.728137036485881,
12.));
#175229=CARTESIAN_POINT('Ctrl Pts',(25.841333461908,0.741234902664698,12.));
#175230=CARTESIAN_POINT('Ctrl Pts',(25.816402705995,0.754245175608291,12.));
#175231=CARTESIAN_POINT('Ctrl Pts',(25.7915041383304,0.767167852648643,
12.));
#175232=CARTESIAN_POINT('Ctrl Pts',(25.7666381946871,0.780002940289028,
12.));
#175233=CARTESIAN_POINT('Ctrl Pts',(25.7418053757671,0.792750451613538,
12.));
#175234=CARTESIAN_POINT('Ctrl Pts',(25.7170062262474,0.805410404552597,
12.));
#175235=CARTESIAN_POINT('Ctrl Pts',(25.6922413110172,0.817982819786722,
12.));
#175236=CARTESIAN_POINT('Ctrl Pts',(25.6675111931957,0.83046771886437,12.));
#175237=CARTESIAN_POINT('Ctrl Pts',(25.6428164100078,0.842865122121547,
12.));
#175238=CARTESIAN_POINT('Ctrl Pts',(25.618157453608,0.855175047037618,12.));
#175239=CARTESIAN_POINT('Ctrl Pts',(25.5935347843616,0.867397509339473,
12.));
#175240=CARTESIAN_POINT('Ctrl Pts',(25.568948840818,0.879532523835094,12.));
#175241=CARTESIAN_POINT('Ctrl Pts',(25.5444000508223,0.891580105349469,
12.));
#175242=CARTESIAN_POINT('Ctrl Pts',(25.5198888424195,0.903540269651155,
12.));
#175243=CARTESIAN_POINT('Ctrl Pts',(25.4954156541787,0.915413034335334,
12.));
#175244=CARTESIAN_POINT('Ctrl Pts',(25.4709809474996,0.927198419885607,
12.));
#175245=CARTESIAN_POINT('Ctrl Pts',(25.4465852044835,0.938896449495636,
12.));
#175246=CARTESIAN_POINT('Ctrl Pts',(25.4222289223155,0.950507148596971,
12.));
#175247=CARTESIAN_POINT('Ctrl Pts',(25.3979126089155,0.962030544502806,
12.));
#175248=CARTESIAN_POINT('Ctrl Pts',(25.3736367778842,0.97346666600005,12.));
#175249=CARTESIAN_POINT('Ctrl Pts',(25.3494019441444,0.984815543004091,
12.));
#175250=CARTESIAN_POINT('Ctrl Pts',(25.3252086182976,0.996077206120921,
12.));
#175251=CARTESIAN_POINT('Ctrl Pts',(25.3010573055557,1.00725168656934,12.));
#175252=CARTESIAN_POINT('Ctrl Pts',(25.2769485087268,1.01833901642273,12.));
#175253=CARTESIAN_POINT('Ctrl Pts',(25.2528827300427,1.0293392287683,12.));
#175254=CARTESIAN_POINT('Ctrl Pts',(25.2288604735087,1.04025235791515,12.));
#175255=CARTESIAN_POINT('Ctrl Pts',(25.2048822469027,1.05107843957926,12.));
#175256=CARTESIAN_POINT('Ctrl Pts',(25.1809485642191,1.06181751111754,12.));
#175257=CARTESIAN_POINT('Ctrl Pts',(25.1570599469311,1.0724696116546,12.));
#175258=CARTESIAN_POINT('Ctrl Pts',(25.1332169227415,1.08303478197174,12.));
#175259=CARTESIAN_POINT('Ctrl Pts',(25.1094200248448,1.09351306445299,12.));
#175260=CARTESIAN_POINT('Ctrl Pts',(25.085669790968,1.10390450301741,12.));
#175261=CARTESIAN_POINT('Ctrl Pts',(25.0619667625336,1.1142091430689,12.));
#175262=CARTESIAN_POINT('Ctrl Pts',(25.0383114836898,1.12442703144455,12.));
#175263=CARTESIAN_POINT('Ctrl Pts',(25.0147045006193,1.13455821638536,12.));
#175264=CARTESIAN_POINT('Ctrl Pts',(24.9911463621431,1.14460274758206,12.));
#175265=CARTESIAN_POINT('Ctrl Pts',(24.9676376201501,1.15456067621894,12.));
#175266=CARTESIAN_POINT('Ctrl Pts',(24.9441788300932,1.16443205502852,12.));
#175267=CARTESIAN_POINT('Ctrl Pts',(24.9207705514449,1.1742169383504,12.));
#175268=CARTESIAN_POINT('Ctrl Pts',(24.8974133481829,1.18391538220098,12.));
#175269=CARTESIAN_POINT('Ctrl Pts',(24.8741077892074,1.19352744434059,12.));
#175270=CARTESIAN_POINT('Ctrl Pts',(24.8508544481973,1.20305318426016,12.));
#175271=CARTESIAN_POINT('Ctrl Pts',(24.8276539035092,1.21249266318205,12.));
#175272=CARTESIAN_POINT('Ctrl Pts',(24.8045067380536,1.22184594406527,12.));
#175273=CARTESIAN_POINT('Ctrl Pts',(24.78141353918,1.23111309161843,12.));
#175274=CARTESIAN_POINT('Ctrl Pts',(24.7583748985439,1.24029417231988,12.));
#175275=CARTESIAN_POINT('Ctrl Pts',(24.7353914120012,1.24938925444324,12.));
#175276=CARTESIAN_POINT('Ctrl Pts',(24.7124636797895,1.25839840807415,12.));
#175277=CARTESIAN_POINT('Ctrl Pts',(24.6895923066837,1.26732170513497,12.));
#175278=CARTESIAN_POINT('Ctrl Pts',(24.666777902156,1.2761592194164,12.));
#175279=CARTESIAN_POINT('Ctrl Pts',(24.6440210805278,1.28491102661514,12.));
#175280=CARTESIAN_POINT('Ctrl Pts',(24.6213224611228,1.29357720438108,12.));
#175281=CARTESIAN_POINT('Ctrl Pts',(24.5986826684025,1.30215783236364,12.));
#175282=CARTESIAN_POINT('Ctrl Pts',(24.576102332018,1.31065299222023,12.));
#175283=CARTESIAN_POINT('Ctrl Pts',(24.5535820868671,1.31906276763669,12.));
#175284=CARTESIAN_POINT('Ctrl Pts',(24.5311225731434,1.32738724435326,12.));
#175285=CARTESIAN_POINT('Ctrl Pts',(24.5087244363856,1.33562651019684,12.));
#175286=CARTESIAN_POINT('Ctrl Pts',(24.4863883275135,1.34378065512335,12.));
#175287=CARTESIAN_POINT('Ctrl Pts',(24.4641149028894,1.35184977125645,12.));
#175288=CARTESIAN_POINT('Ctrl Pts',(24.4419048244524,1.35983395290624,12.));
#175289=CARTESIAN_POINT('Ctrl Pts',(24.4197587598337,1.36773329659954,12.));
#175290=CARTESIAN_POINT('Ctrl Pts',(24.3976773824731,1.37554790111608,12.));
#175291=CARTESIAN_POINT('Ctrl Pts',(24.37566137173,1.38327786752998,12.));
#175292=CARTESIAN_POINT('Ctrl Pts',(24.3537114129877,1.3909232992639,12.));
#175293=CARTESIAN_POINT('Ctrl Pts',(24.3318281977647,1.3984843021281,12.));
#175294=CARTESIAN_POINT('Ctrl Pts',(24.3100124238316,1.40596098434341,12.));
#175295=CARTESIAN_POINT('Ctrl Pts',(24.2882647953214,1.41335345657685,12.));
#175296=CARTESIAN_POINT('Ctrl Pts',(24.2665860228357,1.42066183198252,12.));
#175297=CARTESIAN_POINT('Ctrl Pts',(24.2449768235485,1.42788622624851,12.));
#175298=CARTESIAN_POINT('Ctrl Pts',(24.2234379212978,1.43502675765502,12.));
#175299=CARTESIAN_POINT('Ctrl Pts',(24.2019700467214,1.44208354711074,12.));
#175300=CARTESIAN_POINT('Ctrl Pts',(24.1805739374033,1.44905671818721,12.));
#175301=CARTESIAN_POINT('Ctrl Pts',(24.1592503380105,1.45594639716314,12.));
#175302=CARTESIAN_POINT('Ctrl Pts',(24.1380000004272,1.46275271307398,12.));
#175303=CARTESIAN_POINT('Ctrl Pts',(24.1168236838827,1.46947579776992,12.));
#175304=CARTESIAN_POINT('Ctrl Pts',(24.0957221550782,1.47611578597742,12.));
#175305=CARTESIAN_POINT('Ctrl Pts',(24.074696188353,1.4826728153368,12.));
#175306=CARTESIAN_POINT('Ctrl Pts',(24.053746565843,1.48914702644883,12.));
#175307=CARTESIAN_POINT('Ctrl Pts',(24.0328740776331,1.49553856292798,12.));
#175308=CARTESIAN_POINT('Ctrl Pts',(24.0120795219086,1.50184757146099,12.));
#175309=CARTESIAN_POINT('Ctrl Pts',(23.991363705093,1.50807420187703,12.));
#175310=CARTESIAN_POINT('Ctrl Pts',(23.9707274420145,1.51421860720628,12.));
#175311=CARTESIAN_POINT('Ctrl Pts',(23.9501715561038,1.52028094372806,12.));
#175312=CARTESIAN_POINT('Ctrl Pts',(23.9296968795761,1.5262613710304,12.));
#175313=CARTESIAN_POINT('Ctrl Pts',(23.9093042536119,1.53216005207462,12.));
#175314=CARTESIAN_POINT('Ctrl Pts',(23.8889945285313,1.53797715326748,12.));
#175315=CARTESIAN_POINT('Ctrl Pts',(23.8687685639635,1.54371284453978,12.));
#175316=CARTESIAN_POINT('Ctrl Pts',(23.8486272290698,1.5493672994053,12.));
#175317=CARTESIAN_POINT('Ctrl Pts',(23.8285714027631,1.55494069502628,12.));
#175318=CARTESIAN_POINT('Ctrl Pts',(23.8086019739192,1.56043321228631,12.));
#175319=CARTESIAN_POINT('Ctrl Pts',(23.788719841588,1.56584503586844,12.));
#175320=CARTESIAN_POINT('Ctrl Pts',(23.7689259151869,1.57117635434412,12.));
#175321=CARTESIAN_POINT('Ctrl Pts',(23.7492211147369,1.57642736025251,12.));
#175322=CARTESIAN_POINT('Ctrl Pts',(23.7296063711308,1.58159825017362,12.));
#175323=CARTESIAN_POINT('Ctrl Pts',(23.7100826263835,1.58668922481222,12.));
#175324=CARTESIAN_POINT('Ctrl Pts',(23.6906508338832,1.59170048908631,12.));
#175325=CARTESIAN_POINT('Ctrl Pts',(23.6713119586302,1.59663225222459,12.));
#175326=CARTESIAN_POINT('Ctrl Pts',(23.6520669774863,1.60148472786588,12.));
#175327=CARTESIAN_POINT('Ctrl Pts',(23.6329168794916,1.60625813414666,12.));
#175328=CARTESIAN_POINT('Ctrl Pts',(23.6138626661644,1.61095269379773,12.));
#175329=CARTESIAN_POINT('Ctrl Pts',(23.5949053517996,1.61556863424697,12.));
#175330=CARTESIAN_POINT('Ctrl Pts',(23.5760459637608,1.62010618772869,12.));
#175331=CARTESIAN_POINT('Ctrl Pts',(23.5572855427617,1.62456559140072,12.));
#175332=CARTESIAN_POINT('Ctrl Pts',(23.5386251432278,1.62894708745231,12.));
#175333=CARTESIAN_POINT('Ctrl Pts',(23.5200658336624,1.63325092321731,12.));
#175334=CARTESIAN_POINT('Ctrl Pts',(23.5016086970006,1.63747735129474,12.));
#175335=CARTESIAN_POINT('Ctrl Pts',(23.4832548309638,1.64162662967525,12.));
#175336=CARTESIAN_POINT('Ctrl Pts',(23.4650053483919,1.64569902187608,12.));
#175337=CARTESIAN_POINT('Ctrl Pts',(23.446861377656,1.6496947970734,12.));
#175338=CARTESIAN_POINT('Ctrl Pts',(23.4288240631034,1.6536142302373,12.));
#175339=CARTESIAN_POINT('Ctrl Pts',(23.4108945654803,1.65745760227507,12.));
#175340=CARTESIAN_POINT('Ctrl Pts',(23.3930740623622,1.66122520018008,12.));
#175341=CARTESIAN_POINT('Ctrl Pts',(23.375363748555,1.66491731718864,12.));
#175342=CARTESIAN_POINT('Ctrl Pts',(23.3577648365747,1.66853425293978,12.));
#175343=CARTESIAN_POINT('Ctrl Pts',(23.3402785571866,1.67207631363905,12.));
#175344=CARTESIAN_POINT('Ctrl Pts',(23.3229061599145,1.67554381222988,12.));
#175345=CARTESIAN_POINT('Ctrl Pts',(23.3056489135611,1.67893706857123,12.));
#175346=CARTESIAN_POINT('Ctrl Pts',(23.2885081066949,1.68225640962181,12.));
#175347=CARTESIAN_POINT('Ctrl Pts',(23.2714850482245,1.68550216963275,12.));
#175348=CARTESIAN_POINT('Ctrl Pts',(23.2545810680536,1.6886746903491,12.));
#175349=CARTESIAN_POINT('Ctrl Pts',(23.2377975177014,1.69177432121716,12.));
#175350=CARTESIAN_POINT('Ctrl Pts',(23.2211357709374,1.69480141959946,12.));
#175351=CARTESIAN_POINT('Ctrl Pts',(23.2045972243765,1.69775635099425,12.));
#175352=CARTESIAN_POINT('Ctrl Pts',(23.1881832981848,1.70063948926988,12.));
#175353=CARTESIAN_POINT('Ctrl Pts',(23.1718954368749,1.70345121691259,12.));
#175354=CARTESIAN_POINT('Ctrl Pts',(23.1557351100613,1.70619192527847,12.));
#175355=CARTESIAN_POINT('Ctrl Pts',(23.1397038132358,1.7088620148546,12.));
#175356=CARTESIAN_POINT('Ctrl Pts',(23.1238030684929,1.71146189552192,12.));
#175357=CARTESIAN_POINT('Ctrl Pts',(23.1080344254291,1.71399198684725,12.));
#175358=CARTESIAN_POINT('Ctrl Pts',(23.0923994621216,1.71645271839311,12.));
#175359=CARTESIAN_POINT('Ctrl Pts',(23.0768997860709,1.71884453003027,12.));
#175360=CARTESIAN_POINT('Ctrl Pts',(23.0615370351559,1.72116787225981,12.));
#175361=CARTESIAN_POINT('Ctrl Pts',(23.0463128785528,1.72342320653731,12.));
#175362=CARTESIAN_POINT('Ctrl Pts',(23.031229017888,1.72561100564033,12.));
#175363=CARTESIAN_POINT('Ctrl Pts',(23.0162871884167,1.72773175404703,12.));
#175364=CARTESIAN_POINT('Ctrl Pts',(23.0014891601891,1.72978594832137,12.));
#175365=CARTESIAN_POINT('Ctrl Pts',(22.9868367391978,1.73177409750194,12.));
#175366=CARTESIAN_POINT('Ctrl Pts',(22.9723317685688,1.73369672350818,12.));
#175367=CARTESIAN_POINT('Ctrl Pts',(22.9579761301062,1.73555436162771,12.));
#175368=CARTESIAN_POINT('Ctrl Pts',(22.9437717457825,1.73734756100038,12.));
#175369=CARTESIAN_POINT('Ctrl Pts',(22.9297205792587,1.73907688511665,12.));
#175370=CARTESIAN_POINT('Ctrl Pts',(22.9158246373365,1.74074291231057,12.));
#175371=CARTESIAN_POINT('Ctrl Pts',(22.9020859716144,1.74234623630079,12.));
#175372=CARTESIAN_POINT('Ctrl Pts',(22.8885066803351,1.74388746677702,12.));
#175373=CARTESIAN_POINT('Ctrl Pts',(22.8750889101696,1.745367229982,12.));
#175374=CARTESIAN_POINT('Ctrl Pts',(22.8618348580234,1.74678616930663,12.));
#175375=CARTESIAN_POINT('Ctrl Pts',(22.8487467728075,1.74814494588492,12.));
#175376=CARTESIAN_POINT('Ctrl Pts',(22.8358269579854,1.74944423940117,12.));
#175377=CARTESIAN_POINT('Ctrl Pts',(22.8230777741285,1.75068474890884,12.));
#175378=CARTESIAN_POINT('Ctrl Pts',(22.8105016414712,1.7518671936559,12.));
#175379=CARTESIAN_POINT('Ctrl Pts',(22.7981010424312,1.75299231391461,12.));
#175380=CARTESIAN_POINT('Ctrl Pts',(22.7858785242358,1.7540608718293,12.));
#175381=CARTESIAN_POINT('Ctrl Pts',(22.7738367016115,1.75507365227127,12.));
#175382=CARTESIAN_POINT('Ctrl Pts',(22.7619782595013,1.75603146371641,12.));
#175383=CARTESIAN_POINT('Ctrl Pts',(22.7503059556455,1.75693513908911,12.));
#175384=CARTESIAN_POINT('Ctrl Pts',(22.7388226235565,1.75778553673249,12.));
#175385=CARTESIAN_POINT('Ctrl Pts',(22.7275311777305,1.75858354204635,12.));
#175386=CARTESIAN_POINT('Ctrl Pts',(22.7164346186007,1.75933006905924,12.));
#175387=CARTESIAN_POINT('Ctrl Pts',(22.7055360375481,1.76002606202399,12.));
#175388=CARTESIAN_POINT('Ctrl Pts',(22.6948386219843,1.76067249704884,12.));
#175389=CARTESIAN_POINT('Ctrl Pts',(22.6843456585245,1.76127038310613,12.));
#175390=CARTESIAN_POINT('Ctrl Pts',(22.6740605356699,1.76182076289525,12.));
#175391=CARTESIAN_POINT('Ctrl Pts',(22.6639867471756,1.76232471392568,12.));
#175392=CARTESIAN_POINT('Ctrl Pts',(22.6541278938413,1.76278334912559,12.));
#175393=CARTESIAN_POINT('Ctrl Pts',(22.6444876940425,1.76319782013914,12.));
#175394=CARTESIAN_POINT('Ctrl Pts',(22.635069997936,1.76356932176272,12.));
#175395=CARTESIAN_POINT('Ctrl Pts',(22.6258787994847,1.76389909571402,12.));
#175396=CARTESIAN_POINT('Ctrl Pts',(22.6169182517693,1.76418843543739,12.));
#175397=CARTESIAN_POINT('Ctrl Pts',(22.6081926681342,1.76443868648015,12.));
#175398=CARTESIAN_POINT('Ctrl Pts',(22.5997065145638,1.76465124413556,12.));
#175399=CARTESIAN_POINT('Ctrl Pts',(22.5914644078106,1.76482755288411,12.));
#175400=CARTESIAN_POINT('Ctrl Pts',(22.5834711038024,1.76496910283089,12.));
#175401=CARTESIAN_POINT('Ctrl Pts',(22.5757315316355,1.76507744026747,12.));
#175402=CARTESIAN_POINT('Ctrl Pts',(22.5682508499873,1.76515418518829,12.));
#175403=CARTESIAN_POINT('Ctrl Pts',(22.5610344912501,1.7652010450045,12.));
#175404=CARTESIAN_POINT('Ctrl Pts',(22.5540882235837,1.76521983384063,12.));
#175405=CARTESIAN_POINT('Ctrl Pts',(22.5474180954006,1.76521245524047,12.));
#175406=CARTESIAN_POINT('Ctrl Pts',(22.5410303590891,1.76518087841493,12.));
#175407=CARTESIAN_POINT('Ctrl Pts',(22.5349313983571,1.7651271156325,12.));
#175408=CARTESIAN_POINT('Ctrl Pts',(22.529127665298,1.76505320262752,12.));
#175409=CARTESIAN_POINT('Ctrl Pts',(22.5236259635515,1.76496128643369,12.));
#175410=CARTESIAN_POINT('Ctrl Pts',(22.5184336670207,1.76485369319896,12.));
#175411=CARTESIAN_POINT('Ctrl Pts',(22.5135590569554,1.76473303281159,12.));
#175412=CARTESIAN_POINT('Ctrl Pts',(22.5090112700212,1.76460218257323,12.));
#175413=CARTESIAN_POINT('Ctrl Pts',(22.5047996391978,1.76446408210366,12.));
#175414=CARTESIAN_POINT('Ctrl Pts',(22.5009332677316,1.76432160068726,12.));
#175415=CARTESIAN_POINT('Ctrl Pts',(22.4974203063191,1.76417731243462,12.));
#175416=CARTESIAN_POINT('Ctrl Pts',(22.4942693792449,1.76403393880301,12.));
#175417=CARTESIAN_POINT('Ctrl Pts',(22.4914909094908,1.76389475965724,12.));
#175418=CARTESIAN_POINT('Ctrl Pts',(22.4890991659478,1.76376424879505,12.));
#175419=CARTESIAN_POINT('Ctrl Pts',(22.4871115206571,1.76364784232963,12.));
#175420=CARTESIAN_POINT('Ctrl Pts',(22.4855446605991,1.76355076045546,12.));
#175421=CARTESIAN_POINT('Ctrl Pts',(22.4844112933129,1.76347698284792,12.));
#175422=CARTESIAN_POINT('Ctrl Pts',(22.4838562517069,1.76343813434565,12.));
#175423=CARTESIAN_POINT('Ctrl Pts',(22.4836387052232,1.7634206426357,12.));
#175424=CARTESIAN_POINT('Ctrl Pts',(22.483581992979,1.76341415538764,12.));
#175425=CARTESIAN_POINT('Ctrl Pts',(22.4835757167854,1.76341220531179,12.));
#175426=CARTESIAN_POINT('',(21.9269795755927,1.71975774210841,12.));
#175427=CARTESIAN_POINT('',(10.7170877657712,0.840553282521227,12.));
#175428=CARTESIAN_POINT('',(21.3904321633055,2.16781269186828,12.));
#175429=CARTESIAN_POINT('Origin',(21.8878840740801,2.21822694051638,12.));
#175430=CARTESIAN_POINT('',(21.2226420728916,3.44230496120419,12.));
#175431=CARTESIAN_POINT('Origin',(7.7715611723761E-13,7.16093850883226E-14,
12.));
#175432=CARTESIAN_POINT('',(21.624941921198,4.01396149767428,12.));
#175433=CARTESIAN_POINT('Origin',(21.7161918885402,3.52235856495312,12.));
#175434=CARTESIAN_POINT('',(22.1738711152697,4.11585220600461,12.));
#175435=CARTESIAN_POINT('',(11.0869355576349,2.05792610300232,12.));
#175436=CARTESIAN_POINT('',(25.2771067246846,6.08833931617698,12.));
#175437=CARTESIAN_POINT('Ctrl Pts',(22.1738711152697,4.11585220600461,12.));
#175438=CARTESIAN_POINT('Ctrl Pts',(22.1738776823239,4.11585194677412,12.));
#175439=CARTESIAN_POINT('Ctrl Pts',(22.1739341411684,4.1158603587821,12.));
#175440=CARTESIAN_POINT('Ctrl Pts',(22.174148802123,4.11589976826061,12.));
#175441=CARTESIAN_POINT('Ctrl Pts',(22.1746949858773,4.11600589882768,12.));
#175442=CARTESIAN_POINT('Ctrl Pts',(22.1758088296598,4.11622797217066,12.));
#175443=CARTESIAN_POINT('Ctrl Pts',(22.177347426894,4.11653973150558,12.));
#175444=CARTESIAN_POINT('Ctrl Pts',(22.179297473024,4.11694173195041,12.));
#175445=CARTESIAN_POINT('Ctrl Pts',(22.1816414985788,4.11743469691765,12.));
#175446=CARTESIAN_POINT('Ctrl Pts',(22.1843613164855,4.11801938107464,12.));
#175447=CARTESIAN_POINT('Ctrl Pts',(22.1874419861496,4.11869641271752,12.));
#175448=CARTESIAN_POINT('Ctrl Pts',(22.1908725908525,4.11946626228623,12.));
#175449=CARTESIAN_POINT('Ctrl Pts',(22.1946440958098,4.12032932637738,12.));
#175450=CARTESIAN_POINT('Ctrl Pts',(22.1987479618246,4.12128598183533,12.));
#175451=CARTESIAN_POINT('Ctrl Pts',(22.2031746532106,4.12233664408237,12.));
#175452=CARTESIAN_POINT('Ctrl Pts',(22.2079143941719,4.12348173702025,12.));
#175453=CARTESIAN_POINT('Ctrl Pts',(22.2129576146671,4.12472167516602,12.));
#175454=CARTESIAN_POINT('Ctrl Pts',(22.2182956401341,4.126056836133,12.));
#175455=CARTESIAN_POINT('Ctrl Pts',(22.2239207458781,4.127487558301,12.));
#175456=CARTESIAN_POINT('Ctrl Pts',(22.2298258043947,4.12901415463379,12.));
#175457=CARTESIAN_POINT('Ctrl Pts',(22.2360040565534,4.13063692157499,12.));
#175458=CARTESIAN_POINT('Ctrl Pts',(22.2424488153523,4.1323561506016,12.));
#175459=CARTESIAN_POINT('Ctrl Pts',(22.2491535317789,4.13417212558809,12.));
#175460=CARTESIAN_POINT('Ctrl Pts',(22.2561118708422,4.13608511977226,12.));
#175461=CARTESIAN_POINT('Ctrl Pts',(22.263317791397,4.13809539255419,12.));
#175462=CARTESIAN_POINT('Ctrl Pts',(22.2707656042456,4.14020318715988,12.));
#175463=CARTESIAN_POINT('Ctrl Pts',(22.2784499072026,4.14240873321982,12.));
#175464=CARTESIAN_POINT('Ctrl Pts',(22.2863655389167,4.14471224859295,12.));
#175465=CARTESIAN_POINT('Ctrl Pts',(22.2945075198468,4.14711394168559,12.));
#175466=CARTESIAN_POINT('Ctrl Pts',(22.3028710166935,4.14961401285526,12.));
#175467=CARTESIAN_POINT('Ctrl Pts',(22.3114513545186,4.15221265396993,12.));
#175468=CARTESIAN_POINT('Ctrl Pts',(22.3202440186979,4.15491004835278,12.));
#175469=CARTESIAN_POINT('Ctrl Pts',(22.3292446628957,4.15770637047882,12.));
#175470=CARTESIAN_POINT('Ctrl Pts',(22.3384491078599,4.16060178604154,12.));
#175471=CARTESIAN_POINT('Ctrl Pts',(22.3478533253886,4.1635964526318,12.));
#175472=CARTESIAN_POINT('Ctrl Pts',(22.3574534257397,4.16669052026602,12.));
#175473=CARTESIAN_POINT('Ctrl Pts',(22.3672456427605,4.1698841319947,12.));
#175474=CARTESIAN_POINT('Ctrl Pts',(22.3772263228624,4.17317742436162,12.));
#175475=CARTESIAN_POINT('Ctrl Pts',(22.3873919231339,4.17657052752834,12.));
#175476=CARTESIAN_POINT('Ctrl Pts',(22.3977390078074,4.18006356544879,12.));
#175477=CARTESIAN_POINT('Ctrl Pts',(22.4082642454448,4.18365665600839,12.));
#175478=CARTESIAN_POINT('Ctrl Pts',(22.4189644056109,4.18734991117707,12.));
#175479=CARTESIAN_POINT('Ctrl Pts',(22.4298363535416,4.19114343726932,12.));
#175480=CARTESIAN_POINT('Ctrl Pts',(22.4408770448917,4.1950373351886,12.));
#175481=CARTESIAN_POINT('Ctrl Pts',(22.4520835205422,4.19903170066358,12.));
#175482=CARTESIAN_POINT('Ctrl Pts',(22.4634529011437,4.20312662448174,12.));
#175483=CARTESIAN_POINT('Ctrl Pts',(22.4749823839917,4.20732219265649,12.));
#175484=CARTESIAN_POINT('Ctrl Pts',(22.4866692403147,4.21161848657428,12.));
#175485=CARTESIAN_POINT('Ctrl Pts',(22.4985108124228,4.21601558313906,12.));
#175486=CARTESIAN_POINT('Ctrl Pts',(22.5105045108881,4.22051355490196,12.));
#175487=CARTESIAN_POINT('Ctrl Pts',(22.5226478117886,4.22511247020041,12.));
#175488=CARTESIAN_POINT('Ctrl Pts',(22.5349382540588,4.22981239330733,12.));
#175489=CARTESIAN_POINT('Ctrl Pts',(22.5473734368086,4.23461338456712,12.));
#175490=CARTESIAN_POINT('Ctrl Pts',(22.5599510166429,4.23951550052523,12.));
#175491=CARTESIAN_POINT('Ctrl Pts',(22.572668704992,4.24451879404851,12.));
#175492=CARTESIAN_POINT('Ctrl Pts',(22.5855242662477,4.24962331444177,12.));
#175493=CARTESIAN_POINT('Ctrl Pts',(22.5985155158636,4.25482910755481,12.));
#175494=CARTESIAN_POINT('Ctrl Pts',(22.6116403184821,4.26013621588305,12.));
#175495=CARTESIAN_POINT('Ctrl Pts',(22.6248965859977,4.26554467865576,12.));
#175496=CARTESIAN_POINT('Ctrl Pts',(22.6382822758172,4.27105453193004,12.));
#175497=CARTESIAN_POINT('Ctrl Pts',(22.6517953893303,4.2766658086912,12.));
#175498=CARTESIAN_POINT('Ctrl Pts',(22.6654339703109,4.28237853894059,12.));
#175499=CARTESIAN_POINT('Ctrl Pts',(22.6791961033537,4.28819274977763,12.));
#175500=CARTESIAN_POINT('Ctrl Pts',(22.6930799122548,4.29410846547056,12.));
#175501=CARTESIAN_POINT('Ctrl Pts',(22.7070835587564,4.3001257075406,12.));
#175502=CARTESIAN_POINT('Ctrl Pts',(22.7212052413386,4.30624449484069,12.));
#175503=CARTESIAN_POINT('Ctrl Pts',(22.7354431939926,4.31246484362549,12.));
#175504=CARTESIAN_POINT('Ctrl Pts',(22.7497956849848,4.31878676761235,12.));
#175505=CARTESIAN_POINT('Ctrl Pts',(22.7642610156475,4.32521027803754,12.));
#175506=CARTESIAN_POINT('Ctrl Pts',(22.7788375194076,4.3317353837319,12.));
#175507=CARTESIAN_POINT('Ctrl Pts',(22.7935235607806,4.33836209118446,12.));
#175508=CARTESIAN_POINT('Ctrl Pts',(22.8083175343791,4.34509040460062,12.));
#175509=CARTESIAN_POINT('Ctrl Pts',(22.8232178638876,4.35192032594791,12.));
#175510=CARTESIAN_POINT('Ctrl Pts',(22.8382230011184,4.35885185500546,12.));
#175511=CARTESIAN_POINT('Ctrl Pts',(22.8533314252422,4.36588498942997,12.));
#175512=CARTESIAN_POINT('Ctrl Pts',(22.8685416419725,4.37301972480746,12.));
#175513=CARTESIAN_POINT('Ctrl Pts',(22.8838521827701,4.38025605470093,12.));
#175514=CARTESIAN_POINT('Ctrl Pts',(22.8992616040108,4.38759397068406,12.));
#175515=CARTESIAN_POINT('Ctrl Pts',(22.9147684862426,4.39503346238473,12.));
#175516=CARTESIAN_POINT('Ctrl Pts',(22.930371433555,4.40257451754324,12.));
#175517=CARTESIAN_POINT('Ctrl Pts',(22.9460690729093,4.41021712205554,12.));
#175518=CARTESIAN_POINT('Ctrl Pts',(22.9618600534866,4.41796126001302,12.));
#175519=CARTESIAN_POINT('Ctrl Pts',(22.977743046002,4.42580691372752,12.));
#175520=CARTESIAN_POINT('Ctrl Pts',(22.9937167421006,4.43375406376879,12.));
#175521=CARTESIAN_POINT('Ctrl Pts',(23.0097798538395,4.44180268901643,12.));
#175522=CARTESIAN_POINT('Ctrl Pts',(23.0259311131392,4.44995276669687,12.));
#175523=CARTESIAN_POINT('Ctrl Pts',(23.0421692712467,4.45820427241683,12.));
#175524=CARTESIAN_POINT('Ctrl Pts',(23.0584930981732,4.46655718018231,12.));
#175525=CARTESIAN_POINT('Ctrl Pts',(23.0749013821881,4.47501146242856,12.));
#175526=CARTESIAN_POINT('Ctrl Pts',(23.0913929293922,4.48356709006788,12.));
#175527=CARTESIAN_POINT('Ctrl Pts',(23.1079665632636,4.49222403252216,12.));
#175528=CARTESIAN_POINT('Ctrl Pts',(23.1246211242115,4.50098225775171,12.));
#175529=CARTESIAN_POINT('Ctrl Pts',(23.1413554691123,4.5098417322706,12.));
#175530=CARTESIAN_POINT('Ctrl Pts',(23.1581684708761,4.51880242116748,12.));
#175531=CARTESIAN_POINT('Ctrl Pts',(23.1750590180908,4.52786428815015,12.));
#175532=CARTESIAN_POINT('Ctrl Pts',(23.1920260146465,4.53702729557566,12.));
#175533=CARTESIAN_POINT('Ctrl Pts',(23.2090683793629,4.54629140447544,12.));
#175534=CARTESIAN_POINT('Ctrl Pts',(23.2261850456064,4.55565657456975,12.));
#175535=CARTESIAN_POINT('Ctrl Pts',(23.2433749609131,4.56512276427839,12.));
#175536=CARTESIAN_POINT('Ctrl Pts',(23.2606370866866,4.57468993076097,12.));
#175537=CARTESIAN_POINT('Ctrl Pts',(23.2779703978876,4.5843580299469,12.));
#175538=CARTESIAN_POINT('Ctrl Pts',(23.2953738827191,4.5941270165575,12.));
#175539=CARTESIAN_POINT('Ctrl Pts',(23.3128465423115,4.60399684412163,12.));
#175540=CARTESIAN_POINT('Ctrl Pts',(23.3303873903938,4.6139674649783,12.));
#175541=CARTESIAN_POINT('Ctrl Pts',(23.3479954530272,4.62403883030805,12.));
#175542=CARTESIAN_POINT('Ctrl Pts',(23.3656697683489,4.63421089016541,12.));
#175543=CARTESIAN_POINT('Ctrl Pts',(23.3834093863068,4.6444835934993,12.));
#175544=CARTESIAN_POINT('Ctrl Pts',(23.4012133683959,4.65485688816924,12.));
#175545=CARTESIAN_POINT('Ctrl Pts',(23.4190807873803,4.6653307209467,12.));
#175546=CARTESIAN_POINT('Ctrl Pts',(23.4370107270451,4.67590503753059,12.));
#175547=CARTESIAN_POINT('Ctrl Pts',(23.455002281986,4.68657978258303,12.));
#175548=CARTESIAN_POINT('Ctrl Pts',(23.4730545573853,4.69735489975024,12.));
#175549=CARTESIAN_POINT('Ctrl Pts',(23.491166668789,4.70823033167819,12.));
#175550=CARTESIAN_POINT('Ctrl Pts',(23.509337741878,4.71920602001902,12.));
#175551=CARTESIAN_POINT('Ctrl Pts',(23.5275669122372,4.7302819054303,12.));
#175552=CARTESIAN_POINT('Ctrl Pts',(23.545853325171,4.74145792760699,12.));
#175553=CARTESIAN_POINT('Ctrl Pts',(23.5641961355168,4.75273402530617,12.));
#175554=CARTESIAN_POINT('Ctrl Pts',(23.5825945074535,4.76411013636251,12.));
#175555=CARTESIAN_POINT('Ctrl Pts',(23.6010476143099,4.77558619769872,12.));
#175556=CARTESIAN_POINT('Ctrl Pts',(23.6195546383624,4.78716214532098,12.));
#175557=CARTESIAN_POINT('Ctrl Pts',(23.6381147706579,4.7988379143322,12.));
#175558=CARTESIAN_POINT('Ctrl Pts',(23.6567272108628,4.81061343896432,12.));
#175559=CARTESIAN_POINT('Ctrl Pts',(23.675391167102,4.82248865259562,12.));
#175560=CARTESIAN_POINT('Ctrl Pts',(23.6941058557971,4.83446348776266,12.));
#175561=CARTESIAN_POINT('Ctrl Pts',(23.7128705015017,4.84653787616426,12.));
#175562=CARTESIAN_POINT('Ctrl Pts',(23.7316843367313,4.85871174865499,12.));
#175563=CARTESIAN_POINT('Ctrl Pts',(23.7505466018245,4.87098503527152,12.));
#175564=CARTESIAN_POINT('Ctrl Pts',(23.7694565448049,4.88335766525573,12.));
#175565=CARTESIAN_POINT('Ctrl Pts',(23.7884134212384,4.89582956706775,12.));
#175566=CARTESIAN_POINT('Ctrl Pts',(23.8074164940896,4.90840066839344,12.));
#175567=CARTESIAN_POINT('Ctrl Pts',(23.8264650335717,4.92107089613969,12.));
#175568=CARTESIAN_POINT('Ctrl Pts',(23.8455583170057,4.93384017643432,12.));
#175569=CARTESIAN_POINT('Ctrl Pts',(23.8646956287168,4.9467084346586,12.));
#175570=CARTESIAN_POINT('Ctrl Pts',(23.8838762599218,4.95967559546561,12.));
#175571=CARTESIAN_POINT('Ctrl Pts',(23.9030995086163,4.97274158279227,12.));
#175572=CARTESIAN_POINT('Ctrl Pts',(23.9223646794592,4.98590631986533,12.));
#175573=CARTESIAN_POINT('Ctrl Pts',(23.9416710836529,4.99916972919307,12.));
#175574=CARTESIAN_POINT('Ctrl Pts',(23.961018038827,5.01253173257453,12.));
#175575=CARTESIAN_POINT('Ctrl Pts',(23.9804048689227,5.02599225112454,12.));
#175576=CARTESIAN_POINT('Ctrl Pts',(23.9998309040746,5.03955120528521,12.));
#175577=CARTESIAN_POINT('Ctrl Pts',(24.0192954804896,5.05320851483065,12.));
#175578=CARTESIAN_POINT('Ctrl Pts',(24.0387979403268,5.06696409886641,12.));
#175579=CARTESIAN_POINT('Ctrl Pts',(24.0583376315638,5.08081787581277,12.));
#175580=CARTESIAN_POINT('Ctrl Pts',(24.0779139079266,5.09476976342625,12.));
#175581=CARTESIAN_POINT('Ctrl Pts',(24.0975261288446,5.10881967883132,12.));
#175582=CARTESIAN_POINT('Ctrl Pts',(24.117173659394,5.1229675385386,12.));
#175583=CARTESIAN_POINT('Ctrl Pts',(24.1368558702443,5.13721325845745,12.));
#175584=CARTESIAN_POINT('Ctrl Pts',(24.156572137597,5.15155675390075,12.));
#175585=CARTESIAN_POINT('Ctrl Pts',(24.1763218431343,5.16599793957979,12.));
#175586=CARTESIAN_POINT('Ctrl Pts',(24.1961043738754,5.18053672961392,12.));
#175587=CARTESIAN_POINT('Ctrl Pts',(24.215919122017,5.19517303753643,12.));
#175588=CARTESIAN_POINT('Ctrl Pts',(24.2357654847765,5.20990677629173,12.));
#175589=CARTESIAN_POINT('Ctrl Pts',(24.2556428642294,5.22473785822441,12.));
#175590=CARTESIAN_POINT('Ctrl Pts',(24.2755506671526,5.23966619506289,12.));
#175591=CARTESIAN_POINT('Ctrl Pts',(24.2954883048448,5.25469169788856,12.));
#175592=CARTESIAN_POINT('Ctrl Pts',(24.3154551932222,5.26981427718796,12.));
#175593=CARTESIAN_POINT('Ctrl Pts',(24.3354507529415,5.28503384290644,12.));
#175594=CARTESIAN_POINT('Ctrl Pts',(24.3554744095075,5.30035030449059,12.));
#175595=CARTESIAN_POINT('Ctrl Pts',(24.3755255933917,5.31576357092525,12.));
#175596=CARTESIAN_POINT('Ctrl Pts',(24.3956037401293,5.33127355076037,12.));
#175597=CARTESIAN_POINT('Ctrl Pts',(24.4157082904615,5.34688015213546,12.));
#175598=CARTESIAN_POINT('Ctrl Pts',(24.4358386899152,5.36258328273639,12.));
#175599=CARTESIAN_POINT('Ctrl Pts',(24.4559943883159,5.37838284973706,12.));
#175600=CARTESIAN_POINT('Ctrl Pts',(24.4761748393322,5.39427875973831,12.));
#175601=CARTESIAN_POINT('Ctrl Pts',(24.4963794999831,5.41027091869242,12.));
#175602=CARTESIAN_POINT('Ctrl Pts',(24.5166078302107,5.42635923183411,12.));
#175603=CARTESIAN_POINT('Ctrl Pts',(24.5368592922861,5.44254360356866,12.));
#175604=CARTESIAN_POINT('Ctrl Pts',(24.5571333514841,5.45882393762244,12.));
#175605=CARTESIAN_POINT('Ctrl Pts',(24.5774294770329,5.47520013724403,12.));
#175606=CARTESIAN_POINT('Ctrl Pts',(24.5977471429365,5.49167210537235,12.));
#175607=CARTESIAN_POINT('Ctrl Pts',(24.618085828918,5.50823974481959,12.));
#175608=CARTESIAN_POINT('Ctrl Pts',(24.6384450211466,5.52490295840996,12.));
#175609=CARTESIAN_POINT('Ctrl Pts',(24.6588242134733,5.54166164919593,12.));
#175610=CARTESIAN_POINT('Ctrl Pts',(24.6792229061785,5.55851572025389,12.));
#175611=CARTESIAN_POINT('Ctrl Pts',(24.6996406035507,5.57546507427767,12.));
#175612=CARTESIAN_POINT('Ctrl Pts',(24.7200768119079,5.59250961323995,12.));
#175613=CARTESIAN_POINT('Ctrl Pts',(24.7405310372736,5.60964923798495,12.));
#175614=CARTESIAN_POINT('Ctrl Pts',(24.76100278357,5.62688384790919,12.));
#175615=CARTESIAN_POINT('Ctrl Pts',(24.7814915496728,5.64421334042248,12.));
#175616=CARTESIAN_POINT('Ctrl Pts',(24.8019968304618,5.66163761114903,12.));
#175617=CARTESIAN_POINT('Ctrl Pts',(24.822518122386,5.67915655496524,12.));
#175618=CARTESIAN_POINT('Ctrl Pts',(24.8430549277634,5.6967700667943,12.));
#175619=CARTESIAN_POINT('Ctrl Pts',(24.8636067597677,5.71447804252019,12.));
#175620=CARTESIAN_POINT('Ctrl Pts',(24.8841731467219,5.73228037976927,12.));
#175621=CARTESIAN_POINT('Ctrl Pts',(24.9047536376467,5.75017697890813,12.));
#175622=CARTESIAN_POINT('Ctrl Pts',(24.9253478043632,5.76816774342236,12.));
#175623=CARTESIAN_POINT('Ctrl Pts',(24.9459552293308,5.78625257775703,12.));
#175624=CARTESIAN_POINT('Ctrl Pts',(24.9665754954462,5.80443138549747,12.));
#175625=CARTESIAN_POINT('Ctrl Pts',(24.9872081752709,5.82270406744214,12.));
#175626=CARTESIAN_POINT('Ctrl Pts',(25.0078528200558,5.84107051963074,12.));
#175627=CARTESIAN_POINT('Ctrl Pts',(25.0285089498922,5.8595306315681,12.));
#175628=CARTESIAN_POINT('Ctrl Pts',(25.0491760405965,5.87808428385329,12.));
#175629=CARTESIAN_POINT('Ctrl Pts',(25.0698535426593,5.89673135155459,12.));
#175630=CARTESIAN_POINT('Ctrl Pts',(25.0905409050863,5.91547170844382,12.));
#175631=CARTESIAN_POINT('Ctrl Pts',(25.1112375971182,5.93430523086776,12.));
#175632=CARTESIAN_POINT('Ctrl Pts',(25.1319431317273,5.95323180187348,12.));
#175633=CARTESIAN_POINT('Ctrl Pts',(25.1526570863065,5.97225131495636,12.));
#175634=CARTESIAN_POINT('Ctrl Pts',(25.1733791296154,5.99136367859839,12.));
#175635=CARTESIAN_POINT('Ctrl Pts',(25.1941090269638,6.0105688180476,12.));
#175636=CARTESIAN_POINT('Ctrl Pts',(25.2148466201368,6.02986667390187,12.));
#175637=CARTESIAN_POINT('Ctrl Pts',(25.2355918138798,6.04925720151412,12.));
#175638=CARTESIAN_POINT('Ctrl Pts',(25.2521940105523,6.06484373634697,12.));
#175639=CARTESIAN_POINT('Ctrl Pts',(25.2646490489816,6.07657531787578,12.));
#175640=CARTESIAN_POINT('Ctrl Pts',(25.2729539149479,6.08441489609824,12.));
#175641=CARTESIAN_POINT('Ctrl Pts',(25.2771067246846,6.08833931617698,12.));
#175642=CARTESIAN_POINT('',(24.9347862158358,7.36589684767344,12.));
#175643=CARTESIAN_POINT('Origin',(0.,0.,12.));
#175644=CARTESIAN_POINT('',(21.2610617890679,7.52250298901264,12.));
#175645=CARTESIAN_POINT('Ctrl Pts',(24.9347862158358,7.36589684767344,12.));
#175646=CARTESIAN_POINT('Ctrl Pts',(24.9292275670705,7.3672190902906,12.));
#175647=CARTESIAN_POINT('Ctrl Pts',(24.9181155530631,7.36985593120697,12.));
#175648=CARTESIAN_POINT('Ctrl Pts',(24.9014633826201,7.37378825962718,12.));
#175649=CARTESIAN_POINT('Ctrl Pts',(24.8792921911309,7.3789854964161,12.));
#175650=CARTESIAN_POINT('Ctrl Pts',(24.8516310625367,7.38540558904946,12.));
#175651=CARTESIAN_POINT('Ctrl Pts',(24.8240228521042,7.39174922586841,12.));
#175652=CARTESIAN_POINT('Ctrl Pts',(24.7964676646518,7.39801641583613,12.));
#175653=CARTESIAN_POINT('Ctrl Pts',(24.7689656669005,7.40420718661755,12.));
#175654=CARTESIAN_POINT('Ctrl Pts',(24.7415170994754,7.41032159082173,12.));
#175655=CARTESIAN_POINT('Ctrl Pts',(24.7141222949988,7.41635971481243,12.));
#175656=CARTESIAN_POINT('Ctrl Pts',(24.6867816727118,7.42232167765763,12.));
#175657=CARTESIAN_POINT('Ctrl Pts',(24.659495712869,7.42820762158681,12.));
#175658=CARTESIAN_POINT('Ctrl Pts',(24.6322649369472,7.43401770489221,12.));
#175659=CARTESIAN_POINT('Ctrl Pts',(24.6050898852349,7.43975209375375,12.));
#175660=CARTESIAN_POINT('Ctrl Pts',(24.5779710960865,7.44541095473163,12.));
#175661=CARTESIAN_POINT('Ctrl Pts',(24.5509090831579,7.45099444651296,12.));
#175662=CARTESIAN_POINT('Ctrl Pts',(24.52390431731,7.45650271336046,12.));
#175663=CARTESIAN_POINT('Ctrl Pts',(24.4969572391509,7.46193588961642,12.));
#175664=CARTESIAN_POINT('Ctrl Pts',(24.4700682684544,7.46729410308923,12.));
#175665=CARTESIAN_POINT('Ctrl Pts',(24.4432378146501,7.47257747883319,12.));
#175666=CARTESIAN_POINT('Ctrl Pts',(24.4164662871165,7.47778614286574,12.));
#175667=CARTESIAN_POINT('Ctrl Pts',(24.3897541049248,7.48292022569254,12.));
#175668=CARTESIAN_POINT('Ctrl Pts',(24.3631017084513,7.48797986651828,12.));
#175669=CARTESIAN_POINT('Ctrl Pts',(24.3365095573673,7.4929652125233,12.));
#175670=CARTESIAN_POINT('Ctrl Pts',(24.3099781253345,7.49787641695359,12.));
#175671=CARTESIAN_POINT('Ctrl Pts',(24.2835078958966,7.50271363765099,12.));
#175672=CARTESIAN_POINT('Ctrl Pts',(24.2570993577032,7.50747703535115,12.));
#175673=CARTESIAN_POINT('Ctrl Pts',(24.230753000389,7.51216677222199,12.));
#175674=CARTESIAN_POINT('Ctrl Pts',(24.2044693092356,7.51678300997998,12.));
#175675=CARTESIAN_POINT('Ctrl Pts',(24.1782487641602,7.52132590953863,12.));
#175676=CARTESIAN_POINT('Ctrl Pts',(24.152091842537,7.52579563201479,12.));
#175677=CARTESIAN_POINT('Ctrl Pts',(24.1259990209211,7.53019233935537,12.));
#175678=CARTESIAN_POINT('Ctrl Pts',(24.0999707772642,7.53451619514659,12.));
#175679=CARTESIAN_POINT('Ctrl Pts',(24.0740075927984,7.53876736531005,12.));
#175680=CARTESIAN_POINT('Ctrl Pts',(24.0481099543353,7.54294601896128,12.));
#175681=CARTESIAN_POINT('Ctrl Pts',(24.0222783554531,7.54705232885895,12.));
#175682=CARTESIAN_POINT('Ctrl Pts',(23.9965132953187,7.55108647097432,12.));
#175683=CARTESIAN_POINT('Ctrl Pts',(23.9708152779886,7.55504862424808,12.));
#175684=CARTESIAN_POINT('Ctrl Pts',(23.9451848115002,7.5589389702768,12.));
#175685=CARTESIAN_POINT('Ctrl Pts',(23.9196224070759,7.56275769304773,12.));
#175686=CARTESIAN_POINT('Ctrl Pts',(23.8941285782002,7.56650497863791,12.));
#175687=CARTESIAN_POINT('Ctrl Pts',(23.8687038399595,7.57018101500709,12.));
#175688=CARTESIAN_POINT('Ctrl Pts',(23.8433487096132,7.57378599219814,12.));
#175689=CARTESIAN_POINT('Ctrl Pts',(23.8180637069976,7.57732010249066,12.));
#175690=CARTESIAN_POINT('Ctrl Pts',(23.7928493549908,7.58078354058213,12.));
#175691=CARTESIAN_POINT('Ctrl Pts',(23.7677061799376,7.58417650376271,12.));
#175692=CARTESIAN_POINT('Ctrl Pts',(23.7426347121006,7.58749919210826,12.));
#175693=CARTESIAN_POINT('Ctrl Pts',(23.7176354860456,7.59075180865321,12.));
#175694=CARTESIAN_POINT('Ctrl Pts',(23.6927090405066,7.59393455934035,12.));
#175695=CARTESIAN_POINT('Ctrl Pts',(23.6678559182875,7.59704765299567,12.));
#175696=CARTESIAN_POINT('Ctrl Pts',(23.6430766661418,7.60009130130126,12.));
#175697=CARTESIAN_POINT('Ctrl Pts',(23.6183718346576,7.60306571877806,12.));
#175698=CARTESIAN_POINT('Ctrl Pts',(23.5937419781245,7.60597112277094,12.));
#175699=CARTESIAN_POINT('Ctrl Pts',(23.5691876544244,7.608807733446,12.));
#175700=CARTESIAN_POINT('Ctrl Pts',(23.544709425203,7.61157577385372,12.));
#175701=CARTESIAN_POINT('Ctrl Pts',(23.5203078560129,7.61427546999298,12.));
#175702=CARTESIAN_POINT('Ctrl Pts',(23.4959835164609,7.61690705088319,12.));
#175703=CARTESIAN_POINT('Ctrl Pts',(23.4717369803438,7.61947074863977,12.));
#175704=CARTESIAN_POINT('Ctrl Pts',(23.4475688257854,7.62196679855955,12.));
#175705=CARTESIAN_POINT('Ctrl Pts',(23.4234796353542,7.6243954392005,12.));
#175706=CARTESIAN_POINT('Ctrl Pts',(23.399469996112,7.62675691240329,12.));
#175707=CARTESIAN_POINT('Ctrl Pts',(23.3755404996636,7.62905146332593,12.));
#175708=CARTESIAN_POINT('Ctrl Pts',(23.3516917421972,7.63127934048137,12.));
#175709=CARTESIAN_POINT('Ctrl Pts',(23.3279243245241,7.63344079578162,12.));
#175710=CARTESIAN_POINT('Ctrl Pts',(23.3042388521022,7.63553608458783,12.));
#175711=CARTESIAN_POINT('Ctrl Pts',(23.2806359350855,7.63756546576374,12.));
#175712=CARTESIAN_POINT('Ctrl Pts',(23.2571161884488,7.63952920172835,12.));
#175713=CARTESIAN_POINT('Ctrl Pts',(23.2336802320912,7.64142755851505,12.));
#175714=CARTESIAN_POINT('Ctrl Pts',(23.2103286909398,7.6432608058368,12.));
#175715=CARTESIAN_POINT('Ctrl Pts',(23.1870621950452,7.64502921715483,12.));
#175716=CARTESIAN_POINT('Ctrl Pts',(23.1638813796694,7.64673306975805,12.));
#175717=CARTESIAN_POINT('Ctrl Pts',(23.1407868853819,7.64837264482943,12.));
#175718=CARTESIAN_POINT('Ctrl Pts',(23.1177793581679,7.6499482274986,12.));
#175719=CARTESIAN_POINT('Ctrl Pts',(23.094859449525,7.65146010690476,12.));
#175720=CARTESIAN_POINT('Ctrl Pts',(23.072027816555,7.65290857626358,12.));
#175721=CARTESIAN_POINT('Ctrl Pts',(23.0492851220528,7.65429393293946,12.));
#175722=CARTESIAN_POINT('Ctrl Pts',(23.0266320345787,7.65561647852534,12.));
#175723=CARTESIAN_POINT('Ctrl Pts',(23.0040692285814,7.65687651891305,12.));
#175724=CARTESIAN_POINT('Ctrl Pts',(22.9815973845296,7.65807436436432,12.));
#175725=CARTESIAN_POINT('Ctrl Pts',(22.959217189033,7.65921032958902,12.));
#175726=CARTESIAN_POINT('Ctrl Pts',(22.9369293349593,7.66028473382778,12.));
#175727=CARTESIAN_POINT('Ctrl Pts',(22.9147345215421,7.66129790094108,12.));
#175728=CARTESIAN_POINT('Ctrl Pts',(22.8926334544883,7.66225015950156,12.));
#175729=CARTESIAN_POINT('Ctrl Pts',(22.8706268461283,7.66314184287337,12.));
#175730=CARTESIAN_POINT('Ctrl Pts',(22.848715415557,7.66397328929803,12.));
#175731=CARTESIAN_POINT('Ctrl Pts',(22.8268998887678,7.66474484198549,12.));
#175732=CARTESIAN_POINT('Ctrl Pts',(22.8051809987833,7.66545684920987,12.));
#175733=CARTESIAN_POINT('Ctrl Pts',(22.7835594857699,7.66610966441273,12.));
#175734=CARTESIAN_POINT('Ctrl Pts',(22.7620360971843,7.66670364630299,12.));
#175735=CARTESIAN_POINT('Ctrl Pts',(22.7406115879513,7.6672391589544,12.));
#175736=CARTESIAN_POINT('Ctrl Pts',(22.7192867206245,7.66771657191028,12.));
#175737=CARTESIAN_POINT('Ctrl Pts',(22.6980622655446,7.66813626029275,12.));
#175738=CARTESIAN_POINT('Ctrl Pts',(22.6769390009885,7.66849860491743,12.));
#175739=CARTESIAN_POINT('Ctrl Pts',(22.6559177133127,7.66880399241323,12.));
#175740=CARTESIAN_POINT('Ctrl Pts',(22.6349991971541,7.66905281533715,12.));
#175741=CARTESIAN_POINT('Ctrl Pts',(22.6141842556243,7.66924547229414,12.));
#175742=CARTESIAN_POINT('Ctrl Pts',(22.5934737004953,7.66938236806233,12.));
#175743=CARTESIAN_POINT('Ctrl Pts',(22.5728683523831,7.66946391372306,12.));
#175744=CARTESIAN_POINT('Ctrl Pts',(22.5523690409116,7.66949052679693,12.));
#175745=CARTESIAN_POINT('Ctrl Pts',(22.53197660492,7.66946263138144,12.));
#175746=CARTESIAN_POINT('Ctrl Pts',(22.5116918927031,7.66938065829108,12.));
#175747=CARTESIAN_POINT('Ctrl Pts',(22.4915157622312,7.66924504520315,12.));
#175748=CARTESIAN_POINT('Ctrl Pts',(22.4714490813699,7.66905623680831,12.));
#175749=CARTESIAN_POINT('Ctrl Pts',(22.4514927280855,7.66881468496635,12.));
#175750=CARTESIAN_POINT('Ctrl Pts',(22.4316475906603,7.66852084886704,12.));
#175751=CARTESIAN_POINT('Ctrl Pts',(22.4119145679758,7.6681751951964,12.));
#175752=CARTESIAN_POINT('Ctrl Pts',(22.3922945697773,7.6677781983079,12.));
#175753=CARTESIAN_POINT('Ctrl Pts',(22.372788516936,7.66733034039883,12.));
#175754=CARTESIAN_POINT('Ctrl Pts',(22.3533973417021,7.66683211169159,12.));
#175755=CARTESIAN_POINT('Ctrl Pts',(22.3341219879469,7.66628401061952,12.));
#175756=CARTESIAN_POINT('Ctrl Pts',(22.314963411484,7.66568654402494,12.));
#175757=CARTESIAN_POINT('Ctrl Pts',(22.2959225803937,7.66504022736299,12.));
#175758=CARTESIAN_POINT('Ctrl Pts',(22.2770004753335,7.66434558490979,12.));
#175759=CARTESIAN_POINT('Ctrl Pts',(22.258198089848,7.66360314997641,12.));
#175760=CARTESIAN_POINT('Ctrl Pts',(22.2395164306547,7.66281346512509,12.));
#175761=CARTESIAN_POINT('Ctrl Pts',(22.2209565180085,7.661977082404,12.));
#175762=CARTESIAN_POINT('Ctrl Pts',(22.2025193860964,7.66109456359271,12.));
#175763=CARTESIAN_POINT('Ctrl Pts',(22.1842060834091,7.66016648045005,12.));
#175764=CARTESIAN_POINT('Ctrl Pts',(22.1660176731178,7.65919341496931,12.));
#175765=CARTESIAN_POINT('Ctrl Pts',(22.1479552334211,7.65817595963349,12.));
#175766=CARTESIAN_POINT('Ctrl Pts',(22.1300198579675,7.65711471769397,12.));
#175767=CARTESIAN_POINT('Ctrl Pts',(22.1122126563329,7.65601030346807,12.));
#175768=CARTESIAN_POINT('Ctrl Pts',(22.094534754469,7.65486334263644,12.));
#175769=CARTESIAN_POINT('Ctrl Pts',(22.0769872951596,7.65367447254949,12.));
#175770=CARTESIAN_POINT('Ctrl Pts',(22.0595714384431,7.65244434253113,12.));
#175771=CARTESIAN_POINT('Ctrl Pts',(22.0422883621174,7.65117361421359,12.));
#175772=CARTESIAN_POINT('Ctrl Pts',(22.0251392623209,7.64986296190169,12.));
#175773=CARTESIAN_POINT('Ctrl Pts',(22.0081253540774,7.64851307293352,12.));
#175774=CARTESIAN_POINT('Ctrl Pts',(21.9912478718542,7.6471246480525,12.));
#175775=CARTESIAN_POINT('Ctrl Pts',(21.9745080700798,7.64569840177336,12.));
#175776=CARTESIAN_POINT('Ctrl Pts',(21.9579072237651,7.64423506279123,12.));
#175777=CARTESIAN_POINT('Ctrl Pts',(21.9414466292072,7.64273537442682,12.));
#175778=CARTESIAN_POINT('Ctrl Pts',(21.9251276046545,7.64120009506532,12.));
#175779=CARTESIAN_POINT('Ctrl Pts',(21.9089514909874,7.63962999860927,12.));
#175780=CARTESIAN_POINT('Ctrl Pts',(21.8929196523514,7.63802587492035,12.));
#175781=CARTESIAN_POINT('Ctrl Pts',(21.8770334769496,7.636388530334,12.));
#175782=CARTESIAN_POINT('Ctrl Pts',(21.8612943779089,7.63471878821226,12.));
#175783=CARTESIAN_POINT('Ctrl Pts',(21.8457037941084,7.63301748948936,12.));
#175784=CARTESIAN_POINT('Ctrl Pts',(21.8302631910195,7.63128549323023,12.));
#175785=CARTESIAN_POINT('Ctrl Pts',(21.814974061509,7.62952367718127,12.));
#175786=CARTESIAN_POINT('Ctrl Pts',(21.799837926858,7.62773293842389,12.));
#175787=CARTESIAN_POINT('Ctrl Pts',(21.7848563378021,7.62591419404513,12.));
#175788=CARTESIAN_POINT('Ctrl Pts',(21.7700308755584,7.62406838181166,12.));
#175789=CARTESIAN_POINT('Ctrl Pts',(21.7553631528328,7.62219646084229,12.));
#175790=CARTESIAN_POINT('Ctrl Pts',(21.7408548148656,7.62029941230855,12.));
#175791=CARTESIAN_POINT('Ctrl Pts',(21.7265075407975,7.61837824030538,12.));
#175792=CARTESIAN_POINT('Ctrl Pts',(21.7123230449834,7.61643397270421,12.));
#175793=CARTESIAN_POINT('Ctrl Pts',(21.6983030783322,7.61446766202787,12.));
#175794=CARTESIAN_POINT('Ctrl Pts',(21.6844494295815,7.61248038630269,12.));
#175795=CARTESIAN_POINT('Ctrl Pts',(21.6707639267576,7.61047325000956,12.));
#175796=CARTESIAN_POINT('Ctrl Pts',(21.6572484388081,7.60844738512874,12.));
#175797=CARTESIAN_POINT('Ctrl Pts',(21.6439048771743,7.60640395216357,12.));
#175798=CARTESIAN_POINT('Ctrl Pts',(21.6307351973822,7.60434414118296,12.));
#175799=CARTESIAN_POINT('Ctrl Pts',(21.617741400599,7.60226917285429,12.));
#175800=CARTESIAN_POINT('Ctrl Pts',(21.6049255358843,7.60018029988241,12.));
#175801=CARTESIAN_POINT('Ctrl Pts',(21.5922897024466,7.59807880846195,12.));
#175802=CARTESIAN_POINT('Ctrl Pts',(21.5798360518978,7.59596601973584,12.));
#175803=CARTESIAN_POINT('Ctrl Pts',(21.5675667904726,7.59384329124918,12.));
#175804=CARTESIAN_POINT('Ctrl Pts',(21.5554841813462,7.59171201844777,12.));
#175805=CARTESIAN_POINT('Ctrl Pts',(21.543590547011,7.58957363620014,12.));
#175806=CARTESIAN_POINT('Ctrl Pts',(21.5318882716736,7.58742962034834,12.));
#175807=CARTESIAN_POINT('Ctrl Pts',(21.5203798035299,7.5852814891913,12.));
#175808=CARTESIAN_POINT('Ctrl Pts',(21.5090676573873,7.5831308051918,12.));
#175809=CARTESIAN_POINT('Ctrl Pts',(21.4979544192744,7.58097917790744,12.));
#175810=CARTESIAN_POINT('Ctrl Pts',(21.4870427508194,7.57882826679132,12.));
#175811=CARTESIAN_POINT('Ctrl Pts',(21.4763353936762,7.57667978402987,12.));
#175812=CARTESIAN_POINT('Ctrl Pts',(21.4658351740128,7.57453549743412,12.));
#175813=CARTESIAN_POINT('Ctrl Pts',(21.4555450053142,7.57239723223506,12.));
#175814=CARTESIAN_POINT('Ctrl Pts',(21.4454678907509,7.57026687261166,12.));
#175815=CARTESIAN_POINT('Ctrl Pts',(21.4356069261513,7.56814636360848,12.));
#175816=CARTESIAN_POINT('Ctrl Pts',(21.4259653015736,7.56603771218712,12.));
#175817=CARTESIAN_POINT('Ctrl Pts',(21.4165463106254,7.56394299313685,12.));
#175818=CARTESIAN_POINT('Ctrl Pts',(21.4073533630365,7.56186435703622,12.));
#175819=CARTESIAN_POINT('Ctrl Pts',(21.3983899952987,7.55980403700611,12.));
#175820=CARTESIAN_POINT('Ctrl Pts',(21.3896598842117,7.55776435731417,12.));
#175821=CARTESIAN_POINT('Ctrl Pts',(21.3811668478932,7.55574773403503,12.));
#175822=CARTESIAN_POINT('Ctrl Pts',(21.3729148390243,7.55375667080029,12.));
#175823=CARTESIAN_POINT('Ctrl Pts',(21.3649079431865,7.55179375777444,12.));
#175824=CARTESIAN_POINT('Ctrl Pts',(21.3571503685855,7.5498616652131,12.));
#175825=CARTESIAN_POINT('Ctrl Pts',(21.3496464761531,7.54796316246331,12.));
#175826=CARTESIAN_POINT('Ctrl Pts',(21.3424008295038,7.54610114948347,12.));
#175827=CARTESIAN_POINT('Ctrl Pts',(21.3354182340149,7.54427868151268,12.));
#175828=CARTESIAN_POINT('Ctrl Pts',(21.328703791771,7.54249900377031,12.));
#175829=CARTESIAN_POINT('Ctrl Pts',(21.3222628524165,7.54076552038279,12.));
#175830=CARTESIAN_POINT('Ctrl Pts',(21.3161009456256,7.53908175169899,12.));
#175831=CARTESIAN_POINT('Ctrl Pts',(21.310223716773,7.53745129364616,12.));
#175832=CARTESIAN_POINT('Ctrl Pts',(21.3046368712157,7.53587778251736,12.));
#175833=CARTESIAN_POINT('Ctrl Pts',(21.2993464250717,7.53436505309943,12.));
#175834=CARTESIAN_POINT('Ctrl Pts',(21.2943588989331,7.53291726078527,12.));
#175835=CARTESIAN_POINT('Ctrl Pts',(21.2896816163842,7.53153906987856,12.));
#175836=CARTESIAN_POINT('Ctrl Pts',(21.2853226580657,7.5302356243823,12.));
#175837=CARTESIAN_POINT('Ctrl Pts',(21.2812902781143,7.52901217930408,12.));
#175838=CARTESIAN_POINT('Ctrl Pts',(21.2775925269652,7.52787386225333,12.));
#175839=CARTESIAN_POINT('Ctrl Pts',(21.2742366113579,7.52682526918541,12.));
#175840=CARTESIAN_POINT('Ctrl Pts',(21.2712301573466,7.5258712609553,12.));
#175841=CARTESIAN_POINT('Ctrl Pts',(21.2685823838671,7.52501770333531,12.));
#175842=CARTESIAN_POINT('Ctrl Pts',(21.2663059157058,7.52427261074298,12.));
#175843=CARTESIAN_POINT('Ctrl Pts',(21.2644161259962,7.52364573027553,12.));
#175844=CARTESIAN_POINT('Ctrl Pts',(21.262927782038,7.52314642316199,12.));
#175845=CARTESIAN_POINT('Ctrl Pts',(21.2618521283555,7.5227818224267,12.));
#175846=CARTESIAN_POINT('Ctrl Pts',(21.261326054066,7.52260064231661,12.));
#175847=CARTESIAN_POINT('Ctrl Pts',(21.2611204474866,7.52252744144904,12.));
#175848=CARTESIAN_POINT('Ctrl Pts',(21.2610673466886,7.5225064970397,12.));
#175849=CARTESIAN_POINT('Ctrl Pts',(21.2610617890679,7.52250298901264,12.));
#175850=CARTESIAN_POINT('',(20.7347298079577,7.33627833380046,12.));
#175851=CARTESIAN_POINT('',(10.1343606576251,3.58569854577611,12.));
#175852=CARTESIAN_POINT('',(20.1004996511507,7.63019749246977,12.));
#175853=CARTESIAN_POINT('Origin',(20.56795313141,7.80764394578302,12.));
#175854=CARTESIAN_POINT('',(19.6085639972844,8.8178352198485,12.));
#175855=CARTESIAN_POINT('Origin',(7.32141292029404E-13,2.70312158620511E-13,
12.));
#175856=CARTESIAN_POINT('',(19.84920021178,9.47413589477548,12.));
#175857=CARTESIAN_POINT('Origin',(20.0645771135003,9.02290115519381,12.));
#175858=CARTESIAN_POINT('',(20.353053841303,9.71462809124916,12.));
#175859=CARTESIAN_POINT('',(10.1765269206515,4.85731404562459,12.));
#175860=CARTESIAN_POINT('',(22.8400320311648,12.4230808101438,12.));
#175861=CARTESIAN_POINT('Ctrl Pts',(20.353053841303,9.71462809124916,12.));
#175862=CARTESIAN_POINT('Ctrl Pts',(20.353060251684,9.71462954053042,12.));
#175863=CARTESIAN_POINT('Ctrl Pts',(20.3531126095522,9.71465227853042,12.));
#175864=CARTESIAN_POINT('Ctrl Pts',(20.3533097561886,9.71474590350681,12.));
#175865=CARTESIAN_POINT('Ctrl Pts',(20.3538098605706,9.71498978052021,12.));
#175866=CARTESIAN_POINT('Ctrl Pts',(20.3548282742361,9.71549257088173,12.));
#175867=CARTESIAN_POINT('Ctrl Pts',(20.3562337557875,9.71619192554186,12.));
#175868=CARTESIAN_POINT('Ctrl Pts',(20.3580133103356,9.71708493723096,12.));
#175869=CARTESIAN_POINT('Ctrl Pts',(20.3601498764344,9.71816778328007,12.));
#175870=CARTESIAN_POINT('Ctrl Pts',(20.3626256913981,9.71943648548099,12.));
#175871=CARTESIAN_POINT('Ctrl Pts',(20.3654261611056,9.72088778381081,12.));
#175872=CARTESIAN_POINT('Ctrl Pts',(20.3685406190576,9.7225193072249,12.));
#175873=CARTESIAN_POINT('Ctrl Pts',(20.371960235676,9.72432910043194,12.));
#175874=CARTESIAN_POINT('Ctrl Pts',(20.3756766651951,9.72631531732881,12.));
#175875=CARTESIAN_POINT('Ctrl Pts',(20.3796805893304,9.72847589116542,12.));
#175876=CARTESIAN_POINT('Ctrl Pts',(20.3839624556742,9.73080870123727,12.));
#175877=CARTESIAN_POINT('Ctrl Pts',(20.3885129129912,9.73331167102808,12.));
#175878=CARTESIAN_POINT('Ctrl Pts',(20.3933234845647,9.73598292014243,12.));
#175879=CARTESIAN_POINT('Ctrl Pts',(20.3983866213331,9.73882077613201,12.));
#175880=CARTESIAN_POINT('Ctrl Pts',(20.4036953576549,9.74182369656272,12.));
#175881=CARTESIAN_POINT('Ctrl Pts',(20.4092430879861,9.74499021838538,12.));
#175882=CARTESIAN_POINT('Ctrl Pts',(20.4150232777393,9.74831889242174,12.));
#175883=CARTESIAN_POINT('Ctrl Pts',(20.4210295275817,9.7518082978643,12.));
#175884=CARTESIAN_POINT('Ctrl Pts',(20.4272556476629,9.75545705902418,12.));
#175885=CARTESIAN_POINT('Ctrl Pts',(20.4336957355473,9.75926386289923,12.));
#175886=CARTESIAN_POINT('Ctrl Pts',(20.44034423294,9.76322747195495,12.));
#175887=CARTESIAN_POINT('Ctrl Pts',(20.447195862298,9.76734670980892,12.));
#175888=CARTESIAN_POINT('Ctrl Pts',(20.4542455817527,9.7716204510407,12.));
#175889=CARTESIAN_POINT('Ctrl Pts',(20.4614885274975,9.77604760815529,12.));
#175890=CARTESIAN_POINT('Ctrl Pts',(20.4689199790669,9.78062712373321,12.));
#175891=CARTESIAN_POINT('Ctrl Pts',(20.4765353711586,9.78535797314167,12.));
#175892=CARTESIAN_POINT('Ctrl Pts',(20.4843302955329,9.79023916498656,12.));
#175893=CARTESIAN_POINT('Ctrl Pts',(20.4923005087943,9.79526974288331,12.));
#175894=CARTESIAN_POINT('Ctrl Pts',(20.5004419312107,9.80044878520949,12.));
#175895=CARTESIAN_POINT('Ctrl Pts',(20.5087506310505,9.80577540161088,12.));
#175896=CARTESIAN_POINT('Ctrl Pts',(20.517222812284,9.81124873025282,12.));
#175897=CARTESIAN_POINT('Ctrl Pts',(20.5258548000629,9.81686793455943,12.));
#175898=CARTESIAN_POINT('Ctrl Pts',(20.5346430299517,9.82263220080363,12.));
#175899=CARTESIAN_POINT('Ctrl Pts',(20.5435840460721,9.82854073773878,12.));
#175900=CARTESIAN_POINT('Ctrl Pts',(20.552674497646,9.83459277585315,12.));
#175901=CARTESIAN_POINT('Ctrl Pts',(20.5619111362402,9.84078756677565,12.));
#175902=CARTESIAN_POINT('Ctrl Pts',(20.5712908125139,9.84712438256278,12.));
#175903=CARTESIAN_POINT('Ctrl Pts',(20.5808104710015,9.85360251456981,12.));
#175904=CARTESIAN_POINT('Ctrl Pts',(20.5904671449754,9.86022127232748,12.));
#175905=CARTESIAN_POINT('Ctrl Pts',(20.6002579513699,9.86697998242623,12.));
#175906=CARTESIAN_POINT('Ctrl Pts',(20.6101800854494,9.87387798732956,12.));
#175907=CARTESIAN_POINT('Ctrl Pts',(20.6202308177474,9.88091464472676,12.));
#175908=CARTESIAN_POINT('Ctrl Pts',(20.6304074914087,9.88808932697306,12.));
#175909=CARTESIAN_POINT('Ctrl Pts',(20.6407075193976,9.8954014204912,12.));
#175910=CARTESIAN_POINT('Ctrl Pts',(20.6511283817414,9.90285032516693,12.));
#175911=CARTESIAN_POINT('Ctrl Pts',(20.6616676228315,9.91043545377008,12.));
#175912=CARTESIAN_POINT('Ctrl Pts',(20.6723228488263,9.91815623141289,12.));
#175913=CARTESIAN_POINT('Ctrl Pts',(20.6830917250255,9.92601209498749,12.));
#175914=CARTESIAN_POINT('Ctrl Pts',(20.6939719732484,9.9340024925973,12.));
#175915=CARTESIAN_POINT('Ctrl Pts',(20.7049613692234,9.94212688298236,12.));
#175916=CARTESIAN_POINT('Ctrl Pts',(20.7160577407579,9.95038473514949,12.));
#175917=CARTESIAN_POINT('Ctrl Pts',(20.7272589658751,9.95877552798398,12.));
#175918=CARTESIAN_POINT('Ctrl Pts',(20.7385629709795,9.96729874986202,12.));
#175919=CARTESIAN_POINT('Ctrl Pts',(20.7499677289627,9.9759538982347,12.));
#175920=CARTESIAN_POINT('Ctrl Pts',(20.761471257499,9.98474047926853,12.));
#175921=CARTESIAN_POINT('Ctrl Pts',(20.7730716175417,9.9936580075464,12.));
#175922=CARTESIAN_POINT('Ctrl Pts',(20.7847669117568,10.0027060057389,12.));
#175923=CARTESIAN_POINT('Ctrl Pts',(20.7965552829908,10.0118840042786,12.));
#175924=CARTESIAN_POINT('Ctrl Pts',(20.8084349126888,10.0211915410095,12.));
#175925=CARTESIAN_POINT('Ctrl Pts',(20.8204040196602,10.0306281609435,12.));
#175926=CARTESIAN_POINT('Ctrl Pts',(20.8324608588909,10.0401934160234,12.));
#175927=CARTESIAN_POINT('Ctrl Pts',(20.8446037203402,10.0498868648733,12.));
#175928=CARTESIAN_POINT('Ctrl Pts',(20.8568309277316,10.0597080725375,12.));
#175929=CARTESIAN_POINT('Ctrl Pts',(20.86914083737,10.0696566102218,12.));
#175930=CARTESIAN_POINT('Ctrl Pts',(20.881531837184,10.0797320551154,12.));
#175931=CARTESIAN_POINT('Ctrl Pts',(20.894002345737,10.0899339901916,12.));
#175932=CARTESIAN_POINT('Ctrl Pts',(20.9065508112557,10.1002620040076,12.));
#175933=CARTESIAN_POINT('Ctrl Pts',(20.919175710627,10.1107156904836,12.));
#175934=CARTESIAN_POINT('Ctrl Pts',(20.9318755484734,10.1212946487057,12.));
#175935=CARTESIAN_POINT('Ctrl Pts',(20.9446488563933,10.1319984827908,12.));
#175936=CARTESIAN_POINT('Ctrl Pts',(20.9574941921591,10.1428268017256,12.));
#175937=CARTESIAN_POINT('Ctrl Pts',(20.9704101389369,10.1537792192065,12.));
#175938=CARTESIAN_POINT('Ctrl Pts',(20.9833953044736,10.1648553534568,12.));
#175939=CARTESIAN_POINT('Ctrl Pts',(20.9964483203686,10.1760548270767,12.));
#175940=CARTESIAN_POINT('Ctrl Pts',(21.0095678414486,10.187377266936,12.));
#175941=CARTESIAN_POINT('Ctrl Pts',(21.0227525451107,10.1988223040425,12.));
#175942=CARTESIAN_POINT('Ctrl Pts',(21.0360011306815,10.2103895734123,12.));
#175943=CARTESIAN_POINT('Ctrl Pts',(21.0493123187483,10.2220787139155,12.));
#175944=CARTESIAN_POINT('Ctrl Pts',(21.0626848505663,10.2338893681567,12.));
#175945=CARTESIAN_POINT('Ctrl Pts',(21.0761174875444,10.2458211823912,12.));
#175946=CARTESIAN_POINT('Ctrl Pts',(21.0896090107063,10.2578738064181,12.));
#175947=CARTESIAN_POINT('Ctrl Pts',(21.1031582201627,10.2700468934744,12.));
#175948=CARTESIAN_POINT('Ctrl Pts',(21.1167639345631,10.2823401001072,12.));
#175949=CARTESIAN_POINT('Ctrl Pts',(21.1304249906002,10.2947530860721,12.));
#175950=CARTESIAN_POINT('Ctrl Pts',(21.1441402425843,10.3072855142687,12.));
#175951=CARTESIAN_POINT('Ctrl Pts',(21.1579085619965,10.3199370506544,12.));
#175952=CARTESIAN_POINT('Ctrl Pts',(21.1717288370509,10.3327073641572,12.));
#175953=CARTESIAN_POINT('Ctrl Pts',(21.1855999722416,10.3455961265701,12.));
#175954=CARTESIAN_POINT('Ctrl Pts',(21.199520887919,10.3586030124587,12.));
#175955=CARTESIAN_POINT('Ctrl Pts',(21.2134905199345,10.371727699113,12.));
#175956=CARTESIAN_POINT('Ctrl Pts',(21.22750781927,10.3849698664786,12.));
#175957=CARTESIAN_POINT('Ctrl Pts',(21.2415717516714,10.3983291970846,12.));
#175958=CARTESIAN_POINT('Ctrl Pts',(21.255681297275,10.4118053759588,12.));
#175959=CARTESIAN_POINT('Ctrl Pts',(21.2698354502403,10.42539809054,12.));
#175960=CARTESIAN_POINT('Ctrl Pts',(21.2840332184483,10.4391070306391,12.));
#175961=CARTESIAN_POINT('Ctrl Pts',(21.2982736231931,10.4529318883874,12.));
#175962=CARTESIAN_POINT('Ctrl Pts',(21.3125556988731,10.4668723581768,12.));
#175963=CARTESIAN_POINT('Ctrl Pts',(21.3268784926819,10.4809281365931,12.));
#175964=CARTESIAN_POINT('Ctrl Pts',(21.3412410642904,10.4950989223337,12.));
#175965=CARTESIAN_POINT('Ctrl Pts',(21.3556424855814,10.5093844161685,12.));
#175966=CARTESIAN_POINT('Ctrl Pts',(21.3700818403936,10.5237843209057,12.));
#175967=CARTESIAN_POINT('Ctrl Pts',(21.3845582242602,10.5382983413421,12.));
#175968=CARTESIAN_POINT('Ctrl Pts',(21.3990707441497,10.5529261842108,12.));
#175969=CARTESIAN_POINT('Ctrl Pts',(21.4136185181979,10.5676675581108,12.));
#175970=CARTESIAN_POINT('Ctrl Pts',(21.4282006754631,10.5825221734573,12.));
#175971=CARTESIAN_POINT('Ctrl Pts',(21.4428163557144,10.5974897424622,12.));
#175972=CARTESIAN_POINT('Ctrl Pts',(21.4574647092097,10.6125699790961,12.));
#175973=CARTESIAN_POINT('Ctrl Pts',(21.4721448964766,10.6277625990456,12.));
#175974=CARTESIAN_POINT('Ctrl Pts',(21.4868560880889,10.6430673196607,12.));
#175975=CARTESIAN_POINT('Ctrl Pts',(21.5015974644449,10.6584838598939,12.));
#175976=CARTESIAN_POINT('Ctrl Pts',(21.51636821558,10.6740119402834,12.));
#175977=CARTESIAN_POINT('Ctrl Pts',(21.5311675409807,10.689651282929,12.));
#175978=CARTESIAN_POINT('Ctrl Pts',(21.5459946493955,10.7054016114571,12.));
#175979=CARTESIAN_POINT('Ctrl Pts',(21.5608487586468,10.7212626509816,12.));
#175980=CARTESIAN_POINT('Ctrl Pts',(21.5757290954371,10.7372341280467,12.));
#175981=CARTESIAN_POINT('Ctrl Pts',(21.5906348951743,10.7533157705941,12.));
#175982=CARTESIAN_POINT('Ctrl Pts',(21.6055654018176,10.7695073079552,12.));
#175983=CARTESIAN_POINT('Ctrl Pts',(21.6205198677173,10.7858084708261,12.));
#175984=CARTESIAN_POINT('Ctrl Pts',(21.6354975534557,10.8022189912369,12.));
#175985=CARTESIAN_POINT('Ctrl Pts',(21.6504977276866,10.8187386025136,12.));
#175986=CARTESIAN_POINT('Ctrl Pts',(21.6655196669732,10.8353670392272,12.));
#175987=CARTESIAN_POINT('Ctrl Pts',(21.6805626556467,10.8521040371835,12.));
#175988=CARTESIAN_POINT('Ctrl Pts',(21.6956259856672,10.8689493334095,12.));
#175989=CARTESIAN_POINT('Ctrl Pts',(21.7107089564825,10.8859026661293,12.));
#175990=CARTESIAN_POINT('Ctrl Pts',(21.7258108748873,10.902963774734,12.));
#175991=CARTESIAN_POINT('Ctrl Pts',(21.7409310548797,10.9201323997384,12.));
#175992=CARTESIAN_POINT('Ctrl Pts',(21.7560688175247,10.9374082827444,12.));
#175993=CARTESIAN_POINT('Ctrl Pts',(21.7712234908464,10.9547911664455,12.));
#175994=CARTESIAN_POINT('Ctrl Pts',(21.7863944097141,10.9722807946156,12.));
#175995=CARTESIAN_POINT('Ctrl Pts',(21.8015809157301,10.9898769120912,12.));
#175996=CARTESIAN_POINT('Ctrl Pts',(21.8167823571168,11.0075792647477,12.));
#175997=CARTESIAN_POINT('Ctrl Pts',(21.8319980886033,11.0253875994598,12.));
#175998=CARTESIAN_POINT('Ctrl Pts',(21.8472274713103,11.0433016640807,12.));
#175999=CARTESIAN_POINT('Ctrl Pts',(21.8624698726318,11.0613212074363,12.));
#176000=CARTESIAN_POINT('Ctrl Pts',(21.877724666119,11.0794459793057,12.));
#176001=CARTESIAN_POINT('Ctrl Pts',(21.8929912313608,11.0976757303944,12.));
#176002=CARTESIAN_POINT('Ctrl Pts',(21.9082689538688,11.1160102123024,12.));
#176003=CARTESIAN_POINT('Ctrl Pts',(21.923557224952,11.1344491774741,12.));
#176004=CARTESIAN_POINT('Ctrl Pts',(21.9388554416439,11.1529923792003,12.));
#176005=CARTESIAN_POINT('Ctrl Pts',(21.9541630066506,11.1716395716376,12.));
#176006=CARTESIAN_POINT('Ctrl Pts',(21.9694793282914,11.190390509811,12.));
#176007=CARTESIAN_POINT('Ctrl Pts',(21.9848038204439,11.2092449496125,12.));
#176008=CARTESIAN_POINT('Ctrl Pts',(22.0001359024839,11.2282026477896,12.));
#176009=CARTESIAN_POINT('Ctrl Pts',(22.0154749992363,11.2472633619275,12.));
#176010=CARTESIAN_POINT('Ctrl Pts',(22.030820540835,11.2664268504206,12.));
#176011=CARTESIAN_POINT('Ctrl Pts',(22.046171962566,11.2856928724374,12.));
#176012=CARTESIAN_POINT('Ctrl Pts',(22.0615287047179,11.3050611878771,12.));
#176013=CARTESIAN_POINT('Ctrl Pts',(22.0768902124267,11.3245315573168,12.));
#176014=CARTESIAN_POINT('Ctrl Pts',(22.0922559355294,11.3441037419553,12.));
#176015=CARTESIAN_POINT('Ctrl Pts',(22.1076253283979,11.3637775035367,12.));
#176016=CARTESIAN_POINT('Ctrl Pts',(22.1229978500186,11.3835526044256,12.));
#176017=CARTESIAN_POINT('Ctrl Pts',(22.1383729640964,11.4034288076908,12.));
#176018=CARTESIAN_POINT('Ctrl Pts',(22.1537501391487,11.4234058771742,12.));
#176019=CARTESIAN_POINT('Ctrl Pts',(22.1691288486096,11.443483577557,12.));
#176020=CARTESIAN_POINT('Ctrl Pts',(22.184508570917,11.463661674411,12.));
#176021=CARTESIAN_POINT('Ctrl Pts',(22.1998887896436,11.483939934259,12.));
#176022=CARTESIAN_POINT('Ctrl Pts',(22.2152689931022,11.5043181244242,12.));
#176023=CARTESIAN_POINT('Ctrl Pts',(22.2306486738901,11.5247960128477,12.));
#176024=CARTESIAN_POINT('Ctrl Pts',(22.2460273284654,11.5453733679121,12.));
#176025=CARTESIAN_POINT('Ctrl Pts',(22.2614044566898,11.5660499582403,12.));
#176026=CARTESIAN_POINT('Ctrl Pts',(22.2767795614348,11.5868255525188,12.));
#176027=CARTESIAN_POINT('Ctrl Pts',(22.2921521480356,11.6076999192357,12.));
#176028=CARTESIAN_POINT('Ctrl Pts',(22.3075217249049,11.6286728270009,12.));
#176029=CARTESIAN_POINT('Ctrl Pts',(22.3228878043976,11.6497440449857,12.));
#176030=CARTESIAN_POINT('Ctrl Pts',(22.3382499035619,11.6709133432985,12.));
#176031=CARTESIAN_POINT('Ctrl Pts',(22.3536075450029,11.6921804934056,12.));
#176032=CARTESIAN_POINT('Ctrl Pts',(22.3689602575491,11.7135452684532,12.));
#176033=CARTESIAN_POINT('Ctrl Pts',(22.3843075773899,11.7350074437961,12.));
#176034=CARTESIAN_POINT('Ctrl Pts',(22.3996490469191,11.7565667964764,12.));
#176035=CARTESIAN_POINT('Ctrl Pts',(22.4149842125008,11.7782231042039,12.));
#176036=CARTESIAN_POINT('Ctrl Pts',(22.430312622646,11.7999761445173,12.));
#176037=CARTESIAN_POINT('Ctrl Pts',(22.4456338258735,11.8218256937889,12.));
#176038=CARTESIAN_POINT('Ctrl Pts',(22.4609473690471,11.8437715264487,12.));
#176039=CARTESIAN_POINT('Ctrl Pts',(22.4762527946702,11.8658134137019,12.));
#176040=CARTESIAN_POINT('Ctrl Pts',(22.4915496418485,11.8879511239943,12.));
#176041=CARTESIAN_POINT('Ctrl Pts',(22.5068374513973,11.9101844254557,12.));
#176042=CARTESIAN_POINT('Ctrl Pts',(22.5221157697883,11.9325130877803,12.));
#176043=CARTESIAN_POINT('Ctrl Pts',(22.5373841537307,11.9549368843997,12.));
#176044=CARTESIAN_POINT('Ctrl Pts',(22.5526421741158,11.9774555943496,12.));
#176045=CARTESIAN_POINT('Ctrl Pts',(22.5678894211181,12.0000690046695,12.));
#176046=CARTESIAN_POINT('Ctrl Pts',(22.5831255061282,12.0227769113127,12.));
#176047=CARTESIAN_POINT('Ctrl Pts',(22.5983500505644,12.0455791139128,12.));
#176048=CARTESIAN_POINT('Ctrl Pts',(22.6135626764898,12.0684754113862,12.));
#176049=CARTESIAN_POINT('Ctrl Pts',(22.6287629967056,12.0914655972823,12.));
#176050=CARTESIAN_POINT('Ctrl Pts',(22.6439506046605,12.1145494550383,12.));
#176051=CARTESIAN_POINT('Ctrl Pts',(22.6591250653965,12.1377267537145,12.));
#176052=CARTESIAN_POINT('Ctrl Pts',(22.6742859034944,12.1609972423099,12.));
#176053=CARTESIAN_POINT('Ctrl Pts',(22.6894326205037,12.1843606579262,12.));
#176054=CARTESIAN_POINT('Ctrl Pts',(22.7045647168747,12.2078167360284,12.));
#176055=CARTESIAN_POINT('Ctrl Pts',(22.7196817119374,12.2313652198061,12.));
#176056=CARTESIAN_POINT('Ctrl Pts',(22.7347831655287,12.2550058702395,12.));
#176057=CARTESIAN_POINT('Ctrl Pts',(22.7498686970069,12.2787384750742,12.));
#176058=CARTESIAN_POINT('Ctrl Pts',(22.764938010105,12.3025628601792,12.));
#176059=CARTESIAN_POINT('Ctrl Pts',(22.7799908974768,12.3264788926075,12.));
#176060=CARTESIAN_POINT('Ctrl Pts',(22.795027221673,12.3504864740319,12.));
#176061=CARTESIAN_POINT('Ctrl Pts',(22.81004690224,12.374585536673,12.));
#176062=CARTESIAN_POINT('Ctrl Pts',(22.8220493007173,12.3939379378998,12.));
#176063=CARTESIAN_POINT('Ctrl Pts',(22.8310435872747,12.4084933766347,12.));
#176064=CARTESIAN_POINT('Ctrl Pts',(22.8370364396459,12.418215285186,12.));
#176065=CARTESIAN_POINT('Ctrl Pts',(22.8400320311648,12.4230808101438,12.));
#176066=CARTESIAN_POINT('',(22.1787195904339,13.5685075571671,12.));
#176067=CARTESIAN_POINT('Origin',(0.,0.,12.));
#176068=CARTESIAN_POINT('',(18.5896416359912,12.7689476255363,12.));
#176069=CARTESIAN_POINT('Ctrl Pts',(22.1787195904339,13.5685075571671,12.));
#176070=CARTESIAN_POINT('Ctrl Pts',(22.1730081264608,13.5683460612942,12.));
#176071=CARTESIAN_POINT('Ctrl Pts',(22.1615922805008,13.5680170531805,12.));
#176072=CARTESIAN_POINT('Ctrl Pts',(22.1444897575194,13.5675054919061,12.));
#176073=CARTESIAN_POINT('Ctrl Pts',(22.1217288871975,13.5667873105359,12.));
#176074=CARTESIAN_POINT('Ctrl Pts',(22.0933486464593,13.5658294169284,12.));
#176075=CARTESIAN_POINT('Ctrl Pts',(22.0650393089609,13.5648113689033,12.));
#176076=CARTESIAN_POINT('Ctrl Pts',(22.0368009736295,13.5637332022473,12.));
#176077=CARTESIAN_POINT('Ctrl Pts',(22.0086337943449,13.5625949868333,12.));
#176078=CARTESIAN_POINT('Ctrl Pts',(21.9805379899168,13.5613968357561,12.));
#176079=CARTESIAN_POINT('Ctrl Pts',(21.9525138592813,13.5601389185257,12.));
#176080=CARTESIAN_POINT('Ctrl Pts',(21.9245617765769,13.5588214586604,12.));
#176081=CARTESIAN_POINT('Ctrl Pts',(21.8966821688824,13.5574447178425,12.));
#176082=CARTESIAN_POINT('Ctrl Pts',(21.8688754989365,13.5560089839385,12.));
#176083=CARTESIAN_POINT('Ctrl Pts',(21.8411422456075,13.5545145573031,12.));
#176084=CARTESIAN_POINT('Ctrl Pts',(21.8134828857967,13.5529617381573,12.));
#176085=CARTESIAN_POINT('Ctrl Pts',(21.7858978745865,13.551350812725,12.));
#176086=CARTESIAN_POINT('Ctrl Pts',(21.7583876294554,13.5496820422211,12.));
#176087=CARTESIAN_POINT('Ctrl Pts',(21.7309525412281,13.5479556704481,12.));
#176088=CARTESIAN_POINT('Ctrl Pts',(21.7035929822955,13.5461719295048,12.));
#176089=CARTESIAN_POINT('Ctrl Pts',(21.6763093157699,13.5443310461526,12.));
#176090=CARTESIAN_POINT('Ctrl Pts',(21.6491019044648,13.5424332480699,12.));
#176091=CARTESIAN_POINT('Ctrl Pts',(21.6219711193946,13.5404787697792,12.));
#176092=CARTESIAN_POINT('Ctrl Pts',(21.5949173499013,13.5384678597195,12.));
#176093=CARTESIAN_POINT('Ctrl Pts',(21.5679410019001,13.536400779028,12.));
#176094=CARTESIAN_POINT('Ctrl Pts',(21.5410424932503,13.5342777983215,12.));
#176095=CARTESIAN_POINT('Ctrl Pts',(21.5142222501666,13.5320991952138,12.));
#176096=CARTESIAN_POINT('Ctrl Pts',(21.4874807030468,13.5298652514355,12.));
#176097=CARTESIAN_POINT('Ctrl Pts',(21.4608182828697,13.5275762503555,12.));
#176098=CARTESIAN_POINT('Ctrl Pts',(21.4342354165259,13.5252324737802,12.));
#176099=CARTESIAN_POINT('Ctrl Pts',(21.4077325259324,13.5228342013516,12.));
#176100=CARTESIAN_POINT('Ctrl Pts',(21.3813100304973,13.5203817122504,12.));
#176101=CARTESIAN_POINT('Ctrl Pts',(21.3549683486222,13.5178752862466,12.));
#176102=CARTESIAN_POINT('Ctrl Pts',(21.3287078996341,13.5153152050555,12.));
#176103=CARTESIAN_POINT('Ctrl Pts',(21.3025291054235,13.5127017534971,12.));
#176104=CARTESIAN_POINT('Ctrl Pts',(21.2764323924442,13.5100352209205,12.));
#176105=CARTESIAN_POINT('Ctrl Pts',(21.250418192743,13.5073159019452,12.));
#176106=CARTESIAN_POINT('Ctrl Pts',(21.2244869429332,13.5045440957404,12.));
#176107=CARTESIAN_POINT('Ctrl Pts',(21.1986390835828,13.5017201056088,12.));
#176108=CARTESIAN_POINT('Ctrl Pts',(21.1728750584175,13.4988442384491,12.));
#176109=CARTESIAN_POINT('Ctrl Pts',(21.1471953136209,13.4959168042934,12.));
#176110=CARTESIAN_POINT('Ctrl Pts',(21.1216002970207,13.4929381157778,12.));
#176111=CARTESIAN_POINT('Ctrl Pts',(21.0960904575046,13.4899084877717,12.));
#176112=CARTESIAN_POINT('Ctrl Pts',(21.0706662455199,13.4868282377191,12.));
#176113=CARTESIAN_POINT('Ctrl Pts',(21.0453281134245,13.4836976858912,12.));
#176114=CARTESIAN_POINT('Ctrl Pts',(21.0200765158884,13.4805171556822,12.));
#176115=CARTESIAN_POINT('Ctrl Pts',(20.9949119102592,13.4772869738879,12.));
#176116=CARTESIAN_POINT('Ctrl Pts',(20.9698347569477,13.4740074710086,12.));
#176117=CARTESIAN_POINT('Ctrl Pts',(20.9448455197557,13.4706789815166,12.));
#176118=CARTESIAN_POINT('Ctrl Pts',(20.9199446657583,13.4673018437717,12.));
#176119=CARTESIAN_POINT('Ctrl Pts',(20.8951326652158,13.4638763999725,12.));
#176120=CARTESIAN_POINT('Ctrl Pts',(20.8704099914641,13.4604029960983,12.));
#176121=CARTESIAN_POINT('Ctrl Pts',(20.8457771208083,13.4568819818631,12.));
#176122=CARTESIAN_POINT('Ctrl Pts',(20.821234532398,13.4533137106667,12.));
#176123=CARTESIAN_POINT('Ctrl Pts',(20.7967827081228,13.4496985395637,12.));
#176124=CARTESIAN_POINT('Ctrl Pts',(20.7724221327609,13.4460368293689,12.));
#176125=CARTESIAN_POINT('Ctrl Pts',(20.7481532941014,13.4423289447561,12.));
#176126=CARTESIAN_POINT('Ctrl Pts',(20.7239766830675,13.4385752543663,12.));
#176127=CARTESIAN_POINT('Ctrl Pts',(20.6998927938288,13.4347761309154,12.));
#176128=CARTESIAN_POINT('Ctrl Pts',(20.6759021239102,13.4309319513119,12.));
#176129=CARTESIAN_POINT('Ctrl Pts',(20.6520051742867,13.4270430967651,12.));
#176130=CARTESIAN_POINT('Ctrl Pts',(20.6282024494234,13.4231099528178,12.));
#176131=CARTESIAN_POINT('Ctrl Pts',(20.6044944573151,13.4191329093932,12.));
#176132=CARTESIAN_POINT('Ctrl Pts',(20.5808817095155,13.4151123608411,12.));
#176133=CARTESIAN_POINT('Ctrl Pts',(20.557364721164,13.4110487059912,12.));
#176134=CARTESIAN_POINT('Ctrl Pts',(20.5339440109957,13.4069423482077,12.));
#176135=CARTESIAN_POINT('Ctrl Pts',(20.5106201013755,13.4027936954529,12.));
#176136=CARTESIAN_POINT('Ctrl Pts',(20.4873935184041,13.3986031603716,12.));
#176137=CARTESIAN_POINT('Ctrl Pts',(20.4642647920038,13.3943711603739,12.));
#176138=CARTESIAN_POINT('Ctrl Pts',(20.4412344560007,13.3900981177254,12.));
#176139=CARTESIAN_POINT('Ctrl Pts',(20.4183030482002,13.3857844596387,12.));
#176140=CARTESIAN_POINT('Ctrl Pts',(20.3954711104504,13.3814306183721,12.));
#176141=CARTESIAN_POINT('Ctrl Pts',(20.3727391887187,13.377037031319,12.));
#176142=CARTESIAN_POINT('Ctrl Pts',(20.3501078331818,13.372604141087,12.));
#176143=CARTESIAN_POINT('Ctrl Pts',(20.3275775983032,13.3681323955828,12.));
#176144=CARTESIAN_POINT('Ctrl Pts',(20.3051490429049,13.3636222481017,12.));
#176145=CARTESIAN_POINT('Ctrl Pts',(20.2828227302337,13.3590741574194,12.));
#176146=CARTESIAN_POINT('Ctrl Pts',(20.2605992280117,13.3544885878886,12.));
#176147=CARTESIAN_POINT('Ctrl Pts',(20.2384791085354,13.3498660095382,12.));
#176148=CARTESIAN_POINT('Ctrl Pts',(20.2164629487855,13.3452068981763,12.));
#176149=CARTESIAN_POINT('Ctrl Pts',(20.1945513305233,13.3405117354969,12.));
#176150=CARTESIAN_POINT('Ctrl Pts',(20.1727448403818,13.3357810091903,12.));
#176151=CARTESIAN_POINT('Ctrl Pts',(20.1510440699477,13.3310152130565,12.));
#176152=CARTESIAN_POINT('Ctrl Pts',(20.1294496158405,13.3262148471228,12.));
#176153=CARTESIAN_POINT('Ctrl Pts',(20.1079620798377,13.3213804177588,12.));
#176154=CARTESIAN_POINT('Ctrl Pts',(20.0865820689883,13.3165124377963,12.));
#176155=CARTESIAN_POINT('Ctrl Pts',(20.0653101957188,13.3116114266514,12.));
#176156=CARTESIAN_POINT('Ctrl Pts',(20.0441470779345,13.3066779104515,12.));
#176157=CARTESIAN_POINT('Ctrl Pts',(20.0230933391039,13.3017124221639,12.));
#176158=CARTESIAN_POINT('Ctrl Pts',(20.0021496083742,13.296715501731,12.));
#176159=CARTESIAN_POINT('Ctrl Pts',(19.9813165207174,13.2916876962098,12.));
#176160=CARTESIAN_POINT('Ctrl Pts',(19.9605947170589,13.2866295599152,12.));
#176161=CARTESIAN_POINT('Ctrl Pts',(19.9399848444019,13.2815416545663,12.));
#176162=CARTESIAN_POINT('Ctrl Pts',(19.9194875559419,13.2764245494354,12.));
#176163=CARTESIAN_POINT('Ctrl Pts',(19.8991035111739,13.2712788215015,12.));
#176164=CARTESIAN_POINT('Ctrl Pts',(19.8788333760571,13.2661050556128,12.));
#176165=CARTESIAN_POINT('Ctrl Pts',(19.8586778231711,13.2609038446525,12.));
#176166=CARTESIAN_POINT('Ctrl Pts',(19.8386375318632,13.2556757897085,12.));
#176167=CARTESIAN_POINT('Ctrl Pts',(19.8187131883919,13.2504215002458,12.));
#176168=CARTESIAN_POINT('Ctrl Pts',(19.7989054860501,13.2451415942809,12.));
#176169=CARTESIAN_POINT('Ctrl Pts',(19.7792151253297,13.239836698568,12.));
#176170=CARTESIAN_POINT('Ctrl Pts',(19.7596428141176,13.2345074487968,12.));
#176171=CARTESIAN_POINT('Ctrl Pts',(19.7401892678701,13.2291544897902,12.));
#176172=CARTESIAN_POINT('Ctrl Pts',(19.7208552097867,13.2237784757065,12.));
#176173=CARTESIAN_POINT('Ctrl Pts',(19.7016413709678,13.2183800702431,12.));
#176174=CARTESIAN_POINT('Ctrl Pts',(19.6825484905812,13.2129599468478,12.));
#176175=CARTESIAN_POINT('Ctrl Pts',(19.6635773160924,13.2075187889522,12.));
#176176=CARTESIAN_POINT('Ctrl Pts',(19.6447286034764,13.202057290206,12.));
#176177=CARTESIAN_POINT('Ctrl Pts',(19.6260031174244,13.196576154715,12.));
#176178=CARTESIAN_POINT('Ctrl Pts',(19.6074016315421,13.1910760972818,12.));
#176179=CARTESIAN_POINT('Ctrl Pts',(19.5889249285352,13.185557843648,12.));
#176180=CARTESIAN_POINT('Ctrl Pts',(19.5705738004682,13.1800221307683,12.));
#176181=CARTESIAN_POINT('Ctrl Pts',(19.5523490490254,13.1744697070918,12.));
#176182=CARTESIAN_POINT('Ctrl Pts',(19.5342514857564,13.1689013328432,12.));
#176183=CARTESIAN_POINT('Ctrl Pts',(19.5162819323207,13.1633177803097,12.));
#176184=CARTESIAN_POINT('Ctrl Pts',(19.498441220707,13.1577198341238,12.));
#176185=CARTESIAN_POINT('Ctrl Pts',(19.4807301935256,13.1521082915846,12.));
#176186=CARTESIAN_POINT('Ctrl Pts',(19.463149704325,13.1464839629966,12.));
#176187=CARTESIAN_POINT('Ctrl Pts',(19.4457006178875,13.140847672006,12.));
#176188=CARTESIAN_POINT('Ctrl Pts',(19.4283838105265,13.135200255944,12.));
#176189=CARTESIAN_POINT('Ctrl Pts',(19.4112001703561,13.1295425661635,12.));
#176190=CARTESIAN_POINT('Ctrl Pts',(19.3941505976267,13.1238754684177,12.));
#176191=CARTESIAN_POINT('Ctrl Pts',(19.3772360051093,13.118199843271,12.));
#176192=CARTESIAN_POINT('Ctrl Pts',(19.3604573184516,13.1125165865021,12.));
#176193=CARTESIAN_POINT('Ctrl Pts',(19.3438154765395,13.1068266095186,12.));
#176194=CARTESIAN_POINT('Ctrl Pts',(19.3273114318268,13.1011308397592,12.));
#176195=CARTESIAN_POINT('Ctrl Pts',(19.3109461507358,13.095430221148,12.));
#176196=CARTESIAN_POINT('Ctrl Pts',(19.2947206141246,13.089725714597,12.));
#176197=CARTESIAN_POINT('Ctrl Pts',(19.2786358177198,13.0840182984949,12.));
#176198=CARTESIAN_POINT('Ctrl Pts',(19.2626927725596,13.0783089692118,12.));
#176199=CARTESIAN_POINT('Ctrl Pts',(19.2468925053988,13.0725987415856,12.));
#176200=CARTESIAN_POINT('Ctrl Pts',(19.2312360592031,13.0668886494791,12.));
#176201=CARTESIAN_POINT('Ctrl Pts',(19.2157244937141,13.0611797463913,12.));
#176202=CARTESIAN_POINT('Ctrl Pts',(19.2003588859771,13.0554731060537,12.));
#176203=CARTESIAN_POINT('Ctrl Pts',(19.1851403308825,13.0497698230442,12.));
#176204=CARTESIAN_POINT('Ctrl Pts',(19.1700699416625,13.0440710133775,12.));
#176205=CARTESIAN_POINT('Ctrl Pts',(19.1551488505233,13.0383778152072,12.));
#176206=CARTESIAN_POINT('Ctrl Pts',(19.1403782093389,13.0326913895841,12.));
#176207=CARTESIAN_POINT('Ctrl Pts',(19.1257591903099,13.0270129211976,12.));
#176208=CARTESIAN_POINT('Ctrl Pts',(19.1112929866308,13.0213436191326,12.));
#176209=CARTESIAN_POINT('Ctrl Pts',(19.0969808131226,13.0156847176094,12.));
#176210=CARTESIAN_POINT('Ctrl Pts',(19.0828239070482,13.0100374768786,12.));
#176211=CARTESIAN_POINT('Ctrl Pts',(19.0688235289437,13.0044031841381,12.));
#176212=CARTESIAN_POINT('Ctrl Pts',(19.0549809634355,12.9987831544502,12.));
#176213=CARTESIAN_POINT('Ctrl Pts',(19.0412975200398,12.9931787316515,12.));
#176214=CARTESIAN_POINT('Ctrl Pts',(19.0277745339908,12.9875912893003,12.));
#176215=CARTESIAN_POINT('Ctrl Pts',(19.0144133673348,12.9820222318716,12.));
#176216=CARTESIAN_POINT('Ctrl Pts',(19.0012154099791,12.9764729959205,12.));
#176217=CARTESIAN_POINT('Ctrl Pts',(18.9881820807585,12.9709450512747,12.));
#176218=CARTESIAN_POINT('Ctrl Pts',(18.9753148284475,12.9654399021869,12.));
#176219=CARTESIAN_POINT('Ctrl Pts',(18.9626151329229,12.9599590886319,12.));
#176220=CARTESIAN_POINT('Ctrl Pts',(18.9500845064715,12.9545041877377,12.));
#176221=CARTESIAN_POINT('Ctrl Pts',(18.9377244950435,12.9490768151821,12.));
#176222=CARTESIAN_POINT('Ctrl Pts',(18.9255366795195,12.9436786266105,12.));
#176223=CARTESIAN_POINT('Ctrl Pts',(18.9135226769465,12.9383113190375,12.));
#176224=CARTESIAN_POINT('Ctrl Pts',(18.9016841423403,12.9329766328185,12.));
#176225=CARTESIAN_POINT('Ctrl Pts',(18.8900227704889,12.9276763536373,12.));
#176226=CARTESIAN_POINT('Ctrl Pts',(18.8785402977527,12.9224123144982,12.));
#176227=CARTESIAN_POINT('Ctrl Pts',(18.8672385038326,12.9171863977045,12.));
#176228=CARTESIAN_POINT('Ctrl Pts',(18.8561192136198,12.9120005369063,12.));
#176229=CARTESIAN_POINT('Ctrl Pts',(18.8451842990984,12.9068567191854,12.));
#176230=CARTESIAN_POINT('Ctrl Pts',(18.834435681259,12.9017569871738,12.));
#176231=CARTESIAN_POINT('Ctrl Pts',(18.8238753319129,12.8967034410755,12.));
#176232=CARTESIAN_POINT('Ctrl Pts',(18.813505275782,12.8916982409935,12.));
#176233=CARTESIAN_POINT('Ctrl Pts',(18.8033275941943,12.8867436109546,12.));
#176234=CARTESIAN_POINT('Ctrl Pts',(18.7933444285868,12.8818418427475,12.));
#176235=CARTESIAN_POINT('Ctrl Pts',(18.7835579840477,12.8769952998095,12.));
#176236=CARTESIAN_POINT('Ctrl Pts',(18.7739705329022,12.872206421181,12.));
#176237=CARTESIAN_POINT('Ctrl Pts',(18.7645844169564,12.8674777239653,12.));
#176238=CARTESIAN_POINT('Ctrl Pts',(18.7554020493887,12.8628118054171,12.));
#176239=CARTESIAN_POINT('Ctrl Pts',(18.7464259171251,12.8582113455646,12.));
#176240=CARTESIAN_POINT('Ctrl Pts',(18.7376585820854,12.8536791086316,12.));
#176241=CARTESIAN_POINT('Ctrl Pts',(18.7291026886554,12.8492179511591,12.));
#176242=CARTESIAN_POINT('Ctrl Pts',(18.7207609737702,12.8448308329494,12.));
#176243=CARTESIAN_POINT('Ctrl Pts',(18.7126362754445,12.8405208263431,12.));
#176244=CARTESIAN_POINT('Ctrl Pts',(18.7047315436294,12.8362911280361,12.));
#176245=CARTESIAN_POINT('Ctrl Pts',(18.6970498410172,12.8321450599789,12.));
#176246=CARTESIAN_POINT('Ctrl Pts',(18.6895943376171,12.8280860635231,12.));
#176247=CARTESIAN_POINT('Ctrl Pts',(18.6823683094139,12.8241176980017,12.));
#176248=CARTESIAN_POINT('Ctrl Pts',(18.6753751301092,12.8202436318474,12.));
#176249=CARTESIAN_POINT('Ctrl Pts',(18.6686182952799,12.8164676687362,12.));
#176250=CARTESIAN_POINT('Ctrl Pts',(18.6621014624746,12.8127937909631,12.));
#176251=CARTESIAN_POINT('Ctrl Pts',(18.6558284825773,12.8092261933858,12.));
#176252=CARTESIAN_POINT('Ctrl Pts',(18.6498034438987,12.805769331162,12.));
#176253=CARTESIAN_POINT('Ctrl Pts',(18.6440306327456,12.8024278770153,12.));
#176254=CARTESIAN_POINT('Ctrl Pts',(18.63851447924,12.7992066625264,12.));
#176255=CARTESIAN_POINT('Ctrl Pts',(18.6332595057006,12.7961106222251,12.));
#176256=CARTESIAN_POINT('Ctrl Pts',(18.6282702819371,12.7931447451555,12.));
#176257=CARTESIAN_POINT('Ctrl Pts',(18.6235516265575,12.7903142925234,12.));
#176258=CARTESIAN_POINT('Ctrl Pts',(18.6191087624752,12.7876249657834,12.));
#176259=CARTESIAN_POINT('Ctrl Pts',(18.6149475565188,12.7850831657901,12.));
#176260=CARTESIAN_POINT('Ctrl Pts',(18.6110744826219,12.7826959526925,12.));
#176261=CARTESIAN_POINT('Ctrl Pts',(18.6074961535723,12.7804705387658,12.));
#176262=CARTESIAN_POINT('Ctrl Pts',(18.6042190183704,12.7784139605066,12.));
#176263=CARTESIAN_POINT('Ctrl Pts',(18.6012488486709,12.7765325225081,12.));
#176264=CARTESIAN_POINT('Ctrl Pts',(18.598591752595,12.7748328937638,12.));
#176265=CARTESIAN_POINT('Ctrl Pts',(18.5962551167772,12.7733231262108,12.));
#176266=CARTESIAN_POINT('Ctrl Pts',(18.5942490615407,12.7720142287172,12.));
#176267=CARTESIAN_POINT('Ctrl Pts',(18.5925859134579,12.7709195951156,12.));
#176268=CARTESIAN_POINT('Ctrl Pts',(18.5912775137806,12.7700520897173,12.));
#176269=CARTESIAN_POINT('Ctrl Pts',(18.5903328777227,12.7694215127919,12.));
#176270=CARTESIAN_POINT('Ctrl Pts',(18.589871621843,12.769110348199,12.));
#176271=CARTESIAN_POINT('Ctrl Pts',(18.5896919669165,12.768986426692,12.));
#176272=CARTESIAN_POINT('Ctrl Pts',(18.5896460962964,12.7689524524483,12.));
#176273=CARTESIAN_POINT('Ctrl Pts',(18.5896416359912,12.7689476255363,12.));
#176274=CARTESIAN_POINT('',(18.1294424696716,12.4528436808172,12.));
#176275=CARTESIAN_POINT('',(8.86099361848466,6.08648437878338,12.));
#176276=CARTESIAN_POINT('',(17.4407513054162,12.572596943457,12.));
#176277=CARTESIAN_POINT('Origin',(17.846350172984,12.8649829188862,12.));
#176278=CARTESIAN_POINT('',(16.6581946899465,13.5924445804218,12.));
#176279=CARTESIAN_POINT('Origin',(6.37232247690086E-13,4.50593605254675E-13,
12.));
#176280=CARTESIAN_POINT('',(16.7207683102834,14.2886635873976,12.));
#176281=CARTESIAN_POINT('Origin',(17.0455945664569,13.9085479427572,12.));
#176282=CARTESIAN_POINT('',(17.1452095830633,14.6513681262571,12.));
#176283=CARTESIAN_POINT('',(8.57260479153162,7.32568406312855,12.));
#176284=CARTESIAN_POINT('',(18.8464468996588,17.9112098770111,12.));
#176285=CARTESIAN_POINT('Ctrl Pts',(17.1452095830633,14.6513681262571,12.));
#176286=CARTESIAN_POINT('Ctrl Pts',(17.1452153999142,14.651371185284,12.));
#176287=CARTESIAN_POINT('Ctrl Pts',(17.1452600887039,14.6514066997188,12.));
#176288=CARTESIAN_POINT('Ctrl Pts',(17.1454262858045,14.6515481598057,12.));
#176289=CARTESIAN_POINT('Ctrl Pts',(17.1458462295273,14.65191316345,12.));
#176290=CARTESIAN_POINT('Ctrl Pts',(17.1466998098673,14.6526624064978,12.));
#176291=CARTESIAN_POINT('Ctrl Pts',(17.1478763944909,14.6537016966188,12.));
#176292=CARTESIAN_POINT('Ctrl Pts',(17.1493641837556,14.6550248622813,12.));
#176293=CARTESIAN_POINT('Ctrl Pts',(17.1511476869495,14.6566237952435,12.));
#176294=CARTESIAN_POINT('Ctrl Pts',(17.1532107762719,14.6584900555301,12.));
#176295=CARTESIAN_POINT('Ctrl Pts',(17.1555401986403,14.660616716964,12.));
#176296=CARTESIAN_POINT('Ctrl Pts',(17.1581262646789,14.662998728599,12.));
#176297=CARTESIAN_POINT('Ctrl Pts',(17.1609609517369,14.6656319165057,12.));
#176298=CARTESIAN_POINT('Ctrl Pts',(17.1640366762304,14.6685123374424,12.));
#176299=CARTESIAN_POINT('Ctrl Pts',(17.1673449723019,14.6716355833321,12.));
#176300=CARTESIAN_POINT('Ctrl Pts',(17.1708771619129,14.6749971333867,12.));
#176301=CARTESIAN_POINT('Ctrl Pts',(17.1746247499057,14.6785925615676,12.));
#176302=CARTESIAN_POINT('Ctrl Pts',(17.1785800350827,14.6824178576167,12.));
#176303=CARTESIAN_POINT('Ctrl Pts',(17.182736158472,14.6864694522319,12.));
#176304=CARTESIAN_POINT('Ctrl Pts',(17.1870867909918,14.6907440526958,12.));
#176305=CARTESIAN_POINT('Ctrl Pts',(17.1916259308415,14.6952385361706,12.));
#176306=CARTESIAN_POINT('Ctrl Pts',(17.1963476411694,14.699949811582,12.));
#176307=CARTESIAN_POINT('Ctrl Pts',(17.2012461084268,14.7048748502663,12.));
#176308=CARTESIAN_POINT('Ctrl Pts',(17.2063157097316,14.7100107213587,12.));
#176309=CARTESIAN_POINT('Ctrl Pts',(17.2115510835988,14.7153546289338,12.));
#176310=CARTESIAN_POINT('Ctrl Pts',(17.2169471814255,14.7209039390326,12.));
#176311=CARTESIAN_POINT('Ctrl Pts',(17.2224992099666,14.7266561494282,12.));
#176312=CARTESIAN_POINT('Ctrl Pts',(17.2282025904314,14.7326088681163,12.));
#176313=CARTESIAN_POINT('Ctrl Pts',(17.2340529062077,14.7387597858117,12.));
#176314=CARTESIAN_POINT('Ctrl Pts',(17.2400458713566,14.7451066593793,12.));
#176315=CARTESIAN_POINT('Ctrl Pts',(17.2461773413289,14.7516473175125,12.));
#176316=CARTESIAN_POINT('Ctrl Pts',(17.2524433146837,14.7583796616617,12.));
#176317=CARTESIAN_POINT('Ctrl Pts',(17.2588399401464,14.7653016697589,12.));
#176318=CARTESIAN_POINT('Ctrl Pts',(17.2653635155317,14.7724113956728,12.));
#176319=CARTESIAN_POINT('Ctrl Pts',(17.2720104735192,14.7797069617802,12.));
#176320=CARTESIAN_POINT('Ctrl Pts',(17.278777370485,14.787186553128,12.));
#176321=CARTESIAN_POINT('Ctrl Pts',(17.28566087332,14.7948484105253,12.));
#176322=CARTESIAN_POINT('Ctrl Pts',(17.2926577496519,14.8026908254281,12.));
#176323=CARTESIAN_POINT('Ctrl Pts',(17.2997648661483,14.8107121391038,12.));
#176324=CARTESIAN_POINT('Ctrl Pts',(17.3069791853705,14.8189107410161,12.));
#176325=CARTESIAN_POINT('Ctrl Pts',(17.3142977632656,14.8272850675375,12.));
#176326=CARTESIAN_POINT('Ctrl Pts',(17.3217177462096,14.8358336004193,12.));
#176327=CARTESIAN_POINT('Ctrl Pts',(17.3292363662601,14.8445548643505,12.));
#176328=CARTESIAN_POINT('Ctrl Pts',(17.336850936485,14.8534474245433,12.));
#176329=CARTESIAN_POINT('Ctrl Pts',(17.3445588463477,14.8625098843419,12.));
#176330=CARTESIAN_POINT('Ctrl Pts',(17.3523575568648,14.8717408826958,12.));
#176331=CARTESIAN_POINT('Ctrl Pts',(17.3602445978163,14.8811390927424,12.));
#176332=CARTESIAN_POINT('Ctrl Pts',(17.3682175653236,14.8907032205789,12.));
#176333=CARTESIAN_POINT('Ctrl Pts',(17.3762741193075,14.9004320039609,12.));
#176334=CARTESIAN_POINT('Ctrl Pts',(17.3844119809823,14.9103242110057,12.));
#176335=CARTESIAN_POINT('Ctrl Pts',(17.3926289303987,14.9203786389343,12.));
#176336=CARTESIAN_POINT('Ctrl Pts',(17.400922804075,14.9305941128758,12.));
#176337=CARTESIAN_POINT('Ctrl Pts',(17.4092914926071,14.940969484645,12.));
#176338=CARTESIAN_POINT('Ctrl Pts',(17.4177329382827,14.9515036315142,12.));
#176339=CARTESIAN_POINT('Ctrl Pts',(17.4262451327088,14.9621954549825,12.));
#176340=CARTESIAN_POINT('Ctrl Pts',(17.4348261151395,14.973043879945,12.));
#176341=CARTESIAN_POINT('Ctrl Pts',(17.4434739707773,14.9840478538357,12.));
#176342=CARTESIAN_POINT('Ctrl Pts',(17.4521868291005,14.9952063457779,12.));
#176343=CARTESIAN_POINT('Ctrl Pts',(17.4609628621419,15.0065183456923,12.));
#176344=CARTESIAN_POINT('Ctrl Pts',(17.4698002829357,15.0179828635087,12.));
#176345=CARTESIAN_POINT('Ctrl Pts',(17.4786973441417,15.029598928488,12.));
#176346=CARTESIAN_POINT('Ctrl Pts',(17.4876523366178,15.0413655884993,12.));
#176347=CARTESIAN_POINT('Ctrl Pts',(17.4966635880246,15.0532819093085,12.));
#176348=CARTESIAN_POINT('Ctrl Pts',(17.5057294613877,15.0653469738307,12.));
#176349=CARTESIAN_POINT('Ctrl Pts',(17.5148483539687,15.0775598815749,12.));
#176350=CARTESIAN_POINT('Ctrl Pts',(17.524018696179,15.0899197481082,12.));
#176351=CARTESIAN_POINT('Ctrl Pts',(17.5332389504829,15.1024257045033,12.));
#176352=CARTESIAN_POINT('Ctrl Pts',(17.5425076102963,15.1150768967728,12.));
#176353=CARTESIAN_POINT('Ctrl Pts',(17.5518231989117,15.1278724853138,12.));
#176354=CARTESIAN_POINT('Ctrl Pts',(17.5611842686192,15.1408116444876,12.));
#176355=CARTESIAN_POINT('Ctrl Pts',(17.5705893998029,15.1538935621714,12.));
#176356=CARTESIAN_POINT('Ctrl Pts',(17.580037200054,15.1671174393137,12.));
#176357=CARTESIAN_POINT('Ctrl Pts',(17.5895263032595,15.1804824894605,12.));
#176358=CARTESIAN_POINT('Ctrl Pts',(17.5990553687599,15.1939879383268,12.));
#176359=CARTESIAN_POINT('Ctrl Pts',(17.60862308065,15.2076330234686,12.));
#176360=CARTESIAN_POINT('Ctrl Pts',(17.6182281470468,15.22141699392,12.));
#176361=CARTESIAN_POINT('Ctrl Pts',(17.6278692993764,15.2353391098367,12.));
#176362=CARTESIAN_POINT('Ctrl Pts',(17.6375452916369,15.2493986421092,12.));
#176363=CARTESIAN_POINT('Ctrl Pts',(17.6472548997328,15.2635948720292,12.));
#176364=CARTESIAN_POINT('Ctrl Pts',(17.6569969209,15.2779270910239,12.));
#176365=CARTESIAN_POINT('Ctrl Pts',(17.6667701731041,15.2923946003598,12.));
#176366=CARTESIAN_POINT('Ctrl Pts',(17.676573494456,15.3069967108501,12.));
#176367=CARTESIAN_POINT('Ctrl Pts',(17.6864057426052,15.3217327425338,12.));
#176368=CARTESIAN_POINT('Ctrl Pts',(17.6962657941983,15.3366020244066,12.));
#176369=CARTESIAN_POINT('Ctrl Pts',(17.7061525444042,15.351603894206,12.));
#176370=CARTESIAN_POINT('Ctrl Pts',(17.7160649064206,15.3667376981699,12.));
#176371=CARTESIAN_POINT('Ctrl Pts',(17.7260018109924,15.3820027907967,12.));
#176372=CARTESIAN_POINT('Ctrl Pts',(17.7359622059149,15.3973985345802,12.));
#176373=CARTESIAN_POINT('Ctrl Pts',(17.7459450555812,15.4129242997837,12.));
#176374=CARTESIAN_POINT('Ctrl Pts',(17.7559493405881,15.4285794642668,12.));
#176375=CARTESIAN_POINT('Ctrl Pts',(17.7659740573265,15.4443634132869,12.));
#176376=CARTESIAN_POINT('Ctrl Pts',(17.7760182175815,15.4602755393018,12.));
#176377=CARTESIAN_POINT('Ctrl Pts',(17.7860808481219,15.4763152417497,12.));
#176378=CARTESIAN_POINT('Ctrl Pts',(17.7961609903148,15.4924819268517,12.));
#176379=CARTESIAN_POINT('Ctrl Pts',(17.8062576997952,15.5087750074718,12.));
#176380=CARTESIAN_POINT('Ctrl Pts',(17.8163700461256,15.5251939029552,12.));
#176381=CARTESIAN_POINT('Ctrl Pts',(17.8264971124606,15.541738038964,12.));
#176382=CARTESIAN_POINT('Ctrl Pts',(17.8366379952085,15.5584068472982,12.));
#176383=CARTESIAN_POINT('Ctrl Pts',(17.8467918036987,15.5751997657163,12.));
#176384=CARTESIAN_POINT('Ctrl Pts',(17.8569576599006,15.5921162378192,12.));
#176385=CARTESIAN_POINT('Ctrl Pts',(17.8671346981394,15.609155712921,12.));
#176386=CARTESIAN_POINT('Ctrl Pts',(17.8773220648125,15.6263176459108,12.));
#176387=CARTESIAN_POINT('Ctrl Pts',(17.8875189181091,15.6436014971085,12.));
#176388=CARTESIAN_POINT('Ctrl Pts',(17.897724427724,15.661006732103,12.));
#176389=CARTESIAN_POINT('Ctrl Pts',(17.9079377746111,15.6785328216461,12.));
#176390=CARTESIAN_POINT('Ctrl Pts',(17.9181581507455,15.6961792415522,12.));
#176391=CARTESIAN_POINT('Ctrl Pts',(17.9283847588836,15.7139454725839,12.));
#176392=CARTESIAN_POINT('Ctrl Pts',(17.9386168123262,15.7318310003335,12.));
#176393=CARTESIAN_POINT('Ctrl Pts',(17.9488535346781,15.749835315086,12.));
#176394=CARTESIAN_POINT('Ctrl Pts',(17.9590941596242,15.7679579117077,12.));
#176395=CARTESIAN_POINT('Ctrl Pts',(17.9693379307303,15.7861982895724,12.));
#176396=CARTESIAN_POINT('Ctrl Pts',(17.9795841012386,15.8045559524677,12.));
#176397=CARTESIAN_POINT('Ctrl Pts',(17.9898319338664,15.8230304084962,12.));
#176398=CARTESIAN_POINT('Ctrl Pts',(18.0000807006052,15.8416211699679,12.));
#176399=CARTESIAN_POINT('Ctrl Pts',(18.0103296825205,15.8603277532831,12.));
#176400=CARTESIAN_POINT('Ctrl Pts',(18.0205781695769,15.8791496788683,12.));
#176401=CARTESIAN_POINT('Ctrl Pts',(18.0308254604636,15.8980864711042,12.));
#176402=CARTESIAN_POINT('Ctrl Pts',(18.0410708624208,15.9171376582436,12.));
#176403=CARTESIAN_POINT('Ctrl Pts',(18.0513136910691,15.9363027723244,12.));
#176404=CARTESIAN_POINT('Ctrl Pts',(18.061553270236,15.9555813490644,12.));
#176405=CARTESIAN_POINT('Ctrl Pts',(18.0717889317958,15.9749729277846,12.));
#176406=CARTESIAN_POINT('Ctrl Pts',(18.0820200155236,15.9944770513613,12.));
#176407=CARTESIAN_POINT('Ctrl Pts',(18.0922458689462,16.014093266161,12.));
#176408=CARTESIAN_POINT('Ctrl Pts',(18.1024658471966,16.0338211219693,12.));
#176409=CARTESIAN_POINT('Ctrl Pts',(18.112679312869,16.0536601719126,12.));
#176410=CARTESIAN_POINT('Ctrl Pts',(18.1228856358751,16.0736099723668,12.));
#176411=CARTESIAN_POINT('Ctrl Pts',(18.1330841933105,16.0936700829112,12.));
#176412=CARTESIAN_POINT('Ctrl Pts',(18.1432743693235,16.1138400662794,12.));
#176413=CARTESIAN_POINT('Ctrl Pts',(18.1534555549852,16.1341194882988,12.));
#176414=CARTESIAN_POINT('Ctrl Pts',(18.1636271481615,16.154507917826,12.));
#176415=CARTESIAN_POINT('Ctrl Pts',(18.1737885533849,16.1750049266671,12.));
#176416=CARTESIAN_POINT('Ctrl Pts',(18.1839391817331,16.1956100895073,12.));
#176417=CARTESIAN_POINT('Ctrl Pts',(18.1940784507229,16.2163229838875,12.));
#176418=CARTESIAN_POINT('Ctrl Pts',(18.2042057842035,16.2371431901638,12.));
#176419=CARTESIAN_POINT('Ctrl Pts',(18.2143206122529,16.2580702914615,12.));
#176420=CARTESIAN_POINT('Ctrl Pts',(18.2244223710745,16.2791038736223,12.));
#176421=CARTESIAN_POINT('Ctrl Pts',(18.2345105028982,16.3002435251378,12.));
#176422=CARTESIAN_POINT('Ctrl Pts',(18.2445844558742,16.3214888370987,12.));
#176423=CARTESIAN_POINT('Ctrl Pts',(18.2546436839608,16.3428394031589,12.));
#176424=CARTESIAN_POINT('Ctrl Pts',(18.2646876468169,16.3642948194868,12.));
#176425=CARTESIAN_POINT('Ctrl Pts',(18.2747158096934,16.385854684708,12.));
#176426=CARTESIAN_POINT('Ctrl Pts',(18.2847276433309,16.4075185998455,12.));
#176427=CARTESIAN_POINT('Ctrl Pts',(18.294722623851,16.4292861682379,12.));
#176428=CARTESIAN_POINT('Ctrl Pts',(18.304700232686,16.4511569955233,12.));
#176429=CARTESIAN_POINT('Ctrl Pts',(18.3146599565231,16.4731306896441,12.));
#176430=CARTESIAN_POINT('Ctrl Pts',(18.3246012872469,16.4952068608345,12.));
#176431=CARTESIAN_POINT('Ctrl Pts',(18.3345237218864,16.5173851216045,12.));
#176432=CARTESIAN_POINT('Ctrl Pts',(18.34442676256,16.5396650867139,12.));
#176433=CARTESIAN_POINT('Ctrl Pts',(18.354309916433,16.5620463731413,12.));
#176434=CARTESIAN_POINT('Ctrl Pts',(18.3641726955889,16.5845286000217,12.));
#176435=CARTESIAN_POINT('Ctrl Pts',(18.3740146168879,16.607111388571,12.));
#176436=CARTESIAN_POINT('Ctrl Pts',(18.3838352018327,16.6297943620056,12.));
#176437=CARTESIAN_POINT('Ctrl Pts',(18.3936339764332,16.6525771454513,12.));
#176438=CARTESIAN_POINT('Ctrl Pts',(18.403410471079,16.6754593658513,12.));
#176439=CARTESIAN_POINT('Ctrl Pts',(18.413164220399,16.6984406518491,12.));
#176440=CARTESIAN_POINT('Ctrl Pts',(18.4228947633187,16.7215206338818,12.));
#176441=CARTESIAN_POINT('Ctrl Pts',(18.4326016431392,16.7446989442882,12.));
#176442=CARTESIAN_POINT('Ctrl Pts',(18.44228440761,16.7679752173992,12.));
#176443=CARTESIAN_POINT('Ctrl Pts',(18.4519426090123,16.791349089629,12.));
#176444=CARTESIAN_POINT('Ctrl Pts',(18.4615758042305,16.8148201995472,12.));
#176445=CARTESIAN_POINT('Ctrl Pts',(18.4711835548623,16.8383881879709,12.));
#176446=CARTESIAN_POINT('Ctrl Pts',(18.4807654268771,16.8620526977171,12.));
#176447=CARTESIAN_POINT('Ctrl Pts',(18.4903209902227,16.8858133733088,12.));
#176448=CARTESIAN_POINT('Ctrl Pts',(18.499849818462,16.9096698606943,12.));
#176449=CARTESIAN_POINT('Ctrl Pts',(18.5093514883835,16.9336218069353,12.));
#176450=CARTESIAN_POINT('Ctrl Pts',(18.5188255796659,16.9576688599339,12.));
#176451=CARTESIAN_POINT('Ctrl Pts',(18.5282716744197,16.981810668038,12.));
#176452=CARTESIAN_POINT('Ctrl Pts',(18.5376893576961,17.0060468805097,12.));
#176453=CARTESIAN_POINT('Ctrl Pts',(18.547078218209,17.0303771481738,12.));
#176454=CARTESIAN_POINT('Ctrl Pts',(18.556437848963,17.0548011239751,12.));
#176455=CARTESIAN_POINT('Ctrl Pts',(18.5657678479789,17.0793184636079,12.));
#176456=CARTESIAN_POINT('Ctrl Pts',(18.5750678188542,17.1039288260001,12.));
#176457=CARTESIAN_POINT('Ctrl Pts',(18.5843373717247,17.1286318741183,12.));
#176458=CARTESIAN_POINT('Ctrl Pts',(18.5935761222825,17.1534272741643,12.));
#176459=CARTESIAN_POINT('Ctrl Pts',(18.6027836898817,17.1783146940127,12.));
#176460=CARTESIAN_POINT('Ctrl Pts',(18.6119596959949,17.2032938019284,12.));
#176461=CARTESIAN_POINT('Ctrl Pts',(18.6211037624038,17.2283642650518,12.));
#176462=CARTESIAN_POINT('Ctrl Pts',(18.6302155097943,17.2535257482187,12.));
#176463=CARTESIAN_POINT('Ctrl Pts',(18.6392945554748,17.2787779120213,12.));
#176464=CARTESIAN_POINT('Ctrl Pts',(18.6483405141865,17.3041204135074,12.));
#176465=CARTESIAN_POINT('Ctrl Pts',(18.6573530024033,17.3295529098618,12.));
#176466=CARTESIAN_POINT('Ctrl Pts',(18.6663316416582,17.3550750612443,12.));
#176467=CARTESIAN_POINT('Ctrl Pts',(18.6752760624052,17.3806865340747,12.));
#176468=CARTESIAN_POINT('Ctrl Pts',(18.6841859073471,17.4063870038562,12.));
#176469=CARTESIAN_POINT('Ctrl Pts',(18.6930608357409,17.4321761588142,12.));
#176470=CARTESIAN_POINT('Ctrl Pts',(18.70190052503,17.4580537012753,12.));
#176471=CARTESIAN_POINT('Ctrl Pts',(18.7107046613912,17.4840193397162,12.));
#176472=CARTESIAN_POINT('Ctrl Pts',(18.7194729318098,17.5100727820876,12.));
#176473=CARTESIAN_POINT('Ctrl Pts',(18.7282050157138,17.5362137287593,12.));
#176474=CARTESIAN_POINT('Ctrl Pts',(18.7369005764553,17.5624418653245,12.));
#176475=CARTESIAN_POINT('Ctrl Pts',(18.7455592536687,17.5887568561371,12.));
#176476=CARTESIAN_POINT('Ctrl Pts',(18.7541806530984,17.6151583357012,12.));
#176477=CARTESIAN_POINT('Ctrl Pts',(18.762764361321,17.6416459210681,12.));
#176478=CARTESIAN_POINT('Ctrl Pts',(18.7713099642754,17.6682192274236,12.));
#176479=CARTESIAN_POINT('Ctrl Pts',(18.7798170641374,17.6948778823014,12.));
#176480=CARTESIAN_POINT('Ctrl Pts',(18.7882852976049,17.7216215409035,12.));
#176481=CARTESIAN_POINT('Ctrl Pts',(18.7967143519419,17.7484498996905,12.));
#176482=CARTESIAN_POINT('Ctrl Pts',(18.8051039860448,17.7753627137853,12.));
#176483=CARTESIAN_POINT('Ctrl Pts',(18.8134540340417,17.8023598011057,12.));
#176484=CARTESIAN_POINT('Ctrl Pts',(18.8217643886157,17.8294410311006,12.));
#176485=CARTESIAN_POINT('Ctrl Pts',(18.8300349895974,17.8566063174771,12.));
#176486=CARTESIAN_POINT('Ctrl Pts',(18.8366196462581,17.8784057509356,12.));
#176487=CARTESIAN_POINT('Ctrl Pts',(18.8415402351786,17.8947931177807,12.));
#176488=CARTESIAN_POINT('Ctrl Pts',(18.8448126709691,17.9057348246595,12.));
#176489=CARTESIAN_POINT('Ctrl Pts',(18.8464468996588,17.9112098770111,12.));
#176490=CARTESIAN_POINT('',(17.9112098770111,18.8464468996588,12.));
#176491=CARTESIAN_POINT('Origin',(0.,0.,12.));
#176492=CARTESIAN_POINT('',(14.6513681262571,17.1452095830633,12.));
#176493=CARTESIAN_POINT('Ctrl Pts',(17.9112098770111,18.8464468996588,12.));
#176494=CARTESIAN_POINT('Ctrl Pts',(17.9057348246611,18.8448126709726,12.));
#176495=CARTESIAN_POINT('Ctrl Pts',(17.8947931177853,18.8415402351882,12.));
#176496=CARTESIAN_POINT('Ctrl Pts',(17.8784057509434,18.8366196462746,12.));
#176497=CARTESIAN_POINT('Ctrl Pts',(17.8566063174871,18.8300349896187,12.));
#176498=CARTESIAN_POINT('Ctrl Pts',(17.8294410311105,18.8217643886368,12.));
#176499=CARTESIAN_POINT('Ctrl Pts',(17.8023598011135,18.8134540340581,12.));
#176500=CARTESIAN_POINT('Ctrl Pts',(17.7753627137898,18.8051039860543,12.));
#176501=CARTESIAN_POINT('Ctrl Pts',(17.7484498996916,18.7967143519444,12.));
#176502=CARTESIAN_POINT('Ctrl Pts',(17.7216215409019,18.7882852976016,12.));
#176503=CARTESIAN_POINT('Ctrl Pts',(17.6948778822981,18.7798170641305,12.));
#176504=CARTESIAN_POINT('Ctrl Pts',(17.6682192274197,18.7713099642673,12.));
#176505=CARTESIAN_POINT('Ctrl Pts',(17.6416459210646,18.7627643613139,12.));
#176506=CARTESIAN_POINT('Ctrl Pts',(17.6151583356988,18.7541806530935,12.));
#176507=CARTESIAN_POINT('Ctrl Pts',(17.5887568561361,18.7455592536667,12.));
#176508=CARTESIAN_POINT('Ctrl Pts',(17.5624418653248,18.7369005764558,12.));
#176509=CARTESIAN_POINT('Ctrl Pts',(17.5362137287604,18.728205015716,12.));
#176510=CARTESIAN_POINT('Ctrl Pts',(17.5100727820891,18.7194729318128,12.));
#176511=CARTESIAN_POINT('Ctrl Pts',(17.4840193397176,18.7107046613941,12.));
#176512=CARTESIAN_POINT('Ctrl Pts',(17.4580537012764,18.7019005250322,12.));
#176513=CARTESIAN_POINT('Ctrl Pts',(17.4321761588148,18.6930608357421,12.));
#176514=CARTESIAN_POINT('Ctrl Pts',(17.4063870038563,18.6841859073472,12.));
#176515=CARTESIAN_POINT('Ctrl Pts',(17.3806865340744,18.6752760624045,12.));
#176516=CARTESIAN_POINT('Ctrl Pts',(17.3550750612438,18.6663316416569,12.));
#176517=CARTESIAN_POINT('Ctrl Pts',(17.3295529098612,18.6573530024019,12.));
#176518=CARTESIAN_POINT('Ctrl Pts',(17.3041204135069,18.6483405141853,12.));
#176519=CARTESIAN_POINT('Ctrl Pts',(17.278777912021,18.639294555474,12.));
#176520=CARTESIAN_POINT('Ctrl Pts',(17.2535257482186,18.630215509794,12.));
#176521=CARTESIAN_POINT('Ctrl Pts',(17.2283642650519,18.6211037624041,12.));
#176522=CARTESIAN_POINT('Ctrl Pts',(17.2032938019288,18.6119596959957,12.));
#176523=CARTESIAN_POINT('Ctrl Pts',(17.1783146940131,18.6027836898826,12.));
#176524=CARTESIAN_POINT('Ctrl Pts',(17.1534272741646,18.5935761222833,12.));
#176525=CARTESIAN_POINT('Ctrl Pts',(17.1286318741185,18.5843373717253,12.));
#176526=CARTESIAN_POINT('Ctrl Pts',(17.1039288260001,18.5750678188543,12.));
#176527=CARTESIAN_POINT('Ctrl Pts',(17.0793184636079,18.5657678479788,12.));
#176528=CARTESIAN_POINT('Ctrl Pts',(17.0548011239751,18.5564378489628,12.));
#176529=CARTESIAN_POINT('Ctrl Pts',(17.030377148174,18.5470782182089,12.));
#176530=CARTESIAN_POINT('Ctrl Pts',(17.0060468805099,18.5376893576961,12.));
#176531=CARTESIAN_POINT('Ctrl Pts',(16.9818106680382,18.5282716744198,12.));
#176532=CARTESIAN_POINT('Ctrl Pts',(16.957668859934,18.518825579666,12.));
#176533=CARTESIAN_POINT('Ctrl Pts',(16.9336218069353,18.5093514883835,12.));
#176534=CARTESIAN_POINT('Ctrl Pts',(16.9096698606942,18.4998498184619,12.));
#176535=CARTESIAN_POINT('Ctrl Pts',(16.8858133733086,18.4903209902226,12.));
#176536=CARTESIAN_POINT('Ctrl Pts',(16.8620526977169,18.4807654268769,12.));
#176537=CARTESIAN_POINT('Ctrl Pts',(16.8383881879707,18.4711835548622,12.));
#176538=CARTESIAN_POINT('Ctrl Pts',(16.8148201995472,18.4615758042305,12.));
#176539=CARTESIAN_POINT('Ctrl Pts',(16.791349089629,18.4519426090124,12.));
#176540=CARTESIAN_POINT('Ctrl Pts',(16.7679752173992,18.4422844076099,12.));
#176541=CARTESIAN_POINT('Ctrl Pts',(16.7446989442882,18.4326016431392,12.));
#176542=CARTESIAN_POINT('Ctrl Pts',(16.7215206338818,18.4228947633186,12.));
#176543=CARTESIAN_POINT('Ctrl Pts',(16.698440651849,18.413164220399,12.));
#176544=CARTESIAN_POINT('Ctrl Pts',(16.6754593658513,18.4034104710789,12.));
#176545=CARTESIAN_POINT('Ctrl Pts',(16.6525771454513,18.3936339764332,12.));
#176546=CARTESIAN_POINT('Ctrl Pts',(16.6297943620056,18.3838352018327,12.));
#176547=CARTESIAN_POINT('Ctrl Pts',(16.6071113885711,18.3740146168879,12.));
#176548=CARTESIAN_POINT('Ctrl Pts',(16.5845286000218,18.364172695589,12.));
#176549=CARTESIAN_POINT('Ctrl Pts',(16.5620463731414,18.3543099164331,12.));
#176550=CARTESIAN_POINT('Ctrl Pts',(16.5396650867139,18.3444267625601,12.));
#176551=CARTESIAN_POINT('Ctrl Pts',(16.5173851216045,18.3345237218864,12.));
#176552=CARTESIAN_POINT('Ctrl Pts',(16.4952068608344,18.3246012872468,12.));
#176553=CARTESIAN_POINT('Ctrl Pts',(16.4731306896439,18.3146599565229,12.));
#176554=CARTESIAN_POINT('Ctrl Pts',(16.4511569955231,18.3047002326858,12.));
#176555=CARTESIAN_POINT('Ctrl Pts',(16.4292861682377,18.2947226238509,12.));
#176556=CARTESIAN_POINT('Ctrl Pts',(16.4075185998454,18.2847276433308,12.));
#176557=CARTESIAN_POINT('Ctrl Pts',(16.385854684708,18.2747158096934,12.));
#176558=CARTESIAN_POINT('Ctrl Pts',(16.3642948194869,18.2646876468169,12.));
#176559=CARTESIAN_POINT('Ctrl Pts',(16.342839403159,18.2546436839609,12.));
#176560=CARTESIAN_POINT('Ctrl Pts',(16.3214888370988,18.2445844558742,12.));
#176561=CARTESIAN_POINT('Ctrl Pts',(16.3002435251378,18.2345105028981,12.));
#176562=CARTESIAN_POINT('Ctrl Pts',(16.2791038736223,18.2244223710745,12.));
#176563=CARTESIAN_POINT('Ctrl Pts',(16.2580702914615,18.214320612253,12.));
#176564=CARTESIAN_POINT('Ctrl Pts',(16.237143190164,18.2042057842037,12.));
#176565=CARTESIAN_POINT('Ctrl Pts',(16.2163229838878,18.1940784507232,12.));
#176566=CARTESIAN_POINT('Ctrl Pts',(16.1956100895076,18.1839391817335,12.));
#176567=CARTESIAN_POINT('Ctrl Pts',(16.1750049266673,18.1737885533852,12.));
#176568=CARTESIAN_POINT('Ctrl Pts',(16.1545079178261,18.1636271481616,12.));
#176569=CARTESIAN_POINT('Ctrl Pts',(16.1341194882987,18.1534555549851,12.));
#176570=CARTESIAN_POINT('Ctrl Pts',(16.113840066279,18.1432743693231,12.));
#176571=CARTESIAN_POINT('Ctrl Pts',(16.0936700829108,18.1330841933099,12.));
#176572=CARTESIAN_POINT('Ctrl Pts',(16.0736099723664,18.1228856358746,12.));
#176573=CARTESIAN_POINT('Ctrl Pts',(16.0536601719124,18.1126793128688,12.));
#176574=CARTESIAN_POINT('Ctrl Pts',(16.0338211219693,18.1024658471966,12.));
#176575=CARTESIAN_POINT('Ctrl Pts',(16.0140932661612,18.0922458689464,12.));
#176576=CARTESIAN_POINT('Ctrl Pts',(15.9944770513616,18.0820200155239,12.));
#176577=CARTESIAN_POINT('Ctrl Pts',(15.9749729277848,18.071788931796,12.));
#176578=CARTESIAN_POINT('Ctrl Pts',(15.9555813490645,18.061553270236,12.));
#176579=CARTESIAN_POINT('Ctrl Pts',(15.9363027723244,18.0513136910691,12.));
#176580=CARTESIAN_POINT('Ctrl Pts',(15.9171376582436,18.0410708624208,12.));
#176581=CARTESIAN_POINT('Ctrl Pts',(15.8980864711043,18.0308254604638,12.));
#176582=CARTESIAN_POINT('Ctrl Pts',(15.8791496788685,18.0205781695773,12.));
#176583=CARTESIAN_POINT('Ctrl Pts',(15.8603277532834,18.010329682521,12.));
#176584=CARTESIAN_POINT('Ctrl Pts',(15.8416211699681,18.0000807006055,12.));
#176585=CARTESIAN_POINT('Ctrl Pts',(15.8230304084963,17.9898319338664,12.));
#176586=CARTESIAN_POINT('Ctrl Pts',(15.8045559524674,17.9795841012383,12.));
#176587=CARTESIAN_POINT('Ctrl Pts',(15.786198289572,17.9693379307297,12.));
#176588=CARTESIAN_POINT('Ctrl Pts',(15.7679579117072,17.9590941596236,12.));
#176589=CARTESIAN_POINT('Ctrl Pts',(15.7498353150856,17.9488535346776,12.));
#176590=CARTESIAN_POINT('Ctrl Pts',(15.7318310003334,17.9386168123261,12.));
#176591=CARTESIAN_POINT('Ctrl Pts',(15.713945472584,17.9283847588837,12.));
#176592=CARTESIAN_POINT('Ctrl Pts',(15.6961792415526,17.918158150746,12.));
#176593=CARTESIAN_POINT('Ctrl Pts',(15.6785328216467,17.9079377746118,12.));
#176594=CARTESIAN_POINT('Ctrl Pts',(15.6610067321036,17.8977244277247,12.));
#176595=CARTESIAN_POINT('Ctrl Pts',(15.6436014971088,17.8875189181095,12.));
#176596=CARTESIAN_POINT('Ctrl Pts',(15.6263176459107,17.8773220648125,12.));
#176597=CARTESIAN_POINT('Ctrl Pts',(15.6091557129205,17.8671346981388,12.));
#176598=CARTESIAN_POINT('Ctrl Pts',(15.5921162378183,17.8569576598996,12.));
#176599=CARTESIAN_POINT('Ctrl Pts',(15.5751997657153,17.8467918036977,12.));
#176600=CARTESIAN_POINT('Ctrl Pts',(15.5584068472976,17.8366379952078,12.));
#176601=CARTESIAN_POINT('Ctrl Pts',(15.5417380389639,17.8264971124606,12.));
#176602=CARTESIAN_POINT('Ctrl Pts',(15.5251939029558,17.8163700461263,12.));
#176603=CARTESIAN_POINT('Ctrl Pts',(15.5087750074728,17.8062576997964,12.));
#176604=CARTESIAN_POINT('Ctrl Pts',(15.4924819268529,17.7961609903161,12.));
#176605=CARTESIAN_POINT('Ctrl Pts',(15.4763152417506,17.7860808481229,12.));
#176606=CARTESIAN_POINT('Ctrl Pts',(15.4602755393019,17.7760182175817,12.));
#176607=CARTESIAN_POINT('Ctrl Pts',(15.4443634132865,17.765974057326,12.));
#176608=CARTESIAN_POINT('Ctrl Pts',(15.4285794642658,17.7559493405871,12.));
#176609=CARTESIAN_POINT('Ctrl Pts',(15.4129242997828,17.7459450555803,12.));
#176610=CARTESIAN_POINT('Ctrl Pts',(15.3973985345796,17.7359622059143,12.));
#176611=CARTESIAN_POINT('Ctrl Pts',(15.3820027907965,17.7260018109923,12.));
#176612=CARTESIAN_POINT('Ctrl Pts',(15.3667376981702,17.7160649064208,12.));
#176613=CARTESIAN_POINT('Ctrl Pts',(15.3516038942064,17.7061525444044,12.));
#176614=CARTESIAN_POINT('Ctrl Pts',(15.3366020244069,17.6962657941984,12.));
#176615=CARTESIAN_POINT('Ctrl Pts',(15.3217327425341,17.6864057426052,12.));
#176616=CARTESIAN_POINT('Ctrl Pts',(15.3069967108501,17.6765734944559,12.));
#176617=CARTESIAN_POINT('Ctrl Pts',(15.2923946003598,17.6667701731041,12.));
#176618=CARTESIAN_POINT('Ctrl Pts',(15.2779270910238,17.6569969209,12.));
#176619=CARTESIAN_POINT('Ctrl Pts',(15.263594872029,17.6472548997329,12.));
#176620=CARTESIAN_POINT('Ctrl Pts',(15.2493986421091,17.637545291637,12.));
#176621=CARTESIAN_POINT('Ctrl Pts',(15.2353391098367,17.6278692993765,12.));
#176622=CARTESIAN_POINT('Ctrl Pts',(15.22141699392,17.6182281470467,12.));
#176623=CARTESIAN_POINT('Ctrl Pts',(15.2076330234686,17.6086230806497,12.));
#176624=CARTESIAN_POINT('Ctrl Pts',(15.1939879383268,17.5990553687595,12.));
#176625=CARTESIAN_POINT('Ctrl Pts',(15.1804824894605,17.5895263032592,12.));
#176626=CARTESIAN_POINT('Ctrl Pts',(15.1671174393136,17.5800372000539,12.));
#176627=CARTESIAN_POINT('Ctrl Pts',(15.1538935621714,17.570589399803,12.));
#176628=CARTESIAN_POINT('Ctrl Pts',(15.1408116444877,17.5611842686196,12.));
#176629=CARTESIAN_POINT('Ctrl Pts',(15.127872485314,17.5518231989122,12.));
#176630=CARTESIAN_POINT('Ctrl Pts',(15.1150768967729,17.5425076102966,12.));
#176631=CARTESIAN_POINT('Ctrl Pts',(15.1024257045033,17.5332389504829,12.));
#176632=CARTESIAN_POINT('Ctrl Pts',(15.0899197481082,17.5240186961788,12.));
#176633=CARTESIAN_POINT('Ctrl Pts',(15.0775598815748,17.5148483539684,12.));
#176634=CARTESIAN_POINT('Ctrl Pts',(15.0653469738306,17.5057294613874,12.));
#176635=CARTESIAN_POINT('Ctrl Pts',(15.0532819093085,17.4966635880245,12.));
#176636=CARTESIAN_POINT('Ctrl Pts',(15.0413655884993,17.4876523366178,12.));
#176637=CARTESIAN_POINT('Ctrl Pts',(15.029598928488,17.4786973441417,12.));
#176638=CARTESIAN_POINT('Ctrl Pts',(15.0179828635086,17.4698002829357,12.));
#176639=CARTESIAN_POINT('Ctrl Pts',(15.0065183456921,17.4609628621418,12.));
#176640=CARTESIAN_POINT('Ctrl Pts',(14.9952063457778,17.4521868291004,12.));
#176641=CARTESIAN_POINT('Ctrl Pts',(14.9840478538358,17.4434739707773,12.));
#176642=CARTESIAN_POINT('Ctrl Pts',(14.9730438799452,17.4348261151396,12.));
#176643=CARTESIAN_POINT('Ctrl Pts',(14.9621954549827,17.426245132709,12.));
#176644=CARTESIAN_POINT('Ctrl Pts',(14.9515036315143,17.4177329382828,12.));
#176645=CARTESIAN_POINT('Ctrl Pts',(14.940969484645,17.4092914926071,12.));
#176646=CARTESIAN_POINT('Ctrl Pts',(14.9305941128757,17.4009228040749,12.));
#176647=CARTESIAN_POINT('Ctrl Pts',(14.9203786389342,17.3926289303986,12.));
#176648=CARTESIAN_POINT('Ctrl Pts',(14.9103242110057,17.3844119809824,12.));
#176649=CARTESIAN_POINT('Ctrl Pts',(14.900432003961,17.3762741193076,12.));
#176650=CARTESIAN_POINT('Ctrl Pts',(14.8907032205788,17.3682175653235,12.));
#176651=CARTESIAN_POINT('Ctrl Pts',(14.8811390927423,17.3602445978161,12.));
#176652=CARTESIAN_POINT('Ctrl Pts',(14.8717408826955,17.3523575568645,12.));
#176653=CARTESIAN_POINT('Ctrl Pts',(14.8625098843417,17.3445588463475,12.));
#176654=CARTESIAN_POINT('Ctrl Pts',(14.8534474245433,17.336850936485,12.));
#176655=CARTESIAN_POINT('Ctrl Pts',(14.8445548643508,17.3292363662605,12.));
#176656=CARTESIAN_POINT('Ctrl Pts',(14.8358336004197,17.3217177462101,12.));
#176657=CARTESIAN_POINT('Ctrl Pts',(14.8272850675379,17.3142977632659,12.));
#176658=CARTESIAN_POINT('Ctrl Pts',(14.8189107410162,17.3069791853706,12.));
#176659=CARTESIAN_POINT('Ctrl Pts',(14.8107121391035,17.299764866148,12.));
#176660=CARTESIAN_POINT('Ctrl Pts',(14.8026908254276,17.2926577496513,12.));
#176661=CARTESIAN_POINT('Ctrl Pts',(14.7948484105249,17.2856608733196,12.));
#176662=CARTESIAN_POINT('Ctrl Pts',(14.787186553128,17.2787773704849,12.));
#176663=CARTESIAN_POINT('Ctrl Pts',(14.7797069617804,17.2720104735194,12.));
#176664=CARTESIAN_POINT('Ctrl Pts',(14.7724113956731,17.2653635155319,12.));
#176665=CARTESIAN_POINT('Ctrl Pts',(14.7653016697591,17.2588399401465,12.));
#176666=CARTESIAN_POINT('Ctrl Pts',(14.7583796616617,17.2524433146837,12.));
#176667=CARTESIAN_POINT('Ctrl Pts',(14.7516473175124,17.2461773413288,12.));
#176668=CARTESIAN_POINT('Ctrl Pts',(14.7451066593792,17.2400458713565,12.));
#176669=CARTESIAN_POINT('Ctrl Pts',(14.7387597858116,17.2340529062076,12.));
#176670=CARTESIAN_POINT('Ctrl Pts',(14.7326088681163,17.2282025904314,12.));
#176671=CARTESIAN_POINT('Ctrl Pts',(14.7266561494282,17.2224992099667,12.));
#176672=CARTESIAN_POINT('Ctrl Pts',(14.7209039390327,17.2169471814256,12.));
#176673=CARTESIAN_POINT('Ctrl Pts',(14.7153546289339,17.2115510835989,12.));
#176674=CARTESIAN_POINT('Ctrl Pts',(14.7100107213586,17.2063157097315,12.));
#176675=CARTESIAN_POINT('Ctrl Pts',(14.7048748502663,17.2012461084268,12.));
#176676=CARTESIAN_POINT('Ctrl Pts',(14.699949811582,17.1963476411694,12.));
#176677=CARTESIAN_POINT('Ctrl Pts',(14.6952385361705,17.1916259308415,12.));
#176678=CARTESIAN_POINT('Ctrl Pts',(14.6907440526958,17.1870867909918,12.));
#176679=CARTESIAN_POINT('Ctrl Pts',(14.686469452232,17.182736158472,12.));
#176680=CARTESIAN_POINT('Ctrl Pts',(14.6824178576167,17.1785800350826,12.));
#176681=CARTESIAN_POINT('Ctrl Pts',(14.6785925615677,17.1746247499057,12.));
#176682=CARTESIAN_POINT('Ctrl Pts',(14.6749971333867,17.1708771619129,12.));
#176683=CARTESIAN_POINT('Ctrl Pts',(14.671635583332,17.167344972302,12.));
#176684=CARTESIAN_POINT('Ctrl Pts',(14.6685123374423,17.1640366762305,12.));
#176685=CARTESIAN_POINT('Ctrl Pts',(14.6656319165057,17.1609609517369,12.));
#176686=CARTESIAN_POINT('Ctrl Pts',(14.6629987285992,17.1581262646789,12.));
#176687=CARTESIAN_POINT('Ctrl Pts',(14.6606167169642,17.1555401986401,12.));
#176688=CARTESIAN_POINT('Ctrl Pts',(14.6584900555302,17.1532107762718,12.));
#176689=CARTESIAN_POINT('Ctrl Pts',(14.6566237952435,17.1511476869496,12.));
#176690=CARTESIAN_POINT('Ctrl Pts',(14.655024862281,17.1493641837558,12.));
#176691=CARTESIAN_POINT('Ctrl Pts',(14.6537016966184,17.147876394491,12.));
#176692=CARTESIAN_POINT('Ctrl Pts',(14.6526624064978,17.1466998098673,12.));
#176693=CARTESIAN_POINT('Ctrl Pts',(14.6519131634508,17.1458462295271,12.));
#176694=CARTESIAN_POINT('Ctrl Pts',(14.6515481598068,17.1454262858043,12.));
#176695=CARTESIAN_POINT('Ctrl Pts',(14.6514066997196,17.1452600887037,12.));
#176696=CARTESIAN_POINT('Ctrl Pts',(14.6513711852843,17.1452153999142,12.));
#176697=CARTESIAN_POINT('Ctrl Pts',(14.6513681262571,17.1452095830633,12.));
#176698=CARTESIAN_POINT('',(14.2886635873976,16.7207683102834,12.));
#176699=CARTESIAN_POINT('',(6.98376450772883,8.17248635976757,12.));
#176700=CARTESIAN_POINT('',(13.5924445804218,16.6581946899465,12.));
#176701=CARTESIAN_POINT('Origin',(13.9085479427572,17.0455945664569,12.));
#176702=CARTESIAN_POINT('',(12.572596943457,17.4407513054162,12.));
#176703=CARTESIAN_POINT('Origin',(4.9889687874677E-13,6.00167842331873E-13,
12.));
#176704=CARTESIAN_POINT('',(12.4528436808172,18.1294424696716,12.));
#176705=CARTESIAN_POINT('Origin',(12.8649829188862,17.846350172984,12.));
#176706=CARTESIAN_POINT('',(12.7689476255363,18.5896416359912,12.));
#176707=CARTESIAN_POINT('',(6.38447381276812,9.29482081799561,12.));
#176708=CARTESIAN_POINT('',(13.5685075571671,22.1787195904339,12.));
#176709=CARTESIAN_POINT('Ctrl Pts',(12.7689476255363,18.5896416359912,12.));
#176710=CARTESIAN_POINT('Ctrl Pts',(12.7689524524484,18.5896460962961,12.));
#176711=CARTESIAN_POINT('Ctrl Pts',(12.7689864266924,18.5896919669158,12.));
#176712=CARTESIAN_POINT('Ctrl Pts',(12.7691103481996,18.589871621842,12.));
#176713=CARTESIAN_POINT('Ctrl Pts',(12.7694215127923,18.590332877722,12.));
#176714=CARTESIAN_POINT('Ctrl Pts',(12.7700520897174,18.5912775137806,12.));
#176715=CARTESIAN_POINT('Ctrl Pts',(12.7709195951153,18.5925859134582,12.));
#176716=CARTESIAN_POINT('Ctrl Pts',(12.7720142287169,18.5942490615409,12.));
#176717=CARTESIAN_POINT('Ctrl Pts',(12.7733231262107,18.5962551167772,12.));
#176718=CARTESIAN_POINT('Ctrl Pts',(12.7748328937639,18.5985917525949,12.));
#176719=CARTESIAN_POINT('Ctrl Pts',(12.7765325225082,18.6012488486708,12.));
#176720=CARTESIAN_POINT('Ctrl Pts',(12.7784139605067,18.6042190183703,12.));
#176721=CARTESIAN_POINT('Ctrl Pts',(12.7804705387658,18.6074961535723,12.));
#176722=CARTESIAN_POINT('Ctrl Pts',(12.7826959526924,18.611074482622,12.));
#176723=CARTESIAN_POINT('Ctrl Pts',(12.78508316579,18.6149475565189,12.));
#176724=CARTESIAN_POINT('Ctrl Pts',(12.7876249657834,18.6191087624752,12.));
#176725=CARTESIAN_POINT('Ctrl Pts',(12.7903142925234,18.6235516265575,12.));
#176726=CARTESIAN_POINT('Ctrl Pts',(12.7931447451556,18.6282702819371,12.));
#176727=CARTESIAN_POINT('Ctrl Pts',(12.7961106222251,18.6332595057005,12.));
#176728=CARTESIAN_POINT('Ctrl Pts',(12.7992066625264,18.63851447924,12.));
#176729=CARTESIAN_POINT('Ctrl Pts',(12.8024278770153,18.6440306327457,12.));
#176730=CARTESIAN_POINT('Ctrl Pts',(12.805769331162,18.6498034438986,12.));
#176731=CARTESIAN_POINT('Ctrl Pts',(12.8092261933858,18.6558284825772,12.));
#176732=CARTESIAN_POINT('Ctrl Pts',(12.8127937909632,18.6621014624746,12.));
#176733=CARTESIAN_POINT('Ctrl Pts',(12.8164676687361,18.6686182952798,12.));
#176734=CARTESIAN_POINT('Ctrl Pts',(12.8202436318473,18.6753751301091,12.));
#176735=CARTESIAN_POINT('Ctrl Pts',(12.8241176980016,18.6823683094139,12.));
#176736=CARTESIAN_POINT('Ctrl Pts',(12.8280860635231,18.6895943376172,12.));
#176737=CARTESIAN_POINT('Ctrl Pts',(12.832145059979,18.6970498410173,12.));
#176738=CARTESIAN_POINT('Ctrl Pts',(12.8362911280362,18.7047315436296,12.));
#176739=CARTESIAN_POINT('Ctrl Pts',(12.8405208263432,18.7126362754446,12.));
#176740=CARTESIAN_POINT('Ctrl Pts',(12.8448308329494,18.7207609737701,12.));
#176741=CARTESIAN_POINT('Ctrl Pts',(12.849217951159,18.7291026886552,12.));
#176742=CARTESIAN_POINT('Ctrl Pts',(12.8536791086315,18.7376585820851,12.));
#176743=CARTESIAN_POINT('Ctrl Pts',(12.8582113455644,18.7464259171248,12.));
#176744=CARTESIAN_POINT('Ctrl Pts',(12.8628118054172,18.7554020493888,12.));
#176745=CARTESIAN_POINT('Ctrl Pts',(12.8674777239656,18.7645844169568,12.));
#176746=CARTESIAN_POINT('Ctrl Pts',(12.8722064211814,18.7739705329029,12.));
#176747=CARTESIAN_POINT('Ctrl Pts',(12.8769952998097,18.7835579840481,12.));
#176748=CARTESIAN_POINT('Ctrl Pts',(12.8818418427474,18.7933444285867,12.));
#176749=CARTESIAN_POINT('Ctrl Pts',(12.8867436109543,18.8033275941939,12.));
#176750=CARTESIAN_POINT('Ctrl Pts',(12.8916982409931,18.8135052757815,12.));
#176751=CARTESIAN_POINT('Ctrl Pts',(12.8967034410752,18.8238753319124,12.));
#176752=CARTESIAN_POINT('Ctrl Pts',(12.9017569871738,18.834435681259,12.));
#176753=CARTESIAN_POINT('Ctrl Pts',(12.9068567191856,18.8451842990986,12.));
#176754=CARTESIAN_POINT('Ctrl Pts',(12.9120005369066,18.8561192136201,12.));
#176755=CARTESIAN_POINT('Ctrl Pts',(12.9171863977047,18.8672385038328,12.));
#176756=CARTESIAN_POINT('Ctrl Pts',(12.9224123144982,18.8785402977528,12.));
#176757=CARTESIAN_POINT('Ctrl Pts',(12.9276763536372,18.8900227704888,12.));
#176758=CARTESIAN_POINT('Ctrl Pts',(12.9329766328184,18.9016841423402,12.));
#176759=CARTESIAN_POINT('Ctrl Pts',(12.9383113190375,18.9135226769466,12.));
#176760=CARTESIAN_POINT('Ctrl Pts',(12.9436786266106,18.9255366795196,12.));
#176761=CARTESIAN_POINT('Ctrl Pts',(12.9490768151821,18.9377244950435,12.));
#176762=CARTESIAN_POINT('Ctrl Pts',(12.9545041877377,18.9500845064714,12.));
#176763=CARTESIAN_POINT('Ctrl Pts',(12.9599590886317,18.9626151329226,12.));
#176764=CARTESIAN_POINT('Ctrl Pts',(12.9654399021868,18.9753148284473,12.));
#176765=CARTESIAN_POINT('Ctrl Pts',(12.9709450512747,18.9881820807585,12.));
#176766=CARTESIAN_POINT('Ctrl Pts',(12.9764729959206,19.0012154099792,12.));
#176767=CARTESIAN_POINT('Ctrl Pts',(12.9820222318716,19.014413367335,12.));
#176768=CARTESIAN_POINT('Ctrl Pts',(12.9875912893003,19.0277745339909,12.));
#176769=CARTESIAN_POINT('Ctrl Pts',(12.9931787316514,19.0412975200398,12.));
#176770=CARTESIAN_POINT('Ctrl Pts',(12.9987831544502,19.0549809634354,12.));
#176771=CARTESIAN_POINT('Ctrl Pts',(13.0044031841382,19.0688235289437,12.));
#176772=CARTESIAN_POINT('Ctrl Pts',(13.0100374768788,19.0828239070484,12.));
#176773=CARTESIAN_POINT('Ctrl Pts',(13.0156847176096,19.0969808131228,12.));
#176774=CARTESIAN_POINT('Ctrl Pts',(13.0213436191328,19.111292986631,12.));
#176775=CARTESIAN_POINT('Ctrl Pts',(13.0270129211976,19.1257591903099,12.));
#176776=CARTESIAN_POINT('Ctrl Pts',(13.0326913895838,19.1403782093386,12.));
#176777=CARTESIAN_POINT('Ctrl Pts',(13.0383778152068,19.155148850523,12.));
#176778=CARTESIAN_POINT('Ctrl Pts',(13.0440710133772,19.1700699416622,12.));
#176779=CARTESIAN_POINT('Ctrl Pts',(13.0497698230441,19.1851403308825,12.));
#176780=CARTESIAN_POINT('Ctrl Pts',(13.0554731060538,19.2003588859772,12.));
#176781=CARTESIAN_POINT('Ctrl Pts',(13.0611797463915,19.2157244937142,12.));
#176782=CARTESIAN_POINT('Ctrl Pts',(13.0668886494795,19.2312360592033,12.));
#176783=CARTESIAN_POINT('Ctrl Pts',(13.0725987415859,19.2468925053989,12.));
#176784=CARTESIAN_POINT('Ctrl Pts',(13.0783089692118,19.2626927725596,12.));
#176785=CARTESIAN_POINT('Ctrl Pts',(13.0840182984949,19.2786358177198,12.));
#176786=CARTESIAN_POINT('Ctrl Pts',(13.0897257145968,19.2947206141247,12.));
#176787=CARTESIAN_POINT('Ctrl Pts',(13.0954302211479,19.310946150736,12.));
#176788=CARTESIAN_POINT('Ctrl Pts',(13.1011308397591,19.3273114318269,12.));
#176789=CARTESIAN_POINT('Ctrl Pts',(13.1068266095186,19.3438154765395,12.));
#176790=CARTESIAN_POINT('Ctrl Pts',(13.1125165865022,19.3604573184515,12.));
#176791=CARTESIAN_POINT('Ctrl Pts',(13.118199843271,19.3772360051091,12.));
#176792=CARTESIAN_POINT('Ctrl Pts',(13.1238754684177,19.3941505976263,12.));
#176793=CARTESIAN_POINT('Ctrl Pts',(13.1295425661634,19.4112001703557,12.));
#176794=CARTESIAN_POINT('Ctrl Pts',(13.1352002559438,19.4283838105262,12.));
#176795=CARTESIAN_POINT('Ctrl Pts',(13.1408476720061,19.4457006178876,12.));
#176796=CARTESIAN_POINT('Ctrl Pts',(13.1464839629971,19.4631497043258,12.));
#176797=CARTESIAN_POINT('Ctrl Pts',(13.1521082915853,19.4807301935268,12.));
#176798=CARTESIAN_POINT('Ctrl Pts',(13.1577198341245,19.4984412207082,12.));
#176799=CARTESIAN_POINT('Ctrl Pts',(13.1633177803101,19.5162819323213,12.));
#176800=CARTESIAN_POINT('Ctrl Pts',(13.168901332843,19.5342514857562,12.));
#176801=CARTESIAN_POINT('Ctrl Pts',(13.1744697070911,19.5523490490244,12.));
#176802=CARTESIAN_POINT('Ctrl Pts',(13.1800221307673,19.5705738004667,12.));
#176803=CARTESIAN_POINT('Ctrl Pts',(13.1855578436471,19.5889249285338,12.));
#176804=CARTESIAN_POINT('Ctrl Pts',(13.1910760972814,19.6074016315414,12.));
#176805=CARTESIAN_POINT('Ctrl Pts',(13.1965761547151,19.6260031174244,12.));
#176806=CARTESIAN_POINT('Ctrl Pts',(13.2020572902065,19.6447286034772,12.));
#176807=CARTESIAN_POINT('Ctrl Pts',(13.2075187889529,19.6635773160936,12.));
#176808=CARTESIAN_POINT('Ctrl Pts',(13.2129599468485,19.6825484905823,12.));
#176809=CARTESIAN_POINT('Ctrl Pts',(13.2183800702436,19.7016413709685,12.));
#176810=CARTESIAN_POINT('Ctrl Pts',(13.2237784757065,19.7208552097868,12.));
#176811=CARTESIAN_POINT('Ctrl Pts',(13.2291544897899,19.7401892678697,12.));
#176812=CARTESIAN_POINT('Ctrl Pts',(13.2345074487963,19.7596428141168,12.));
#176813=CARTESIAN_POINT('Ctrl Pts',(13.2398366985675,19.7792151253289,12.));
#176814=CARTESIAN_POINT('Ctrl Pts',(13.2451415942805,19.7989054860495,12.));
#176815=CARTESIAN_POINT('Ctrl Pts',(13.2504215002457,19.8187131883917,12.));
#176816=CARTESIAN_POINT('Ctrl Pts',(13.2556757897086,19.8386375318634,12.));
#176817=CARTESIAN_POINT('Ctrl Pts',(13.2609038446529,19.8586778231715,12.));
#176818=CARTESIAN_POINT('Ctrl Pts',(13.2661050556132,19.8788333760577,12.));
#176819=CARTESIAN_POINT('Ctrl Pts',(13.271278821502,19.8991035111745,12.));
#176820=CARTESIAN_POINT('Ctrl Pts',(13.2764245494357,19.9194875559422,12.));
#176821=CARTESIAN_POINT('Ctrl Pts',(13.2815416545663,19.9399848444019,12.));
#176822=CARTESIAN_POINT('Ctrl Pts',(13.286629559915,19.9605947170586,12.));
#176823=CARTESIAN_POINT('Ctrl Pts',(13.2916876962094,19.981316520717,12.));
#176824=CARTESIAN_POINT('Ctrl Pts',(13.2967155017306,20.0021496083738,12.));
#176825=CARTESIAN_POINT('Ctrl Pts',(13.3017124221637,20.0230933391038,12.));
#176826=CARTESIAN_POINT('Ctrl Pts',(13.3066779104515,20.0441470779345,12.));
#176827=CARTESIAN_POINT('Ctrl Pts',(13.3116114266515,20.0653101957188,12.));
#176828=CARTESIAN_POINT('Ctrl Pts',(13.3165124377962,20.0865820689883,12.));
#176829=CARTESIAN_POINT('Ctrl Pts',(13.3213804177587,20.1079620798375,12.));
#176830=CARTESIAN_POINT('Ctrl Pts',(13.3262148471226,20.1294496158402,12.));
#176831=CARTESIAN_POINT('Ctrl Pts',(13.3310152130564,20.1510440699474,12.));
#176832=CARTESIAN_POINT('Ctrl Pts',(13.3357810091903,20.1727448403817,12.));
#176833=CARTESIAN_POINT('Ctrl Pts',(13.3405117354971,20.1945513305235,12.));
#176834=CARTESIAN_POINT('Ctrl Pts',(13.3452068981766,20.216462948786,12.));
#176835=CARTESIAN_POINT('Ctrl Pts',(13.3498660095386,20.2384791085359,12.));
#176836=CARTESIAN_POINT('Ctrl Pts',(13.3544885878889,20.2605992280122,12.));
#176837=CARTESIAN_POINT('Ctrl Pts',(13.3590741574195,20.2828227302339,12.));
#176838=CARTESIAN_POINT('Ctrl Pts',(13.3636222481016,20.3051490429048,12.));
#176839=CARTESIAN_POINT('Ctrl Pts',(13.3681323955826,20.3275775983029,12.));
#176840=CARTESIAN_POINT('Ctrl Pts',(13.3726041410867,20.3501078331814,12.));
#176841=CARTESIAN_POINT('Ctrl Pts',(13.3770370313188,20.3727391887184,12.));
#176842=CARTESIAN_POINT('Ctrl Pts',(13.3814306183719,20.3954711104502,12.));
#176843=CARTESIAN_POINT('Ctrl Pts',(13.3857844596387,20.4183030482002,12.));
#176844=CARTESIAN_POINT('Ctrl Pts',(13.3900981177255,20.4412344560008,12.));
#176845=CARTESIAN_POINT('Ctrl Pts',(13.3943711603739,20.4642647920038,12.));
#176846=CARTESIAN_POINT('Ctrl Pts',(13.3986031603716,20.487393518404,12.));
#176847=CARTESIAN_POINT('Ctrl Pts',(13.4027936954529,20.5106201013753,12.));
#176848=CARTESIAN_POINT('Ctrl Pts',(13.4069423482076,20.5339440109956,12.));
#176849=CARTESIAN_POINT('Ctrl Pts',(13.4110487059912,20.5573647211639,12.));
#176850=CARTESIAN_POINT('Ctrl Pts',(13.4151123608411,20.5808817095155,12.));
#176851=CARTESIAN_POINT('Ctrl Pts',(13.4191329093932,20.6044944573153,12.));
#176852=CARTESIAN_POINT('Ctrl Pts',(13.4231099528179,20.6282024494237,12.));
#176853=CARTESIAN_POINT('Ctrl Pts',(13.4270430967651,20.6520051742869,12.));
#176854=CARTESIAN_POINT('Ctrl Pts',(13.4309319513119,20.6759021239103,12.));
#176855=CARTESIAN_POINT('Ctrl Pts',(13.4347761309154,20.6998927938288,12.));
#176856=CARTESIAN_POINT('Ctrl Pts',(13.4385752543663,20.7239766830675,12.));
#176857=CARTESIAN_POINT('Ctrl Pts',(13.4423289447561,20.7481532941013,12.));
#176858=CARTESIAN_POINT('Ctrl Pts',(13.4460368293688,20.7724221327608,12.));
#176859=CARTESIAN_POINT('Ctrl Pts',(13.4496985395637,20.7967827081227,12.));
#176860=CARTESIAN_POINT('Ctrl Pts',(13.4533137106667,20.821234532398,12.));
#176861=CARTESIAN_POINT('Ctrl Pts',(13.4568819818631,20.8457771208082,12.));
#176862=CARTESIAN_POINT('Ctrl Pts',(13.4604029960983,20.8704099914641,12.));
#176863=CARTESIAN_POINT('Ctrl Pts',(13.4638763999725,20.8951326652158,12.));
#176864=CARTESIAN_POINT('Ctrl Pts',(13.4673018437718,20.9199446657584,12.));
#176865=CARTESIAN_POINT('Ctrl Pts',(13.4706789815166,20.9448455197557,12.));
#176866=CARTESIAN_POINT('Ctrl Pts',(13.4740074710087,20.9698347569476,12.));
#176867=CARTESIAN_POINT('Ctrl Pts',(13.4772869738879,20.9949119102592,12.));
#176868=CARTESIAN_POINT('Ctrl Pts',(13.4805171556822,21.0200765158885,12.));
#176869=CARTESIAN_POINT('Ctrl Pts',(13.4836976858912,21.0453281134247,12.));
#176870=CARTESIAN_POINT('Ctrl Pts',(13.4868282377191,21.0706662455202,12.));
#176871=CARTESIAN_POINT('Ctrl Pts',(13.4899084877718,21.0960904575048,12.));
#176872=CARTESIAN_POINT('Ctrl Pts',(13.4929381157778,21.1216002970209,12.));
#176873=CARTESIAN_POINT('Ctrl Pts',(13.4959168042934,21.1471953136209,12.));
#176874=CARTESIAN_POINT('Ctrl Pts',(13.4988442384491,21.1728750584173,12.));
#176875=CARTESIAN_POINT('Ctrl Pts',(13.5017201056088,21.1986390835825,12.));
#176876=CARTESIAN_POINT('Ctrl Pts',(13.5045440957404,21.224486942933,12.));
#176877=CARTESIAN_POINT('Ctrl Pts',(13.5073159019454,21.2504181927429,12.));
#176878=CARTESIAN_POINT('Ctrl Pts',(13.5100352209207,21.2764323924442,12.));
#176879=CARTESIAN_POINT('Ctrl Pts',(13.5127017534972,21.3025291054236,12.));
#176880=CARTESIAN_POINT('Ctrl Pts',(13.5153152050554,21.328707899634,12.));
#176881=CARTESIAN_POINT('Ctrl Pts',(13.5178752862461,21.3549683486219,12.));
#176882=CARTESIAN_POINT('Ctrl Pts',(13.5203817122496,21.3813100304967,12.));
#176883=CARTESIAN_POINT('Ctrl Pts',(13.5228342013508,21.4077325259318,12.));
#176884=CARTESIAN_POINT('Ctrl Pts',(13.5252324737795,21.4342354165254,12.));
#176885=CARTESIAN_POINT('Ctrl Pts',(13.5275762503553,21.4608182828695,12.));
#176886=CARTESIAN_POINT('Ctrl Pts',(13.5298652514357,21.487480703047,12.));
#176887=CARTESIAN_POINT('Ctrl Pts',(13.5320991952145,21.5142222501671,12.));
#176888=CARTESIAN_POINT('Ctrl Pts',(13.5342777983225,21.5410424932511,12.));
#176889=CARTESIAN_POINT('Ctrl Pts',(13.5364007790292,21.5679410019011,12.));
#176890=CARTESIAN_POINT('Ctrl Pts',(13.5384678597206,21.5949173499022,12.));
#176891=CARTESIAN_POINT('Ctrl Pts',(13.5404787697798,21.6219711193951,12.));
#176892=CARTESIAN_POINT('Ctrl Pts',(13.5424332480698,21.6491019044647,12.));
#176893=CARTESIAN_POINT('Ctrl Pts',(13.5443310461516,21.676309315769,12.));
#176894=CARTESIAN_POINT('Ctrl Pts',(13.546171929503,21.7035929822939,12.));
#176895=CARTESIAN_POINT('Ctrl Pts',(13.5479556704457,21.730952541226,12.));
#176896=CARTESIAN_POINT('Ctrl Pts',(13.5496820422186,21.7583876294532,12.));
#176897=CARTESIAN_POINT('Ctrl Pts',(13.5513508127232,21.7858978745848,12.));
#176898=CARTESIAN_POINT('Ctrl Pts',(13.5529617381569,21.8134828857963,12.));
#176899=CARTESIAN_POINT('Ctrl Pts',(13.5545145573048,21.841142245609,12.));
#176900=CARTESIAN_POINT('Ctrl Pts',(13.5560089839426,21.8688754989401,12.));
#176901=CARTESIAN_POINT('Ctrl Pts',(13.5574447178484,21.8966821688876,12.));
#176902=CARTESIAN_POINT('Ctrl Pts',(13.5588214586672,21.9245617765827,12.));
#176903=CARTESIAN_POINT('Ctrl Pts',(13.5601389185315,21.9525138592862,12.));
#176904=CARTESIAN_POINT('Ctrl Pts',(13.5613968357589,21.9805379899192,12.));
#176905=CARTESIAN_POINT('Ctrl Pts',(13.5625949868313,22.0086337943431,12.));
#176906=CARTESIAN_POINT('Ctrl Pts',(13.5637332022393,22.0368009736227,12.));
#176907=CARTESIAN_POINT('Ctrl Pts',(13.5648113688894,22.0650393089492,12.));
#176908=CARTESIAN_POINT('Ctrl Pts',(13.5658294169106,22.0933486464442,12.));
#176909=CARTESIAN_POINT('Ctrl Pts',(13.5667873105179,22.1217288871823,12.));
#176910=CARTESIAN_POINT('Ctrl Pts',(13.5675054918922,22.1444897575076,12.));
#176911=CARTESIAN_POINT('Ctrl Pts',(13.5680170531724,22.1615922804939,12.));
#176912=CARTESIAN_POINT('Ctrl Pts',(13.5683460612913,22.1730081264583,12.));
#176913=CARTESIAN_POINT('Ctrl Pts',(13.5685075571671,22.1787195904339,12.));
#176914=CARTESIAN_POINT('',(12.4230808101438,22.8400320311648,12.));
#176915=CARTESIAN_POINT('Origin',(0.,0.,12.));
#176916=CARTESIAN_POINT('',(9.71462809124917,20.353053841303,12.));
#176917=CARTESIAN_POINT('Ctrl Pts',(12.4230808101438,22.8400320311648,12.));
#176918=CARTESIAN_POINT('Ctrl Pts',(12.4182152851867,22.8370364396497,12.));
#176919=CARTESIAN_POINT('Ctrl Pts',(12.4084933766366,22.8310435872852,12.));
#176920=CARTESIAN_POINT('Ctrl Pts',(12.393937937903,22.8220493007353,12.));
#176921=CARTESIAN_POINT('Ctrl Pts',(12.3745855366772,22.8100469022632,12.));
#176922=CARTESIAN_POINT('Ctrl Pts',(12.3504864740361,22.7950272216959,12.));
#176923=CARTESIAN_POINT('Ctrl Pts',(12.3264788926108,22.7799908974947,12.));
#176924=CARTESIAN_POINT('Ctrl Pts',(12.3025628601811,22.7649380101154,12.));
#176925=CARTESIAN_POINT('Ctrl Pts',(12.2787384750747,22.7498686970096,12.));
#176926=CARTESIAN_POINT('Ctrl Pts',(12.2550058702389,22.7347831655251,12.));
#176927=CARTESIAN_POINT('Ctrl Pts',(12.2313652198047,22.7196817119299,12.));
#176928=CARTESIAN_POINT('Ctrl Pts',(12.2078167360267,22.7045647168659,12.));
#176929=CARTESIAN_POINT('Ctrl Pts',(12.1843606579246,22.6894326204959,12.));
#176930=CARTESIAN_POINT('Ctrl Pts',(12.1609972423088,22.6742859034891,12.));
#176931=CARTESIAN_POINT('Ctrl Pts',(12.1377267537141,22.6591250653942,12.));
#176932=CARTESIAN_POINT('Ctrl Pts',(12.1145494550384,22.6439506046611,12.));
#176933=CARTESIAN_POINT('Ctrl Pts',(12.0914655972828,22.628762996708,12.));
#176934=CARTESIAN_POINT('Ctrl Pts',(12.0684754113869,22.613562676493,12.));
#176935=CARTESIAN_POINT('Ctrl Pts',(12.0455791139135,22.5983500505675,12.));
#176936=CARTESIAN_POINT('Ctrl Pts',(12.0227769113132,22.5831255061306,12.));
#176937=CARTESIAN_POINT('Ctrl Pts',(12.0000690046697,22.5678894211194,12.));
#176938=CARTESIAN_POINT('Ctrl Pts',(11.9774555943496,22.5526421741159,12.));
#176939=CARTESIAN_POINT('Ctrl Pts',(11.9549368843996,22.5373841537299,12.));
#176940=CARTESIAN_POINT('Ctrl Pts',(11.9325130877801,22.5221157697869,12.));
#176941=CARTESIAN_POINT('Ctrl Pts',(11.9101844254555,22.5068374513958,12.));
#176942=CARTESIAN_POINT('Ctrl Pts',(11.8879511239941,22.4915496418472,12.));
#176943=CARTESIAN_POINT('Ctrl Pts',(11.8658134137018,22.4762527946694,12.));
#176944=CARTESIAN_POINT('Ctrl Pts',(11.8437715264487,22.4609473690469,12.));
#176945=CARTESIAN_POINT('Ctrl Pts',(11.8218256937889,22.4456338258738,12.));
#176946=CARTESIAN_POINT('Ctrl Pts',(11.7999761445175,22.4303126226468,12.));
#176947=CARTESIAN_POINT('Ctrl Pts',(11.7782231042041,22.4149842125018,12.));
#176948=CARTESIAN_POINT('Ctrl Pts',(11.7565667964765,22.39964904692,12.));
#176949=CARTESIAN_POINT('Ctrl Pts',(11.7350074437961,22.3843075773905,12.));
#176950=CARTESIAN_POINT('Ctrl Pts',(11.7135452684532,22.3689602575492,12.));
#176951=CARTESIAN_POINT('Ctrl Pts',(11.6921804934056,22.3536075450028,12.));
#176952=CARTESIAN_POINT('Ctrl Pts',(11.6709133432986,22.3382499035618,12.));
#176953=CARTESIAN_POINT('Ctrl Pts',(11.6497440449858,22.3228878043976,12.));
#176954=CARTESIAN_POINT('Ctrl Pts',(11.6286728270011,22.3075217249049,12.));
#176955=CARTESIAN_POINT('Ctrl Pts',(11.6076999192359,22.2921521480358,12.));
#176956=CARTESIAN_POINT('Ctrl Pts',(11.5868255525189,22.2767795614349,12.));
#176957=CARTESIAN_POINT('Ctrl Pts',(11.5660499582403,22.2614044566898,12.));
#176958=CARTESIAN_POINT('Ctrl Pts',(11.545373367912,22.2460273284653,12.));
#176959=CARTESIAN_POINT('Ctrl Pts',(11.5247960128476,22.2306486738899,12.));
#176960=CARTESIAN_POINT('Ctrl Pts',(11.504318124424,22.215268993102,12.));
#176961=CARTESIAN_POINT('Ctrl Pts',(11.4839399342589,22.1998887896435,12.));
#176962=CARTESIAN_POINT('Ctrl Pts',(11.463661674411,22.184508570917,12.));
#176963=CARTESIAN_POINT('Ctrl Pts',(11.443483577557,22.1691288486096,12.));
#176964=CARTESIAN_POINT('Ctrl Pts',(11.4234058771742,22.1537501391486,12.));
#176965=CARTESIAN_POINT('Ctrl Pts',(11.4034288076908,22.1383729640963,12.));
#176966=CARTESIAN_POINT('Ctrl Pts',(11.3835526044256,22.1229978500185,12.));
#176967=CARTESIAN_POINT('Ctrl Pts',(11.3637775035367,22.1076253283978,12.));
#176968=CARTESIAN_POINT('Ctrl Pts',(11.3441037419553,22.0922559355293,12.));
#176969=CARTESIAN_POINT('Ctrl Pts',(11.3245315573168,22.0768902124267,12.));
#176970=CARTESIAN_POINT('Ctrl Pts',(11.3050611878771,22.0615287047179,12.));
#176971=CARTESIAN_POINT('Ctrl Pts',(11.2856928724374,22.0461719625661,12.));
#176972=CARTESIAN_POINT('Ctrl Pts',(11.2664268504207,22.0308205408351,12.));
#176973=CARTESIAN_POINT('Ctrl Pts',(11.2472633619276,22.0154749992364,12.));
#176974=CARTESIAN_POINT('Ctrl Pts',(11.2282026477897,22.000135902484,12.));
#176975=CARTESIAN_POINT('Ctrl Pts',(11.2092449496125,21.9848038204439,12.));
#176976=CARTESIAN_POINT('Ctrl Pts',(11.1903905098109,21.9694793282913,12.));
#176977=CARTESIAN_POINT('Ctrl Pts',(11.1716395716375,21.9541630066504,12.));
#176978=CARTESIAN_POINT('Ctrl Pts',(11.1529923792002,21.9388554416437,12.));
#176979=CARTESIAN_POINT('Ctrl Pts',(11.134449177474,21.9235572249518,12.));
#176980=CARTESIAN_POINT('Ctrl Pts',(11.1160102123024,21.9082689538687,12.));
#176981=CARTESIAN_POINT('Ctrl Pts',(11.0976757303944,21.8929912313608,12.));
#176982=CARTESIAN_POINT('Ctrl Pts',(11.0794459793058,21.8777246661191,12.));
#176983=CARTESIAN_POINT('Ctrl Pts',(11.0613212074364,21.8624698726319,12.));
#176984=CARTESIAN_POINT('Ctrl Pts',(11.0433016640808,21.8472274713103,12.));
#176985=CARTESIAN_POINT('Ctrl Pts',(11.0253875994598,21.8319980886033,12.));
#176986=CARTESIAN_POINT('Ctrl Pts',(11.0075792647477,21.8167823571168,12.));
#176987=CARTESIAN_POINT('Ctrl Pts',(10.9898769120913,21.8015809157302,12.));
#176988=CARTESIAN_POINT('Ctrl Pts',(10.9722807946157,21.7863944097143,12.));
#176989=CARTESIAN_POINT('Ctrl Pts',(10.9547911664457,21.7712234908468,12.));
#176990=CARTESIAN_POINT('Ctrl Pts',(10.9374082827446,21.7560688175252,12.));
#176991=CARTESIAN_POINT('Ctrl Pts',(10.9201323997386,21.74093105488,12.));
#176992=CARTESIAN_POINT('Ctrl Pts',(10.9029637747341,21.7258108748874,12.));
#176993=CARTESIAN_POINT('Ctrl Pts',(10.8859026661292,21.7107089564822,12.));
#176994=CARTESIAN_POINT('Ctrl Pts',(10.8689493334093,21.6956259856667,12.));
#176995=CARTESIAN_POINT('Ctrl Pts',(10.8521040371832,21.6805626556461,12.));
#176996=CARTESIAN_POINT('Ctrl Pts',(10.835367039227,21.6655196669727,12.));
#176997=CARTESIAN_POINT('Ctrl Pts',(10.8187386025135,21.6504977276864,12.));
#176998=CARTESIAN_POINT('Ctrl Pts',(10.8022189912369,21.6354975534558,12.));
#176999=CARTESIAN_POINT('Ctrl Pts',(10.7858084708262,21.6205198677176,12.));
#177000=CARTESIAN_POINT('Ctrl Pts',(10.7695073079554,21.6055654018179,12.));
#177001=CARTESIAN_POINT('Ctrl Pts',(10.7533157705943,21.5906348951745,12.));
#177002=CARTESIAN_POINT('Ctrl Pts',(10.7372341280468,21.5757290954372,12.));
#177003=CARTESIAN_POINT('Ctrl Pts',(10.7212626509816,21.5608487586467,12.));
#177004=CARTESIAN_POINT('Ctrl Pts',(10.7054016114571,21.5459946493955,12.));
#177005=CARTESIAN_POINT('Ctrl Pts',(10.689651282929,21.531167540981,12.));
#177006=CARTESIAN_POINT('Ctrl Pts',(10.6740119402835,21.5163682155805,12.));
#177007=CARTESIAN_POINT('Ctrl Pts',(10.658483859894,21.5015974644454,12.));
#177008=CARTESIAN_POINT('Ctrl Pts',(10.6430673196609,21.4868560880893,12.));
#177009=CARTESIAN_POINT('Ctrl Pts',(10.6277625990456,21.4721448964766,12.));
#177010=CARTESIAN_POINT('Ctrl Pts',(10.612569979096,21.4574647092093,12.));
#177011=CARTESIAN_POINT('Ctrl Pts',(10.597489742462,21.4428163557137,12.));
#177012=CARTESIAN_POINT('Ctrl Pts',(10.582522173457,21.4282006754624,12.));
#177013=CARTESIAN_POINT('Ctrl Pts',(10.5676675581106,21.4136185181974,12.));
#177014=CARTESIAN_POINT('Ctrl Pts',(10.5529261842107,21.3990707441495,12.));
#177015=CARTESIAN_POINT('Ctrl Pts',(10.5382983413422,21.3845582242604,12.));
#177016=CARTESIAN_POINT('Ctrl Pts',(10.523784320906,21.3700818403942,12.));
#177017=CARTESIAN_POINT('Ctrl Pts',(10.5093844161689,21.3556424855822,12.));
#177018=CARTESIAN_POINT('Ctrl Pts',(10.4950989223341,21.3412410642912,12.));
#177019=CARTESIAN_POINT('Ctrl Pts',(10.4809281365933,21.3268784926823,12.));
#177020=CARTESIAN_POINT('Ctrl Pts',(10.4668723581768,21.312555698873,12.));
#177021=CARTESIAN_POINT('Ctrl Pts',(10.452931888387,21.2982736231924,12.));
#177022=CARTESIAN_POINT('Ctrl Pts',(10.4391070306385,21.2840332184471,12.));
#177023=CARTESIAN_POINT('Ctrl Pts',(10.4253980905394,21.2698354502391,12.));
#177024=CARTESIAN_POINT('Ctrl Pts',(10.4118053759584,21.2556812972741,12.));
#177025=CARTESIAN_POINT('Ctrl Pts',(10.3983291970846,21.2415717516713,12.));
#177026=CARTESIAN_POINT('Ctrl Pts',(10.384969866479,21.2275078192708,12.));
#177027=CARTESIAN_POINT('Ctrl Pts',(10.3717276991137,21.2134905199359,12.));
#177028=CARTESIAN_POINT('Ctrl Pts',(10.3586030124595,21.1995208879205,12.));
#177029=CARTESIAN_POINT('Ctrl Pts',(10.3455961265706,21.1855999722427,12.));
#177030=CARTESIAN_POINT('Ctrl Pts',(10.3327073641574,21.1717288370512,12.));
#177031=CARTESIAN_POINT('Ctrl Pts',(10.3199370506541,21.1579085619959,12.));
#177032=CARTESIAN_POINT('Ctrl Pts',(10.307285514268,21.1441402425831,12.));
#177033=CARTESIAN_POINT('Ctrl Pts',(10.2947530860714,21.130424990599,12.));
#177034=CARTESIAN_POINT('Ctrl Pts',(10.2823401001067,21.1167639345623,12.));
#177035=CARTESIAN_POINT('Ctrl Pts',(10.2700468934743,21.1031582201625,12.));
#177036=CARTESIAN_POINT('Ctrl Pts',(10.2578738064183,21.0896090107066,12.));
#177037=CARTESIAN_POINT('Ctrl Pts',(10.2458211823915,21.0761174875448,12.));
#177038=CARTESIAN_POINT('Ctrl Pts',(10.233889368157,21.0626848505665,12.));
#177039=CARTESIAN_POINT('Ctrl Pts',(10.2220787139157,21.0493123187484,12.));
#177040=CARTESIAN_POINT('Ctrl Pts',(10.2103895734123,21.0360011306814,12.));
#177041=CARTESIAN_POINT('Ctrl Pts',(10.1988223040425,21.0227525451107,12.));
#177042=CARTESIAN_POINT('Ctrl Pts',(10.1873772669358,21.0095678414486,12.));
#177043=CARTESIAN_POINT('Ctrl Pts',(10.1760548270765,20.9964483203685,12.));
#177044=CARTESIAN_POINT('Ctrl Pts',(10.1648553534567,20.9833953044737,12.));
#177045=CARTESIAN_POINT('Ctrl Pts',(10.1537792192065,20.970410138937,12.));
#177046=CARTESIAN_POINT('Ctrl Pts',(10.1428268017257,20.9574941921591,12.));
#177047=CARTESIAN_POINT('Ctrl Pts',(10.1319984827909,20.944648856393,12.));
#177048=CARTESIAN_POINT('Ctrl Pts',(10.1212946487057,20.931875548473,12.));
#177049=CARTESIAN_POINT('Ctrl Pts',(10.1107156904836,20.9191757106266,12.));
#177050=CARTESIAN_POINT('Ctrl Pts',(10.1002620040076,20.9065508112556,12.));
#177051=CARTESIAN_POINT('Ctrl Pts',(10.0899339901916,20.8940023457371,12.));
#177052=CARTESIAN_POINT('Ctrl Pts',(10.0797320551154,20.8815318371844,12.));
#177053=CARTESIAN_POINT('Ctrl Pts',(10.0696566102219,20.8691408373705,12.));
#177054=CARTESIAN_POINT('Ctrl Pts',(10.0597080725375,20.856830927732,12.));
#177055=CARTESIAN_POINT('Ctrl Pts',(10.0498868648733,20.8446037203402,12.));
#177056=CARTESIAN_POINT('Ctrl Pts',(10.0401934160234,20.8324608588906,12.));
#177057=CARTESIAN_POINT('Ctrl Pts',(10.0306281609435,20.8204040196599,12.));
#177058=CARTESIAN_POINT('Ctrl Pts',(10.0211915410095,20.8084349126885,12.));
#177059=CARTESIAN_POINT('Ctrl Pts',(10.0118840042786,20.7965552829907,12.));
#177060=CARTESIAN_POINT('Ctrl Pts',(10.0027060057389,20.7847669117568,12.));
#177061=CARTESIAN_POINT('Ctrl Pts',(9.99365800754637,20.7730716175417,12.));
#177062=CARTESIAN_POINT('Ctrl Pts',(9.98474047926846,20.7614712574989,12.));
#177063=CARTESIAN_POINT('Ctrl Pts',(9.97595389823461,20.7499677289626,12.));
#177064=CARTESIAN_POINT('Ctrl Pts',(9.96729874986198,20.7385629709795,12.));
#177065=CARTESIAN_POINT('Ctrl Pts',(9.95877552798403,20.7272589658752,12.));
#177066=CARTESIAN_POINT('Ctrl Pts',(9.95038473514962,20.7160577407581,12.));
#177067=CARTESIAN_POINT('Ctrl Pts',(9.9421268829825,20.7049613692237,12.));
#177068=CARTESIAN_POINT('Ctrl Pts',(9.93400249259736,20.6939719732485,12.));
#177069=CARTESIAN_POINT('Ctrl Pts',(9.9260120949875,20.6830917250255,12.));
#177070=CARTESIAN_POINT('Ctrl Pts',(9.91815623141284,20.6723228488262,12.));
#177071=CARTESIAN_POINT('Ctrl Pts',(9.91043545377004,20.6616676228315,12.));
#177072=CARTESIAN_POINT('Ctrl Pts',(9.90285032516695,20.6511283817415,12.));
#177073=CARTESIAN_POINT('Ctrl Pts',(9.89540142049123,20.6407075193977,12.));
#177074=CARTESIAN_POINT('Ctrl Pts',(9.88808932697304,20.6304074914086,12.));
#177075=CARTESIAN_POINT('Ctrl Pts',(9.88091464472669,20.6202308177472,12.));
#177076=CARTESIAN_POINT('Ctrl Pts',(9.87387798732943,20.6101800854491,12.));
#177077=CARTESIAN_POINT('Ctrl Pts',(9.86697998242612,20.6002579513696,12.));
#177078=CARTESIAN_POINT('Ctrl Pts',(9.86022127232749,20.5904671449755,12.));
#177079=CARTESIAN_POINT('Ctrl Pts',(9.85360251457004,20.580810471002,12.));
#177080=CARTESIAN_POINT('Ctrl Pts',(9.84712438256308,20.5712908125145,12.));
#177081=CARTESIAN_POINT('Ctrl Pts',(9.84078756677589,20.5619111362406,12.));
#177082=CARTESIAN_POINT('Ctrl Pts',(9.8345927758532,20.5526744976461,12.));
#177083=CARTESIAN_POINT('Ctrl Pts',(9.82854073773857,20.5435840460717,12.));
#177084=CARTESIAN_POINT('Ctrl Pts',(9.82263220080327,20.534643029951,12.));
#177085=CARTESIAN_POINT('Ctrl Pts',(9.81686793455918,20.5258548000625,12.));
#177086=CARTESIAN_POINT('Ctrl Pts',(9.81124873025278,20.5172228122839,12.));
#177087=CARTESIAN_POINT('Ctrl Pts',(9.80577540161102,20.5087506310507,12.));
#177088=CARTESIAN_POINT('Ctrl Pts',(9.80044878520967,20.500441931211,12.));
#177089=CARTESIAN_POINT('Ctrl Pts',(9.79526974288343,20.4923005087945,12.));
#177090=CARTESIAN_POINT('Ctrl Pts',(9.79023916498659,20.4843302955329,12.));
#177091=CARTESIAN_POINT('Ctrl Pts',(9.78535797314162,20.4765353711585,12.));
#177092=CARTESIAN_POINT('Ctrl Pts',(9.78062712373313,20.4689199790668,12.));
#177093=CARTESIAN_POINT('Ctrl Pts',(9.77604760815522,20.4614885274973,12.));
#177094=CARTESIAN_POINT('Ctrl Pts',(9.77162045104069,20.4542455817527,12.));
#177095=CARTESIAN_POINT('Ctrl Pts',(9.76734670980896,20.447195862298,12.));
#177096=CARTESIAN_POINT('Ctrl Pts',(9.76322747195502,20.4403442329401,12.));
#177097=CARTESIAN_POINT('Ctrl Pts',(9.75926386289929,20.4336957355474,12.));
#177098=CARTESIAN_POINT('Ctrl Pts',(9.75545705902416,20.4272556476629,12.));
#177099=CARTESIAN_POINT('Ctrl Pts',(9.75180829786433,20.4210295275818,12.));
#177100=CARTESIAN_POINT('Ctrl Pts',(9.74831889242174,20.4150232777393,12.));
#177101=CARTESIAN_POINT('Ctrl Pts',(9.74499021838536,20.4092430879861,12.));
#177102=CARTESIAN_POINT('Ctrl Pts',(9.74182369656272,20.4036953576549,12.));
#177103=CARTESIAN_POINT('Ctrl Pts',(9.73882077613206,20.3983866213331,12.));
#177104=CARTESIAN_POINT('Ctrl Pts',(9.73598292014249,20.3933234845646,12.));
#177105=CARTESIAN_POINT('Ctrl Pts',(9.73331167102812,20.3885129129912,12.));
#177106=CARTESIAN_POINT('Ctrl Pts',(9.73080870123726,20.3839624556742,12.));
#177107=CARTESIAN_POINT('Ctrl Pts',(9.72847589116532,20.3796805893304,12.));
#177108=CARTESIAN_POINT('Ctrl Pts',(9.7263153173287,20.3756766651952,12.));
#177109=CARTESIAN_POINT('Ctrl Pts',(9.72432910043192,20.371960235676,12.));
#177110=CARTESIAN_POINT('Ctrl Pts',(9.72251930722503,20.3685406190576,12.));
#177111=CARTESIAN_POINT('Ctrl Pts',(9.72088778381101,20.3654261611055,12.));
#177112=CARTESIAN_POINT('Ctrl Pts',(9.71943648548114,20.362625691398,12.));
#177113=CARTESIAN_POINT('Ctrl Pts',(9.71816778327998,20.3601498764344,12.));
#177114=CARTESIAN_POINT('Ctrl Pts',(9.71708493723061,20.3580133103357,12.));
#177115=CARTESIAN_POINT('Ctrl Pts',(9.71619192554146,20.3562337557875,12.));
#177116=CARTESIAN_POINT('Ctrl Pts',(9.71549257088174,20.3548282742361,12.));
#177117=CARTESIAN_POINT('Ctrl Pts',(9.714989780521,20.3538098605706,12.));
#177118=CARTESIAN_POINT('Ctrl Pts',(9.71474590350791,20.3533097561886,12.));
#177119=CARTESIAN_POINT('Ctrl Pts',(9.71465227853122,20.3531126095522,12.));
#177120=CARTESIAN_POINT('Ctrl Pts',(9.71462954053074,20.353060251684,12.));
#177121=CARTESIAN_POINT('Ctrl Pts',(9.71462809124917,20.353053841303,12.));
#177122=CARTESIAN_POINT('',(9.47413589477549,19.84920021178,12.));
#177123=CARTESIAN_POINT('',(4.63060338698782,9.70154690100589,12.));
#177124=CARTESIAN_POINT('',(8.8178352198485,19.6085639972844,12.));
#177125=CARTESIAN_POINT('Origin',(9.02290115519382,20.0645771135003,12.));
#177126=CARTESIAN_POINT('',(7.63019749246978,20.1004996511507,12.));
#177127=CARTESIAN_POINT('Origin',(3.26562511982935E-13,7.08841632778409E-13,
12.));
#177128=CARTESIAN_POINT('',(7.33627833380047,20.7347298079577,12.));
#177129=CARTESIAN_POINT('Origin',(7.80764394578303,20.56795313141,12.));
#177130=CARTESIAN_POINT('',(7.52250298901265,21.2610617890679,12.));
#177131=CARTESIAN_POINT('',(3.76125149450631,10.6305308945339,12.));
#177132=CARTESIAN_POINT('',(7.36589684767344,24.9347862158358,12.));
#177133=CARTESIAN_POINT('Ctrl Pts',(7.52250298901265,21.2610617890679,12.));
#177134=CARTESIAN_POINT('Ctrl Pts',(7.52250649703991,21.2610673466883,12.));
#177135=CARTESIAN_POINT('Ctrl Pts',(7.52252744144957,21.261120447486,12.));
#177136=CARTESIAN_POINT('Ctrl Pts',(7.52260064231736,21.2613260540651,12.));
#177137=CARTESIAN_POINT('Ctrl Pts',(7.52278182242727,21.261852128355,12.));
#177138=CARTESIAN_POINT('Ctrl Pts',(7.52314642316202,21.262927782038,12.));
#177139=CARTESIAN_POINT('Ctrl Pts',(7.52364573027521,21.2644161259965,12.));
#177140=CARTESIAN_POINT('Ctrl Pts',(7.52427261074263,21.266305915706,12.));
#177141=CARTESIAN_POINT('Ctrl Pts',(7.52501770333521,21.2685823838672,12.));
#177142=CARTESIAN_POINT('Ctrl Pts',(7.52587126095544,21.2712301573465,12.));
#177143=CARTESIAN_POINT('Ctrl Pts',(7.5268252691856,21.2742366113578,12.));
#177144=CARTESIAN_POINT('Ctrl Pts',(7.52787386225343,21.2775925269652,12.));
#177145=CARTESIAN_POINT('Ctrl Pts',(7.52901217930407,21.2812902781143,12.));
#177146=CARTESIAN_POINT('Ctrl Pts',(7.5302356243822,21.2853226580658,12.));
#177147=CARTESIAN_POINT('Ctrl Pts',(7.53153906987846,21.2896816163843,12.));
#177148=CARTESIAN_POINT('Ctrl Pts',(7.53291726078526,21.2943588989331,12.));
#177149=CARTESIAN_POINT('Ctrl Pts',(7.53436505309948,21.2993464250717,12.));
#177150=CARTESIAN_POINT('Ctrl Pts',(7.53587778251743,21.3046368712157,12.));
#177151=CARTESIAN_POINT('Ctrl Pts',(7.53745129364619,21.3102237167729,12.));
#177152=CARTESIAN_POINT('Ctrl Pts',(7.53908175169898,21.3161009456256,12.));
#177153=CARTESIAN_POINT('Ctrl Pts',(7.54076552038279,21.3222628524165,12.));
#177154=CARTESIAN_POINT('Ctrl Pts',(7.54249900377031,21.328703791771,12.));
#177155=CARTESIAN_POINT('Ctrl Pts',(7.54427868151268,21.3354182340149,12.));
#177156=CARTESIAN_POINT('Ctrl Pts',(7.5461011494835,21.3424008295038,12.));
#177157=CARTESIAN_POINT('Ctrl Pts',(7.54796316246326,21.349646476153,12.));
#177158=CARTESIAN_POINT('Ctrl Pts',(7.54986166521306,21.3571503685853,12.));
#177159=CARTESIAN_POINT('Ctrl Pts',(7.55179375777441,21.3649079431864,12.));
#177160=CARTESIAN_POINT('Ctrl Pts',(7.55375667080031,21.3729148390244,12.));
#177161=CARTESIAN_POINT('Ctrl Pts',(7.55574773403507,21.3811668478933,12.));
#177162=CARTESIAN_POINT('Ctrl Pts',(7.55776435731421,21.3896598842119,12.));
#177163=CARTESIAN_POINT('Ctrl Pts',(7.55980403700614,21.3983899952988,12.));
#177164=CARTESIAN_POINT('Ctrl Pts',(7.56186435703622,21.4073533630364,12.));
#177165=CARTESIAN_POINT('Ctrl Pts',(7.56394299313682,21.4165463106252,12.));
#177166=CARTESIAN_POINT('Ctrl Pts',(7.56603771218706,21.4259653015732,12.));
#177167=CARTESIAN_POINT('Ctrl Pts',(7.56814636360841,21.435606926151,12.));
#177168=CARTESIAN_POINT('Ctrl Pts',(7.57026687261169,21.445467890751,12.));
#177169=CARTESIAN_POINT('Ctrl Pts',(7.57239723223521,21.4555450053147,12.));
#177170=CARTESIAN_POINT('Ctrl Pts',(7.57453549743434,21.4658351740135,12.));
#177171=CARTESIAN_POINT('Ctrl Pts',(7.57667978403001,21.4763353936766,12.));
#177172=CARTESIAN_POINT('Ctrl Pts',(7.57882826679131,21.4870427508193,12.));
#177173=CARTESIAN_POINT('Ctrl Pts',(7.58097917790729,21.497954419274,12.));
#177174=CARTESIAN_POINT('Ctrl Pts',(7.58313080519158,21.5090676573866,12.));
#177175=CARTESIAN_POINT('Ctrl Pts',(7.58528148919113,21.5203798035294,12.));
#177176=CARTESIAN_POINT('Ctrl Pts',(7.58742962034834,21.5318882716736,12.));
#177177=CARTESIAN_POINT('Ctrl Pts',(7.58957363620026,21.5435905470113,12.));
#177178=CARTESIAN_POINT('Ctrl Pts',(7.59171201844792,21.5554841813466,12.));
#177179=CARTESIAN_POINT('Ctrl Pts',(7.59384329124929,21.5675667904728,12.));
#177180=CARTESIAN_POINT('Ctrl Pts',(7.59596601973588,21.5798360518978,12.));
#177181=CARTESIAN_POINT('Ctrl Pts',(7.59807880846192,21.5922897024466,12.));
#177182=CARTESIAN_POINT('Ctrl Pts',(7.60018029988238,21.6049255358843,12.));
#177183=CARTESIAN_POINT('Ctrl Pts',(7.60226917285431,21.6177414005991,12.));
#177184=CARTESIAN_POINT('Ctrl Pts',(7.60434414118299,21.6307351973823,12.));
#177185=CARTESIAN_POINT('Ctrl Pts',(7.60640395216358,21.6439048771743,12.));
#177186=CARTESIAN_POINT('Ctrl Pts',(7.60844738512871,21.6572484388079,12.));
#177187=CARTESIAN_POINT('Ctrl Pts',(7.61047325000949,21.6707639267573,12.));
#177188=CARTESIAN_POINT('Ctrl Pts',(7.61248038630264,21.6844494295813,12.));
#177189=CARTESIAN_POINT('Ctrl Pts',(7.61446766202786,21.6983030783321,12.));
#177190=CARTESIAN_POINT('Ctrl Pts',(7.61643397270424,21.7123230449835,12.));
#177191=CARTESIAN_POINT('Ctrl Pts',(7.61837824030541,21.7265075407977,12.));
#177192=CARTESIAN_POINT('Ctrl Pts',(7.62029941230854,21.7408548148657,12.));
#177193=CARTESIAN_POINT('Ctrl Pts',(7.62219646084225,21.7553631528329,12.));
#177194=CARTESIAN_POINT('Ctrl Pts',(7.62406838181164,21.7700308755584,12.));
#177195=CARTESIAN_POINT('Ctrl Pts',(7.6259141940452,21.7848563378022,12.));
#177196=CARTESIAN_POINT('Ctrl Pts',(7.62773293842409,21.7998379268583,12.));
#177197=CARTESIAN_POINT('Ctrl Pts',(7.62952367718151,21.8149740615093,12.));
#177198=CARTESIAN_POINT('Ctrl Pts',(7.6312854932304,21.8302631910197,12.));
#177199=CARTESIAN_POINT('Ctrl Pts',(7.63301748948936,21.8457037941084,12.));
#177200=CARTESIAN_POINT('Ctrl Pts',(7.63471878821203,21.8612943779086,12.));
#177201=CARTESIAN_POINT('Ctrl Pts',(7.63638853033367,21.8770334769492,12.));
#177202=CARTESIAN_POINT('Ctrl Pts',(7.63802587492007,21.8929196523511,12.));
#177203=CARTESIAN_POINT('Ctrl Pts',(7.63962999860916,21.9089514909873,12.));
#177204=CARTESIAN_POINT('Ctrl Pts',(7.64120009506539,21.9251276046546,12.));
#177205=CARTESIAN_POINT('Ctrl Pts',(7.64273537442706,21.9414466292074,12.));
#177206=CARTESIAN_POINT('Ctrl Pts',(7.64423506279153,21.9579072237653,12.));
#177207=CARTESIAN_POINT('Ctrl Pts',(7.64569840177359,21.97450807008,12.));
#177208=CARTESIAN_POINT('Ctrl Pts',(7.64712464805257,21.9912478718542,12.));
#177209=CARTESIAN_POINT('Ctrl Pts',(7.64851307293345,22.0081253540774,12.));
#177210=CARTESIAN_POINT('Ctrl Pts',(7.64986296190156,22.025139262321,12.));
#177211=CARTESIAN_POINT('Ctrl Pts',(7.65117361421346,22.0422883621176,12.));
#177212=CARTESIAN_POINT('Ctrl Pts',(7.65244434253103,22.0595714384432,12.));
#177213=CARTESIAN_POINT('Ctrl Pts',(7.65367447254944,22.0769872951596,12.));
#177214=CARTESIAN_POINT('Ctrl Pts',(7.6548633426365,22.094534754469,12.));
#177215=CARTESIAN_POINT('Ctrl Pts',(7.65601030346818,22.1122126563327,12.));
#177216=CARTESIAN_POINT('Ctrl Pts',(7.65711471769406,22.1300198579671,12.));
#177217=CARTESIAN_POINT('Ctrl Pts',(7.6581759596335,22.1479552334206,12.));
#177218=CARTESIAN_POINT('Ctrl Pts',(7.65919341496925,22.1660176731174,12.));
#177219=CARTESIAN_POINT('Ctrl Pts',(7.66016648045007,22.1842060834093,12.));
#177220=CARTESIAN_POINT('Ctrl Pts',(7.66109456359292,22.2025193860972,12.));
#177221=CARTESIAN_POINT('Ctrl Pts',(7.66197708240435,22.2209565180098,12.));
#177222=CARTESIAN_POINT('Ctrl Pts',(7.66281346512545,22.239516430656,12.));
#177223=CARTESIAN_POINT('Ctrl Pts',(7.66360314997661,22.2581980898487,12.));
#177224=CARTESIAN_POINT('Ctrl Pts',(7.66434558490972,22.2770004753332,12.));
#177225=CARTESIAN_POINT('Ctrl Pts',(7.66504022736262,22.2959225803925,12.));
#177226=CARTESIAN_POINT('Ctrl Pts',(7.66568654402441,22.3149634114823,12.));
#177227=CARTESIAN_POINT('Ctrl Pts',(7.66628401061905,22.3341219879454,12.));
#177228=CARTESIAN_POINT('Ctrl Pts',(7.66683211169133,22.3533973417013,12.));
#177229=CARTESIAN_POINT('Ctrl Pts',(7.66733034039887,22.3727885169361,12.));
#177230=CARTESIAN_POINT('Ctrl Pts',(7.66777819830819,22.3922945697782,12.));
#177231=CARTESIAN_POINT('Ctrl Pts',(7.66817519519681,22.411914567977,12.));
#177232=CARTESIAN_POINT('Ctrl Pts',(7.66852084886745,22.4316475906616,12.));
#177233=CARTESIAN_POINT('Ctrl Pts',(7.66881468496659,22.4514927280863,12.));
#177234=CARTESIAN_POINT('Ctrl Pts',(7.66905623680835,22.47144908137,12.));
#177235=CARTESIAN_POINT('Ctrl Pts',(7.66924504520301,22.4915157622308,12.));
#177236=CARTESIAN_POINT('Ctrl Pts',(7.66938065829082,22.5116918927023,12.));
#177237=CARTESIAN_POINT('Ctrl Pts',(7.66946263138115,22.5319766049191,12.));
#177238=CARTESIAN_POINT('Ctrl Pts',(7.66949052679671,22.5523690409109,12.));
#177239=CARTESIAN_POINT('Ctrl Pts',(7.66946391372299,22.5728683523829,12.));
#177240=CARTESIAN_POINT('Ctrl Pts',(7.6693823680624,22.5934737004955,12.));
#177241=CARTESIAN_POINT('Ctrl Pts',(7.66924547229434,22.6141842556248,12.));
#177242=CARTESIAN_POINT('Ctrl Pts',(7.66905281533744,22.6349991971548,12.));
#177243=CARTESIAN_POINT('Ctrl Pts',(7.66880399241353,22.6559177133133,12.));
#177244=CARTESIAN_POINT('Ctrl Pts',(7.66849860491762,22.6769390009889,12.));
#177245=CARTESIAN_POINT('Ctrl Pts',(7.66813626029276,22.6980622655446,12.));
#177246=CARTESIAN_POINT('Ctrl Pts',(7.6677165719101,22.7192867206242,12.));
#177247=CARTESIAN_POINT('Ctrl Pts',(7.66723915895412,22.7406115879508,12.));
#177248=CARTESIAN_POINT('Ctrl Pts',(7.66670364630273,22.7620360971839,12.));
#177249=CARTESIAN_POINT('Ctrl Pts',(7.66610966441259,22.7835594857697,12.));
#177250=CARTESIAN_POINT('Ctrl Pts',(7.66545684920987,22.8051809987834,12.));
#177251=CARTESIAN_POINT('Ctrl Pts',(7.66474484198552,22.8268998887679,12.));
#177252=CARTESIAN_POINT('Ctrl Pts',(7.66397328929805,22.8487154155569,12.));
#177253=CARTESIAN_POINT('Ctrl Pts',(7.66314184287333,22.870626846128,12.));
#177254=CARTESIAN_POINT('Ctrl Pts',(7.66225015950147,22.8926334544879,12.));
#177255=CARTESIAN_POINT('Ctrl Pts',(7.66129790094099,22.9147345215418,12.));
#177256=CARTESIAN_POINT('Ctrl Pts',(7.66028473382776,22.9369293349592,12.));
#177257=CARTESIAN_POINT('Ctrl Pts',(7.65921032958911,22.9592171890332,12.));
#177258=CARTESIAN_POINT('Ctrl Pts',(7.65807436436452,22.9815973845301,12.));
#177259=CARTESIAN_POINT('Ctrl Pts',(7.6568765189133,23.004069228582,12.));
#177260=CARTESIAN_POINT('Ctrl Pts',(7.65561647852554,23.0266320345792,12.));
#177261=CARTESIAN_POINT('Ctrl Pts',(7.65429393293955,23.049285122053,12.));
#177262=CARTESIAN_POINT('Ctrl Pts',(7.65290857626356,23.072027816555,12.));
#177263=CARTESIAN_POINT('Ctrl Pts',(7.65146010690464,23.0948594495246,12.));
#177264=CARTESIAN_POINT('Ctrl Pts',(7.64994822749844,23.1177793581674,12.));
#177265=CARTESIAN_POINT('Ctrl Pts',(7.64837264482929,23.1407868853815,12.));
#177266=CARTESIAN_POINT('Ctrl Pts',(7.64673306975796,23.1638813796691,12.));
#177267=CARTESIAN_POINT('Ctrl Pts',(7.64502921715482,23.1870621950452,12.));
#177268=CARTESIAN_POINT('Ctrl Pts',(7.64326080583683,23.2103286909399,12.));
#177269=CARTESIAN_POINT('Ctrl Pts',(7.64142755851507,23.2336802320912,12.));
#177270=CARTESIAN_POINT('Ctrl Pts',(7.63952920172837,23.2571161884487,12.));
#177271=CARTESIAN_POINT('Ctrl Pts',(7.63756546576374,23.2806359350853,12.));
#177272=CARTESIAN_POINT('Ctrl Pts',(7.63553608458783,23.3042388521021,12.));
#177273=CARTESIAN_POINT('Ctrl Pts',(7.63344079578162,23.3279243245241,12.));
#177274=CARTESIAN_POINT('Ctrl Pts',(7.63127934048138,23.3516917421973,12.));
#177275=CARTESIAN_POINT('Ctrl Pts',(7.62905146332597,23.3755404996638,12.));
#177276=CARTESIAN_POINT('Ctrl Pts',(7.62675691240334,23.3994699961122,12.));
#177277=CARTESIAN_POINT('Ctrl Pts',(7.62439543920053,23.4234796353544,12.));
#177278=CARTESIAN_POINT('Ctrl Pts',(7.62196679855957,23.4475688257855,12.));
#177279=CARTESIAN_POINT('Ctrl Pts',(7.61947074863977,23.4717369803438,12.));
#177280=CARTESIAN_POINT('Ctrl Pts',(7.61690705088318,23.4959835164608,12.));
#177281=CARTESIAN_POINT('Ctrl Pts',(7.61427546999298,23.5203078560128,12.));
#177282=CARTESIAN_POINT('Ctrl Pts',(7.61157577385371,23.5447094252029,12.));
#177283=CARTESIAN_POINT('Ctrl Pts',(7.60880773344599,23.5691876544243,12.));
#177284=CARTESIAN_POINT('Ctrl Pts',(7.60597112277094,23.5937419781244,12.));
#177285=CARTESIAN_POINT('Ctrl Pts',(7.60306571877806,23.6183718346576,12.));
#177286=CARTESIAN_POINT('Ctrl Pts',(7.60009130130129,23.6430766661419,12.));
#177287=CARTESIAN_POINT('Ctrl Pts',(7.59704765299572,23.6678559182876,12.));
#177288=CARTESIAN_POINT('Ctrl Pts',(7.59393455934041,23.6927090405067,12.));
#177289=CARTESIAN_POINT('Ctrl Pts',(7.59075180865326,23.7176354860457,12.));
#177290=CARTESIAN_POINT('Ctrl Pts',(7.58749919210831,23.7426347121006,12.));
#177291=CARTESIAN_POINT('Ctrl Pts',(7.58417650376271,23.7677061799376,12.));
#177292=CARTESIAN_POINT('Ctrl Pts',(7.58078354058211,23.7928493549908,12.));
#177293=CARTESIAN_POINT('Ctrl Pts',(7.57732010249065,23.8180637069977,12.));
#177294=CARTESIAN_POINT('Ctrl Pts',(7.57378599219816,23.8433487096134,12.));
#177295=CARTESIAN_POINT('Ctrl Pts',(7.5701810150071,23.8687038399598,12.));
#177296=CARTESIAN_POINT('Ctrl Pts',(7.56650497863791,23.8941285782003,12.));
#177297=CARTESIAN_POINT('Ctrl Pts',(7.56275769304773,23.9196224070759,12.));
#177298=CARTESIAN_POINT('Ctrl Pts',(7.55893897027682,23.9451848115,12.));
#177299=CARTESIAN_POINT('Ctrl Pts',(7.55504862424811,23.9708152779884,12.));
#177300=CARTESIAN_POINT('Ctrl Pts',(7.5510864709744,23.9965132953185,12.));
#177301=CARTESIAN_POINT('Ctrl Pts',(7.5470523288591,24.022278355453,12.));
#177302=CARTESIAN_POINT('Ctrl Pts',(7.54294601896144,24.0481099543353,12.));
#177303=CARTESIAN_POINT('Ctrl Pts',(7.53876736531013,24.0740075927985,12.));
#177304=CARTESIAN_POINT('Ctrl Pts',(7.53451619514649,24.0999707772642,12.));
#177305=CARTESIAN_POINT('Ctrl Pts',(7.53019233935501,24.1259990209207,12.));
#177306=CARTESIAN_POINT('Ctrl Pts',(7.52579563201423,24.1520918425364,12.));
#177307=CARTESIAN_POINT('Ctrl Pts',(7.52132590953801,24.1782487641594,12.));
#177308=CARTESIAN_POINT('Ctrl Pts',(7.51678300997949,24.2044693092349,12.));
#177309=CARTESIAN_POINT('Ctrl Pts',(7.5121667722218,24.2307530003887,12.));
#177310=CARTESIAN_POINT('Ctrl Pts',(7.50747703535133,24.2570993577034,12.));
#177311=CARTESIAN_POINT('Ctrl Pts',(7.50271363765151,24.2835078958973,12.));
#177312=CARTESIAN_POINT('Ctrl Pts',(7.49787641695438,24.3099781253355,12.));
#177313=CARTESIAN_POINT('Ctrl Pts',(7.4929652125242,24.3365095573685,12.));
#177314=CARTESIAN_POINT('Ctrl Pts',(7.48797986651908,24.3631017084524,12.));
#177315=CARTESIAN_POINT('Ctrl Pts',(7.482920225693,24.3897541049254,12.));
#177316=CARTESIAN_POINT('Ctrl Pts',(7.47778614286564,24.4164662871163,12.));
#177317=CARTESIAN_POINT('Ctrl Pts',(7.47257747883246,24.443237814649,12.));
#177318=CARTESIAN_POINT('Ctrl Pts',(7.46729410308786,24.4700682684524,12.));
#177319=CARTESIAN_POINT('Ctrl Pts',(7.46193588961463,24.4969572391483,12.));
#177320=CARTESIAN_POINT('Ctrl Pts',(7.45650271335861,24.5239043173072,12.));
#177321=CARTESIAN_POINT('Ctrl Pts',(7.4509944465116,24.5509090831559,12.));
#177322=CARTESIAN_POINT('Ctrl Pts',(7.44541095473134,24.577971096086,12.));
#177323=CARTESIAN_POINT('Ctrl Pts',(7.43975209375503,24.6050898852368,12.));
#177324=CARTESIAN_POINT('Ctrl Pts',(7.43401770489523,24.6322649369517,12.));
#177325=CARTESIAN_POINT('Ctrl Pts',(7.42820762159125,24.6594957128756,12.));
#177326=CARTESIAN_POINT('Ctrl Pts',(7.42232167766265,24.6867816727192,12.));
#177327=CARTESIAN_POINT('Ctrl Pts',(7.41635971481674,24.7141222950051,12.));
#177328=CARTESIAN_POINT('Ctrl Pts',(7.41032159082381,24.7415170994784,12.));
#177329=CARTESIAN_POINT('Ctrl Pts',(7.40420718661602,24.7689656668983,12.));
#177330=CARTESIAN_POINT('Ctrl Pts',(7.39801641583012,24.7964676646431,12.));
#177331=CARTESIAN_POINT('Ctrl Pts',(7.39174922585808,24.8240228520893,12.));
#177332=CARTESIAN_POINT('Ctrl Pts',(7.3854055890362,24.8516310625176,12.));
#177333=CARTESIAN_POINT('Ctrl Pts',(7.37898549640269,24.8792921911115,12.));
#177334=CARTESIAN_POINT('Ctrl Pts',(7.37378825961676,24.901463382605,12.));
#177335=CARTESIAN_POINT('Ctrl Pts',(7.3698559312009,24.9181155530543,12.));
#177336=CARTESIAN_POINT('Ctrl Pts',(7.36721909028842,24.9292275670674,12.));
#177337=CARTESIAN_POINT('Ctrl Pts',(7.36589684767344,24.9347862158358,12.));
#177338=CARTESIAN_POINT('',(6.08833931617699,25.2771067246846,12.));
#177339=CARTESIAN_POINT('Origin',(0.,0.,12.));
#177340=CARTESIAN_POINT('',(4.11585220600461,22.1738711152697,12.));
#177341=CARTESIAN_POINT('Ctrl Pts',(6.08833931617699,25.2771067246846,12.));
#177342=CARTESIAN_POINT('Ctrl Pts',(6.08441489609793,25.2729539149517,12.));
#177343=CARTESIAN_POINT('Ctrl Pts',(6.0765753178749,25.2646490489923,12.));
#177344=CARTESIAN_POINT('Ctrl Pts',(6.06484373634546,25.2521940105705,12.));
#177345=CARTESIAN_POINT('Ctrl Pts',(6.04925720151218,25.2355918139032,12.));
#177346=CARTESIAN_POINT('Ctrl Pts',(6.02986667389996,25.21484662016,12.));
#177347=CARTESIAN_POINT('Ctrl Pts',(6.01056881804612,25.1941090269819,12.));
#177348=CARTESIAN_POINT('Ctrl Pts',(5.99136367859754,25.1733791296259,12.));
#177349=CARTESIAN_POINT('Ctrl Pts',(5.97225131495616,25.1526570863092,12.));
#177350=CARTESIAN_POINT('Ctrl Pts',(5.95323180187378,25.1319431317237,12.));
#177351=CARTESIAN_POINT('Ctrl Pts',(5.93430523086834,25.1112375971106,12.));
#177352=CARTESIAN_POINT('Ctrl Pts',(5.91547170844447,25.0905409050773,12.));
#177353=CARTESIAN_POINT('Ctrl Pts',(5.89673135155514,25.0698535426514,12.));
#177354=CARTESIAN_POINT('Ctrl Pts',(5.87808428385365,25.0491760405911,12.));
#177355=CARTESIAN_POINT('Ctrl Pts',(5.85953063156826,25.0285089498899,12.));
#177356=CARTESIAN_POINT('Ctrl Pts',(5.84107051963071,25.0078528200564,12.));
#177357=CARTESIAN_POINT('Ctrl Pts',(5.82270406744198,24.9872081752734,12.));
#177358=CARTESIAN_POINT('Ctrl Pts',(5.80443138549726,24.9665754954496,12.));
#177359=CARTESIAN_POINT('Ctrl Pts',(5.78625257775681,24.945955229334,12.));
#177360=CARTESIAN_POINT('Ctrl Pts',(5.76816774342219,24.9253478043656,12.));
#177361=CARTESIAN_POINT('Ctrl Pts',(5.75017697890804,24.904753637648,12.));
#177362=CARTESIAN_POINT('Ctrl Pts',(5.73228037976926,24.884173146722,12.));
#177363=CARTESIAN_POINT('Ctrl Pts',(5.71447804252027,24.8636067597669,12.));
#177364=CARTESIAN_POINT('Ctrl Pts',(5.69677006679444,24.8430549277621,12.));
#177365=CARTESIAN_POINT('Ctrl Pts',(5.67915655496542,24.8225181223845,12.));
#177366=CARTESIAN_POINT('Ctrl Pts',(5.66163761114921,24.8019968304605,12.));
#177367=CARTESIAN_POINT('Ctrl Pts',(5.6442133404226,24.781491549672,12.));
#177368=CARTESIAN_POINT('Ctrl Pts',(5.62688384790923,24.7610027835697,12.));
#177369=CARTESIAN_POINT('Ctrl Pts',(5.60964923798491,24.7405310372739,12.));
#177370=CARTESIAN_POINT('Ctrl Pts',(5.59250961323987,24.7200768119088,12.));
#177371=CARTESIAN_POINT('Ctrl Pts',(5.57546507427754,24.6996406035517,12.));
#177372=CARTESIAN_POINT('Ctrl Pts',(5.55851572025376,24.6792229061794,12.));
#177373=CARTESIAN_POINT('Ctrl Pts',(5.54166164919583,24.6588242134738,12.));
#177374=CARTESIAN_POINT('Ctrl Pts',(5.52490295840991,24.6384450211467,12.));
#177375=CARTESIAN_POINT('Ctrl Pts',(5.50823974481962,24.6180858289179,12.));
#177376=CARTESIAN_POINT('Ctrl Pts',(5.49167210537246,24.5977471429364,12.));
#177377=CARTESIAN_POINT('Ctrl Pts',(5.47520013724419,24.5774294770329,12.));
#177378=CARTESIAN_POINT('Ctrl Pts',(5.45882393762261,24.5571333514842,12.));
#177379=CARTESIAN_POINT('Ctrl Pts',(5.4425436035688,24.5368592922863,12.));
#177380=CARTESIAN_POINT('Ctrl Pts',(5.42635923183419,24.5166078302108,12.));
#177381=CARTESIAN_POINT('Ctrl Pts',(5.41027091869241,24.4963794999831,12.));
#177382=CARTESIAN_POINT('Ctrl Pts',(5.39427875973824,24.4761748393321,12.));
#177383=CARTESIAN_POINT('Ctrl Pts',(5.37838284973695,24.4559943883157,12.));
#177384=CARTESIAN_POINT('Ctrl Pts',(5.36258328273627,24.435838689915,12.));
#177385=CARTESIAN_POINT('Ctrl Pts',(5.34688015213537,24.4157082904614,12.));
#177386=CARTESIAN_POINT('Ctrl Pts',(5.33127355076033,24.3956037401293,12.));
#177387=CARTESIAN_POINT('Ctrl Pts',(5.31576357092526,24.3755255933917,12.));
#177388=CARTESIAN_POINT('Ctrl Pts',(5.30035030449063,24.3554744095075,12.));
#177389=CARTESIAN_POINT('Ctrl Pts',(5.28503384290648,24.3354507529414,12.));
#177390=CARTESIAN_POINT('Ctrl Pts',(5.26981427718798,24.3154551932221,12.));
#177391=CARTESIAN_POINT('Ctrl Pts',(5.25469169788856,24.2954883048447,12.));
#177392=CARTESIAN_POINT('Ctrl Pts',(5.23966619506289,24.2755506671525,12.));
#177393=CARTESIAN_POINT('Ctrl Pts',(5.22473785822442,24.2556428642294,12.));
#177394=CARTESIAN_POINT('Ctrl Pts',(5.20990677629176,24.2357654847766,12.));
#177395=CARTESIAN_POINT('Ctrl Pts',(5.19517303753647,24.2159191220171,12.));
#177396=CARTESIAN_POINT('Ctrl Pts',(5.18053672961398,24.1961043738756,12.));
#177397=CARTESIAN_POINT('Ctrl Pts',(5.16599793957985,24.1763218431344,12.));
#177398=CARTESIAN_POINT('Ctrl Pts',(5.15155675390079,24.1565721375971,12.));
#177399=CARTESIAN_POINT('Ctrl Pts',(5.13721325845745,24.1368558702443,12.));
#177400=CARTESIAN_POINT('Ctrl Pts',(5.12296753853857,24.117173659394,12.));
#177401=CARTESIAN_POINT('Ctrl Pts',(5.10881967883124,24.0975261288444,12.));
#177402=CARTESIAN_POINT('Ctrl Pts',(5.09476976342616,24.0779139079264,12.));
#177403=CARTESIAN_POINT('Ctrl Pts',(5.0808178758127,24.0583376315636,12.));
#177404=CARTESIAN_POINT('Ctrl Pts',(5.06696409886639,24.0387979403268,12.));
#177405=CARTESIAN_POINT('Ctrl Pts',(5.05320851483068,24.0192954804896,12.));
#177406=CARTESIAN_POINT('Ctrl Pts',(5.03955120528527,23.9998309040747,12.));
#177407=CARTESIAN_POINT('Ctrl Pts',(5.02599225112461,23.9804048689228,12.));
#177408=CARTESIAN_POINT('Ctrl Pts',(5.01253173257458,23.9610180388271,12.));
#177409=CARTESIAN_POINT('Ctrl Pts',(4.99916972919309,23.9416710836529,12.));
#177410=CARTESIAN_POINT('Ctrl Pts',(4.98590631986532,23.9223646794591,12.));
#177411=CARTESIAN_POINT('Ctrl Pts',(4.97274158279228,23.9030995086164,12.));
#177412=CARTESIAN_POINT('Ctrl Pts',(4.95967559546565,23.883876259922,12.));
#177413=CARTESIAN_POINT('Ctrl Pts',(4.94670843465868,23.8646956287172,12.));
#177414=CARTESIAN_POINT('Ctrl Pts',(4.93384017643441,23.8455583170062,12.));
#177415=CARTESIAN_POINT('Ctrl Pts',(4.92107089613976,23.8264650335721,12.));
#177416=CARTESIAN_POINT('Ctrl Pts',(4.90840066839346,23.8074164940897,12.));
#177417=CARTESIAN_POINT('Ctrl Pts',(4.89582956706771,23.7884134212381,12.));
#177418=CARTESIAN_POINT('Ctrl Pts',(4.88335766525565,23.7694565448044,12.));
#177419=CARTESIAN_POINT('Ctrl Pts',(4.87098503527142,23.7505466018239,12.));
#177420=CARTESIAN_POINT('Ctrl Pts',(4.85871174865491,23.7316843367308,12.));
#177421=CARTESIAN_POINT('Ctrl Pts',(4.84653787616422,23.7128705015014,12.));
#177422=CARTESIAN_POINT('Ctrl Pts',(4.83446348776267,23.6941058557971,12.));
#177423=CARTESIAN_POINT('Ctrl Pts',(4.82248865259569,23.6753911671023,12.));
#177424=CARTESIAN_POINT('Ctrl Pts',(4.81061343896442,23.6567272108631,12.));
#177425=CARTESIAN_POINT('Ctrl Pts',(4.79883791433229,23.6381147706581,12.));
#177426=CARTESIAN_POINT('Ctrl Pts',(4.78716214532104,23.6195546383625,12.));
#177427=CARTESIAN_POINT('Ctrl Pts',(4.77558619769875,23.6010476143099,12.));
#177428=CARTESIAN_POINT('Ctrl Pts',(4.7641101363625,23.5825945074535,12.));
#177429=CARTESIAN_POINT('Ctrl Pts',(4.75273402530615,23.564196135517,12.));
#177430=CARTESIAN_POINT('Ctrl Pts',(4.74145792760698,23.5458533251715,12.));
#177431=CARTESIAN_POINT('Ctrl Pts',(4.73028190543031,23.5275669122378,12.));
#177432=CARTESIAN_POINT('Ctrl Pts',(4.71920602001904,23.5093377418784,12.));
#177433=CARTESIAN_POINT('Ctrl Pts',(4.7082303316782,23.491166668789,12.));
#177434=CARTESIAN_POINT('Ctrl Pts',(4.69735489975023,23.4730545573849,12.));
#177435=CARTESIAN_POINT('Ctrl Pts',(4.68657978258297,23.4550022819853,12.));
#177436=CARTESIAN_POINT('Ctrl Pts',(4.6759050375305,23.4370107270444,12.));
#177437=CARTESIAN_POINT('Ctrl Pts',(4.66533072094663,23.4190807873798,12.));
#177438=CARTESIAN_POINT('Ctrl Pts',(4.65485688816921,23.4012133683957,12.));
#177439=CARTESIAN_POINT('Ctrl Pts',(4.64448359349935,23.383409386307,12.));
#177440=CARTESIAN_POINT('Ctrl Pts',(4.63421089016554,23.3656697683496,12.));
#177441=CARTESIAN_POINT('Ctrl Pts',(4.62403883030823,23.3479954530281,12.));
#177442=CARTESIAN_POINT('Ctrl Pts',(4.61396746497848,23.3303873903947,12.));
#177443=CARTESIAN_POINT('Ctrl Pts',(4.60399684412174,23.3128465423119,12.));
#177444=CARTESIAN_POINT('Ctrl Pts',(4.59412701655749,23.295373882719,12.));
#177445=CARTESIAN_POINT('Ctrl Pts',(4.58435802994674,23.2779703978868,12.));
#177446=CARTESIAN_POINT('Ctrl Pts',(4.5746899307607,23.2606370866853,12.));
#177447=CARTESIAN_POINT('Ctrl Pts',(4.5651227642781,23.2433749609117,12.));
#177448=CARTESIAN_POINT('Ctrl Pts',(4.55565657456956,23.2261850456055,12.));
#177449=CARTESIAN_POINT('Ctrl Pts',(4.54629140447542,23.2090683793627,12.));
#177450=CARTESIAN_POINT('Ctrl Pts',(4.53702729557585,23.1920260146474,12.));
#177451=CARTESIAN_POINT('Ctrl Pts',(4.52786428815047,23.1750590180923,12.));
#177452=CARTESIAN_POINT('Ctrl Pts',(4.51880242116785,23.1581684708778,12.));
#177453=CARTESIAN_POINT('Ctrl Pts',(4.50984173227087,23.1413554691136,12.));
#177454=CARTESIAN_POINT('Ctrl Pts',(4.50098225775178,23.1246211242117,12.));
#177455=CARTESIAN_POINT('Ctrl Pts',(4.49222403252201,23.1079665632629,12.));
#177456=CARTESIAN_POINT('Ctrl Pts',(4.48356709006756,23.0913929293909,12.));
#177457=CARTESIAN_POINT('Ctrl Pts',(4.47501146242821,23.0749013821868,12.));
#177458=CARTESIAN_POINT('Ctrl Pts',(4.46655718018205,23.0584930981723,12.));
#177459=CARTESIAN_POINT('Ctrl Pts',(4.45820427241676,23.0421692712466,12.));
#177460=CARTESIAN_POINT('Ctrl Pts',(4.44995276669698,23.0259311131395,12.));
#177461=CARTESIAN_POINT('Ctrl Pts',(4.44180268901666,23.0097798538399,12.));
#177462=CARTESIAN_POINT('Ctrl Pts',(4.43375406376904,22.9937167421009,12.));
#177463=CARTESIAN_POINT('Ctrl Pts',(4.42580691372771,22.9777430460021,12.));
#177464=CARTESIAN_POINT('Ctrl Pts',(4.41796126001309,22.9618600534866,12.));
#177465=CARTESIAN_POINT('Ctrl Pts',(4.41021712205547,22.9460690729093,12.));
#177466=CARTESIAN_POINT('Ctrl Pts',(4.40257451754307,22.9303714335549,12.));
#177467=CARTESIAN_POINT('Ctrl Pts',(4.39503346238454,22.9147684862425,12.));
#177468=CARTESIAN_POINT('Ctrl Pts',(4.38759397068391,22.8992616040108,12.));
#177469=CARTESIAN_POINT('Ctrl Pts',(4.38025605470089,22.8838521827702,12.));
#177470=CARTESIAN_POINT('Ctrl Pts',(4.37301972480752,22.8685416419725,12.));
#177471=CARTESIAN_POINT('Ctrl Pts',(4.36588498943009,22.8533314252419,12.));
#177472=CARTESIAN_POINT('Ctrl Pts',(4.35885185500559,22.838223001118,12.));
#177473=CARTESIAN_POINT('Ctrl Pts',(4.35192032594801,22.8232178638873,12.));
#177474=CARTESIAN_POINT('Ctrl Pts',(4.34509040460065,22.808317534379,12.));
#177475=CARTESIAN_POINT('Ctrl Pts',(4.33836209118442,22.7935235607807,12.));
#177476=CARTESIAN_POINT('Ctrl Pts',(4.33173538373182,22.7788375194081,12.));
#177477=CARTESIAN_POINT('Ctrl Pts',(4.32521027803747,22.764261015648,12.));
#177478=CARTESIAN_POINT('Ctrl Pts',(4.3187867676123,22.7497956849852,12.));
#177479=CARTESIAN_POINT('Ctrl Pts',(4.3124648436255,22.7354431939927,12.));
#177480=CARTESIAN_POINT('Ctrl Pts',(4.30624449484074,22.7212052413384,12.));
#177481=CARTESIAN_POINT('Ctrl Pts',(4.30012570754066,22.707083558756,12.));
#177482=CARTESIAN_POINT('Ctrl Pts',(4.29410846547061,22.6930799122545,12.));
#177483=CARTESIAN_POINT('Ctrl Pts',(4.28819274977766,22.6791961033537,12.));
#177484=CARTESIAN_POINT('Ctrl Pts',(4.28237853894059,22.665433970311,12.));
#177485=CARTESIAN_POINT('Ctrl Pts',(4.27666580869117,22.6517953893303,12.));
#177486=CARTESIAN_POINT('Ctrl Pts',(4.27105453192999,22.6382822758171,12.));
#177487=CARTESIAN_POINT('Ctrl Pts',(4.26554467865571,22.6248965859975,12.));
#177488=CARTESIAN_POINT('Ctrl Pts',(4.26013621588303,22.611640318482,12.));
#177489=CARTESIAN_POINT('Ctrl Pts',(4.25482910755485,22.5985155158637,12.));
#177490=CARTESIAN_POINT('Ctrl Pts',(4.24962331444184,22.5855242662479,12.));
#177491=CARTESIAN_POINT('Ctrl Pts',(4.24451879404858,22.5726687049922,12.));
#177492=CARTESIAN_POINT('Ctrl Pts',(4.23951550052526,22.559951016643,12.));
#177493=CARTESIAN_POINT('Ctrl Pts',(4.23461338456713,22.5473734368086,12.));
#177494=CARTESIAN_POINT('Ctrl Pts',(4.22981239330731,22.5349382540587,12.));
#177495=CARTESIAN_POINT('Ctrl Pts',(4.2251124702004,22.5226478117885,12.));
#177496=CARTESIAN_POINT('Ctrl Pts',(4.22051355490196,22.5105045108882,12.));
#177497=CARTESIAN_POINT('Ctrl Pts',(4.21601558313908,22.4985108124229,12.));
#177498=CARTESIAN_POINT('Ctrl Pts',(4.21161848657428,22.4866692403147,12.));
#177499=CARTESIAN_POINT('Ctrl Pts',(4.20732219265648,22.4749823839915,12.));
#177500=CARTESIAN_POINT('Ctrl Pts',(4.2031266244817,22.4634529011433,12.));
#177501=CARTESIAN_POINT('Ctrl Pts',(4.19903170066354,22.4520835205419,12.));
#177502=CARTESIAN_POINT('Ctrl Pts',(4.1950373351886,22.4408770448917,12.));
#177503=CARTESIAN_POINT('Ctrl Pts',(4.19114343726941,22.4298363535421,12.));
#177504=CARTESIAN_POINT('Ctrl Pts',(4.1873499111772,22.4189644056115,12.));
#177505=CARTESIAN_POINT('Ctrl Pts',(4.1836566560085,22.4082642454453,12.));
#177506=CARTESIAN_POINT('Ctrl Pts',(4.18006356544882,22.3977390078075,12.));
#177507=CARTESIAN_POINT('Ctrl Pts',(4.17657052752825,22.3873919231334,12.));
#177508=CARTESIAN_POINT('Ctrl Pts',(4.17317742436145,22.3772263228617,12.));
#177509=CARTESIAN_POINT('Ctrl Pts',(4.16988413199457,22.36724564276,12.));
#177510=CARTESIAN_POINT('Ctrl Pts',(4.166690520266,22.3574534257396,12.));
#177511=CARTESIAN_POINT('Ctrl Pts',(4.16359645263187,22.3478533253889,12.));
#177512=CARTESIAN_POINT('Ctrl Pts',(4.16060178604164,22.3384491078602,12.));
#177513=CARTESIAN_POINT('Ctrl Pts',(4.15770637047889,22.3292446628959,12.));
#177514=CARTESIAN_POINT('Ctrl Pts',(4.15491004835281,22.3202440186979,12.));
#177515=CARTESIAN_POINT('Ctrl Pts',(4.1522126539699,22.3114513545185,12.));
#177516=CARTESIAN_POINT('Ctrl Pts',(4.14961401285522,22.3028710166933,12.));
#177517=CARTESIAN_POINT('Ctrl Pts',(4.14711394168556,22.2945075198467,12.));
#177518=CARTESIAN_POINT('Ctrl Pts',(4.14471224859295,22.2863655389166,12.));
#177519=CARTESIAN_POINT('Ctrl Pts',(4.14240873321984,22.2784499072027,12.));
#177520=CARTESIAN_POINT('Ctrl Pts',(4.14020318715991,22.2707656042457,12.));
#177521=CARTESIAN_POINT('Ctrl Pts',(4.13809539255421,22.2633177913972,12.));
#177522=CARTESIAN_POINT('Ctrl Pts',(4.13608511977225,22.2561118708421,12.));
#177523=CARTESIAN_POINT('Ctrl Pts',(4.1341721255881,22.249153531779,12.));
#177524=CARTESIAN_POINT('Ctrl Pts',(4.1323561506016,22.2424488153523,12.));
#177525=CARTESIAN_POINT('Ctrl Pts',(4.13063692157498,22.2360040565533,12.));
#177526=CARTESIAN_POINT('Ctrl Pts',(4.12901415463379,22.2298258043947,12.));
#177527=CARTESIAN_POINT('Ctrl Pts',(4.12748755830104,22.2239207458781,12.));
#177528=CARTESIAN_POINT('Ctrl Pts',(4.12605683613307,22.2182956401341,12.));
#177529=CARTESIAN_POINT('Ctrl Pts',(4.12472167516607,22.2129576146671,12.));
#177530=CARTESIAN_POINT('Ctrl Pts',(4.12348173702023,22.2079143941719,12.));
#177531=CARTESIAN_POINT('Ctrl Pts',(4.12233664408227,22.2031746532106,12.));
#177532=CARTESIAN_POINT('Ctrl Pts',(4.12128598183522,22.1987479618246,12.));
#177533=CARTESIAN_POINT('Ctrl Pts',(4.12032932637736,22.1946440958098,12.));
#177534=CARTESIAN_POINT('Ctrl Pts',(4.11946626228636,22.1908725908525,12.));
#177535=CARTESIAN_POINT('Ctrl Pts',(4.11869641271773,22.1874419861496,12.));
#177536=CARTESIAN_POINT('Ctrl Pts',(4.11801938107479,22.1843613164855,12.));
#177537=CARTESIAN_POINT('Ctrl Pts',(4.11743469691756,22.1816414985788,12.));
#177538=CARTESIAN_POINT('Ctrl Pts',(4.11694173195003,22.179297473024,12.));
#177539=CARTESIAN_POINT('Ctrl Pts',(4.11653973150518,22.177347426894,12.));
#177540=CARTESIAN_POINT('Ctrl Pts',(4.11622797217068,22.1758088296598,12.));
#177541=CARTESIAN_POINT('Ctrl Pts',(4.11600589882845,22.1746949858775,12.));
#177542=CARTESIAN_POINT('Ctrl Pts',(4.11589976826166,22.1741488021234,12.));
#177543=CARTESIAN_POINT('Ctrl Pts',(4.11586035878287,22.1739341411687,12.));
#177544=CARTESIAN_POINT('Ctrl Pts',(4.11585194677442,22.173877682324,12.));
#177545=CARTESIAN_POINT('Ctrl Pts',(4.11585220600461,22.1738711152697,12.));
#177546=CARTESIAN_POINT('',(4.01396149767429,21.624941921198,12.));
#177547=CARTESIAN_POINT('',(1.96187429785751,10.5694630535049,12.));
#177548=CARTESIAN_POINT('',(3.44230496120419,21.2226420728916,12.));
#177549=CARTESIAN_POINT('Origin',(3.52235856495312,21.7161918885402,12.));
#177550=CARTESIAN_POINT('',(2.16781269186828,21.3904321633055,12.));
#177551=CARTESIAN_POINT('Origin',(1.31973449697531E-13,7.6920903736728E-13,
12.));
#177552=CARTESIAN_POINT('',(1.71975774210842,21.9269795755927,12.));
#177553=CARTESIAN_POINT('Origin',(2.21822694051638,21.8878840740801,12.));
#177554=CARTESIAN_POINT('',(1.7634122053118,22.4835757167854,12.));
#177555=CARTESIAN_POINT('',(0.881706102655883,11.2417878583927,12.));
#177556=CARTESIAN_POINT('',(0.661312440730901,25.991588367311,12.));
#177557=CARTESIAN_POINT('Ctrl Pts',(1.7634122053118,22.4835757167854,12.));
#177558=CARTESIAN_POINT('Ctrl Pts',(1.7634141553879,22.4835819929788,12.));
#177559=CARTESIAN_POINT('Ctrl Pts',(1.76342064263637,22.4836387052228,12.));
#177560=CARTESIAN_POINT('Ctrl Pts',(1.76343813434659,22.4838562517064,12.));
#177561=CARTESIAN_POINT('Ctrl Pts',(1.76347698284861,22.4844112933125,12.));
#177562=CARTESIAN_POINT('Ctrl Pts',(1.76355076045549,22.4855446605991,12.));
#177563=CARTESIAN_POINT('Ctrl Pts',(1.76364784232925,22.4871115206572,12.));
#177564=CARTESIAN_POINT('Ctrl Pts',(1.76376424879468,22.4890991659479,12.));
#177565=CARTESIAN_POINT('Ctrl Pts',(1.76389475965714,22.4914909094908,12.));
#177566=CARTESIAN_POINT('Ctrl Pts',(1.76403393880316,22.4942693792449,12.));
#177567=CARTESIAN_POINT('Ctrl Pts',(1.76417731243483,22.4974203063191,12.));
#177568=CARTESIAN_POINT('Ctrl Pts',(1.76432160068737,22.5009332677316,12.));
#177569=CARTESIAN_POINT('Ctrl Pts',(1.76446408210364,22.5047996391978,12.));
#177570=CARTESIAN_POINT('Ctrl Pts',(1.76460218257313,22.5090112700212,12.));
#177571=CARTESIAN_POINT('Ctrl Pts',(1.76473303281149,22.5135590569554,12.));
#177572=CARTESIAN_POINT('Ctrl Pts',(1.76485369319895,22.5184336670207,12.));
#177573=CARTESIAN_POINT('Ctrl Pts',(1.76496128643375,22.5236259635515,12.));
#177574=CARTESIAN_POINT('Ctrl Pts',(1.76505320262759,22.529127665298,12.));
#177575=CARTESIAN_POINT('Ctrl Pts',(1.76512711563254,22.5349313983571,12.));
#177576=CARTESIAN_POINT('Ctrl Pts',(1.76518087841493,22.5410303590892,12.));
#177577=CARTESIAN_POINT('Ctrl Pts',(1.76521245524047,22.5474180954006,12.));
#177578=CARTESIAN_POINT('Ctrl Pts',(1.76521983384062,22.5540882235837,12.));
#177579=CARTESIAN_POINT('Ctrl Pts',(1.7652010450045,22.5610344912501,12.));
#177580=CARTESIAN_POINT('Ctrl Pts',(1.76515418518831,22.5682508499873,12.));
#177581=CARTESIAN_POINT('Ctrl Pts',(1.76507744026746,22.5757315316353,12.));
#177582=CARTESIAN_POINT('Ctrl Pts',(1.76496910283088,22.5834711038022,12.));
#177583=CARTESIAN_POINT('Ctrl Pts',(1.76482755288411,22.5914644078106,12.));
#177584=CARTESIAN_POINT('Ctrl Pts',(1.76465124413557,22.5997065145638,12.));
#177585=CARTESIAN_POINT('Ctrl Pts',(1.76443868648015,22.6081926681343,12.));
#177586=CARTESIAN_POINT('Ctrl Pts',(1.76418843543739,22.6169182517694,12.));
#177587=CARTESIAN_POINT('Ctrl Pts',(1.76389909571403,22.6258787994848,12.));
#177588=CARTESIAN_POINT('Ctrl Pts',(1.76356932176273,22.6350699979359,12.));
#177589=CARTESIAN_POINT('Ctrl Pts',(1.76319782013916,22.6444876940423,12.));
#177590=CARTESIAN_POINT('Ctrl Pts',(1.76278334912561,22.6541278938409,12.));
#177591=CARTESIAN_POINT('Ctrl Pts',(1.76232471392568,22.6639867471753,12.));
#177592=CARTESIAN_POINT('Ctrl Pts',(1.76182076289525,22.67406053567,12.));
#177593=CARTESIAN_POINT('Ctrl Pts',(1.76127038310614,22.684345658525,12.));
#177594=CARTESIAN_POINT('Ctrl Pts',(1.76067249704886,22.6948386219851,12.));
#177595=CARTESIAN_POINT('Ctrl Pts',(1.76002606202401,22.7055360375485,12.));
#177596=CARTESIAN_POINT('Ctrl Pts',(1.75933006905925,22.7164346186006,12.));
#177597=CARTESIAN_POINT('Ctrl Pts',(1.75858354204633,22.72753117773,12.));
#177598=CARTESIAN_POINT('Ctrl Pts',(1.75778553673244,22.7388226235559,12.));
#177599=CARTESIAN_POINT('Ctrl Pts',(1.75693513908907,22.750305955645,12.));
#177600=CARTESIAN_POINT('Ctrl Pts',(1.75603146371641,22.7619782595013,12.));
#177601=CARTESIAN_POINT('Ctrl Pts',(1.75507365227131,22.7738367016118,12.));
#177602=CARTESIAN_POINT('Ctrl Pts',(1.75406087182936,22.7858785242361,12.));
#177603=CARTESIAN_POINT('Ctrl Pts',(1.75299231391466,22.7981010424314,12.));
#177604=CARTESIAN_POINT('Ctrl Pts',(1.75186719365592,22.8105016414713,12.));
#177605=CARTESIAN_POINT('Ctrl Pts',(1.75068474890883,22.8230777741284,12.));
#177606=CARTESIAN_POINT('Ctrl Pts',(1.74944423940115,22.8358269579853,12.));
#177607=CARTESIAN_POINT('Ctrl Pts',(1.74814494588492,22.8487467728076,12.));
#177608=CARTESIAN_POINT('Ctrl Pts',(1.74678616930664,22.8618348580235,12.));
#177609=CARTESIAN_POINT('Ctrl Pts',(1.74536722998201,22.8750889101696,12.));
#177610=CARTESIAN_POINT('Ctrl Pts',(1.74388746677702,22.888506680335,12.));
#177611=CARTESIAN_POINT('Ctrl Pts',(1.7423462363008,22.9020859716141,12.));
#177612=CARTESIAN_POINT('Ctrl Pts',(1.74074291231058,22.9158246373363,12.));
#177613=CARTESIAN_POINT('Ctrl Pts',(1.73907688511666,22.9297205792586,12.));
#177614=CARTESIAN_POINT('Ctrl Pts',(1.73734756100039,22.9437717457826,12.));
#177615=CARTESIAN_POINT('Ctrl Pts',(1.73555436162769,22.9579761301063,12.));
#177616=CARTESIAN_POINT('Ctrl Pts',(1.73369672350814,22.9723317685688,12.));
#177617=CARTESIAN_POINT('Ctrl Pts',(1.7317740975019,22.9868367391978,12.));
#177618=CARTESIAN_POINT('Ctrl Pts',(1.72978594832136,23.001489160189,12.));
#177619=CARTESIAN_POINT('Ctrl Pts',(1.72773175404708,23.0162871884168,12.));
#177620=CARTESIAN_POINT('Ctrl Pts',(1.72561100564045,23.0312290178883,12.));
#177621=CARTESIAN_POINT('Ctrl Pts',(1.72342320653746,23.0463128785531,12.));
#177622=CARTESIAN_POINT('Ctrl Pts',(1.72116787225991,23.0615370351562,12.));
#177623=CARTESIAN_POINT('Ctrl Pts',(1.71884453003027,23.0768997860709,12.));
#177624=CARTESIAN_POINT('Ctrl Pts',(1.71645271839296,23.0923994621213,12.));
#177625=CARTESIAN_POINT('Ctrl Pts',(1.71399198684704,23.1080344254286,12.));
#177626=CARTESIAN_POINT('Ctrl Pts',(1.71146189552174,23.1238030684925,12.));
#177627=CARTESIAN_POINT('Ctrl Pts',(1.70886201485452,23.1397038132356,12.));
#177628=CARTESIAN_POINT('Ctrl Pts',(1.70619192527852,23.1557351100614,12.));
#177629=CARTESIAN_POINT('Ctrl Pts',(1.70345121691276,23.1718954368751,12.));
#177630=CARTESIAN_POINT('Ctrl Pts',(1.7006394892701,23.1881832981851,12.));
#177631=CARTESIAN_POINT('Ctrl Pts',(1.69775635099443,23.2045972243767,12.));
#177632=CARTESIAN_POINT('Ctrl Pts',(1.69480141959953,23.2211357709374,12.));
#177633=CARTESIAN_POINT('Ctrl Pts',(1.69177432121711,23.2377975177013,12.));
#177634=CARTESIAN_POINT('Ctrl Pts',(1.68867469034896,23.2545810680537,12.));
#177635=CARTESIAN_POINT('Ctrl Pts',(1.68550216963258,23.2714850482246,12.));
#177636=CARTESIAN_POINT('Ctrl Pts',(1.68225640962168,23.2885081066951,12.));
#177637=CARTESIAN_POINT('Ctrl Pts',(1.67893706857117,23.3056489135611,12.));
#177638=CARTESIAN_POINT('Ctrl Pts',(1.67554381222994,23.3229061599145,12.));
#177639=CARTESIAN_POINT('Ctrl Pts',(1.67207631363921,23.3402785571865,12.));
#177640=CARTESIAN_POINT('Ctrl Pts',(1.66853425293995,23.3577648365744,12.));
#177641=CARTESIAN_POINT('Ctrl Pts',(1.66491731718876,23.3753637485545,12.));
#177642=CARTESIAN_POINT('Ctrl Pts',(1.66122520018011,23.3930740623619,12.));
#177643=CARTESIAN_POINT('Ctrl Pts',(1.65745760227505,23.4108945654805,12.));
#177644=CARTESIAN_POINT('Ctrl Pts',(1.65361423023728,23.4288240631043,12.));
#177645=CARTESIAN_POINT('Ctrl Pts',(1.6496947970734,23.4468613776574,12.));
#177646=CARTESIAN_POINT('Ctrl Pts',(1.64569902187611,23.4650053483932,12.));
#177647=CARTESIAN_POINT('Ctrl Pts',(1.64162662967528,23.4832548309645,12.));
#177648=CARTESIAN_POINT('Ctrl Pts',(1.63747735129474,23.5016086970003,12.));
#177649=CARTESIAN_POINT('Ctrl Pts',(1.63325092321725,23.5200658336612,12.));
#177650=CARTESIAN_POINT('Ctrl Pts',(1.62894708745223,23.538625143226,12.));
#177651=CARTESIAN_POINT('Ctrl Pts',(1.62456559140064,23.5572855427601,12.));
#177652=CARTESIAN_POINT('Ctrl Pts',(1.62010618772866,23.57604596376,12.));
#177653=CARTESIAN_POINT('Ctrl Pts',(1.61556863424698,23.5949053517997,12.));
#177654=CARTESIAN_POINT('Ctrl Pts',(1.61095269379778,23.6138626661653,12.));
#177655=CARTESIAN_POINT('Ctrl Pts',(1.60625813414672,23.6329168794929,12.));
#177656=CARTESIAN_POINT('Ctrl Pts',(1.60148472786595,23.6520669774876,12.));
#177657=CARTESIAN_POINT('Ctrl Pts',(1.59663225222463,23.671311958631,12.));
#177658=CARTESIAN_POINT('Ctrl Pts',(1.59170048908633,23.6906508338833,12.));
#177659=CARTESIAN_POINT('Ctrl Pts',(1.58668922481221,23.710082626383,12.));
#177660=CARTESIAN_POINT('Ctrl Pts',(1.58159825017358,23.72960637113,12.));
#177661=CARTESIAN_POINT('Ctrl Pts',(1.57642736025246,23.749221114736,12.));
#177662=CARTESIAN_POINT('Ctrl Pts',(1.57117635434408,23.7689259151862,12.));
#177663=CARTESIAN_POINT('Ctrl Pts',(1.56584503586843,23.7887198415878,12.));
#177664=CARTESIAN_POINT('Ctrl Pts',(1.56043321228633,23.8086019739194,12.));
#177665=CARTESIAN_POINT('Ctrl Pts',(1.55494069502635,23.8285714027636,12.));
#177666=CARTESIAN_POINT('Ctrl Pts',(1.54936729940541,23.8486272290705,12.));
#177667=CARTESIAN_POINT('Ctrl Pts',(1.5437128445399,23.8687685639642,12.));
#177668=CARTESIAN_POINT('Ctrl Pts',(1.53797715326758,23.8889945285318,12.));
#177669=CARTESIAN_POINT('Ctrl Pts',(1.53216005207463,23.9093042536119,12.));
#177670=CARTESIAN_POINT('Ctrl Pts',(1.52626137103032,23.9296968795757,12.));
#177671=CARTESIAN_POINT('Ctrl Pts',(1.52028094372792,23.9501715561033,12.));
#177672=CARTESIAN_POINT('Ctrl Pts',(1.51421860720614,23.970727442014,12.));
#177673=CARTESIAN_POINT('Ctrl Pts',(1.50807420187694,23.9913637050927,12.));
#177674=CARTESIAN_POINT('Ctrl Pts',(1.50184757146098,24.0120795219086,12.));
#177675=CARTESIAN_POINT('Ctrl Pts',(1.49553856292801,24.0328740776331,12.));
#177676=CARTESIAN_POINT('Ctrl Pts',(1.48914702644887,24.0537465658429,12.));
#177677=CARTESIAN_POINT('Ctrl Pts',(1.48267281533683,24.0746961883528,12.));
#177678=CARTESIAN_POINT('Ctrl Pts',(1.47611578597742,24.0957221550778,12.));
#177679=CARTESIAN_POINT('Ctrl Pts',(1.46947579776991,24.1168236838824,12.));
#177680=CARTESIAN_POINT('Ctrl Pts',(1.46275271307397,24.1380000004272,12.));
#177681=CARTESIAN_POINT('Ctrl Pts',(1.45594639716317,24.1592503380107,12.));
#177682=CARTESIAN_POINT('Ctrl Pts',(1.44905671818727,24.1805739374038,12.));
#177683=CARTESIAN_POINT('Ctrl Pts',(1.44208354711082,24.201970046722,12.));
#177684=CARTESIAN_POINT('Ctrl Pts',(1.43502675765508,24.2234379212984,12.));
#177685=CARTESIAN_POINT('Ctrl Pts',(1.42788622624854,24.2449768235488,12.));
#177686=CARTESIAN_POINT('Ctrl Pts',(1.42066183198252,24.2665860228356,12.));
#177687=CARTESIAN_POINT('Ctrl Pts',(1.41335345657682,24.288264795321,12.));
#177688=CARTESIAN_POINT('Ctrl Pts',(1.40596098434337,24.3100124238311,12.));
#177689=CARTESIAN_POINT('Ctrl Pts',(1.39848430212807,24.3318281977643,12.));
#177690=CARTESIAN_POINT('Ctrl Pts',(1.39092329926388,24.3537114129875,12.));
#177691=CARTESIAN_POINT('Ctrl Pts',(1.38327786752998,24.3756613717299,12.));
#177692=CARTESIAN_POINT('Ctrl Pts',(1.37554790111609,24.3976773824732,12.));
#177693=CARTESIAN_POINT('Ctrl Pts',(1.36773329659956,24.4197587598337,12.));
#177694=CARTESIAN_POINT('Ctrl Pts',(1.35983395290627,24.4419048244523,12.));
#177695=CARTESIAN_POINT('Ctrl Pts',(1.35184977125648,24.4641149028892,12.));
#177696=CARTESIAN_POINT('Ctrl Pts',(1.34378065512337,24.4863883275134,12.));
#177697=CARTESIAN_POINT('Ctrl Pts',(1.33562651019686,24.5087244363856,12.));
#177698=CARTESIAN_POINT('Ctrl Pts',(1.32738724435326,24.5311225731435,12.));
#177699=CARTESIAN_POINT('Ctrl Pts',(1.31906276763668,24.5535820868674,12.));
#177700=CARTESIAN_POINT('Ctrl Pts',(1.31065299222021,24.5761023320183,12.));
#177701=CARTESIAN_POINT('Ctrl Pts',(1.30215783236362,24.5986826684027,12.));
#177702=CARTESIAN_POINT('Ctrl Pts',(1.29357720438107,24.6213224611229,12.));
#177703=CARTESIAN_POINT('Ctrl Pts',(1.28491102661514,24.6440210805278,12.));
#177704=CARTESIAN_POINT('Ctrl Pts',(1.27615921941642,24.666777902156,12.));
#177705=CARTESIAN_POINT('Ctrl Pts',(1.267321705135,24.6895923066836,12.));
#177706=CARTESIAN_POINT('Ctrl Pts',(1.25839840807418,24.7124636797894,12.));
#177707=CARTESIAN_POINT('Ctrl Pts',(1.24938925444325,24.7353914120011,12.));
#177708=CARTESIAN_POINT('Ctrl Pts',(1.24029417231989,24.7583748985438,12.));
#177709=CARTESIAN_POINT('Ctrl Pts',(1.23111309161843,24.7814135391799,12.));
#177710=CARTESIAN_POINT('Ctrl Pts',(1.22184594406528,24.8045067380536,12.));
#177711=CARTESIAN_POINT('Ctrl Pts',(1.21249266318208,24.8276539035092,12.));
#177712=CARTESIAN_POINT('Ctrl Pts',(1.2030531842602,24.8508544481974,12.));
#177713=CARTESIAN_POINT('Ctrl Pts',(1.19352744434064,24.8741077892075,12.));
#177714=CARTESIAN_POINT('Ctrl Pts',(1.18391538220103,24.8974133481829,12.));
#177715=CARTESIAN_POINT('Ctrl Pts',(1.17421693835041,24.9207705514449,12.));
#177716=CARTESIAN_POINT('Ctrl Pts',(1.16443205502849,24.9441788300932,12.));
#177717=CARTESIAN_POINT('Ctrl Pts',(1.15456067621889,24.9676376201502,12.));
#177718=CARTESIAN_POINT('Ctrl Pts',(1.144602747582,24.9911463621433,12.));
#177719=CARTESIAN_POINT('Ctrl Pts',(1.1345582163853,25.0147045006196,12.));
#177720=CARTESIAN_POINT('Ctrl Pts',(1.12442703144451,25.0383114836899,12.));
#177721=CARTESIAN_POINT('Ctrl Pts',(1.11420914306889,25.0619667625336,12.));
#177722=CARTESIAN_POINT('Ctrl Pts',(1.10390450301745,25.0856697909679,12.));
#177723=CARTESIAN_POINT('Ctrl Pts',(1.09351306445308,25.1094200248446,12.));
#177724=CARTESIAN_POINT('Ctrl Pts',(1.08303478197187,25.1332169227413,12.));
#177725=CARTESIAN_POINT('Ctrl Pts',(1.07246961165475,25.157059946931,12.));
#177726=CARTESIAN_POINT('Ctrl Pts',(1.06181751111768,25.1809485642192,12.));
#177727=CARTESIAN_POINT('Ctrl Pts',(1.05107843957931,25.2048822469028,12.));
#177728=CARTESIAN_POINT('Ctrl Pts',(1.04025235791507,25.2288604735086,12.));
#177729=CARTESIAN_POINT('Ctrl Pts',(1.02933922876806,25.2528827300422,12.));
#177730=CARTESIAN_POINT('Ctrl Pts',(1.01833901642237,25.276948508726,12.));
#177731=CARTESIAN_POINT('Ctrl Pts',(1.00725168656896,25.3010573055547,12.));
#177732=CARTESIAN_POINT('Ctrl Pts',(0.996077206120624,25.3252086182968,
12.));
#177733=CARTESIAN_POINT('Ctrl Pts',(0.984815543003973,25.3494019441441,
12.));
#177734=CARTESIAN_POINT('Ctrl Pts',(0.973466666000163,25.3736367778845,
12.));
#177735=CARTESIAN_POINT('Ctrl Pts',(0.962030544503142,25.3979126089163,
12.));
#177736=CARTESIAN_POINT('Ctrl Pts',(0.950507148597468,25.4222289223167,
12.));
#177737=CARTESIAN_POINT('Ctrl Pts',(0.938896449496192,25.4465852044849,
12.));
#177738=CARTESIAN_POINT('Ctrl Pts',(0.927198419886094,25.4709809475009,
12.));
#177739=CARTESIAN_POINT('Ctrl Pts',(0.915413034335613,25.4954156541795,
12.));
#177740=CARTESIAN_POINT('Ctrl Pts',(0.903540269651106,25.5198888424194,
12.));
#177741=CARTESIAN_POINT('Ctrl Pts',(0.89158010534904,25.5444000508211,12.));
#177742=CARTESIAN_POINT('Ctrl Pts',(0.879532523834294,25.5689488408156,
12.));
#177743=CARTESIAN_POINT('Ctrl Pts',(0.867397509338431,25.5935347843585,
12.));
#177744=CARTESIAN_POINT('Ctrl Pts',(0.855175047036549,25.6181574536049,
12.));
#177745=CARTESIAN_POINT('Ctrl Pts',(0.842865122120758,25.6428164100055,
12.));
#177746=CARTESIAN_POINT('Ctrl Pts',(0.830467718864205,25.6675111931952,
12.));
#177747=CARTESIAN_POINT('Ctrl Pts',(0.817982819787464,25.6922413110194,
12.));
#177748=CARTESIAN_POINT('Ctrl Pts',(0.805410404554352,25.7170062262525,
12.));
#177749=CARTESIAN_POINT('Ctrl Pts',(0.792750451616127,25.7418053757746,
12.));
#177750=CARTESIAN_POINT('Ctrl Pts',(0.780002940291965,25.7666381946955,
12.));
#177751=CARTESIAN_POINT('Ctrl Pts',(0.767167852651168,25.7915041383376,
12.));
#177752=CARTESIAN_POINT('Ctrl Pts',(0.754245175609524,25.8164027059984,
12.));
#177753=CARTESIAN_POINT('Ctrl Pts',(0.741234902663807,25.8413334619055,
12.));
#177754=CARTESIAN_POINT('Ctrl Pts',(0.728137036482335,25.8662960624185,
12.));
#177755=CARTESIAN_POINT('Ctrl Pts',(0.714951588527638,25.891290261497,12.));
#177756=CARTESIAN_POINT('Ctrl Pts',(0.701678575228756,25.9163158909426,
12.));
#177757=CARTESIAN_POINT('Ctrl Pts',(0.688318015057729,25.9413728471909,
12.));
#177758=CARTESIAN_POINT('Ctrl Pts',(0.677559543209725,25.9614434297919,
12.));
#177759=CARTESIAN_POINT('Ctrl Pts',(0.669451306780825,25.9765104298071,
12.));
#177760=CARTESIAN_POINT('Ctrl Pts',(0.664028313187627,25.9865613464773,
12.));
#177761=CARTESIAN_POINT('Ctrl Pts',(0.661312440730901,25.991588367311,12.));
#177762=CARTESIAN_POINT('',(-0.661312440730891,25.991588367311,12.));
#177763=CARTESIAN_POINT('Origin',(0.,0.,12.));
#177764=CARTESIAN_POINT('',(-1.76341220531179,22.4835757167854,12.));
#177765=CARTESIAN_POINT('Ctrl Pts',(-0.661312440730891,25.991588367311,
12.));
#177766=CARTESIAN_POINT('Ctrl Pts',(-0.664028313188914,25.9865613464809,
12.));
#177767=CARTESIAN_POINT('Ctrl Pts',(-0.669451306784418,25.9765104298171,
12.));
#177768=CARTESIAN_POINT('Ctrl Pts',(-0.677559543215903,25.9614434298092,
12.));
#177769=CARTESIAN_POINT('Ctrl Pts',(-0.688318015065679,25.941372847213,
12.));
#177770=CARTESIAN_POINT('Ctrl Pts',(-0.701678575236603,25.9163158909645,
12.));
#177771=CARTESIAN_POINT('Ctrl Pts',(-0.714951588533753,25.8912902615141,
12.));
#177772=CARTESIAN_POINT('Ctrl Pts',(-0.728137036485879,25.8662960624285,
12.));
#177773=CARTESIAN_POINT('Ctrl Pts',(-0.741234902664698,25.841333461908,
12.));
#177774=CARTESIAN_POINT('Ctrl Pts',(-0.75424517560829,25.816402705995,12.));
#177775=CARTESIAN_POINT('Ctrl Pts',(-0.767167852648641,25.7915041383304,
12.));
#177776=CARTESIAN_POINT('Ctrl Pts',(-0.780002940289027,25.7666381946871,
12.));
#177777=CARTESIAN_POINT('Ctrl Pts',(-0.792750451613536,25.7418053757671,
12.));
#177778=CARTESIAN_POINT('Ctrl Pts',(-0.805410404552596,25.7170062262474,
12.));
#177779=CARTESIAN_POINT('Ctrl Pts',(-0.81798281978672,25.6922413110172,
12.));
#177780=CARTESIAN_POINT('Ctrl Pts',(-0.830467718864369,25.6675111931957,
12.));
#177781=CARTESIAN_POINT('Ctrl Pts',(-0.842865122121547,25.6428164100078,
12.));
#177782=CARTESIAN_POINT('Ctrl Pts',(-0.855175047037615,25.618157453608,
12.));
#177783=CARTESIAN_POINT('Ctrl Pts',(-0.86739750933947,25.5935347843616,
12.));
#177784=CARTESIAN_POINT('Ctrl Pts',(-0.879532523835092,25.568948840818,
12.));
#177785=CARTESIAN_POINT('Ctrl Pts',(-0.891580105349468,25.5444000508223,
12.));
#177786=CARTESIAN_POINT('Ctrl Pts',(-0.903540269651155,25.5198888424195,
12.));
#177787=CARTESIAN_POINT('Ctrl Pts',(-0.915413034335334,25.4954156541787,
12.));
#177788=CARTESIAN_POINT('Ctrl Pts',(-0.927198419885605,25.4709809474996,
12.));
#177789=CARTESIAN_POINT('Ctrl Pts',(-0.938896449495633,25.4465852044835,
12.));
#177790=CARTESIAN_POINT('Ctrl Pts',(-0.95050714859697,25.4222289223155,
12.));
#177791=CARTESIAN_POINT('Ctrl Pts',(-0.962030544502803,25.3979126089155,
12.));
#177792=CARTESIAN_POINT('Ctrl Pts',(-0.973466666000049,25.3736367778842,
12.));
#177793=CARTESIAN_POINT('Ctrl Pts',(-0.984815543004092,25.3494019441444,
12.));
#177794=CARTESIAN_POINT('Ctrl Pts',(-0.99607720612092,25.3252086182976,
12.));
#177795=CARTESIAN_POINT('Ctrl Pts',(-1.00725168656934,25.3010573055557,
12.));
#177796=CARTESIAN_POINT('Ctrl Pts',(-1.01833901642272,25.2769485087268,
12.));
#177797=CARTESIAN_POINT('Ctrl Pts',(-1.0293392287683,25.2528827300427,12.));
#177798=CARTESIAN_POINT('Ctrl Pts',(-1.04025235791515,25.2288604735087,
12.));
#177799=CARTESIAN_POINT('Ctrl Pts',(-1.05107843957926,25.2048822469027,
12.));
#177800=CARTESIAN_POINT('Ctrl Pts',(-1.06181751111754,25.1809485642191,
12.));
#177801=CARTESIAN_POINT('Ctrl Pts',(-1.0724696116546,25.1570599469311,12.));
#177802=CARTESIAN_POINT('Ctrl Pts',(-1.08303478197174,25.1332169227415,
12.));
#177803=CARTESIAN_POINT('Ctrl Pts',(-1.09351306445299,25.1094200248448,
12.));
#177804=CARTESIAN_POINT('Ctrl Pts',(-1.1039045030174,25.085669790968,12.));
#177805=CARTESIAN_POINT('Ctrl Pts',(-1.1142091430689,25.0619667625336,12.));
#177806=CARTESIAN_POINT('Ctrl Pts',(-1.12442703144455,25.0383114836898,
12.));
#177807=CARTESIAN_POINT('Ctrl Pts',(-1.13455821638536,25.0147045006193,
12.));
#177808=CARTESIAN_POINT('Ctrl Pts',(-1.14460274758206,24.9911463621431,
12.));
#177809=CARTESIAN_POINT('Ctrl Pts',(-1.15456067621894,24.9676376201501,
12.));
#177810=CARTESIAN_POINT('Ctrl Pts',(-1.16443205502852,24.9441788300932,
12.));
#177811=CARTESIAN_POINT('Ctrl Pts',(-1.17421693835039,24.9207705514449,
12.));
#177812=CARTESIAN_POINT('Ctrl Pts',(-1.18391538220098,24.8974133481829,
12.));
#177813=CARTESIAN_POINT('Ctrl Pts',(-1.19352744434059,24.8741077892074,
12.));
#177814=CARTESIAN_POINT('Ctrl Pts',(-1.20305318426015,24.8508544481973,
12.));
#177815=CARTESIAN_POINT('Ctrl Pts',(-1.21249266318205,24.8276539035092,
12.));
#177816=CARTESIAN_POINT('Ctrl Pts',(-1.22184594406526,24.8045067380536,
12.));
#177817=CARTESIAN_POINT('Ctrl Pts',(-1.23111309161843,24.78141353918,12.));
#177818=CARTESIAN_POINT('Ctrl Pts',(-1.24029417231988,24.7583748985439,
12.));
#177819=CARTESIAN_POINT('Ctrl Pts',(-1.24938925444324,24.7353914120012,
12.));
#177820=CARTESIAN_POINT('Ctrl Pts',(-1.25839840807415,24.7124636797895,
12.));
#177821=CARTESIAN_POINT('Ctrl Pts',(-1.26732170513497,24.6895923066837,
12.));
#177822=CARTESIAN_POINT('Ctrl Pts',(-1.2761592194164,24.666777902156,12.));
#177823=CARTESIAN_POINT('Ctrl Pts',(-1.28491102661514,24.6440210805278,
12.));
#177824=CARTESIAN_POINT('Ctrl Pts',(-1.29357720438108,24.6213224611228,
12.));
#177825=CARTESIAN_POINT('Ctrl Pts',(-1.30215783236364,24.5986826684025,
12.));
#177826=CARTESIAN_POINT('Ctrl Pts',(-1.31065299222023,24.576102332018,12.));
#177827=CARTESIAN_POINT('Ctrl Pts',(-1.31906276763669,24.5535820868671,
12.));
#177828=CARTESIAN_POINT('Ctrl Pts',(-1.32738724435326,24.5311225731434,
12.));
#177829=CARTESIAN_POINT('Ctrl Pts',(-1.33562651019684,24.5087244363856,
12.));
#177830=CARTESIAN_POINT('Ctrl Pts',(-1.34378065512335,24.4863883275135,
12.));
#177831=CARTESIAN_POINT('Ctrl Pts',(-1.35184977125645,24.4641149028894,
12.));
#177832=CARTESIAN_POINT('Ctrl Pts',(-1.35983395290624,24.4419048244524,
12.));
#177833=CARTESIAN_POINT('Ctrl Pts',(-1.36773329659954,24.4197587598337,
12.));
#177834=CARTESIAN_POINT('Ctrl Pts',(-1.37554790111608,24.3976773824731,
12.));
#177835=CARTESIAN_POINT('Ctrl Pts',(-1.38327786752998,24.37566137173,12.));
#177836=CARTESIAN_POINT('Ctrl Pts',(-1.3909232992639,24.3537114129877,12.));
#177837=CARTESIAN_POINT('Ctrl Pts',(-1.3984843021281,24.3318281977647,12.));
#177838=CARTESIAN_POINT('Ctrl Pts',(-1.40596098434341,24.3100124238316,
12.));
#177839=CARTESIAN_POINT('Ctrl Pts',(-1.41335345657685,24.2882647953214,
12.));
#177840=CARTESIAN_POINT('Ctrl Pts',(-1.42066183198252,24.2665860228357,
12.));
#177841=CARTESIAN_POINT('Ctrl Pts',(-1.42788622624851,24.2449768235485,
12.));
#177842=CARTESIAN_POINT('Ctrl Pts',(-1.43502675765502,24.2234379212978,
12.));
#177843=CARTESIAN_POINT('Ctrl Pts',(-1.44208354711074,24.2019700467214,
12.));
#177844=CARTESIAN_POINT('Ctrl Pts',(-1.44905671818721,24.1805739374033,
12.));
#177845=CARTESIAN_POINT('Ctrl Pts',(-1.45594639716314,24.1592503380105,
12.));
#177846=CARTESIAN_POINT('Ctrl Pts',(-1.46275271307398,24.1380000004272,
12.));
#177847=CARTESIAN_POINT('Ctrl Pts',(-1.46947579776992,24.1168236838827,
12.));
#177848=CARTESIAN_POINT('Ctrl Pts',(-1.47611578597741,24.0957221550782,
12.));
#177849=CARTESIAN_POINT('Ctrl Pts',(-1.4826728153368,24.074696188353,12.));
#177850=CARTESIAN_POINT('Ctrl Pts',(-1.48914702644883,24.053746565843,12.));
#177851=CARTESIAN_POINT('Ctrl Pts',(-1.49553856292798,24.0328740776331,
12.));
#177852=CARTESIAN_POINT('Ctrl Pts',(-1.50184757146099,24.0120795219086,
12.));
#177853=CARTESIAN_POINT('Ctrl Pts',(-1.50807420187703,23.991363705093,12.));
#177854=CARTESIAN_POINT('Ctrl Pts',(-1.51421860720628,23.9707274420145,
12.));
#177855=CARTESIAN_POINT('Ctrl Pts',(-1.52028094372806,23.9501715561038,
12.));
#177856=CARTESIAN_POINT('Ctrl Pts',(-1.5262613710304,23.9296968795761,12.));
#177857=CARTESIAN_POINT('Ctrl Pts',(-1.53216005207462,23.9093042536119,
12.));
#177858=CARTESIAN_POINT('Ctrl Pts',(-1.53797715326748,23.8889945285313,
12.));
#177859=CARTESIAN_POINT('Ctrl Pts',(-1.54371284453978,23.8687685639635,
12.));
#177860=CARTESIAN_POINT('Ctrl Pts',(-1.5493672994053,23.8486272290698,12.));
#177861=CARTESIAN_POINT('Ctrl Pts',(-1.55494069502628,23.8285714027631,
12.));
#177862=CARTESIAN_POINT('Ctrl Pts',(-1.56043321228631,23.8086019739192,
12.));
#177863=CARTESIAN_POINT('Ctrl Pts',(-1.56584503586844,23.788719841588,12.));
#177864=CARTESIAN_POINT('Ctrl Pts',(-1.57117635434412,23.7689259151869,
12.));
#177865=CARTESIAN_POINT('Ctrl Pts',(-1.57642736025251,23.7492211147369,
12.));
#177866=CARTESIAN_POINT('Ctrl Pts',(-1.58159825017362,23.7296063711308,
12.));
#177867=CARTESIAN_POINT('Ctrl Pts',(-1.58668922481222,23.7100826263835,
12.));
#177868=CARTESIAN_POINT('Ctrl Pts',(-1.59170048908632,23.6906508338833,
12.));
#177869=CARTESIAN_POINT('Ctrl Pts',(-1.59663225222458,23.6713119586302,
12.));
#177870=CARTESIAN_POINT('Ctrl Pts',(-1.60148472786588,23.6520669774863,
12.));
#177871=CARTESIAN_POINT('Ctrl Pts',(-1.60625813414666,23.6329168794916,
12.));
#177872=CARTESIAN_POINT('Ctrl Pts',(-1.61095269379773,23.6138626661644,
12.));
#177873=CARTESIAN_POINT('Ctrl Pts',(-1.61556863424697,23.5949053517996,
12.));
#177874=CARTESIAN_POINT('Ctrl Pts',(-1.62010618772869,23.5760459637608,
12.));
#177875=CARTESIAN_POINT('Ctrl Pts',(-1.62456559140072,23.5572855427617,
12.));
#177876=CARTESIAN_POINT('Ctrl Pts',(-1.62894708745231,23.5386251432278,
12.));
#177877=CARTESIAN_POINT('Ctrl Pts',(-1.63325092321731,23.5200658336624,
12.));
#177878=CARTESIAN_POINT('Ctrl Pts',(-1.63747735129474,23.5016086970006,
12.));
#177879=CARTESIAN_POINT('Ctrl Pts',(-1.64162662967525,23.4832548309638,
12.));
#177880=CARTESIAN_POINT('Ctrl Pts',(-1.64569902187608,23.4650053483919,
12.));
#177881=CARTESIAN_POINT('Ctrl Pts',(-1.6496947970734,23.446861377656,12.));
#177882=CARTESIAN_POINT('Ctrl Pts',(-1.6536142302373,23.4288240631034,12.));
#177883=CARTESIAN_POINT('Ctrl Pts',(-1.65745760227507,23.4108945654803,
12.));
#177884=CARTESIAN_POINT('Ctrl Pts',(-1.66122520018008,23.3930740623622,
12.));
#177885=CARTESIAN_POINT('Ctrl Pts',(-1.66491731718864,23.375363748555,12.));
#177886=CARTESIAN_POINT('Ctrl Pts',(-1.66853425293978,23.3577648365747,
12.));
#177887=CARTESIAN_POINT('Ctrl Pts',(-1.67207631363905,23.3402785571866,
12.));
#177888=CARTESIAN_POINT('Ctrl Pts',(-1.67554381222987,23.3229061599145,
12.));
#177889=CARTESIAN_POINT('Ctrl Pts',(-1.67893706857123,23.3056489135611,
12.));
#177890=CARTESIAN_POINT('Ctrl Pts',(-1.68225640962181,23.2885081066949,
12.));
#177891=CARTESIAN_POINT('Ctrl Pts',(-1.68550216963275,23.2714850482245,
12.));
#177892=CARTESIAN_POINT('Ctrl Pts',(-1.6886746903491,23.2545810680536,12.));
#177893=CARTESIAN_POINT('Ctrl Pts',(-1.69177432121716,23.2377975177014,
12.));
#177894=CARTESIAN_POINT('Ctrl Pts',(-1.69480141959946,23.2211357709374,
12.));
#177895=CARTESIAN_POINT('Ctrl Pts',(-1.69775635099425,23.2045972243765,
12.));
#177896=CARTESIAN_POINT('Ctrl Pts',(-1.70063948926987,23.1881832981848,
12.));
#177897=CARTESIAN_POINT('Ctrl Pts',(-1.70345121691259,23.1718954368749,
12.));
#177898=CARTESIAN_POINT('Ctrl Pts',(-1.70619192527847,23.1557351100613,
12.));
#177899=CARTESIAN_POINT('Ctrl Pts',(-1.7088620148546,23.1397038132358,12.));
#177900=CARTESIAN_POINT('Ctrl Pts',(-1.71146189552192,23.1238030684929,
12.));
#177901=CARTESIAN_POINT('Ctrl Pts',(-1.71399198684725,23.1080344254291,
12.));
#177902=CARTESIAN_POINT('Ctrl Pts',(-1.71645271839311,23.0923994621216,
12.));
#177903=CARTESIAN_POINT('Ctrl Pts',(-1.71884453003027,23.0768997860709,
12.));
#177904=CARTESIAN_POINT('Ctrl Pts',(-1.7211678722598,23.061537035156,12.));
#177905=CARTESIAN_POINT('Ctrl Pts',(-1.72342320653731,23.0463128785528,
12.));
#177906=CARTESIAN_POINT('Ctrl Pts',(-1.72561100564033,23.031229017888,12.));
#177907=CARTESIAN_POINT('Ctrl Pts',(-1.72773175404703,23.0162871884167,
12.));
#177908=CARTESIAN_POINT('Ctrl Pts',(-1.72978594832137,23.0014891601891,
12.));
#177909=CARTESIAN_POINT('Ctrl Pts',(-1.73177409750194,22.9868367391978,
12.));
#177910=CARTESIAN_POINT('Ctrl Pts',(-1.73369672350818,22.9723317685688,
12.));
#177911=CARTESIAN_POINT('Ctrl Pts',(-1.73555436162771,22.9579761301062,
12.));
#177912=CARTESIAN_POINT('Ctrl Pts',(-1.73734756100038,22.9437717457825,
12.));
#177913=CARTESIAN_POINT('Ctrl Pts',(-1.73907688511664,22.9297205792587,
12.));
#177914=CARTESIAN_POINT('Ctrl Pts',(-1.74074291231057,22.9158246373365,
12.));
#177915=CARTESIAN_POINT('Ctrl Pts',(-1.74234623630079,22.9020859716144,
12.));
#177916=CARTESIAN_POINT('Ctrl Pts',(-1.74388746677702,22.8885066803351,
12.));
#177917=CARTESIAN_POINT('Ctrl Pts',(-1.745367229982,22.8750889101696,12.));
#177918=CARTESIAN_POINT('Ctrl Pts',(-1.74678616930663,22.8618348580234,
12.));
#177919=CARTESIAN_POINT('Ctrl Pts',(-1.74814494588492,22.8487467728075,
12.));
#177920=CARTESIAN_POINT('Ctrl Pts',(-1.74944423940117,22.8358269579854,
12.));
#177921=CARTESIAN_POINT('Ctrl Pts',(-1.75068474890884,22.8230777741285,
12.));
#177922=CARTESIAN_POINT('Ctrl Pts',(-1.7518671936559,22.8105016414712,12.));
#177923=CARTESIAN_POINT('Ctrl Pts',(-1.75299231391461,22.7981010424312,
12.));
#177924=CARTESIAN_POINT('Ctrl Pts',(-1.7540608718293,22.7858785242358,12.));
#177925=CARTESIAN_POINT('Ctrl Pts',(-1.75507365227127,22.7738367016115,
12.));
#177926=CARTESIAN_POINT('Ctrl Pts',(-1.7560314637164,22.7619782595013,12.));
#177927=CARTESIAN_POINT('Ctrl Pts',(-1.75693513908911,22.7503059556455,
12.));
#177928=CARTESIAN_POINT('Ctrl Pts',(-1.75778553673249,22.7388226235565,
12.));
#177929=CARTESIAN_POINT('Ctrl Pts',(-1.75858354204635,22.7275311777305,
12.));
#177930=CARTESIAN_POINT('Ctrl Pts',(-1.75933006905924,22.7164346186007,
12.));
#177931=CARTESIAN_POINT('Ctrl Pts',(-1.76002606202399,22.7055360375481,
12.));
#177932=CARTESIAN_POINT('Ctrl Pts',(-1.76067249704884,22.6948386219843,
12.));
#177933=CARTESIAN_POINT('Ctrl Pts',(-1.76127038310613,22.6843456585245,
12.));
#177934=CARTESIAN_POINT('Ctrl Pts',(-1.76182076289525,22.6740605356699,
12.));
#177935=CARTESIAN_POINT('Ctrl Pts',(-1.76232471392567,22.6639867471756,
12.));
#177936=CARTESIAN_POINT('Ctrl Pts',(-1.76278334912559,22.6541278938413,
12.));
#177937=CARTESIAN_POINT('Ctrl Pts',(-1.76319782013914,22.6444876940425,
12.));
#177938=CARTESIAN_POINT('Ctrl Pts',(-1.76356932176272,22.635069997936,12.));
#177939=CARTESIAN_POINT('Ctrl Pts',(-1.76389909571402,22.6258787994847,
12.));
#177940=CARTESIAN_POINT('Ctrl Pts',(-1.76418843543739,22.6169182517693,
12.));
#177941=CARTESIAN_POINT('Ctrl Pts',(-1.76443868648015,22.6081926681342,
12.));
#177942=CARTESIAN_POINT('Ctrl Pts',(-1.76465124413556,22.5997065145638,
12.));
#177943=CARTESIAN_POINT('Ctrl Pts',(-1.76482755288411,22.5914644078106,
12.));
#177944=CARTESIAN_POINT('Ctrl Pts',(-1.76496910283088,22.5834711038024,
12.));
#177945=CARTESIAN_POINT('Ctrl Pts',(-1.76507744026747,22.5757315316355,
12.));
#177946=CARTESIAN_POINT('Ctrl Pts',(-1.76515418518829,22.5682508499873,
12.));
#177947=CARTESIAN_POINT('Ctrl Pts',(-1.76520104500449,22.5610344912501,
12.));
#177948=CARTESIAN_POINT('Ctrl Pts',(-1.76521983384063,22.5540882235837,
12.));
#177949=CARTESIAN_POINT('Ctrl Pts',(-1.76521245524047,22.5474180954006,
12.));
#177950=CARTESIAN_POINT('Ctrl Pts',(-1.76518087841493,22.5410303590891,
12.));
#177951=CARTESIAN_POINT('Ctrl Pts',(-1.7651271156325,22.5349313983571,12.));
#177952=CARTESIAN_POINT('Ctrl Pts',(-1.76505320262752,22.529127665298,12.));
#177953=CARTESIAN_POINT('Ctrl Pts',(-1.76496128643369,22.5236259635515,
12.));
#177954=CARTESIAN_POINT('Ctrl Pts',(-1.76485369319896,22.5184336670207,
12.));
#177955=CARTESIAN_POINT('Ctrl Pts',(-1.76473303281159,22.5135590569554,
12.));
#177956=CARTESIAN_POINT('Ctrl Pts',(-1.76460218257323,22.5090112700212,
12.));
#177957=CARTESIAN_POINT('Ctrl Pts',(-1.76446408210366,22.5047996391978,
12.));
#177958=CARTESIAN_POINT('Ctrl Pts',(-1.76432160068725,22.5009332677316,
12.));
#177959=CARTESIAN_POINT('Ctrl Pts',(-1.76417731243462,22.4974203063191,
12.));
#177960=CARTESIAN_POINT('Ctrl Pts',(-1.76403393880301,22.4942693792449,
12.));
#177961=CARTESIAN_POINT('Ctrl Pts',(-1.76389475965724,22.4914909094908,
12.));
#177962=CARTESIAN_POINT('Ctrl Pts',(-1.76376424879505,22.4890991659478,
12.));
#177963=CARTESIAN_POINT('Ctrl Pts',(-1.76364784232963,22.4871115206571,
12.));
#177964=CARTESIAN_POINT('Ctrl Pts',(-1.76355076045546,22.4855446605991,
12.));
#177965=CARTESIAN_POINT('Ctrl Pts',(-1.76347698284792,22.4844112933129,
12.));
#177966=CARTESIAN_POINT('Ctrl Pts',(-1.76343813434565,22.483856251707,12.));
#177967=CARTESIAN_POINT('Ctrl Pts',(-1.7634206426357,22.4836387052232,12.));
#177968=CARTESIAN_POINT('Ctrl Pts',(-1.76341415538764,22.483581992979,12.));
#177969=CARTESIAN_POINT('Ctrl Pts',(-1.76341220531179,22.4835757167854,
12.));
#177970=CARTESIAN_POINT('',(-1.71975774210841,21.9269795755927,12.));
#177971=CARTESIAN_POINT('',(-0.840553282521227,10.7170877657712,12.));
#177972=CARTESIAN_POINT('',(-2.16781269186828,21.3904321633055,12.));
#177973=CARTESIAN_POINT('Origin',(-2.21822694051637,21.8878840740801,12.));
#177974=CARTESIAN_POINT('',(-3.44230496120418,21.2226420728916,12.));
#177975=CARTESIAN_POINT('Origin',(-7.16093850883226E-14,7.7715611723761E-13,
12.));
#177976=CARTESIAN_POINT('',(-4.01396149767428,21.624941921198,12.));
#177977=CARTESIAN_POINT('Origin',(-3.52235856495312,21.7161918885402,12.));
#177978=CARTESIAN_POINT('',(-4.11585220600461,22.1738711152697,12.));
#177979=CARTESIAN_POINT('',(-2.05792610300232,11.0869355576349,12.));
#177980=CARTESIAN_POINT('',(-6.08833931617698,25.2771067246846,12.));
#177981=CARTESIAN_POINT('Ctrl Pts',(-4.11585220600461,22.1738711152697,
12.));
#177982=CARTESIAN_POINT('Ctrl Pts',(-4.11585194677412,22.1738776823239,
12.));
#177983=CARTESIAN_POINT('Ctrl Pts',(-4.1158603587821,22.1739341411684,12.));
#177984=CARTESIAN_POINT('Ctrl Pts',(-4.11589976826061,22.174148802123,12.));
#177985=CARTESIAN_POINT('Ctrl Pts',(-4.11600589882767,22.1746949858773,
12.));
#177986=CARTESIAN_POINT('Ctrl Pts',(-4.11622797217066,22.1758088296598,
12.));
#177987=CARTESIAN_POINT('Ctrl Pts',(-4.11653973150558,22.177347426894,12.));
#177988=CARTESIAN_POINT('Ctrl Pts',(-4.11694173195041,22.179297473024,12.));
#177989=CARTESIAN_POINT('Ctrl Pts',(-4.11743469691765,22.1816414985788,
12.));
#177990=CARTESIAN_POINT('Ctrl Pts',(-4.11801938107464,22.1843613164855,
12.));
#177991=CARTESIAN_POINT('Ctrl Pts',(-4.11869641271752,22.1874419861496,
12.));
#177992=CARTESIAN_POINT('Ctrl Pts',(-4.11946626228623,22.1908725908525,
12.));
#177993=CARTESIAN_POINT('Ctrl Pts',(-4.12032932637738,22.1946440958098,
12.));
#177994=CARTESIAN_POINT('Ctrl Pts',(-4.12128598183533,22.1987479618246,
12.));
#177995=CARTESIAN_POINT('Ctrl Pts',(-4.12233664408237,22.2031746532106,
12.));
#177996=CARTESIAN_POINT('Ctrl Pts',(-4.12348173702025,22.2079143941719,
12.));
#177997=CARTESIAN_POINT('Ctrl Pts',(-4.12472167516602,22.2129576146671,
12.));
#177998=CARTESIAN_POINT('Ctrl Pts',(-4.126056836133,22.2182956401341,12.));
#177999=CARTESIAN_POINT('Ctrl Pts',(-4.12748755830099,22.2239207458781,
12.));
#178000=CARTESIAN_POINT('Ctrl Pts',(-4.12901415463379,22.2298258043947,
12.));
#178001=CARTESIAN_POINT('Ctrl Pts',(-4.13063692157499,22.2360040565534,
12.));
#178002=CARTESIAN_POINT('Ctrl Pts',(-4.1323561506016,22.2424488153523,12.));
#178003=CARTESIAN_POINT('Ctrl Pts',(-4.13417212558808,22.2491535317789,
12.));
#178004=CARTESIAN_POINT('Ctrl Pts',(-4.13608511977226,22.2561118708422,
12.));
#178005=CARTESIAN_POINT('Ctrl Pts',(-4.13809539255419,22.263317791397,12.));
#178006=CARTESIAN_POINT('Ctrl Pts',(-4.14020318715988,22.2707656042456,
12.));
#178007=CARTESIAN_POINT('Ctrl Pts',(-4.14240873321982,22.2784499072026,
12.));
#178008=CARTESIAN_POINT('Ctrl Pts',(-4.14471224859295,22.2863655389166,
12.));
#178009=CARTESIAN_POINT('Ctrl Pts',(-4.14711394168559,22.2945075198468,
12.));
#178010=CARTESIAN_POINT('Ctrl Pts',(-4.14961401285526,22.3028710166935,
12.));
#178011=CARTESIAN_POINT('Ctrl Pts',(-4.15221265396992,22.3114513545186,
12.));
#178012=CARTESIAN_POINT('Ctrl Pts',(-4.15491004835278,22.3202440186979,
12.));
#178013=CARTESIAN_POINT('Ctrl Pts',(-4.15770637047882,22.3292446628957,
12.));
#178014=CARTESIAN_POINT('Ctrl Pts',(-4.16060178604154,22.3384491078599,
12.));
#178015=CARTESIAN_POINT('Ctrl Pts',(-4.1635964526318,22.3478533253886,12.));
#178016=CARTESIAN_POINT('Ctrl Pts',(-4.16669052026602,22.3574534257397,
12.));
#178017=CARTESIAN_POINT('Ctrl Pts',(-4.1698841319947,22.3672456427605,12.));
#178018=CARTESIAN_POINT('Ctrl Pts',(-4.17317742436162,22.3772263228624,
12.));
#178019=CARTESIAN_POINT('Ctrl Pts',(-4.17657052752834,22.3873919231339,
12.));
#178020=CARTESIAN_POINT('Ctrl Pts',(-4.18006356544879,22.3977390078074,
12.));
#178021=CARTESIAN_POINT('Ctrl Pts',(-4.18365665600839,22.4082642454448,
12.));
#178022=CARTESIAN_POINT('Ctrl Pts',(-4.18734991117707,22.4189644056109,
12.));
#178023=CARTESIAN_POINT('Ctrl Pts',(-4.19114343726932,22.4298363535416,
12.));
#178024=CARTESIAN_POINT('Ctrl Pts',(-4.1950373351886,22.4408770448917,12.));
#178025=CARTESIAN_POINT('Ctrl Pts',(-4.19903170066358,22.4520835205422,
12.));
#178026=CARTESIAN_POINT('Ctrl Pts',(-4.20312662448174,22.4634529011437,
12.));
#178027=CARTESIAN_POINT('Ctrl Pts',(-4.20732219265649,22.4749823839917,
12.));
#178028=CARTESIAN_POINT('Ctrl Pts',(-4.21161848657428,22.4866692403147,
12.));
#178029=CARTESIAN_POINT('Ctrl Pts',(-4.21601558313906,22.4985108124228,
12.));
#178030=CARTESIAN_POINT('Ctrl Pts',(-4.22051355490196,22.5105045108881,
12.));
#178031=CARTESIAN_POINT('Ctrl Pts',(-4.22511247020041,22.5226478117886,
12.));
#178032=CARTESIAN_POINT('Ctrl Pts',(-4.22981239330733,22.5349382540588,
12.));
#178033=CARTESIAN_POINT('Ctrl Pts',(-4.23461338456712,22.5473734368086,
12.));
#178034=CARTESIAN_POINT('Ctrl Pts',(-4.23951550052523,22.5599510166429,
12.));
#178035=CARTESIAN_POINT('Ctrl Pts',(-4.24451879404851,22.572668704992,12.));
#178036=CARTESIAN_POINT('Ctrl Pts',(-4.24962331444177,22.5855242662477,
12.));
#178037=CARTESIAN_POINT('Ctrl Pts',(-4.25482910755481,22.5985155158636,
12.));
#178038=CARTESIAN_POINT('Ctrl Pts',(-4.26013621588305,22.6116403184821,
12.));
#178039=CARTESIAN_POINT('Ctrl Pts',(-4.26554467865576,22.6248965859977,
12.));
#178040=CARTESIAN_POINT('Ctrl Pts',(-4.27105453193004,22.6382822758172,
12.));
#178041=CARTESIAN_POINT('Ctrl Pts',(-4.2766658086912,22.6517953893303,12.));
#178042=CARTESIAN_POINT('Ctrl Pts',(-4.28237853894059,22.6654339703109,
12.));
#178043=CARTESIAN_POINT('Ctrl Pts',(-4.28819274977763,22.6791961033538,
12.));
#178044=CARTESIAN_POINT('Ctrl Pts',(-4.29410846547056,22.6930799122548,
12.));
#178045=CARTESIAN_POINT('Ctrl Pts',(-4.3001257075406,22.7070835587564,12.));
#178046=CARTESIAN_POINT('Ctrl Pts',(-4.30624449484069,22.7212052413386,
12.));
#178047=CARTESIAN_POINT('Ctrl Pts',(-4.31246484362549,22.7354431939926,
12.));
#178048=CARTESIAN_POINT('Ctrl Pts',(-4.31878676761235,22.7497956849848,
12.));
#178049=CARTESIAN_POINT('Ctrl Pts',(-4.32521027803754,22.7642610156475,
12.));
#178050=CARTESIAN_POINT('Ctrl Pts',(-4.3317353837319,22.7788375194076,12.));
#178051=CARTESIAN_POINT('Ctrl Pts',(-4.33836209118446,22.7935235607806,
12.));
#178052=CARTESIAN_POINT('Ctrl Pts',(-4.34509040460062,22.8083175343791,
12.));
#178053=CARTESIAN_POINT('Ctrl Pts',(-4.35192032594791,22.8232178638876,
12.));
#178054=CARTESIAN_POINT('Ctrl Pts',(-4.35885185500546,22.8382230011184,
12.));
#178055=CARTESIAN_POINT('Ctrl Pts',(-4.36588498942997,22.8533314252422,
12.));
#178056=CARTESIAN_POINT('Ctrl Pts',(-4.37301972480746,22.8685416419725,
12.));
#178057=CARTESIAN_POINT('Ctrl Pts',(-4.38025605470093,22.8838521827701,
12.));
#178058=CARTESIAN_POINT('Ctrl Pts',(-4.38759397068406,22.8992616040108,
12.));
#178059=CARTESIAN_POINT('Ctrl Pts',(-4.39503346238473,22.9147684862426,
12.));
#178060=CARTESIAN_POINT('Ctrl Pts',(-4.40257451754323,22.930371433555,12.));
#178061=CARTESIAN_POINT('Ctrl Pts',(-4.41021712205553,22.9460690729093,
12.));
#178062=CARTESIAN_POINT('Ctrl Pts',(-4.41796126001302,22.9618600534866,
12.));
#178063=CARTESIAN_POINT('Ctrl Pts',(-4.42580691372751,22.977743046002,12.));
#178064=CARTESIAN_POINT('Ctrl Pts',(-4.43375406376879,22.9937167421006,
12.));
#178065=CARTESIAN_POINT('Ctrl Pts',(-4.44180268901643,23.0097798538395,
12.));
#178066=CARTESIAN_POINT('Ctrl Pts',(-4.44995276669686,23.0259311131392,
12.));
#178067=CARTESIAN_POINT('Ctrl Pts',(-4.45820427241683,23.0421692712467,
12.));
#178068=CARTESIAN_POINT('Ctrl Pts',(-4.4665571801823,23.0584930981732,12.));
#178069=CARTESIAN_POINT('Ctrl Pts',(-4.47501146242856,23.0749013821881,
12.));
#178070=CARTESIAN_POINT('Ctrl Pts',(-4.48356709006788,23.0913929293922,
12.));
#178071=CARTESIAN_POINT('Ctrl Pts',(-4.49222403252216,23.1079665632636,
12.));
#178072=CARTESIAN_POINT('Ctrl Pts',(-4.50098225775171,23.1246211242115,
12.));
#178073=CARTESIAN_POINT('Ctrl Pts',(-4.5098417322706,23.1413554691123,12.));
#178074=CARTESIAN_POINT('Ctrl Pts',(-4.51880242116748,23.1581684708761,
12.));
#178075=CARTESIAN_POINT('Ctrl Pts',(-4.52786428815015,23.1750590180908,
12.));
#178076=CARTESIAN_POINT('Ctrl Pts',(-4.53702729557566,23.1920260146465,
12.));
#178077=CARTESIAN_POINT('Ctrl Pts',(-4.54629140447544,23.2090683793629,
12.));
#178078=CARTESIAN_POINT('Ctrl Pts',(-4.55565657456975,23.2261850456064,
12.));
#178079=CARTESIAN_POINT('Ctrl Pts',(-4.56512276427839,23.2433749609131,
12.));
#178080=CARTESIAN_POINT('Ctrl Pts',(-4.57468993076097,23.2606370866866,
12.));
#178081=CARTESIAN_POINT('Ctrl Pts',(-4.5843580299469,23.2779703978876,12.));
#178082=CARTESIAN_POINT('Ctrl Pts',(-4.5941270165575,23.2953738827191,12.));
#178083=CARTESIAN_POINT('Ctrl Pts',(-4.60399684412163,23.3128465423115,
12.));
#178084=CARTESIAN_POINT('Ctrl Pts',(-4.6139674649783,23.3303873903938,12.));
#178085=CARTESIAN_POINT('Ctrl Pts',(-4.62403883030805,23.3479954530272,
12.));
#178086=CARTESIAN_POINT('Ctrl Pts',(-4.63421089016541,23.3656697683489,
12.));
#178087=CARTESIAN_POINT('Ctrl Pts',(-4.6444835934993,23.3834093863068,12.));
#178088=CARTESIAN_POINT('Ctrl Pts',(-4.65485688816924,23.4012133683959,
12.));
#178089=CARTESIAN_POINT('Ctrl Pts',(-4.6653307209467,23.4190807873803,12.));
#178090=CARTESIAN_POINT('Ctrl Pts',(-4.67590503753058,23.4370107270451,
12.));
#178091=CARTESIAN_POINT('Ctrl Pts',(-4.68657978258303,23.455002281986,12.));
#178092=CARTESIAN_POINT('Ctrl Pts',(-4.69735489975024,23.4730545573853,
12.));
#178093=CARTESIAN_POINT('Ctrl Pts',(-4.70823033167819,23.491166668789,12.));
#178094=CARTESIAN_POINT('Ctrl Pts',(-4.71920602001902,23.509337741878,12.));
#178095=CARTESIAN_POINT('Ctrl Pts',(-4.7302819054303,23.5275669122372,12.));
#178096=CARTESIAN_POINT('Ctrl Pts',(-4.74145792760698,23.545853325171,12.));
#178097=CARTESIAN_POINT('Ctrl Pts',(-4.75273402530617,23.5641961355168,
12.));
#178098=CARTESIAN_POINT('Ctrl Pts',(-4.76411013636251,23.5825945074535,
12.));
#178099=CARTESIAN_POINT('Ctrl Pts',(-4.77558619769872,23.6010476143099,
12.));
#178100=CARTESIAN_POINT('Ctrl Pts',(-4.78716214532098,23.6195546383624,
12.));
#178101=CARTESIAN_POINT('Ctrl Pts',(-4.7988379143322,23.6381147706579,12.));
#178102=CARTESIAN_POINT('Ctrl Pts',(-4.81061343896432,23.6567272108628,
12.));
#178103=CARTESIAN_POINT('Ctrl Pts',(-4.82248865259562,23.675391167102,12.));
#178104=CARTESIAN_POINT('Ctrl Pts',(-4.83446348776266,23.6941058557971,
12.));
#178105=CARTESIAN_POINT('Ctrl Pts',(-4.84653787616425,23.7128705015017,
12.));
#178106=CARTESIAN_POINT('Ctrl Pts',(-4.85871174865499,23.7316843367313,
12.));
#178107=CARTESIAN_POINT('Ctrl Pts',(-4.87098503527152,23.7505466018245,
12.));
#178108=CARTESIAN_POINT('Ctrl Pts',(-4.88335766525573,23.7694565448049,
12.));
#178109=CARTESIAN_POINT('Ctrl Pts',(-4.89582956706775,23.7884134212384,
12.));
#178110=CARTESIAN_POINT('Ctrl Pts',(-4.90840066839344,23.8074164940896,
12.));
#178111=CARTESIAN_POINT('Ctrl Pts',(-4.92107089613969,23.8264650335717,
12.));
#178112=CARTESIAN_POINT('Ctrl Pts',(-4.93384017643432,23.8455583170057,
12.));
#178113=CARTESIAN_POINT('Ctrl Pts',(-4.9467084346586,23.8646956287168,12.));
#178114=CARTESIAN_POINT('Ctrl Pts',(-4.95967559546561,23.8838762599218,
12.));
#178115=CARTESIAN_POINT('Ctrl Pts',(-4.97274158279227,23.9030995086163,
12.));
#178116=CARTESIAN_POINT('Ctrl Pts',(-4.98590631986533,23.9223646794592,
12.));
#178117=CARTESIAN_POINT('Ctrl Pts',(-4.99916972919307,23.9416710836529,
12.));
#178118=CARTESIAN_POINT('Ctrl Pts',(-5.01253173257453,23.9610180388271,
12.));
#178119=CARTESIAN_POINT('Ctrl Pts',(-5.02599225112454,23.9804048689227,
12.));
#178120=CARTESIAN_POINT('Ctrl Pts',(-5.03955120528521,23.9998309040746,
12.));
#178121=CARTESIAN_POINT('Ctrl Pts',(-5.05320851483065,24.0192954804896,
12.));
#178122=CARTESIAN_POINT('Ctrl Pts',(-5.06696409886641,24.0387979403268,
12.));
#178123=CARTESIAN_POINT('Ctrl Pts',(-5.08081787581276,24.0583376315638,
12.));
#178124=CARTESIAN_POINT('Ctrl Pts',(-5.09476976342625,24.0779139079266,
12.));
#178125=CARTESIAN_POINT('Ctrl Pts',(-5.10881967883132,24.0975261288446,
12.));
#178126=CARTESIAN_POINT('Ctrl Pts',(-5.12296753853859,24.117173659394,12.));
#178127=CARTESIAN_POINT('Ctrl Pts',(-5.13721325845745,24.1368558702443,
12.));
#178128=CARTESIAN_POINT('Ctrl Pts',(-5.15155675390075,24.156572137597,12.));
#178129=CARTESIAN_POINT('Ctrl Pts',(-5.16599793957979,24.1763218431343,
12.));
#178130=CARTESIAN_POINT('Ctrl Pts',(-5.18053672961392,24.1961043738754,
12.));
#178131=CARTESIAN_POINT('Ctrl Pts',(-5.19517303753643,24.215919122017,12.));
#178132=CARTESIAN_POINT('Ctrl Pts',(-5.20990677629173,24.2357654847765,
12.));
#178133=CARTESIAN_POINT('Ctrl Pts',(-5.22473785822441,24.2556428642294,
12.));
#178134=CARTESIAN_POINT('Ctrl Pts',(-5.23966619506289,24.2755506671526,
12.));
#178135=CARTESIAN_POINT('Ctrl Pts',(-5.25469169788856,24.2954883048448,
12.));
#178136=CARTESIAN_POINT('Ctrl Pts',(-5.26981427718796,24.3154551932222,
12.));
#178137=CARTESIAN_POINT('Ctrl Pts',(-5.28503384290644,24.3354507529415,
12.));
#178138=CARTESIAN_POINT('Ctrl Pts',(-5.30035030449059,24.3554744095075,
12.));
#178139=CARTESIAN_POINT('Ctrl Pts',(-5.31576357092524,24.3755255933917,
12.));
#178140=CARTESIAN_POINT('Ctrl Pts',(-5.33127355076037,24.3956037401293,
12.));
#178141=CARTESIAN_POINT('Ctrl Pts',(-5.34688015213546,24.4157082904615,
12.));
#178142=CARTESIAN_POINT('Ctrl Pts',(-5.36258328273639,24.4358386899152,
12.));
#178143=CARTESIAN_POINT('Ctrl Pts',(-5.37838284973706,24.4559943883159,
12.));
#178144=CARTESIAN_POINT('Ctrl Pts',(-5.3942787597383,24.4761748393322,12.));
#178145=CARTESIAN_POINT('Ctrl Pts',(-5.41027091869242,24.4963794999831,
12.));
#178146=CARTESIAN_POINT('Ctrl Pts',(-5.42635923183411,24.5166078302107,
12.));
#178147=CARTESIAN_POINT('Ctrl Pts',(-5.44254360356865,24.5368592922861,
12.));
#178148=CARTESIAN_POINT('Ctrl Pts',(-5.45882393762244,24.5571333514841,
12.));
#178149=CARTESIAN_POINT('Ctrl Pts',(-5.47520013724403,24.5774294770329,
12.));
#178150=CARTESIAN_POINT('Ctrl Pts',(-5.49167210537235,24.5977471429365,
12.));
#178151=CARTESIAN_POINT('Ctrl Pts',(-5.50823974481959,24.618085828918,12.));
#178152=CARTESIAN_POINT('Ctrl Pts',(-5.52490295840996,24.6384450211466,
12.));
#178153=CARTESIAN_POINT('Ctrl Pts',(-5.54166164919593,24.6588242134733,
12.));
#178154=CARTESIAN_POINT('Ctrl Pts',(-5.55851572025389,24.6792229061785,
12.));
#178155=CARTESIAN_POINT('Ctrl Pts',(-5.57546507427767,24.6996406035507,
12.));
#178156=CARTESIAN_POINT('Ctrl Pts',(-5.59250961323995,24.7200768119079,
12.));
#178157=CARTESIAN_POINT('Ctrl Pts',(-5.60964923798495,24.7405310372736,
12.));
#178158=CARTESIAN_POINT('Ctrl Pts',(-5.62688384790919,24.76100278357,12.));
#178159=CARTESIAN_POINT('Ctrl Pts',(-5.64421334042248,24.7814915496728,
12.));
#178160=CARTESIAN_POINT('Ctrl Pts',(-5.66163761114903,24.8019968304618,
12.));
#178161=CARTESIAN_POINT('Ctrl Pts',(-5.67915655496524,24.822518122386,12.));
#178162=CARTESIAN_POINT('Ctrl Pts',(-5.69677006679429,24.8430549277634,
12.));
#178163=CARTESIAN_POINT('Ctrl Pts',(-5.71447804252019,24.8636067597677,
12.));
#178164=CARTESIAN_POINT('Ctrl Pts',(-5.73228037976927,24.8841731467219,
12.));
#178165=CARTESIAN_POINT('Ctrl Pts',(-5.75017697890813,24.9047536376467,
12.));
#178166=CARTESIAN_POINT('Ctrl Pts',(-5.76816774342236,24.9253478043632,
12.));
#178167=CARTESIAN_POINT('Ctrl Pts',(-5.78625257775703,24.9459552293308,
12.));
#178168=CARTESIAN_POINT('Ctrl Pts',(-5.80443138549747,24.9665754954462,
12.));
#178169=CARTESIAN_POINT('Ctrl Pts',(-5.82270406744214,24.9872081752709,
12.));
#178170=CARTESIAN_POINT('Ctrl Pts',(-5.84107051963073,25.0078528200558,
12.));
#178171=CARTESIAN_POINT('Ctrl Pts',(-5.8595306315681,25.0285089498922,12.));
#178172=CARTESIAN_POINT('Ctrl Pts',(-5.87808428385329,25.0491760405965,
12.));
#178173=CARTESIAN_POINT('Ctrl Pts',(-5.89673135155459,25.0698535426593,
12.));
#178174=CARTESIAN_POINT('Ctrl Pts',(-5.91547170844382,25.0905409050863,
12.));
#178175=CARTESIAN_POINT('Ctrl Pts',(-5.93430523086776,25.1112375971182,
12.));
#178176=CARTESIAN_POINT('Ctrl Pts',(-5.95323180187348,25.1319431317273,
12.));
#178177=CARTESIAN_POINT('Ctrl Pts',(-5.97225131495636,25.1526570863065,
12.));
#178178=CARTESIAN_POINT('Ctrl Pts',(-5.99136367859838,25.1733791296154,
12.));
#178179=CARTESIAN_POINT('Ctrl Pts',(-6.0105688180476,25.1941090269638,12.));
#178180=CARTESIAN_POINT('Ctrl Pts',(-6.02986667390187,25.2148466201368,
12.));
#178181=CARTESIAN_POINT('Ctrl Pts',(-6.04925720151412,25.2355918138798,
12.));
#178182=CARTESIAN_POINT('Ctrl Pts',(-6.06484373634697,25.2521940105523,
12.));
#178183=CARTESIAN_POINT('Ctrl Pts',(-6.07657531787578,25.2646490489816,
12.));
#178184=CARTESIAN_POINT('Ctrl Pts',(-6.08441489609824,25.2729539149479,
12.));
#178185=CARTESIAN_POINT('Ctrl Pts',(-6.08833931617698,25.2771067246846,
12.));
#178186=CARTESIAN_POINT('',(-7.36589684767344,24.9347862158358,12.));
#178187=CARTESIAN_POINT('Origin',(0.,0.,12.));
#178188=CARTESIAN_POINT('',(-7.52250298901264,21.2610617890679,12.));
#178189=CARTESIAN_POINT('Ctrl Pts',(-7.36589684767344,24.9347862158358,
12.));
#178190=CARTESIAN_POINT('Ctrl Pts',(-7.3672190902906,24.9292275670705,12.));
#178191=CARTESIAN_POINT('Ctrl Pts',(-7.36985593120696,24.9181155530631,
12.));
#178192=CARTESIAN_POINT('Ctrl Pts',(-7.37378825962718,24.9014633826201,
12.));
#178193=CARTESIAN_POINT('Ctrl Pts',(-7.3789854964161,24.8792921911309,12.));
#178194=CARTESIAN_POINT('Ctrl Pts',(-7.38540558904946,24.8516310625367,
12.));
#178195=CARTESIAN_POINT('Ctrl Pts',(-7.39174922586841,24.8240228521042,
12.));
#178196=CARTESIAN_POINT('Ctrl Pts',(-7.39801641583612,24.7964676646518,
12.));
#178197=CARTESIAN_POINT('Ctrl Pts',(-7.40420718661754,24.7689656669005,
12.));
#178198=CARTESIAN_POINT('Ctrl Pts',(-7.41032159082173,24.7415170994754,
12.));
#178199=CARTESIAN_POINT('Ctrl Pts',(-7.41635971481243,24.7141222949988,
12.));
#178200=CARTESIAN_POINT('Ctrl Pts',(-7.42232167765763,24.6867816727118,
12.));
#178201=CARTESIAN_POINT('Ctrl Pts',(-7.42820762158681,24.659495712869,12.));
#178202=CARTESIAN_POINT('Ctrl Pts',(-7.4340177048922,24.6322649369472,12.));
#178203=CARTESIAN_POINT('Ctrl Pts',(-7.43975209375375,24.6050898852349,
12.));
#178204=CARTESIAN_POINT('Ctrl Pts',(-7.44541095473163,24.5779710960865,
12.));
#178205=CARTESIAN_POINT('Ctrl Pts',(-7.45099444651296,24.5509090831579,
12.));
#178206=CARTESIAN_POINT('Ctrl Pts',(-7.45650271336045,24.52390431731,12.));
#178207=CARTESIAN_POINT('Ctrl Pts',(-7.46193588961642,24.4969572391509,
12.));
#178208=CARTESIAN_POINT('Ctrl Pts',(-7.46729410308923,24.4700682684544,
12.));
#178209=CARTESIAN_POINT('Ctrl Pts',(-7.47257747883319,24.4432378146501,
12.));
#178210=CARTESIAN_POINT('Ctrl Pts',(-7.47778614286573,24.4164662871165,
12.));
#178211=CARTESIAN_POINT('Ctrl Pts',(-7.48292022569254,24.3897541049248,
12.));
#178212=CARTESIAN_POINT('Ctrl Pts',(-7.48797986651828,24.3631017084513,
12.));
#178213=CARTESIAN_POINT('Ctrl Pts',(-7.4929652125233,24.3365095573673,12.));
#178214=CARTESIAN_POINT('Ctrl Pts',(-7.49787641695359,24.3099781253345,
12.));
#178215=CARTESIAN_POINT('Ctrl Pts',(-7.50271363765098,24.2835078958966,
12.));
#178216=CARTESIAN_POINT('Ctrl Pts',(-7.50747703535115,24.2570993577032,
12.));
#178217=CARTESIAN_POINT('Ctrl Pts',(-7.51216677222199,24.230753000389,12.));
#178218=CARTESIAN_POINT('Ctrl Pts',(-7.51678300997998,24.2044693092356,
12.));
#178219=CARTESIAN_POINT('Ctrl Pts',(-7.52132590953862,24.1782487641602,
12.));
#178220=CARTESIAN_POINT('Ctrl Pts',(-7.52579563201479,24.152091842537,12.));
#178221=CARTESIAN_POINT('Ctrl Pts',(-7.53019233935536,24.1259990209211,
12.));
#178222=CARTESIAN_POINT('Ctrl Pts',(-7.53451619514658,24.0999707772643,
12.));
#178223=CARTESIAN_POINT('Ctrl Pts',(-7.53876736531005,24.0740075927984,
12.));
#178224=CARTESIAN_POINT('Ctrl Pts',(-7.54294601896128,24.0481099543353,
12.));
#178225=CARTESIAN_POINT('Ctrl Pts',(-7.54705232885895,24.0222783554531,
12.));
#178226=CARTESIAN_POINT('Ctrl Pts',(-7.55108647097432,23.9965132953187,
12.));
#178227=CARTESIAN_POINT('Ctrl Pts',(-7.55504862424808,23.9708152779886,
12.));
#178228=CARTESIAN_POINT('Ctrl Pts',(-7.5589389702768,23.9451848115002,12.));
#178229=CARTESIAN_POINT('Ctrl Pts',(-7.56275769304773,23.9196224070759,
12.));
#178230=CARTESIAN_POINT('Ctrl Pts',(-7.56650497863791,23.8941285782002,
12.));
#178231=CARTESIAN_POINT('Ctrl Pts',(-7.57018101500709,23.8687038399595,
12.));
#178232=CARTESIAN_POINT('Ctrl Pts',(-7.57378599219814,23.8433487096132,
12.));
#178233=CARTESIAN_POINT('Ctrl Pts',(-7.57732010249066,23.8180637069976,
12.));
#178234=CARTESIAN_POINT('Ctrl Pts',(-7.58078354058213,23.7928493549908,
12.));
#178235=CARTESIAN_POINT('Ctrl Pts',(-7.58417650376271,23.7677061799376,
12.));
#178236=CARTESIAN_POINT('Ctrl Pts',(-7.58749919210826,23.7426347121006,
12.));
#178237=CARTESIAN_POINT('Ctrl Pts',(-7.5907518086532,23.7176354860456,12.));
#178238=CARTESIAN_POINT('Ctrl Pts',(-7.59393455934035,23.6927090405066,
12.));
#178239=CARTESIAN_POINT('Ctrl Pts',(-7.59704765299567,23.6678559182875,
12.));
#178240=CARTESIAN_POINT('Ctrl Pts',(-7.60009130130126,23.6430766661418,
12.));
#178241=CARTESIAN_POINT('Ctrl Pts',(-7.60306571877806,23.6183718346576,
12.));
#178242=CARTESIAN_POINT('Ctrl Pts',(-7.60597112277094,23.5937419781245,
12.));
#178243=CARTESIAN_POINT('Ctrl Pts',(-7.608807733446,23.5691876544244,12.));
#178244=CARTESIAN_POINT('Ctrl Pts',(-7.61157577385372,23.544709425203,12.));
#178245=CARTESIAN_POINT('Ctrl Pts',(-7.61427546999298,23.5203078560129,
12.));
#178246=CARTESIAN_POINT('Ctrl Pts',(-7.61690705088319,23.4959835164609,
12.));
#178247=CARTESIAN_POINT('Ctrl Pts',(-7.61947074863977,23.4717369803438,
12.));
#178248=CARTESIAN_POINT('Ctrl Pts',(-7.62196679855955,23.4475688257854,
12.));
#178249=CARTESIAN_POINT('Ctrl Pts',(-7.6243954392005,23.4234796353542,12.));
#178250=CARTESIAN_POINT('Ctrl Pts',(-7.62675691240329,23.399469996112,12.));
#178251=CARTESIAN_POINT('Ctrl Pts',(-7.62905146332593,23.3755404996636,
12.));
#178252=CARTESIAN_POINT('Ctrl Pts',(-7.63127934048136,23.3516917421972,
12.));
#178253=CARTESIAN_POINT('Ctrl Pts',(-7.63344079578161,23.3279243245241,
12.));
#178254=CARTESIAN_POINT('Ctrl Pts',(-7.63553608458783,23.3042388521022,
12.));
#178255=CARTESIAN_POINT('Ctrl Pts',(-7.63756546576374,23.2806359350855,
12.));
#178256=CARTESIAN_POINT('Ctrl Pts',(-7.63952920172835,23.2571161884488,
12.));
#178257=CARTESIAN_POINT('Ctrl Pts',(-7.64142755851504,23.2336802320912,
12.));
#178258=CARTESIAN_POINT('Ctrl Pts',(-7.6432608058368,23.2103286909398,12.));
#178259=CARTESIAN_POINT('Ctrl Pts',(-7.64502921715483,23.1870621950452,
12.));
#178260=CARTESIAN_POINT('Ctrl Pts',(-7.64673306975805,23.1638813796694,
12.));
#178261=CARTESIAN_POINT('Ctrl Pts',(-7.64837264482943,23.1407868853819,
12.));
#178262=CARTESIAN_POINT('Ctrl Pts',(-7.6499482274986,23.1177793581679,12.));
#178263=CARTESIAN_POINT('Ctrl Pts',(-7.65146010690476,23.094859449525,12.));
#178264=CARTESIAN_POINT('Ctrl Pts',(-7.65290857626358,23.072027816555,12.));
#178265=CARTESIAN_POINT('Ctrl Pts',(-7.65429393293946,23.0492851220528,
12.));
#178266=CARTESIAN_POINT('Ctrl Pts',(-7.65561647852534,23.0266320345787,
12.));
#178267=CARTESIAN_POINT('Ctrl Pts',(-7.65687651891304,23.0040692285814,
12.));
#178268=CARTESIAN_POINT('Ctrl Pts',(-7.65807436436432,22.9815973845296,
12.));
#178269=CARTESIAN_POINT('Ctrl Pts',(-7.65921032958902,22.959217189033,12.));
#178270=CARTESIAN_POINT('Ctrl Pts',(-7.66028473382778,22.9369293349593,
12.));
#178271=CARTESIAN_POINT('Ctrl Pts',(-7.66129790094108,22.9147345215421,
12.));
#178272=CARTESIAN_POINT('Ctrl Pts',(-7.66225015950156,22.8926334544883,
12.));
#178273=CARTESIAN_POINT('Ctrl Pts',(-7.66314184287337,22.8706268461283,
12.));
#178274=CARTESIAN_POINT('Ctrl Pts',(-7.66397328929803,22.848715415557,12.));
#178275=CARTESIAN_POINT('Ctrl Pts',(-7.66474484198549,22.8268998887678,
12.));
#178276=CARTESIAN_POINT('Ctrl Pts',(-7.66545684920987,22.8051809987833,
12.));
#178277=CARTESIAN_POINT('Ctrl Pts',(-7.66610966441273,22.7835594857699,
12.));
#178278=CARTESIAN_POINT('Ctrl Pts',(-7.66670364630299,22.7620360971843,
12.));
#178279=CARTESIAN_POINT('Ctrl Pts',(-7.6672391589544,22.7406115879513,12.));
#178280=CARTESIAN_POINT('Ctrl Pts',(-7.66771657191027,22.7192867206245,
12.));
#178281=CARTESIAN_POINT('Ctrl Pts',(-7.66813626029275,22.6980622655446,
12.));
#178282=CARTESIAN_POINT('Ctrl Pts',(-7.66849860491743,22.6769390009885,
12.));
#178283=CARTESIAN_POINT('Ctrl Pts',(-7.66880399241323,22.6559177133127,
12.));
#178284=CARTESIAN_POINT('Ctrl Pts',(-7.66905281533715,22.6349991971541,
12.));
#178285=CARTESIAN_POINT('Ctrl Pts',(-7.66924547229414,22.6141842556243,
12.));
#178286=CARTESIAN_POINT('Ctrl Pts',(-7.66938236806233,22.5934737004953,
12.));
#178287=CARTESIAN_POINT('Ctrl Pts',(-7.66946391372306,22.5728683523831,
12.));
#178288=CARTESIAN_POINT('Ctrl Pts',(-7.66949052679693,22.5523690409116,
12.));
#178289=CARTESIAN_POINT('Ctrl Pts',(-7.66946263138144,22.53197660492,12.));
#178290=CARTESIAN_POINT('Ctrl Pts',(-7.66938065829108,22.5116918927031,
12.));
#178291=CARTESIAN_POINT('Ctrl Pts',(-7.66924504520315,22.4915157622312,
12.));
#178292=CARTESIAN_POINT('Ctrl Pts',(-7.66905623680831,22.47144908137,12.));
#178293=CARTESIAN_POINT('Ctrl Pts',(-7.66881468496635,22.4514927280855,
12.));
#178294=CARTESIAN_POINT('Ctrl Pts',(-7.66852084886704,22.4316475906603,
12.));
#178295=CARTESIAN_POINT('Ctrl Pts',(-7.6681751951964,22.4119145679758,12.));
#178296=CARTESIAN_POINT('Ctrl Pts',(-7.6677781983079,22.3922945697773,12.));
#178297=CARTESIAN_POINT('Ctrl Pts',(-7.66733034039883,22.372788516936,12.));
#178298=CARTESIAN_POINT('Ctrl Pts',(-7.66683211169158,22.3533973417021,
12.));
#178299=CARTESIAN_POINT('Ctrl Pts',(-7.66628401061952,22.3341219879469,
12.));
#178300=CARTESIAN_POINT('Ctrl Pts',(-7.66568654402494,22.314963411484,12.));
#178301=CARTESIAN_POINT('Ctrl Pts',(-7.66504022736299,22.2959225803937,
12.));
#178302=CARTESIAN_POINT('Ctrl Pts',(-7.66434558490979,22.2770004753335,
12.));
#178303=CARTESIAN_POINT('Ctrl Pts',(-7.66360314997641,22.258198089848,12.));
#178304=CARTESIAN_POINT('Ctrl Pts',(-7.66281346512509,22.2395164306547,
12.));
#178305=CARTESIAN_POINT('Ctrl Pts',(-7.661977082404,22.2209565180085,12.));
#178306=CARTESIAN_POINT('Ctrl Pts',(-7.66109456359271,22.2025193860964,
12.));
#178307=CARTESIAN_POINT('Ctrl Pts',(-7.66016648045005,22.1842060834091,
12.));
#178308=CARTESIAN_POINT('Ctrl Pts',(-7.6591934149693,22.1660176731178,12.));
#178309=CARTESIAN_POINT('Ctrl Pts',(-7.65817595963349,22.1479552334211,
12.));
#178310=CARTESIAN_POINT('Ctrl Pts',(-7.65711471769397,22.1300198579675,
12.));
#178311=CARTESIAN_POINT('Ctrl Pts',(-7.65601030346807,22.1122126563329,
12.));
#178312=CARTESIAN_POINT('Ctrl Pts',(-7.65486334263644,22.094534754469,12.));
#178313=CARTESIAN_POINT('Ctrl Pts',(-7.65367447254949,22.0769872951596,
12.));
#178314=CARTESIAN_POINT('Ctrl Pts',(-7.65244434253113,22.0595714384431,
12.));
#178315=CARTESIAN_POINT('Ctrl Pts',(-7.65117361421358,22.0422883621174,
12.));
#178316=CARTESIAN_POINT('Ctrl Pts',(-7.64986296190168,22.0251392623209,
12.));
#178317=CARTESIAN_POINT('Ctrl Pts',(-7.64851307293352,22.0081253540774,
12.));
#178318=CARTESIAN_POINT('Ctrl Pts',(-7.6471246480525,21.9912478718542,12.));
#178319=CARTESIAN_POINT('Ctrl Pts',(-7.64569840177336,21.9745080700798,
12.));
#178320=CARTESIAN_POINT('Ctrl Pts',(-7.64423506279123,21.9579072237651,
12.));
#178321=CARTESIAN_POINT('Ctrl Pts',(-7.64273537442682,21.9414466292072,
12.));
#178322=CARTESIAN_POINT('Ctrl Pts',(-7.64120009506532,21.9251276046546,
12.));
#178323=CARTESIAN_POINT('Ctrl Pts',(-7.63962999860927,21.9089514909874,
12.));
#178324=CARTESIAN_POINT('Ctrl Pts',(-7.63802587492035,21.8929196523514,
12.));
#178325=CARTESIAN_POINT('Ctrl Pts',(-7.636388530334,21.8770334769496,12.));
#178326=CARTESIAN_POINT('Ctrl Pts',(-7.63471878821226,21.8612943779089,
12.));
#178327=CARTESIAN_POINT('Ctrl Pts',(-7.63301748948936,21.8457037941084,
12.));
#178328=CARTESIAN_POINT('Ctrl Pts',(-7.63128549323023,21.8302631910195,
12.));
#178329=CARTESIAN_POINT('Ctrl Pts',(-7.62952367718127,21.814974061509,12.));
#178330=CARTESIAN_POINT('Ctrl Pts',(-7.62773293842389,21.799837926858,12.));
#178331=CARTESIAN_POINT('Ctrl Pts',(-7.62591419404512,21.7848563378021,
12.));
#178332=CARTESIAN_POINT('Ctrl Pts',(-7.62406838181166,21.7700308755584,
12.));
#178333=CARTESIAN_POINT('Ctrl Pts',(-7.62219646084228,21.7553631528328,
12.));
#178334=CARTESIAN_POINT('Ctrl Pts',(-7.62029941230855,21.7408548148656,
12.));
#178335=CARTESIAN_POINT('Ctrl Pts',(-7.61837824030538,21.7265075407975,
12.));
#178336=CARTESIAN_POINT('Ctrl Pts',(-7.61643397270421,21.7123230449834,
12.));
#178337=CARTESIAN_POINT('Ctrl Pts',(-7.61446766202787,21.6983030783322,
12.));
#178338=CARTESIAN_POINT('Ctrl Pts',(-7.61248038630268,21.6844494295815,
12.));
#178339=CARTESIAN_POINT('Ctrl Pts',(-7.61047325000956,21.6707639267576,
12.));
#178340=CARTESIAN_POINT('Ctrl Pts',(-7.60844738512874,21.6572484388081,
12.));
#178341=CARTESIAN_POINT('Ctrl Pts',(-7.60640395216357,21.6439048771743,
12.));
#178342=CARTESIAN_POINT('Ctrl Pts',(-7.60434414118296,21.6307351973822,
12.));
#178343=CARTESIAN_POINT('Ctrl Pts',(-7.60226917285429,21.617741400599,12.));
#178344=CARTESIAN_POINT('Ctrl Pts',(-7.60018029988241,21.6049255358843,
12.));
#178345=CARTESIAN_POINT('Ctrl Pts',(-7.59807880846195,21.5922897024466,
12.));
#178346=CARTESIAN_POINT('Ctrl Pts',(-7.59596601973584,21.5798360518978,
12.));
#178347=CARTESIAN_POINT('Ctrl Pts',(-7.59384329124918,21.5675667904726,
12.));
#178348=CARTESIAN_POINT('Ctrl Pts',(-7.59171201844777,21.5554841813462,
12.));
#178349=CARTESIAN_POINT('Ctrl Pts',(-7.58957363620014,21.543590547011,12.));
#178350=CARTESIAN_POINT('Ctrl Pts',(-7.58742962034834,21.5318882716736,
12.));
#178351=CARTESIAN_POINT('Ctrl Pts',(-7.5852814891913,21.5203798035299,12.));
#178352=CARTESIAN_POINT('Ctrl Pts',(-7.5831308051918,21.5090676573873,12.));
#178353=CARTESIAN_POINT('Ctrl Pts',(-7.58097917790744,21.4979544192744,
12.));
#178354=CARTESIAN_POINT('Ctrl Pts',(-7.57882826679132,21.4870427508194,
12.));
#178355=CARTESIAN_POINT('Ctrl Pts',(-7.57667978402987,21.4763353936762,
12.));
#178356=CARTESIAN_POINT('Ctrl Pts',(-7.57453549743412,21.4658351740128,
12.));
#178357=CARTESIAN_POINT('Ctrl Pts',(-7.57239723223506,21.4555450053142,
12.));
#178358=CARTESIAN_POINT('Ctrl Pts',(-7.57026687261166,21.4454678907509,
12.));
#178359=CARTESIAN_POINT('Ctrl Pts',(-7.56814636360847,21.4356069261513,
12.));
#178360=CARTESIAN_POINT('Ctrl Pts',(-7.56603771218712,21.4259653015736,
12.));
#178361=CARTESIAN_POINT('Ctrl Pts',(-7.56394299313685,21.4165463106254,
12.));
#178362=CARTESIAN_POINT('Ctrl Pts',(-7.56186435703622,21.4073533630365,
12.));
#178363=CARTESIAN_POINT('Ctrl Pts',(-7.55980403700611,21.3983899952987,
12.));
#178364=CARTESIAN_POINT('Ctrl Pts',(-7.55776435731417,21.3896598842117,
12.));
#178365=CARTESIAN_POINT('Ctrl Pts',(-7.55574773403503,21.3811668478932,
12.));
#178366=CARTESIAN_POINT('Ctrl Pts',(-7.55375667080029,21.3729148390243,
12.));
#178367=CARTESIAN_POINT('Ctrl Pts',(-7.55179375777444,21.3649079431865,
12.));
#178368=CARTESIAN_POINT('Ctrl Pts',(-7.5498616652131,21.3571503685855,12.));
#178369=CARTESIAN_POINT('Ctrl Pts',(-7.5479631624633,21.3496464761531,12.));
#178370=CARTESIAN_POINT('Ctrl Pts',(-7.54610114948347,21.3424008295038,
12.));
#178371=CARTESIAN_POINT('Ctrl Pts',(-7.54427868151268,21.3354182340149,
12.));
#178372=CARTESIAN_POINT('Ctrl Pts',(-7.54249900377031,21.328703791771,12.));
#178373=CARTESIAN_POINT('Ctrl Pts',(-7.54076552038279,21.3222628524165,
12.));
#178374=CARTESIAN_POINT('Ctrl Pts',(-7.53908175169898,21.3161009456256,
12.));
#178375=CARTESIAN_POINT('Ctrl Pts',(-7.53745129364616,21.310223716773,12.));
#178376=CARTESIAN_POINT('Ctrl Pts',(-7.53587778251736,21.3046368712157,
12.));
#178377=CARTESIAN_POINT('Ctrl Pts',(-7.53436505309943,21.2993464250717,
12.));
#178378=CARTESIAN_POINT('Ctrl Pts',(-7.53291726078527,21.2943588989331,
12.));
#178379=CARTESIAN_POINT('Ctrl Pts',(-7.53153906987855,21.2896816163842,
12.));
#178380=CARTESIAN_POINT('Ctrl Pts',(-7.53023562438229,21.2853226580657,
12.));
#178381=CARTESIAN_POINT('Ctrl Pts',(-7.52901217930408,21.2812902781143,
12.));
#178382=CARTESIAN_POINT('Ctrl Pts',(-7.52787386225333,21.2775925269652,
12.));
#178383=CARTESIAN_POINT('Ctrl Pts',(-7.52682526918541,21.2742366113579,
12.));
#178384=CARTESIAN_POINT('Ctrl Pts',(-7.5258712609553,21.2712301573466,12.));
#178385=CARTESIAN_POINT('Ctrl Pts',(-7.5250177033353,21.2685823838671,12.));
#178386=CARTESIAN_POINT('Ctrl Pts',(-7.52427261074298,21.2663059157058,
12.));
#178387=CARTESIAN_POINT('Ctrl Pts',(-7.52364573027553,21.2644161259962,
12.));
#178388=CARTESIAN_POINT('Ctrl Pts',(-7.52314642316199,21.262927782038,12.));
#178389=CARTESIAN_POINT('Ctrl Pts',(-7.5227818224267,21.2618521283555,12.));
#178390=CARTESIAN_POINT('Ctrl Pts',(-7.52260064231661,21.261326054066,12.));
#178391=CARTESIAN_POINT('Ctrl Pts',(-7.52252744144904,21.2611204474866,
12.));
#178392=CARTESIAN_POINT('Ctrl Pts',(-7.5225064970397,21.2610673466886,12.));
#178393=CARTESIAN_POINT('Ctrl Pts',(-7.52250298901264,21.2610617890679,
12.));
#178394=CARTESIAN_POINT('',(-7.33627833380046,20.7347298079577,12.));
#178395=CARTESIAN_POINT('',(-3.58569854577611,10.1343606576251,12.));
#178396=CARTESIAN_POINT('',(-7.63019749246977,20.1004996511507,12.));
#178397=CARTESIAN_POINT('Origin',(-7.80764394578302,20.56795313141,12.));
#178398=CARTESIAN_POINT('',(-8.8178352198485,19.6085639972844,12.));
#178399=CARTESIAN_POINT('Origin',(-2.70312158620511E-13,7.32141292029404E-13,
12.));
#178400=CARTESIAN_POINT('',(-9.47413589477548,19.84920021178,12.));
#178401=CARTESIAN_POINT('Origin',(-9.02290115519381,20.0645771135003,12.));
#178402=CARTESIAN_POINT('',(-9.71462809124916,20.353053841303,12.));
#178403=CARTESIAN_POINT('',(-4.85731404562459,10.1765269206515,12.));
#178404=CARTESIAN_POINT('',(-12.4230808101438,22.8400320311648,12.));
#178405=CARTESIAN_POINT('Ctrl Pts',(-9.71462809124916,20.353053841303,12.));
#178406=CARTESIAN_POINT('Ctrl Pts',(-9.71462954053042,20.353060251684,12.));
#178407=CARTESIAN_POINT('Ctrl Pts',(-9.71465227853041,20.3531126095522,
12.));
#178408=CARTESIAN_POINT('Ctrl Pts',(-9.71474590350681,20.3533097561886,
12.));
#178409=CARTESIAN_POINT('Ctrl Pts',(-9.71498978052021,20.3538098605706,
12.));
#178410=CARTESIAN_POINT('Ctrl Pts',(-9.71549257088172,20.3548282742361,
12.));
#178411=CARTESIAN_POINT('Ctrl Pts',(-9.71619192554186,20.3562337557875,
12.));
#178412=CARTESIAN_POINT('Ctrl Pts',(-9.71708493723096,20.3580133103356,
12.));
#178413=CARTESIAN_POINT('Ctrl Pts',(-9.71816778328006,20.3601498764344,
12.));
#178414=CARTESIAN_POINT('Ctrl Pts',(-9.71943648548099,20.3626256913981,
12.));
#178415=CARTESIAN_POINT('Ctrl Pts',(-9.72088778381081,20.3654261611056,
12.));
#178416=CARTESIAN_POINT('Ctrl Pts',(-9.7225193072249,20.3685406190576,12.));
#178417=CARTESIAN_POINT('Ctrl Pts',(-9.72432910043194,20.371960235676,12.));
#178418=CARTESIAN_POINT('Ctrl Pts',(-9.7263153173288,20.3756766651951,12.));
#178419=CARTESIAN_POINT('Ctrl Pts',(-9.72847589116542,20.3796805893304,
12.));
#178420=CARTESIAN_POINT('Ctrl Pts',(-9.73080870123727,20.3839624556742,
12.));
#178421=CARTESIAN_POINT('Ctrl Pts',(-9.73331167102808,20.3885129129912,
12.));
#178422=CARTESIAN_POINT('Ctrl Pts',(-9.73598292014243,20.3933234845647,
12.));
#178423=CARTESIAN_POINT('Ctrl Pts',(-9.73882077613201,20.3983866213331,
12.));
#178424=CARTESIAN_POINT('Ctrl Pts',(-9.74182369656272,20.4036953576549,
12.));
#178425=CARTESIAN_POINT('Ctrl Pts',(-9.74499021838538,20.4092430879861,
12.));
#178426=CARTESIAN_POINT('Ctrl Pts',(-9.74831889242174,20.4150232777393,
12.));
#178427=CARTESIAN_POINT('Ctrl Pts',(-9.7518082978643,20.4210295275817,12.));
#178428=CARTESIAN_POINT('Ctrl Pts',(-9.75545705902418,20.4272556476629,
12.));
#178429=CARTESIAN_POINT('Ctrl Pts',(-9.75926386289923,20.4336957355473,
12.));
#178430=CARTESIAN_POINT('Ctrl Pts',(-9.76322747195495,20.44034423294,12.));
#178431=CARTESIAN_POINT('Ctrl Pts',(-9.76734670980892,20.447195862298,12.));
#178432=CARTESIAN_POINT('Ctrl Pts',(-9.7716204510407,20.4542455817527,12.));
#178433=CARTESIAN_POINT('Ctrl Pts',(-9.77604760815529,20.4614885274975,
12.));
#178434=CARTESIAN_POINT('Ctrl Pts',(-9.78062712373321,20.4689199790669,
12.));
#178435=CARTESIAN_POINT('Ctrl Pts',(-9.78535797314167,20.4765353711586,
12.));
#178436=CARTESIAN_POINT('Ctrl Pts',(-9.79023916498656,20.4843302955329,
12.));
#178437=CARTESIAN_POINT('Ctrl Pts',(-9.79526974288331,20.4923005087943,
12.));
#178438=CARTESIAN_POINT('Ctrl Pts',(-9.80044878520949,20.5004419312107,
12.));
#178439=CARTESIAN_POINT('Ctrl Pts',(-9.80577540161088,20.5087506310505,
12.));
#178440=CARTESIAN_POINT('Ctrl Pts',(-9.81124873025282,20.517222812284,12.));
#178441=CARTESIAN_POINT('Ctrl Pts',(-9.81686793455943,20.5258548000629,
12.));
#178442=CARTESIAN_POINT('Ctrl Pts',(-9.82263220080363,20.5346430299517,
12.));
#178443=CARTESIAN_POINT('Ctrl Pts',(-9.82854073773877,20.5435840460721,
12.));
#178444=CARTESIAN_POINT('Ctrl Pts',(-9.83459277585315,20.552674497646,12.));
#178445=CARTESIAN_POINT('Ctrl Pts',(-9.84078756677565,20.5619111362402,
12.));
#178446=CARTESIAN_POINT('Ctrl Pts',(-9.84712438256278,20.5712908125139,
12.));
#178447=CARTESIAN_POINT('Ctrl Pts',(-9.85360251456981,20.5808104710015,
12.));
#178448=CARTESIAN_POINT('Ctrl Pts',(-9.86022127232748,20.5904671449754,
12.));
#178449=CARTESIAN_POINT('Ctrl Pts',(-9.86697998242623,20.6002579513699,
12.));
#178450=CARTESIAN_POINT('Ctrl Pts',(-9.87387798732956,20.6101800854494,
12.));
#178451=CARTESIAN_POINT('Ctrl Pts',(-9.88091464472676,20.6202308177474,
12.));
#178452=CARTESIAN_POINT('Ctrl Pts',(-9.88808932697306,20.6304074914087,
12.));
#178453=CARTESIAN_POINT('Ctrl Pts',(-9.8954014204912,20.6407075193976,12.));
#178454=CARTESIAN_POINT('Ctrl Pts',(-9.90285032516693,20.6511283817414,
12.));
#178455=CARTESIAN_POINT('Ctrl Pts',(-9.91043545377007,20.6616676228315,
12.));
#178456=CARTESIAN_POINT('Ctrl Pts',(-9.91815623141289,20.6723228488263,
12.));
#178457=CARTESIAN_POINT('Ctrl Pts',(-9.92601209498749,20.6830917250255,
12.));
#178458=CARTESIAN_POINT('Ctrl Pts',(-9.9340024925973,20.6939719732484,12.));
#178459=CARTESIAN_POINT('Ctrl Pts',(-9.94212688298236,20.7049613692234,
12.));
#178460=CARTESIAN_POINT('Ctrl Pts',(-9.95038473514949,20.7160577407579,
12.));
#178461=CARTESIAN_POINT('Ctrl Pts',(-9.95877552798398,20.7272589658751,
12.));
#178462=CARTESIAN_POINT('Ctrl Pts',(-9.96729874986202,20.7385629709795,
12.));
#178463=CARTESIAN_POINT('Ctrl Pts',(-9.9759538982347,20.7499677289627,12.));
#178464=CARTESIAN_POINT('Ctrl Pts',(-9.98474047926852,20.761471257499,12.));
#178465=CARTESIAN_POINT('Ctrl Pts',(-9.9936580075464,20.7730716175417,12.));
#178466=CARTESIAN_POINT('Ctrl Pts',(-10.0027060057389,20.7847669117568,
12.));
#178467=CARTESIAN_POINT('Ctrl Pts',(-10.0118840042786,20.7965552829908,
12.));
#178468=CARTESIAN_POINT('Ctrl Pts',(-10.0211915410095,20.8084349126888,
12.));
#178469=CARTESIAN_POINT('Ctrl Pts',(-10.0306281609435,20.8204040196602,
12.));
#178470=CARTESIAN_POINT('Ctrl Pts',(-10.0401934160234,20.8324608588909,
12.));
#178471=CARTESIAN_POINT('Ctrl Pts',(-10.0498868648733,20.8446037203402,
12.));
#178472=CARTESIAN_POINT('Ctrl Pts',(-10.0597080725375,20.8568309277316,
12.));
#178473=CARTESIAN_POINT('Ctrl Pts',(-10.0696566102218,20.86914083737,12.));
#178474=CARTESIAN_POINT('Ctrl Pts',(-10.0797320551154,20.881531837184,12.));
#178475=CARTESIAN_POINT('Ctrl Pts',(-10.0899339901916,20.894002345737,12.));
#178476=CARTESIAN_POINT('Ctrl Pts',(-10.1002620040076,20.9065508112557,
12.));
#178477=CARTESIAN_POINT('Ctrl Pts',(-10.1107156904836,20.919175710627,12.));
#178478=CARTESIAN_POINT('Ctrl Pts',(-10.1212946487057,20.9318755484734,
12.));
#178479=CARTESIAN_POINT('Ctrl Pts',(-10.1319984827908,20.9446488563933,
12.));
#178480=CARTESIAN_POINT('Ctrl Pts',(-10.1428268017256,20.9574941921591,
12.));
#178481=CARTESIAN_POINT('Ctrl Pts',(-10.1537792192065,20.9704101389369,
12.));
#178482=CARTESIAN_POINT('Ctrl Pts',(-10.1648553534568,20.9833953044736,
12.));
#178483=CARTESIAN_POINT('Ctrl Pts',(-10.1760548270767,20.9964483203686,
12.));
#178484=CARTESIAN_POINT('Ctrl Pts',(-10.187377266936,21.0095678414486,12.));
#178485=CARTESIAN_POINT('Ctrl Pts',(-10.1988223040425,21.0227525451107,
12.));
#178486=CARTESIAN_POINT('Ctrl Pts',(-10.2103895734123,21.0360011306815,
12.));
#178487=CARTESIAN_POINT('Ctrl Pts',(-10.2220787139155,21.0493123187483,
12.));
#178488=CARTESIAN_POINT('Ctrl Pts',(-10.2338893681567,21.0626848505663,
12.));
#178489=CARTESIAN_POINT('Ctrl Pts',(-10.2458211823912,21.0761174875445,
12.));
#178490=CARTESIAN_POINT('Ctrl Pts',(-10.2578738064181,21.0896090107063,
12.));
#178491=CARTESIAN_POINT('Ctrl Pts',(-10.2700468934744,21.1031582201627,
12.));
#178492=CARTESIAN_POINT('Ctrl Pts',(-10.2823401001072,21.1167639345631,
12.));
#178493=CARTESIAN_POINT('Ctrl Pts',(-10.2947530860721,21.1304249906002,
12.));
#178494=CARTESIAN_POINT('Ctrl Pts',(-10.3072855142687,21.1441402425843,
12.));
#178495=CARTESIAN_POINT('Ctrl Pts',(-10.3199370506544,21.1579085619965,
12.));
#178496=CARTESIAN_POINT('Ctrl Pts',(-10.3327073641572,21.1717288370509,
12.));
#178497=CARTESIAN_POINT('Ctrl Pts',(-10.3455961265701,21.1855999722416,
12.));
#178498=CARTESIAN_POINT('Ctrl Pts',(-10.3586030124587,21.199520887919,12.));
#178499=CARTESIAN_POINT('Ctrl Pts',(-10.371727699113,21.2134905199345,12.));
#178500=CARTESIAN_POINT('Ctrl Pts',(-10.3849698664786,21.22750781927,12.));
#178501=CARTESIAN_POINT('Ctrl Pts',(-10.3983291970846,21.2415717516714,
12.));
#178502=CARTESIAN_POINT('Ctrl Pts',(-10.4118053759588,21.255681297275,12.));
#178503=CARTESIAN_POINT('Ctrl Pts',(-10.42539809054,21.2698354502403,12.));
#178504=CARTESIAN_POINT('Ctrl Pts',(-10.4391070306391,21.2840332184483,
12.));
#178505=CARTESIAN_POINT('Ctrl Pts',(-10.4529318883874,21.2982736231931,
12.));
#178506=CARTESIAN_POINT('Ctrl Pts',(-10.4668723581768,21.3125556988731,
12.));
#178507=CARTESIAN_POINT('Ctrl Pts',(-10.4809281365931,21.3268784926819,
12.));
#178508=CARTESIAN_POINT('Ctrl Pts',(-10.4950989223337,21.3412410642904,
12.));
#178509=CARTESIAN_POINT('Ctrl Pts',(-10.5093844161685,21.3556424855814,
12.));
#178510=CARTESIAN_POINT('Ctrl Pts',(-10.5237843209057,21.3700818403936,
12.));
#178511=CARTESIAN_POINT('Ctrl Pts',(-10.5382983413421,21.3845582242602,
12.));
#178512=CARTESIAN_POINT('Ctrl Pts',(-10.5529261842108,21.3990707441497,
12.));
#178513=CARTESIAN_POINT('Ctrl Pts',(-10.5676675581108,21.4136185181979,
12.));
#178514=CARTESIAN_POINT('Ctrl Pts',(-10.5825221734573,21.4282006754631,
12.));
#178515=CARTESIAN_POINT('Ctrl Pts',(-10.5974897424622,21.4428163557144,
12.));
#178516=CARTESIAN_POINT('Ctrl Pts',(-10.6125699790961,21.4574647092097,
12.));
#178517=CARTESIAN_POINT('Ctrl Pts',(-10.6277625990456,21.4721448964766,
12.));
#178518=CARTESIAN_POINT('Ctrl Pts',(-10.6430673196607,21.4868560880889,
12.));
#178519=CARTESIAN_POINT('Ctrl Pts',(-10.6584838598939,21.5015974644449,
12.));
#178520=CARTESIAN_POINT('Ctrl Pts',(-10.6740119402834,21.51636821558,12.));
#178521=CARTESIAN_POINT('Ctrl Pts',(-10.689651282929,21.5311675409807,12.));
#178522=CARTESIAN_POINT('Ctrl Pts',(-10.7054016114571,21.5459946493955,
12.));
#178523=CARTESIAN_POINT('Ctrl Pts',(-10.7212626509816,21.5608487586468,
12.));
#178524=CARTESIAN_POINT('Ctrl Pts',(-10.7372341280467,21.5757290954371,
12.));
#178525=CARTESIAN_POINT('Ctrl Pts',(-10.7533157705941,21.5906348951743,
12.));
#178526=CARTESIAN_POINT('Ctrl Pts',(-10.7695073079552,21.6055654018176,
12.));
#178527=CARTESIAN_POINT('Ctrl Pts',(-10.7858084708261,21.6205198677173,
12.));
#178528=CARTESIAN_POINT('Ctrl Pts',(-10.8022189912369,21.6354975534557,
12.));
#178529=CARTESIAN_POINT('Ctrl Pts',(-10.8187386025136,21.6504977276866,
12.));
#178530=CARTESIAN_POINT('Ctrl Pts',(-10.8353670392272,21.6655196669732,
12.));
#178531=CARTESIAN_POINT('Ctrl Pts',(-10.8521040371835,21.6805626556467,
12.));
#178532=CARTESIAN_POINT('Ctrl Pts',(-10.8689493334095,21.6956259856672,
12.));
#178533=CARTESIAN_POINT('Ctrl Pts',(-10.8859026661293,21.7107089564825,
12.));
#178534=CARTESIAN_POINT('Ctrl Pts',(-10.902963774734,21.7258108748873,12.));
#178535=CARTESIAN_POINT('Ctrl Pts',(-10.9201323997384,21.7409310548797,
12.));
#178536=CARTESIAN_POINT('Ctrl Pts',(-10.9374082827444,21.7560688175247,
12.));
#178537=CARTESIAN_POINT('Ctrl Pts',(-10.9547911664455,21.7712234908464,
12.));
#178538=CARTESIAN_POINT('Ctrl Pts',(-10.9722807946156,21.7863944097141,
12.));
#178539=CARTESIAN_POINT('Ctrl Pts',(-10.9898769120912,21.8015809157301,
12.));
#178540=CARTESIAN_POINT('Ctrl Pts',(-11.0075792647477,21.8167823571168,
12.));
#178541=CARTESIAN_POINT('Ctrl Pts',(-11.0253875994598,21.8319980886033,
12.));
#178542=CARTESIAN_POINT('Ctrl Pts',(-11.0433016640807,21.8472274713103,
12.));
#178543=CARTESIAN_POINT('Ctrl Pts',(-11.0613212074363,21.8624698726318,
12.));
#178544=CARTESIAN_POINT('Ctrl Pts',(-11.0794459793057,21.877724666119,12.));
#178545=CARTESIAN_POINT('Ctrl Pts',(-11.0976757303944,21.8929912313608,
12.));
#178546=CARTESIAN_POINT('Ctrl Pts',(-11.1160102123024,21.9082689538688,
12.));
#178547=CARTESIAN_POINT('Ctrl Pts',(-11.1344491774741,21.923557224952,12.));
#178548=CARTESIAN_POINT('Ctrl Pts',(-11.1529923792003,21.9388554416439,
12.));
#178549=CARTESIAN_POINT('Ctrl Pts',(-11.1716395716376,21.9541630066506,
12.));
#178550=CARTESIAN_POINT('Ctrl Pts',(-11.190390509811,21.9694793282914,12.));
#178551=CARTESIAN_POINT('Ctrl Pts',(-11.2092449496125,21.9848038204439,
12.));
#178552=CARTESIAN_POINT('Ctrl Pts',(-11.2282026477896,22.0001359024839,
12.));
#178553=CARTESIAN_POINT('Ctrl Pts',(-11.2472633619275,22.0154749992363,
12.));
#178554=CARTESIAN_POINT('Ctrl Pts',(-11.2664268504206,22.030820540835,12.));
#178555=CARTESIAN_POINT('Ctrl Pts',(-11.2856928724374,22.046171962566,12.));
#178556=CARTESIAN_POINT('Ctrl Pts',(-11.3050611878771,22.0615287047179,
12.));
#178557=CARTESIAN_POINT('Ctrl Pts',(-11.3245315573168,22.0768902124267,
12.));
#178558=CARTESIAN_POINT('Ctrl Pts',(-11.3441037419553,22.0922559355294,
12.));
#178559=CARTESIAN_POINT('Ctrl Pts',(-11.3637775035367,22.1076253283979,
12.));
#178560=CARTESIAN_POINT('Ctrl Pts',(-11.3835526044256,22.1229978500186,
12.));
#178561=CARTESIAN_POINT('Ctrl Pts',(-11.4034288076908,22.1383729640964,
12.));
#178562=CARTESIAN_POINT('Ctrl Pts',(-11.4234058771742,22.1537501391487,
12.));
#178563=CARTESIAN_POINT('Ctrl Pts',(-11.443483577557,22.1691288486096,12.));
#178564=CARTESIAN_POINT('Ctrl Pts',(-11.463661674411,22.184508570917,12.));
#178565=CARTESIAN_POINT('Ctrl Pts',(-11.483939934259,22.1998887896436,12.));
#178566=CARTESIAN_POINT('Ctrl Pts',(-11.5043181244242,22.2152689931022,
12.));
#178567=CARTESIAN_POINT('Ctrl Pts',(-11.5247960128477,22.2306486738901,
12.));
#178568=CARTESIAN_POINT('Ctrl Pts',(-11.5453733679121,22.2460273284654,
12.));
#178569=CARTESIAN_POINT('Ctrl Pts',(-11.5660499582403,22.2614044566898,
12.));
#178570=CARTESIAN_POINT('Ctrl Pts',(-11.5868255525188,22.2767795614348,
12.));
#178571=CARTESIAN_POINT('Ctrl Pts',(-11.6076999192357,22.2921521480356,
12.));
#178572=CARTESIAN_POINT('Ctrl Pts',(-11.6286728270009,22.3075217249049,
12.));
#178573=CARTESIAN_POINT('Ctrl Pts',(-11.6497440449857,22.3228878043976,
12.));
#178574=CARTESIAN_POINT('Ctrl Pts',(-11.6709133432985,22.3382499035619,
12.));
#178575=CARTESIAN_POINT('Ctrl Pts',(-11.6921804934056,22.3536075450029,
12.));
#178576=CARTESIAN_POINT('Ctrl Pts',(-11.7135452684532,22.3689602575491,
12.));
#178577=CARTESIAN_POINT('Ctrl Pts',(-11.7350074437961,22.3843075773899,
12.));
#178578=CARTESIAN_POINT('Ctrl Pts',(-11.7565667964764,22.3996490469191,
12.));
#178579=CARTESIAN_POINT('Ctrl Pts',(-11.7782231042039,22.4149842125008,
12.));
#178580=CARTESIAN_POINT('Ctrl Pts',(-11.7999761445173,22.430312622646,12.));
#178581=CARTESIAN_POINT('Ctrl Pts',(-11.8218256937889,22.4456338258735,
12.));
#178582=CARTESIAN_POINT('Ctrl Pts',(-11.8437715264487,22.4609473690471,
12.));
#178583=CARTESIAN_POINT('Ctrl Pts',(-11.8658134137019,22.4762527946702,
12.));
#178584=CARTESIAN_POINT('Ctrl Pts',(-11.8879511239943,22.4915496418485,
12.));
#178585=CARTESIAN_POINT('Ctrl Pts',(-11.9101844254557,22.5068374513973,
12.));
#178586=CARTESIAN_POINT('Ctrl Pts',(-11.9325130877803,22.5221157697883,
12.));
#178587=CARTESIAN_POINT('Ctrl Pts',(-11.9549368843997,22.5373841537307,
12.));
#178588=CARTESIAN_POINT('Ctrl Pts',(-11.9774555943496,22.5526421741158,
12.));
#178589=CARTESIAN_POINT('Ctrl Pts',(-12.0000690046695,22.5678894211181,
12.));
#178590=CARTESIAN_POINT('Ctrl Pts',(-12.0227769113127,22.5831255061282,
12.));
#178591=CARTESIAN_POINT('Ctrl Pts',(-12.0455791139128,22.5983500505644,
12.));
#178592=CARTESIAN_POINT('Ctrl Pts',(-12.0684754113862,22.6135626764898,
12.));
#178593=CARTESIAN_POINT('Ctrl Pts',(-12.0914655972823,22.6287629967056,
12.));
#178594=CARTESIAN_POINT('Ctrl Pts',(-12.1145494550383,22.6439506046605,
12.));
#178595=CARTESIAN_POINT('Ctrl Pts',(-12.1377267537145,22.6591250653965,
12.));
#178596=CARTESIAN_POINT('Ctrl Pts',(-12.1609972423099,22.6742859034944,
12.));
#178597=CARTESIAN_POINT('Ctrl Pts',(-12.1843606579262,22.6894326205037,
12.));
#178598=CARTESIAN_POINT('Ctrl Pts',(-12.2078167360284,22.7045647168747,
12.));
#178599=CARTESIAN_POINT('Ctrl Pts',(-12.2313652198061,22.7196817119374,
12.));
#178600=CARTESIAN_POINT('Ctrl Pts',(-12.2550058702395,22.7347831655287,
12.));
#178601=CARTESIAN_POINT('Ctrl Pts',(-12.2787384750742,22.7498686970069,
12.));
#178602=CARTESIAN_POINT('Ctrl Pts',(-12.3025628601792,22.764938010105,12.));
#178603=CARTESIAN_POINT('Ctrl Pts',(-12.3264788926075,22.7799908974768,
12.));
#178604=CARTESIAN_POINT('Ctrl Pts',(-12.3504864740319,22.795027221673,12.));
#178605=CARTESIAN_POINT('Ctrl Pts',(-12.374585536673,22.81004690224,12.));
#178606=CARTESIAN_POINT('Ctrl Pts',(-12.3939379378998,22.8220493007173,
12.));
#178607=CARTESIAN_POINT('Ctrl Pts',(-12.4084933766347,22.8310435872747,
12.));
#178608=CARTESIAN_POINT('Ctrl Pts',(-12.418215285186,22.8370364396459,12.));
#178609=CARTESIAN_POINT('Ctrl Pts',(-12.4230808101438,22.8400320311648,
12.));
#178610=CARTESIAN_POINT('',(-13.5685075571671,22.1787195904339,12.));
#178611=CARTESIAN_POINT('Origin',(0.,0.,12.));
#178612=CARTESIAN_POINT('',(-12.7689476255363,18.5896416359912,12.));
#178613=CARTESIAN_POINT('Ctrl Pts',(-13.5685075571671,22.1787195904339,
12.));
#178614=CARTESIAN_POINT('Ctrl Pts',(-13.5683460612942,22.1730081264608,
12.));
#178615=CARTESIAN_POINT('Ctrl Pts',(-13.5680170531805,22.1615922805008,
12.));
#178616=CARTESIAN_POINT('Ctrl Pts',(-13.5675054919061,22.1444897575194,
12.));
#178617=CARTESIAN_POINT('Ctrl Pts',(-13.5667873105359,22.1217288871975,
12.));
#178618=CARTESIAN_POINT('Ctrl Pts',(-13.5658294169284,22.0933486464593,
12.));
#178619=CARTESIAN_POINT('Ctrl Pts',(-13.5648113689033,22.0650393089609,
12.));
#178620=CARTESIAN_POINT('Ctrl Pts',(-13.5637332022473,22.0368009736295,
12.));
#178621=CARTESIAN_POINT('Ctrl Pts',(-13.5625949868333,22.0086337943449,
12.));
#178622=CARTESIAN_POINT('Ctrl Pts',(-13.5613968357561,21.9805379899168,
12.));
#178623=CARTESIAN_POINT('Ctrl Pts',(-13.5601389185257,21.9525138592813,
12.));
#178624=CARTESIAN_POINT('Ctrl Pts',(-13.5588214586604,21.9245617765769,
12.));
#178625=CARTESIAN_POINT('Ctrl Pts',(-13.5574447178424,21.8966821688824,
12.));
#178626=CARTESIAN_POINT('Ctrl Pts',(-13.5560089839385,21.8688754989365,
12.));
#178627=CARTESIAN_POINT('Ctrl Pts',(-13.5545145573031,21.8411422456075,
12.));
#178628=CARTESIAN_POINT('Ctrl Pts',(-13.5529617381573,21.8134828857967,
12.));
#178629=CARTESIAN_POINT('Ctrl Pts',(-13.551350812725,21.7858978745865,12.));
#178630=CARTESIAN_POINT('Ctrl Pts',(-13.5496820422211,21.7583876294554,
12.));
#178631=CARTESIAN_POINT('Ctrl Pts',(-13.5479556704481,21.7309525412281,
12.));
#178632=CARTESIAN_POINT('Ctrl Pts',(-13.5461719295048,21.7035929822955,
12.));
#178633=CARTESIAN_POINT('Ctrl Pts',(-13.5443310461526,21.6763093157699,
12.));
#178634=CARTESIAN_POINT('Ctrl Pts',(-13.5424332480699,21.6491019044648,
12.));
#178635=CARTESIAN_POINT('Ctrl Pts',(-13.5404787697792,21.6219711193946,
12.));
#178636=CARTESIAN_POINT('Ctrl Pts',(-13.5384678597195,21.5949173499013,
12.));
#178637=CARTESIAN_POINT('Ctrl Pts',(-13.536400779028,21.5679410019001,12.));
#178638=CARTESIAN_POINT('Ctrl Pts',(-13.5342777983215,21.5410424932503,
12.));
#178639=CARTESIAN_POINT('Ctrl Pts',(-13.5320991952138,21.5142222501666,
12.));
#178640=CARTESIAN_POINT('Ctrl Pts',(-13.5298652514355,21.4874807030468,
12.));
#178641=CARTESIAN_POINT('Ctrl Pts',(-13.5275762503555,21.4608182828697,
12.));
#178642=CARTESIAN_POINT('Ctrl Pts',(-13.5252324737802,21.4342354165259,
12.));
#178643=CARTESIAN_POINT('Ctrl Pts',(-13.5228342013516,21.4077325259324,
12.));
#178644=CARTESIAN_POINT('Ctrl Pts',(-13.5203817122504,21.3813100304973,
12.));
#178645=CARTESIAN_POINT('Ctrl Pts',(-13.5178752862466,21.3549683486222,
12.));
#178646=CARTESIAN_POINT('Ctrl Pts',(-13.5153152050555,21.328707899634,12.));
#178647=CARTESIAN_POINT('Ctrl Pts',(-13.5127017534971,21.3025291054235,
12.));
#178648=CARTESIAN_POINT('Ctrl Pts',(-13.5100352209205,21.2764323924442,
12.));
#178649=CARTESIAN_POINT('Ctrl Pts',(-13.5073159019452,21.250418192743,12.));
#178650=CARTESIAN_POINT('Ctrl Pts',(-13.5045440957404,21.2244869429332,
12.));
#178651=CARTESIAN_POINT('Ctrl Pts',(-13.5017201056088,21.1986390835828,
12.));
#178652=CARTESIAN_POINT('Ctrl Pts',(-13.4988442384491,21.1728750584175,
12.));
#178653=CARTESIAN_POINT('Ctrl Pts',(-13.4959168042934,21.1471953136209,
12.));
#178654=CARTESIAN_POINT('Ctrl Pts',(-13.4929381157778,21.1216002970207,
12.));
#178655=CARTESIAN_POINT('Ctrl Pts',(-13.4899084877717,21.0960904575046,
12.));
#178656=CARTESIAN_POINT('Ctrl Pts',(-13.4868282377191,21.0706662455199,
12.));
#178657=CARTESIAN_POINT('Ctrl Pts',(-13.4836976858912,21.0453281134245,
12.));
#178658=CARTESIAN_POINT('Ctrl Pts',(-13.4805171556822,21.0200765158884,
12.));
#178659=CARTESIAN_POINT('Ctrl Pts',(-13.4772869738879,20.9949119102592,
12.));
#178660=CARTESIAN_POINT('Ctrl Pts',(-13.4740074710086,20.9698347569476,
12.));
#178661=CARTESIAN_POINT('Ctrl Pts',(-13.4706789815166,20.9448455197557,
12.));
#178662=CARTESIAN_POINT('Ctrl Pts',(-13.4673018437717,20.9199446657583,
12.));
#178663=CARTESIAN_POINT('Ctrl Pts',(-13.4638763999725,20.8951326652158,
12.));
#178664=CARTESIAN_POINT('Ctrl Pts',(-13.4604029960983,20.8704099914641,
12.));
#178665=CARTESIAN_POINT('Ctrl Pts',(-13.4568819818631,20.8457771208083,
12.));
#178666=CARTESIAN_POINT('Ctrl Pts',(-13.4533137106667,20.821234532398,12.));
#178667=CARTESIAN_POINT('Ctrl Pts',(-13.4496985395637,20.7967827081228,
12.));
#178668=CARTESIAN_POINT('Ctrl Pts',(-13.4460368293689,20.7724221327609,
12.));
#178669=CARTESIAN_POINT('Ctrl Pts',(-13.4423289447561,20.7481532941014,
12.));
#178670=CARTESIAN_POINT('Ctrl Pts',(-13.4385752543663,20.7239766830675,
12.));
#178671=CARTESIAN_POINT('Ctrl Pts',(-13.4347761309154,20.6998927938288,
12.));
#178672=CARTESIAN_POINT('Ctrl Pts',(-13.4309319513119,20.6759021239102,
12.));
#178673=CARTESIAN_POINT('Ctrl Pts',(-13.427043096765,20.6520051742867,12.));
#178674=CARTESIAN_POINT('Ctrl Pts',(-13.4231099528178,20.6282024494234,
12.));
#178675=CARTESIAN_POINT('Ctrl Pts',(-13.4191329093932,20.6044944573151,
12.));
#178676=CARTESIAN_POINT('Ctrl Pts',(-13.4151123608411,20.5808817095155,
12.));
#178677=CARTESIAN_POINT('Ctrl Pts',(-13.4110487059912,20.557364721164,12.));
#178678=CARTESIAN_POINT('Ctrl Pts',(-13.4069423482076,20.5339440109957,
12.));
#178679=CARTESIAN_POINT('Ctrl Pts',(-13.4027936954529,20.5106201013755,
12.));
#178680=CARTESIAN_POINT('Ctrl Pts',(-13.3986031603716,20.4873935184041,
12.));
#178681=CARTESIAN_POINT('Ctrl Pts',(-13.3943711603739,20.4642647920038,
12.));
#178682=CARTESIAN_POINT('Ctrl Pts',(-13.3900981177254,20.4412344560007,
12.));
#178683=CARTESIAN_POINT('Ctrl Pts',(-13.3857844596387,20.4183030482002,
12.));
#178684=CARTESIAN_POINT('Ctrl Pts',(-13.3814306183721,20.3954711104504,
12.));
#178685=CARTESIAN_POINT('Ctrl Pts',(-13.377037031319,20.3727391887187,12.));
#178686=CARTESIAN_POINT('Ctrl Pts',(-13.3726041410869,20.3501078331818,
12.));
#178687=CARTESIAN_POINT('Ctrl Pts',(-13.3681323955828,20.3275775983032,
12.));
#178688=CARTESIAN_POINT('Ctrl Pts',(-13.3636222481017,20.3051490429049,
12.));
#178689=CARTESIAN_POINT('Ctrl Pts',(-13.3590741574194,20.2828227302337,
12.));
#178690=CARTESIAN_POINT('Ctrl Pts',(-13.3544885878886,20.2605992280117,
12.));
#178691=CARTESIAN_POINT('Ctrl Pts',(-13.3498660095382,20.2384791085354,
12.));
#178692=CARTESIAN_POINT('Ctrl Pts',(-13.3452068981763,20.2164629487855,
12.));
#178693=CARTESIAN_POINT('Ctrl Pts',(-13.3405117354969,20.1945513305233,
12.));
#178694=CARTESIAN_POINT('Ctrl Pts',(-13.3357810091903,20.1727448403818,
12.));
#178695=CARTESIAN_POINT('Ctrl Pts',(-13.3310152130565,20.1510440699477,
12.));
#178696=CARTESIAN_POINT('Ctrl Pts',(-13.3262148471228,20.1294496158405,
12.));
#178697=CARTESIAN_POINT('Ctrl Pts',(-13.3213804177588,20.1079620798377,
12.));
#178698=CARTESIAN_POINT('Ctrl Pts',(-13.3165124377963,20.0865820689883,
12.));
#178699=CARTESIAN_POINT('Ctrl Pts',(-13.3116114266514,20.0653101957188,
12.));
#178700=CARTESIAN_POINT('Ctrl Pts',(-13.3066779104515,20.0441470779345,
12.));
#178701=CARTESIAN_POINT('Ctrl Pts',(-13.3017124221639,20.0230933391039,
12.));
#178702=CARTESIAN_POINT('Ctrl Pts',(-13.296715501731,20.0021496083742,12.));
#178703=CARTESIAN_POINT('Ctrl Pts',(-13.2916876962098,19.9813165207174,
12.));
#178704=CARTESIAN_POINT('Ctrl Pts',(-13.2866295599152,19.9605947170589,
12.));
#178705=CARTESIAN_POINT('Ctrl Pts',(-13.2815416545663,19.9399848444019,
12.));
#178706=CARTESIAN_POINT('Ctrl Pts',(-13.2764245494354,19.9194875559419,
12.));
#178707=CARTESIAN_POINT('Ctrl Pts',(-13.2712788215015,19.8991035111739,
12.));
#178708=CARTESIAN_POINT('Ctrl Pts',(-13.2661050556128,19.8788333760571,
12.));
#178709=CARTESIAN_POINT('Ctrl Pts',(-13.2609038446525,19.8586778231711,
12.));
#178710=CARTESIAN_POINT('Ctrl Pts',(-13.2556757897085,19.8386375318632,
12.));
#178711=CARTESIAN_POINT('Ctrl Pts',(-13.2504215002458,19.8187131883919,
12.));
#178712=CARTESIAN_POINT('Ctrl Pts',(-13.2451415942809,19.7989054860501,
12.));
#178713=CARTESIAN_POINT('Ctrl Pts',(-13.239836698568,19.7792151253297,12.));
#178714=CARTESIAN_POINT('Ctrl Pts',(-13.2345074487968,19.7596428141176,
12.));
#178715=CARTESIAN_POINT('Ctrl Pts',(-13.2291544897902,19.7401892678701,
12.));
#178716=CARTESIAN_POINT('Ctrl Pts',(-13.2237784757065,19.7208552097867,
12.));
#178717=CARTESIAN_POINT('Ctrl Pts',(-13.2183800702431,19.7016413709678,
12.));
#178718=CARTESIAN_POINT('Ctrl Pts',(-13.2129599468478,19.6825484905812,
12.));
#178719=CARTESIAN_POINT('Ctrl Pts',(-13.2075187889522,19.6635773160924,
12.));
#178720=CARTESIAN_POINT('Ctrl Pts',(-13.202057290206,19.6447286034764,12.));
#178721=CARTESIAN_POINT('Ctrl Pts',(-13.196576154715,19.6260031174244,12.));
#178722=CARTESIAN_POINT('Ctrl Pts',(-13.1910760972818,19.6074016315421,
12.));
#178723=CARTESIAN_POINT('Ctrl Pts',(-13.1855578436479,19.5889249285351,
12.));
#178724=CARTESIAN_POINT('Ctrl Pts',(-13.1800221307683,19.5705738004682,
12.));
#178725=CARTESIAN_POINT('Ctrl Pts',(-13.1744697070918,19.5523490490254,
12.));
#178726=CARTESIAN_POINT('Ctrl Pts',(-13.1689013328432,19.5342514857564,
12.));
#178727=CARTESIAN_POINT('Ctrl Pts',(-13.1633177803097,19.5162819323207,
12.));
#178728=CARTESIAN_POINT('Ctrl Pts',(-13.1577198341238,19.498441220707,12.));
#178729=CARTESIAN_POINT('Ctrl Pts',(-13.1521082915846,19.4807301935256,
12.));
#178730=CARTESIAN_POINT('Ctrl Pts',(-13.1464839629966,19.463149704325,12.));
#178731=CARTESIAN_POINT('Ctrl Pts',(-13.140847672006,19.4457006178875,12.));
#178732=CARTESIAN_POINT('Ctrl Pts',(-13.1352002559439,19.4283838105265,
12.));
#178733=CARTESIAN_POINT('Ctrl Pts',(-13.1295425661635,19.4112001703561,
12.));
#178734=CARTESIAN_POINT('Ctrl Pts',(-13.1238754684177,19.3941505976267,
12.));
#178735=CARTESIAN_POINT('Ctrl Pts',(-13.118199843271,19.3772360051093,12.));
#178736=CARTESIAN_POINT('Ctrl Pts',(-13.1125165865021,19.3604573184516,
12.));
#178737=CARTESIAN_POINT('Ctrl Pts',(-13.1068266095186,19.3438154765395,
12.));
#178738=CARTESIAN_POINT('Ctrl Pts',(-13.1011308397592,19.3273114318268,
12.));
#178739=CARTESIAN_POINT('Ctrl Pts',(-13.095430221148,19.3109461507358,12.));
#178740=CARTESIAN_POINT('Ctrl Pts',(-13.089725714597,19.2947206141246,12.));
#178741=CARTESIAN_POINT('Ctrl Pts',(-13.0840182984949,19.2786358177198,
12.));
#178742=CARTESIAN_POINT('Ctrl Pts',(-13.0783089692118,19.2626927725596,
12.));
#178743=CARTESIAN_POINT('Ctrl Pts',(-13.0725987415856,19.2468925053988,
12.));
#178744=CARTESIAN_POINT('Ctrl Pts',(-13.0668886494791,19.2312360592031,
12.));
#178745=CARTESIAN_POINT('Ctrl Pts',(-13.0611797463913,19.2157244937141,
12.));
#178746=CARTESIAN_POINT('Ctrl Pts',(-13.0554731060537,19.2003588859771,
12.));
#178747=CARTESIAN_POINT('Ctrl Pts',(-13.0497698230442,19.1851403308825,
12.));
#178748=CARTESIAN_POINT('Ctrl Pts',(-13.0440710133775,19.1700699416625,
12.));
#178749=CARTESIAN_POINT('Ctrl Pts',(-13.0383778152072,19.1551488505233,
12.));
#178750=CARTESIAN_POINT('Ctrl Pts',(-13.0326913895841,19.1403782093389,
12.));
#178751=CARTESIAN_POINT('Ctrl Pts',(-13.0270129211976,19.1257591903099,
12.));
#178752=CARTESIAN_POINT('Ctrl Pts',(-13.0213436191326,19.1112929866308,
12.));
#178753=CARTESIAN_POINT('Ctrl Pts',(-13.0156847176093,19.0969808131225,
12.));
#178754=CARTESIAN_POINT('Ctrl Pts',(-13.0100374768785,19.0828239070482,
12.));
#178755=CARTESIAN_POINT('Ctrl Pts',(-13.0044031841381,19.0688235289437,
12.));
#178756=CARTESIAN_POINT('Ctrl Pts',(-12.9987831544502,19.0549809634355,
12.));
#178757=CARTESIAN_POINT('Ctrl Pts',(-12.9931787316515,19.0412975200398,
12.));
#178758=CARTESIAN_POINT('Ctrl Pts',(-12.9875912893003,19.0277745339908,
12.));
#178759=CARTESIAN_POINT('Ctrl Pts',(-12.9820222318716,19.0144133673348,
12.));
#178760=CARTESIAN_POINT('Ctrl Pts',(-12.9764729959205,19.0012154099791,
12.));
#178761=CARTESIAN_POINT('Ctrl Pts',(-12.9709450512747,18.9881820807585,
12.));
#178762=CARTESIAN_POINT('Ctrl Pts',(-12.9654399021869,18.9753148284475,
12.));
#178763=CARTESIAN_POINT('Ctrl Pts',(-12.9599590886319,18.9626151329229,
12.));
#178764=CARTESIAN_POINT('Ctrl Pts',(-12.9545041877377,18.9500845064715,
12.));
#178765=CARTESIAN_POINT('Ctrl Pts',(-12.9490768151821,18.9377244950435,
12.));
#178766=CARTESIAN_POINT('Ctrl Pts',(-12.9436786266105,18.9255366795195,
12.));
#178767=CARTESIAN_POINT('Ctrl Pts',(-12.9383113190375,18.9135226769465,
12.));
#178768=CARTESIAN_POINT('Ctrl Pts',(-12.9329766328185,18.9016841423403,
12.));
#178769=CARTESIAN_POINT('Ctrl Pts',(-12.9276763536373,18.8900227704889,
12.));
#178770=CARTESIAN_POINT('Ctrl Pts',(-12.9224123144982,18.8785402977527,
12.));
#178771=CARTESIAN_POINT('Ctrl Pts',(-12.9171863977045,18.8672385038326,
12.));
#178772=CARTESIAN_POINT('Ctrl Pts',(-12.9120005369063,18.8561192136198,
12.));
#178773=CARTESIAN_POINT('Ctrl Pts',(-12.9068567191854,18.8451842990984,
12.));
#178774=CARTESIAN_POINT('Ctrl Pts',(-12.9017569871738,18.834435681259,12.));
#178775=CARTESIAN_POINT('Ctrl Pts',(-12.8967034410755,18.8238753319128,
12.));
#178776=CARTESIAN_POINT('Ctrl Pts',(-12.8916982409935,18.813505275782,12.));
#178777=CARTESIAN_POINT('Ctrl Pts',(-12.8867436109546,18.8033275941943,
12.));
#178778=CARTESIAN_POINT('Ctrl Pts',(-12.8818418427475,18.7933444285868,
12.));
#178779=CARTESIAN_POINT('Ctrl Pts',(-12.8769952998095,18.7835579840477,
12.));
#178780=CARTESIAN_POINT('Ctrl Pts',(-12.872206421181,18.7739705329022,12.));
#178781=CARTESIAN_POINT('Ctrl Pts',(-12.8674777239653,18.7645844169564,
12.));
#178782=CARTESIAN_POINT('Ctrl Pts',(-12.8628118054171,18.7554020493887,
12.));
#178783=CARTESIAN_POINT('Ctrl Pts',(-12.8582113455646,18.7464259171251,
12.));
#178784=CARTESIAN_POINT('Ctrl Pts',(-12.8536791086316,18.7376585820854,
12.));
#178785=CARTESIAN_POINT('Ctrl Pts',(-12.8492179511591,18.7291026886554,
12.));
#178786=CARTESIAN_POINT('Ctrl Pts',(-12.8448308329494,18.7207609737702,
12.));
#178787=CARTESIAN_POINT('Ctrl Pts',(-12.8405208263431,18.7126362754445,
12.));
#178788=CARTESIAN_POINT('Ctrl Pts',(-12.8362911280361,18.7047315436294,
12.));
#178789=CARTESIAN_POINT('Ctrl Pts',(-12.8321450599789,18.6970498410172,
12.));
#178790=CARTESIAN_POINT('Ctrl Pts',(-12.8280860635231,18.6895943376171,
12.));
#178791=CARTESIAN_POINT('Ctrl Pts',(-12.8241176980017,18.6823683094139,
12.));
#178792=CARTESIAN_POINT('Ctrl Pts',(-12.8202436318474,18.6753751301092,
12.));
#178793=CARTESIAN_POINT('Ctrl Pts',(-12.8164676687362,18.6686182952799,
12.));
#178794=CARTESIAN_POINT('Ctrl Pts',(-12.8127937909631,18.6621014624746,
12.));
#178795=CARTESIAN_POINT('Ctrl Pts',(-12.8092261933858,18.6558284825773,
12.));
#178796=CARTESIAN_POINT('Ctrl Pts',(-12.805769331162,18.6498034438986,12.));
#178797=CARTESIAN_POINT('Ctrl Pts',(-12.8024278770152,18.6440306327456,
12.));
#178798=CARTESIAN_POINT('Ctrl Pts',(-12.7992066625264,18.63851447924,12.));
#178799=CARTESIAN_POINT('Ctrl Pts',(-12.7961106222251,18.6332595057006,
12.));
#178800=CARTESIAN_POINT('Ctrl Pts',(-12.7931447451555,18.6282702819371,
12.));
#178801=CARTESIAN_POINT('Ctrl Pts',(-12.7903142925234,18.6235516265575,
12.));
#178802=CARTESIAN_POINT('Ctrl Pts',(-12.7876249657834,18.6191087624752,
12.));
#178803=CARTESIAN_POINT('Ctrl Pts',(-12.7850831657901,18.6149475565188,
12.));
#178804=CARTESIAN_POINT('Ctrl Pts',(-12.7826959526925,18.6110744826219,
12.));
#178805=CARTESIAN_POINT('Ctrl Pts',(-12.7804705387658,18.6074961535723,
12.));
#178806=CARTESIAN_POINT('Ctrl Pts',(-12.7784139605066,18.6042190183704,
12.));
#178807=CARTESIAN_POINT('Ctrl Pts',(-12.7765325225081,18.6012488486709,
12.));
#178808=CARTESIAN_POINT('Ctrl Pts',(-12.7748328937638,18.598591752595,12.));
#178809=CARTESIAN_POINT('Ctrl Pts',(-12.7733231262108,18.5962551167772,
12.));
#178810=CARTESIAN_POINT('Ctrl Pts',(-12.7720142287172,18.5942490615407,
12.));
#178811=CARTESIAN_POINT('Ctrl Pts',(-12.7709195951156,18.5925859134579,
12.));
#178812=CARTESIAN_POINT('Ctrl Pts',(-12.7700520897173,18.5912775137806,
12.));
#178813=CARTESIAN_POINT('Ctrl Pts',(-12.7694215127919,18.5903328777227,
12.));
#178814=CARTESIAN_POINT('Ctrl Pts',(-12.769110348199,18.589871621843,12.));
#178815=CARTESIAN_POINT('Ctrl Pts',(-12.768986426692,18.5896919669165,12.));
#178816=CARTESIAN_POINT('Ctrl Pts',(-12.7689524524483,18.5896460962964,
12.));
#178817=CARTESIAN_POINT('Ctrl Pts',(-12.7689476255363,18.5896416359912,
12.));
#178818=CARTESIAN_POINT('',(-12.4528436808172,18.1294424696716,12.));
#178819=CARTESIAN_POINT('',(-6.08648437878338,8.86099361848466,12.));
#178820=CARTESIAN_POINT('',(-12.572596943457,17.4407513054162,12.));
#178821=CARTESIAN_POINT('Origin',(-12.8649829188862,17.846350172984,12.));
#178822=CARTESIAN_POINT('',(-13.5924445804218,16.6581946899465,12.));
#178823=CARTESIAN_POINT('Origin',(-4.50593605254675E-13,6.37232247690086E-13,
12.));
#178824=CARTESIAN_POINT('',(-14.2886635873976,16.7207683102834,12.));
#178825=CARTESIAN_POINT('Origin',(-13.9085479427572,17.0455945664569,12.));
#178826=CARTESIAN_POINT('',(-14.6513681262571,17.1452095830633,12.));
#178827=CARTESIAN_POINT('',(-7.32568406312854,8.57260479153162,12.));
#178828=CARTESIAN_POINT('',(-17.9112098770111,18.8464468996588,12.));
#178829=CARTESIAN_POINT('Ctrl Pts',(-14.6513681262571,17.1452095830633,
12.));
#178830=CARTESIAN_POINT('Ctrl Pts',(-14.651371185284,17.1452153999142,12.));
#178831=CARTESIAN_POINT('Ctrl Pts',(-14.6514066997188,17.1452600887039,
12.));
#178832=CARTESIAN_POINT('Ctrl Pts',(-14.6515481598057,17.1454262858045,
12.));
#178833=CARTESIAN_POINT('Ctrl Pts',(-14.65191316345,17.1458462295273,12.));
#178834=CARTESIAN_POINT('Ctrl Pts',(-14.6526624064978,17.1466998098673,
12.));
#178835=CARTESIAN_POINT('Ctrl Pts',(-14.6537016966188,17.1478763944909,
12.));
#178836=CARTESIAN_POINT('Ctrl Pts',(-14.6550248622813,17.1493641837556,
12.));
#178837=CARTESIAN_POINT('Ctrl Pts',(-14.6566237952435,17.1511476869495,
12.));
#178838=CARTESIAN_POINT('Ctrl Pts',(-14.6584900555301,17.1532107762719,
12.));
#178839=CARTESIAN_POINT('Ctrl Pts',(-14.660616716964,17.1555401986403,12.));
#178840=CARTESIAN_POINT('Ctrl Pts',(-14.662998728599,17.1581262646789,12.));
#178841=CARTESIAN_POINT('Ctrl Pts',(-14.6656319165057,17.1609609517369,
12.));
#178842=CARTESIAN_POINT('Ctrl Pts',(-14.6685123374424,17.1640366762304,
12.));
#178843=CARTESIAN_POINT('Ctrl Pts',(-14.6716355833321,17.1673449723019,
12.));
#178844=CARTESIAN_POINT('Ctrl Pts',(-14.6749971333867,17.1708771619129,
12.));
#178845=CARTESIAN_POINT('Ctrl Pts',(-14.6785925615676,17.1746247499057,
12.));
#178846=CARTESIAN_POINT('Ctrl Pts',(-14.6824178576167,17.1785800350827,
12.));
#178847=CARTESIAN_POINT('Ctrl Pts',(-14.6864694522319,17.182736158472,12.));
#178848=CARTESIAN_POINT('Ctrl Pts',(-14.6907440526958,17.1870867909918,
12.));
#178849=CARTESIAN_POINT('Ctrl Pts',(-14.6952385361706,17.1916259308415,
12.));
#178850=CARTESIAN_POINT('Ctrl Pts',(-14.699949811582,17.1963476411694,12.));
#178851=CARTESIAN_POINT('Ctrl Pts',(-14.7048748502663,17.2012461084268,
12.));
#178852=CARTESIAN_POINT('Ctrl Pts',(-14.7100107213586,17.2063157097316,
12.));
#178853=CARTESIAN_POINT('Ctrl Pts',(-14.7153546289338,17.2115510835988,
12.));
#178854=CARTESIAN_POINT('Ctrl Pts',(-14.7209039390326,17.2169471814255,
12.));
#178855=CARTESIAN_POINT('Ctrl Pts',(-14.7266561494282,17.2224992099666,
12.));
#178856=CARTESIAN_POINT('Ctrl Pts',(-14.7326088681163,17.2282025904314,
12.));
#178857=CARTESIAN_POINT('Ctrl Pts',(-14.7387597858117,17.2340529062077,
12.));
#178858=CARTESIAN_POINT('Ctrl Pts',(-14.7451066593793,17.2400458713566,
12.));
#178859=CARTESIAN_POINT('Ctrl Pts',(-14.7516473175125,17.2461773413289,
12.));
#178860=CARTESIAN_POINT('Ctrl Pts',(-14.7583796616617,17.2524433146837,
12.));
#178861=CARTESIAN_POINT('Ctrl Pts',(-14.7653016697589,17.2588399401464,
12.));
#178862=CARTESIAN_POINT('Ctrl Pts',(-14.7724113956728,17.2653635155317,
12.));
#178863=CARTESIAN_POINT('Ctrl Pts',(-14.7797069617802,17.2720104735192,
12.));
#178864=CARTESIAN_POINT('Ctrl Pts',(-14.787186553128,17.278777370485,12.));
#178865=CARTESIAN_POINT('Ctrl Pts',(-14.7948484105253,17.28566087332,12.));
#178866=CARTESIAN_POINT('Ctrl Pts',(-14.8026908254281,17.2926577496519,
12.));
#178867=CARTESIAN_POINT('Ctrl Pts',(-14.8107121391038,17.2997648661483,
12.));
#178868=CARTESIAN_POINT('Ctrl Pts',(-14.8189107410161,17.3069791853705,
12.));
#178869=CARTESIAN_POINT('Ctrl Pts',(-14.8272850675375,17.3142977632656,
12.));
#178870=CARTESIAN_POINT('Ctrl Pts',(-14.8358336004193,17.3217177462096,
12.));
#178871=CARTESIAN_POINT('Ctrl Pts',(-14.8445548643504,17.3292363662601,
12.));
#178872=CARTESIAN_POINT('Ctrl Pts',(-14.8534474245433,17.336850936485,12.));
#178873=CARTESIAN_POINT('Ctrl Pts',(-14.8625098843419,17.3445588463477,
12.));
#178874=CARTESIAN_POINT('Ctrl Pts',(-14.8717408826958,17.3523575568648,
12.));
#178875=CARTESIAN_POINT('Ctrl Pts',(-14.8811390927424,17.3602445978163,
12.));
#178876=CARTESIAN_POINT('Ctrl Pts',(-14.8907032205789,17.3682175653236,
12.));
#178877=CARTESIAN_POINT('Ctrl Pts',(-14.9004320039609,17.3762741193075,
12.));
#178878=CARTESIAN_POINT('Ctrl Pts',(-14.9103242110057,17.3844119809823,
12.));
#178879=CARTESIAN_POINT('Ctrl Pts',(-14.9203786389343,17.3926289303987,
12.));
#178880=CARTESIAN_POINT('Ctrl Pts',(-14.9305941128758,17.400922804075,12.));
#178881=CARTESIAN_POINT('Ctrl Pts',(-14.940969484645,17.4092914926071,12.));
#178882=CARTESIAN_POINT('Ctrl Pts',(-14.9515036315142,17.4177329382827,
12.));
#178883=CARTESIAN_POINT('Ctrl Pts',(-14.9621954549825,17.4262451327088,
12.));
#178884=CARTESIAN_POINT('Ctrl Pts',(-14.973043879945,17.4348261151395,12.));
#178885=CARTESIAN_POINT('Ctrl Pts',(-14.9840478538357,17.4434739707773,
12.));
#178886=CARTESIAN_POINT('Ctrl Pts',(-14.9952063457779,17.4521868291005,
12.));
#178887=CARTESIAN_POINT('Ctrl Pts',(-15.0065183456922,17.4609628621419,
12.));
#178888=CARTESIAN_POINT('Ctrl Pts',(-15.0179828635087,17.4698002829357,
12.));
#178889=CARTESIAN_POINT('Ctrl Pts',(-15.029598928488,17.4786973441417,12.));
#178890=CARTESIAN_POINT('Ctrl Pts',(-15.0413655884993,17.4876523366178,
12.));
#178891=CARTESIAN_POINT('Ctrl Pts',(-15.0532819093085,17.4966635880246,
12.));
#178892=CARTESIAN_POINT('Ctrl Pts',(-15.0653469738307,17.5057294613877,
12.));
#178893=CARTESIAN_POINT('Ctrl Pts',(-15.0775598815749,17.5148483539687,
12.));
#178894=CARTESIAN_POINT('Ctrl Pts',(-15.0899197481082,17.524018696179,12.));
#178895=CARTESIAN_POINT('Ctrl Pts',(-15.1024257045033,17.5332389504829,
12.));
#178896=CARTESIAN_POINT('Ctrl Pts',(-15.1150768967728,17.5425076102963,
12.));
#178897=CARTESIAN_POINT('Ctrl Pts',(-15.1278724853138,17.5518231989117,
12.));
#178898=CARTESIAN_POINT('Ctrl Pts',(-15.1408116444876,17.5611842686192,
12.));
#178899=CARTESIAN_POINT('Ctrl Pts',(-15.1538935621714,17.5705893998029,
12.));
#178900=CARTESIAN_POINT('Ctrl Pts',(-15.1671174393137,17.580037200054,12.));
#178901=CARTESIAN_POINT('Ctrl Pts',(-15.1804824894605,17.5895263032595,
12.));
#178902=CARTESIAN_POINT('Ctrl Pts',(-15.1939879383268,17.5990553687599,
12.));
#178903=CARTESIAN_POINT('Ctrl Pts',(-15.2076330234686,17.60862308065,12.));
#178904=CARTESIAN_POINT('Ctrl Pts',(-15.2214169939199,17.6182281470468,
12.));
#178905=CARTESIAN_POINT('Ctrl Pts',(-15.2353391098366,17.6278692993764,
12.));
#178906=CARTESIAN_POINT('Ctrl Pts',(-15.2493986421092,17.6375452916369,
12.));
#178907=CARTESIAN_POINT('Ctrl Pts',(-15.2635948720292,17.6472548997328,
12.));
#178908=CARTESIAN_POINT('Ctrl Pts',(-15.2779270910239,17.6569969209,12.));
#178909=CARTESIAN_POINT('Ctrl Pts',(-15.2923946003598,17.6667701731041,
12.));
#178910=CARTESIAN_POINT('Ctrl Pts',(-15.3069967108501,17.676573494456,12.));
#178911=CARTESIAN_POINT('Ctrl Pts',(-15.3217327425338,17.6864057426052,
12.));
#178912=CARTESIAN_POINT('Ctrl Pts',(-15.3366020244066,17.6962657941983,
12.));
#178913=CARTESIAN_POINT('Ctrl Pts',(-15.351603894206,17.7061525444042,12.));
#178914=CARTESIAN_POINT('Ctrl Pts',(-15.3667376981699,17.7160649064206,
12.));
#178915=CARTESIAN_POINT('Ctrl Pts',(-15.3820027907967,17.7260018109924,
12.));
#178916=CARTESIAN_POINT('Ctrl Pts',(-15.3973985345802,17.7359622059149,
12.));
#178917=CARTESIAN_POINT('Ctrl Pts',(-15.4129242997837,17.7459450555812,
12.));
#178918=CARTESIAN_POINT('Ctrl Pts',(-15.4285794642668,17.7559493405881,
12.));
#178919=CARTESIAN_POINT('Ctrl Pts',(-15.4443634132869,17.7659740573265,
12.));
#178920=CARTESIAN_POINT('Ctrl Pts',(-15.4602755393017,17.7760182175815,
12.));
#178921=CARTESIAN_POINT('Ctrl Pts',(-15.4763152417497,17.7860808481219,
12.));
#178922=CARTESIAN_POINT('Ctrl Pts',(-15.4924819268517,17.7961609903148,
12.));
#178923=CARTESIAN_POINT('Ctrl Pts',(-15.5087750074718,17.8062576997952,
12.));
#178924=CARTESIAN_POINT('Ctrl Pts',(-15.5251939029552,17.8163700461256,
12.));
#178925=CARTESIAN_POINT('Ctrl Pts',(-15.541738038964,17.8264971124606,12.));
#178926=CARTESIAN_POINT('Ctrl Pts',(-15.5584068472982,17.8366379952085,
12.));
#178927=CARTESIAN_POINT('Ctrl Pts',(-15.5751997657163,17.8467918036987,
12.));
#178928=CARTESIAN_POINT('Ctrl Pts',(-15.5921162378192,17.8569576599006,
12.));
#178929=CARTESIAN_POINT('Ctrl Pts',(-15.609155712921,17.8671346981394,12.));
#178930=CARTESIAN_POINT('Ctrl Pts',(-15.6263176459108,17.8773220648125,
12.));
#178931=CARTESIAN_POINT('Ctrl Pts',(-15.6436014971084,17.8875189181091,
12.));
#178932=CARTESIAN_POINT('Ctrl Pts',(-15.661006732103,17.897724427724,12.));
#178933=CARTESIAN_POINT('Ctrl Pts',(-15.678532821646,17.9079377746111,12.));
#178934=CARTESIAN_POINT('Ctrl Pts',(-15.6961792415522,17.9181581507455,
12.));
#178935=CARTESIAN_POINT('Ctrl Pts',(-15.7139454725838,17.9283847588835,
12.));
#178936=CARTESIAN_POINT('Ctrl Pts',(-15.7318310003335,17.9386168123262,
12.));
#178937=CARTESIAN_POINT('Ctrl Pts',(-15.749835315086,17.9488535346781,12.));
#178938=CARTESIAN_POINT('Ctrl Pts',(-15.7679579117077,17.9590941596242,
12.));
#178939=CARTESIAN_POINT('Ctrl Pts',(-15.7861982895724,17.9693379307303,
12.));
#178940=CARTESIAN_POINT('Ctrl Pts',(-15.8045559524676,17.9795841012386,
12.));
#178941=CARTESIAN_POINT('Ctrl Pts',(-15.8230304084962,17.9898319338664,
12.));
#178942=CARTESIAN_POINT('Ctrl Pts',(-15.8416211699679,18.0000807006052,
12.));
#178943=CARTESIAN_POINT('Ctrl Pts',(-15.8603277532831,18.0103296825205,
12.));
#178944=CARTESIAN_POINT('Ctrl Pts',(-15.8791496788683,18.0205781695769,
12.));
#178945=CARTESIAN_POINT('Ctrl Pts',(-15.8980864711042,18.0308254604636,
12.));
#178946=CARTESIAN_POINT('Ctrl Pts',(-15.9171376582436,18.0410708624208,
12.));
#178947=CARTESIAN_POINT('Ctrl Pts',(-15.9363027723244,18.0513136910691,
12.));
#178948=CARTESIAN_POINT('Ctrl Pts',(-15.9555813490644,18.0615532702359,
12.));
#178949=CARTESIAN_POINT('Ctrl Pts',(-15.9749729277846,18.0717889317958,
12.));
#178950=CARTESIAN_POINT('Ctrl Pts',(-15.9944770513613,18.0820200155236,
12.));
#178951=CARTESIAN_POINT('Ctrl Pts',(-16.014093266161,18.0922458689462,12.));
#178952=CARTESIAN_POINT('Ctrl Pts',(-16.0338211219693,18.1024658471966,
12.));
#178953=CARTESIAN_POINT('Ctrl Pts',(-16.0536601719126,18.112679312869,12.));
#178954=CARTESIAN_POINT('Ctrl Pts',(-16.0736099723668,18.1228856358751,
12.));
#178955=CARTESIAN_POINT('Ctrl Pts',(-16.0936700829112,18.1330841933105,
12.));
#178956=CARTESIAN_POINT('Ctrl Pts',(-16.1138400662794,18.1432743693235,
12.));
#178957=CARTESIAN_POINT('Ctrl Pts',(-16.1341194882988,18.1534555549852,
12.));
#178958=CARTESIAN_POINT('Ctrl Pts',(-16.154507917826,18.1636271481615,12.));
#178959=CARTESIAN_POINT('Ctrl Pts',(-16.1750049266671,18.1737885533849,
12.));
#178960=CARTESIAN_POINT('Ctrl Pts',(-16.1956100895073,18.1839391817331,
12.));
#178961=CARTESIAN_POINT('Ctrl Pts',(-16.2163229838875,18.1940784507229,
12.));
#178962=CARTESIAN_POINT('Ctrl Pts',(-16.2371431901638,18.2042057842035,
12.));
#178963=CARTESIAN_POINT('Ctrl Pts',(-16.2580702914615,18.2143206122529,
12.));
#178964=CARTESIAN_POINT('Ctrl Pts',(-16.2791038736223,18.2244223710745,
12.));
#178965=CARTESIAN_POINT('Ctrl Pts',(-16.3002435251378,18.2345105028982,
12.));
#178966=CARTESIAN_POINT('Ctrl Pts',(-16.3214888370987,18.2445844558741,
12.));
#178967=CARTESIAN_POINT('Ctrl Pts',(-16.3428394031589,18.2546436839608,
12.));
#178968=CARTESIAN_POINT('Ctrl Pts',(-16.3642948194868,18.2646876468169,
12.));
#178969=CARTESIAN_POINT('Ctrl Pts',(-16.385854684708,18.2747158096934,12.));
#178970=CARTESIAN_POINT('Ctrl Pts',(-16.4075185998455,18.2847276433309,
12.));
#178971=CARTESIAN_POINT('Ctrl Pts',(-16.4292861682379,18.294722623851,12.));
#178972=CARTESIAN_POINT('Ctrl Pts',(-16.4511569955233,18.304700232686,12.));
#178973=CARTESIAN_POINT('Ctrl Pts',(-16.4731306896441,18.3146599565231,
12.));
#178974=CARTESIAN_POINT('Ctrl Pts',(-16.4952068608345,18.3246012872469,
12.));
#178975=CARTESIAN_POINT('Ctrl Pts',(-16.5173851216045,18.3345237218864,
12.));
#178976=CARTESIAN_POINT('Ctrl Pts',(-16.5396650867139,18.34442676256,12.));
#178977=CARTESIAN_POINT('Ctrl Pts',(-16.5620463731413,18.354309916433,12.));
#178978=CARTESIAN_POINT('Ctrl Pts',(-16.5845286000217,18.3641726955889,
12.));
#178979=CARTESIAN_POINT('Ctrl Pts',(-16.607111388571,18.3740146168879,12.));
#178980=CARTESIAN_POINT('Ctrl Pts',(-16.6297943620056,18.3838352018327,
12.));
#178981=CARTESIAN_POINT('Ctrl Pts',(-16.6525771454513,18.3936339764332,
12.));
#178982=CARTESIAN_POINT('Ctrl Pts',(-16.6754593658513,18.403410471079,12.));
#178983=CARTESIAN_POINT('Ctrl Pts',(-16.6984406518491,18.413164220399,12.));
#178984=CARTESIAN_POINT('Ctrl Pts',(-16.7215206338818,18.4228947633187,
12.));
#178985=CARTESIAN_POINT('Ctrl Pts',(-16.7446989442882,18.4326016431392,
12.));
#178986=CARTESIAN_POINT('Ctrl Pts',(-16.7679752173992,18.44228440761,12.));
#178987=CARTESIAN_POINT('Ctrl Pts',(-16.791349089629,18.4519426090123,12.));
#178988=CARTESIAN_POINT('Ctrl Pts',(-16.8148201995472,18.4615758042305,
12.));
#178989=CARTESIAN_POINT('Ctrl Pts',(-16.8383881879709,18.4711835548623,
12.));
#178990=CARTESIAN_POINT('Ctrl Pts',(-16.8620526977171,18.480765426877,12.));
#178991=CARTESIAN_POINT('Ctrl Pts',(-16.8858133733088,18.4903209902227,
12.));
#178992=CARTESIAN_POINT('Ctrl Pts',(-16.9096698606943,18.499849818462,12.));
#178993=CARTESIAN_POINT('Ctrl Pts',(-16.9336218069353,18.5093514883835,
12.));
#178994=CARTESIAN_POINT('Ctrl Pts',(-16.9576688599339,18.5188255796659,
12.));
#178995=CARTESIAN_POINT('Ctrl Pts',(-16.981810668038,18.5282716744197,12.));
#178996=CARTESIAN_POINT('Ctrl Pts',(-17.0060468805097,18.5376893576961,
12.));
#178997=CARTESIAN_POINT('Ctrl Pts',(-17.0303771481738,18.547078218209,12.));
#178998=CARTESIAN_POINT('Ctrl Pts',(-17.0548011239751,18.556437848963,12.));
#178999=CARTESIAN_POINT('Ctrl Pts',(-17.0793184636079,18.5657678479789,
12.));
#179000=CARTESIAN_POINT('Ctrl Pts',(-17.1039288260001,18.5750678188542,
12.));
#179001=CARTESIAN_POINT('Ctrl Pts',(-17.1286318741183,18.5843373717247,
12.));
#179002=CARTESIAN_POINT('Ctrl Pts',(-17.1534272741643,18.5935761222825,
12.));
#179003=CARTESIAN_POINT('Ctrl Pts',(-17.1783146940127,18.6027836898817,
12.));
#179004=CARTESIAN_POINT('Ctrl Pts',(-17.2032938019284,18.6119596959949,
12.));
#179005=CARTESIAN_POINT('Ctrl Pts',(-17.2283642650518,18.6211037624038,
12.));
#179006=CARTESIAN_POINT('Ctrl Pts',(-17.2535257482187,18.6302155097943,
12.));
#179007=CARTESIAN_POINT('Ctrl Pts',(-17.2787779120213,18.6392945554748,
12.));
#179008=CARTESIAN_POINT('Ctrl Pts',(-17.3041204135074,18.6483405141865,
12.));
#179009=CARTESIAN_POINT('Ctrl Pts',(-17.3295529098618,18.6573530024033,
12.));
#179010=CARTESIAN_POINT('Ctrl Pts',(-17.3550750612443,18.6663316416582,
12.));
#179011=CARTESIAN_POINT('Ctrl Pts',(-17.3806865340747,18.6752760624052,
12.));
#179012=CARTESIAN_POINT('Ctrl Pts',(-17.4063870038562,18.6841859073471,
12.));
#179013=CARTESIAN_POINT('Ctrl Pts',(-17.4321761588142,18.6930608357409,
12.));
#179014=CARTESIAN_POINT('Ctrl Pts',(-17.4580537012753,18.70190052503,12.));
#179015=CARTESIAN_POINT('Ctrl Pts',(-17.4840193397162,18.7107046613912,
12.));
#179016=CARTESIAN_POINT('Ctrl Pts',(-17.5100727820876,18.7194729318098,
12.));
#179017=CARTESIAN_POINT('Ctrl Pts',(-17.5362137287593,18.7282050157138,
12.));
#179018=CARTESIAN_POINT('Ctrl Pts',(-17.5624418653245,18.7369005764553,
12.));
#179019=CARTESIAN_POINT('Ctrl Pts',(-17.5887568561371,18.7455592536687,
12.));
#179020=CARTESIAN_POINT('Ctrl Pts',(-17.6151583357012,18.7541806530984,
12.));
#179021=CARTESIAN_POINT('Ctrl Pts',(-17.6416459210681,18.762764361321,12.));
#179022=CARTESIAN_POINT('Ctrl Pts',(-17.6682192274236,18.7713099642754,
12.));
#179023=CARTESIAN_POINT('Ctrl Pts',(-17.6948778823014,18.7798170641374,
12.));
#179024=CARTESIAN_POINT('Ctrl Pts',(-17.7216215409035,18.7882852976049,
12.));
#179025=CARTESIAN_POINT('Ctrl Pts',(-17.7484498996905,18.7967143519419,
12.));
#179026=CARTESIAN_POINT('Ctrl Pts',(-17.7753627137853,18.8051039860448,
12.));
#179027=CARTESIAN_POINT('Ctrl Pts',(-17.8023598011057,18.8134540340417,
12.));
#179028=CARTESIAN_POINT('Ctrl Pts',(-17.8294410311006,18.8217643886157,
12.));
#179029=CARTESIAN_POINT('Ctrl Pts',(-17.8566063174771,18.8300349895974,
12.));
#179030=CARTESIAN_POINT('Ctrl Pts',(-17.8784057509356,18.8366196462581,
12.));
#179031=CARTESIAN_POINT('Ctrl Pts',(-17.8947931177807,18.8415402351786,
12.));
#179032=CARTESIAN_POINT('Ctrl Pts',(-17.9057348246595,18.8448126709691,
12.));
#179033=CARTESIAN_POINT('Ctrl Pts',(-17.9112098770111,18.8464468996588,
12.));
#179034=CARTESIAN_POINT('',(-18.8464468996588,17.9112098770111,12.));
#179035=CARTESIAN_POINT('Origin',(0.,0.,12.));
#179036=CARTESIAN_POINT('',(-17.1452095830633,14.6513681262571,12.));
#179037=CARTESIAN_POINT('Ctrl Pts',(-18.8464468996588,17.9112098770111,
12.));
#179038=CARTESIAN_POINT('Ctrl Pts',(-18.8448126709726,17.9057348246611,
12.));
#179039=CARTESIAN_POINT('Ctrl Pts',(-18.8415402351882,17.8947931177853,
12.));
#179040=CARTESIAN_POINT('Ctrl Pts',(-18.8366196462746,17.8784057509434,
12.));
#179041=CARTESIAN_POINT('Ctrl Pts',(-18.8300349896187,17.8566063174871,
12.));
#179042=CARTESIAN_POINT('Ctrl Pts',(-18.8217643886368,17.8294410311105,
12.));
#179043=CARTESIAN_POINT('Ctrl Pts',(-18.8134540340581,17.8023598011135,
12.));
#179044=CARTESIAN_POINT('Ctrl Pts',(-18.8051039860543,17.7753627137898,
12.));
#179045=CARTESIAN_POINT('Ctrl Pts',(-18.7967143519444,17.7484498996916,
12.));
#179046=CARTESIAN_POINT('Ctrl Pts',(-18.7882852976016,17.7216215409019,
12.));
#179047=CARTESIAN_POINT('Ctrl Pts',(-18.7798170641305,17.6948778822981,
12.));
#179048=CARTESIAN_POINT('Ctrl Pts',(-18.7713099642673,17.6682192274197,
12.));
#179049=CARTESIAN_POINT('Ctrl Pts',(-18.7627643613139,17.6416459210646,
12.));
#179050=CARTESIAN_POINT('Ctrl Pts',(-18.7541806530935,17.6151583356988,
12.));
#179051=CARTESIAN_POINT('Ctrl Pts',(-18.7455592536667,17.5887568561361,
12.));
#179052=CARTESIAN_POINT('Ctrl Pts',(-18.7369005764558,17.5624418653248,
12.));
#179053=CARTESIAN_POINT('Ctrl Pts',(-18.728205015716,17.5362137287604,12.));
#179054=CARTESIAN_POINT('Ctrl Pts',(-18.7194729318128,17.5100727820891,
12.));
#179055=CARTESIAN_POINT('Ctrl Pts',(-18.7107046613941,17.4840193397176,
12.));
#179056=CARTESIAN_POINT('Ctrl Pts',(-18.7019005250322,17.4580537012764,
12.));
#179057=CARTESIAN_POINT('Ctrl Pts',(-18.6930608357421,17.4321761588148,
12.));
#179058=CARTESIAN_POINT('Ctrl Pts',(-18.6841859073472,17.4063870038563,
12.));
#179059=CARTESIAN_POINT('Ctrl Pts',(-18.6752760624045,17.3806865340744,
12.));
#179060=CARTESIAN_POINT('Ctrl Pts',(-18.6663316416569,17.3550750612438,
12.));
#179061=CARTESIAN_POINT('Ctrl Pts',(-18.6573530024019,17.3295529098612,
12.));
#179062=CARTESIAN_POINT('Ctrl Pts',(-18.6483405141853,17.3041204135069,
12.));
#179063=CARTESIAN_POINT('Ctrl Pts',(-18.639294555474,17.278777912021,12.));
#179064=CARTESIAN_POINT('Ctrl Pts',(-18.630215509794,17.2535257482186,12.));
#179065=CARTESIAN_POINT('Ctrl Pts',(-18.6211037624041,17.2283642650519,
12.));
#179066=CARTESIAN_POINT('Ctrl Pts',(-18.6119596959957,17.2032938019288,
12.));
#179067=CARTESIAN_POINT('Ctrl Pts',(-18.6027836898826,17.1783146940131,
12.));
#179068=CARTESIAN_POINT('Ctrl Pts',(-18.5935761222833,17.1534272741646,
12.));
#179069=CARTESIAN_POINT('Ctrl Pts',(-18.5843373717253,17.1286318741185,
12.));
#179070=CARTESIAN_POINT('Ctrl Pts',(-18.5750678188543,17.1039288260001,
12.));
#179071=CARTESIAN_POINT('Ctrl Pts',(-18.5657678479788,17.0793184636079,
12.));
#179072=CARTESIAN_POINT('Ctrl Pts',(-18.5564378489628,17.0548011239751,
12.));
#179073=CARTESIAN_POINT('Ctrl Pts',(-18.5470782182089,17.030377148174,12.));
#179074=CARTESIAN_POINT('Ctrl Pts',(-18.5376893576961,17.0060468805099,
12.));
#179075=CARTESIAN_POINT('Ctrl Pts',(-18.5282716744198,16.9818106680382,
12.));
#179076=CARTESIAN_POINT('Ctrl Pts',(-18.518825579666,16.957668859934,12.));
#179077=CARTESIAN_POINT('Ctrl Pts',(-18.5093514883835,16.9336218069353,
12.));
#179078=CARTESIAN_POINT('Ctrl Pts',(-18.4998498184619,16.9096698606942,
12.));
#179079=CARTESIAN_POINT('Ctrl Pts',(-18.4903209902226,16.8858133733086,
12.));
#179080=CARTESIAN_POINT('Ctrl Pts',(-18.4807654268769,16.8620526977169,
12.));
#179081=CARTESIAN_POINT('Ctrl Pts',(-18.4711835548622,16.8383881879707,
12.));
#179082=CARTESIAN_POINT('Ctrl Pts',(-18.4615758042305,16.8148201995472,
12.));
#179083=CARTESIAN_POINT('Ctrl Pts',(-18.4519426090124,16.791349089629,12.));
#179084=CARTESIAN_POINT('Ctrl Pts',(-18.4422844076099,16.7679752173992,
12.));
#179085=CARTESIAN_POINT('Ctrl Pts',(-18.4326016431392,16.7446989442882,
12.));
#179086=CARTESIAN_POINT('Ctrl Pts',(-18.4228947633186,16.7215206338818,
12.));
#179087=CARTESIAN_POINT('Ctrl Pts',(-18.413164220399,16.698440651849,12.));
#179088=CARTESIAN_POINT('Ctrl Pts',(-18.4034104710789,16.6754593658513,
12.));
#179089=CARTESIAN_POINT('Ctrl Pts',(-18.3936339764332,16.6525771454513,
12.));
#179090=CARTESIAN_POINT('Ctrl Pts',(-18.3838352018327,16.6297943620056,
12.));
#179091=CARTESIAN_POINT('Ctrl Pts',(-18.3740146168879,16.6071113885711,
12.));
#179092=CARTESIAN_POINT('Ctrl Pts',(-18.364172695589,16.5845286000218,12.));
#179093=CARTESIAN_POINT('Ctrl Pts',(-18.3543099164331,16.5620463731414,
12.));
#179094=CARTESIAN_POINT('Ctrl Pts',(-18.3444267625601,16.5396650867139,
12.));
#179095=CARTESIAN_POINT('Ctrl Pts',(-18.3345237218864,16.5173851216045,
12.));
#179096=CARTESIAN_POINT('Ctrl Pts',(-18.3246012872468,16.4952068608344,
12.));
#179097=CARTESIAN_POINT('Ctrl Pts',(-18.3146599565229,16.4731306896439,
12.));
#179098=CARTESIAN_POINT('Ctrl Pts',(-18.3047002326858,16.4511569955231,
12.));
#179099=CARTESIAN_POINT('Ctrl Pts',(-18.2947226238509,16.4292861682377,
12.));
#179100=CARTESIAN_POINT('Ctrl Pts',(-18.2847276433308,16.4075185998454,
12.));
#179101=CARTESIAN_POINT('Ctrl Pts',(-18.2747158096934,16.385854684708,12.));
#179102=CARTESIAN_POINT('Ctrl Pts',(-18.2646876468169,16.3642948194869,
12.));
#179103=CARTESIAN_POINT('Ctrl Pts',(-18.2546436839609,16.342839403159,12.));
#179104=CARTESIAN_POINT('Ctrl Pts',(-18.2445844558742,16.3214888370988,
12.));
#179105=CARTESIAN_POINT('Ctrl Pts',(-18.2345105028981,16.3002435251378,
12.));
#179106=CARTESIAN_POINT('Ctrl Pts',(-18.2244223710745,16.2791038736223,
12.));
#179107=CARTESIAN_POINT('Ctrl Pts',(-18.214320612253,16.2580702914615,12.));
#179108=CARTESIAN_POINT('Ctrl Pts',(-18.2042057842037,16.237143190164,12.));
#179109=CARTESIAN_POINT('Ctrl Pts',(-18.1940784507232,16.2163229838878,
12.));
#179110=CARTESIAN_POINT('Ctrl Pts',(-18.1839391817335,16.1956100895076,
12.));
#179111=CARTESIAN_POINT('Ctrl Pts',(-18.1737885533852,16.1750049266673,
12.));
#179112=CARTESIAN_POINT('Ctrl Pts',(-18.1636271481616,16.1545079178261,
12.));
#179113=CARTESIAN_POINT('Ctrl Pts',(-18.1534555549851,16.1341194882987,
12.));
#179114=CARTESIAN_POINT('Ctrl Pts',(-18.1432743693231,16.113840066279,12.));
#179115=CARTESIAN_POINT('Ctrl Pts',(-18.1330841933099,16.0936700829108,
12.));
#179116=CARTESIAN_POINT('Ctrl Pts',(-18.1228856358746,16.0736099723664,
12.));
#179117=CARTESIAN_POINT('Ctrl Pts',(-18.1126793128688,16.0536601719124,
12.));
#179118=CARTESIAN_POINT('Ctrl Pts',(-18.1024658471966,16.0338211219693,
12.));
#179119=CARTESIAN_POINT('Ctrl Pts',(-18.0922458689464,16.0140932661612,
12.));
#179120=CARTESIAN_POINT('Ctrl Pts',(-18.0820200155239,15.9944770513616,
12.));
#179121=CARTESIAN_POINT('Ctrl Pts',(-18.071788931796,15.9749729277848,12.));
#179122=CARTESIAN_POINT('Ctrl Pts',(-18.061553270236,15.9555813490645,12.));
#179123=CARTESIAN_POINT('Ctrl Pts',(-18.0513136910691,15.9363027723244,
12.));
#179124=CARTESIAN_POINT('Ctrl Pts',(-18.0410708624208,15.9171376582436,
12.));
#179125=CARTESIAN_POINT('Ctrl Pts',(-18.0308254604638,15.8980864711043,
12.));
#179126=CARTESIAN_POINT('Ctrl Pts',(-18.0205781695773,15.8791496788685,
12.));
#179127=CARTESIAN_POINT('Ctrl Pts',(-18.010329682521,15.8603277532834,12.));
#179128=CARTESIAN_POINT('Ctrl Pts',(-18.0000807006055,15.8416211699681,
12.));
#179129=CARTESIAN_POINT('Ctrl Pts',(-17.9898319338664,15.8230304084963,
12.));
#179130=CARTESIAN_POINT('Ctrl Pts',(-17.9795841012383,15.8045559524674,
12.));
#179131=CARTESIAN_POINT('Ctrl Pts',(-17.9693379307297,15.786198289572,12.));
#179132=CARTESIAN_POINT('Ctrl Pts',(-17.9590941596236,15.7679579117072,
12.));
#179133=CARTESIAN_POINT('Ctrl Pts',(-17.9488535346776,15.7498353150856,
12.));
#179134=CARTESIAN_POINT('Ctrl Pts',(-17.9386168123261,15.7318310003334,
12.));
#179135=CARTESIAN_POINT('Ctrl Pts',(-17.9283847588837,15.713945472584,12.));
#179136=CARTESIAN_POINT('Ctrl Pts',(-17.918158150746,15.6961792415526,12.));
#179137=CARTESIAN_POINT('Ctrl Pts',(-17.9079377746118,15.6785328216467,
12.));
#179138=CARTESIAN_POINT('Ctrl Pts',(-17.8977244277247,15.6610067321036,
12.));
#179139=CARTESIAN_POINT('Ctrl Pts',(-17.8875189181095,15.6436014971088,
12.));
#179140=CARTESIAN_POINT('Ctrl Pts',(-17.8773220648125,15.6263176459107,
12.));
#179141=CARTESIAN_POINT('Ctrl Pts',(-17.8671346981388,15.6091557129205,
12.));
#179142=CARTESIAN_POINT('Ctrl Pts',(-17.8569576598996,15.5921162378183,
12.));
#179143=CARTESIAN_POINT('Ctrl Pts',(-17.8467918036977,15.5751997657153,
12.));
#179144=CARTESIAN_POINT('Ctrl Pts',(-17.8366379952078,15.5584068472976,
12.));
#179145=CARTESIAN_POINT('Ctrl Pts',(-17.8264971124606,15.5417380389639,
12.));
#179146=CARTESIAN_POINT('Ctrl Pts',(-17.8163700461263,15.5251939029558,
12.));
#179147=CARTESIAN_POINT('Ctrl Pts',(-17.8062576997964,15.5087750074728,
12.));
#179148=CARTESIAN_POINT('Ctrl Pts',(-17.7961609903161,15.4924819268529,
12.));
#179149=CARTESIAN_POINT('Ctrl Pts',(-17.7860808481229,15.4763152417506,
12.));
#179150=CARTESIAN_POINT('Ctrl Pts',(-17.7760182175817,15.4602755393019,
12.));
#179151=CARTESIAN_POINT('Ctrl Pts',(-17.765974057326,15.4443634132865,12.));
#179152=CARTESIAN_POINT('Ctrl Pts',(-17.7559493405871,15.4285794642658,
12.));
#179153=CARTESIAN_POINT('Ctrl Pts',(-17.7459450555803,15.4129242997828,
12.));
#179154=CARTESIAN_POINT('Ctrl Pts',(-17.7359622059143,15.3973985345796,
12.));
#179155=CARTESIAN_POINT('Ctrl Pts',(-17.7260018109923,15.3820027907965,
12.));
#179156=CARTESIAN_POINT('Ctrl Pts',(-17.7160649064208,15.3667376981702,
12.));
#179157=CARTESIAN_POINT('Ctrl Pts',(-17.7061525444044,15.3516038942064,
12.));
#179158=CARTESIAN_POINT('Ctrl Pts',(-17.6962657941984,15.3366020244069,
12.));
#179159=CARTESIAN_POINT('Ctrl Pts',(-17.6864057426052,15.3217327425341,
12.));
#179160=CARTESIAN_POINT('Ctrl Pts',(-17.6765734944559,15.3069967108501,
12.));
#179161=CARTESIAN_POINT('Ctrl Pts',(-17.6667701731041,15.2923946003598,
12.));
#179162=CARTESIAN_POINT('Ctrl Pts',(-17.6569969209,15.2779270910238,12.));
#179163=CARTESIAN_POINT('Ctrl Pts',(-17.6472548997329,15.263594872029,12.));
#179164=CARTESIAN_POINT('Ctrl Pts',(-17.637545291637,15.2493986421091,12.));
#179165=CARTESIAN_POINT('Ctrl Pts',(-17.6278692993765,15.2353391098367,
12.));
#179166=CARTESIAN_POINT('Ctrl Pts',(-17.6182281470467,15.22141699392,12.));
#179167=CARTESIAN_POINT('Ctrl Pts',(-17.6086230806497,15.2076330234686,
12.));
#179168=CARTESIAN_POINT('Ctrl Pts',(-17.5990553687595,15.1939879383268,
12.));
#179169=CARTESIAN_POINT('Ctrl Pts',(-17.5895263032592,15.1804824894605,
12.));
#179170=CARTESIAN_POINT('Ctrl Pts',(-17.5800372000539,15.1671174393136,
12.));
#179171=CARTESIAN_POINT('Ctrl Pts',(-17.570589399803,15.1538935621714,12.));
#179172=CARTESIAN_POINT('Ctrl Pts',(-17.5611842686196,15.1408116444877,
12.));
#179173=CARTESIAN_POINT('Ctrl Pts',(-17.5518231989122,15.127872485314,12.));
#179174=CARTESIAN_POINT('Ctrl Pts',(-17.5425076102966,15.1150768967729,
12.));
#179175=CARTESIAN_POINT('Ctrl Pts',(-17.5332389504829,15.1024257045033,
12.));
#179176=CARTESIAN_POINT('Ctrl Pts',(-17.5240186961788,15.0899197481082,
12.));
#179177=CARTESIAN_POINT('Ctrl Pts',(-17.5148483539684,15.0775598815748,
12.));
#179178=CARTESIAN_POINT('Ctrl Pts',(-17.5057294613874,15.0653469738306,
12.));
#179179=CARTESIAN_POINT('Ctrl Pts',(-17.4966635880245,15.0532819093085,
12.));
#179180=CARTESIAN_POINT('Ctrl Pts',(-17.4876523366178,15.0413655884993,
12.));
#179181=CARTESIAN_POINT('Ctrl Pts',(-17.4786973441417,15.029598928488,12.));
#179182=CARTESIAN_POINT('Ctrl Pts',(-17.4698002829357,15.0179828635086,
12.));
#179183=CARTESIAN_POINT('Ctrl Pts',(-17.4609628621418,15.0065183456921,
12.));
#179184=CARTESIAN_POINT('Ctrl Pts',(-17.4521868291004,14.9952063457778,
12.));
#179185=CARTESIAN_POINT('Ctrl Pts',(-17.4434739707773,14.9840478538358,
12.));
#179186=CARTESIAN_POINT('Ctrl Pts',(-17.4348261151396,14.9730438799452,
12.));
#179187=CARTESIAN_POINT('Ctrl Pts',(-17.426245132709,14.9621954549827,12.));
#179188=CARTESIAN_POINT('Ctrl Pts',(-17.4177329382828,14.9515036315143,
12.));
#179189=CARTESIAN_POINT('Ctrl Pts',(-17.4092914926071,14.940969484645,12.));
#179190=CARTESIAN_POINT('Ctrl Pts',(-17.4009228040749,14.9305941128757,
12.));
#179191=CARTESIAN_POINT('Ctrl Pts',(-17.3926289303986,14.9203786389342,
12.));
#179192=CARTESIAN_POINT('Ctrl Pts',(-17.3844119809824,14.9103242110057,
12.));
#179193=CARTESIAN_POINT('Ctrl Pts',(-17.3762741193076,14.900432003961,12.));
#179194=CARTESIAN_POINT('Ctrl Pts',(-17.3682175653235,14.8907032205788,
12.));
#179195=CARTESIAN_POINT('Ctrl Pts',(-17.3602445978161,14.8811390927423,
12.));
#179196=CARTESIAN_POINT('Ctrl Pts',(-17.3523575568645,14.8717408826955,
12.));
#179197=CARTESIAN_POINT('Ctrl Pts',(-17.3445588463475,14.8625098843417,
12.));
#179198=CARTESIAN_POINT('Ctrl Pts',(-17.336850936485,14.8534474245433,12.));
#179199=CARTESIAN_POINT('Ctrl Pts',(-17.3292363662605,14.8445548643508,
12.));
#179200=CARTESIAN_POINT('Ctrl Pts',(-17.3217177462101,14.8358336004197,
12.));
#179201=CARTESIAN_POINT('Ctrl Pts',(-17.3142977632659,14.8272850675379,
12.));
#179202=CARTESIAN_POINT('Ctrl Pts',(-17.3069791853706,14.8189107410162,
12.));
#179203=CARTESIAN_POINT('Ctrl Pts',(-17.299764866148,14.8107121391035,12.));
#179204=CARTESIAN_POINT('Ctrl Pts',(-17.2926577496513,14.8026908254276,
12.));
#179205=CARTESIAN_POINT('Ctrl Pts',(-17.2856608733196,14.7948484105249,
12.));
#179206=CARTESIAN_POINT('Ctrl Pts',(-17.2787773704849,14.787186553128,12.));
#179207=CARTESIAN_POINT('Ctrl Pts',(-17.2720104735194,14.7797069617804,
12.));
#179208=CARTESIAN_POINT('Ctrl Pts',(-17.2653635155319,14.7724113956731,
12.));
#179209=CARTESIAN_POINT('Ctrl Pts',(-17.2588399401465,14.7653016697591,
12.));
#179210=CARTESIAN_POINT('Ctrl Pts',(-17.2524433146837,14.7583796616617,
12.));
#179211=CARTESIAN_POINT('Ctrl Pts',(-17.2461773413288,14.7516473175124,
12.));
#179212=CARTESIAN_POINT('Ctrl Pts',(-17.2400458713565,14.7451066593792,
12.));
#179213=CARTESIAN_POINT('Ctrl Pts',(-17.2340529062076,14.7387597858116,
12.));
#179214=CARTESIAN_POINT('Ctrl Pts',(-17.2282025904314,14.7326088681163,
12.));
#179215=CARTESIAN_POINT('Ctrl Pts',(-17.2224992099667,14.7266561494282,
12.));
#179216=CARTESIAN_POINT('Ctrl Pts',(-17.2169471814256,14.7209039390327,
12.));
#179217=CARTESIAN_POINT('Ctrl Pts',(-17.2115510835989,14.7153546289339,
12.));
#179218=CARTESIAN_POINT('Ctrl Pts',(-17.2063157097315,14.7100107213586,
12.));
#179219=CARTESIAN_POINT('Ctrl Pts',(-17.2012461084268,14.7048748502663,
12.));
#179220=CARTESIAN_POINT('Ctrl Pts',(-17.1963476411694,14.699949811582,12.));
#179221=CARTESIAN_POINT('Ctrl Pts',(-17.1916259308415,14.6952385361705,
12.));
#179222=CARTESIAN_POINT('Ctrl Pts',(-17.1870867909918,14.6907440526958,
12.));
#179223=CARTESIAN_POINT('Ctrl Pts',(-17.182736158472,14.686469452232,12.));
#179224=CARTESIAN_POINT('Ctrl Pts',(-17.1785800350826,14.6824178576167,
12.));
#179225=CARTESIAN_POINT('Ctrl Pts',(-17.1746247499057,14.6785925615677,
12.));
#179226=CARTESIAN_POINT('Ctrl Pts',(-17.1708771619129,14.6749971333867,
12.));
#179227=CARTESIAN_POINT('Ctrl Pts',(-17.167344972302,14.671635583332,12.));
#179228=CARTESIAN_POINT('Ctrl Pts',(-17.1640366762305,14.6685123374423,
12.));
#179229=CARTESIAN_POINT('Ctrl Pts',(-17.1609609517369,14.6656319165057,
12.));
#179230=CARTESIAN_POINT('Ctrl Pts',(-17.1581262646789,14.6629987285992,
12.));
#179231=CARTESIAN_POINT('Ctrl Pts',(-17.1555401986401,14.6606167169642,
12.));
#179232=CARTESIAN_POINT('Ctrl Pts',(-17.1532107762718,14.6584900555302,
12.));
#179233=CARTESIAN_POINT('Ctrl Pts',(-17.1511476869496,14.6566237952435,
12.));
#179234=CARTESIAN_POINT('Ctrl Pts',(-17.1493641837558,14.655024862281,12.));
#179235=CARTESIAN_POINT('Ctrl Pts',(-17.147876394491,14.6537016966184,12.));
#179236=CARTESIAN_POINT('Ctrl Pts',(-17.1466998098673,14.6526624064978,
12.));
#179237=CARTESIAN_POINT('Ctrl Pts',(-17.1458462295271,14.6519131634508,
12.));
#179238=CARTESIAN_POINT('Ctrl Pts',(-17.1454262858043,14.6515481598068,
12.));
#179239=CARTESIAN_POINT('Ctrl Pts',(-17.1452600887037,14.6514066997196,
12.));
#179240=CARTESIAN_POINT('Ctrl Pts',(-17.1452153999142,14.6513711852843,
12.));
#179241=CARTESIAN_POINT('Ctrl Pts',(-17.1452095830633,14.6513681262571,
12.));
#179242=CARTESIAN_POINT('',(-16.7207683102834,14.2886635873976,12.));
#179243=CARTESIAN_POINT('',(-8.17248635976757,6.98376450772883,12.));
#179244=CARTESIAN_POINT('',(-16.6581946899465,13.5924445804218,12.));
#179245=CARTESIAN_POINT('Origin',(-17.0455945664569,13.9085479427572,12.));
#179246=CARTESIAN_POINT('',(-17.4407513054162,12.572596943457,12.));
#179247=CARTESIAN_POINT('Origin',(-6.00167842331873E-13,4.9889687874677E-13,
12.));
#179248=CARTESIAN_POINT('',(-18.1294424696716,12.4528436808172,12.));
#179249=CARTESIAN_POINT('Origin',(-17.846350172984,12.8649829188862,12.));
#179250=CARTESIAN_POINT('',(-18.5896416359912,12.7689476255363,12.));
#179251=CARTESIAN_POINT('',(-9.29482081799561,6.38447381276812,12.));
#179252=CARTESIAN_POINT('',(-22.1787195904339,13.5685075571671,12.));
#179253=CARTESIAN_POINT('Ctrl Pts',(-18.5896416359912,12.7689476255363,
12.));
#179254=CARTESIAN_POINT('Ctrl Pts',(-18.5896460962961,12.7689524524484,
12.));
#179255=CARTESIAN_POINT('Ctrl Pts',(-18.5896919669158,12.7689864266924,
12.));
#179256=CARTESIAN_POINT('Ctrl Pts',(-18.589871621842,12.7691103481996,12.));
#179257=CARTESIAN_POINT('Ctrl Pts',(-18.590332877722,12.7694215127923,12.));
#179258=CARTESIAN_POINT('Ctrl Pts',(-18.5912775137806,12.7700520897174,
12.));
#179259=CARTESIAN_POINT('Ctrl Pts',(-18.5925859134582,12.7709195951153,
12.));
#179260=CARTESIAN_POINT('Ctrl Pts',(-18.5942490615409,12.7720142287169,
12.));
#179261=CARTESIAN_POINT('Ctrl Pts',(-18.5962551167772,12.7733231262107,
12.));
#179262=CARTESIAN_POINT('Ctrl Pts',(-18.5985917525949,12.7748328937639,
12.));
#179263=CARTESIAN_POINT('Ctrl Pts',(-18.6012488486708,12.7765325225082,
12.));
#179264=CARTESIAN_POINT('Ctrl Pts',(-18.6042190183703,12.7784139605067,
12.));
#179265=CARTESIAN_POINT('Ctrl Pts',(-18.6074961535723,12.7804705387658,
12.));
#179266=CARTESIAN_POINT('Ctrl Pts',(-18.611074482622,12.7826959526924,12.));
#179267=CARTESIAN_POINT('Ctrl Pts',(-18.6149475565189,12.78508316579,12.));
#179268=CARTESIAN_POINT('Ctrl Pts',(-18.6191087624752,12.7876249657834,
12.));
#179269=CARTESIAN_POINT('Ctrl Pts',(-18.6235516265575,12.7903142925234,
12.));
#179270=CARTESIAN_POINT('Ctrl Pts',(-18.6282702819371,12.7931447451556,
12.));
#179271=CARTESIAN_POINT('Ctrl Pts',(-18.6332595057005,12.7961106222251,
12.));
#179272=CARTESIAN_POINT('Ctrl Pts',(-18.63851447924,12.7992066625264,12.));
#179273=CARTESIAN_POINT('Ctrl Pts',(-18.6440306327457,12.8024278770153,
12.));
#179274=CARTESIAN_POINT('Ctrl Pts',(-18.6498034438986,12.805769331162,12.));
#179275=CARTESIAN_POINT('Ctrl Pts',(-18.6558284825772,12.8092261933858,
12.));
#179276=CARTESIAN_POINT('Ctrl Pts',(-18.6621014624746,12.8127937909632,
12.));
#179277=CARTESIAN_POINT('Ctrl Pts',(-18.6686182952798,12.8164676687361,
12.));
#179278=CARTESIAN_POINT('Ctrl Pts',(-18.6753751301091,12.8202436318473,
12.));
#179279=CARTESIAN_POINT('Ctrl Pts',(-18.6823683094139,12.8241176980016,
12.));
#179280=CARTESIAN_POINT('Ctrl Pts',(-18.6895943376172,12.8280860635231,
12.));
#179281=CARTESIAN_POINT('Ctrl Pts',(-18.6970498410173,12.832145059979,12.));
#179282=CARTESIAN_POINT('Ctrl Pts',(-18.7047315436296,12.8362911280362,
12.));
#179283=CARTESIAN_POINT('Ctrl Pts',(-18.7126362754446,12.8405208263432,
12.));
#179284=CARTESIAN_POINT('Ctrl Pts',(-18.7207609737701,12.8448308329494,
12.));
#179285=CARTESIAN_POINT('Ctrl Pts',(-18.7291026886552,12.849217951159,12.));
#179286=CARTESIAN_POINT('Ctrl Pts',(-18.7376585820851,12.8536791086315,
12.));
#179287=CARTESIAN_POINT('Ctrl Pts',(-18.7464259171248,12.8582113455644,
12.));
#179288=CARTESIAN_POINT('Ctrl Pts',(-18.7554020493888,12.8628118054172,
12.));
#179289=CARTESIAN_POINT('Ctrl Pts',(-18.7645844169568,12.8674777239656,
12.));
#179290=CARTESIAN_POINT('Ctrl Pts',(-18.7739705329029,12.8722064211814,
12.));
#179291=CARTESIAN_POINT('Ctrl Pts',(-18.7835579840481,12.8769952998097,
12.));
#179292=CARTESIAN_POINT('Ctrl Pts',(-18.7933444285867,12.8818418427474,
12.));
#179293=CARTESIAN_POINT('Ctrl Pts',(-18.8033275941939,12.8867436109543,
12.));
#179294=CARTESIAN_POINT('Ctrl Pts',(-18.8135052757815,12.8916982409931,
12.));
#179295=CARTESIAN_POINT('Ctrl Pts',(-18.8238753319124,12.8967034410752,
12.));
#179296=CARTESIAN_POINT('Ctrl Pts',(-18.834435681259,12.9017569871738,12.));
#179297=CARTESIAN_POINT('Ctrl Pts',(-18.8451842990986,12.9068567191856,
12.));
#179298=CARTESIAN_POINT('Ctrl Pts',(-18.8561192136201,12.9120005369066,
12.));
#179299=CARTESIAN_POINT('Ctrl Pts',(-18.8672385038328,12.9171863977047,
12.));
#179300=CARTESIAN_POINT('Ctrl Pts',(-18.8785402977528,12.9224123144982,
12.));
#179301=CARTESIAN_POINT('Ctrl Pts',(-18.8900227704888,12.9276763536372,
12.));
#179302=CARTESIAN_POINT('Ctrl Pts',(-18.9016841423402,12.9329766328184,
12.));
#179303=CARTESIAN_POINT('Ctrl Pts',(-18.9135226769466,12.9383113190375,
12.));
#179304=CARTESIAN_POINT('Ctrl Pts',(-18.9255366795196,12.9436786266106,
12.));
#179305=CARTESIAN_POINT('Ctrl Pts',(-18.9377244950435,12.9490768151821,
12.));
#179306=CARTESIAN_POINT('Ctrl Pts',(-18.9500845064714,12.9545041877377,
12.));
#179307=CARTESIAN_POINT('Ctrl Pts',(-18.9626151329226,12.9599590886317,
12.));
#179308=CARTESIAN_POINT('Ctrl Pts',(-18.9753148284473,12.9654399021868,
12.));
#179309=CARTESIAN_POINT('Ctrl Pts',(-18.9881820807585,12.9709450512747,
12.));
#179310=CARTESIAN_POINT('Ctrl Pts',(-19.0012154099792,12.9764729959206,
12.));
#179311=CARTESIAN_POINT('Ctrl Pts',(-19.014413367335,12.9820222318716,12.));
#179312=CARTESIAN_POINT('Ctrl Pts',(-19.0277745339909,12.9875912893003,
12.));
#179313=CARTESIAN_POINT('Ctrl Pts',(-19.0412975200398,12.9931787316514,
12.));
#179314=CARTESIAN_POINT('Ctrl Pts',(-19.0549809634354,12.9987831544502,
12.));
#179315=CARTESIAN_POINT('Ctrl Pts',(-19.0688235289437,13.0044031841382,
12.));
#179316=CARTESIAN_POINT('Ctrl Pts',(-19.0828239070484,13.0100374768788,
12.));
#179317=CARTESIAN_POINT('Ctrl Pts',(-19.0969808131228,13.0156847176096,
12.));
#179318=CARTESIAN_POINT('Ctrl Pts',(-19.111292986631,13.0213436191328,12.));
#179319=CARTESIAN_POINT('Ctrl Pts',(-19.1257591903099,13.0270129211976,
12.));
#179320=CARTESIAN_POINT('Ctrl Pts',(-19.1403782093386,13.0326913895838,
12.));
#179321=CARTESIAN_POINT('Ctrl Pts',(-19.155148850523,13.0383778152068,12.));
#179322=CARTESIAN_POINT('Ctrl Pts',(-19.1700699416622,13.0440710133772,
12.));
#179323=CARTESIAN_POINT('Ctrl Pts',(-19.1851403308825,13.0497698230441,
12.));
#179324=CARTESIAN_POINT('Ctrl Pts',(-19.2003588859772,13.0554731060538,
12.));
#179325=CARTESIAN_POINT('Ctrl Pts',(-19.2157244937142,13.0611797463915,
12.));
#179326=CARTESIAN_POINT('Ctrl Pts',(-19.2312360592033,13.0668886494795,
12.));
#179327=CARTESIAN_POINT('Ctrl Pts',(-19.2468925053989,13.0725987415859,
12.));
#179328=CARTESIAN_POINT('Ctrl Pts',(-19.2626927725596,13.0783089692118,
12.));
#179329=CARTESIAN_POINT('Ctrl Pts',(-19.2786358177198,13.0840182984949,
12.));
#179330=CARTESIAN_POINT('Ctrl Pts',(-19.2947206141247,13.0897257145968,
12.));
#179331=CARTESIAN_POINT('Ctrl Pts',(-19.310946150736,13.0954302211479,12.));
#179332=CARTESIAN_POINT('Ctrl Pts',(-19.3273114318269,13.1011308397591,
12.));
#179333=CARTESIAN_POINT('Ctrl Pts',(-19.3438154765395,13.1068266095186,
12.));
#179334=CARTESIAN_POINT('Ctrl Pts',(-19.3604573184515,13.1125165865022,
12.));
#179335=CARTESIAN_POINT('Ctrl Pts',(-19.3772360051091,13.118199843271,12.));
#179336=CARTESIAN_POINT('Ctrl Pts',(-19.3941505976263,13.1238754684177,
12.));
#179337=CARTESIAN_POINT('Ctrl Pts',(-19.4112001703557,13.1295425661634,
12.));
#179338=CARTESIAN_POINT('Ctrl Pts',(-19.4283838105262,13.1352002559438,
12.));
#179339=CARTESIAN_POINT('Ctrl Pts',(-19.4457006178876,13.1408476720061,
12.));
#179340=CARTESIAN_POINT('Ctrl Pts',(-19.4631497043258,13.1464839629971,
12.));
#179341=CARTESIAN_POINT('Ctrl Pts',(-19.4807301935268,13.1521082915853,
12.));
#179342=CARTESIAN_POINT('Ctrl Pts',(-19.4984412207082,13.1577198341245,
12.));
#179343=CARTESIAN_POINT('Ctrl Pts',(-19.5162819323213,13.1633177803101,
12.));
#179344=CARTESIAN_POINT('Ctrl Pts',(-19.5342514857562,13.168901332843,12.));
#179345=CARTESIAN_POINT('Ctrl Pts',(-19.5523490490244,13.1744697070911,
12.));
#179346=CARTESIAN_POINT('Ctrl Pts',(-19.5705738004667,13.1800221307673,
12.));
#179347=CARTESIAN_POINT('Ctrl Pts',(-19.5889249285338,13.1855578436471,
12.));
#179348=CARTESIAN_POINT('Ctrl Pts',(-19.6074016315414,13.1910760972814,
12.));
#179349=CARTESIAN_POINT('Ctrl Pts',(-19.6260031174244,13.1965761547151,
12.));
#179350=CARTESIAN_POINT('Ctrl Pts',(-19.6447286034772,13.2020572902065,
12.));
#179351=CARTESIAN_POINT('Ctrl Pts',(-19.6635773160936,13.2075187889529,
12.));
#179352=CARTESIAN_POINT('Ctrl Pts',(-19.6825484905823,13.2129599468485,
12.));
#179353=CARTESIAN_POINT('Ctrl Pts',(-19.7016413709685,13.2183800702436,
12.));
#179354=CARTESIAN_POINT('Ctrl Pts',(-19.7208552097868,13.2237784757065,
12.));
#179355=CARTESIAN_POINT('Ctrl Pts',(-19.7401892678697,13.2291544897899,
12.));
#179356=CARTESIAN_POINT('Ctrl Pts',(-19.7596428141168,13.2345074487963,
12.));
#179357=CARTESIAN_POINT('Ctrl Pts',(-19.7792151253289,13.2398366985675,
12.));
#179358=CARTESIAN_POINT('Ctrl Pts',(-19.7989054860495,13.2451415942805,
12.));
#179359=CARTESIAN_POINT('Ctrl Pts',(-19.8187131883917,13.2504215002457,
12.));
#179360=CARTESIAN_POINT('Ctrl Pts',(-19.8386375318634,13.2556757897086,
12.));
#179361=CARTESIAN_POINT('Ctrl Pts',(-19.8586778231715,13.2609038446529,
12.));
#179362=CARTESIAN_POINT('Ctrl Pts',(-19.8788333760577,13.2661050556132,
12.));
#179363=CARTESIAN_POINT('Ctrl Pts',(-19.8991035111745,13.271278821502,12.));
#179364=CARTESIAN_POINT('Ctrl Pts',(-19.9194875559422,13.2764245494357,
12.));
#179365=CARTESIAN_POINT('Ctrl Pts',(-19.9399848444019,13.2815416545663,
12.));
#179366=CARTESIAN_POINT('Ctrl Pts',(-19.9605947170586,13.286629559915,12.));
#179367=CARTESIAN_POINT('Ctrl Pts',(-19.981316520717,13.2916876962094,12.));
#179368=CARTESIAN_POINT('Ctrl Pts',(-20.0021496083738,13.2967155017306,
12.));
#179369=CARTESIAN_POINT('Ctrl Pts',(-20.0230933391038,13.3017124221637,
12.));
#179370=CARTESIAN_POINT('Ctrl Pts',(-20.0441470779345,13.3066779104515,
12.));
#179371=CARTESIAN_POINT('Ctrl Pts',(-20.0653101957188,13.3116114266515,
12.));
#179372=CARTESIAN_POINT('Ctrl Pts',(-20.0865820689883,13.3165124377962,
12.));
#179373=CARTESIAN_POINT('Ctrl Pts',(-20.1079620798375,13.3213804177587,
12.));
#179374=CARTESIAN_POINT('Ctrl Pts',(-20.1294496158402,13.3262148471226,
12.));
#179375=CARTESIAN_POINT('Ctrl Pts',(-20.1510440699474,13.3310152130564,
12.));
#179376=CARTESIAN_POINT('Ctrl Pts',(-20.1727448403817,13.3357810091903,
12.));
#179377=CARTESIAN_POINT('Ctrl Pts',(-20.1945513305235,13.3405117354971,
12.));
#179378=CARTESIAN_POINT('Ctrl Pts',(-20.216462948786,13.3452068981766,12.));
#179379=CARTESIAN_POINT('Ctrl Pts',(-20.2384791085359,13.3498660095386,
12.));
#179380=CARTESIAN_POINT('Ctrl Pts',(-20.2605992280122,13.3544885878889,
12.));
#179381=CARTESIAN_POINT('Ctrl Pts',(-20.2828227302339,13.3590741574195,
12.));
#179382=CARTESIAN_POINT('Ctrl Pts',(-20.3051490429048,13.3636222481016,
12.));
#179383=CARTESIAN_POINT('Ctrl Pts',(-20.3275775983029,13.3681323955826,
12.));
#179384=CARTESIAN_POINT('Ctrl Pts',(-20.3501078331814,13.3726041410867,
12.));
#179385=CARTESIAN_POINT('Ctrl Pts',(-20.3727391887184,13.3770370313188,
12.));
#179386=CARTESIAN_POINT('Ctrl Pts',(-20.3954711104502,13.3814306183719,
12.));
#179387=CARTESIAN_POINT('Ctrl Pts',(-20.4183030482002,13.3857844596387,
12.));
#179388=CARTESIAN_POINT('Ctrl Pts',(-20.4412344560008,13.3900981177255,
12.));
#179389=CARTESIAN_POINT('Ctrl Pts',(-20.4642647920038,13.3943711603739,
12.));
#179390=CARTESIAN_POINT('Ctrl Pts',(-20.487393518404,13.3986031603716,12.));
#179391=CARTESIAN_POINT('Ctrl Pts',(-20.5106201013753,13.4027936954529,
12.));
#179392=CARTESIAN_POINT('Ctrl Pts',(-20.5339440109956,13.4069423482076,
12.));
#179393=CARTESIAN_POINT('Ctrl Pts',(-20.5573647211639,13.4110487059912,
12.));
#179394=CARTESIAN_POINT('Ctrl Pts',(-20.5808817095155,13.4151123608411,
12.));
#179395=CARTESIAN_POINT('Ctrl Pts',(-20.6044944573153,13.4191329093932,
12.));
#179396=CARTESIAN_POINT('Ctrl Pts',(-20.6282024494237,13.4231099528179,
12.));
#179397=CARTESIAN_POINT('Ctrl Pts',(-20.6520051742869,13.4270430967651,
12.));
#179398=CARTESIAN_POINT('Ctrl Pts',(-20.6759021239103,13.4309319513119,
12.));
#179399=CARTESIAN_POINT('Ctrl Pts',(-20.6998927938288,13.4347761309154,
12.));
#179400=CARTESIAN_POINT('Ctrl Pts',(-20.7239766830675,13.4385752543663,
12.));
#179401=CARTESIAN_POINT('Ctrl Pts',(-20.7481532941013,13.4423289447561,
12.));
#179402=CARTESIAN_POINT('Ctrl Pts',(-20.7724221327608,13.4460368293688,
12.));
#179403=CARTESIAN_POINT('Ctrl Pts',(-20.7967827081227,13.4496985395637,
12.));
#179404=CARTESIAN_POINT('Ctrl Pts',(-20.821234532398,13.4533137106667,12.));
#179405=CARTESIAN_POINT('Ctrl Pts',(-20.8457771208082,13.4568819818631,
12.));
#179406=CARTESIAN_POINT('Ctrl Pts',(-20.8704099914641,13.4604029960983,
12.));
#179407=CARTESIAN_POINT('Ctrl Pts',(-20.8951326652158,13.4638763999725,
12.));
#179408=CARTESIAN_POINT('Ctrl Pts',(-20.9199446657584,13.4673018437718,
12.));
#179409=CARTESIAN_POINT('Ctrl Pts',(-20.9448455197557,13.4706789815166,
12.));
#179410=CARTESIAN_POINT('Ctrl Pts',(-20.9698347569476,13.4740074710087,
12.));
#179411=CARTESIAN_POINT('Ctrl Pts',(-20.9949119102592,13.4772869738879,
12.));
#179412=CARTESIAN_POINT('Ctrl Pts',(-21.0200765158885,13.4805171556822,
12.));
#179413=CARTESIAN_POINT('Ctrl Pts',(-21.0453281134247,13.4836976858912,
12.));
#179414=CARTESIAN_POINT('Ctrl Pts',(-21.0706662455202,13.4868282377191,
12.));
#179415=CARTESIAN_POINT('Ctrl Pts',(-21.0960904575048,13.4899084877718,
12.));
#179416=CARTESIAN_POINT('Ctrl Pts',(-21.1216002970209,13.4929381157778,
12.));
#179417=CARTESIAN_POINT('Ctrl Pts',(-21.1471953136209,13.4959168042934,
12.));
#179418=CARTESIAN_POINT('Ctrl Pts',(-21.1728750584173,13.4988442384491,
12.));
#179419=CARTESIAN_POINT('Ctrl Pts',(-21.1986390835825,13.5017201056088,
12.));
#179420=CARTESIAN_POINT('Ctrl Pts',(-21.224486942933,13.5045440957404,12.));
#179421=CARTESIAN_POINT('Ctrl Pts',(-21.2504181927429,13.5073159019454,
12.));
#179422=CARTESIAN_POINT('Ctrl Pts',(-21.2764323924442,13.5100352209207,
12.));
#179423=CARTESIAN_POINT('Ctrl Pts',(-21.3025291054236,13.5127017534972,
12.));
#179424=CARTESIAN_POINT('Ctrl Pts',(-21.328707899634,13.5153152050554,12.));
#179425=CARTESIAN_POINT('Ctrl Pts',(-21.3549683486219,13.5178752862461,
12.));
#179426=CARTESIAN_POINT('Ctrl Pts',(-21.3813100304967,13.5203817122496,
12.));
#179427=CARTESIAN_POINT('Ctrl Pts',(-21.4077325259318,13.5228342013508,
12.));
#179428=CARTESIAN_POINT('Ctrl Pts',(-21.4342354165254,13.5252324737795,
12.));
#179429=CARTESIAN_POINT('Ctrl Pts',(-21.4608182828695,13.5275762503553,
12.));
#179430=CARTESIAN_POINT('Ctrl Pts',(-21.487480703047,13.5298652514357,12.));
#179431=CARTESIAN_POINT('Ctrl Pts',(-21.5142222501671,13.5320991952145,
12.));
#179432=CARTESIAN_POINT('Ctrl Pts',(-21.5410424932511,13.5342777983225,
12.));
#179433=CARTESIAN_POINT('Ctrl Pts',(-21.5679410019011,13.5364007790292,
12.));
#179434=CARTESIAN_POINT('Ctrl Pts',(-21.5949173499022,13.5384678597206,
12.));
#179435=CARTESIAN_POINT('Ctrl Pts',(-21.6219711193951,13.5404787697798,
12.));
#179436=CARTESIAN_POINT('Ctrl Pts',(-21.6491019044647,13.5424332480698,
12.));
#179437=CARTESIAN_POINT('Ctrl Pts',(-21.676309315769,13.5443310461516,12.));
#179438=CARTESIAN_POINT('Ctrl Pts',(-21.7035929822939,13.546171929503,12.));
#179439=CARTESIAN_POINT('Ctrl Pts',(-21.730952541226,13.5479556704457,12.));
#179440=CARTESIAN_POINT('Ctrl Pts',(-21.7583876294532,13.5496820422186,
12.));
#179441=CARTESIAN_POINT('Ctrl Pts',(-21.7858978745848,13.5513508127232,
12.));
#179442=CARTESIAN_POINT('Ctrl Pts',(-21.8134828857963,13.5529617381569,
12.));
#179443=CARTESIAN_POINT('Ctrl Pts',(-21.841142245609,13.5545145573048,12.));
#179444=CARTESIAN_POINT('Ctrl Pts',(-21.8688754989401,13.5560089839426,
12.));
#179445=CARTESIAN_POINT('Ctrl Pts',(-21.8966821688876,13.5574447178484,
12.));
#179446=CARTESIAN_POINT('Ctrl Pts',(-21.9245617765827,13.5588214586672,
12.));
#179447=CARTESIAN_POINT('Ctrl Pts',(-21.9525138592862,13.5601389185315,
12.));
#179448=CARTESIAN_POINT('Ctrl Pts',(-21.9805379899192,13.5613968357589,
12.));
#179449=CARTESIAN_POINT('Ctrl Pts',(-22.0086337943431,13.5625949868313,
12.));
#179450=CARTESIAN_POINT('Ctrl Pts',(-22.0368009736227,13.5637332022393,
12.));
#179451=CARTESIAN_POINT('Ctrl Pts',(-22.0650393089492,13.5648113688894,
12.));
#179452=CARTESIAN_POINT('Ctrl Pts',(-22.0933486464442,13.5658294169106,
12.));
#179453=CARTESIAN_POINT('Ctrl Pts',(-22.1217288871823,13.5667873105179,
12.));
#179454=CARTESIAN_POINT('Ctrl Pts',(-22.1444897575076,13.5675054918922,
12.));
#179455=CARTESIAN_POINT('Ctrl Pts',(-22.1615922804939,13.5680170531724,
12.));
#179456=CARTESIAN_POINT('Ctrl Pts',(-22.1730081264583,13.5683460612913,
12.));
#179457=CARTESIAN_POINT('Ctrl Pts',(-22.1787195904339,13.5685075571671,
12.));
#179458=CARTESIAN_POINT('',(-22.8400320311648,12.4230808101438,12.));
#179459=CARTESIAN_POINT('Origin',(0.,0.,12.));
#179460=CARTESIAN_POINT('',(-20.353053841303,9.71462809124917,12.));
#179461=CARTESIAN_POINT('Ctrl Pts',(-22.8400320311648,12.4230808101438,
12.));
#179462=CARTESIAN_POINT('Ctrl Pts',(-22.8370364396497,12.4182152851867,
12.));
#179463=CARTESIAN_POINT('Ctrl Pts',(-22.8310435872852,12.4084933766366,
12.));
#179464=CARTESIAN_POINT('Ctrl Pts',(-22.8220493007353,12.393937937903,12.));
#179465=CARTESIAN_POINT('Ctrl Pts',(-22.8100469022632,12.3745855366772,
12.));
#179466=CARTESIAN_POINT('Ctrl Pts',(-22.7950272216959,12.3504864740361,
12.));
#179467=CARTESIAN_POINT('Ctrl Pts',(-22.7799908974947,12.3264788926108,
12.));
#179468=CARTESIAN_POINT('Ctrl Pts',(-22.7649380101154,12.3025628601812,
12.));
#179469=CARTESIAN_POINT('Ctrl Pts',(-22.7498686970096,12.2787384750747,
12.));
#179470=CARTESIAN_POINT('Ctrl Pts',(-22.7347831655251,12.2550058702389,
12.));
#179471=CARTESIAN_POINT('Ctrl Pts',(-22.7196817119299,12.2313652198047,
12.));
#179472=CARTESIAN_POINT('Ctrl Pts',(-22.7045647168659,12.2078167360267,
12.));
#179473=CARTESIAN_POINT('Ctrl Pts',(-22.6894326204959,12.1843606579246,
12.));
#179474=CARTESIAN_POINT('Ctrl Pts',(-22.6742859034891,12.1609972423088,
12.));
#179475=CARTESIAN_POINT('Ctrl Pts',(-22.6591250653942,12.1377267537141,
12.));
#179476=CARTESIAN_POINT('Ctrl Pts',(-22.6439506046611,12.1145494550384,
12.));
#179477=CARTESIAN_POINT('Ctrl Pts',(-22.628762996708,12.0914655972828,12.));
#179478=CARTESIAN_POINT('Ctrl Pts',(-22.613562676493,12.0684754113869,12.));
#179479=CARTESIAN_POINT('Ctrl Pts',(-22.5983500505675,12.0455791139135,
12.));
#179480=CARTESIAN_POINT('Ctrl Pts',(-22.5831255061306,12.0227769113132,
12.));
#179481=CARTESIAN_POINT('Ctrl Pts',(-22.5678894211194,12.0000690046697,
12.));
#179482=CARTESIAN_POINT('Ctrl Pts',(-22.5526421741159,11.9774555943496,
12.));
#179483=CARTESIAN_POINT('Ctrl Pts',(-22.5373841537299,11.9549368843996,
12.));
#179484=CARTESIAN_POINT('Ctrl Pts',(-22.5221157697869,11.9325130877801,
12.));
#179485=CARTESIAN_POINT('Ctrl Pts',(-22.5068374513958,11.9101844254555,
12.));
#179486=CARTESIAN_POINT('Ctrl Pts',(-22.4915496418472,11.8879511239941,
12.));
#179487=CARTESIAN_POINT('Ctrl Pts',(-22.4762527946694,11.8658134137018,
12.));
#179488=CARTESIAN_POINT('Ctrl Pts',(-22.4609473690469,11.8437715264487,
12.));
#179489=CARTESIAN_POINT('Ctrl Pts',(-22.4456338258738,11.8218256937889,
12.));
#179490=CARTESIAN_POINT('Ctrl Pts',(-22.4303126226468,11.7999761445175,
12.));
#179491=CARTESIAN_POINT('Ctrl Pts',(-22.4149842125018,11.7782231042041,
12.));
#179492=CARTESIAN_POINT('Ctrl Pts',(-22.39964904692,11.7565667964765,12.));
#179493=CARTESIAN_POINT('Ctrl Pts',(-22.3843075773905,11.7350074437961,
12.));
#179494=CARTESIAN_POINT('Ctrl Pts',(-22.3689602575492,11.7135452684532,
12.));
#179495=CARTESIAN_POINT('Ctrl Pts',(-22.3536075450028,11.6921804934056,
12.));
#179496=CARTESIAN_POINT('Ctrl Pts',(-22.3382499035618,11.6709133432986,
12.));
#179497=CARTESIAN_POINT('Ctrl Pts',(-22.3228878043976,11.6497440449858,
12.));
#179498=CARTESIAN_POINT('Ctrl Pts',(-22.3075217249049,11.6286728270011,
12.));
#179499=CARTESIAN_POINT('Ctrl Pts',(-22.2921521480358,11.6076999192359,
12.));
#179500=CARTESIAN_POINT('Ctrl Pts',(-22.2767795614349,11.5868255525189,
12.));
#179501=CARTESIAN_POINT('Ctrl Pts',(-22.2614044566898,11.5660499582403,
12.));
#179502=CARTESIAN_POINT('Ctrl Pts',(-22.2460273284653,11.545373367912,12.));
#179503=CARTESIAN_POINT('Ctrl Pts',(-22.2306486738899,11.5247960128476,
12.));
#179504=CARTESIAN_POINT('Ctrl Pts',(-22.215268993102,11.504318124424,12.));
#179505=CARTESIAN_POINT('Ctrl Pts',(-22.1998887896435,11.4839399342589,
12.));
#179506=CARTESIAN_POINT('Ctrl Pts',(-22.184508570917,11.463661674411,12.));
#179507=CARTESIAN_POINT('Ctrl Pts',(-22.1691288486096,11.443483577557,12.));
#179508=CARTESIAN_POINT('Ctrl Pts',(-22.1537501391486,11.4234058771742,
12.));
#179509=CARTESIAN_POINT('Ctrl Pts',(-22.1383729640963,11.4034288076908,
12.));
#179510=CARTESIAN_POINT('Ctrl Pts',(-22.1229978500185,11.3835526044256,
12.));
#179511=CARTESIAN_POINT('Ctrl Pts',(-22.1076253283978,11.3637775035367,
12.));
#179512=CARTESIAN_POINT('Ctrl Pts',(-22.0922559355293,11.3441037419553,
12.));
#179513=CARTESIAN_POINT('Ctrl Pts',(-22.0768902124267,11.3245315573168,
12.));
#179514=CARTESIAN_POINT('Ctrl Pts',(-22.0615287047179,11.3050611878771,
12.));
#179515=CARTESIAN_POINT('Ctrl Pts',(-22.046171962566,11.2856928724374,12.));
#179516=CARTESIAN_POINT('Ctrl Pts',(-22.0308205408351,11.2664268504207,
12.));
#179517=CARTESIAN_POINT('Ctrl Pts',(-22.0154749992364,11.2472633619276,
12.));
#179518=CARTESIAN_POINT('Ctrl Pts',(-22.0001359024839,11.2282026477897,
12.));
#179519=CARTESIAN_POINT('Ctrl Pts',(-21.9848038204439,11.2092449496125,
12.));
#179520=CARTESIAN_POINT('Ctrl Pts',(-21.9694793282913,11.1903905098109,
12.));
#179521=CARTESIAN_POINT('Ctrl Pts',(-21.9541630066504,11.1716395716375,
12.));
#179522=CARTESIAN_POINT('Ctrl Pts',(-21.9388554416437,11.1529923792002,
12.));
#179523=CARTESIAN_POINT('Ctrl Pts',(-21.9235572249518,11.134449177474,12.));
#179524=CARTESIAN_POINT('Ctrl Pts',(-21.9082689538687,11.1160102123024,
12.));
#179525=CARTESIAN_POINT('Ctrl Pts',(-21.8929912313608,11.0976757303944,
12.));
#179526=CARTESIAN_POINT('Ctrl Pts',(-21.8777246661191,11.0794459793058,
12.));
#179527=CARTESIAN_POINT('Ctrl Pts',(-21.8624698726319,11.0613212074364,
12.));
#179528=CARTESIAN_POINT('Ctrl Pts',(-21.8472274713103,11.0433016640808,
12.));
#179529=CARTESIAN_POINT('Ctrl Pts',(-21.8319980886033,11.0253875994598,
12.));
#179530=CARTESIAN_POINT('Ctrl Pts',(-21.8167823571168,11.0075792647477,
12.));
#179531=CARTESIAN_POINT('Ctrl Pts',(-21.8015809157302,10.9898769120913,
12.));
#179532=CARTESIAN_POINT('Ctrl Pts',(-21.7863944097143,10.9722807946157,
12.));
#179533=CARTESIAN_POINT('Ctrl Pts',(-21.7712234908468,10.9547911664457,
12.));
#179534=CARTESIAN_POINT('Ctrl Pts',(-21.7560688175252,10.9374082827446,
12.));
#179535=CARTESIAN_POINT('Ctrl Pts',(-21.74093105488,10.9201323997386,12.));
#179536=CARTESIAN_POINT('Ctrl Pts',(-21.7258108748874,10.9029637747341,
12.));
#179537=CARTESIAN_POINT('Ctrl Pts',(-21.7107089564822,10.8859026661292,
12.));
#179538=CARTESIAN_POINT('Ctrl Pts',(-21.6956259856667,10.8689493334093,
12.));
#179539=CARTESIAN_POINT('Ctrl Pts',(-21.6805626556461,10.8521040371832,
12.));
#179540=CARTESIAN_POINT('Ctrl Pts',(-21.6655196669727,10.835367039227,12.));
#179541=CARTESIAN_POINT('Ctrl Pts',(-21.6504977276864,10.8187386025135,
12.));
#179542=CARTESIAN_POINT('Ctrl Pts',(-21.6354975534557,10.8022189912369,
12.));
#179543=CARTESIAN_POINT('Ctrl Pts',(-21.6205198677176,10.7858084708262,
12.));
#179544=CARTESIAN_POINT('Ctrl Pts',(-21.6055654018179,10.7695073079554,
12.));
#179545=CARTESIAN_POINT('Ctrl Pts',(-21.5906348951745,10.7533157705943,
12.));
#179546=CARTESIAN_POINT('Ctrl Pts',(-21.5757290954372,10.7372341280468,
12.));
#179547=CARTESIAN_POINT('Ctrl Pts',(-21.5608487586467,10.7212626509816,
12.));
#179548=CARTESIAN_POINT('Ctrl Pts',(-21.5459946493955,10.7054016114571,
12.));
#179549=CARTESIAN_POINT('Ctrl Pts',(-21.531167540981,10.689651282929,12.));
#179550=CARTESIAN_POINT('Ctrl Pts',(-21.5163682155805,10.6740119402835,
12.));
#179551=CARTESIAN_POINT('Ctrl Pts',(-21.5015974644454,10.658483859894,12.));
#179552=CARTESIAN_POINT('Ctrl Pts',(-21.4868560880893,10.6430673196609,
12.));
#179553=CARTESIAN_POINT('Ctrl Pts',(-21.4721448964766,10.6277625990457,
12.));
#179554=CARTESIAN_POINT('Ctrl Pts',(-21.4574647092093,10.612569979096,12.));
#179555=CARTESIAN_POINT('Ctrl Pts',(-21.4428163557137,10.597489742462,12.));
#179556=CARTESIAN_POINT('Ctrl Pts',(-21.4282006754624,10.582522173457,12.));
#179557=CARTESIAN_POINT('Ctrl Pts',(-21.4136185181974,10.5676675581106,
12.));
#179558=CARTESIAN_POINT('Ctrl Pts',(-21.3990707441495,10.5529261842107,
12.));
#179559=CARTESIAN_POINT('Ctrl Pts',(-21.3845582242604,10.5382983413422,
12.));
#179560=CARTESIAN_POINT('Ctrl Pts',(-21.3700818403942,10.523784320906,12.));
#179561=CARTESIAN_POINT('Ctrl Pts',(-21.3556424855822,10.5093844161689,
12.));
#179562=CARTESIAN_POINT('Ctrl Pts',(-21.3412410642912,10.4950989223341,
12.));
#179563=CARTESIAN_POINT('Ctrl Pts',(-21.3268784926823,10.4809281365933,
12.));
#179564=CARTESIAN_POINT('Ctrl Pts',(-21.312555698873,10.4668723581768,12.));
#179565=CARTESIAN_POINT('Ctrl Pts',(-21.2982736231924,10.452931888387,12.));
#179566=CARTESIAN_POINT('Ctrl Pts',(-21.2840332184471,10.4391070306385,
12.));
#179567=CARTESIAN_POINT('Ctrl Pts',(-21.2698354502391,10.4253980905394,
12.));
#179568=CARTESIAN_POINT('Ctrl Pts',(-21.2556812972741,10.4118053759584,
12.));
#179569=CARTESIAN_POINT('Ctrl Pts',(-21.2415717516713,10.3983291970846,
12.));
#179570=CARTESIAN_POINT('Ctrl Pts',(-21.2275078192708,10.384969866479,12.));
#179571=CARTESIAN_POINT('Ctrl Pts',(-21.2134905199359,10.3717276991137,
12.));
#179572=CARTESIAN_POINT('Ctrl Pts',(-21.1995208879205,10.3586030124595,
12.));
#179573=CARTESIAN_POINT('Ctrl Pts',(-21.1855999722427,10.3455961265706,
12.));
#179574=CARTESIAN_POINT('Ctrl Pts',(-21.1717288370512,10.3327073641574,
12.));
#179575=CARTESIAN_POINT('Ctrl Pts',(-21.1579085619959,10.3199370506541,
12.));
#179576=CARTESIAN_POINT('Ctrl Pts',(-21.1441402425831,10.307285514268,12.));
#179577=CARTESIAN_POINT('Ctrl Pts',(-21.130424990599,10.2947530860714,12.));
#179578=CARTESIAN_POINT('Ctrl Pts',(-21.1167639345623,10.2823401001067,
12.));
#179579=CARTESIAN_POINT('Ctrl Pts',(-21.1031582201625,10.2700468934743,
12.));
#179580=CARTESIAN_POINT('Ctrl Pts',(-21.0896090107066,10.2578738064183,
12.));
#179581=CARTESIAN_POINT('Ctrl Pts',(-21.0761174875448,10.2458211823915,
12.));
#179582=CARTESIAN_POINT('Ctrl Pts',(-21.0626848505665,10.233889368157,12.));
#179583=CARTESIAN_POINT('Ctrl Pts',(-21.0493123187483,10.2220787139157,
12.));
#179584=CARTESIAN_POINT('Ctrl Pts',(-21.0360011306814,10.2103895734123,
12.));
#179585=CARTESIAN_POINT('Ctrl Pts',(-21.0227525451107,10.1988223040425,
12.));
#179586=CARTESIAN_POINT('Ctrl Pts',(-21.0095678414486,10.1873772669358,
12.));
#179587=CARTESIAN_POINT('Ctrl Pts',(-20.9964483203685,10.1760548270765,
12.));
#179588=CARTESIAN_POINT('Ctrl Pts',(-20.9833953044737,10.1648553534567,
12.));
#179589=CARTESIAN_POINT('Ctrl Pts',(-20.970410138937,10.1537792192065,12.));
#179590=CARTESIAN_POINT('Ctrl Pts',(-20.9574941921591,10.1428268017257,
12.));
#179591=CARTESIAN_POINT('Ctrl Pts',(-20.944648856393,10.1319984827909,12.));
#179592=CARTESIAN_POINT('Ctrl Pts',(-20.931875548473,10.1212946487057,12.));
#179593=CARTESIAN_POINT('Ctrl Pts',(-20.9191757106266,10.1107156904836,
12.));
#179594=CARTESIAN_POINT('Ctrl Pts',(-20.9065508112556,10.1002620040076,
12.));
#179595=CARTESIAN_POINT('Ctrl Pts',(-20.8940023457371,10.0899339901916,
12.));
#179596=CARTESIAN_POINT('Ctrl Pts',(-20.8815318371844,10.0797320551154,
12.));
#179597=CARTESIAN_POINT('Ctrl Pts',(-20.8691408373705,10.0696566102219,
12.));
#179598=CARTESIAN_POINT('Ctrl Pts',(-20.856830927732,10.0597080725375,12.));
#179599=CARTESIAN_POINT('Ctrl Pts',(-20.8446037203402,10.0498868648733,
12.));
#179600=CARTESIAN_POINT('Ctrl Pts',(-20.8324608588906,10.0401934160234,
12.));
#179601=CARTESIAN_POINT('Ctrl Pts',(-20.8204040196599,10.0306281609435,
12.));
#179602=CARTESIAN_POINT('Ctrl Pts',(-20.8084349126885,10.0211915410095,
12.));
#179603=CARTESIAN_POINT('Ctrl Pts',(-20.7965552829907,10.0118840042786,
12.));
#179604=CARTESIAN_POINT('Ctrl Pts',(-20.7847669117568,10.0027060057389,
12.));
#179605=CARTESIAN_POINT('Ctrl Pts',(-20.7730716175417,9.99365800754638,
12.));
#179606=CARTESIAN_POINT('Ctrl Pts',(-20.7614712574989,9.98474047926846,
12.));
#179607=CARTESIAN_POINT('Ctrl Pts',(-20.7499677289625,9.97595389823461,
12.));
#179608=CARTESIAN_POINT('Ctrl Pts',(-20.7385629709795,9.96729874986198,
12.));
#179609=CARTESIAN_POINT('Ctrl Pts',(-20.7272589658752,9.95877552798403,
12.));
#179610=CARTESIAN_POINT('Ctrl Pts',(-20.716057740758,9.95038473514962,12.));
#179611=CARTESIAN_POINT('Ctrl Pts',(-20.7049613692237,9.94212688298251,
12.));
#179612=CARTESIAN_POINT('Ctrl Pts',(-20.6939719732485,9.93400249259736,
12.));
#179613=CARTESIAN_POINT('Ctrl Pts',(-20.6830917250255,9.9260120949875,12.));
#179614=CARTESIAN_POINT('Ctrl Pts',(-20.6723228488262,9.91815623141284,
12.));
#179615=CARTESIAN_POINT('Ctrl Pts',(-20.6616676228315,9.91043545377004,
12.));
#179616=CARTESIAN_POINT('Ctrl Pts',(-20.6511283817415,9.90285032516696,
12.));
#179617=CARTESIAN_POINT('Ctrl Pts',(-20.6407075193977,9.89540142049124,
12.));
#179618=CARTESIAN_POINT('Ctrl Pts',(-20.6304074914086,9.88808932697305,
12.));
#179619=CARTESIAN_POINT('Ctrl Pts',(-20.6202308177472,9.88091464472669,
12.));
#179620=CARTESIAN_POINT('Ctrl Pts',(-20.6101800854491,9.87387798732944,
12.));
#179621=CARTESIAN_POINT('Ctrl Pts',(-20.6002579513696,9.86697998242612,
12.));
#179622=CARTESIAN_POINT('Ctrl Pts',(-20.5904671449754,9.86022127232749,
12.));
#179623=CARTESIAN_POINT('Ctrl Pts',(-20.580810471002,9.85360251457004,12.));
#179624=CARTESIAN_POINT('Ctrl Pts',(-20.5712908125145,9.84712438256308,
12.));
#179625=CARTESIAN_POINT('Ctrl Pts',(-20.5619111362406,9.84078756677589,
12.));
#179626=CARTESIAN_POINT('Ctrl Pts',(-20.5526744976461,9.83459277585321,
12.));
#179627=CARTESIAN_POINT('Ctrl Pts',(-20.5435840460717,9.82854073773857,
12.));
#179628=CARTESIAN_POINT('Ctrl Pts',(-20.534643029951,9.82263220080328,12.));
#179629=CARTESIAN_POINT('Ctrl Pts',(-20.5258548000625,9.81686793455918,
12.));
#179630=CARTESIAN_POINT('Ctrl Pts',(-20.5172228122839,9.81124873025278,
12.));
#179631=CARTESIAN_POINT('Ctrl Pts',(-20.5087506310507,9.80577540161103,
12.));
#179632=CARTESIAN_POINT('Ctrl Pts',(-20.500441931211,9.80044878520967,12.));
#179633=CARTESIAN_POINT('Ctrl Pts',(-20.4923005087945,9.79526974288344,
12.));
#179634=CARTESIAN_POINT('Ctrl Pts',(-20.4843302955329,9.7902391649866,12.));
#179635=CARTESIAN_POINT('Ctrl Pts',(-20.4765353711585,9.78535797314162,
12.));
#179636=CARTESIAN_POINT('Ctrl Pts',(-20.4689199790668,9.78062712373313,
12.));
#179637=CARTESIAN_POINT('Ctrl Pts',(-20.4614885274973,9.77604760815523,
12.));
#179638=CARTESIAN_POINT('Ctrl Pts',(-20.4542455817527,9.7716204510407,12.));
#179639=CARTESIAN_POINT('Ctrl Pts',(-20.447195862298,9.76734670980897,12.));
#179640=CARTESIAN_POINT('Ctrl Pts',(-20.4403442329401,9.76322747195502,
12.));
#179641=CARTESIAN_POINT('Ctrl Pts',(-20.4336957355474,9.7592638628993,12.));
#179642=CARTESIAN_POINT('Ctrl Pts',(-20.4272556476629,9.75545705902416,
12.));
#179643=CARTESIAN_POINT('Ctrl Pts',(-20.4210295275818,9.75180829786433,
12.));
#179644=CARTESIAN_POINT('Ctrl Pts',(-20.4150232777393,9.74831889242175,
12.));
#179645=CARTESIAN_POINT('Ctrl Pts',(-20.4092430879861,9.74499021838536,
12.));
#179646=CARTESIAN_POINT('Ctrl Pts',(-20.4036953576549,9.74182369656272,
12.));
#179647=CARTESIAN_POINT('Ctrl Pts',(-20.3983866213331,9.73882077613206,
12.));
#179648=CARTESIAN_POINT('Ctrl Pts',(-20.3933234845646,9.7359829201425,12.));
#179649=CARTESIAN_POINT('Ctrl Pts',(-20.3885129129912,9.73331167102812,
12.));
#179650=CARTESIAN_POINT('Ctrl Pts',(-20.3839624556742,9.73080870123726,
12.));
#179651=CARTESIAN_POINT('Ctrl Pts',(-20.3796805893304,9.72847589116533,
12.));
#179652=CARTESIAN_POINT('Ctrl Pts',(-20.3756766651952,9.72631531732871,
12.));
#179653=CARTESIAN_POINT('Ctrl Pts',(-20.371960235676,9.72432910043193,12.));
#179654=CARTESIAN_POINT('Ctrl Pts',(-20.3685406190576,9.72251930722504,
12.));
#179655=CARTESIAN_POINT('Ctrl Pts',(-20.3654261611055,9.72088778381102,
12.));
#179656=CARTESIAN_POINT('Ctrl Pts',(-20.362625691398,9.71943648548114,12.));
#179657=CARTESIAN_POINT('Ctrl Pts',(-20.3601498764344,9.71816778327999,
12.));
#179658=CARTESIAN_POINT('Ctrl Pts',(-20.3580133103357,9.71708493723061,
12.));
#179659=CARTESIAN_POINT('Ctrl Pts',(-20.3562337557875,9.71619192554147,
12.));
#179660=CARTESIAN_POINT('Ctrl Pts',(-20.3548282742361,9.71549257088175,
12.));
#179661=CARTESIAN_POINT('Ctrl Pts',(-20.3538098605706,9.71498978052101,
12.));
#179662=CARTESIAN_POINT('Ctrl Pts',(-20.3533097561886,9.71474590350791,
12.));
#179663=CARTESIAN_POINT('Ctrl Pts',(-20.3531126095522,9.71465227853122,
12.));
#179664=CARTESIAN_POINT('Ctrl Pts',(-20.353060251684,9.71462954053074,12.));
#179665=CARTESIAN_POINT('Ctrl Pts',(-20.353053841303,9.71462809124917,12.));
#179666=CARTESIAN_POINT('',(-19.84920021178,9.47413589477549,12.));
#179667=CARTESIAN_POINT('',(-9.70154690100589,4.63060338698782,12.));
#179668=CARTESIAN_POINT('',(-19.6085639972844,8.81783521984851,12.));
#179669=CARTESIAN_POINT('Origin',(-20.0645771135003,9.02290115519382,12.));
#179670=CARTESIAN_POINT('',(-20.1004996511507,7.63019749246978,12.));
#179671=CARTESIAN_POINT('Origin',(-7.08841632778408E-13,3.26562511982935E-13,
12.));
#179672=CARTESIAN_POINT('',(-20.7347298079577,7.33627833380047,12.));
#179673=CARTESIAN_POINT('Origin',(-20.56795313141,7.80764394578303,12.));
#179674=CARTESIAN_POINT('',(-21.2610617890679,7.52250298901265,12.));
#179675=CARTESIAN_POINT('',(-10.6305308945339,3.76125149450631,12.));
#179676=CARTESIAN_POINT('',(-24.9347862158358,7.36589684767345,12.));
#179677=CARTESIAN_POINT('Ctrl Pts',(-21.2610617890679,7.52250298901265,
12.));
#179678=CARTESIAN_POINT('Ctrl Pts',(-21.2610673466883,7.52250649703992,
12.));
#179679=CARTESIAN_POINT('Ctrl Pts',(-21.261120447486,7.52252744144958,12.));
#179680=CARTESIAN_POINT('Ctrl Pts',(-21.2613260540651,7.52260064231736,
12.));
#179681=CARTESIAN_POINT('Ctrl Pts',(-21.261852128355,7.52278182242727,12.));
#179682=CARTESIAN_POINT('Ctrl Pts',(-21.262927782038,7.52314642316202,12.));
#179683=CARTESIAN_POINT('Ctrl Pts',(-21.2644161259965,7.52364573027521,
12.));
#179684=CARTESIAN_POINT('Ctrl Pts',(-21.266305915706,7.52427261074264,12.));
#179685=CARTESIAN_POINT('Ctrl Pts',(-21.2685823838672,7.52501770333522,
12.));
#179686=CARTESIAN_POINT('Ctrl Pts',(-21.2712301573465,7.52587126095544,
12.));
#179687=CARTESIAN_POINT('Ctrl Pts',(-21.2742366113578,7.5268252691856,12.));
#179688=CARTESIAN_POINT('Ctrl Pts',(-21.2775925269651,7.52787386225343,
12.));
#179689=CARTESIAN_POINT('Ctrl Pts',(-21.2812902781143,7.52901217930407,
12.));
#179690=CARTESIAN_POINT('Ctrl Pts',(-21.2853226580658,7.53023562438221,
12.));
#179691=CARTESIAN_POINT('Ctrl Pts',(-21.2896816163843,7.53153906987847,
12.));
#179692=CARTESIAN_POINT('Ctrl Pts',(-21.2943588989331,7.53291726078526,
12.));
#179693=CARTESIAN_POINT('Ctrl Pts',(-21.2993464250717,7.53436505309949,
12.));
#179694=CARTESIAN_POINT('Ctrl Pts',(-21.3046368712156,7.53587778251743,
12.));
#179695=CARTESIAN_POINT('Ctrl Pts',(-21.3102237167729,7.53745129364619,
12.));
#179696=CARTESIAN_POINT('Ctrl Pts',(-21.3161009456256,7.53908175169899,
12.));
#179697=CARTESIAN_POINT('Ctrl Pts',(-21.3222628524165,7.5407655203828,12.));
#179698=CARTESIAN_POINT('Ctrl Pts',(-21.328703791771,7.54249900377031,12.));
#179699=CARTESIAN_POINT('Ctrl Pts',(-21.3354182340149,7.54427868151268,
12.));
#179700=CARTESIAN_POINT('Ctrl Pts',(-21.3424008295038,7.54610114948351,
12.));
#179701=CARTESIAN_POINT('Ctrl Pts',(-21.349646476153,7.54796316246327,12.));
#179702=CARTESIAN_POINT('Ctrl Pts',(-21.3571503685853,7.54986166521306,
12.));
#179703=CARTESIAN_POINT('Ctrl Pts',(-21.3649079431864,7.55179375777441,
12.));
#179704=CARTESIAN_POINT('Ctrl Pts',(-21.3729148390244,7.55375667080032,
12.));
#179705=CARTESIAN_POINT('Ctrl Pts',(-21.3811668478933,7.55574773403507,
12.));
#179706=CARTESIAN_POINT('Ctrl Pts',(-21.3896598842119,7.55776435731422,
12.));
#179707=CARTESIAN_POINT('Ctrl Pts',(-21.3983899952988,7.55980403700615,
12.));
#179708=CARTESIAN_POINT('Ctrl Pts',(-21.4073533630364,7.56186435703622,
12.));
#179709=CARTESIAN_POINT('Ctrl Pts',(-21.4165463106252,7.56394299313682,
12.));
#179710=CARTESIAN_POINT('Ctrl Pts',(-21.4259653015732,7.56603771218706,
12.));
#179711=CARTESIAN_POINT('Ctrl Pts',(-21.435606926151,7.56814636360842,12.));
#179712=CARTESIAN_POINT('Ctrl Pts',(-21.445467890751,7.57026687261169,12.));
#179713=CARTESIAN_POINT('Ctrl Pts',(-21.4555450053147,7.57239723223521,
12.));
#179714=CARTESIAN_POINT('Ctrl Pts',(-21.4658351740135,7.57453549743435,
12.));
#179715=CARTESIAN_POINT('Ctrl Pts',(-21.4763353936766,7.57667978403002,
12.));
#179716=CARTESIAN_POINT('Ctrl Pts',(-21.4870427508193,7.57882826679131,
12.));
#179717=CARTESIAN_POINT('Ctrl Pts',(-21.497954419274,7.5809791779073,12.));
#179718=CARTESIAN_POINT('Ctrl Pts',(-21.5090676573866,7.58313080519158,
12.));
#179719=CARTESIAN_POINT('Ctrl Pts',(-21.5203798035294,7.58528148919113,
12.));
#179720=CARTESIAN_POINT('Ctrl Pts',(-21.5318882716735,7.58742962034834,
12.));
#179721=CARTESIAN_POINT('Ctrl Pts',(-21.5435905470113,7.58957363620026,
12.));
#179722=CARTESIAN_POINT('Ctrl Pts',(-21.5554841813465,7.59171201844793,
12.));
#179723=CARTESIAN_POINT('Ctrl Pts',(-21.5675667904728,7.5938432912493,12.));
#179724=CARTESIAN_POINT('Ctrl Pts',(-21.5798360518978,7.59596601973588,
12.));
#179725=CARTESIAN_POINT('Ctrl Pts',(-21.5922897024466,7.59807880846192,
12.));
#179726=CARTESIAN_POINT('Ctrl Pts',(-21.6049255358843,7.60018029988238,
12.));
#179727=CARTESIAN_POINT('Ctrl Pts',(-21.6177414005991,7.60226917285432,
12.));
#179728=CARTESIAN_POINT('Ctrl Pts',(-21.6307351973823,7.604344141183,12.));
#179729=CARTESIAN_POINT('Ctrl Pts',(-21.6439048771743,7.60640395216358,
12.));
#179730=CARTESIAN_POINT('Ctrl Pts',(-21.6572484388079,7.60844738512872,
12.));
#179731=CARTESIAN_POINT('Ctrl Pts',(-21.6707639267573,7.6104732500095,12.));
#179732=CARTESIAN_POINT('Ctrl Pts',(-21.6844494295813,7.61248038630265,
12.));
#179733=CARTESIAN_POINT('Ctrl Pts',(-21.6983030783321,7.61446766202787,
12.));
#179734=CARTESIAN_POINT('Ctrl Pts',(-21.7123230449835,7.61643397270425,
12.));
#179735=CARTESIAN_POINT('Ctrl Pts',(-21.7265075407977,7.61837824030541,
12.));
#179736=CARTESIAN_POINT('Ctrl Pts',(-21.7408548148657,7.62029941230855,
12.));
#179737=CARTESIAN_POINT('Ctrl Pts',(-21.7553631528329,7.62219646084226,
12.));
#179738=CARTESIAN_POINT('Ctrl Pts',(-21.7700308755583,7.62406838181164,
12.));
#179739=CARTESIAN_POINT('Ctrl Pts',(-21.7848563378022,7.62591419404521,
12.));
#179740=CARTESIAN_POINT('Ctrl Pts',(-21.7998379268583,7.62773293842409,
12.));
#179741=CARTESIAN_POINT('Ctrl Pts',(-21.8149740615093,7.62952367718151,
12.));
#179742=CARTESIAN_POINT('Ctrl Pts',(-21.8302631910197,7.6312854932304,12.));
#179743=CARTESIAN_POINT('Ctrl Pts',(-21.8457037941084,7.63301748948936,
12.));
#179744=CARTESIAN_POINT('Ctrl Pts',(-21.8612943779086,7.63471878821203,
12.));
#179745=CARTESIAN_POINT('Ctrl Pts',(-21.8770334769492,7.63638853033367,
12.));
#179746=CARTESIAN_POINT('Ctrl Pts',(-21.8929196523511,7.63802587492007,
12.));
#179747=CARTESIAN_POINT('Ctrl Pts',(-21.9089514909873,7.63962999860916,
12.));
#179748=CARTESIAN_POINT('Ctrl Pts',(-21.9251276046546,7.6412000950654,12.));
#179749=CARTESIAN_POINT('Ctrl Pts',(-21.9414466292074,7.64273537442706,
12.));
#179750=CARTESIAN_POINT('Ctrl Pts',(-21.9579072237653,7.64423506279153,
12.));
#179751=CARTESIAN_POINT('Ctrl Pts',(-21.97450807008,7.64569840177359,12.));
#179752=CARTESIAN_POINT('Ctrl Pts',(-21.9912478718542,7.64712464805258,
12.));
#179753=CARTESIAN_POINT('Ctrl Pts',(-22.0081253540773,7.64851307293346,
12.));
#179754=CARTESIAN_POINT('Ctrl Pts',(-22.0251392623209,7.64986296190156,
12.));
#179755=CARTESIAN_POINT('Ctrl Pts',(-22.0422883621176,7.65117361421346,
12.));
#179756=CARTESIAN_POINT('Ctrl Pts',(-22.0595714384432,7.65244434253104,
12.));
#179757=CARTESIAN_POINT('Ctrl Pts',(-22.0769872951596,7.65367447254945,
12.));
#179758=CARTESIAN_POINT('Ctrl Pts',(-22.094534754469,7.6548633426365,12.));
#179759=CARTESIAN_POINT('Ctrl Pts',(-22.1122126563327,7.65601030346819,
12.));
#179760=CARTESIAN_POINT('Ctrl Pts',(-22.1300198579671,7.65711471769407,
12.));
#179761=CARTESIAN_POINT('Ctrl Pts',(-22.1479552334206,7.65817595963351,
12.));
#179762=CARTESIAN_POINT('Ctrl Pts',(-22.1660176731174,7.65919341496925,
12.));
#179763=CARTESIAN_POINT('Ctrl Pts',(-22.1842060834092,7.66016648045008,
12.));
#179764=CARTESIAN_POINT('Ctrl Pts',(-22.2025193860972,7.66109456359292,
12.));
#179765=CARTESIAN_POINT('Ctrl Pts',(-22.2209565180098,7.66197708240435,
12.));
#179766=CARTESIAN_POINT('Ctrl Pts',(-22.239516430656,7.66281346512545,12.));
#179767=CARTESIAN_POINT('Ctrl Pts',(-22.2581980898487,7.66360314997662,
12.));
#179768=CARTESIAN_POINT('Ctrl Pts',(-22.2770004753332,7.66434558490972,
12.));
#179769=CARTESIAN_POINT('Ctrl Pts',(-22.2959225803925,7.66504022736262,
12.));
#179770=CARTESIAN_POINT('Ctrl Pts',(-22.3149634114823,7.66568654402441,
12.));
#179771=CARTESIAN_POINT('Ctrl Pts',(-22.3341219879454,7.66628401061905,
12.));
#179772=CARTESIAN_POINT('Ctrl Pts',(-22.3533973417013,7.66683211169134,
12.));
#179773=CARTESIAN_POINT('Ctrl Pts',(-22.3727885169361,7.66733034039887,
12.));
#179774=CARTESIAN_POINT('Ctrl Pts',(-22.3922945697782,7.66777819830819,
12.));
#179775=CARTESIAN_POINT('Ctrl Pts',(-22.411914567977,7.66817519519682,12.));
#179776=CARTESIAN_POINT('Ctrl Pts',(-22.4316475906616,7.66852084886745,
12.));
#179777=CARTESIAN_POINT('Ctrl Pts',(-22.4514927280863,7.6688146849666,12.));
#179778=CARTESIAN_POINT('Ctrl Pts',(-22.47144908137,7.66905623680835,12.));
#179779=CARTESIAN_POINT('Ctrl Pts',(-22.4915157622308,7.66924504520302,
12.));
#179780=CARTESIAN_POINT('Ctrl Pts',(-22.5116918927023,7.66938065829082,
12.));
#179781=CARTESIAN_POINT('Ctrl Pts',(-22.5319766049191,7.66946263138116,
12.));
#179782=CARTESIAN_POINT('Ctrl Pts',(-22.5523690409109,7.66949052679671,
12.));
#179783=CARTESIAN_POINT('Ctrl Pts',(-22.5728683523829,7.66946391372299,
12.));
#179784=CARTESIAN_POINT('Ctrl Pts',(-22.5934737004955,7.66938236806241,
12.));
#179785=CARTESIAN_POINT('Ctrl Pts',(-22.6141842556248,7.66924547229435,
12.));
#179786=CARTESIAN_POINT('Ctrl Pts',(-22.6349991971547,7.66905281533745,
12.));
#179787=CARTESIAN_POINT('Ctrl Pts',(-22.6559177133133,7.66880399241354,
12.));
#179788=CARTESIAN_POINT('Ctrl Pts',(-22.6769390009889,7.66849860491763,
12.));
#179789=CARTESIAN_POINT('Ctrl Pts',(-22.6980622655446,7.66813626029276,
12.));
#179790=CARTESIAN_POINT('Ctrl Pts',(-22.7192867206242,7.6677165719101,12.));
#179791=CARTESIAN_POINT('Ctrl Pts',(-22.7406115879508,7.66723915895412,
12.));
#179792=CARTESIAN_POINT('Ctrl Pts',(-22.7620360971839,7.66670364630273,
12.));
#179793=CARTESIAN_POINT('Ctrl Pts',(-22.7835594857697,7.66610966441259,
12.));
#179794=CARTESIAN_POINT('Ctrl Pts',(-22.8051809987834,7.66545684920987,
12.));
#179795=CARTESIAN_POINT('Ctrl Pts',(-22.8268998887679,7.66474484198553,
12.));
#179796=CARTESIAN_POINT('Ctrl Pts',(-22.8487154155569,7.66397328929805,
12.));
#179797=CARTESIAN_POINT('Ctrl Pts',(-22.870626846128,7.66314184287334,12.));
#179798=CARTESIAN_POINT('Ctrl Pts',(-22.8926334544879,7.66225015950147,
12.));
#179799=CARTESIAN_POINT('Ctrl Pts',(-22.9147345215418,7.661297900941,12.));
#179800=CARTESIAN_POINT('Ctrl Pts',(-22.9369293349592,7.66028473382777,
12.));
#179801=CARTESIAN_POINT('Ctrl Pts',(-22.9592171890332,7.65921032958912,
12.));
#179802=CARTESIAN_POINT('Ctrl Pts',(-22.9815973845301,7.65807436436453,
12.));
#179803=CARTESIAN_POINT('Ctrl Pts',(-23.004069228582,7.6568765189133,12.));
#179804=CARTESIAN_POINT('Ctrl Pts',(-23.0266320345792,7.65561647852555,
12.));
#179805=CARTESIAN_POINT('Ctrl Pts',(-23.049285122053,7.65429393293955,12.));
#179806=CARTESIAN_POINT('Ctrl Pts',(-23.072027816555,7.65290857626356,12.));
#179807=CARTESIAN_POINT('Ctrl Pts',(-23.0948594495246,7.65146010690464,
12.));
#179808=CARTESIAN_POINT('Ctrl Pts',(-23.1177793581674,7.64994822749845,
12.));
#179809=CARTESIAN_POINT('Ctrl Pts',(-23.1407868853815,7.64837264482929,
12.));
#179810=CARTESIAN_POINT('Ctrl Pts',(-23.1638813796691,7.64673306975797,
12.));
#179811=CARTESIAN_POINT('Ctrl Pts',(-23.1870621950452,7.64502921715483,
12.));
#179812=CARTESIAN_POINT('Ctrl Pts',(-23.2103286909399,7.64326080583684,
12.));
#179813=CARTESIAN_POINT('Ctrl Pts',(-23.2336802320912,7.64142755851508,
12.));
#179814=CARTESIAN_POINT('Ctrl Pts',(-23.2571161884487,7.63952920172837,
12.));
#179815=CARTESIAN_POINT('Ctrl Pts',(-23.2806359350853,7.63756546576375,
12.));
#179816=CARTESIAN_POINT('Ctrl Pts',(-23.3042388521021,7.63553608458784,
12.));
#179817=CARTESIAN_POINT('Ctrl Pts',(-23.3279243245241,7.63344079578162,
12.));
#179818=CARTESIAN_POINT('Ctrl Pts',(-23.3516917421973,7.63127934048139,
12.));
#179819=CARTESIAN_POINT('Ctrl Pts',(-23.3755404996638,7.62905146332598,
12.));
#179820=CARTESIAN_POINT('Ctrl Pts',(-23.3994699961122,7.62675691240335,
12.));
#179821=CARTESIAN_POINT('Ctrl Pts',(-23.4234796353544,7.62439543920054,
12.));
#179822=CARTESIAN_POINT('Ctrl Pts',(-23.4475688257854,7.62196679855957,
12.));
#179823=CARTESIAN_POINT('Ctrl Pts',(-23.4717369803438,7.61947074863977,
12.));
#179824=CARTESIAN_POINT('Ctrl Pts',(-23.4959835164608,7.61690705088319,
12.));
#179825=CARTESIAN_POINT('Ctrl Pts',(-23.5203078560128,7.61427546999299,
12.));
#179826=CARTESIAN_POINT('Ctrl Pts',(-23.5447094252029,7.61157577385372,
12.));
#179827=CARTESIAN_POINT('Ctrl Pts',(-23.5691876544243,7.60880773344599,
12.));
#179828=CARTESIAN_POINT('Ctrl Pts',(-23.5937419781244,7.60597112277094,
12.));
#179829=CARTESIAN_POINT('Ctrl Pts',(-23.6183718346576,7.60306571877806,
12.));
#179830=CARTESIAN_POINT('Ctrl Pts',(-23.6430766661419,7.60009130130129,
12.));
#179831=CARTESIAN_POINT('Ctrl Pts',(-23.6678559182876,7.59704765299572,
12.));
#179832=CARTESIAN_POINT('Ctrl Pts',(-23.6927090405067,7.59393455934042,
12.));
#179833=CARTESIAN_POINT('Ctrl Pts',(-23.7176354860457,7.59075180865327,
12.));
#179834=CARTESIAN_POINT('Ctrl Pts',(-23.7426347121006,7.58749919210832,
12.));
#179835=CARTESIAN_POINT('Ctrl Pts',(-23.7677061799376,7.58417650376272,
12.));
#179836=CARTESIAN_POINT('Ctrl Pts',(-23.7928493549908,7.58078354058212,
12.));
#179837=CARTESIAN_POINT('Ctrl Pts',(-23.8180637069977,7.57732010249066,
12.));
#179838=CARTESIAN_POINT('Ctrl Pts',(-23.8433487096134,7.57378599219816,
12.));
#179839=CARTESIAN_POINT('Ctrl Pts',(-23.8687038399598,7.57018101500711,
12.));
#179840=CARTESIAN_POINT('Ctrl Pts',(-23.8941285782003,7.56650497863792,
12.));
#179841=CARTESIAN_POINT('Ctrl Pts',(-23.9196224070759,7.56275769304773,
12.));
#179842=CARTESIAN_POINT('Ctrl Pts',(-23.9451848115,7.55893897027682,12.));
#179843=CARTESIAN_POINT('Ctrl Pts',(-23.9708152779884,7.55504862424812,
12.));
#179844=CARTESIAN_POINT('Ctrl Pts',(-23.9965132953185,7.55108647097441,
12.));
#179845=CARTESIAN_POINT('Ctrl Pts',(-24.022278355453,7.5470523288591,12.));
#179846=CARTESIAN_POINT('Ctrl Pts',(-24.0481099543353,7.54294601896144,
12.));
#179847=CARTESIAN_POINT('Ctrl Pts',(-24.0740075927985,7.53876736531014,
12.));
#179848=CARTESIAN_POINT('Ctrl Pts',(-24.0999707772642,7.53451619514649,
12.));
#179849=CARTESIAN_POINT('Ctrl Pts',(-24.1259990209207,7.53019233935501,
12.));
#179850=CARTESIAN_POINT('Ctrl Pts',(-24.1520918425364,7.52579563201424,
12.));
#179851=CARTESIAN_POINT('Ctrl Pts',(-24.1782487641594,7.52132590953802,
12.));
#179852=CARTESIAN_POINT('Ctrl Pts',(-24.2044693092349,7.51678300997949,
12.));
#179853=CARTESIAN_POINT('Ctrl Pts',(-24.2307530003887,7.51216677222181,
12.));
#179854=CARTESIAN_POINT('Ctrl Pts',(-24.2570993577034,7.50747703535133,
12.));
#179855=CARTESIAN_POINT('Ctrl Pts',(-24.2835078958973,7.50271363765152,
12.));
#179856=CARTESIAN_POINT('Ctrl Pts',(-24.3099781253355,7.49787641695439,
12.));
#179857=CARTESIAN_POINT('Ctrl Pts',(-24.3365095573685,7.4929652125242,12.));
#179858=CARTESIAN_POINT('Ctrl Pts',(-24.3631017084524,7.48797986651908,
12.));
#179859=CARTESIAN_POINT('Ctrl Pts',(-24.3897541049254,7.48292022569301,
12.));
#179860=CARTESIAN_POINT('Ctrl Pts',(-24.4164662871163,7.47778614286565,
12.));
#179861=CARTESIAN_POINT('Ctrl Pts',(-24.443237814649,7.47257747883246,12.));
#179862=CARTESIAN_POINT('Ctrl Pts',(-24.4700682684524,7.46729410308786,
12.));
#179863=CARTESIAN_POINT('Ctrl Pts',(-24.4969572391483,7.46193588961463,
12.));
#179864=CARTESIAN_POINT('Ctrl Pts',(-24.5239043173072,7.45650271335862,
12.));
#179865=CARTESIAN_POINT('Ctrl Pts',(-24.5509090831559,7.4509944465116,12.));
#179866=CARTESIAN_POINT('Ctrl Pts',(-24.577971096086,7.44541095473134,12.));
#179867=CARTESIAN_POINT('Ctrl Pts',(-24.6050898852368,7.43975209375504,
12.));
#179868=CARTESIAN_POINT('Ctrl Pts',(-24.6322649369517,7.43401770489524,
12.));
#179869=CARTESIAN_POINT('Ctrl Pts',(-24.6594957128756,7.42820762159126,
12.));
#179870=CARTESIAN_POINT('Ctrl Pts',(-24.6867816727192,7.42232167766265,
12.));
#179871=CARTESIAN_POINT('Ctrl Pts',(-24.7141222950051,7.41635971481674,
12.));
#179872=CARTESIAN_POINT('Ctrl Pts',(-24.7415170994784,7.41032159082382,
12.));
#179873=CARTESIAN_POINT('Ctrl Pts',(-24.7689656668983,7.40420718661603,
12.));
#179874=CARTESIAN_POINT('Ctrl Pts',(-24.7964676646431,7.39801641583013,
12.));
#179875=CARTESIAN_POINT('Ctrl Pts',(-24.8240228520893,7.39174922585808,
12.));
#179876=CARTESIAN_POINT('Ctrl Pts',(-24.8516310625176,7.38540558903621,
12.));
#179877=CARTESIAN_POINT('Ctrl Pts',(-24.8792921911115,7.3789854964027,12.));
#179878=CARTESIAN_POINT('Ctrl Pts',(-24.901463382605,7.37378825961676,12.));
#179879=CARTESIAN_POINT('Ctrl Pts',(-24.9181155530543,7.3698559312009,12.));
#179880=CARTESIAN_POINT('Ctrl Pts',(-24.9292275670674,7.36721909028843,
12.));
#179881=CARTESIAN_POINT('Ctrl Pts',(-24.9347862158358,7.36589684767345,
12.));
#179882=CARTESIAN_POINT('',(-25.2771067246846,6.08833931617699,12.));
#179883=CARTESIAN_POINT('Origin',(0.,0.,12.));
#179884=CARTESIAN_POINT('',(-22.1738711152697,4.11585220600461,12.));
#179885=CARTESIAN_POINT('Ctrl Pts',(-25.2771067246846,6.08833931617699,
12.));
#179886=CARTESIAN_POINT('Ctrl Pts',(-25.2729539149517,6.08441489609793,
12.));
#179887=CARTESIAN_POINT('Ctrl Pts',(-25.2646490489923,6.0765753178749,12.));
#179888=CARTESIAN_POINT('Ctrl Pts',(-25.2521940105705,6.06484373634546,
12.));
#179889=CARTESIAN_POINT('Ctrl Pts',(-25.2355918139032,6.04925720151218,
12.));
#179890=CARTESIAN_POINT('Ctrl Pts',(-25.21484662016,6.02986667389996,12.));
#179891=CARTESIAN_POINT('Ctrl Pts',(-25.1941090269819,6.01056881804612,
12.));
#179892=CARTESIAN_POINT('Ctrl Pts',(-25.1733791296259,5.99136367859754,
12.));
#179893=CARTESIAN_POINT('Ctrl Pts',(-25.1526570863092,5.97225131495616,
12.));
#179894=CARTESIAN_POINT('Ctrl Pts',(-25.1319431317237,5.95323180187378,
12.));
#179895=CARTESIAN_POINT('Ctrl Pts',(-25.1112375971106,5.93430523086834,
12.));
#179896=CARTESIAN_POINT('Ctrl Pts',(-25.0905409050773,5.91547170844447,
12.));
#179897=CARTESIAN_POINT('Ctrl Pts',(-25.0698535426514,5.89673135155514,
12.));
#179898=CARTESIAN_POINT('Ctrl Pts',(-25.0491760405911,5.87808428385365,
12.));
#179899=CARTESIAN_POINT('Ctrl Pts',(-25.0285089498899,5.85953063156826,
12.));
#179900=CARTESIAN_POINT('Ctrl Pts',(-25.0078528200564,5.84107051963071,
12.));
#179901=CARTESIAN_POINT('Ctrl Pts',(-24.9872081752734,5.82270406744198,
12.));
#179902=CARTESIAN_POINT('Ctrl Pts',(-24.9665754954496,5.80443138549726,
12.));
#179903=CARTESIAN_POINT('Ctrl Pts',(-24.945955229334,5.78625257775681,12.));
#179904=CARTESIAN_POINT('Ctrl Pts',(-24.9253478043656,5.76816774342219,
12.));
#179905=CARTESIAN_POINT('Ctrl Pts',(-24.904753637648,5.75017697890804,12.));
#179906=CARTESIAN_POINT('Ctrl Pts',(-24.884173146722,5.73228037976926,12.));
#179907=CARTESIAN_POINT('Ctrl Pts',(-24.8636067597669,5.71447804252027,
12.));
#179908=CARTESIAN_POINT('Ctrl Pts',(-24.8430549277621,5.69677006679444,
12.));
#179909=CARTESIAN_POINT('Ctrl Pts',(-24.8225181223845,5.67915655496542,
12.));
#179910=CARTESIAN_POINT('Ctrl Pts',(-24.8019968304605,5.66163761114921,
12.));
#179911=CARTESIAN_POINT('Ctrl Pts',(-24.781491549672,5.6442133404226,12.));
#179912=CARTESIAN_POINT('Ctrl Pts',(-24.7610027835697,5.62688384790923,
12.));
#179913=CARTESIAN_POINT('Ctrl Pts',(-24.7405310372739,5.60964923798491,
12.));
#179914=CARTESIAN_POINT('Ctrl Pts',(-24.7200768119088,5.59250961323987,
12.));
#179915=CARTESIAN_POINT('Ctrl Pts',(-24.6996406035517,5.57546507427754,
12.));
#179916=CARTESIAN_POINT('Ctrl Pts',(-24.6792229061794,5.55851572025376,
12.));
#179917=CARTESIAN_POINT('Ctrl Pts',(-24.6588242134738,5.54166164919583,
12.));
#179918=CARTESIAN_POINT('Ctrl Pts',(-24.6384450211467,5.52490295840991,
12.));
#179919=CARTESIAN_POINT('Ctrl Pts',(-24.6180858289179,5.50823974481962,
12.));
#179920=CARTESIAN_POINT('Ctrl Pts',(-24.5977471429364,5.49167210537246,
12.));
#179921=CARTESIAN_POINT('Ctrl Pts',(-24.5774294770329,5.47520013724419,
12.));
#179922=CARTESIAN_POINT('Ctrl Pts',(-24.5571333514842,5.45882393762261,
12.));
#179923=CARTESIAN_POINT('Ctrl Pts',(-24.5368592922863,5.4425436035688,12.));
#179924=CARTESIAN_POINT('Ctrl Pts',(-24.5166078302108,5.42635923183419,
12.));
#179925=CARTESIAN_POINT('Ctrl Pts',(-24.4963794999831,5.41027091869241,
12.));
#179926=CARTESIAN_POINT('Ctrl Pts',(-24.4761748393321,5.39427875973824,
12.));
#179927=CARTESIAN_POINT('Ctrl Pts',(-24.4559943883157,5.37838284973695,
12.));
#179928=CARTESIAN_POINT('Ctrl Pts',(-24.435838689915,5.36258328273627,12.));
#179929=CARTESIAN_POINT('Ctrl Pts',(-24.4157082904614,5.34688015213537,
12.));
#179930=CARTESIAN_POINT('Ctrl Pts',(-24.3956037401293,5.33127355076033,
12.));
#179931=CARTESIAN_POINT('Ctrl Pts',(-24.3755255933917,5.31576357092526,
12.));
#179932=CARTESIAN_POINT('Ctrl Pts',(-24.3554744095075,5.30035030449063,
12.));
#179933=CARTESIAN_POINT('Ctrl Pts',(-24.3354507529414,5.28503384290648,
12.));
#179934=CARTESIAN_POINT('Ctrl Pts',(-24.3154551932221,5.26981427718798,
12.));
#179935=CARTESIAN_POINT('Ctrl Pts',(-24.2954883048447,5.25469169788856,
12.));
#179936=CARTESIAN_POINT('Ctrl Pts',(-24.2755506671525,5.23966619506289,
12.));
#179937=CARTESIAN_POINT('Ctrl Pts',(-24.2556428642294,5.22473785822442,
12.));
#179938=CARTESIAN_POINT('Ctrl Pts',(-24.2357654847766,5.20990677629176,
12.));
#179939=CARTESIAN_POINT('Ctrl Pts',(-24.2159191220171,5.19517303753647,
12.));
#179940=CARTESIAN_POINT('Ctrl Pts',(-24.1961043738756,5.18053672961398,
12.));
#179941=CARTESIAN_POINT('Ctrl Pts',(-24.1763218431344,5.16599793957985,
12.));
#179942=CARTESIAN_POINT('Ctrl Pts',(-24.1565721375971,5.15155675390079,
12.));
#179943=CARTESIAN_POINT('Ctrl Pts',(-24.1368558702443,5.13721325845745,
12.));
#179944=CARTESIAN_POINT('Ctrl Pts',(-24.117173659394,5.12296753853857,12.));
#179945=CARTESIAN_POINT('Ctrl Pts',(-24.0975261288444,5.10881967883124,
12.));
#179946=CARTESIAN_POINT('Ctrl Pts',(-24.0779139079264,5.09476976342616,
12.));
#179947=CARTESIAN_POINT('Ctrl Pts',(-24.0583376315636,5.0808178758127,12.));
#179948=CARTESIAN_POINT('Ctrl Pts',(-24.0387979403268,5.06696409886639,
12.));
#179949=CARTESIAN_POINT('Ctrl Pts',(-24.0192954804896,5.05320851483068,
12.));
#179950=CARTESIAN_POINT('Ctrl Pts',(-23.9998309040747,5.03955120528527,
12.));
#179951=CARTESIAN_POINT('Ctrl Pts',(-23.9804048689228,5.02599225112461,
12.));
#179952=CARTESIAN_POINT('Ctrl Pts',(-23.9610180388271,5.01253173257458,
12.));
#179953=CARTESIAN_POINT('Ctrl Pts',(-23.9416710836529,4.99916972919309,
12.));
#179954=CARTESIAN_POINT('Ctrl Pts',(-23.9223646794591,4.98590631986532,
12.));
#179955=CARTESIAN_POINT('Ctrl Pts',(-23.9030995086164,4.97274158279228,
12.));
#179956=CARTESIAN_POINT('Ctrl Pts',(-23.883876259922,4.95967559546565,12.));
#179957=CARTESIAN_POINT('Ctrl Pts',(-23.8646956287172,4.94670843465868,
12.));
#179958=CARTESIAN_POINT('Ctrl Pts',(-23.8455583170062,4.93384017643441,
12.));
#179959=CARTESIAN_POINT('Ctrl Pts',(-23.8264650335721,4.92107089613976,
12.));
#179960=CARTESIAN_POINT('Ctrl Pts',(-23.8074164940897,4.90840066839346,
12.));
#179961=CARTESIAN_POINT('Ctrl Pts',(-23.7884134212381,4.89582956706771,
12.));
#179962=CARTESIAN_POINT('Ctrl Pts',(-23.7694565448044,4.88335766525565,
12.));
#179963=CARTESIAN_POINT('Ctrl Pts',(-23.7505466018239,4.87098503527142,
12.));
#179964=CARTESIAN_POINT('Ctrl Pts',(-23.7316843367308,4.85871174865491,
12.));
#179965=CARTESIAN_POINT('Ctrl Pts',(-23.7128705015014,4.84653787616422,
12.));
#179966=CARTESIAN_POINT('Ctrl Pts',(-23.6941058557971,4.83446348776267,
12.));
#179967=CARTESIAN_POINT('Ctrl Pts',(-23.6753911671023,4.82248865259569,
12.));
#179968=CARTESIAN_POINT('Ctrl Pts',(-23.6567272108631,4.81061343896442,
12.));
#179969=CARTESIAN_POINT('Ctrl Pts',(-23.6381147706581,4.79883791433229,
12.));
#179970=CARTESIAN_POINT('Ctrl Pts',(-23.6195546383625,4.78716214532104,
12.));
#179971=CARTESIAN_POINT('Ctrl Pts',(-23.6010476143099,4.77558619769875,
12.));
#179972=CARTESIAN_POINT('Ctrl Pts',(-23.5825945074535,4.7641101363625,12.));
#179973=CARTESIAN_POINT('Ctrl Pts',(-23.564196135517,4.75273402530615,12.));
#179974=CARTESIAN_POINT('Ctrl Pts',(-23.5458533251715,4.74145792760698,
12.));
#179975=CARTESIAN_POINT('Ctrl Pts',(-23.5275669122378,4.73028190543031,
12.));
#179976=CARTESIAN_POINT('Ctrl Pts',(-23.5093377418784,4.71920602001904,
12.));
#179977=CARTESIAN_POINT('Ctrl Pts',(-23.491166668789,4.7082303316782,12.));
#179978=CARTESIAN_POINT('Ctrl Pts',(-23.4730545573849,4.69735489975023,
12.));
#179979=CARTESIAN_POINT('Ctrl Pts',(-23.4550022819853,4.68657978258297,
12.));
#179980=CARTESIAN_POINT('Ctrl Pts',(-23.4370107270444,4.6759050375305,12.));
#179981=CARTESIAN_POINT('Ctrl Pts',(-23.4190807873798,4.66533072094663,
12.));
#179982=CARTESIAN_POINT('Ctrl Pts',(-23.4012133683957,4.65485688816921,
12.));
#179983=CARTESIAN_POINT('Ctrl Pts',(-23.383409386307,4.64448359349935,12.));
#179984=CARTESIAN_POINT('Ctrl Pts',(-23.3656697683496,4.63421089016554,
12.));
#179985=CARTESIAN_POINT('Ctrl Pts',(-23.3479954530281,4.62403883030823,
12.));
#179986=CARTESIAN_POINT('Ctrl Pts',(-23.3303873903947,4.61396746497848,
12.));
#179987=CARTESIAN_POINT('Ctrl Pts',(-23.3128465423119,4.60399684412174,
12.));
#179988=CARTESIAN_POINT('Ctrl Pts',(-23.295373882719,4.59412701655749,12.));
#179989=CARTESIAN_POINT('Ctrl Pts',(-23.2779703978868,4.58435802994674,
12.));
#179990=CARTESIAN_POINT('Ctrl Pts',(-23.2606370866853,4.5746899307607,12.));
#179991=CARTESIAN_POINT('Ctrl Pts',(-23.2433749609117,4.5651227642781,12.));
#179992=CARTESIAN_POINT('Ctrl Pts',(-23.2261850456055,4.55565657456956,
12.));
#179993=CARTESIAN_POINT('Ctrl Pts',(-23.2090683793627,4.54629140447542,
12.));
#179994=CARTESIAN_POINT('Ctrl Pts',(-23.1920260146474,4.53702729557585,
12.));
#179995=CARTESIAN_POINT('Ctrl Pts',(-23.1750590180923,4.52786428815047,
12.));
#179996=CARTESIAN_POINT('Ctrl Pts',(-23.1581684708778,4.51880242116785,
12.));
#179997=CARTESIAN_POINT('Ctrl Pts',(-23.1413554691136,4.50984173227087,
12.));
#179998=CARTESIAN_POINT('Ctrl Pts',(-23.1246211242117,4.50098225775178,
12.));
#179999=CARTESIAN_POINT('Ctrl Pts',(-23.1079665632629,4.49222403252201,
12.));
#180000=CARTESIAN_POINT('Ctrl Pts',(-23.0913929293909,4.48356709006756,
12.));
#180001=CARTESIAN_POINT('Ctrl Pts',(-23.0749013821868,4.47501146242821,
12.));
#180002=CARTESIAN_POINT('Ctrl Pts',(-23.0584930981723,4.46655718018205,
12.));
#180003=CARTESIAN_POINT('Ctrl Pts',(-23.0421692712466,4.45820427241676,
12.));
#180004=CARTESIAN_POINT('Ctrl Pts',(-23.0259311131395,4.44995276669698,
12.));
#180005=CARTESIAN_POINT('Ctrl Pts',(-23.0097798538399,4.44180268901666,
12.));
#180006=CARTESIAN_POINT('Ctrl Pts',(-22.9937167421009,4.43375406376904,
12.));
#180007=CARTESIAN_POINT('Ctrl Pts',(-22.9777430460021,4.42580691372771,
12.));
#180008=CARTESIAN_POINT('Ctrl Pts',(-22.9618600534866,4.41796126001309,
12.));
#180009=CARTESIAN_POINT('Ctrl Pts',(-22.9460690729093,4.41021712205547,
12.));
#180010=CARTESIAN_POINT('Ctrl Pts',(-22.9303714335549,4.40257451754307,
12.));
#180011=CARTESIAN_POINT('Ctrl Pts',(-22.9147684862425,4.39503346238454,
12.));
#180012=CARTESIAN_POINT('Ctrl Pts',(-22.8992616040108,4.38759397068391,
12.));
#180013=CARTESIAN_POINT('Ctrl Pts',(-22.8838521827702,4.38025605470089,
12.));
#180014=CARTESIAN_POINT('Ctrl Pts',(-22.8685416419725,4.37301972480752,
12.));
#180015=CARTESIAN_POINT('Ctrl Pts',(-22.8533314252419,4.36588498943009,
12.));
#180016=CARTESIAN_POINT('Ctrl Pts',(-22.838223001118,4.35885185500559,12.));
#180017=CARTESIAN_POINT('Ctrl Pts',(-22.8232178638873,4.35192032594801,
12.));
#180018=CARTESIAN_POINT('Ctrl Pts',(-22.808317534379,4.34509040460065,12.));
#180019=CARTESIAN_POINT('Ctrl Pts',(-22.7935235607807,4.33836209118442,
12.));
#180020=CARTESIAN_POINT('Ctrl Pts',(-22.7788375194081,4.33173538373182,
12.));
#180021=CARTESIAN_POINT('Ctrl Pts',(-22.764261015648,4.32521027803747,12.));
#180022=CARTESIAN_POINT('Ctrl Pts',(-22.7497956849852,4.3187867676123,12.));
#180023=CARTESIAN_POINT('Ctrl Pts',(-22.7354431939927,4.3124648436255,12.));
#180024=CARTESIAN_POINT('Ctrl Pts',(-22.7212052413384,4.30624449484074,
12.));
#180025=CARTESIAN_POINT('Ctrl Pts',(-22.707083558756,4.30012570754066,12.));
#180026=CARTESIAN_POINT('Ctrl Pts',(-22.6930799122545,4.29410846547061,
12.));
#180027=CARTESIAN_POINT('Ctrl Pts',(-22.6791961033537,4.28819274977766,
12.));
#180028=CARTESIAN_POINT('Ctrl Pts',(-22.665433970311,4.28237853894059,12.));
#180029=CARTESIAN_POINT('Ctrl Pts',(-22.6517953893303,4.27666580869117,
12.));
#180030=CARTESIAN_POINT('Ctrl Pts',(-22.6382822758171,4.27105453192999,
12.));
#180031=CARTESIAN_POINT('Ctrl Pts',(-22.6248965859975,4.26554467865571,
12.));
#180032=CARTESIAN_POINT('Ctrl Pts',(-22.611640318482,4.26013621588303,12.));
#180033=CARTESIAN_POINT('Ctrl Pts',(-22.5985155158637,4.25482910755485,
12.));
#180034=CARTESIAN_POINT('Ctrl Pts',(-22.5855242662479,4.24962331444184,
12.));
#180035=CARTESIAN_POINT('Ctrl Pts',(-22.5726687049922,4.24451879404858,
12.));
#180036=CARTESIAN_POINT('Ctrl Pts',(-22.559951016643,4.23951550052526,12.));
#180037=CARTESIAN_POINT('Ctrl Pts',(-22.5473734368086,4.23461338456713,
12.));
#180038=CARTESIAN_POINT('Ctrl Pts',(-22.5349382540587,4.22981239330731,
12.));
#180039=CARTESIAN_POINT('Ctrl Pts',(-22.5226478117885,4.2251124702004,12.));
#180040=CARTESIAN_POINT('Ctrl Pts',(-22.5105045108882,4.22051355490196,
12.));
#180041=CARTESIAN_POINT('Ctrl Pts',(-22.4985108124229,4.21601558313908,
12.));
#180042=CARTESIAN_POINT('Ctrl Pts',(-22.4866692403147,4.21161848657428,
12.));
#180043=CARTESIAN_POINT('Ctrl Pts',(-22.4749823839915,4.20732219265648,
12.));
#180044=CARTESIAN_POINT('Ctrl Pts',(-22.4634529011433,4.2031266244817,12.));
#180045=CARTESIAN_POINT('Ctrl Pts',(-22.4520835205419,4.19903170066354,
12.));
#180046=CARTESIAN_POINT('Ctrl Pts',(-22.4408770448917,4.1950373351886,12.));
#180047=CARTESIAN_POINT('Ctrl Pts',(-22.4298363535421,4.19114343726941,
12.));
#180048=CARTESIAN_POINT('Ctrl Pts',(-22.4189644056115,4.1873499111772,12.));
#180049=CARTESIAN_POINT('Ctrl Pts',(-22.4082642454453,4.1836566560085,12.));
#180050=CARTESIAN_POINT('Ctrl Pts',(-22.3977390078075,4.18006356544882,
12.));
#180051=CARTESIAN_POINT('Ctrl Pts',(-22.3873919231334,4.17657052752825,
12.));
#180052=CARTESIAN_POINT('Ctrl Pts',(-22.3772263228617,4.17317742436145,
12.));
#180053=CARTESIAN_POINT('Ctrl Pts',(-22.36724564276,4.16988413199457,12.));
#180054=CARTESIAN_POINT('Ctrl Pts',(-22.3574534257396,4.166690520266,12.));
#180055=CARTESIAN_POINT('Ctrl Pts',(-22.3478533253889,4.16359645263187,
12.));
#180056=CARTESIAN_POINT('Ctrl Pts',(-22.3384491078602,4.16060178604164,
12.));
#180057=CARTESIAN_POINT('Ctrl Pts',(-22.3292446628959,4.15770637047889,
12.));
#180058=CARTESIAN_POINT('Ctrl Pts',(-22.3202440186979,4.15491004835281,
12.));
#180059=CARTESIAN_POINT('Ctrl Pts',(-22.3114513545185,4.1522126539699,12.));
#180060=CARTESIAN_POINT('Ctrl Pts',(-22.3028710166933,4.14961401285522,
12.));
#180061=CARTESIAN_POINT('Ctrl Pts',(-22.2945075198467,4.14711394168556,
12.));
#180062=CARTESIAN_POINT('Ctrl Pts',(-22.2863655389166,4.14471224859295,
12.));
#180063=CARTESIAN_POINT('Ctrl Pts',(-22.2784499072027,4.14240873321984,
12.));
#180064=CARTESIAN_POINT('Ctrl Pts',(-22.2707656042457,4.14020318715991,
12.));
#180065=CARTESIAN_POINT('Ctrl Pts',(-22.2633177913972,4.13809539255421,
12.));
#180066=CARTESIAN_POINT('Ctrl Pts',(-22.2561118708421,4.13608511977225,
12.));
#180067=CARTESIAN_POINT('Ctrl Pts',(-22.249153531779,4.1341721255881,12.));
#180068=CARTESIAN_POINT('Ctrl Pts',(-22.2424488153523,4.1323561506016,12.));
#180069=CARTESIAN_POINT('Ctrl Pts',(-22.2360040565533,4.13063692157498,
12.));
#180070=CARTESIAN_POINT('Ctrl Pts',(-22.2298258043947,4.12901415463379,
12.));
#180071=CARTESIAN_POINT('Ctrl Pts',(-22.2239207458781,4.12748755830104,
12.));
#180072=CARTESIAN_POINT('Ctrl Pts',(-22.2182956401341,4.12605683613307,
12.));
#180073=CARTESIAN_POINT('Ctrl Pts',(-22.2129576146671,4.12472167516607,
12.));
#180074=CARTESIAN_POINT('Ctrl Pts',(-22.2079143941719,4.12348173702023,
12.));
#180075=CARTESIAN_POINT('Ctrl Pts',(-22.2031746532106,4.12233664408227,
12.));
#180076=CARTESIAN_POINT('Ctrl Pts',(-22.1987479618246,4.12128598183522,
12.));
#180077=CARTESIAN_POINT('Ctrl Pts',(-22.1946440958098,4.12032932637736,
12.));
#180078=CARTESIAN_POINT('Ctrl Pts',(-22.1908725908525,4.11946626228636,
12.));
#180079=CARTESIAN_POINT('Ctrl Pts',(-22.1874419861496,4.11869641271773,
12.));
#180080=CARTESIAN_POINT('Ctrl Pts',(-22.1843613164855,4.11801938107479,
12.));
#180081=CARTESIAN_POINT('Ctrl Pts',(-22.1816414985788,4.11743469691756,
12.));
#180082=CARTESIAN_POINT('Ctrl Pts',(-22.179297473024,4.11694173195003,12.));
#180083=CARTESIAN_POINT('Ctrl Pts',(-22.177347426894,4.11653973150518,12.));
#180084=CARTESIAN_POINT('Ctrl Pts',(-22.1758088296598,4.11622797217068,
12.));
#180085=CARTESIAN_POINT('Ctrl Pts',(-22.1746949858775,4.11600589882845,
12.));
#180086=CARTESIAN_POINT('Ctrl Pts',(-22.1741488021234,4.11589976826166,
12.));
#180087=CARTESIAN_POINT('Ctrl Pts',(-22.1739341411687,4.11586035878287,
12.));
#180088=CARTESIAN_POINT('Ctrl Pts',(-22.173877682324,4.11585194677442,12.));
#180089=CARTESIAN_POINT('Ctrl Pts',(-22.1738711152697,4.11585220600461,
12.));
#180090=CARTESIAN_POINT('',(-21.624941921198,4.01396149767429,12.));
#180091=CARTESIAN_POINT('',(-10.5694630535049,1.96187429785751,12.));
#180092=CARTESIAN_POINT('',(-21.2226420728916,3.44230496120419,12.));
#180093=CARTESIAN_POINT('Origin',(-21.7161918885402,3.52235856495312,12.));
#180094=CARTESIAN_POINT('',(-21.3904321633055,2.16781269186828,12.));
#180095=CARTESIAN_POINT('Origin',(-7.6920903736728E-13,1.31973449697531E-13,
12.));
#180096=CARTESIAN_POINT('',(-21.9269795755927,1.71975774210842,12.));
#180097=CARTESIAN_POINT('Origin',(-21.8878840740801,2.21822694051638,12.));
#180098=CARTESIAN_POINT('',(-22.4835757167854,1.7634122053118,12.));
#180099=CARTESIAN_POINT('',(-11.2417878583927,0.881706102655883,12.));
#180100=CARTESIAN_POINT('',(-25.991588367311,0.661312440730901,12.));
#180101=CARTESIAN_POINT('Ctrl Pts',(-22.4835757167854,1.7634122053118,12.));
#180102=CARTESIAN_POINT('Ctrl Pts',(-22.4835819929788,1.7634141553879,12.));
#180103=CARTESIAN_POINT('Ctrl Pts',(-22.4836387052228,1.76342064263637,
12.));
#180104=CARTESIAN_POINT('Ctrl Pts',(-22.4838562517064,1.76343813434659,
12.));
#180105=CARTESIAN_POINT('Ctrl Pts',(-22.4844112933125,1.76347698284861,
12.));
#180106=CARTESIAN_POINT('Ctrl Pts',(-22.4855446605991,1.76355076045549,
12.));
#180107=CARTESIAN_POINT('Ctrl Pts',(-22.4871115206572,1.76364784232925,
12.));
#180108=CARTESIAN_POINT('Ctrl Pts',(-22.4890991659479,1.76376424879468,
12.));
#180109=CARTESIAN_POINT('Ctrl Pts',(-22.4914909094908,1.76389475965714,
12.));
#180110=CARTESIAN_POINT('Ctrl Pts',(-22.4942693792449,1.76403393880316,
12.));
#180111=CARTESIAN_POINT('Ctrl Pts',(-22.4974203063191,1.76417731243483,
12.));
#180112=CARTESIAN_POINT('Ctrl Pts',(-22.5009332677316,1.76432160068737,
12.));
#180113=CARTESIAN_POINT('Ctrl Pts',(-22.5047996391978,1.76446408210364,
12.));
#180114=CARTESIAN_POINT('Ctrl Pts',(-22.5090112700212,1.76460218257313,
12.));
#180115=CARTESIAN_POINT('Ctrl Pts',(-22.5135590569554,1.76473303281149,
12.));
#180116=CARTESIAN_POINT('Ctrl Pts',(-22.5184336670207,1.76485369319895,
12.));
#180117=CARTESIAN_POINT('Ctrl Pts',(-22.5236259635515,1.76496128643375,
12.));
#180118=CARTESIAN_POINT('Ctrl Pts',(-22.529127665298,1.76505320262759,12.));
#180119=CARTESIAN_POINT('Ctrl Pts',(-22.5349313983571,1.76512711563254,
12.));
#180120=CARTESIAN_POINT('Ctrl Pts',(-22.5410303590892,1.76518087841493,
12.));
#180121=CARTESIAN_POINT('Ctrl Pts',(-22.5474180954006,1.76521245524047,
12.));
#180122=CARTESIAN_POINT('Ctrl Pts',(-22.5540882235837,1.76521983384062,
12.));
#180123=CARTESIAN_POINT('Ctrl Pts',(-22.5610344912501,1.7652010450045,12.));
#180124=CARTESIAN_POINT('Ctrl Pts',(-22.5682508499873,1.76515418518831,
12.));
#180125=CARTESIAN_POINT('Ctrl Pts',(-22.5757315316353,1.76507744026746,
12.));
#180126=CARTESIAN_POINT('Ctrl Pts',(-22.5834711038022,1.76496910283088,
12.));
#180127=CARTESIAN_POINT('Ctrl Pts',(-22.5914644078106,1.76482755288411,
12.));
#180128=CARTESIAN_POINT('Ctrl Pts',(-22.5997065145638,1.76465124413557,
12.));
#180129=CARTESIAN_POINT('Ctrl Pts',(-22.6081926681343,1.76443868648015,
12.));
#180130=CARTESIAN_POINT('Ctrl Pts',(-22.6169182517694,1.76418843543739,
12.));
#180131=CARTESIAN_POINT('Ctrl Pts',(-22.6258787994848,1.76389909571403,
12.));
#180132=CARTESIAN_POINT('Ctrl Pts',(-22.6350699979359,1.76356932176273,
12.));
#180133=CARTESIAN_POINT('Ctrl Pts',(-22.6444876940423,1.76319782013916,
12.));
#180134=CARTESIAN_POINT('Ctrl Pts',(-22.6541278938409,1.76278334912561,
12.));
#180135=CARTESIAN_POINT('Ctrl Pts',(-22.6639867471753,1.76232471392568,
12.));
#180136=CARTESIAN_POINT('Ctrl Pts',(-22.67406053567,1.76182076289525,12.));
#180137=CARTESIAN_POINT('Ctrl Pts',(-22.684345658525,1.76127038310614,12.));
#180138=CARTESIAN_POINT('Ctrl Pts',(-22.6948386219851,1.76067249704886,
12.));
#180139=CARTESIAN_POINT('Ctrl Pts',(-22.7055360375485,1.76002606202401,
12.));
#180140=CARTESIAN_POINT('Ctrl Pts',(-22.7164346186006,1.75933006905925,
12.));
#180141=CARTESIAN_POINT('Ctrl Pts',(-22.72753117773,1.75858354204633,12.));
#180142=CARTESIAN_POINT('Ctrl Pts',(-22.7388226235559,1.75778553673244,
12.));
#180143=CARTESIAN_POINT('Ctrl Pts',(-22.750305955645,1.75693513908907,12.));
#180144=CARTESIAN_POINT('Ctrl Pts',(-22.7619782595013,1.75603146371641,
12.));
#180145=CARTESIAN_POINT('Ctrl Pts',(-22.7738367016118,1.75507365227131,
12.));
#180146=CARTESIAN_POINT('Ctrl Pts',(-22.7858785242361,1.75406087182936,
12.));
#180147=CARTESIAN_POINT('Ctrl Pts',(-22.7981010424314,1.75299231391466,
12.));
#180148=CARTESIAN_POINT('Ctrl Pts',(-22.8105016414713,1.75186719365592,
12.));
#180149=CARTESIAN_POINT('Ctrl Pts',(-22.8230777741284,1.75068474890883,
12.));
#180150=CARTESIAN_POINT('Ctrl Pts',(-22.8358269579853,1.74944423940115,
12.));
#180151=CARTESIAN_POINT('Ctrl Pts',(-22.8487467728076,1.74814494588492,
12.));
#180152=CARTESIAN_POINT('Ctrl Pts',(-22.8618348580235,1.74678616930664,
12.));
#180153=CARTESIAN_POINT('Ctrl Pts',(-22.8750889101696,1.74536722998201,
12.));
#180154=CARTESIAN_POINT('Ctrl Pts',(-22.888506680335,1.74388746677702,12.));
#180155=CARTESIAN_POINT('Ctrl Pts',(-22.9020859716141,1.7423462363008,12.));
#180156=CARTESIAN_POINT('Ctrl Pts',(-22.9158246373363,1.74074291231058,
12.));
#180157=CARTESIAN_POINT('Ctrl Pts',(-22.9297205792586,1.73907688511666,
12.));
#180158=CARTESIAN_POINT('Ctrl Pts',(-22.9437717457826,1.73734756100039,
12.));
#180159=CARTESIAN_POINT('Ctrl Pts',(-22.9579761301063,1.73555436162769,
12.));
#180160=CARTESIAN_POINT('Ctrl Pts',(-22.9723317685688,1.73369672350814,
12.));
#180161=CARTESIAN_POINT('Ctrl Pts',(-22.9868367391978,1.7317740975019,12.));
#180162=CARTESIAN_POINT('Ctrl Pts',(-23.001489160189,1.72978594832136,12.));
#180163=CARTESIAN_POINT('Ctrl Pts',(-23.0162871884168,1.72773175404708,
12.));
#180164=CARTESIAN_POINT('Ctrl Pts',(-23.0312290178883,1.72561100564045,
12.));
#180165=CARTESIAN_POINT('Ctrl Pts',(-23.0463128785531,1.72342320653746,
12.));
#180166=CARTESIAN_POINT('Ctrl Pts',(-23.0615370351562,1.72116787225991,
12.));
#180167=CARTESIAN_POINT('Ctrl Pts',(-23.0768997860709,1.71884453003027,
12.));
#180168=CARTESIAN_POINT('Ctrl Pts',(-23.0923994621213,1.71645271839296,
12.));
#180169=CARTESIAN_POINT('Ctrl Pts',(-23.1080344254286,1.71399198684704,
12.));
#180170=CARTESIAN_POINT('Ctrl Pts',(-23.1238030684925,1.71146189552174,
12.));
#180171=CARTESIAN_POINT('Ctrl Pts',(-23.1397038132356,1.70886201485452,
12.));
#180172=CARTESIAN_POINT('Ctrl Pts',(-23.1557351100614,1.70619192527852,
12.));
#180173=CARTESIAN_POINT('Ctrl Pts',(-23.1718954368751,1.70345121691276,
12.));
#180174=CARTESIAN_POINT('Ctrl Pts',(-23.1881832981851,1.7006394892701,12.));
#180175=CARTESIAN_POINT('Ctrl Pts',(-23.2045972243767,1.69775635099443,
12.));
#180176=CARTESIAN_POINT('Ctrl Pts',(-23.2211357709374,1.69480141959953,
12.));
#180177=CARTESIAN_POINT('Ctrl Pts',(-23.2377975177013,1.69177432121711,
12.));
#180178=CARTESIAN_POINT('Ctrl Pts',(-23.2545810680537,1.68867469034896,
12.));
#180179=CARTESIAN_POINT('Ctrl Pts',(-23.2714850482246,1.68550216963258,
12.));
#180180=CARTESIAN_POINT('Ctrl Pts',(-23.2885081066951,1.68225640962168,
12.));
#180181=CARTESIAN_POINT('Ctrl Pts',(-23.3056489135611,1.67893706857117,
12.));
#180182=CARTESIAN_POINT('Ctrl Pts',(-23.3229061599145,1.67554381222994,
12.));
#180183=CARTESIAN_POINT('Ctrl Pts',(-23.3402785571865,1.67207631363921,
12.));
#180184=CARTESIAN_POINT('Ctrl Pts',(-23.3577648365744,1.66853425293995,
12.));
#180185=CARTESIAN_POINT('Ctrl Pts',(-23.3753637485545,1.66491731718876,
12.));
#180186=CARTESIAN_POINT('Ctrl Pts',(-23.3930740623619,1.66122520018011,
12.));
#180187=CARTESIAN_POINT('Ctrl Pts',(-23.4108945654805,1.65745760227505,
12.));
#180188=CARTESIAN_POINT('Ctrl Pts',(-23.4288240631043,1.65361423023728,
12.));
#180189=CARTESIAN_POINT('Ctrl Pts',(-23.4468613776574,1.6496947970734,12.));
#180190=CARTESIAN_POINT('Ctrl Pts',(-23.4650053483932,1.64569902187611,
12.));
#180191=CARTESIAN_POINT('Ctrl Pts',(-23.4832548309645,1.64162662967528,
12.));
#180192=CARTESIAN_POINT('Ctrl Pts',(-23.5016086970003,1.63747735129474,
12.));
#180193=CARTESIAN_POINT('Ctrl Pts',(-23.5200658336612,1.63325092321725,
12.));
#180194=CARTESIAN_POINT('Ctrl Pts',(-23.538625143226,1.62894708745223,12.));
#180195=CARTESIAN_POINT('Ctrl Pts',(-23.5572855427601,1.62456559140064,
12.));
#180196=CARTESIAN_POINT('Ctrl Pts',(-23.57604596376,1.62010618772866,12.));
#180197=CARTESIAN_POINT('Ctrl Pts',(-23.5949053517997,1.61556863424698,
12.));
#180198=CARTESIAN_POINT('Ctrl Pts',(-23.6138626661653,1.61095269379778,
12.));
#180199=CARTESIAN_POINT('Ctrl Pts',(-23.6329168794929,1.60625813414672,
12.));
#180200=CARTESIAN_POINT('Ctrl Pts',(-23.6520669774876,1.60148472786595,
12.));
#180201=CARTESIAN_POINT('Ctrl Pts',(-23.671311958631,1.59663225222463,12.));
#180202=CARTESIAN_POINT('Ctrl Pts',(-23.6906508338833,1.59170048908633,
12.));
#180203=CARTESIAN_POINT('Ctrl Pts',(-23.710082626383,1.58668922481221,12.));
#180204=CARTESIAN_POINT('Ctrl Pts',(-23.72960637113,1.58159825017358,12.));
#180205=CARTESIAN_POINT('Ctrl Pts',(-23.749221114736,1.57642736025246,12.));
#180206=CARTESIAN_POINT('Ctrl Pts',(-23.7689259151862,1.57117635434408,
12.));
#180207=CARTESIAN_POINT('Ctrl Pts',(-23.7887198415878,1.56584503586843,
12.));
#180208=CARTESIAN_POINT('Ctrl Pts',(-23.8086019739194,1.56043321228633,
12.));
#180209=CARTESIAN_POINT('Ctrl Pts',(-23.8285714027636,1.55494069502635,
12.));
#180210=CARTESIAN_POINT('Ctrl Pts',(-23.8486272290705,1.54936729940541,
12.));
#180211=CARTESIAN_POINT('Ctrl Pts',(-23.8687685639642,1.5437128445399,12.));
#180212=CARTESIAN_POINT('Ctrl Pts',(-23.8889945285318,1.53797715326758,
12.));
#180213=CARTESIAN_POINT('Ctrl Pts',(-23.9093042536119,1.53216005207463,
12.));
#180214=CARTESIAN_POINT('Ctrl Pts',(-23.9296968795757,1.52626137103032,
12.));
#180215=CARTESIAN_POINT('Ctrl Pts',(-23.9501715561033,1.52028094372792,
12.));
#180216=CARTESIAN_POINT('Ctrl Pts',(-23.970727442014,1.51421860720614,12.));
#180217=CARTESIAN_POINT('Ctrl Pts',(-23.9913637050927,1.50807420187694,
12.));
#180218=CARTESIAN_POINT('Ctrl Pts',(-24.0120795219086,1.50184757146098,
12.));
#180219=CARTESIAN_POINT('Ctrl Pts',(-24.0328740776331,1.49553856292801,
12.));
#180220=CARTESIAN_POINT('Ctrl Pts',(-24.0537465658429,1.48914702644887,
12.));
#180221=CARTESIAN_POINT('Ctrl Pts',(-24.0746961883528,1.48267281533683,
12.));
#180222=CARTESIAN_POINT('Ctrl Pts',(-24.0957221550778,1.47611578597742,
12.));
#180223=CARTESIAN_POINT('Ctrl Pts',(-24.1168236838824,1.46947579776991,
12.));
#180224=CARTESIAN_POINT('Ctrl Pts',(-24.1380000004272,1.46275271307397,
12.));
#180225=CARTESIAN_POINT('Ctrl Pts',(-24.1592503380107,1.45594639716317,
12.));
#180226=CARTESIAN_POINT('Ctrl Pts',(-24.1805739374038,1.44905671818727,
12.));
#180227=CARTESIAN_POINT('Ctrl Pts',(-24.201970046722,1.44208354711082,12.));
#180228=CARTESIAN_POINT('Ctrl Pts',(-24.2234379212984,1.43502675765508,
12.));
#180229=CARTESIAN_POINT('Ctrl Pts',(-24.2449768235488,1.42788622624854,
12.));
#180230=CARTESIAN_POINT('Ctrl Pts',(-24.2665860228356,1.42066183198252,
12.));
#180231=CARTESIAN_POINT('Ctrl Pts',(-24.288264795321,1.41335345657682,12.));
#180232=CARTESIAN_POINT('Ctrl Pts',(-24.3100124238311,1.40596098434337,
12.));
#180233=CARTESIAN_POINT('Ctrl Pts',(-24.3318281977643,1.39848430212807,
12.));
#180234=CARTESIAN_POINT('Ctrl Pts',(-24.3537114129875,1.39092329926388,
12.));
#180235=CARTESIAN_POINT('Ctrl Pts',(-24.3756613717299,1.38327786752998,
12.));
#180236=CARTESIAN_POINT('Ctrl Pts',(-24.3976773824732,1.37554790111609,
12.));
#180237=CARTESIAN_POINT('Ctrl Pts',(-24.4197587598337,1.36773329659956,
12.));
#180238=CARTESIAN_POINT('Ctrl Pts',(-24.4419048244523,1.35983395290627,
12.));
#180239=CARTESIAN_POINT('Ctrl Pts',(-24.4641149028892,1.35184977125648,
12.));
#180240=CARTESIAN_POINT('Ctrl Pts',(-24.4863883275134,1.34378065512337,
12.));
#180241=CARTESIAN_POINT('Ctrl Pts',(-24.5087244363856,1.33562651019686,
12.));
#180242=CARTESIAN_POINT('Ctrl Pts',(-24.5311225731435,1.32738724435326,
12.));
#180243=CARTESIAN_POINT('Ctrl Pts',(-24.5535820868674,1.31906276763668,
12.));
#180244=CARTESIAN_POINT('Ctrl Pts',(-24.5761023320183,1.31065299222021,
12.));
#180245=CARTESIAN_POINT('Ctrl Pts',(-24.5986826684027,1.30215783236362,
12.));
#180246=CARTESIAN_POINT('Ctrl Pts',(-24.6213224611229,1.29357720438107,
12.));
#180247=CARTESIAN_POINT('Ctrl Pts',(-24.6440210805278,1.28491102661514,
12.));
#180248=CARTESIAN_POINT('Ctrl Pts',(-24.666777902156,1.27615921941642,12.));
#180249=CARTESIAN_POINT('Ctrl Pts',(-24.6895923066836,1.267321705135,12.));
#180250=CARTESIAN_POINT('Ctrl Pts',(-24.7124636797894,1.25839840807418,
12.));
#180251=CARTESIAN_POINT('Ctrl Pts',(-24.7353914120011,1.24938925444325,
12.));
#180252=CARTESIAN_POINT('Ctrl Pts',(-24.7583748985438,1.24029417231989,
12.));
#180253=CARTESIAN_POINT('Ctrl Pts',(-24.7814135391799,1.23111309161843,
12.));
#180254=CARTESIAN_POINT('Ctrl Pts',(-24.8045067380536,1.22184594406528,
12.));
#180255=CARTESIAN_POINT('Ctrl Pts',(-24.8276539035092,1.21249266318208,
12.));
#180256=CARTESIAN_POINT('Ctrl Pts',(-24.8508544481974,1.2030531842602,12.));
#180257=CARTESIAN_POINT('Ctrl Pts',(-24.8741077892075,1.19352744434064,
12.));
#180258=CARTESIAN_POINT('Ctrl Pts',(-24.8974133481829,1.18391538220103,
12.));
#180259=CARTESIAN_POINT('Ctrl Pts',(-24.9207705514449,1.17421693835041,
12.));
#180260=CARTESIAN_POINT('Ctrl Pts',(-24.9441788300932,1.16443205502849,
12.));
#180261=CARTESIAN_POINT('Ctrl Pts',(-24.9676376201502,1.15456067621889,
12.));
#180262=CARTESIAN_POINT('Ctrl Pts',(-24.9911463621433,1.144602747582,12.));
#180263=CARTESIAN_POINT('Ctrl Pts',(-25.0147045006196,1.1345582163853,12.));
#180264=CARTESIAN_POINT('Ctrl Pts',(-25.0383114836899,1.12442703144451,
12.));
#180265=CARTESIAN_POINT('Ctrl Pts',(-25.0619667625336,1.11420914306889,
12.));
#180266=CARTESIAN_POINT('Ctrl Pts',(-25.0856697909679,1.10390450301745,
12.));
#180267=CARTESIAN_POINT('Ctrl Pts',(-25.1094200248446,1.09351306445308,
12.));
#180268=CARTESIAN_POINT('Ctrl Pts',(-25.1332169227413,1.08303478197187,
12.));
#180269=CARTESIAN_POINT('Ctrl Pts',(-25.157059946931,1.07246961165475,12.));
#180270=CARTESIAN_POINT('Ctrl Pts',(-25.1809485642192,1.06181751111768,
12.));
#180271=CARTESIAN_POINT('Ctrl Pts',(-25.2048822469028,1.05107843957931,
12.));
#180272=CARTESIAN_POINT('Ctrl Pts',(-25.2288604735086,1.04025235791507,
12.));
#180273=CARTESIAN_POINT('Ctrl Pts',(-25.2528827300422,1.02933922876806,
12.));
#180274=CARTESIAN_POINT('Ctrl Pts',(-25.276948508726,1.01833901642237,12.));
#180275=CARTESIAN_POINT('Ctrl Pts',(-25.3010573055547,1.00725168656896,
12.));
#180276=CARTESIAN_POINT('Ctrl Pts',(-25.3252086182968,0.996077206120624,
12.));
#180277=CARTESIAN_POINT('Ctrl Pts',(-25.3494019441441,0.984815543003973,
12.));
#180278=CARTESIAN_POINT('Ctrl Pts',(-25.3736367778845,0.973466666000163,
12.));
#180279=CARTESIAN_POINT('Ctrl Pts',(-25.3979126089163,0.962030544503142,
12.));
#180280=CARTESIAN_POINT('Ctrl Pts',(-25.4222289223167,0.950507148597468,
12.));
#180281=CARTESIAN_POINT('Ctrl Pts',(-25.4465852044849,0.938896449496192,
12.));
#180282=CARTESIAN_POINT('Ctrl Pts',(-25.4709809475009,0.927198419886094,
12.));
#180283=CARTESIAN_POINT('Ctrl Pts',(-25.4954156541795,0.915413034335613,
12.));
#180284=CARTESIAN_POINT('Ctrl Pts',(-25.5198888424194,0.903540269651106,
12.));
#180285=CARTESIAN_POINT('Ctrl Pts',(-25.5444000508211,0.89158010534904,
12.));
#180286=CARTESIAN_POINT('Ctrl Pts',(-25.5689488408156,0.879532523834294,
12.));
#180287=CARTESIAN_POINT('Ctrl Pts',(-25.5935347843585,0.867397509338431,
12.));
#180288=CARTESIAN_POINT('Ctrl Pts',(-25.6181574536049,0.855175047036549,
12.));
#180289=CARTESIAN_POINT('Ctrl Pts',(-25.6428164100055,0.842865122120758,
12.));
#180290=CARTESIAN_POINT('Ctrl Pts',(-25.6675111931952,0.830467718864205,
12.));
#180291=CARTESIAN_POINT('Ctrl Pts',(-25.6922413110194,0.817982819787464,
12.));
#180292=CARTESIAN_POINT('Ctrl Pts',(-25.7170062262525,0.805410404554352,
12.));
#180293=CARTESIAN_POINT('Ctrl Pts',(-25.7418053757746,0.792750451616127,
12.));
#180294=CARTESIAN_POINT('Ctrl Pts',(-25.7666381946955,0.780002940291965,
12.));
#180295=CARTESIAN_POINT('Ctrl Pts',(-25.7915041383376,0.767167852651168,
12.));
#180296=CARTESIAN_POINT('Ctrl Pts',(-25.8164027059984,0.754245175609524,
12.));
#180297=CARTESIAN_POINT('Ctrl Pts',(-25.8413334619055,0.741234902663807,
12.));
#180298=CARTESIAN_POINT('Ctrl Pts',(-25.8662960624185,0.728137036482335,
12.));
#180299=CARTESIAN_POINT('Ctrl Pts',(-25.891290261497,0.714951588527638,
12.));
#180300=CARTESIAN_POINT('Ctrl Pts',(-25.9163158909426,0.701678575228756,
12.));
#180301=CARTESIAN_POINT('Ctrl Pts',(-25.9413728471909,0.688318015057729,
12.));
#180302=CARTESIAN_POINT('Ctrl Pts',(-25.9614434297919,0.677559543209725,
12.));
#180303=CARTESIAN_POINT('Ctrl Pts',(-25.9765104298071,0.669451306780825,
12.));
#180304=CARTESIAN_POINT('Ctrl Pts',(-25.9865613464773,0.664028313187627,
12.));
#180305=CARTESIAN_POINT('Ctrl Pts',(-25.991588367311,0.661312440730901,
12.));
#180306=CARTESIAN_POINT('',(-25.991588367311,-0.661312440730891,12.));
#180307=CARTESIAN_POINT('Origin',(0.,0.,12.));
#180308=CARTESIAN_POINT('',(-22.4835757167854,-1.76341220531179,12.));
#180309=CARTESIAN_POINT('Ctrl Pts',(-25.991588367311,-0.661312440730891,
12.));
#180310=CARTESIAN_POINT('Ctrl Pts',(-25.9865613464809,-0.664028313188912,
12.));
#180311=CARTESIAN_POINT('Ctrl Pts',(-25.9765104298171,-0.669451306784415,
12.));
#180312=CARTESIAN_POINT('Ctrl Pts',(-25.9614434298092,-0.677559543215902,
12.));
#180313=CARTESIAN_POINT('Ctrl Pts',(-25.941372847213,-0.688318015065678,
12.));
#180314=CARTESIAN_POINT('Ctrl Pts',(-25.9163158909645,-0.701678575236602,
12.));
#180315=CARTESIAN_POINT('Ctrl Pts',(-25.8912902615141,-0.714951588533753,
12.));
#180316=CARTESIAN_POINT('Ctrl Pts',(-25.8662960624285,-0.728137036485877,
12.));
#180317=CARTESIAN_POINT('Ctrl Pts',(-25.841333461908,-0.741234902664697,
12.));
#180318=CARTESIAN_POINT('Ctrl Pts',(-25.816402705995,-0.754245175608288,
12.));
#180319=CARTESIAN_POINT('Ctrl Pts',(-25.7915041383304,-0.767167852648639,
12.));
#180320=CARTESIAN_POINT('Ctrl Pts',(-25.7666381946871,-0.780002940289025,
12.));
#180321=CARTESIAN_POINT('Ctrl Pts',(-25.7418053757671,-0.792750451613534,
12.));
#180322=CARTESIAN_POINT('Ctrl Pts',(-25.7170062262474,-0.805410404552594,
12.));
#180323=CARTESIAN_POINT('Ctrl Pts',(-25.6922413110172,-0.817982819786719,
12.));
#180324=CARTESIAN_POINT('Ctrl Pts',(-25.6675111931957,-0.830467718864367,
12.));
#180325=CARTESIAN_POINT('Ctrl Pts',(-25.6428164100078,-0.842865122121544,
12.));
#180326=CARTESIAN_POINT('Ctrl Pts',(-25.618157453608,-0.855175047037614,
12.));
#180327=CARTESIAN_POINT('Ctrl Pts',(-25.5935347843616,-0.86739750933947,
12.));
#180328=CARTESIAN_POINT('Ctrl Pts',(-25.568948840818,-0.87953252383509,
12.));
#180329=CARTESIAN_POINT('Ctrl Pts',(-25.5444000508223,-0.891580105349467,
12.));
#180330=CARTESIAN_POINT('Ctrl Pts',(-25.5198888424195,-0.903540269651154,
12.));
#180331=CARTESIAN_POINT('Ctrl Pts',(-25.4954156541787,-0.915413034335333,
12.));
#180332=CARTESIAN_POINT('Ctrl Pts',(-25.4709809474996,-0.927198419885604,
12.));
#180333=CARTESIAN_POINT('Ctrl Pts',(-25.4465852044835,-0.938896449495632,
12.));
#180334=CARTESIAN_POINT('Ctrl Pts',(-25.4222289223155,-0.950507148596968,
12.));
#180335=CARTESIAN_POINT('Ctrl Pts',(-25.3979126089155,-0.962030544502802,
12.));
#180336=CARTESIAN_POINT('Ctrl Pts',(-25.3736367778842,-0.973466666000048,
12.));
#180337=CARTESIAN_POINT('Ctrl Pts',(-25.3494019441444,-0.984815543004089,
12.));
#180338=CARTESIAN_POINT('Ctrl Pts',(-25.3252086182976,-0.996077206120919,
12.));
#180339=CARTESIAN_POINT('Ctrl Pts',(-25.3010573055557,-1.00725168656933,
12.));
#180340=CARTESIAN_POINT('Ctrl Pts',(-25.2769485087268,-1.01833901642272,
12.));
#180341=CARTESIAN_POINT('Ctrl Pts',(-25.2528827300427,-1.0293392287683,
12.));
#180342=CARTESIAN_POINT('Ctrl Pts',(-25.2288604735087,-1.04025235791515,
12.));
#180343=CARTESIAN_POINT('Ctrl Pts',(-25.2048822469027,-1.05107843957925,
12.));
#180344=CARTESIAN_POINT('Ctrl Pts',(-25.1809485642191,-1.06181751111754,
12.));
#180345=CARTESIAN_POINT('Ctrl Pts',(-25.1570599469311,-1.0724696116546,
12.));
#180346=CARTESIAN_POINT('Ctrl Pts',(-25.1332169227415,-1.08303478197174,
12.));
#180347=CARTESIAN_POINT('Ctrl Pts',(-25.1094200248448,-1.09351306445299,
12.));
#180348=CARTESIAN_POINT('Ctrl Pts',(-25.085669790968,-1.1039045030174,12.));
#180349=CARTESIAN_POINT('Ctrl Pts',(-25.0619667625336,-1.1142091430689,
12.));
#180350=CARTESIAN_POINT('Ctrl Pts',(-25.0383114836898,-1.12442703144455,
12.));
#180351=CARTESIAN_POINT('Ctrl Pts',(-25.0147045006193,-1.13455821638535,
12.));
#180352=CARTESIAN_POINT('Ctrl Pts',(-24.9911463621431,-1.14460274758206,
12.));
#180353=CARTESIAN_POINT('Ctrl Pts',(-24.9676376201501,-1.15456067621894,
12.));
#180354=CARTESIAN_POINT('Ctrl Pts',(-24.9441788300932,-1.16443205502852,
12.));
#180355=CARTESIAN_POINT('Ctrl Pts',(-24.9207705514449,-1.17421693835039,
12.));
#180356=CARTESIAN_POINT('Ctrl Pts',(-24.8974133481829,-1.18391538220098,
12.));
#180357=CARTESIAN_POINT('Ctrl Pts',(-24.8741077892074,-1.19352744434059,
12.));
#180358=CARTESIAN_POINT('Ctrl Pts',(-24.8508544481973,-1.20305318426015,
12.));
#180359=CARTESIAN_POINT('Ctrl Pts',(-24.8276539035092,-1.21249266318205,
12.));
#180360=CARTESIAN_POINT('Ctrl Pts',(-24.8045067380536,-1.22184594406526,
12.));
#180361=CARTESIAN_POINT('Ctrl Pts',(-24.78141353918,-1.23111309161843,12.));
#180362=CARTESIAN_POINT('Ctrl Pts',(-24.7583748985439,-1.24029417231988,
12.));
#180363=CARTESIAN_POINT('Ctrl Pts',(-24.7353914120012,-1.24938925444323,
12.));
#180364=CARTESIAN_POINT('Ctrl Pts',(-24.7124636797895,-1.25839840807415,
12.));
#180365=CARTESIAN_POINT('Ctrl Pts',(-24.6895923066837,-1.26732170513497,
12.));
#180366=CARTESIAN_POINT('Ctrl Pts',(-24.666777902156,-1.2761592194164,12.));
#180367=CARTESIAN_POINT('Ctrl Pts',(-24.6440210805278,-1.28491102661513,
12.));
#180368=CARTESIAN_POINT('Ctrl Pts',(-24.6213224611228,-1.29357720438107,
12.));
#180369=CARTESIAN_POINT('Ctrl Pts',(-24.5986826684025,-1.30215783236364,
12.));
#180370=CARTESIAN_POINT('Ctrl Pts',(-24.576102332018,-1.31065299222023,
12.));
#180371=CARTESIAN_POINT('Ctrl Pts',(-24.5535820868671,-1.31906276763669,
12.));
#180372=CARTESIAN_POINT('Ctrl Pts',(-24.5311225731434,-1.32738724435326,
12.));
#180373=CARTESIAN_POINT('Ctrl Pts',(-24.5087244363856,-1.33562651019684,
12.));
#180374=CARTESIAN_POINT('Ctrl Pts',(-24.4863883275135,-1.34378065512335,
12.));
#180375=CARTESIAN_POINT('Ctrl Pts',(-24.4641149028894,-1.35184977125644,
12.));
#180376=CARTESIAN_POINT('Ctrl Pts',(-24.4419048244524,-1.35983395290624,
12.));
#180377=CARTESIAN_POINT('Ctrl Pts',(-24.4197587598337,-1.36773329659954,
12.));
#180378=CARTESIAN_POINT('Ctrl Pts',(-24.3976773824731,-1.37554790111607,
12.));
#180379=CARTESIAN_POINT('Ctrl Pts',(-24.37566137173,-1.38327786752998,12.));
#180380=CARTESIAN_POINT('Ctrl Pts',(-24.3537114129877,-1.3909232992639,
12.));
#180381=CARTESIAN_POINT('Ctrl Pts',(-24.3318281977647,-1.3984843021281,
12.));
#180382=CARTESIAN_POINT('Ctrl Pts',(-24.3100124238316,-1.4059609843434,
12.));
#180383=CARTESIAN_POINT('Ctrl Pts',(-24.2882647953214,-1.41335345657685,
12.));
#180384=CARTESIAN_POINT('Ctrl Pts',(-24.2665860228357,-1.42066183198252,
12.));
#180385=CARTESIAN_POINT('Ctrl Pts',(-24.2449768235485,-1.42788622624851,
12.));
#180386=CARTESIAN_POINT('Ctrl Pts',(-24.2234379212978,-1.43502675765502,
12.));
#180387=CARTESIAN_POINT('Ctrl Pts',(-24.2019700467214,-1.44208354711074,
12.));
#180388=CARTESIAN_POINT('Ctrl Pts',(-24.1805739374033,-1.44905671818721,
12.));
#180389=CARTESIAN_POINT('Ctrl Pts',(-24.1592503380105,-1.45594639716314,
12.));
#180390=CARTESIAN_POINT('Ctrl Pts',(-24.1380000004272,-1.46275271307398,
12.));
#180391=CARTESIAN_POINT('Ctrl Pts',(-24.1168236838827,-1.46947579776992,
12.));
#180392=CARTESIAN_POINT('Ctrl Pts',(-24.0957221550782,-1.47611578597741,
12.));
#180393=CARTESIAN_POINT('Ctrl Pts',(-24.074696188353,-1.4826728153368,12.));
#180394=CARTESIAN_POINT('Ctrl Pts',(-24.053746565843,-1.48914702644883,
12.));
#180395=CARTESIAN_POINT('Ctrl Pts',(-24.0328740776331,-1.49553856292798,
12.));
#180396=CARTESIAN_POINT('Ctrl Pts',(-24.0120795219086,-1.50184757146099,
12.));
#180397=CARTESIAN_POINT('Ctrl Pts',(-23.991363705093,-1.50807420187702,
12.));
#180398=CARTESIAN_POINT('Ctrl Pts',(-23.9707274420145,-1.51421860720628,
12.));
#180399=CARTESIAN_POINT('Ctrl Pts',(-23.9501715561038,-1.52028094372806,
12.));
#180400=CARTESIAN_POINT('Ctrl Pts',(-23.9296968795761,-1.52626137103039,
12.));
#180401=CARTESIAN_POINT('Ctrl Pts',(-23.9093042536119,-1.53216005207462,
12.));
#180402=CARTESIAN_POINT('Ctrl Pts',(-23.8889945285313,-1.53797715326748,
12.));
#180403=CARTESIAN_POINT('Ctrl Pts',(-23.8687685639635,-1.54371284453978,
12.));
#180404=CARTESIAN_POINT('Ctrl Pts',(-23.8486272290698,-1.5493672994053,
12.));
#180405=CARTESIAN_POINT('Ctrl Pts',(-23.8285714027631,-1.55494069502628,
12.));
#180406=CARTESIAN_POINT('Ctrl Pts',(-23.8086019739192,-1.56043321228631,
12.));
#180407=CARTESIAN_POINT('Ctrl Pts',(-23.788719841588,-1.56584503586844,
12.));
#180408=CARTESIAN_POINT('Ctrl Pts',(-23.7689259151869,-1.57117635434412,
12.));
#180409=CARTESIAN_POINT('Ctrl Pts',(-23.7492211147369,-1.57642736025251,
12.));
#180410=CARTESIAN_POINT('Ctrl Pts',(-23.7296063711308,-1.58159825017362,
12.));
#180411=CARTESIAN_POINT('Ctrl Pts',(-23.7100826263835,-1.58668922481222,
12.));
#180412=CARTESIAN_POINT('Ctrl Pts',(-23.6906508338833,-1.59170048908631,
12.));
#180413=CARTESIAN_POINT('Ctrl Pts',(-23.6713119586302,-1.59663225222458,
12.));
#180414=CARTESIAN_POINT('Ctrl Pts',(-23.6520669774863,-1.60148472786588,
12.));
#180415=CARTESIAN_POINT('Ctrl Pts',(-23.6329168794916,-1.60625813414666,
12.));
#180416=CARTESIAN_POINT('Ctrl Pts',(-23.6138626661644,-1.61095269379773,
12.));
#180417=CARTESIAN_POINT('Ctrl Pts',(-23.5949053517996,-1.61556863424697,
12.));
#180418=CARTESIAN_POINT('Ctrl Pts',(-23.5760459637608,-1.62010618772869,
12.));
#180419=CARTESIAN_POINT('Ctrl Pts',(-23.5572855427617,-1.62456559140072,
12.));
#180420=CARTESIAN_POINT('Ctrl Pts',(-23.5386251432278,-1.62894708745231,
12.));
#180421=CARTESIAN_POINT('Ctrl Pts',(-23.5200658336624,-1.63325092321731,
12.));
#180422=CARTESIAN_POINT('Ctrl Pts',(-23.5016086970006,-1.63747735129474,
12.));
#180423=CARTESIAN_POINT('Ctrl Pts',(-23.4832548309638,-1.64162662967524,
12.));
#180424=CARTESIAN_POINT('Ctrl Pts',(-23.4650053483919,-1.64569902187608,
12.));
#180425=CARTESIAN_POINT('Ctrl Pts',(-23.446861377656,-1.64969479707339,
12.));
#180426=CARTESIAN_POINT('Ctrl Pts',(-23.4288240631034,-1.6536142302373,
12.));
#180427=CARTESIAN_POINT('Ctrl Pts',(-23.4108945654803,-1.65745760227507,
12.));
#180428=CARTESIAN_POINT('Ctrl Pts',(-23.3930740623622,-1.66122520018008,
12.));
#180429=CARTESIAN_POINT('Ctrl Pts',(-23.375363748555,-1.66491731718864,
12.));
#180430=CARTESIAN_POINT('Ctrl Pts',(-23.3577648365747,-1.66853425293977,
12.));
#180431=CARTESIAN_POINT('Ctrl Pts',(-23.3402785571866,-1.67207631363905,
12.));
#180432=CARTESIAN_POINT('Ctrl Pts',(-23.3229061599145,-1.67554381222987,
12.));
#180433=CARTESIAN_POINT('Ctrl Pts',(-23.3056489135611,-1.67893706857123,
12.));
#180434=CARTESIAN_POINT('Ctrl Pts',(-23.2885081066949,-1.68225640962181,
12.));
#180435=CARTESIAN_POINT('Ctrl Pts',(-23.2714850482245,-1.68550216963275,
12.));
#180436=CARTESIAN_POINT('Ctrl Pts',(-23.2545810680536,-1.6886746903491,
12.));
#180437=CARTESIAN_POINT('Ctrl Pts',(-23.2377975177014,-1.69177432121716,
12.));
#180438=CARTESIAN_POINT('Ctrl Pts',(-23.2211357709374,-1.69480141959945,
12.));
#180439=CARTESIAN_POINT('Ctrl Pts',(-23.2045972243765,-1.69775635099425,
12.));
#180440=CARTESIAN_POINT('Ctrl Pts',(-23.1881832981848,-1.70063948926987,
12.));
#180441=CARTESIAN_POINT('Ctrl Pts',(-23.1718954368749,-1.70345121691259,
12.));
#180442=CARTESIAN_POINT('Ctrl Pts',(-23.1557351100613,-1.70619192527847,
12.));
#180443=CARTESIAN_POINT('Ctrl Pts',(-23.1397038132358,-1.7088620148546,
12.));
#180444=CARTESIAN_POINT('Ctrl Pts',(-23.1238030684929,-1.71146189552192,
12.));
#180445=CARTESIAN_POINT('Ctrl Pts',(-23.1080344254291,-1.71399198684724,
12.));
#180446=CARTESIAN_POINT('Ctrl Pts',(-23.0923994621216,-1.71645271839311,
12.));
#180447=CARTESIAN_POINT('Ctrl Pts',(-23.0768997860709,-1.71884453003027,
12.));
#180448=CARTESIAN_POINT('Ctrl Pts',(-23.061537035156,-1.7211678722598,12.));
#180449=CARTESIAN_POINT('Ctrl Pts',(-23.0463128785528,-1.72342320653731,
12.));
#180450=CARTESIAN_POINT('Ctrl Pts',(-23.031229017888,-1.72561100564033,
12.));
#180451=CARTESIAN_POINT('Ctrl Pts',(-23.0162871884167,-1.72773175404702,
12.));
#180452=CARTESIAN_POINT('Ctrl Pts',(-23.0014891601891,-1.72978594832137,
12.));
#180453=CARTESIAN_POINT('Ctrl Pts',(-22.9868367391978,-1.73177409750193,
12.));
#180454=CARTESIAN_POINT('Ctrl Pts',(-22.9723317685688,-1.73369672350817,
12.));
#180455=CARTESIAN_POINT('Ctrl Pts',(-22.9579761301062,-1.73555436162771,
12.));
#180456=CARTESIAN_POINT('Ctrl Pts',(-22.9437717457825,-1.73734756100038,
12.));
#180457=CARTESIAN_POINT('Ctrl Pts',(-22.9297205792587,-1.73907688511664,
12.));
#180458=CARTESIAN_POINT('Ctrl Pts',(-22.9158246373365,-1.74074291231057,
12.));
#180459=CARTESIAN_POINT('Ctrl Pts',(-22.9020859716144,-1.74234623630079,
12.));
#180460=CARTESIAN_POINT('Ctrl Pts',(-22.8885066803351,-1.74388746677702,
12.));
#180461=CARTESIAN_POINT('Ctrl Pts',(-22.8750889101696,-1.745367229982,12.));
#180462=CARTESIAN_POINT('Ctrl Pts',(-22.8618348580234,-1.74678616930663,
12.));
#180463=CARTESIAN_POINT('Ctrl Pts',(-22.8487467728075,-1.74814494588492,
12.));
#180464=CARTESIAN_POINT('Ctrl Pts',(-22.8358269579854,-1.74944423940117,
12.));
#180465=CARTESIAN_POINT('Ctrl Pts',(-22.8230777741285,-1.75068474890884,
12.));
#180466=CARTESIAN_POINT('Ctrl Pts',(-22.8105016414712,-1.75186719365589,
12.));
#180467=CARTESIAN_POINT('Ctrl Pts',(-22.7981010424312,-1.75299231391461,
12.));
#180468=CARTESIAN_POINT('Ctrl Pts',(-22.7858785242358,-1.75406087182929,
12.));
#180469=CARTESIAN_POINT('Ctrl Pts',(-22.7738367016115,-1.75507365227127,
12.));
#180470=CARTESIAN_POINT('Ctrl Pts',(-22.7619782595013,-1.7560314637164,
12.));
#180471=CARTESIAN_POINT('Ctrl Pts',(-22.7503059556455,-1.75693513908911,
12.));
#180472=CARTESIAN_POINT('Ctrl Pts',(-22.7388226235565,-1.75778553673249,
12.));
#180473=CARTESIAN_POINT('Ctrl Pts',(-22.7275311777305,-1.75858354204635,
12.));
#180474=CARTESIAN_POINT('Ctrl Pts',(-22.7164346186007,-1.75933006905924,
12.));
#180475=CARTESIAN_POINT('Ctrl Pts',(-22.7055360375481,-1.76002606202399,
12.));
#180476=CARTESIAN_POINT('Ctrl Pts',(-22.6948386219843,-1.76067249704884,
12.));
#180477=CARTESIAN_POINT('Ctrl Pts',(-22.6843456585245,-1.76127038310612,
12.));
#180478=CARTESIAN_POINT('Ctrl Pts',(-22.6740605356699,-1.76182076289525,
12.));
#180479=CARTESIAN_POINT('Ctrl Pts',(-22.6639867471756,-1.76232471392567,
12.));
#180480=CARTESIAN_POINT('Ctrl Pts',(-22.6541278938413,-1.76278334912559,
12.));
#180481=CARTESIAN_POINT('Ctrl Pts',(-22.6444876940425,-1.76319782013914,
12.));
#180482=CARTESIAN_POINT('Ctrl Pts',(-22.635069997936,-1.76356932176272,
12.));
#180483=CARTESIAN_POINT('Ctrl Pts',(-22.6258787994847,-1.76389909571402,
12.));
#180484=CARTESIAN_POINT('Ctrl Pts',(-22.6169182517693,-1.76418843543739,
12.));
#180485=CARTESIAN_POINT('Ctrl Pts',(-22.6081926681342,-1.76443868648015,
12.));
#180486=CARTESIAN_POINT('Ctrl Pts',(-22.5997065145638,-1.76465124413556,
12.));
#180487=CARTESIAN_POINT('Ctrl Pts',(-22.5914644078106,-1.76482755288411,
12.));
#180488=CARTESIAN_POINT('Ctrl Pts',(-22.5834711038024,-1.76496910283088,
12.));
#180489=CARTESIAN_POINT('Ctrl Pts',(-22.5757315316355,-1.76507744026747,
12.));
#180490=CARTESIAN_POINT('Ctrl Pts',(-22.5682508499873,-1.76515418518829,
12.));
#180491=CARTESIAN_POINT('Ctrl Pts',(-22.5610344912501,-1.76520104500449,
12.));
#180492=CARTESIAN_POINT('Ctrl Pts',(-22.5540882235837,-1.76521983384063,
12.));
#180493=CARTESIAN_POINT('Ctrl Pts',(-22.5474180954006,-1.76521245524047,
12.));
#180494=CARTESIAN_POINT('Ctrl Pts',(-22.5410303590891,-1.76518087841492,
12.));
#180495=CARTESIAN_POINT('Ctrl Pts',(-22.5349313983571,-1.7651271156325,
12.));
#180496=CARTESIAN_POINT('Ctrl Pts',(-22.529127665298,-1.76505320262751,
12.));
#180497=CARTESIAN_POINT('Ctrl Pts',(-22.5236259635515,-1.76496128643369,
12.));
#180498=CARTESIAN_POINT('Ctrl Pts',(-22.5184336670207,-1.76485369319896,
12.));
#180499=CARTESIAN_POINT('Ctrl Pts',(-22.5135590569554,-1.76473303281159,
12.));
#180500=CARTESIAN_POINT('Ctrl Pts',(-22.5090112700212,-1.76460218257323,
12.));
#180501=CARTESIAN_POINT('Ctrl Pts',(-22.5047996391978,-1.76446408210366,
12.));
#180502=CARTESIAN_POINT('Ctrl Pts',(-22.5009332677316,-1.76432160068725,
12.));
#180503=CARTESIAN_POINT('Ctrl Pts',(-22.4974203063191,-1.76417731243462,
12.));
#180504=CARTESIAN_POINT('Ctrl Pts',(-22.4942693792449,-1.764033938803,12.));
#180505=CARTESIAN_POINT('Ctrl Pts',(-22.4914909094908,-1.76389475965724,
12.));
#180506=CARTESIAN_POINT('Ctrl Pts',(-22.4890991659478,-1.76376424879505,
12.));
#180507=CARTESIAN_POINT('Ctrl Pts',(-22.4871115206571,-1.76364784232963,
12.));
#180508=CARTESIAN_POINT('Ctrl Pts',(-22.4855446605991,-1.76355076045546,
12.));
#180509=CARTESIAN_POINT('Ctrl Pts',(-22.4844112933129,-1.76347698284792,
12.));
#180510=CARTESIAN_POINT('Ctrl Pts',(-22.483856251707,-1.76343813434565,
12.));
#180511=CARTESIAN_POINT('Ctrl Pts',(-22.4836387052232,-1.7634206426357,
12.));
#180512=CARTESIAN_POINT('Ctrl Pts',(-22.483581992979,-1.76341415538764,
12.));
#180513=CARTESIAN_POINT('Ctrl Pts',(-22.4835757167854,-1.76341220531179,
12.));
#180514=CARTESIAN_POINT('',(-21.9269795755927,-1.71975774210841,12.));
#180515=CARTESIAN_POINT('',(-10.7170877657712,-0.840553282521227,12.));
#180516=CARTESIAN_POINT('',(-21.3904321633055,-2.16781269186828,12.));
#180517=CARTESIAN_POINT('Origin',(-21.8878840740801,-2.21822694051637,12.));
#180518=CARTESIAN_POINT('',(-21.2226420728916,-3.44230496120418,12.));
#180519=CARTESIAN_POINT('Origin',(-7.7715611723761E-13,-7.16093850883225E-14,
12.));
#180520=CARTESIAN_POINT('',(-21.624941921198,-4.01396149767428,12.));
#180521=CARTESIAN_POINT('Origin',(-21.7161918885403,-3.52235856495312,12.));
#180522=CARTESIAN_POINT('',(-22.1738711152697,-4.11585220600461,12.));
#180523=CARTESIAN_POINT('',(-11.0869355576349,-2.05792610300232,12.));
#180524=CARTESIAN_POINT('',(-25.2771067246846,-6.08833931617698,12.));
#180525=CARTESIAN_POINT('Ctrl Pts',(-22.1738711152697,-4.11585220600461,
12.));
#180526=CARTESIAN_POINT('Ctrl Pts',(-22.1738776823239,-4.11585194677412,
12.));
#180527=CARTESIAN_POINT('Ctrl Pts',(-22.1739341411684,-4.1158603587821,
12.));
#180528=CARTESIAN_POINT('Ctrl Pts',(-22.174148802123,-4.11589976826061,
12.));
#180529=CARTESIAN_POINT('Ctrl Pts',(-22.1746949858773,-4.11600589882767,
12.));
#180530=CARTESIAN_POINT('Ctrl Pts',(-22.1758088296598,-4.11622797217066,
12.));
#180531=CARTESIAN_POINT('Ctrl Pts',(-22.177347426894,-4.11653973150558,
12.));
#180532=CARTESIAN_POINT('Ctrl Pts',(-22.179297473024,-4.11694173195041,
12.));
#180533=CARTESIAN_POINT('Ctrl Pts',(-22.1816414985788,-4.11743469691765,
12.));
#180534=CARTESIAN_POINT('Ctrl Pts',(-22.1843613164855,-4.11801938107464,
12.));
#180535=CARTESIAN_POINT('Ctrl Pts',(-22.1874419861496,-4.11869641271752,
12.));
#180536=CARTESIAN_POINT('Ctrl Pts',(-22.1908725908525,-4.11946626228623,
12.));
#180537=CARTESIAN_POINT('Ctrl Pts',(-22.1946440958098,-4.12032932637738,
12.));
#180538=CARTESIAN_POINT('Ctrl Pts',(-22.1987479618246,-4.12128598183533,
12.));
#180539=CARTESIAN_POINT('Ctrl Pts',(-22.2031746532106,-4.12233664408237,
12.));
#180540=CARTESIAN_POINT('Ctrl Pts',(-22.2079143941719,-4.12348173702024,
12.));
#180541=CARTESIAN_POINT('Ctrl Pts',(-22.2129576146671,-4.12472167516602,
12.));
#180542=CARTESIAN_POINT('Ctrl Pts',(-22.2182956401341,-4.126056836133,12.));
#180543=CARTESIAN_POINT('Ctrl Pts',(-22.2239207458781,-4.12748755830099,
12.));
#180544=CARTESIAN_POINT('Ctrl Pts',(-22.2298258043947,-4.12901415463379,
12.));
#180545=CARTESIAN_POINT('Ctrl Pts',(-22.2360040565534,-4.13063692157499,
12.));
#180546=CARTESIAN_POINT('Ctrl Pts',(-22.2424488153523,-4.1323561506016,
12.));
#180547=CARTESIAN_POINT('Ctrl Pts',(-22.2491535317789,-4.13417212558808,
12.));
#180548=CARTESIAN_POINT('Ctrl Pts',(-22.2561118708422,-4.13608511977226,
12.));
#180549=CARTESIAN_POINT('Ctrl Pts',(-22.263317791397,-4.13809539255418,
12.));
#180550=CARTESIAN_POINT('Ctrl Pts',(-22.2707656042456,-4.14020318715988,
12.));
#180551=CARTESIAN_POINT('Ctrl Pts',(-22.2784499072026,-4.14240873321982,
12.));
#180552=CARTESIAN_POINT('Ctrl Pts',(-22.2863655389167,-4.14471224859295,
12.));
#180553=CARTESIAN_POINT('Ctrl Pts',(-22.2945075198468,-4.14711394168559,
12.));
#180554=CARTESIAN_POINT('Ctrl Pts',(-22.3028710166935,-4.14961401285525,
12.));
#180555=CARTESIAN_POINT('Ctrl Pts',(-22.3114513545186,-4.15221265396993,
12.));
#180556=CARTESIAN_POINT('Ctrl Pts',(-22.3202440186979,-4.15491004835278,
12.));
#180557=CARTESIAN_POINT('Ctrl Pts',(-22.3292446628957,-4.15770637047882,
12.));
#180558=CARTESIAN_POINT('Ctrl Pts',(-22.3384491078599,-4.16060178604154,
12.));
#180559=CARTESIAN_POINT('Ctrl Pts',(-22.3478533253886,-4.1635964526318,
12.));
#180560=CARTESIAN_POINT('Ctrl Pts',(-22.3574534257397,-4.16669052026602,
12.));
#180561=CARTESIAN_POINT('Ctrl Pts',(-22.3672456427605,-4.16988413199469,
12.));
#180562=CARTESIAN_POINT('Ctrl Pts',(-22.3772263228624,-4.17317742436162,
12.));
#180563=CARTESIAN_POINT('Ctrl Pts',(-22.3873919231339,-4.17657052752834,
12.));
#180564=CARTESIAN_POINT('Ctrl Pts',(-22.3977390078074,-4.18006356544879,
12.));
#180565=CARTESIAN_POINT('Ctrl Pts',(-22.4082642454448,-4.18365665600839,
12.));
#180566=CARTESIAN_POINT('Ctrl Pts',(-22.4189644056109,-4.18734991117707,
12.));
#180567=CARTESIAN_POINT('Ctrl Pts',(-22.4298363535416,-4.19114343726932,
12.));
#180568=CARTESIAN_POINT('Ctrl Pts',(-22.4408770448917,-4.1950373351886,
12.));
#180569=CARTESIAN_POINT('Ctrl Pts',(-22.4520835205422,-4.19903170066358,
12.));
#180570=CARTESIAN_POINT('Ctrl Pts',(-22.4634529011437,-4.20312662448174,
12.));
#180571=CARTESIAN_POINT('Ctrl Pts',(-22.4749823839917,-4.20732219265649,
12.));
#180572=CARTESIAN_POINT('Ctrl Pts',(-22.4866692403147,-4.21161848657428,
12.));
#180573=CARTESIAN_POINT('Ctrl Pts',(-22.4985108124228,-4.21601558313906,
12.));
#180574=CARTESIAN_POINT('Ctrl Pts',(-22.5105045108881,-4.22051355490196,
12.));
#180575=CARTESIAN_POINT('Ctrl Pts',(-22.5226478117886,-4.22511247020041,
12.));
#180576=CARTESIAN_POINT('Ctrl Pts',(-22.5349382540588,-4.22981239330733,
12.));
#180577=CARTESIAN_POINT('Ctrl Pts',(-22.5473734368086,-4.23461338456712,
12.));
#180578=CARTESIAN_POINT('Ctrl Pts',(-22.5599510166429,-4.23951550052522,
12.));
#180579=CARTESIAN_POINT('Ctrl Pts',(-22.572668704992,-4.24451879404851,
12.));
#180580=CARTESIAN_POINT('Ctrl Pts',(-22.5855242662477,-4.24962331444177,
12.));
#180581=CARTESIAN_POINT('Ctrl Pts',(-22.5985155158636,-4.25482910755481,
12.));
#180582=CARTESIAN_POINT('Ctrl Pts',(-22.6116403184821,-4.26013621588305,
12.));
#180583=CARTESIAN_POINT('Ctrl Pts',(-22.6248965859977,-4.26554467865576,
12.));
#180584=CARTESIAN_POINT('Ctrl Pts',(-22.6382822758172,-4.27105453193004,
12.));
#180585=CARTESIAN_POINT('Ctrl Pts',(-22.6517953893303,-4.2766658086912,
12.));
#180586=CARTESIAN_POINT('Ctrl Pts',(-22.6654339703109,-4.28237853894059,
12.));
#180587=CARTESIAN_POINT('Ctrl Pts',(-22.6791961033538,-4.28819274977763,
12.));
#180588=CARTESIAN_POINT('Ctrl Pts',(-22.6930799122548,-4.29410846547056,
12.));
#180589=CARTESIAN_POINT('Ctrl Pts',(-22.7070835587564,-4.3001257075406,
12.));
#180590=CARTESIAN_POINT('Ctrl Pts',(-22.7212052413386,-4.30624449484069,
12.));
#180591=CARTESIAN_POINT('Ctrl Pts',(-22.7354431939926,-4.31246484362549,
12.));
#180592=CARTESIAN_POINT('Ctrl Pts',(-22.7497956849848,-4.31878676761235,
12.));
#180593=CARTESIAN_POINT('Ctrl Pts',(-22.7642610156475,-4.32521027803754,
12.));
#180594=CARTESIAN_POINT('Ctrl Pts',(-22.7788375194076,-4.3317353837319,
12.));
#180595=CARTESIAN_POINT('Ctrl Pts',(-22.7935235607806,-4.33836209118446,
12.));
#180596=CARTESIAN_POINT('Ctrl Pts',(-22.8083175343791,-4.34509040460062,
12.));
#180597=CARTESIAN_POINT('Ctrl Pts',(-22.8232178638876,-4.35192032594791,
12.));
#180598=CARTESIAN_POINT('Ctrl Pts',(-22.8382230011184,-4.35885185500546,
12.));
#180599=CARTESIAN_POINT('Ctrl Pts',(-22.8533314252422,-4.36588498942997,
12.));
#180600=CARTESIAN_POINT('Ctrl Pts',(-22.8685416419725,-4.37301972480745,
12.));
#180601=CARTESIAN_POINT('Ctrl Pts',(-22.8838521827701,-4.38025605470093,
12.));
#180602=CARTESIAN_POINT('Ctrl Pts',(-22.8992616040108,-4.38759397068406,
12.));
#180603=CARTESIAN_POINT('Ctrl Pts',(-22.9147684862426,-4.39503346238473,
12.));
#180604=CARTESIAN_POINT('Ctrl Pts',(-22.930371433555,-4.40257451754323,
12.));
#180605=CARTESIAN_POINT('Ctrl Pts',(-22.9460690729093,-4.41021712205553,
12.));
#180606=CARTESIAN_POINT('Ctrl Pts',(-22.9618600534866,-4.41796126001302,
12.));
#180607=CARTESIAN_POINT('Ctrl Pts',(-22.977743046002,-4.42580691372751,
12.));
#180608=CARTESIAN_POINT('Ctrl Pts',(-22.9937167421006,-4.43375406376879,
12.));
#180609=CARTESIAN_POINT('Ctrl Pts',(-23.0097798538395,-4.44180268901643,
12.));
#180610=CARTESIAN_POINT('Ctrl Pts',(-23.0259311131392,-4.44995276669686,
12.));
#180611=CARTESIAN_POINT('Ctrl Pts',(-23.0421692712467,-4.45820427241683,
12.));
#180612=CARTESIAN_POINT('Ctrl Pts',(-23.0584930981732,-4.4665571801823,
12.));
#180613=CARTESIAN_POINT('Ctrl Pts',(-23.0749013821881,-4.47501146242856,
12.));
#180614=CARTESIAN_POINT('Ctrl Pts',(-23.0913929293922,-4.48356709006788,
12.));
#180615=CARTESIAN_POINT('Ctrl Pts',(-23.1079665632636,-4.49222403252216,
12.));
#180616=CARTESIAN_POINT('Ctrl Pts',(-23.1246211242115,-4.50098225775171,
12.));
#180617=CARTESIAN_POINT('Ctrl Pts',(-23.1413554691123,-4.5098417322706,
12.));
#180618=CARTESIAN_POINT('Ctrl Pts',(-23.1581684708761,-4.51880242116748,
12.));
#180619=CARTESIAN_POINT('Ctrl Pts',(-23.1750590180908,-4.52786428815014,
12.));
#180620=CARTESIAN_POINT('Ctrl Pts',(-23.1920260146465,-4.53702729557566,
12.));
#180621=CARTESIAN_POINT('Ctrl Pts',(-23.2090683793629,-4.54629140447544,
12.));
#180622=CARTESIAN_POINT('Ctrl Pts',(-23.2261850456064,-4.55565657456975,
12.));
#180623=CARTESIAN_POINT('Ctrl Pts',(-23.2433749609131,-4.56512276427839,
12.));
#180624=CARTESIAN_POINT('Ctrl Pts',(-23.2606370866866,-4.57468993076097,
12.));
#180625=CARTESIAN_POINT('Ctrl Pts',(-23.2779703978876,-4.5843580299469,
12.));
#180626=CARTESIAN_POINT('Ctrl Pts',(-23.2953738827191,-4.5941270165575,
12.));
#180627=CARTESIAN_POINT('Ctrl Pts',(-23.3128465423115,-4.60399684412163,
12.));
#180628=CARTESIAN_POINT('Ctrl Pts',(-23.3303873903938,-4.6139674649783,
12.));
#180629=CARTESIAN_POINT('Ctrl Pts',(-23.3479954530272,-4.62403883030805,
12.));
#180630=CARTESIAN_POINT('Ctrl Pts',(-23.3656697683489,-4.63421089016541,
12.));
#180631=CARTESIAN_POINT('Ctrl Pts',(-23.3834093863068,-4.6444835934993,
12.));
#180632=CARTESIAN_POINT('Ctrl Pts',(-23.4012133683959,-4.65485688816924,
12.));
#180633=CARTESIAN_POINT('Ctrl Pts',(-23.4190807873803,-4.6653307209467,
12.));
#180634=CARTESIAN_POINT('Ctrl Pts',(-23.4370107270451,-4.67590503753058,
12.));
#180635=CARTESIAN_POINT('Ctrl Pts',(-23.455002281986,-4.68657978258303,
12.));
#180636=CARTESIAN_POINT('Ctrl Pts',(-23.4730545573853,-4.69735489975024,
12.));
#180637=CARTESIAN_POINT('Ctrl Pts',(-23.491166668789,-4.70823033167818,
12.));
#180638=CARTESIAN_POINT('Ctrl Pts',(-23.509337741878,-4.71920602001901,
12.));
#180639=CARTESIAN_POINT('Ctrl Pts',(-23.5275669122372,-4.7302819054303,
12.));
#180640=CARTESIAN_POINT('Ctrl Pts',(-23.545853325171,-4.74145792760698,
12.));
#180641=CARTESIAN_POINT('Ctrl Pts',(-23.5641961355168,-4.75273402530617,
12.));
#180642=CARTESIAN_POINT('Ctrl Pts',(-23.5825945074535,-4.76411013636251,
12.));
#180643=CARTESIAN_POINT('Ctrl Pts',(-23.6010476143099,-4.77558619769872,
12.));
#180644=CARTESIAN_POINT('Ctrl Pts',(-23.6195546383624,-4.78716214532098,
12.));
#180645=CARTESIAN_POINT('Ctrl Pts',(-23.6381147706579,-4.7988379143322,
12.));
#180646=CARTESIAN_POINT('Ctrl Pts',(-23.6567272108628,-4.81061343896432,
12.));
#180647=CARTESIAN_POINT('Ctrl Pts',(-23.675391167102,-4.82248865259562,
12.));
#180648=CARTESIAN_POINT('Ctrl Pts',(-23.6941058557971,-4.83446348776265,
12.));
#180649=CARTESIAN_POINT('Ctrl Pts',(-23.7128705015017,-4.84653787616425,
12.));
#180650=CARTESIAN_POINT('Ctrl Pts',(-23.7316843367313,-4.85871174865499,
12.));
#180651=CARTESIAN_POINT('Ctrl Pts',(-23.7505466018245,-4.87098503527152,
12.));
#180652=CARTESIAN_POINT('Ctrl Pts',(-23.7694565448049,-4.88335766525573,
12.));
#180653=CARTESIAN_POINT('Ctrl Pts',(-23.7884134212384,-4.89582956706775,
12.));
#180654=CARTESIAN_POINT('Ctrl Pts',(-23.8074164940896,-4.90840066839344,
12.));
#180655=CARTESIAN_POINT('Ctrl Pts',(-23.8264650335717,-4.92107089613969,
12.));
#180656=CARTESIAN_POINT('Ctrl Pts',(-23.8455583170057,-4.93384017643432,
12.));
#180657=CARTESIAN_POINT('Ctrl Pts',(-23.8646956287168,-4.9467084346586,
12.));
#180658=CARTESIAN_POINT('Ctrl Pts',(-23.8838762599218,-4.9596755954656,
12.));
#180659=CARTESIAN_POINT('Ctrl Pts',(-23.9030995086163,-4.97274158279226,
12.));
#180660=CARTESIAN_POINT('Ctrl Pts',(-23.9223646794592,-4.98590631986532,
12.));
#180661=CARTESIAN_POINT('Ctrl Pts',(-23.9416710836529,-4.99916972919306,
12.));
#180662=CARTESIAN_POINT('Ctrl Pts',(-23.9610180388271,-5.01253173257453,
12.));
#180663=CARTESIAN_POINT('Ctrl Pts',(-23.9804048689227,-5.02599225112454,
12.));
#180664=CARTESIAN_POINT('Ctrl Pts',(-23.9998309040746,-5.03955120528521,
12.));
#180665=CARTESIAN_POINT('Ctrl Pts',(-24.0192954804896,-5.05320851483065,
12.));
#180666=CARTESIAN_POINT('Ctrl Pts',(-24.0387979403268,-5.06696409886641,
12.));
#180667=CARTESIAN_POINT('Ctrl Pts',(-24.0583376315638,-5.08081787581276,
12.));
#180668=CARTESIAN_POINT('Ctrl Pts',(-24.0779139079266,-5.09476976342625,
12.));
#180669=CARTESIAN_POINT('Ctrl Pts',(-24.0975261288446,-5.10881967883132,
12.));
#180670=CARTESIAN_POINT('Ctrl Pts',(-24.117173659394,-5.12296753853859,
12.));
#180671=CARTESIAN_POINT('Ctrl Pts',(-24.1368558702443,-5.13721325845744,
12.));
#180672=CARTESIAN_POINT('Ctrl Pts',(-24.156572137597,-5.15155675390075,
12.));
#180673=CARTESIAN_POINT('Ctrl Pts',(-24.1763218431343,-5.16599793957979,
12.));
#180674=CARTESIAN_POINT('Ctrl Pts',(-24.1961043738754,-5.18053672961392,
12.));
#180675=CARTESIAN_POINT('Ctrl Pts',(-24.215919122017,-5.19517303753643,
12.));
#180676=CARTESIAN_POINT('Ctrl Pts',(-24.2357654847765,-5.20990677629173,
12.));
#180677=CARTESIAN_POINT('Ctrl Pts',(-24.2556428642294,-5.22473785822441,
12.));
#180678=CARTESIAN_POINT('Ctrl Pts',(-24.2755506671526,-5.23966619506289,
12.));
#180679=CARTESIAN_POINT('Ctrl Pts',(-24.2954883048448,-5.25469169788856,
12.));
#180680=CARTESIAN_POINT('Ctrl Pts',(-24.3154551932222,-5.26981427718796,
12.));
#180681=CARTESIAN_POINT('Ctrl Pts',(-24.3354507529415,-5.28503384290644,
12.));
#180682=CARTESIAN_POINT('Ctrl Pts',(-24.3554744095075,-5.30035030449058,
12.));
#180683=CARTESIAN_POINT('Ctrl Pts',(-24.3755255933917,-5.31576357092524,
12.));
#180684=CARTESIAN_POINT('Ctrl Pts',(-24.3956037401293,-5.33127355076036,
12.));
#180685=CARTESIAN_POINT('Ctrl Pts',(-24.4157082904615,-5.34688015213546,
12.));
#180686=CARTESIAN_POINT('Ctrl Pts',(-24.4358386899152,-5.36258328273639,
12.));
#180687=CARTESIAN_POINT('Ctrl Pts',(-24.4559943883159,-5.37838284973706,
12.));
#180688=CARTESIAN_POINT('Ctrl Pts',(-24.4761748393322,-5.3942787597383,
12.));
#180689=CARTESIAN_POINT('Ctrl Pts',(-24.4963794999831,-5.41027091869242,
12.));
#180690=CARTESIAN_POINT('Ctrl Pts',(-24.5166078302107,-5.42635923183411,
12.));
#180691=CARTESIAN_POINT('Ctrl Pts',(-24.5368592922861,-5.44254360356865,
12.));
#180692=CARTESIAN_POINT('Ctrl Pts',(-24.5571333514841,-5.45882393762244,
12.));
#180693=CARTESIAN_POINT('Ctrl Pts',(-24.5774294770329,-5.47520013724403,
12.));
#180694=CARTESIAN_POINT('Ctrl Pts',(-24.5977471429365,-5.49167210537235,
12.));
#180695=CARTESIAN_POINT('Ctrl Pts',(-24.618085828918,-5.50823974481959,
12.));
#180696=CARTESIAN_POINT('Ctrl Pts',(-24.6384450211466,-5.52490295840996,
12.));
#180697=CARTESIAN_POINT('Ctrl Pts',(-24.6588242134733,-5.54166164919593,
12.));
#180698=CARTESIAN_POINT('Ctrl Pts',(-24.6792229061785,-5.55851572025389,
12.));
#180699=CARTESIAN_POINT('Ctrl Pts',(-24.6996406035507,-5.57546507427766,
12.));
#180700=CARTESIAN_POINT('Ctrl Pts',(-24.7200768119079,-5.59250961323995,
12.));
#180701=CARTESIAN_POINT('Ctrl Pts',(-24.7405310372736,-5.60964923798495,
12.));
#180702=CARTESIAN_POINT('Ctrl Pts',(-24.76100278357,-5.62688384790919,12.));
#180703=CARTESIAN_POINT('Ctrl Pts',(-24.7814915496728,-5.64421334042247,
12.));
#180704=CARTESIAN_POINT('Ctrl Pts',(-24.8019968304618,-5.66163761114903,
12.));
#180705=CARTESIAN_POINT('Ctrl Pts',(-24.822518122386,-5.67915655496524,
12.));
#180706=CARTESIAN_POINT('Ctrl Pts',(-24.8430549277634,-5.69677006679429,
12.));
#180707=CARTESIAN_POINT('Ctrl Pts',(-24.8636067597677,-5.71447804252019,
12.));
#180708=CARTESIAN_POINT('Ctrl Pts',(-24.8841731467219,-5.73228037976926,
12.));
#180709=CARTESIAN_POINT('Ctrl Pts',(-24.9047536376467,-5.75017697890813,
12.));
#180710=CARTESIAN_POINT('Ctrl Pts',(-24.9253478043632,-5.76816774342236,
12.));
#180711=CARTESIAN_POINT('Ctrl Pts',(-24.9459552293308,-5.78625257775703,
12.));
#180712=CARTESIAN_POINT('Ctrl Pts',(-24.9665754954462,-5.80443138549747,
12.));
#180713=CARTESIAN_POINT('Ctrl Pts',(-24.9872081752709,-5.82270406744214,
12.));
#180714=CARTESIAN_POINT('Ctrl Pts',(-25.0078528200558,-5.84107051963073,
12.));
#180715=CARTESIAN_POINT('Ctrl Pts',(-25.0285089498922,-5.8595306315681,
12.));
#180716=CARTESIAN_POINT('Ctrl Pts',(-25.0491760405965,-5.87808428385329,
12.));
#180717=CARTESIAN_POINT('Ctrl Pts',(-25.0698535426593,-5.89673135155459,
12.));
#180718=CARTESIAN_POINT('Ctrl Pts',(-25.0905409050863,-5.91547170844382,
12.));
#180719=CARTESIAN_POINT('Ctrl Pts',(-25.1112375971182,-5.93430523086776,
12.));
#180720=CARTESIAN_POINT('Ctrl Pts',(-25.1319431317273,-5.95323180187348,
12.));
#180721=CARTESIAN_POINT('Ctrl Pts',(-25.1526570863065,-5.97225131495636,
12.));
#180722=CARTESIAN_POINT('Ctrl Pts',(-25.1733791296154,-5.99136367859838,
12.));
#180723=CARTESIAN_POINT('Ctrl Pts',(-25.1941090269638,-6.0105688180476,
12.));
#180724=CARTESIAN_POINT('Ctrl Pts',(-25.2148466201368,-6.02986667390187,
12.));
#180725=CARTESIAN_POINT('Ctrl Pts',(-25.2355918138798,-6.04925720151412,
12.));
#180726=CARTESIAN_POINT('Ctrl Pts',(-25.2521940105523,-6.06484373634696,
12.));
#180727=CARTESIAN_POINT('Ctrl Pts',(-25.2646490489816,-6.07657531787577,
12.));
#180728=CARTESIAN_POINT('Ctrl Pts',(-25.2729539149479,-6.08441489609824,
12.));
#180729=CARTESIAN_POINT('Ctrl Pts',(-25.2771067246846,-6.08833931617698,
12.));
#180730=CARTESIAN_POINT('',(-24.9347862158358,-7.36589684767343,12.));
#180731=CARTESIAN_POINT('Origin',(0.,0.,12.));
#180732=CARTESIAN_POINT('',(-21.2610617890679,-7.52250298901264,12.));
#180733=CARTESIAN_POINT('Ctrl Pts',(-24.9347862158358,-7.36589684767343,
12.));
#180734=CARTESIAN_POINT('Ctrl Pts',(-24.9292275670705,-7.36721909029059,
12.));
#180735=CARTESIAN_POINT('Ctrl Pts',(-24.9181155530631,-7.36985593120696,
12.));
#180736=CARTESIAN_POINT('Ctrl Pts',(-24.9014633826201,-7.37378825962717,
12.));
#180737=CARTESIAN_POINT('Ctrl Pts',(-24.8792921911309,-7.3789854964161,
12.));
#180738=CARTESIAN_POINT('Ctrl Pts',(-24.8516310625367,-7.38540558904945,
12.));
#180739=CARTESIAN_POINT('Ctrl Pts',(-24.8240228521042,-7.39174922586841,
12.));
#180740=CARTESIAN_POINT('Ctrl Pts',(-24.7964676646518,-7.39801641583612,
12.));
#180741=CARTESIAN_POINT('Ctrl Pts',(-24.7689656669005,-7.40420718661754,
12.));
#180742=CARTESIAN_POINT('Ctrl Pts',(-24.7415170994754,-7.41032159082173,
12.));
#180743=CARTESIAN_POINT('Ctrl Pts',(-24.7141222949988,-7.41635971481243,
12.));
#180744=CARTESIAN_POINT('Ctrl Pts',(-24.6867816727118,-7.42232167765762,
12.));
#180745=CARTESIAN_POINT('Ctrl Pts',(-24.659495712869,-7.4282076215868,12.));
#180746=CARTESIAN_POINT('Ctrl Pts',(-24.6322649369472,-7.4340177048922,
12.));
#180747=CARTESIAN_POINT('Ctrl Pts',(-24.6050898852349,-7.43975209375374,
12.));
#180748=CARTESIAN_POINT('Ctrl Pts',(-24.5779710960865,-7.44541095473162,
12.));
#180749=CARTESIAN_POINT('Ctrl Pts',(-24.5509090831579,-7.45099444651295,
12.));
#180750=CARTESIAN_POINT('Ctrl Pts',(-24.52390431731,-7.45650271336045,12.));
#180751=CARTESIAN_POINT('Ctrl Pts',(-24.4969572391509,-7.46193588961641,
12.));
#180752=CARTESIAN_POINT('Ctrl Pts',(-24.4700682684544,-7.46729410308922,
12.));
#180753=CARTESIAN_POINT('Ctrl Pts',(-24.4432378146501,-7.47257747883318,
12.));
#180754=CARTESIAN_POINT('Ctrl Pts',(-24.4164662871165,-7.47778614286573,
12.));
#180755=CARTESIAN_POINT('Ctrl Pts',(-24.3897541049248,-7.48292022569253,
12.));
#180756=CARTESIAN_POINT('Ctrl Pts',(-24.3631017084513,-7.48797986651827,
12.));
#180757=CARTESIAN_POINT('Ctrl Pts',(-24.3365095573673,-7.49296521252329,
12.));
#180758=CARTESIAN_POINT('Ctrl Pts',(-24.3099781253345,-7.49787641695358,
12.));
#180759=CARTESIAN_POINT('Ctrl Pts',(-24.2835078958966,-7.50271363765098,
12.));
#180760=CARTESIAN_POINT('Ctrl Pts',(-24.2570993577032,-7.50747703535114,
12.));
#180761=CARTESIAN_POINT('Ctrl Pts',(-24.230753000389,-7.51216677222198,
12.));
#180762=CARTESIAN_POINT('Ctrl Pts',(-24.2044693092356,-7.51678300997997,
12.));
#180763=CARTESIAN_POINT('Ctrl Pts',(-24.1782487641602,-7.52132590953862,
12.));
#180764=CARTESIAN_POINT('Ctrl Pts',(-24.152091842537,-7.52579563201478,
12.));
#180765=CARTESIAN_POINT('Ctrl Pts',(-24.1259990209211,-7.53019233935536,
12.));
#180766=CARTESIAN_POINT('Ctrl Pts',(-24.0999707772643,-7.53451619514658,
12.));
#180767=CARTESIAN_POINT('Ctrl Pts',(-24.0740075927984,-7.53876736531004,
12.));
#180768=CARTESIAN_POINT('Ctrl Pts',(-24.0481099543353,-7.54294601896127,
12.));
#180769=CARTESIAN_POINT('Ctrl Pts',(-24.0222783554531,-7.54705232885894,
12.));
#180770=CARTESIAN_POINT('Ctrl Pts',(-23.9965132953187,-7.55108647097431,
12.));
#180771=CARTESIAN_POINT('Ctrl Pts',(-23.9708152779886,-7.55504862424807,
12.));
#180772=CARTESIAN_POINT('Ctrl Pts',(-23.9451848115002,-7.55893897027679,
12.));
#180773=CARTESIAN_POINT('Ctrl Pts',(-23.9196224070759,-7.56275769304772,
12.));
#180774=CARTESIAN_POINT('Ctrl Pts',(-23.8941285782002,-7.5665049786379,
12.));
#180775=CARTESIAN_POINT('Ctrl Pts',(-23.8687038399595,-7.57018101500709,
12.));
#180776=CARTESIAN_POINT('Ctrl Pts',(-23.8433487096132,-7.57378599219814,
12.));
#180777=CARTESIAN_POINT('Ctrl Pts',(-23.8180637069976,-7.57732010249065,
12.));
#180778=CARTESIAN_POINT('Ctrl Pts',(-23.7928493549908,-7.58078354058212,
12.));
#180779=CARTESIAN_POINT('Ctrl Pts',(-23.7677061799376,-7.5841765037627,
12.));
#180780=CARTESIAN_POINT('Ctrl Pts',(-23.7426347121006,-7.58749919210825,
12.));
#180781=CARTESIAN_POINT('Ctrl Pts',(-23.7176354860457,-7.5907518086532,
12.));
#180782=CARTESIAN_POINT('Ctrl Pts',(-23.6927090405066,-7.59393455934034,
12.));
#180783=CARTESIAN_POINT('Ctrl Pts',(-23.6678559182875,-7.59704765299566,
12.));
#180784=CARTESIAN_POINT('Ctrl Pts',(-23.6430766661418,-7.60009130130125,
12.));
#180785=CARTESIAN_POINT('Ctrl Pts',(-23.6183718346576,-7.60306571877805,
12.));
#180786=CARTESIAN_POINT('Ctrl Pts',(-23.5937419781245,-7.60597112277093,
12.));
#180787=CARTESIAN_POINT('Ctrl Pts',(-23.5691876544244,-7.60880773344599,
12.));
#180788=CARTESIAN_POINT('Ctrl Pts',(-23.544709425203,-7.61157577385371,
12.));
#180789=CARTESIAN_POINT('Ctrl Pts',(-23.5203078560129,-7.61427546999297,
12.));
#180790=CARTESIAN_POINT('Ctrl Pts',(-23.4959835164609,-7.61690705088318,
12.));
#180791=CARTESIAN_POINT('Ctrl Pts',(-23.4717369803438,-7.61947074863976,
12.));
#180792=CARTESIAN_POINT('Ctrl Pts',(-23.4475688257854,-7.62196679855954,
12.));
#180793=CARTESIAN_POINT('Ctrl Pts',(-23.4234796353542,-7.62439543920049,
12.));
#180794=CARTESIAN_POINT('Ctrl Pts',(-23.399469996112,-7.62675691240328,
12.));
#180795=CARTESIAN_POINT('Ctrl Pts',(-23.3755404996636,-7.62905146332592,
12.));
#180796=CARTESIAN_POINT('Ctrl Pts',(-23.3516917421972,-7.63127934048136,
12.));
#180797=CARTESIAN_POINT('Ctrl Pts',(-23.3279243245241,-7.63344079578161,
12.));
#180798=CARTESIAN_POINT('Ctrl Pts',(-23.3042388521022,-7.63553608458782,
12.));
#180799=CARTESIAN_POINT('Ctrl Pts',(-23.2806359350855,-7.63756546576374,
12.));
#180800=CARTESIAN_POINT('Ctrl Pts',(-23.2571161884488,-7.63952920172835,
12.));
#180801=CARTESIAN_POINT('Ctrl Pts',(-23.2336802320912,-7.64142755851504,
12.));
#180802=CARTESIAN_POINT('Ctrl Pts',(-23.2103286909398,-7.64326080583679,
12.));
#180803=CARTESIAN_POINT('Ctrl Pts',(-23.1870621950452,-7.64502921715482,
12.));
#180804=CARTESIAN_POINT('Ctrl Pts',(-23.1638813796694,-7.64673306975804,
12.));
#180805=CARTESIAN_POINT('Ctrl Pts',(-23.1407868853819,-7.64837264482942,
12.));
#180806=CARTESIAN_POINT('Ctrl Pts',(-23.1177793581679,-7.64994822749859,
12.));
#180807=CARTESIAN_POINT('Ctrl Pts',(-23.094859449525,-7.65146010690475,
12.));
#180808=CARTESIAN_POINT('Ctrl Pts',(-23.072027816555,-7.65290857626357,
12.));
#180809=CARTESIAN_POINT('Ctrl Pts',(-23.0492851220528,-7.65429393293945,
12.));
#180810=CARTESIAN_POINT('Ctrl Pts',(-23.0266320345787,-7.65561647852533,
12.));
#180811=CARTESIAN_POINT('Ctrl Pts',(-23.0040692285814,-7.65687651891304,
12.));
#180812=CARTESIAN_POINT('Ctrl Pts',(-22.9815973845296,-7.65807436436431,
12.));
#180813=CARTESIAN_POINT('Ctrl Pts',(-22.959217189033,-7.65921032958901,
12.));
#180814=CARTESIAN_POINT('Ctrl Pts',(-22.9369293349593,-7.66028473382777,
12.));
#180815=CARTESIAN_POINT('Ctrl Pts',(-22.9147345215421,-7.66129790094107,
12.));
#180816=CARTESIAN_POINT('Ctrl Pts',(-22.8926334544883,-7.66225015950155,
12.));
#180817=CARTESIAN_POINT('Ctrl Pts',(-22.8706268461283,-7.66314184287336,
12.));
#180818=CARTESIAN_POINT('Ctrl Pts',(-22.848715415557,-7.66397328929802,
12.));
#180819=CARTESIAN_POINT('Ctrl Pts',(-22.8268998887678,-7.66474484198548,
12.));
#180820=CARTESIAN_POINT('Ctrl Pts',(-22.8051809987833,-7.66545684920987,
12.));
#180821=CARTESIAN_POINT('Ctrl Pts',(-22.7835594857699,-7.66610966441272,
12.));
#180822=CARTESIAN_POINT('Ctrl Pts',(-22.7620360971843,-7.66670364630298,
12.));
#180823=CARTESIAN_POINT('Ctrl Pts',(-22.7406115879513,-7.66723915895439,
12.));
#180824=CARTESIAN_POINT('Ctrl Pts',(-22.7192867206245,-7.66771657191027,
12.));
#180825=CARTESIAN_POINT('Ctrl Pts',(-22.6980622655446,-7.66813626029274,
12.));
#180826=CARTESIAN_POINT('Ctrl Pts',(-22.6769390009885,-7.66849860491742,
12.));
#180827=CARTESIAN_POINT('Ctrl Pts',(-22.6559177133127,-7.66880399241322,
12.));
#180828=CARTESIAN_POINT('Ctrl Pts',(-22.6349991971541,-7.66905281533714,
12.));
#180829=CARTESIAN_POINT('Ctrl Pts',(-22.6141842556243,-7.66924547229413,
12.));
#180830=CARTESIAN_POINT('Ctrl Pts',(-22.5934737004953,-7.66938236806232,
12.));
#180831=CARTESIAN_POINT('Ctrl Pts',(-22.5728683523831,-7.66946391372305,
12.));
#180832=CARTESIAN_POINT('Ctrl Pts',(-22.5523690409116,-7.66949052679692,
12.));
#180833=CARTESIAN_POINT('Ctrl Pts',(-22.53197660492,-7.66946263138143,12.));
#180834=CARTESIAN_POINT('Ctrl Pts',(-22.5116918927032,-7.66938065829107,
12.));
#180835=CARTESIAN_POINT('Ctrl Pts',(-22.4915157622312,-7.66924504520314,
12.));
#180836=CARTESIAN_POINT('Ctrl Pts',(-22.47144908137,-7.6690562368083,12.));
#180837=CARTESIAN_POINT('Ctrl Pts',(-22.4514927280855,-7.66881468496634,
12.));
#180838=CARTESIAN_POINT('Ctrl Pts',(-22.4316475906603,-7.66852084886704,
12.));
#180839=CARTESIAN_POINT('Ctrl Pts',(-22.4119145679758,-7.66817519519639,
12.));
#180840=CARTESIAN_POINT('Ctrl Pts',(-22.3922945697773,-7.66777819830789,
12.));
#180841=CARTESIAN_POINT('Ctrl Pts',(-22.372788516936,-7.66733034039882,
12.));
#180842=CARTESIAN_POINT('Ctrl Pts',(-22.3533973417021,-7.66683211169158,
12.));
#180843=CARTESIAN_POINT('Ctrl Pts',(-22.3341219879469,-7.66628401061952,
12.));
#180844=CARTESIAN_POINT('Ctrl Pts',(-22.314963411484,-7.66568654402493,
12.));
#180845=CARTESIAN_POINT('Ctrl Pts',(-22.2959225803937,-7.66504022736298,
12.));
#180846=CARTESIAN_POINT('Ctrl Pts',(-22.2770004753335,-7.66434558490978,
12.));
#180847=CARTESIAN_POINT('Ctrl Pts',(-22.258198089848,-7.6636031499764,12.));
#180848=CARTESIAN_POINT('Ctrl Pts',(-22.2395164306547,-7.66281346512508,
12.));
#180849=CARTESIAN_POINT('Ctrl Pts',(-22.2209565180085,-7.66197708240399,
12.));
#180850=CARTESIAN_POINT('Ctrl Pts',(-22.2025193860964,-7.6610945635927,
12.));
#180851=CARTESIAN_POINT('Ctrl Pts',(-22.1842060834091,-7.66016648045004,
12.));
#180852=CARTESIAN_POINT('Ctrl Pts',(-22.1660176731178,-7.6591934149693,
12.));
#180853=CARTESIAN_POINT('Ctrl Pts',(-22.1479552334211,-7.65817595963349,
12.));
#180854=CARTESIAN_POINT('Ctrl Pts',(-22.1300198579675,-7.65711471769396,
12.));
#180855=CARTESIAN_POINT('Ctrl Pts',(-22.1122126563329,-7.65601030346806,
12.));
#180856=CARTESIAN_POINT('Ctrl Pts',(-22.094534754469,-7.65486334263643,
12.));
#180857=CARTESIAN_POINT('Ctrl Pts',(-22.0769872951596,-7.65367447254949,
12.));
#180858=CARTESIAN_POINT('Ctrl Pts',(-22.0595714384431,-7.65244434253112,
12.));
#180859=CARTESIAN_POINT('Ctrl Pts',(-22.0422883621174,-7.65117361421358,
12.));
#180860=CARTESIAN_POINT('Ctrl Pts',(-22.0251392623209,-7.64986296190168,
12.));
#180861=CARTESIAN_POINT('Ctrl Pts',(-22.0081253540774,-7.64851307293351,
12.));
#180862=CARTESIAN_POINT('Ctrl Pts',(-21.9912478718542,-7.64712464805249,
12.));
#180863=CARTESIAN_POINT('Ctrl Pts',(-21.9745080700798,-7.64569840177335,
12.));
#180864=CARTESIAN_POINT('Ctrl Pts',(-21.9579072237651,-7.64423506279122,
12.));
#180865=CARTESIAN_POINT('Ctrl Pts',(-21.9414466292072,-7.64273537442682,
12.));
#180866=CARTESIAN_POINT('Ctrl Pts',(-21.9251276046546,-7.64120009506531,
12.));
#180867=CARTESIAN_POINT('Ctrl Pts',(-21.9089514909874,-7.63962999860927,
12.));
#180868=CARTESIAN_POINT('Ctrl Pts',(-21.8929196523514,-7.63802587492034,
12.));
#180869=CARTESIAN_POINT('Ctrl Pts',(-21.8770334769496,-7.63638853033399,
12.));
#180870=CARTESIAN_POINT('Ctrl Pts',(-21.8612943779089,-7.63471878821225,
12.));
#180871=CARTESIAN_POINT('Ctrl Pts',(-21.8457037941084,-7.63301748948935,
12.));
#180872=CARTESIAN_POINT('Ctrl Pts',(-21.8302631910195,-7.63128549323022,
12.));
#180873=CARTESIAN_POINT('Ctrl Pts',(-21.814974061509,-7.62952367718126,
12.));
#180874=CARTESIAN_POINT('Ctrl Pts',(-21.799837926858,-7.62773293842389,
12.));
#180875=CARTESIAN_POINT('Ctrl Pts',(-21.7848563378021,-7.62591419404512,
12.));
#180876=CARTESIAN_POINT('Ctrl Pts',(-21.7700308755584,-7.62406838181166,
12.));
#180877=CARTESIAN_POINT('Ctrl Pts',(-21.7553631528328,-7.62219646084228,
12.));
#180878=CARTESIAN_POINT('Ctrl Pts',(-21.7408548148656,-7.62029941230854,
12.));
#180879=CARTESIAN_POINT('Ctrl Pts',(-21.7265075407975,-7.61837824030537,
12.));
#180880=CARTESIAN_POINT('Ctrl Pts',(-21.7123230449834,-7.6164339727042,
12.));
#180881=CARTESIAN_POINT('Ctrl Pts',(-21.6983030783322,-7.61446766202786,
12.));
#180882=CARTESIAN_POINT('Ctrl Pts',(-21.6844494295815,-7.61248038630268,
12.));
#180883=CARTESIAN_POINT('Ctrl Pts',(-21.6707639267576,-7.61047325000955,
12.));
#180884=CARTESIAN_POINT('Ctrl Pts',(-21.6572484388081,-7.60844738512873,
12.));
#180885=CARTESIAN_POINT('Ctrl Pts',(-21.6439048771743,-7.60640395216356,
12.));
#180886=CARTESIAN_POINT('Ctrl Pts',(-21.6307351973822,-7.60434414118295,
12.));
#180887=CARTESIAN_POINT('Ctrl Pts',(-21.617741400599,-7.60226917285428,
12.));
#180888=CARTESIAN_POINT('Ctrl Pts',(-21.6049255358843,-7.6001802998824,
12.));
#180889=CARTESIAN_POINT('Ctrl Pts',(-21.5922897024466,-7.59807880846194,
12.));
#180890=CARTESIAN_POINT('Ctrl Pts',(-21.5798360518978,-7.59596601973583,
12.));
#180891=CARTESIAN_POINT('Ctrl Pts',(-21.5675667904726,-7.59384329124918,
12.));
#180892=CARTESIAN_POINT('Ctrl Pts',(-21.5554841813462,-7.59171201844776,
12.));
#180893=CARTESIAN_POINT('Ctrl Pts',(-21.543590547011,-7.58957363620013,
12.));
#180894=CARTESIAN_POINT('Ctrl Pts',(-21.5318882716736,-7.58742962034833,
12.));
#180895=CARTESIAN_POINT('Ctrl Pts',(-21.5203798035299,-7.58528148919129,
12.));
#180896=CARTESIAN_POINT('Ctrl Pts',(-21.5090676573873,-7.58313080519179,
12.));
#180897=CARTESIAN_POINT('Ctrl Pts',(-21.4979544192744,-7.58097917790744,
12.));
#180898=CARTESIAN_POINT('Ctrl Pts',(-21.4870427508194,-7.57882826679131,
12.));
#180899=CARTESIAN_POINT('Ctrl Pts',(-21.4763353936762,-7.57667978402987,
12.));
#180900=CARTESIAN_POINT('Ctrl Pts',(-21.4658351740128,-7.57453549743411,
12.));
#180901=CARTESIAN_POINT('Ctrl Pts',(-21.4555450053142,-7.57239723223505,
12.));
#180902=CARTESIAN_POINT('Ctrl Pts',(-21.4454678907509,-7.57026687261165,
12.));
#180903=CARTESIAN_POINT('Ctrl Pts',(-21.4356069261513,-7.56814636360847,
12.));
#180904=CARTESIAN_POINT('Ctrl Pts',(-21.4259653015736,-7.56603771218712,
12.));
#180905=CARTESIAN_POINT('Ctrl Pts',(-21.4165463106254,-7.56394299313684,
12.));
#180906=CARTESIAN_POINT('Ctrl Pts',(-21.4073533630365,-7.56186435703621,
12.));
#180907=CARTESIAN_POINT('Ctrl Pts',(-21.3983899952987,-7.5598040370061,
12.));
#180908=CARTESIAN_POINT('Ctrl Pts',(-21.3896598842117,-7.55776435731416,
12.));
#180909=CARTESIAN_POINT('Ctrl Pts',(-21.3811668478932,-7.55574773403502,
12.));
#180910=CARTESIAN_POINT('Ctrl Pts',(-21.3729148390243,-7.55375667080028,
12.));
#180911=CARTESIAN_POINT('Ctrl Pts',(-21.3649079431865,-7.55179375777443,
12.));
#180912=CARTESIAN_POINT('Ctrl Pts',(-21.3571503685855,-7.54986166521309,
12.));
#180913=CARTESIAN_POINT('Ctrl Pts',(-21.3496464761531,-7.5479631624633,
12.));
#180914=CARTESIAN_POINT('Ctrl Pts',(-21.3424008295038,-7.54610114948346,
12.));
#180915=CARTESIAN_POINT('Ctrl Pts',(-21.3354182340149,-7.54427868151267,
12.));
#180916=CARTESIAN_POINT('Ctrl Pts',(-21.328703791771,-7.5424990037703,12.));
#180917=CARTESIAN_POINT('Ctrl Pts',(-21.3222628524165,-7.54076552038278,
12.));
#180918=CARTESIAN_POINT('Ctrl Pts',(-21.3161009456256,-7.53908175169898,
12.));
#180919=CARTESIAN_POINT('Ctrl Pts',(-21.310223716773,-7.53745129364616,
12.));
#180920=CARTESIAN_POINT('Ctrl Pts',(-21.3046368712157,-7.53587778251735,
12.));
#180921=CARTESIAN_POINT('Ctrl Pts',(-21.2993464250717,-7.53436505309942,
12.));
#180922=CARTESIAN_POINT('Ctrl Pts',(-21.2943588989331,-7.53291726078526,
12.));
#180923=CARTESIAN_POINT('Ctrl Pts',(-21.2896816163842,-7.53153906987855,
12.));
#180924=CARTESIAN_POINT('Ctrl Pts',(-21.2853226580657,-7.53023562438229,
12.));
#180925=CARTESIAN_POINT('Ctrl Pts',(-21.2812902781143,-7.52901217930407,
12.));
#180926=CARTESIAN_POINT('Ctrl Pts',(-21.2775925269652,-7.52787386225332,
12.));
#180927=CARTESIAN_POINT('Ctrl Pts',(-21.2742366113579,-7.5268252691854,
12.));
#180928=CARTESIAN_POINT('Ctrl Pts',(-21.2712301573466,-7.52587126095529,
12.));
#180929=CARTESIAN_POINT('Ctrl Pts',(-21.2685823838671,-7.5250177033353,
12.));
#180930=CARTESIAN_POINT('Ctrl Pts',(-21.2663059157058,-7.52427261074297,
12.));
#180931=CARTESIAN_POINT('Ctrl Pts',(-21.2644161259962,-7.52364573027552,
12.));
#180932=CARTESIAN_POINT('Ctrl Pts',(-21.262927782038,-7.52314642316199,
12.));
#180933=CARTESIAN_POINT('Ctrl Pts',(-21.2618521283555,-7.52278182242669,
12.));
#180934=CARTESIAN_POINT('Ctrl Pts',(-21.261326054066,-7.5226006423166,12.));
#180935=CARTESIAN_POINT('Ctrl Pts',(-21.2611204474866,-7.52252744144903,
12.));
#180936=CARTESIAN_POINT('Ctrl Pts',(-21.2610673466886,-7.5225064970397,
12.));
#180937=CARTESIAN_POINT('Ctrl Pts',(-21.2610617890679,-7.52250298901264,
12.));
#180938=CARTESIAN_POINT('',(-20.7347298079577,-7.33627833380045,12.));
#180939=CARTESIAN_POINT('',(-10.1343606576251,-3.58569854577611,12.));
#180940=CARTESIAN_POINT('',(-20.1004996511507,-7.63019749246977,12.));
#180941=CARTESIAN_POINT('Origin',(-20.56795313141,-7.80764394578302,12.));
#180942=CARTESIAN_POINT('',(-19.6085639972844,-8.81783521984849,12.));
#180943=CARTESIAN_POINT('Origin',(-7.32141292029404E-13,-2.70312158620511E-13,
12.));
#180944=CARTESIAN_POINT('',(-19.84920021178,-9.47413589477548,12.));
#180945=CARTESIAN_POINT('Origin',(-20.0645771135004,-9.0229011551938,12.));
#180946=CARTESIAN_POINT('',(-20.353053841303,-9.71462809124915,12.));
#180947=CARTESIAN_POINT('',(-10.1765269206515,-4.85731404562459,12.));
#180948=CARTESIAN_POINT('',(-22.8400320311649,-12.4230808101438,12.));
#180949=CARTESIAN_POINT('Ctrl Pts',(-20.353053841303,-9.71462809124915,
12.));
#180950=CARTESIAN_POINT('Ctrl Pts',(-20.353060251684,-9.71462954053041,
12.));
#180951=CARTESIAN_POINT('Ctrl Pts',(-20.3531126095522,-9.71465227853041,
12.));
#180952=CARTESIAN_POINT('Ctrl Pts',(-20.3533097561886,-9.7147459035068,
12.));
#180953=CARTESIAN_POINT('Ctrl Pts',(-20.3538098605706,-9.7149897805202,
12.));
#180954=CARTESIAN_POINT('Ctrl Pts',(-20.3548282742361,-9.71549257088172,
12.));
#180955=CARTESIAN_POINT('Ctrl Pts',(-20.3562337557875,-9.71619192554185,
12.));
#180956=CARTESIAN_POINT('Ctrl Pts',(-20.3580133103356,-9.71708493723096,
12.));
#180957=CARTESIAN_POINT('Ctrl Pts',(-20.3601498764344,-9.71816778328006,
12.));
#180958=CARTESIAN_POINT('Ctrl Pts',(-20.3626256913981,-9.71943648548099,
12.));
#180959=CARTESIAN_POINT('Ctrl Pts',(-20.3654261611056,-9.7208877838108,
12.));
#180960=CARTESIAN_POINT('Ctrl Pts',(-20.3685406190576,-9.72251930722489,
12.));
#180961=CARTESIAN_POINT('Ctrl Pts',(-20.371960235676,-9.72432910043194,
12.));
#180962=CARTESIAN_POINT('Ctrl Pts',(-20.3756766651951,-9.7263153173288,
12.));
#180963=CARTESIAN_POINT('Ctrl Pts',(-20.3796805893304,-9.72847589116541,
12.));
#180964=CARTESIAN_POINT('Ctrl Pts',(-20.3839624556742,-9.73080870123727,
12.));
#180965=CARTESIAN_POINT('Ctrl Pts',(-20.3885129129912,-9.73331167102807,
12.));
#180966=CARTESIAN_POINT('Ctrl Pts',(-20.3933234845647,-9.73598292014242,
12.));
#180967=CARTESIAN_POINT('Ctrl Pts',(-20.3983866213331,-9.738820776132,12.));
#180968=CARTESIAN_POINT('Ctrl Pts',(-20.4036953576549,-9.74182369656271,
12.));
#180969=CARTESIAN_POINT('Ctrl Pts',(-20.4092430879861,-9.74499021838537,
12.));
#180970=CARTESIAN_POINT('Ctrl Pts',(-20.4150232777393,-9.74831889242174,
12.));
#180971=CARTESIAN_POINT('Ctrl Pts',(-20.4210295275817,-9.7518082978643,
12.));
#180972=CARTESIAN_POINT('Ctrl Pts',(-20.4272556476629,-9.75545705902417,
12.));
#180973=CARTESIAN_POINT('Ctrl Pts',(-20.4336957355473,-9.75926386289922,
12.));
#180974=CARTESIAN_POINT('Ctrl Pts',(-20.44034423294,-9.76322747195494,12.));
#180975=CARTESIAN_POINT('Ctrl Pts',(-20.447195862298,-9.76734670980891,
12.));
#180976=CARTESIAN_POINT('Ctrl Pts',(-20.4542455817527,-9.77162045104069,
12.));
#180977=CARTESIAN_POINT('Ctrl Pts',(-20.4614885274975,-9.77604760815528,
12.));
#180978=CARTESIAN_POINT('Ctrl Pts',(-20.4689199790669,-9.7806271237332,
12.));
#180979=CARTESIAN_POINT('Ctrl Pts',(-20.4765353711586,-9.78535797314166,
12.));
#180980=CARTESIAN_POINT('Ctrl Pts',(-20.4843302955329,-9.79023916498655,
12.));
#180981=CARTESIAN_POINT('Ctrl Pts',(-20.4923005087943,-9.7952697428833,
12.));
#180982=CARTESIAN_POINT('Ctrl Pts',(-20.5004419312107,-9.80044878520948,
12.));
#180983=CARTESIAN_POINT('Ctrl Pts',(-20.5087506310505,-9.80577540161087,
12.));
#180984=CARTESIAN_POINT('Ctrl Pts',(-20.517222812284,-9.81124873025281,
12.));
#180985=CARTESIAN_POINT('Ctrl Pts',(-20.5258548000629,-9.81686793455942,
12.));
#180986=CARTESIAN_POINT('Ctrl Pts',(-20.5346430299517,-9.82263220080362,
12.));
#180987=CARTESIAN_POINT('Ctrl Pts',(-20.5435840460721,-9.82854073773877,
12.));
#180988=CARTESIAN_POINT('Ctrl Pts',(-20.552674497646,-9.83459277585315,
12.));
#180989=CARTESIAN_POINT('Ctrl Pts',(-20.5619111362402,-9.84078756677565,
12.));
#180990=CARTESIAN_POINT('Ctrl Pts',(-20.5712908125139,-9.84712438256277,
12.));
#180991=CARTESIAN_POINT('Ctrl Pts',(-20.5808104710015,-9.8536025145698,
12.));
#180992=CARTESIAN_POINT('Ctrl Pts',(-20.5904671449754,-9.86022127232747,
12.));
#180993=CARTESIAN_POINT('Ctrl Pts',(-20.6002579513699,-9.86697998242622,
12.));
#180994=CARTESIAN_POINT('Ctrl Pts',(-20.6101800854494,-9.87387798732956,
12.));
#180995=CARTESIAN_POINT('Ctrl Pts',(-20.6202308177474,-9.88091464472675,
12.));
#180996=CARTESIAN_POINT('Ctrl Pts',(-20.6304074914087,-9.88808932697306,
12.));
#180997=CARTESIAN_POINT('Ctrl Pts',(-20.6407075193976,-9.89540142049119,
12.));
#180998=CARTESIAN_POINT('Ctrl Pts',(-20.6511283817414,-9.90285032516692,
12.));
#180999=CARTESIAN_POINT('Ctrl Pts',(-20.6616676228315,-9.91043545377007,
12.));
#181000=CARTESIAN_POINT('Ctrl Pts',(-20.6723228488263,-9.91815623141288,
12.));
#181001=CARTESIAN_POINT('Ctrl Pts',(-20.6830917250255,-9.92601209498748,
12.));
#181002=CARTESIAN_POINT('Ctrl Pts',(-20.6939719732484,-9.93400249259729,
12.));
#181003=CARTESIAN_POINT('Ctrl Pts',(-20.7049613692234,-9.94212688298236,
12.));
#181004=CARTESIAN_POINT('Ctrl Pts',(-20.7160577407579,-9.95038473514948,
12.));
#181005=CARTESIAN_POINT('Ctrl Pts',(-20.7272589658751,-9.95877552798397,
12.));
#181006=CARTESIAN_POINT('Ctrl Pts',(-20.7385629709795,-9.96729874986201,
12.));
#181007=CARTESIAN_POINT('Ctrl Pts',(-20.7499677289627,-9.9759538982347,
12.));
#181008=CARTESIAN_POINT('Ctrl Pts',(-20.761471257499,-9.98474047926852,
12.));
#181009=CARTESIAN_POINT('Ctrl Pts',(-20.7730716175417,-9.9936580075464,
12.));
#181010=CARTESIAN_POINT('Ctrl Pts',(-20.7847669117568,-10.0027060057389,
12.));
#181011=CARTESIAN_POINT('Ctrl Pts',(-20.7965552829908,-10.0118840042786,
12.));
#181012=CARTESIAN_POINT('Ctrl Pts',(-20.8084349126888,-10.0211915410095,
12.));
#181013=CARTESIAN_POINT('Ctrl Pts',(-20.8204040196602,-10.0306281609435,
12.));
#181014=CARTESIAN_POINT('Ctrl Pts',(-20.8324608588909,-10.0401934160234,
12.));
#181015=CARTESIAN_POINT('Ctrl Pts',(-20.8446037203402,-10.0498868648733,
12.));
#181016=CARTESIAN_POINT('Ctrl Pts',(-20.8568309277316,-10.0597080725375,
12.));
#181017=CARTESIAN_POINT('Ctrl Pts',(-20.86914083737,-10.0696566102218,12.));
#181018=CARTESIAN_POINT('Ctrl Pts',(-20.881531837184,-10.0797320551154,
12.));
#181019=CARTESIAN_POINT('Ctrl Pts',(-20.894002345737,-10.0899339901915,
12.));
#181020=CARTESIAN_POINT('Ctrl Pts',(-20.9065508112557,-10.1002620040076,
12.));
#181021=CARTESIAN_POINT('Ctrl Pts',(-20.919175710627,-10.1107156904836,
12.));
#181022=CARTESIAN_POINT('Ctrl Pts',(-20.9318755484734,-10.1212946487057,
12.));
#181023=CARTESIAN_POINT('Ctrl Pts',(-20.9446488563933,-10.1319984827908,
12.));
#181024=CARTESIAN_POINT('Ctrl Pts',(-20.9574941921591,-10.1428268017256,
12.));
#181025=CARTESIAN_POINT('Ctrl Pts',(-20.9704101389369,-10.1537792192065,
12.));
#181026=CARTESIAN_POINT('Ctrl Pts',(-20.9833953044736,-10.1648553534568,
12.));
#181027=CARTESIAN_POINT('Ctrl Pts',(-20.9964483203686,-10.1760548270767,
12.));
#181028=CARTESIAN_POINT('Ctrl Pts',(-21.0095678414486,-10.187377266936,
12.));
#181029=CARTESIAN_POINT('Ctrl Pts',(-21.0227525451107,-10.1988223040425,
12.));
#181030=CARTESIAN_POINT('Ctrl Pts',(-21.0360011306815,-10.2103895734123,
12.));
#181031=CARTESIAN_POINT('Ctrl Pts',(-21.0493123187483,-10.2220787139154,
12.));
#181032=CARTESIAN_POINT('Ctrl Pts',(-21.0626848505663,-10.2338893681567,
12.));
#181033=CARTESIAN_POINT('Ctrl Pts',(-21.0761174875445,-10.2458211823912,
12.));
#181034=CARTESIAN_POINT('Ctrl Pts',(-21.0896090107063,-10.2578738064181,
12.));
#181035=CARTESIAN_POINT('Ctrl Pts',(-21.1031582201627,-10.2700468934744,
12.));
#181036=CARTESIAN_POINT('Ctrl Pts',(-21.1167639345631,-10.2823401001072,
12.));
#181037=CARTESIAN_POINT('Ctrl Pts',(-21.1304249906002,-10.2947530860721,
12.));
#181038=CARTESIAN_POINT('Ctrl Pts',(-21.1441402425843,-10.3072855142687,
12.));
#181039=CARTESIAN_POINT('Ctrl Pts',(-21.1579085619965,-10.3199370506544,
12.));
#181040=CARTESIAN_POINT('Ctrl Pts',(-21.1717288370509,-10.3327073641572,
12.));
#181041=CARTESIAN_POINT('Ctrl Pts',(-21.1855999722416,-10.34559612657,12.));
#181042=CARTESIAN_POINT('Ctrl Pts',(-21.199520887919,-10.3586030124587,
12.));
#181043=CARTESIAN_POINT('Ctrl Pts',(-21.2134905199345,-10.371727699113,
12.));
#181044=CARTESIAN_POINT('Ctrl Pts',(-21.22750781927,-10.3849698664786,12.));
#181045=CARTESIAN_POINT('Ctrl Pts',(-21.2415717516714,-10.3983291970846,
12.));
#181046=CARTESIAN_POINT('Ctrl Pts',(-21.255681297275,-10.4118053759588,
12.));
#181047=CARTESIAN_POINT('Ctrl Pts',(-21.2698354502403,-10.42539809054,12.));
#181048=CARTESIAN_POINT('Ctrl Pts',(-21.2840332184483,-10.4391070306391,
12.));
#181049=CARTESIAN_POINT('Ctrl Pts',(-21.2982736231931,-10.4529318883874,
12.));
#181050=CARTESIAN_POINT('Ctrl Pts',(-21.3125556988731,-10.4668723581768,
12.));
#181051=CARTESIAN_POINT('Ctrl Pts',(-21.3268784926819,-10.4809281365931,
12.));
#181052=CARTESIAN_POINT('Ctrl Pts',(-21.3412410642904,-10.4950989223337,
12.));
#181053=CARTESIAN_POINT('Ctrl Pts',(-21.3556424855814,-10.5093844161685,
12.));
#181054=CARTESIAN_POINT('Ctrl Pts',(-21.3700818403936,-10.5237843209057,
12.));
#181055=CARTESIAN_POINT('Ctrl Pts',(-21.3845582242602,-10.5382983413421,
12.));
#181056=CARTESIAN_POINT('Ctrl Pts',(-21.3990707441497,-10.5529261842108,
12.));
#181057=CARTESIAN_POINT('Ctrl Pts',(-21.4136185181979,-10.5676675581108,
12.));
#181058=CARTESIAN_POINT('Ctrl Pts',(-21.4282006754631,-10.5825221734573,
12.));
#181059=CARTESIAN_POINT('Ctrl Pts',(-21.4428163557144,-10.5974897424622,
12.));
#181060=CARTESIAN_POINT('Ctrl Pts',(-21.4574647092097,-10.6125699790961,
12.));
#181061=CARTESIAN_POINT('Ctrl Pts',(-21.4721448964766,-10.6277625990456,
12.));
#181062=CARTESIAN_POINT('Ctrl Pts',(-21.4868560880889,-10.6430673196607,
12.));
#181063=CARTESIAN_POINT('Ctrl Pts',(-21.5015974644449,-10.6584838598939,
12.));
#181064=CARTESIAN_POINT('Ctrl Pts',(-21.51636821558,-10.6740119402834,12.));
#181065=CARTESIAN_POINT('Ctrl Pts',(-21.5311675409807,-10.689651282929,
12.));
#181066=CARTESIAN_POINT('Ctrl Pts',(-21.5459946493955,-10.7054016114571,
12.));
#181067=CARTESIAN_POINT('Ctrl Pts',(-21.5608487586468,-10.7212626509816,
12.));
#181068=CARTESIAN_POINT('Ctrl Pts',(-21.5757290954371,-10.7372341280467,
12.));
#181069=CARTESIAN_POINT('Ctrl Pts',(-21.5906348951743,-10.7533157705941,
12.));
#181070=CARTESIAN_POINT('Ctrl Pts',(-21.6055654018176,-10.7695073079552,
12.));
#181071=CARTESIAN_POINT('Ctrl Pts',(-21.6205198677173,-10.7858084708261,
12.));
#181072=CARTESIAN_POINT('Ctrl Pts',(-21.6354975534557,-10.8022189912369,
12.));
#181073=CARTESIAN_POINT('Ctrl Pts',(-21.6504977276866,-10.8187386025136,
12.));
#181074=CARTESIAN_POINT('Ctrl Pts',(-21.6655196669732,-10.8353670392272,
12.));
#181075=CARTESIAN_POINT('Ctrl Pts',(-21.6805626556467,-10.8521040371835,
12.));
#181076=CARTESIAN_POINT('Ctrl Pts',(-21.6956259856672,-10.8689493334095,
12.));
#181077=CARTESIAN_POINT('Ctrl Pts',(-21.7107089564825,-10.8859026661293,
12.));
#181078=CARTESIAN_POINT('Ctrl Pts',(-21.7258108748873,-10.902963774734,
12.));
#181079=CARTESIAN_POINT('Ctrl Pts',(-21.7409310548797,-10.9201323997384,
12.));
#181080=CARTESIAN_POINT('Ctrl Pts',(-21.7560688175247,-10.9374082827444,
12.));
#181081=CARTESIAN_POINT('Ctrl Pts',(-21.7712234908464,-10.9547911664455,
12.));
#181082=CARTESIAN_POINT('Ctrl Pts',(-21.7863944097141,-10.9722807946155,
12.));
#181083=CARTESIAN_POINT('Ctrl Pts',(-21.8015809157301,-10.9898769120912,
12.));
#181084=CARTESIAN_POINT('Ctrl Pts',(-21.8167823571168,-11.0075792647477,
12.));
#181085=CARTESIAN_POINT('Ctrl Pts',(-21.8319980886033,-11.0253875994598,
12.));
#181086=CARTESIAN_POINT('Ctrl Pts',(-21.8472274713103,-11.0433016640807,
12.));
#181087=CARTESIAN_POINT('Ctrl Pts',(-21.8624698726318,-11.0613212074363,
12.));
#181088=CARTESIAN_POINT('Ctrl Pts',(-21.877724666119,-11.0794459793057,
12.));
#181089=CARTESIAN_POINT('Ctrl Pts',(-21.8929912313608,-11.0976757303944,
12.));
#181090=CARTESIAN_POINT('Ctrl Pts',(-21.9082689538688,-11.1160102123024,
12.));
#181091=CARTESIAN_POINT('Ctrl Pts',(-21.923557224952,-11.1344491774741,
12.));
#181092=CARTESIAN_POINT('Ctrl Pts',(-21.9388554416439,-11.1529923792003,
12.));
#181093=CARTESIAN_POINT('Ctrl Pts',(-21.9541630066506,-11.1716395716376,
12.));
#181094=CARTESIAN_POINT('Ctrl Pts',(-21.9694793282914,-11.190390509811,
12.));
#181095=CARTESIAN_POINT('Ctrl Pts',(-21.9848038204439,-11.2092449496125,
12.));
#181096=CARTESIAN_POINT('Ctrl Pts',(-22.0001359024839,-11.2282026477896,
12.));
#181097=CARTESIAN_POINT('Ctrl Pts',(-22.0154749992363,-11.2472633619275,
12.));
#181098=CARTESIAN_POINT('Ctrl Pts',(-22.030820540835,-11.2664268504206,
12.));
#181099=CARTESIAN_POINT('Ctrl Pts',(-22.046171962566,-11.2856928724374,
12.));
#181100=CARTESIAN_POINT('Ctrl Pts',(-22.0615287047179,-11.3050611878771,
12.));
#181101=CARTESIAN_POINT('Ctrl Pts',(-22.0768902124267,-11.3245315573168,
12.));
#181102=CARTESIAN_POINT('Ctrl Pts',(-22.0922559355294,-11.3441037419553,
12.));
#181103=CARTESIAN_POINT('Ctrl Pts',(-22.1076253283979,-11.3637775035367,
12.));
#181104=CARTESIAN_POINT('Ctrl Pts',(-22.1229978500186,-11.3835526044256,
12.));
#181105=CARTESIAN_POINT('Ctrl Pts',(-22.1383729640964,-11.4034288076908,
12.));
#181106=CARTESIAN_POINT('Ctrl Pts',(-22.1537501391487,-11.4234058771742,
12.));
#181107=CARTESIAN_POINT('Ctrl Pts',(-22.1691288486096,-11.443483577557,
12.));
#181108=CARTESIAN_POINT('Ctrl Pts',(-22.184508570917,-11.463661674411,12.));
#181109=CARTESIAN_POINT('Ctrl Pts',(-22.1998887896436,-11.483939934259,
12.));
#181110=CARTESIAN_POINT('Ctrl Pts',(-22.2152689931022,-11.5043181244242,
12.));
#181111=CARTESIAN_POINT('Ctrl Pts',(-22.2306486738901,-11.5247960128477,
12.));
#181112=CARTESIAN_POINT('Ctrl Pts',(-22.2460273284654,-11.5453733679121,
12.));
#181113=CARTESIAN_POINT('Ctrl Pts',(-22.2614044566898,-11.5660499582403,
12.));
#181114=CARTESIAN_POINT('Ctrl Pts',(-22.2767795614348,-11.5868255525188,
12.));
#181115=CARTESIAN_POINT('Ctrl Pts',(-22.2921521480356,-11.6076999192357,
12.));
#181116=CARTESIAN_POINT('Ctrl Pts',(-22.3075217249049,-11.6286728270009,
12.));
#181117=CARTESIAN_POINT('Ctrl Pts',(-22.3228878043976,-11.6497440449857,
12.));
#181118=CARTESIAN_POINT('Ctrl Pts',(-22.3382499035619,-11.6709133432985,
12.));
#181119=CARTESIAN_POINT('Ctrl Pts',(-22.3536075450029,-11.6921804934056,
12.));
#181120=CARTESIAN_POINT('Ctrl Pts',(-22.3689602575491,-11.7135452684532,
12.));
#181121=CARTESIAN_POINT('Ctrl Pts',(-22.3843075773899,-11.7350074437961,
12.));
#181122=CARTESIAN_POINT('Ctrl Pts',(-22.3996490469191,-11.7565667964764,
12.));
#181123=CARTESIAN_POINT('Ctrl Pts',(-22.4149842125008,-11.7782231042039,
12.));
#181124=CARTESIAN_POINT('Ctrl Pts',(-22.430312622646,-11.7999761445173,
12.));
#181125=CARTESIAN_POINT('Ctrl Pts',(-22.4456338258735,-11.8218256937889,
12.));
#181126=CARTESIAN_POINT('Ctrl Pts',(-22.4609473690471,-11.8437715264487,
12.));
#181127=CARTESIAN_POINT('Ctrl Pts',(-22.4762527946702,-11.8658134137019,
12.));
#181128=CARTESIAN_POINT('Ctrl Pts',(-22.4915496418485,-11.8879511239942,
12.));
#181129=CARTESIAN_POINT('Ctrl Pts',(-22.5068374513973,-11.9101844254557,
12.));
#181130=CARTESIAN_POINT('Ctrl Pts',(-22.5221157697883,-11.9325130877803,
12.));
#181131=CARTESIAN_POINT('Ctrl Pts',(-22.5373841537307,-11.9549368843997,
12.));
#181132=CARTESIAN_POINT('Ctrl Pts',(-22.5526421741158,-11.9774555943496,
12.));
#181133=CARTESIAN_POINT('Ctrl Pts',(-22.5678894211181,-12.0000690046695,
12.));
#181134=CARTESIAN_POINT('Ctrl Pts',(-22.5831255061282,-12.0227769113127,
12.));
#181135=CARTESIAN_POINT('Ctrl Pts',(-22.5983500505644,-12.0455791139128,
12.));
#181136=CARTESIAN_POINT('Ctrl Pts',(-22.6135626764898,-12.0684754113862,
12.));
#181137=CARTESIAN_POINT('Ctrl Pts',(-22.6287629967056,-12.0914655972823,
12.));
#181138=CARTESIAN_POINT('Ctrl Pts',(-22.6439506046605,-12.1145494550383,
12.));
#181139=CARTESIAN_POINT('Ctrl Pts',(-22.6591250653965,-12.1377267537145,
12.));
#181140=CARTESIAN_POINT('Ctrl Pts',(-22.6742859034944,-12.1609972423099,
12.));
#181141=CARTESIAN_POINT('Ctrl Pts',(-22.6894326205037,-12.1843606579261,
12.));
#181142=CARTESIAN_POINT('Ctrl Pts',(-22.7045647168747,-12.2078167360284,
12.));
#181143=CARTESIAN_POINT('Ctrl Pts',(-22.7196817119374,-12.2313652198061,
12.));
#181144=CARTESIAN_POINT('Ctrl Pts',(-22.7347831655287,-12.2550058702395,
12.));
#181145=CARTESIAN_POINT('Ctrl Pts',(-22.7498686970069,-12.2787384750742,
12.));
#181146=CARTESIAN_POINT('Ctrl Pts',(-22.764938010105,-12.3025628601792,
12.));
#181147=CARTESIAN_POINT('Ctrl Pts',(-22.7799908974768,-12.3264788926075,
12.));
#181148=CARTESIAN_POINT('Ctrl Pts',(-22.795027221673,-12.3504864740319,
12.));
#181149=CARTESIAN_POINT('Ctrl Pts',(-22.81004690224,-12.374585536673,12.));
#181150=CARTESIAN_POINT('Ctrl Pts',(-22.8220493007173,-12.3939379378998,
12.));
#181151=CARTESIAN_POINT('Ctrl Pts',(-22.8310435872748,-12.4084933766346,
12.));
#181152=CARTESIAN_POINT('Ctrl Pts',(-22.8370364396459,-12.418215285186,
12.));
#181153=CARTESIAN_POINT('Ctrl Pts',(-22.8400320311649,-12.4230808101438,
12.));
#181154=CARTESIAN_POINT('',(-22.1787195904339,-13.5685075571671,12.));
#181155=CARTESIAN_POINT('Origin',(0.,0.,12.));
#181156=CARTESIAN_POINT('',(-18.5896416359912,-12.7689476255363,12.));
#181157=CARTESIAN_POINT('Ctrl Pts',(-22.1787195904339,-13.5685075571671,
12.));
#181158=CARTESIAN_POINT('Ctrl Pts',(-22.1730081264608,-13.5683460612942,
12.));
#181159=CARTESIAN_POINT('Ctrl Pts',(-22.1615922805008,-13.5680170531805,
12.));
#181160=CARTESIAN_POINT('Ctrl Pts',(-22.1444897575194,-13.5675054919061,
12.));
#181161=CARTESIAN_POINT('Ctrl Pts',(-22.1217288871975,-13.5667873105359,
12.));
#181162=CARTESIAN_POINT('Ctrl Pts',(-22.0933486464593,-13.5658294169284,
12.));
#181163=CARTESIAN_POINT('Ctrl Pts',(-22.0650393089609,-13.5648113689033,
12.));
#181164=CARTESIAN_POINT('Ctrl Pts',(-22.0368009736295,-13.5637332022473,
12.));
#181165=CARTESIAN_POINT('Ctrl Pts',(-22.0086337943449,-13.5625949868333,
12.));
#181166=CARTESIAN_POINT('Ctrl Pts',(-21.9805379899168,-13.5613968357561,
12.));
#181167=CARTESIAN_POINT('Ctrl Pts',(-21.9525138592813,-13.5601389185257,
12.));
#181168=CARTESIAN_POINT('Ctrl Pts',(-21.9245617765769,-13.5588214586604,
12.));
#181169=CARTESIAN_POINT('Ctrl Pts',(-21.8966821688824,-13.5574447178424,
12.));
#181170=CARTESIAN_POINT('Ctrl Pts',(-21.8688754989365,-13.5560089839385,
12.));
#181171=CARTESIAN_POINT('Ctrl Pts',(-21.8411422456075,-13.5545145573031,
12.));
#181172=CARTESIAN_POINT('Ctrl Pts',(-21.8134828857967,-13.5529617381573,
12.));
#181173=CARTESIAN_POINT('Ctrl Pts',(-21.7858978745865,-13.551350812725,
12.));
#181174=CARTESIAN_POINT('Ctrl Pts',(-21.7583876294554,-13.5496820422211,
12.));
#181175=CARTESIAN_POINT('Ctrl Pts',(-21.7309525412281,-13.5479556704481,
12.));
#181176=CARTESIAN_POINT('Ctrl Pts',(-21.7035929822955,-13.5461719295048,
12.));
#181177=CARTESIAN_POINT('Ctrl Pts',(-21.6763093157699,-13.5443310461526,
12.));
#181178=CARTESIAN_POINT('Ctrl Pts',(-21.6491019044648,-13.5424332480699,
12.));
#181179=CARTESIAN_POINT('Ctrl Pts',(-21.6219711193946,-13.5404787697792,
12.));
#181180=CARTESIAN_POINT('Ctrl Pts',(-21.5949173499013,-13.5384678597195,
12.));
#181181=CARTESIAN_POINT('Ctrl Pts',(-21.5679410019001,-13.536400779028,
12.));
#181182=CARTESIAN_POINT('Ctrl Pts',(-21.5410424932503,-13.5342777983215,
12.));
#181183=CARTESIAN_POINT('Ctrl Pts',(-21.5142222501666,-13.5320991952138,
12.));
#181184=CARTESIAN_POINT('Ctrl Pts',(-21.4874807030468,-13.5298652514355,
12.));
#181185=CARTESIAN_POINT('Ctrl Pts',(-21.4608182828697,-13.5275762503555,
12.));
#181186=CARTESIAN_POINT('Ctrl Pts',(-21.4342354165259,-13.5252324737802,
12.));
#181187=CARTESIAN_POINT('Ctrl Pts',(-21.4077325259324,-13.5228342013516,
12.));
#181188=CARTESIAN_POINT('Ctrl Pts',(-21.3813100304973,-13.5203817122504,
12.));
#181189=CARTESIAN_POINT('Ctrl Pts',(-21.3549683486222,-13.5178752862466,
12.));
#181190=CARTESIAN_POINT('Ctrl Pts',(-21.3287078996341,-13.5153152050555,
12.));
#181191=CARTESIAN_POINT('Ctrl Pts',(-21.3025291054235,-13.5127017534971,
12.));
#181192=CARTESIAN_POINT('Ctrl Pts',(-21.2764323924442,-13.5100352209205,
12.));
#181193=CARTESIAN_POINT('Ctrl Pts',(-21.250418192743,-13.5073159019452,
12.));
#181194=CARTESIAN_POINT('Ctrl Pts',(-21.2244869429332,-13.5045440957404,
12.));
#181195=CARTESIAN_POINT('Ctrl Pts',(-21.1986390835828,-13.5017201056088,
12.));
#181196=CARTESIAN_POINT('Ctrl Pts',(-21.1728750584175,-13.4988442384491,
12.));
#181197=CARTESIAN_POINT('Ctrl Pts',(-21.1471953136209,-13.4959168042934,
12.));
#181198=CARTESIAN_POINT('Ctrl Pts',(-21.1216002970207,-13.4929381157778,
12.));
#181199=CARTESIAN_POINT('Ctrl Pts',(-21.0960904575046,-13.4899084877717,
12.));
#181200=CARTESIAN_POINT('Ctrl Pts',(-21.0706662455199,-13.4868282377191,
12.));
#181201=CARTESIAN_POINT('Ctrl Pts',(-21.0453281134245,-13.4836976858912,
12.));
#181202=CARTESIAN_POINT('Ctrl Pts',(-21.0200765158884,-13.4805171556822,
12.));
#181203=CARTESIAN_POINT('Ctrl Pts',(-20.9949119102592,-13.4772869738879,
12.));
#181204=CARTESIAN_POINT('Ctrl Pts',(-20.9698347569477,-13.4740074710086,
12.));
#181205=CARTESIAN_POINT('Ctrl Pts',(-20.9448455197557,-13.4706789815166,
12.));
#181206=CARTESIAN_POINT('Ctrl Pts',(-20.9199446657583,-13.4673018437717,
12.));
#181207=CARTESIAN_POINT('Ctrl Pts',(-20.8951326652158,-13.4638763999725,
12.));
#181208=CARTESIAN_POINT('Ctrl Pts',(-20.8704099914641,-13.4604029960983,
12.));
#181209=CARTESIAN_POINT('Ctrl Pts',(-20.8457771208083,-13.4568819818631,
12.));
#181210=CARTESIAN_POINT('Ctrl Pts',(-20.821234532398,-13.4533137106667,
12.));
#181211=CARTESIAN_POINT('Ctrl Pts',(-20.7967827081228,-13.4496985395637,
12.));
#181212=CARTESIAN_POINT('Ctrl Pts',(-20.7724221327609,-13.4460368293689,
12.));
#181213=CARTESIAN_POINT('Ctrl Pts',(-20.7481532941014,-13.4423289447561,
12.));
#181214=CARTESIAN_POINT('Ctrl Pts',(-20.7239766830675,-13.4385752543663,
12.));
#181215=CARTESIAN_POINT('Ctrl Pts',(-20.6998927938288,-13.4347761309154,
12.));
#181216=CARTESIAN_POINT('Ctrl Pts',(-20.6759021239102,-13.4309319513119,
12.));
#181217=CARTESIAN_POINT('Ctrl Pts',(-20.6520051742868,-13.427043096765,
12.));
#181218=CARTESIAN_POINT('Ctrl Pts',(-20.6282024494234,-13.4231099528178,
12.));
#181219=CARTESIAN_POINT('Ctrl Pts',(-20.6044944573151,-13.4191329093932,
12.));
#181220=CARTESIAN_POINT('Ctrl Pts',(-20.5808817095155,-13.4151123608411,
12.));
#181221=CARTESIAN_POINT('Ctrl Pts',(-20.557364721164,-13.4110487059912,
12.));
#181222=CARTESIAN_POINT('Ctrl Pts',(-20.5339440109958,-13.4069423482076,
12.));
#181223=CARTESIAN_POINT('Ctrl Pts',(-20.5106201013755,-13.4027936954529,
12.));
#181224=CARTESIAN_POINT('Ctrl Pts',(-20.4873935184041,-13.3986031603716,
12.));
#181225=CARTESIAN_POINT('Ctrl Pts',(-20.4642647920038,-13.3943711603739,
12.));
#181226=CARTESIAN_POINT('Ctrl Pts',(-20.4412344560007,-13.3900981177254,
12.));
#181227=CARTESIAN_POINT('Ctrl Pts',(-20.4183030482002,-13.3857844596387,
12.));
#181228=CARTESIAN_POINT('Ctrl Pts',(-20.3954711104505,-13.3814306183721,
12.));
#181229=CARTESIAN_POINT('Ctrl Pts',(-20.3727391887187,-13.377037031319,
12.));
#181230=CARTESIAN_POINT('Ctrl Pts',(-20.3501078331818,-13.3726041410869,
12.));
#181231=CARTESIAN_POINT('Ctrl Pts',(-20.3275775983032,-13.3681323955828,
12.));
#181232=CARTESIAN_POINT('Ctrl Pts',(-20.3051490429049,-13.3636222481017,
12.));
#181233=CARTESIAN_POINT('Ctrl Pts',(-20.2828227302337,-13.3590741574194,
12.));
#181234=CARTESIAN_POINT('Ctrl Pts',(-20.2605992280117,-13.3544885878886,
12.));
#181235=CARTESIAN_POINT('Ctrl Pts',(-20.2384791085354,-13.3498660095382,
12.));
#181236=CARTESIAN_POINT('Ctrl Pts',(-20.2164629487855,-13.3452068981763,
12.));
#181237=CARTESIAN_POINT('Ctrl Pts',(-20.1945513305233,-13.3405117354969,
12.));
#181238=CARTESIAN_POINT('Ctrl Pts',(-20.1727448403818,-13.3357810091903,
12.));
#181239=CARTESIAN_POINT('Ctrl Pts',(-20.1510440699477,-13.3310152130565,
12.));
#181240=CARTESIAN_POINT('Ctrl Pts',(-20.1294496158405,-13.3262148471228,
12.));
#181241=CARTESIAN_POINT('Ctrl Pts',(-20.1079620798377,-13.3213804177588,
12.));
#181242=CARTESIAN_POINT('Ctrl Pts',(-20.0865820689883,-13.3165124377963,
12.));
#181243=CARTESIAN_POINT('Ctrl Pts',(-20.0653101957188,-13.3116114266514,
12.));
#181244=CARTESIAN_POINT('Ctrl Pts',(-20.0441470779345,-13.3066779104515,
12.));
#181245=CARTESIAN_POINT('Ctrl Pts',(-20.023093339104,-13.3017124221639,
12.));
#181246=CARTESIAN_POINT('Ctrl Pts',(-20.0021496083742,-13.296715501731,
12.));
#181247=CARTESIAN_POINT('Ctrl Pts',(-19.9813165207174,-13.2916876962098,
12.));
#181248=CARTESIAN_POINT('Ctrl Pts',(-19.9605947170589,-13.2866295599152,
12.));
#181249=CARTESIAN_POINT('Ctrl Pts',(-19.9399848444019,-13.2815416545663,
12.));
#181250=CARTESIAN_POINT('Ctrl Pts',(-19.9194875559419,-13.2764245494354,
12.));
#181251=CARTESIAN_POINT('Ctrl Pts',(-19.8991035111739,-13.2712788215015,
12.));
#181252=CARTESIAN_POINT('Ctrl Pts',(-19.8788333760571,-13.2661050556128,
12.));
#181253=CARTESIAN_POINT('Ctrl Pts',(-19.8586778231711,-13.2609038446525,
12.));
#181254=CARTESIAN_POINT('Ctrl Pts',(-19.8386375318632,-13.2556757897085,
12.));
#181255=CARTESIAN_POINT('Ctrl Pts',(-19.8187131883919,-13.2504215002458,
12.));
#181256=CARTESIAN_POINT('Ctrl Pts',(-19.7989054860501,-13.2451415942809,
12.));
#181257=CARTESIAN_POINT('Ctrl Pts',(-19.7792151253297,-13.239836698568,
12.));
#181258=CARTESIAN_POINT('Ctrl Pts',(-19.7596428141176,-13.2345074487968,
12.));
#181259=CARTESIAN_POINT('Ctrl Pts',(-19.7401892678701,-13.2291544897902,
12.));
#181260=CARTESIAN_POINT('Ctrl Pts',(-19.7208552097867,-13.2237784757065,
12.));
#181261=CARTESIAN_POINT('Ctrl Pts',(-19.7016413709678,-13.2183800702431,
12.));
#181262=CARTESIAN_POINT('Ctrl Pts',(-19.6825484905812,-13.2129599468478,
12.));
#181263=CARTESIAN_POINT('Ctrl Pts',(-19.6635773160924,-13.2075187889522,
12.));
#181264=CARTESIAN_POINT('Ctrl Pts',(-19.6447286034764,-13.202057290206,
12.));
#181265=CARTESIAN_POINT('Ctrl Pts',(-19.6260031174244,-13.196576154715,
12.));
#181266=CARTESIAN_POINT('Ctrl Pts',(-19.6074016315421,-13.1910760972818,
12.));
#181267=CARTESIAN_POINT('Ctrl Pts',(-19.5889249285352,-13.1855578436479,
12.));
#181268=CARTESIAN_POINT('Ctrl Pts',(-19.5705738004682,-13.1800221307682,
12.));
#181269=CARTESIAN_POINT('Ctrl Pts',(-19.5523490490254,-13.1744697070918,
12.));
#181270=CARTESIAN_POINT('Ctrl Pts',(-19.5342514857564,-13.1689013328432,
12.));
#181271=CARTESIAN_POINT('Ctrl Pts',(-19.5162819323207,-13.1633177803097,
12.));
#181272=CARTESIAN_POINT('Ctrl Pts',(-19.498441220707,-13.1577198341238,
12.));
#181273=CARTESIAN_POINT('Ctrl Pts',(-19.4807301935256,-13.1521082915846,
12.));
#181274=CARTESIAN_POINT('Ctrl Pts',(-19.463149704325,-13.1464839629966,
12.));
#181275=CARTESIAN_POINT('Ctrl Pts',(-19.4457006178875,-13.140847672006,
12.));
#181276=CARTESIAN_POINT('Ctrl Pts',(-19.4283838105265,-13.1352002559439,
12.));
#181277=CARTESIAN_POINT('Ctrl Pts',(-19.4112001703561,-13.1295425661635,
12.));
#181278=CARTESIAN_POINT('Ctrl Pts',(-19.3941505976267,-13.1238754684177,
12.));
#181279=CARTESIAN_POINT('Ctrl Pts',(-19.3772360051093,-13.118199843271,
12.));
#181280=CARTESIAN_POINT('Ctrl Pts',(-19.3604573184516,-13.1125165865021,
12.));
#181281=CARTESIAN_POINT('Ctrl Pts',(-19.3438154765395,-13.1068266095186,
12.));
#181282=CARTESIAN_POINT('Ctrl Pts',(-19.3273114318268,-13.1011308397592,
12.));
#181283=CARTESIAN_POINT('Ctrl Pts',(-19.3109461507358,-13.095430221148,
12.));
#181284=CARTESIAN_POINT('Ctrl Pts',(-19.2947206141246,-13.0897257145969,
12.));
#181285=CARTESIAN_POINT('Ctrl Pts',(-19.2786358177198,-13.0840182984949,
12.));
#181286=CARTESIAN_POINT('Ctrl Pts',(-19.2626927725596,-13.0783089692118,
12.));
#181287=CARTESIAN_POINT('Ctrl Pts',(-19.2468925053988,-13.0725987415856,
12.));
#181288=CARTESIAN_POINT('Ctrl Pts',(-19.2312360592031,-13.0668886494791,
12.));
#181289=CARTESIAN_POINT('Ctrl Pts',(-19.2157244937141,-13.0611797463913,
12.));
#181290=CARTESIAN_POINT('Ctrl Pts',(-19.2003588859771,-13.0554731060537,
12.));
#181291=CARTESIAN_POINT('Ctrl Pts',(-19.1851403308825,-13.0497698230442,
12.));
#181292=CARTESIAN_POINT('Ctrl Pts',(-19.1700699416625,-13.0440710133775,
12.));
#181293=CARTESIAN_POINT('Ctrl Pts',(-19.1551488505233,-13.0383778152072,
12.));
#181294=CARTESIAN_POINT('Ctrl Pts',(-19.1403782093389,-13.0326913895841,
12.));
#181295=CARTESIAN_POINT('Ctrl Pts',(-19.1257591903099,-13.0270129211976,
12.));
#181296=CARTESIAN_POINT('Ctrl Pts',(-19.1112929866308,-13.0213436191326,
12.));
#181297=CARTESIAN_POINT('Ctrl Pts',(-19.0969808131226,-13.0156847176093,
12.));
#181298=CARTESIAN_POINT('Ctrl Pts',(-19.0828239070482,-13.0100374768785,
12.));
#181299=CARTESIAN_POINT('Ctrl Pts',(-19.0688235289437,-13.0044031841381,
12.));
#181300=CARTESIAN_POINT('Ctrl Pts',(-19.0549809634355,-12.9987831544502,
12.));
#181301=CARTESIAN_POINT('Ctrl Pts',(-19.0412975200398,-12.9931787316515,
12.));
#181302=CARTESIAN_POINT('Ctrl Pts',(-19.0277745339908,-12.9875912893003,
12.));
#181303=CARTESIAN_POINT('Ctrl Pts',(-19.0144133673348,-12.9820222318716,
12.));
#181304=CARTESIAN_POINT('Ctrl Pts',(-19.0012154099791,-12.9764729959205,
12.));
#181305=CARTESIAN_POINT('Ctrl Pts',(-18.9881820807586,-12.9709450512747,
12.));
#181306=CARTESIAN_POINT('Ctrl Pts',(-18.9753148284475,-12.9654399021869,
12.));
#181307=CARTESIAN_POINT('Ctrl Pts',(-18.9626151329229,-12.9599590886319,
12.));
#181308=CARTESIAN_POINT('Ctrl Pts',(-18.9500845064715,-12.9545041877377,
12.));
#181309=CARTESIAN_POINT('Ctrl Pts',(-18.9377244950435,-12.9490768151821,
12.));
#181310=CARTESIAN_POINT('Ctrl Pts',(-18.9255366795195,-12.9436786266105,
12.));
#181311=CARTESIAN_POINT('Ctrl Pts',(-18.9135226769465,-12.9383113190375,
12.));
#181312=CARTESIAN_POINT('Ctrl Pts',(-18.9016841423403,-12.9329766328185,
12.));
#181313=CARTESIAN_POINT('Ctrl Pts',(-18.8900227704889,-12.9276763536373,
12.));
#181314=CARTESIAN_POINT('Ctrl Pts',(-18.8785402977527,-12.9224123144982,
12.));
#181315=CARTESIAN_POINT('Ctrl Pts',(-18.8672385038326,-12.9171863977045,
12.));
#181316=CARTESIAN_POINT('Ctrl Pts',(-18.8561192136198,-12.9120005369063,
12.));
#181317=CARTESIAN_POINT('Ctrl Pts',(-18.8451842990984,-12.9068567191854,
12.));
#181318=CARTESIAN_POINT('Ctrl Pts',(-18.834435681259,-12.9017569871738,
12.));
#181319=CARTESIAN_POINT('Ctrl Pts',(-18.8238753319129,-12.8967034410755,
12.));
#181320=CARTESIAN_POINT('Ctrl Pts',(-18.813505275782,-12.8916982409935,
12.));
#181321=CARTESIAN_POINT('Ctrl Pts',(-18.8033275941943,-12.8867436109546,
12.));
#181322=CARTESIAN_POINT('Ctrl Pts',(-18.7933444285868,-12.8818418427475,
12.));
#181323=CARTESIAN_POINT('Ctrl Pts',(-18.7835579840477,-12.8769952998095,
12.));
#181324=CARTESIAN_POINT('Ctrl Pts',(-18.7739705329022,-12.872206421181,
12.));
#181325=CARTESIAN_POINT('Ctrl Pts',(-18.7645844169564,-12.8674777239653,
12.));
#181326=CARTESIAN_POINT('Ctrl Pts',(-18.7554020493887,-12.8628118054171,
12.));
#181327=CARTESIAN_POINT('Ctrl Pts',(-18.7464259171251,-12.8582113455646,
12.));
#181328=CARTESIAN_POINT('Ctrl Pts',(-18.7376585820854,-12.8536791086316,
12.));
#181329=CARTESIAN_POINT('Ctrl Pts',(-18.7291026886554,-12.8492179511591,
12.));
#181330=CARTESIAN_POINT('Ctrl Pts',(-18.7207609737702,-12.8448308329494,
12.));
#181331=CARTESIAN_POINT('Ctrl Pts',(-18.7126362754445,-12.8405208263431,
12.));
#181332=CARTESIAN_POINT('Ctrl Pts',(-18.7047315436294,-12.8362911280361,
12.));
#181333=CARTESIAN_POINT('Ctrl Pts',(-18.6970498410172,-12.8321450599789,
12.));
#181334=CARTESIAN_POINT('Ctrl Pts',(-18.6895943376171,-12.8280860635231,
12.));
#181335=CARTESIAN_POINT('Ctrl Pts',(-18.6823683094139,-12.8241176980017,
12.));
#181336=CARTESIAN_POINT('Ctrl Pts',(-18.6753751301092,-12.8202436318474,
12.));
#181337=CARTESIAN_POINT('Ctrl Pts',(-18.6686182952799,-12.8164676687362,
12.));
#181338=CARTESIAN_POINT('Ctrl Pts',(-18.6621014624746,-12.8127937909631,
12.));
#181339=CARTESIAN_POINT('Ctrl Pts',(-18.6558284825773,-12.8092261933858,
12.));
#181340=CARTESIAN_POINT('Ctrl Pts',(-18.6498034438987,-12.805769331162,
12.));
#181341=CARTESIAN_POINT('Ctrl Pts',(-18.6440306327456,-12.8024278770152,
12.));
#181342=CARTESIAN_POINT('Ctrl Pts',(-18.63851447924,-12.7992066625264,12.));
#181343=CARTESIAN_POINT('Ctrl Pts',(-18.6332595057006,-12.7961106222251,
12.));
#181344=CARTESIAN_POINT('Ctrl Pts',(-18.6282702819371,-12.7931447451555,
12.));
#181345=CARTESIAN_POINT('Ctrl Pts',(-18.6235516265575,-12.7903142925234,
12.));
#181346=CARTESIAN_POINT('Ctrl Pts',(-18.6191087624752,-12.7876249657834,
12.));
#181347=CARTESIAN_POINT('Ctrl Pts',(-18.6149475565188,-12.7850831657901,
12.));
#181348=CARTESIAN_POINT('Ctrl Pts',(-18.6110744826219,-12.7826959526925,
12.));
#181349=CARTESIAN_POINT('Ctrl Pts',(-18.6074961535723,-12.7804705387658,
12.));
#181350=CARTESIAN_POINT('Ctrl Pts',(-18.6042190183704,-12.7784139605066,
12.));
#181351=CARTESIAN_POINT('Ctrl Pts',(-18.6012488486709,-12.7765325225081,
12.));
#181352=CARTESIAN_POINT('Ctrl Pts',(-18.598591752595,-12.7748328937638,
12.));
#181353=CARTESIAN_POINT('Ctrl Pts',(-18.5962551167772,-12.7733231262108,
12.));
#181354=CARTESIAN_POINT('Ctrl Pts',(-18.5942490615407,-12.7720142287172,
12.));
#181355=CARTESIAN_POINT('Ctrl Pts',(-18.5925859134579,-12.7709195951156,
12.));
#181356=CARTESIAN_POINT('Ctrl Pts',(-18.5912775137806,-12.7700520897173,
12.));
#181357=CARTESIAN_POINT('Ctrl Pts',(-18.5903328777227,-12.7694215127919,
12.));
#181358=CARTESIAN_POINT('Ctrl Pts',(-18.589871621843,-12.769110348199,12.));
#181359=CARTESIAN_POINT('Ctrl Pts',(-18.5896919669165,-12.768986426692,
12.));
#181360=CARTESIAN_POINT('Ctrl Pts',(-18.5896460962964,-12.7689524524483,
12.));
#181361=CARTESIAN_POINT('Ctrl Pts',(-18.5896416359912,-12.7689476255363,
12.));
#181362=CARTESIAN_POINT('',(-18.1294424696716,-12.4528436808172,12.));
#181363=CARTESIAN_POINT('',(-8.86099361848466,-6.08648437878338,12.));
#181364=CARTESIAN_POINT('',(-17.4407513054162,-12.572596943457,12.));
#181365=CARTESIAN_POINT('Origin',(-17.846350172984,-12.8649829188862,12.));
#181366=CARTESIAN_POINT('',(-16.6581946899465,-13.5924445804218,12.));
#181367=CARTESIAN_POINT('Origin',(-6.37232247690086E-13,-4.50593605254675E-13,
12.));
#181368=CARTESIAN_POINT('',(-16.7207683102834,-14.2886635873976,12.));
#181369=CARTESIAN_POINT('Origin',(-17.0455945664569,-13.9085479427572,12.));
#181370=CARTESIAN_POINT('',(-17.1452095830633,-14.6513681262571,12.));
#181371=CARTESIAN_POINT('',(-8.57260479153162,-7.32568406312855,12.));
#181372=CARTESIAN_POINT('',(-18.8464468996588,-17.9112098770111,12.));
#181373=CARTESIAN_POINT('Ctrl Pts',(-17.1452095830633,-14.6513681262571,
12.));
#181374=CARTESIAN_POINT('Ctrl Pts',(-17.1452153999142,-14.651371185284,
12.));
#181375=CARTESIAN_POINT('Ctrl Pts',(-17.1452600887039,-14.6514066997188,
12.));
#181376=CARTESIAN_POINT('Ctrl Pts',(-17.1454262858045,-14.6515481598057,
12.));
#181377=CARTESIAN_POINT('Ctrl Pts',(-17.1458462295273,-14.65191316345,12.));
#181378=CARTESIAN_POINT('Ctrl Pts',(-17.1466998098673,-14.6526624064978,
12.));
#181379=CARTESIAN_POINT('Ctrl Pts',(-17.1478763944909,-14.6537016966188,
12.));
#181380=CARTESIAN_POINT('Ctrl Pts',(-17.1493641837556,-14.6550248622813,
12.));
#181381=CARTESIAN_POINT('Ctrl Pts',(-17.1511476869495,-14.6566237952435,
12.));
#181382=CARTESIAN_POINT('Ctrl Pts',(-17.1532107762719,-14.6584900555301,
12.));
#181383=CARTESIAN_POINT('Ctrl Pts',(-17.1555401986403,-14.660616716964,
12.));
#181384=CARTESIAN_POINT('Ctrl Pts',(-17.1581262646789,-14.662998728599,
12.));
#181385=CARTESIAN_POINT('Ctrl Pts',(-17.1609609517369,-14.6656319165057,
12.));
#181386=CARTESIAN_POINT('Ctrl Pts',(-17.1640366762304,-14.6685123374424,
12.));
#181387=CARTESIAN_POINT('Ctrl Pts',(-17.1673449723019,-14.6716355833321,
12.));
#181388=CARTESIAN_POINT('Ctrl Pts',(-17.1708771619129,-14.6749971333867,
12.));
#181389=CARTESIAN_POINT('Ctrl Pts',(-17.1746247499057,-14.6785925615676,
12.));
#181390=CARTESIAN_POINT('Ctrl Pts',(-17.1785800350827,-14.6824178576167,
12.));
#181391=CARTESIAN_POINT('Ctrl Pts',(-17.182736158472,-14.6864694522319,
12.));
#181392=CARTESIAN_POINT('Ctrl Pts',(-17.1870867909918,-14.6907440526958,
12.));
#181393=CARTESIAN_POINT('Ctrl Pts',(-17.1916259308416,-14.6952385361706,
12.));
#181394=CARTESIAN_POINT('Ctrl Pts',(-17.1963476411694,-14.699949811582,
12.));
#181395=CARTESIAN_POINT('Ctrl Pts',(-17.2012461084268,-14.7048748502663,
12.));
#181396=CARTESIAN_POINT('Ctrl Pts',(-17.2063157097316,-14.7100107213586,
12.));
#181397=CARTESIAN_POINT('Ctrl Pts',(-17.2115510835988,-14.7153546289338,
12.));
#181398=CARTESIAN_POINT('Ctrl Pts',(-17.2169471814255,-14.7209039390326,
12.));
#181399=CARTESIAN_POINT('Ctrl Pts',(-17.2224992099666,-14.7266561494282,
12.));
#181400=CARTESIAN_POINT('Ctrl Pts',(-17.2282025904314,-14.7326088681163,
12.));
#181401=CARTESIAN_POINT('Ctrl Pts',(-17.2340529062077,-14.7387597858117,
12.));
#181402=CARTESIAN_POINT('Ctrl Pts',(-17.2400458713566,-14.7451066593793,
12.));
#181403=CARTESIAN_POINT('Ctrl Pts',(-17.2461773413289,-14.7516473175125,
12.));
#181404=CARTESIAN_POINT('Ctrl Pts',(-17.2524433146837,-14.7583796616617,
12.));
#181405=CARTESIAN_POINT('Ctrl Pts',(-17.2588399401464,-14.7653016697589,
12.));
#181406=CARTESIAN_POINT('Ctrl Pts',(-17.2653635155317,-14.7724113956728,
12.));
#181407=CARTESIAN_POINT('Ctrl Pts',(-17.2720104735192,-14.7797069617802,
12.));
#181408=CARTESIAN_POINT('Ctrl Pts',(-17.278777370485,-14.787186553128,12.));
#181409=CARTESIAN_POINT('Ctrl Pts',(-17.28566087332,-14.7948484105253,12.));
#181410=CARTESIAN_POINT('Ctrl Pts',(-17.2926577496519,-14.8026908254281,
12.));
#181411=CARTESIAN_POINT('Ctrl Pts',(-17.2997648661483,-14.8107121391038,
12.));
#181412=CARTESIAN_POINT('Ctrl Pts',(-17.3069791853705,-14.8189107410161,
12.));
#181413=CARTESIAN_POINT('Ctrl Pts',(-17.3142977632656,-14.8272850675375,
12.));
#181414=CARTESIAN_POINT('Ctrl Pts',(-17.3217177462096,-14.8358336004193,
12.));
#181415=CARTESIAN_POINT('Ctrl Pts',(-17.3292363662601,-14.8445548643505,
12.));
#181416=CARTESIAN_POINT('Ctrl Pts',(-17.336850936485,-14.8534474245433,
12.));
#181417=CARTESIAN_POINT('Ctrl Pts',(-17.3445588463477,-14.8625098843419,
12.));
#181418=CARTESIAN_POINT('Ctrl Pts',(-17.3523575568648,-14.8717408826958,
12.));
#181419=CARTESIAN_POINT('Ctrl Pts',(-17.3602445978163,-14.8811390927424,
12.));
#181420=CARTESIAN_POINT('Ctrl Pts',(-17.3682175653236,-14.8907032205789,
12.));
#181421=CARTESIAN_POINT('Ctrl Pts',(-17.3762741193075,-14.9004320039609,
12.));
#181422=CARTESIAN_POINT('Ctrl Pts',(-17.3844119809823,-14.9103242110057,
12.));
#181423=CARTESIAN_POINT('Ctrl Pts',(-17.3926289303987,-14.9203786389343,
12.));
#181424=CARTESIAN_POINT('Ctrl Pts',(-17.400922804075,-14.9305941128758,
12.));
#181425=CARTESIAN_POINT('Ctrl Pts',(-17.4092914926071,-14.940969484645,
12.));
#181426=CARTESIAN_POINT('Ctrl Pts',(-17.4177329382827,-14.9515036315142,
12.));
#181427=CARTESIAN_POINT('Ctrl Pts',(-17.4262451327088,-14.9621954549825,
12.));
#181428=CARTESIAN_POINT('Ctrl Pts',(-17.4348261151395,-14.973043879945,
12.));
#181429=CARTESIAN_POINT('Ctrl Pts',(-17.4434739707773,-14.9840478538357,
12.));
#181430=CARTESIAN_POINT('Ctrl Pts',(-17.4521868291005,-14.9952063457779,
12.));
#181431=CARTESIAN_POINT('Ctrl Pts',(-17.4609628621419,-15.0065183456922,
12.));
#181432=CARTESIAN_POINT('Ctrl Pts',(-17.4698002829357,-15.0179828635087,
12.));
#181433=CARTESIAN_POINT('Ctrl Pts',(-17.4786973441417,-15.029598928488,
12.));
#181434=CARTESIAN_POINT('Ctrl Pts',(-17.4876523366178,-15.0413655884993,
12.));
#181435=CARTESIAN_POINT('Ctrl Pts',(-17.4966635880246,-15.0532819093085,
12.));
#181436=CARTESIAN_POINT('Ctrl Pts',(-17.5057294613877,-15.0653469738307,
12.));
#181437=CARTESIAN_POINT('Ctrl Pts',(-17.5148483539687,-15.0775598815749,
12.));
#181438=CARTESIAN_POINT('Ctrl Pts',(-17.5240186961791,-15.0899197481082,
12.));
#181439=CARTESIAN_POINT('Ctrl Pts',(-17.5332389504829,-15.1024257045033,
12.));
#181440=CARTESIAN_POINT('Ctrl Pts',(-17.5425076102963,-15.1150768967728,
12.));
#181441=CARTESIAN_POINT('Ctrl Pts',(-17.5518231989117,-15.1278724853138,
12.));
#181442=CARTESIAN_POINT('Ctrl Pts',(-17.5611842686192,-15.1408116444876,
12.));
#181443=CARTESIAN_POINT('Ctrl Pts',(-17.5705893998029,-15.1538935621714,
12.));
#181444=CARTESIAN_POINT('Ctrl Pts',(-17.580037200054,-15.1671174393137,
12.));
#181445=CARTESIAN_POINT('Ctrl Pts',(-17.5895263032595,-15.1804824894605,
12.));
#181446=CARTESIAN_POINT('Ctrl Pts',(-17.5990553687599,-15.1939879383268,
12.));
#181447=CARTESIAN_POINT('Ctrl Pts',(-17.60862308065,-15.2076330234686,12.));
#181448=CARTESIAN_POINT('Ctrl Pts',(-17.6182281470468,-15.2214169939199,
12.));
#181449=CARTESIAN_POINT('Ctrl Pts',(-17.6278692993764,-15.2353391098366,
12.));
#181450=CARTESIAN_POINT('Ctrl Pts',(-17.6375452916369,-15.2493986421092,
12.));
#181451=CARTESIAN_POINT('Ctrl Pts',(-17.6472548997328,-15.2635948720292,
12.));
#181452=CARTESIAN_POINT('Ctrl Pts',(-17.6569969209,-15.2779270910239,12.));
#181453=CARTESIAN_POINT('Ctrl Pts',(-17.6667701731041,-15.2923946003598,
12.));
#181454=CARTESIAN_POINT('Ctrl Pts',(-17.676573494456,-15.3069967108501,
12.));
#181455=CARTESIAN_POINT('Ctrl Pts',(-17.6864057426052,-15.3217327425338,
12.));
#181456=CARTESIAN_POINT('Ctrl Pts',(-17.6962657941983,-15.3366020244066,
12.));
#181457=CARTESIAN_POINT('Ctrl Pts',(-17.7061525444042,-15.351603894206,
12.));
#181458=CARTESIAN_POINT('Ctrl Pts',(-17.7160649064206,-15.3667376981699,
12.));
#181459=CARTESIAN_POINT('Ctrl Pts',(-17.7260018109924,-15.3820027907967,
12.));
#181460=CARTESIAN_POINT('Ctrl Pts',(-17.735962205915,-15.3973985345802,
12.));
#181461=CARTESIAN_POINT('Ctrl Pts',(-17.7459450555812,-15.4129242997837,
12.));
#181462=CARTESIAN_POINT('Ctrl Pts',(-17.7559493405881,-15.4285794642668,
12.));
#181463=CARTESIAN_POINT('Ctrl Pts',(-17.7659740573265,-15.4443634132869,
12.));
#181464=CARTESIAN_POINT('Ctrl Pts',(-17.7760182175815,-15.4602755393017,
12.));
#181465=CARTESIAN_POINT('Ctrl Pts',(-17.786080848122,-15.4763152417497,
12.));
#181466=CARTESIAN_POINT('Ctrl Pts',(-17.7961609903148,-15.4924819268517,
12.));
#181467=CARTESIAN_POINT('Ctrl Pts',(-17.8062576997952,-15.5087750074718,
12.));
#181468=CARTESIAN_POINT('Ctrl Pts',(-17.8163700461256,-15.5251939029552,
12.));
#181469=CARTESIAN_POINT('Ctrl Pts',(-17.8264971124607,-15.541738038964,
12.));
#181470=CARTESIAN_POINT('Ctrl Pts',(-17.8366379952085,-15.5584068472982,
12.));
#181471=CARTESIAN_POINT('Ctrl Pts',(-17.8467918036987,-15.5751997657163,
12.));
#181472=CARTESIAN_POINT('Ctrl Pts',(-17.8569576599006,-15.5921162378192,
12.));
#181473=CARTESIAN_POINT('Ctrl Pts',(-17.8671346981394,-15.609155712921,
12.));
#181474=CARTESIAN_POINT('Ctrl Pts',(-17.8773220648125,-15.6263176459108,
12.));
#181475=CARTESIAN_POINT('Ctrl Pts',(-17.8875189181091,-15.6436014971084,
12.));
#181476=CARTESIAN_POINT('Ctrl Pts',(-17.897724427724,-15.661006732103,12.));
#181477=CARTESIAN_POINT('Ctrl Pts',(-17.9079377746111,-15.678532821646,
12.));
#181478=CARTESIAN_POINT('Ctrl Pts',(-17.9181581507455,-15.6961792415522,
12.));
#181479=CARTESIAN_POINT('Ctrl Pts',(-17.9283847588836,-15.7139454725838,
12.));
#181480=CARTESIAN_POINT('Ctrl Pts',(-17.9386168123262,-15.7318310003335,
12.));
#181481=CARTESIAN_POINT('Ctrl Pts',(-17.9488535346781,-15.749835315086,
12.));
#181482=CARTESIAN_POINT('Ctrl Pts',(-17.9590941596242,-15.7679579117077,
12.));
#181483=CARTESIAN_POINT('Ctrl Pts',(-17.9693379307303,-15.7861982895724,
12.));
#181484=CARTESIAN_POINT('Ctrl Pts',(-17.9795841012386,-15.8045559524676,
12.));
#181485=CARTESIAN_POINT('Ctrl Pts',(-17.9898319338664,-15.8230304084962,
12.));
#181486=CARTESIAN_POINT('Ctrl Pts',(-18.0000807006052,-15.8416211699679,
12.));
#181487=CARTESIAN_POINT('Ctrl Pts',(-18.0103296825205,-15.8603277532831,
12.));
#181488=CARTESIAN_POINT('Ctrl Pts',(-18.0205781695769,-15.8791496788682,
12.));
#181489=CARTESIAN_POINT('Ctrl Pts',(-18.0308254604636,-15.8980864711042,
12.));
#181490=CARTESIAN_POINT('Ctrl Pts',(-18.0410708624208,-15.9171376582436,
12.));
#181491=CARTESIAN_POINT('Ctrl Pts',(-18.0513136910691,-15.9363027723244,
12.));
#181492=CARTESIAN_POINT('Ctrl Pts',(-18.061553270236,-15.9555813490644,
12.));
#181493=CARTESIAN_POINT('Ctrl Pts',(-18.0717889317958,-15.9749729277846,
12.));
#181494=CARTESIAN_POINT('Ctrl Pts',(-18.0820200155236,-15.9944770513613,
12.));
#181495=CARTESIAN_POINT('Ctrl Pts',(-18.0922458689462,-16.014093266161,
12.));
#181496=CARTESIAN_POINT('Ctrl Pts',(-18.1024658471966,-16.0338211219693,
12.));
#181497=CARTESIAN_POINT('Ctrl Pts',(-18.112679312869,-16.0536601719126,
12.));
#181498=CARTESIAN_POINT('Ctrl Pts',(-18.1228856358751,-16.0736099723668,
12.));
#181499=CARTESIAN_POINT('Ctrl Pts',(-18.1330841933105,-16.0936700829112,
12.));
#181500=CARTESIAN_POINT('Ctrl Pts',(-18.1432743693235,-16.1138400662794,
12.));
#181501=CARTESIAN_POINT('Ctrl Pts',(-18.1534555549852,-16.1341194882988,
12.));
#181502=CARTESIAN_POINT('Ctrl Pts',(-18.1636271481615,-16.154507917826,
12.));
#181503=CARTESIAN_POINT('Ctrl Pts',(-18.1737885533849,-16.1750049266671,
12.));
#181504=CARTESIAN_POINT('Ctrl Pts',(-18.1839391817331,-16.1956100895073,
12.));
#181505=CARTESIAN_POINT('Ctrl Pts',(-18.1940784507229,-16.2163229838875,
12.));
#181506=CARTESIAN_POINT('Ctrl Pts',(-18.2042057842035,-16.2371431901638,
12.));
#181507=CARTESIAN_POINT('Ctrl Pts',(-18.2143206122529,-16.2580702914615,
12.));
#181508=CARTESIAN_POINT('Ctrl Pts',(-18.2244223710746,-16.2791038736223,
12.));
#181509=CARTESIAN_POINT('Ctrl Pts',(-18.2345105028982,-16.3002435251378,
12.));
#181510=CARTESIAN_POINT('Ctrl Pts',(-18.2445844558742,-16.3214888370987,
12.));
#181511=CARTESIAN_POINT('Ctrl Pts',(-18.2546436839608,-16.3428394031589,
12.));
#181512=CARTESIAN_POINT('Ctrl Pts',(-18.2646876468169,-16.3642948194868,
12.));
#181513=CARTESIAN_POINT('Ctrl Pts',(-18.2747158096934,-16.385854684708,
12.));
#181514=CARTESIAN_POINT('Ctrl Pts',(-18.2847276433309,-16.4075185998455,
12.));
#181515=CARTESIAN_POINT('Ctrl Pts',(-18.294722623851,-16.4292861682379,
12.));
#181516=CARTESIAN_POINT('Ctrl Pts',(-18.304700232686,-16.4511569955233,
12.));
#181517=CARTESIAN_POINT('Ctrl Pts',(-18.3146599565231,-16.4731306896441,
12.));
#181518=CARTESIAN_POINT('Ctrl Pts',(-18.3246012872469,-16.4952068608345,
12.));
#181519=CARTESIAN_POINT('Ctrl Pts',(-18.3345237218864,-16.5173851216045,
12.));
#181520=CARTESIAN_POINT('Ctrl Pts',(-18.34442676256,-16.5396650867139,12.));
#181521=CARTESIAN_POINT('Ctrl Pts',(-18.354309916433,-16.5620463731413,
12.));
#181522=CARTESIAN_POINT('Ctrl Pts',(-18.3641726955889,-16.5845286000217,
12.));
#181523=CARTESIAN_POINT('Ctrl Pts',(-18.3740146168879,-16.607111388571,
12.));
#181524=CARTESIAN_POINT('Ctrl Pts',(-18.3838352018327,-16.6297943620056,
12.));
#181525=CARTESIAN_POINT('Ctrl Pts',(-18.3936339764332,-16.6525771454513,
12.));
#181526=CARTESIAN_POINT('Ctrl Pts',(-18.403410471079,-16.6754593658513,
12.));
#181527=CARTESIAN_POINT('Ctrl Pts',(-18.413164220399,-16.6984406518491,
12.));
#181528=CARTESIAN_POINT('Ctrl Pts',(-18.4228947633187,-16.7215206338818,
12.));
#181529=CARTESIAN_POINT('Ctrl Pts',(-18.4326016431392,-16.7446989442882,
12.));
#181530=CARTESIAN_POINT('Ctrl Pts',(-18.44228440761,-16.7679752173992,12.));
#181531=CARTESIAN_POINT('Ctrl Pts',(-18.4519426090124,-16.791349089629,
12.));
#181532=CARTESIAN_POINT('Ctrl Pts',(-18.4615758042305,-16.8148201995472,
12.));
#181533=CARTESIAN_POINT('Ctrl Pts',(-18.4711835548623,-16.8383881879709,
12.));
#181534=CARTESIAN_POINT('Ctrl Pts',(-18.4807654268771,-16.8620526977171,
12.));
#181535=CARTESIAN_POINT('Ctrl Pts',(-18.4903209902227,-16.8858133733088,
12.));
#181536=CARTESIAN_POINT('Ctrl Pts',(-18.499849818462,-16.9096698606943,
12.));
#181537=CARTESIAN_POINT('Ctrl Pts',(-18.5093514883835,-16.9336218069353,
12.));
#181538=CARTESIAN_POINT('Ctrl Pts',(-18.5188255796659,-16.9576688599339,
12.));
#181539=CARTESIAN_POINT('Ctrl Pts',(-18.5282716744197,-16.981810668038,
12.));
#181540=CARTESIAN_POINT('Ctrl Pts',(-18.5376893576961,-17.0060468805097,
12.));
#181541=CARTESIAN_POINT('Ctrl Pts',(-18.547078218209,-17.0303771481738,
12.));
#181542=CARTESIAN_POINT('Ctrl Pts',(-18.556437848963,-17.0548011239751,
12.));
#181543=CARTESIAN_POINT('Ctrl Pts',(-18.5657678479789,-17.0793184636079,
12.));
#181544=CARTESIAN_POINT('Ctrl Pts',(-18.5750678188542,-17.1039288260001,
12.));
#181545=CARTESIAN_POINT('Ctrl Pts',(-18.5843373717247,-17.1286318741183,
12.));
#181546=CARTESIAN_POINT('Ctrl Pts',(-18.5935761222825,-17.1534272741643,
12.));
#181547=CARTESIAN_POINT('Ctrl Pts',(-18.6027836898817,-17.1783146940127,
12.));
#181548=CARTESIAN_POINT('Ctrl Pts',(-18.6119596959949,-17.2032938019284,
12.));
#181549=CARTESIAN_POINT('Ctrl Pts',(-18.6211037624038,-17.2283642650518,
12.));
#181550=CARTESIAN_POINT('Ctrl Pts',(-18.6302155097943,-17.2535257482187,
12.));
#181551=CARTESIAN_POINT('Ctrl Pts',(-18.6392945554748,-17.2787779120213,
12.));
#181552=CARTESIAN_POINT('Ctrl Pts',(-18.6483405141865,-17.3041204135074,
12.));
#181553=CARTESIAN_POINT('Ctrl Pts',(-18.6573530024033,-17.3295529098618,
12.));
#181554=CARTESIAN_POINT('Ctrl Pts',(-18.6663316416582,-17.3550750612443,
12.));
#181555=CARTESIAN_POINT('Ctrl Pts',(-18.6752760624052,-17.3806865340747,
12.));
#181556=CARTESIAN_POINT('Ctrl Pts',(-18.6841859073471,-17.4063870038562,
12.));
#181557=CARTESIAN_POINT('Ctrl Pts',(-18.6930608357409,-17.4321761588142,
12.));
#181558=CARTESIAN_POINT('Ctrl Pts',(-18.70190052503,-17.4580537012753,12.));
#181559=CARTESIAN_POINT('Ctrl Pts',(-18.7107046613912,-17.4840193397162,
12.));
#181560=CARTESIAN_POINT('Ctrl Pts',(-18.7194729318098,-17.5100727820876,
12.));
#181561=CARTESIAN_POINT('Ctrl Pts',(-18.7282050157138,-17.5362137287593,
12.));
#181562=CARTESIAN_POINT('Ctrl Pts',(-18.7369005764553,-17.5624418653245,
12.));
#181563=CARTESIAN_POINT('Ctrl Pts',(-18.7455592536687,-17.5887568561371,
12.));
#181564=CARTESIAN_POINT('Ctrl Pts',(-18.7541806530984,-17.6151583357012,
12.));
#181565=CARTESIAN_POINT('Ctrl Pts',(-18.762764361321,-17.6416459210681,
12.));
#181566=CARTESIAN_POINT('Ctrl Pts',(-18.7713099642754,-17.6682192274236,
12.));
#181567=CARTESIAN_POINT('Ctrl Pts',(-18.7798170641374,-17.6948778823014,
12.));
#181568=CARTESIAN_POINT('Ctrl Pts',(-18.788285297605,-17.7216215409035,
12.));
#181569=CARTESIAN_POINT('Ctrl Pts',(-18.7967143519419,-17.7484498996905,
12.));
#181570=CARTESIAN_POINT('Ctrl Pts',(-18.8051039860448,-17.7753627137853,
12.));
#181571=CARTESIAN_POINT('Ctrl Pts',(-18.8134540340417,-17.8023598011057,
12.));
#181572=CARTESIAN_POINT('Ctrl Pts',(-18.8217643886157,-17.8294410311006,
12.));
#181573=CARTESIAN_POINT('Ctrl Pts',(-18.8300349895974,-17.8566063174771,
12.));
#181574=CARTESIAN_POINT('Ctrl Pts',(-18.8366196462581,-17.8784057509356,
12.));
#181575=CARTESIAN_POINT('Ctrl Pts',(-18.8415402351786,-17.8947931177807,
12.));
#181576=CARTESIAN_POINT('Ctrl Pts',(-18.8448126709692,-17.9057348246595,
12.));
#181577=CARTESIAN_POINT('Ctrl Pts',(-18.8464468996588,-17.9112098770111,
12.));
#181578=CARTESIAN_POINT('',(-17.9112098770111,-18.8464468996588,12.));
#181579=CARTESIAN_POINT('Origin',(0.,0.,12.));
#181580=CARTESIAN_POINT('',(-14.6513681262571,-17.1452095830632,12.));
#181581=CARTESIAN_POINT('Ctrl Pts',(-17.9112098770111,-18.8464468996588,
12.));
#181582=CARTESIAN_POINT('Ctrl Pts',(-17.9057348246611,-18.8448126709726,
12.));
#181583=CARTESIAN_POINT('Ctrl Pts',(-17.8947931177853,-18.8415402351882,
12.));
#181584=CARTESIAN_POINT('Ctrl Pts',(-17.8784057509434,-18.8366196462746,
12.));
#181585=CARTESIAN_POINT('Ctrl Pts',(-17.8566063174871,-18.8300349896187,
12.));
#181586=CARTESIAN_POINT('Ctrl Pts',(-17.8294410311105,-18.8217643886368,
12.));
#181587=CARTESIAN_POINT('Ctrl Pts',(-17.8023598011135,-18.8134540340581,
12.));
#181588=CARTESIAN_POINT('Ctrl Pts',(-17.7753627137898,-18.8051039860543,
12.));
#181589=CARTESIAN_POINT('Ctrl Pts',(-17.7484498996917,-18.7967143519444,
12.));
#181590=CARTESIAN_POINT('Ctrl Pts',(-17.7216215409019,-18.7882852976016,
12.));
#181591=CARTESIAN_POINT('Ctrl Pts',(-17.6948778822982,-18.7798170641305,
12.));
#181592=CARTESIAN_POINT('Ctrl Pts',(-17.6682192274197,-18.7713099642673,
12.));
#181593=CARTESIAN_POINT('Ctrl Pts',(-17.6416459210646,-18.7627643613138,
12.));
#181594=CARTESIAN_POINT('Ctrl Pts',(-17.6151583356989,-18.7541806530935,
12.));
#181595=CARTESIAN_POINT('Ctrl Pts',(-17.5887568561361,-18.7455592536667,
12.));
#181596=CARTESIAN_POINT('Ctrl Pts',(-17.5624418653248,-18.7369005764558,
12.));
#181597=CARTESIAN_POINT('Ctrl Pts',(-17.5362137287604,-18.728205015716,
12.));
#181598=CARTESIAN_POINT('Ctrl Pts',(-17.5100727820891,-18.7194729318127,
12.));
#181599=CARTESIAN_POINT('Ctrl Pts',(-17.4840193397176,-18.7107046613941,
12.));
#181600=CARTESIAN_POINT('Ctrl Pts',(-17.4580537012764,-18.7019005250322,
12.));
#181601=CARTESIAN_POINT('Ctrl Pts',(-17.4321761588148,-18.6930608357421,
12.));
#181602=CARTESIAN_POINT('Ctrl Pts',(-17.4063870038563,-18.6841859073472,
12.));
#181603=CARTESIAN_POINT('Ctrl Pts',(-17.3806865340744,-18.6752760624045,
12.));
#181604=CARTESIAN_POINT('Ctrl Pts',(-17.3550750612438,-18.6663316416569,
12.));
#181605=CARTESIAN_POINT('Ctrl Pts',(-17.3295529098612,-18.6573530024019,
12.));
#181606=CARTESIAN_POINT('Ctrl Pts',(-17.3041204135069,-18.6483405141853,
12.));
#181607=CARTESIAN_POINT('Ctrl Pts',(-17.278777912021,-18.639294555474,12.));
#181608=CARTESIAN_POINT('Ctrl Pts',(-17.2535257482186,-18.630215509794,
12.));
#181609=CARTESIAN_POINT('Ctrl Pts',(-17.2283642650519,-18.6211037624041,
12.));
#181610=CARTESIAN_POINT('Ctrl Pts',(-17.2032938019288,-18.6119596959957,
12.));
#181611=CARTESIAN_POINT('Ctrl Pts',(-17.1783146940131,-18.6027836898826,
12.));
#181612=CARTESIAN_POINT('Ctrl Pts',(-17.1534272741646,-18.5935761222833,
12.));
#181613=CARTESIAN_POINT('Ctrl Pts',(-17.1286318741185,-18.5843373717253,
12.));
#181614=CARTESIAN_POINT('Ctrl Pts',(-17.1039288260002,-18.5750678188543,
12.));
#181615=CARTESIAN_POINT('Ctrl Pts',(-17.0793184636079,-18.5657678479788,
12.));
#181616=CARTESIAN_POINT('Ctrl Pts',(-17.0548011239751,-18.5564378489628,
12.));
#181617=CARTESIAN_POINT('Ctrl Pts',(-17.030377148174,-18.5470782182089,
12.));
#181618=CARTESIAN_POINT('Ctrl Pts',(-17.0060468805099,-18.5376893576961,
12.));
#181619=CARTESIAN_POINT('Ctrl Pts',(-16.9818106680382,-18.5282716744198,
12.));
#181620=CARTESIAN_POINT('Ctrl Pts',(-16.957668859934,-18.518825579666,12.));
#181621=CARTESIAN_POINT('Ctrl Pts',(-16.9336218069353,-18.5093514883835,
12.));
#181622=CARTESIAN_POINT('Ctrl Pts',(-16.9096698606942,-18.4998498184619,
12.));
#181623=CARTESIAN_POINT('Ctrl Pts',(-16.8858133733086,-18.4903209902226,
12.));
#181624=CARTESIAN_POINT('Ctrl Pts',(-16.8620526977169,-18.4807654268769,
12.));
#181625=CARTESIAN_POINT('Ctrl Pts',(-16.8383881879707,-18.4711835548622,
12.));
#181626=CARTESIAN_POINT('Ctrl Pts',(-16.8148201995472,-18.4615758042305,
12.));
#181627=CARTESIAN_POINT('Ctrl Pts',(-16.791349089629,-18.4519426090124,
12.));
#181628=CARTESIAN_POINT('Ctrl Pts',(-16.7679752173992,-18.4422844076099,
12.));
#181629=CARTESIAN_POINT('Ctrl Pts',(-16.7446989442882,-18.4326016431392,
12.));
#181630=CARTESIAN_POINT('Ctrl Pts',(-16.7215206338818,-18.4228947633186,
12.));
#181631=CARTESIAN_POINT('Ctrl Pts',(-16.698440651849,-18.4131642203989,
12.));
#181632=CARTESIAN_POINT('Ctrl Pts',(-16.6754593658513,-18.4034104710789,
12.));
#181633=CARTESIAN_POINT('Ctrl Pts',(-16.6525771454513,-18.3936339764332,
12.));
#181634=CARTESIAN_POINT('Ctrl Pts',(-16.6297943620056,-18.3838352018327,
12.));
#181635=CARTESIAN_POINT('Ctrl Pts',(-16.6071113885711,-18.3740146168879,
12.));
#181636=CARTESIAN_POINT('Ctrl Pts',(-16.5845286000219,-18.364172695589,
12.));
#181637=CARTESIAN_POINT('Ctrl Pts',(-16.5620463731414,-18.3543099164331,
12.));
#181638=CARTESIAN_POINT('Ctrl Pts',(-16.539665086714,-18.3444267625601,
12.));
#181639=CARTESIAN_POINT('Ctrl Pts',(-16.5173851216045,-18.3345237218864,
12.));
#181640=CARTESIAN_POINT('Ctrl Pts',(-16.4952068608344,-18.3246012872468,
12.));
#181641=CARTESIAN_POINT('Ctrl Pts',(-16.4731306896439,-18.3146599565229,
12.));
#181642=CARTESIAN_POINT('Ctrl Pts',(-16.4511569955231,-18.3047002326858,
12.));
#181643=CARTESIAN_POINT('Ctrl Pts',(-16.4292861682377,-18.2947226238509,
12.));
#181644=CARTESIAN_POINT('Ctrl Pts',(-16.4075185998454,-18.2847276433308,
12.));
#181645=CARTESIAN_POINT('Ctrl Pts',(-16.385854684708,-18.2747158096934,
12.));
#181646=CARTESIAN_POINT('Ctrl Pts',(-16.3642948194869,-18.2646876468169,
12.));
#181647=CARTESIAN_POINT('Ctrl Pts',(-16.342839403159,-18.2546436839609,
12.));
#181648=CARTESIAN_POINT('Ctrl Pts',(-16.3214888370988,-18.2445844558742,
12.));
#181649=CARTESIAN_POINT('Ctrl Pts',(-16.3002435251378,-18.2345105028981,
12.));
#181650=CARTESIAN_POINT('Ctrl Pts',(-16.2791038736223,-18.2244223710745,
12.));
#181651=CARTESIAN_POINT('Ctrl Pts',(-16.2580702914615,-18.214320612253,
12.));
#181652=CARTESIAN_POINT('Ctrl Pts',(-16.237143190164,-18.2042057842037,
12.));
#181653=CARTESIAN_POINT('Ctrl Pts',(-16.2163229838878,-18.1940784507232,
12.));
#181654=CARTESIAN_POINT('Ctrl Pts',(-16.1956100895076,-18.1839391817335,
12.));
#181655=CARTESIAN_POINT('Ctrl Pts',(-16.1750049266673,-18.1737885533852,
12.));
#181656=CARTESIAN_POINT('Ctrl Pts',(-16.1545079178261,-18.1636271481616,
12.));
#181657=CARTESIAN_POINT('Ctrl Pts',(-16.1341194882987,-18.153455554985,
12.));
#181658=CARTESIAN_POINT('Ctrl Pts',(-16.1138400662791,-18.1432743693231,
12.));
#181659=CARTESIAN_POINT('Ctrl Pts',(-16.0936700829108,-18.1330841933099,
12.));
#181660=CARTESIAN_POINT('Ctrl Pts',(-16.0736099723665,-18.1228856358746,
12.));
#181661=CARTESIAN_POINT('Ctrl Pts',(-16.0536601719124,-18.1126793128688,
12.));
#181662=CARTESIAN_POINT('Ctrl Pts',(-16.0338211219694,-18.1024658471966,
12.));
#181663=CARTESIAN_POINT('Ctrl Pts',(-16.0140932661612,-18.0922458689464,
12.));
#181664=CARTESIAN_POINT('Ctrl Pts',(-15.9944770513616,-18.0820200155238,
12.));
#181665=CARTESIAN_POINT('Ctrl Pts',(-15.9749729277848,-18.071788931796,
12.));
#181666=CARTESIAN_POINT('Ctrl Pts',(-15.9555813490645,-18.061553270236,
12.));
#181667=CARTESIAN_POINT('Ctrl Pts',(-15.9363027723244,-18.0513136910691,
12.));
#181668=CARTESIAN_POINT('Ctrl Pts',(-15.9171376582436,-18.0410708624208,
12.));
#181669=CARTESIAN_POINT('Ctrl Pts',(-15.8980864711043,-18.0308254604638,
12.));
#181670=CARTESIAN_POINT('Ctrl Pts',(-15.8791496788685,-18.0205781695773,
12.));
#181671=CARTESIAN_POINT('Ctrl Pts',(-15.8603277532834,-18.010329682521,
12.));
#181672=CARTESIAN_POINT('Ctrl Pts',(-15.8416211699682,-18.0000807006055,
12.));
#181673=CARTESIAN_POINT('Ctrl Pts',(-15.8230304084963,-17.9898319338664,
12.));
#181674=CARTESIAN_POINT('Ctrl Pts',(-15.8045559524674,-17.9795841012383,
12.));
#181675=CARTESIAN_POINT('Ctrl Pts',(-15.786198289572,-17.9693379307297,
12.));
#181676=CARTESIAN_POINT('Ctrl Pts',(-15.7679579117072,-17.9590941596236,
12.));
#181677=CARTESIAN_POINT('Ctrl Pts',(-15.7498353150856,-17.9488535346776,
12.));
#181678=CARTESIAN_POINT('Ctrl Pts',(-15.7318310003334,-17.9386168123261,
12.));
#181679=CARTESIAN_POINT('Ctrl Pts',(-15.713945472584,-17.9283847588837,
12.));
#181680=CARTESIAN_POINT('Ctrl Pts',(-15.6961792415526,-17.918158150746,
12.));
#181681=CARTESIAN_POINT('Ctrl Pts',(-15.6785328216467,-17.9079377746118,
12.));
#181682=CARTESIAN_POINT('Ctrl Pts',(-15.6610067321036,-17.8977244277247,
12.));
#181683=CARTESIAN_POINT('Ctrl Pts',(-15.6436014971088,-17.8875189181095,
12.));
#181684=CARTESIAN_POINT('Ctrl Pts',(-15.6263176459107,-17.8773220648125,
12.));
#181685=CARTESIAN_POINT('Ctrl Pts',(-15.6091557129205,-17.8671346981388,
12.));
#181686=CARTESIAN_POINT('Ctrl Pts',(-15.5921162378183,-17.8569576598996,
12.));
#181687=CARTESIAN_POINT('Ctrl Pts',(-15.5751997657154,-17.8467918036976,
12.));
#181688=CARTESIAN_POINT('Ctrl Pts',(-15.5584068472976,-17.8366379952078,
12.));
#181689=CARTESIAN_POINT('Ctrl Pts',(-15.5417380389639,-17.8264971124606,
12.));
#181690=CARTESIAN_POINT('Ctrl Pts',(-15.5251939029558,-17.8163700461262,
12.));
#181691=CARTESIAN_POINT('Ctrl Pts',(-15.5087750074728,-17.8062576997964,
12.));
#181692=CARTESIAN_POINT('Ctrl Pts',(-15.4924819268529,-17.7961609903161,
12.));
#181693=CARTESIAN_POINT('Ctrl Pts',(-15.4763152417506,-17.7860808481229,
12.));
#181694=CARTESIAN_POINT('Ctrl Pts',(-15.460275539302,-17.7760182175817,
12.));
#181695=CARTESIAN_POINT('Ctrl Pts',(-15.4443634132865,-17.765974057326,
12.));
#181696=CARTESIAN_POINT('Ctrl Pts',(-15.4285794642658,-17.7559493405871,
12.));
#181697=CARTESIAN_POINT('Ctrl Pts',(-15.4129242997828,-17.7459450555803,
12.));
#181698=CARTESIAN_POINT('Ctrl Pts',(-15.3973985345796,-17.7359622059143,
12.));
#181699=CARTESIAN_POINT('Ctrl Pts',(-15.3820027907965,-17.7260018109923,
12.));
#181700=CARTESIAN_POINT('Ctrl Pts',(-15.3667376981702,-17.7160649064208,
12.));
#181701=CARTESIAN_POINT('Ctrl Pts',(-15.3516038942064,-17.7061525444044,
12.));
#181702=CARTESIAN_POINT('Ctrl Pts',(-15.3366020244069,-17.6962657941984,
12.));
#181703=CARTESIAN_POINT('Ctrl Pts',(-15.3217327425341,-17.6864057426052,
12.));
#181704=CARTESIAN_POINT('Ctrl Pts',(-15.3069967108501,-17.6765734944559,
12.));
#181705=CARTESIAN_POINT('Ctrl Pts',(-15.2923946003598,-17.6667701731041,
12.));
#181706=CARTESIAN_POINT('Ctrl Pts',(-15.2779270910238,-17.6569969209,12.));
#181707=CARTESIAN_POINT('Ctrl Pts',(-15.263594872029,-17.6472548997329,
12.));
#181708=CARTESIAN_POINT('Ctrl Pts',(-15.2493986421091,-17.637545291637,
12.));
#181709=CARTESIAN_POINT('Ctrl Pts',(-15.2353391098367,-17.6278692993765,
12.));
#181710=CARTESIAN_POINT('Ctrl Pts',(-15.22141699392,-17.6182281470467,12.));
#181711=CARTESIAN_POINT('Ctrl Pts',(-15.2076330234686,-17.6086230806497,
12.));
#181712=CARTESIAN_POINT('Ctrl Pts',(-15.1939879383268,-17.5990553687595,
12.));
#181713=CARTESIAN_POINT('Ctrl Pts',(-15.1804824894605,-17.5895263032592,
12.));
#181714=CARTESIAN_POINT('Ctrl Pts',(-15.1671174393137,-17.5800372000539,
12.));
#181715=CARTESIAN_POINT('Ctrl Pts',(-15.1538935621715,-17.570589399803,
12.));
#181716=CARTESIAN_POINT('Ctrl Pts',(-15.1408116444877,-17.5611842686196,
12.));
#181717=CARTESIAN_POINT('Ctrl Pts',(-15.127872485314,-17.5518231989122,
12.));
#181718=CARTESIAN_POINT('Ctrl Pts',(-15.1150768967729,-17.5425076102966,
12.));
#181719=CARTESIAN_POINT('Ctrl Pts',(-15.1024257045033,-17.5332389504829,
12.));
#181720=CARTESIAN_POINT('Ctrl Pts',(-15.0899197481082,-17.5240186961788,
12.));
#181721=CARTESIAN_POINT('Ctrl Pts',(-15.0775598815748,-17.5148483539683,
12.));
#181722=CARTESIAN_POINT('Ctrl Pts',(-15.0653469738306,-17.5057294613874,
12.));
#181723=CARTESIAN_POINT('Ctrl Pts',(-15.0532819093085,-17.4966635880245,
12.));
#181724=CARTESIAN_POINT('Ctrl Pts',(-15.0413655884993,-17.4876523366178,
12.));
#181725=CARTESIAN_POINT('Ctrl Pts',(-15.029598928488,-17.4786973441417,
12.));
#181726=CARTESIAN_POINT('Ctrl Pts',(-15.0179828635086,-17.4698002829356,
12.));
#181727=CARTESIAN_POINT('Ctrl Pts',(-15.0065183456921,-17.4609628621418,
12.));
#181728=CARTESIAN_POINT('Ctrl Pts',(-14.9952063457778,-17.4521868291004,
12.));
#181729=CARTESIAN_POINT('Ctrl Pts',(-14.9840478538358,-17.4434739707773,
12.));
#181730=CARTESIAN_POINT('Ctrl Pts',(-14.9730438799452,-17.4348261151396,
12.));
#181731=CARTESIAN_POINT('Ctrl Pts',(-14.9621954549827,-17.426245132709,
12.));
#181732=CARTESIAN_POINT('Ctrl Pts',(-14.9515036315143,-17.4177329382828,
12.));
#181733=CARTESIAN_POINT('Ctrl Pts',(-14.940969484645,-17.4092914926071,
12.));
#181734=CARTESIAN_POINT('Ctrl Pts',(-14.9305941128757,-17.4009228040749,
12.));
#181735=CARTESIAN_POINT('Ctrl Pts',(-14.9203786389342,-17.3926289303986,
12.));
#181736=CARTESIAN_POINT('Ctrl Pts',(-14.9103242110058,-17.3844119809824,
12.));
#181737=CARTESIAN_POINT('Ctrl Pts',(-14.900432003961,-17.3762741193076,
12.));
#181738=CARTESIAN_POINT('Ctrl Pts',(-14.8907032205788,-17.3682175653235,
12.));
#181739=CARTESIAN_POINT('Ctrl Pts',(-14.8811390927423,-17.3602445978161,
12.));
#181740=CARTESIAN_POINT('Ctrl Pts',(-14.8717408826956,-17.3523575568645,
12.));
#181741=CARTESIAN_POINT('Ctrl Pts',(-14.8625098843417,-17.3445588463474,
12.));
#181742=CARTESIAN_POINT('Ctrl Pts',(-14.8534474245434,-17.336850936485,
12.));
#181743=CARTESIAN_POINT('Ctrl Pts',(-14.8445548643508,-17.3292363662605,
12.));
#181744=CARTESIAN_POINT('Ctrl Pts',(-14.8358336004197,-17.3217177462101,
12.));
#181745=CARTESIAN_POINT('Ctrl Pts',(-14.8272850675379,-17.3142977632659,
12.));
#181746=CARTESIAN_POINT('Ctrl Pts',(-14.8189107410162,-17.3069791853706,
12.));
#181747=CARTESIAN_POINT('Ctrl Pts',(-14.8107121391036,-17.299764866148,
12.));
#181748=CARTESIAN_POINT('Ctrl Pts',(-14.8026908254276,-17.2926577496513,
12.));
#181749=CARTESIAN_POINT('Ctrl Pts',(-14.7948484105249,-17.2856608733196,
12.));
#181750=CARTESIAN_POINT('Ctrl Pts',(-14.787186553128,-17.2787773704849,
12.));
#181751=CARTESIAN_POINT('Ctrl Pts',(-14.7797069617804,-17.2720104735194,
12.));
#181752=CARTESIAN_POINT('Ctrl Pts',(-14.7724113956731,-17.2653635155319,
12.));
#181753=CARTESIAN_POINT('Ctrl Pts',(-14.7653016697591,-17.2588399401465,
12.));
#181754=CARTESIAN_POINT('Ctrl Pts',(-14.7583796616617,-17.2524433146837,
12.));
#181755=CARTESIAN_POINT('Ctrl Pts',(-14.7516473175124,-17.2461773413288,
12.));
#181756=CARTESIAN_POINT('Ctrl Pts',(-14.7451066593792,-17.2400458713565,
12.));
#181757=CARTESIAN_POINT('Ctrl Pts',(-14.7387597858117,-17.2340529062076,
12.));
#181758=CARTESIAN_POINT('Ctrl Pts',(-14.7326088681163,-17.2282025904314,
12.));
#181759=CARTESIAN_POINT('Ctrl Pts',(-14.7266561494282,-17.2224992099666,
12.));
#181760=CARTESIAN_POINT('Ctrl Pts',(-14.7209039390327,-17.2169471814256,
12.));
#181761=CARTESIAN_POINT('Ctrl Pts',(-14.7153546289339,-17.2115510835989,
12.));
#181762=CARTESIAN_POINT('Ctrl Pts',(-14.7100107213586,-17.2063157097315,
12.));
#181763=CARTESIAN_POINT('Ctrl Pts',(-14.7048748502663,-17.2012461084268,
12.));
#181764=CARTESIAN_POINT('Ctrl Pts',(-14.699949811582,-17.1963476411694,
12.));
#181765=CARTESIAN_POINT('Ctrl Pts',(-14.6952385361706,-17.1916259308415,
12.));
#181766=CARTESIAN_POINT('Ctrl Pts',(-14.6907440526958,-17.1870867909918,
12.));
#181767=CARTESIAN_POINT('Ctrl Pts',(-14.686469452232,-17.1827361584719,
12.));
#181768=CARTESIAN_POINT('Ctrl Pts',(-14.6824178576167,-17.1785800350826,
12.));
#181769=CARTESIAN_POINT('Ctrl Pts',(-14.6785925615677,-17.1746247499056,
12.));
#181770=CARTESIAN_POINT('Ctrl Pts',(-14.6749971333867,-17.1708771619129,
12.));
#181771=CARTESIAN_POINT('Ctrl Pts',(-14.671635583332,-17.167344972302,12.));
#181772=CARTESIAN_POINT('Ctrl Pts',(-14.6685123374423,-17.1640366762305,
12.));
#181773=CARTESIAN_POINT('Ctrl Pts',(-14.6656319165057,-17.1609609517369,
12.));
#181774=CARTESIAN_POINT('Ctrl Pts',(-14.6629987285992,-17.1581262646789,
12.));
#181775=CARTESIAN_POINT('Ctrl Pts',(-14.6606167169642,-17.1555401986401,
12.));
#181776=CARTESIAN_POINT('Ctrl Pts',(-14.6584900555302,-17.1532107762718,
12.));
#181777=CARTESIAN_POINT('Ctrl Pts',(-14.6566237952435,-17.1511476869496,
12.));
#181778=CARTESIAN_POINT('Ctrl Pts',(-14.655024862281,-17.1493641837558,
12.));
#181779=CARTESIAN_POINT('Ctrl Pts',(-14.6537016966184,-17.147876394491,
12.));
#181780=CARTESIAN_POINT('Ctrl Pts',(-14.6526624064978,-17.1466998098673,
12.));
#181781=CARTESIAN_POINT('Ctrl Pts',(-14.6519131634508,-17.1458462295271,
12.));
#181782=CARTESIAN_POINT('Ctrl Pts',(-14.6515481598068,-17.1454262858043,
12.));
#181783=CARTESIAN_POINT('Ctrl Pts',(-14.6514066997196,-17.1452600887037,
12.));
#181784=CARTESIAN_POINT('Ctrl Pts',(-14.6513711852843,-17.1452153999142,
12.));
#181785=CARTESIAN_POINT('Ctrl Pts',(-14.6513681262571,-17.1452095830632,
12.));
#181786=CARTESIAN_POINT('',(-14.2886635873976,-16.7207683102834,12.));
#181787=CARTESIAN_POINT('',(-6.98376450772884,-8.17248635976757,12.));
#181788=CARTESIAN_POINT('',(-13.5924445804218,-16.6581946899465,12.));
#181789=CARTESIAN_POINT('Origin',(-13.9085479427572,-17.0455945664569,12.));
#181790=CARTESIAN_POINT('',(-12.572596943457,-17.4407513054161,12.));
#181791=CARTESIAN_POINT('Origin',(-4.9889687874677E-13,-6.00167842331873E-13,
12.));
#181792=CARTESIAN_POINT('',(-12.4528436808172,-18.1294424696716,12.));
#181793=CARTESIAN_POINT('Origin',(-12.8649829188863,-17.846350172984,12.));
#181794=CARTESIAN_POINT('',(-12.7689476255363,-18.5896416359912,12.));
#181795=CARTESIAN_POINT('',(-6.38447381276812,-9.29482081799561,12.));
#181796=CARTESIAN_POINT('',(-13.5685075571671,-22.1787195904339,12.));
#181797=CARTESIAN_POINT('Ctrl Pts',(-12.7689476255363,-18.5896416359912,
12.));
#181798=CARTESIAN_POINT('Ctrl Pts',(-12.7689524524484,-18.5896460962961,
12.));
#181799=CARTESIAN_POINT('Ctrl Pts',(-12.7689864266924,-18.5896919669158,
12.));
#181800=CARTESIAN_POINT('Ctrl Pts',(-12.7691103481996,-18.589871621842,
12.));
#181801=CARTESIAN_POINT('Ctrl Pts',(-12.7694215127923,-18.590332877722,
12.));
#181802=CARTESIAN_POINT('Ctrl Pts',(-12.7700520897174,-18.5912775137806,
12.));
#181803=CARTESIAN_POINT('Ctrl Pts',(-12.7709195951154,-18.5925859134582,
12.));
#181804=CARTESIAN_POINT('Ctrl Pts',(-12.7720142287169,-18.5942490615409,
12.));
#181805=CARTESIAN_POINT('Ctrl Pts',(-12.7733231262107,-18.5962551167772,
12.));
#181806=CARTESIAN_POINT('Ctrl Pts',(-12.7748328937639,-18.5985917525949,
12.));
#181807=CARTESIAN_POINT('Ctrl Pts',(-12.7765325225083,-18.6012488486708,
12.));
#181808=CARTESIAN_POINT('Ctrl Pts',(-12.7784139605067,-18.6042190183703,
12.));
#181809=CARTESIAN_POINT('Ctrl Pts',(-12.7804705387658,-18.6074961535723,
12.));
#181810=CARTESIAN_POINT('Ctrl Pts',(-12.7826959526924,-18.611074482622,
12.));
#181811=CARTESIAN_POINT('Ctrl Pts',(-12.78508316579,-18.6149475565189,12.));
#181812=CARTESIAN_POINT('Ctrl Pts',(-12.7876249657834,-18.6191087624752,
12.));
#181813=CARTESIAN_POINT('Ctrl Pts',(-12.7903142925235,-18.6235516265575,
12.));
#181814=CARTESIAN_POINT('Ctrl Pts',(-12.7931447451556,-18.6282702819371,
12.));
#181815=CARTESIAN_POINT('Ctrl Pts',(-12.7961106222251,-18.6332595057005,
12.));
#181816=CARTESIAN_POINT('Ctrl Pts',(-12.7992066625264,-18.63851447924,12.));
#181817=CARTESIAN_POINT('Ctrl Pts',(-12.8024278770153,-18.6440306327457,
12.));
#181818=CARTESIAN_POINT('Ctrl Pts',(-12.805769331162,-18.6498034438986,
12.));
#181819=CARTESIAN_POINT('Ctrl Pts',(-12.8092261933858,-18.6558284825772,
12.));
#181820=CARTESIAN_POINT('Ctrl Pts',(-12.8127937909632,-18.6621014624746,
12.));
#181821=CARTESIAN_POINT('Ctrl Pts',(-12.8164676687361,-18.6686182952798,
12.));
#181822=CARTESIAN_POINT('Ctrl Pts',(-12.8202436318473,-18.6753751301091,
12.));
#181823=CARTESIAN_POINT('Ctrl Pts',(-12.8241176980016,-18.6823683094138,
12.));
#181824=CARTESIAN_POINT('Ctrl Pts',(-12.8280860635231,-18.6895943376172,
12.));
#181825=CARTESIAN_POINT('Ctrl Pts',(-12.832145059979,-18.6970498410173,
12.));
#181826=CARTESIAN_POINT('Ctrl Pts',(-12.8362911280362,-18.7047315436296,
12.));
#181827=CARTESIAN_POINT('Ctrl Pts',(-12.8405208263432,-18.7126362754446,
12.));
#181828=CARTESIAN_POINT('Ctrl Pts',(-12.8448308329494,-18.7207609737701,
12.));
#181829=CARTESIAN_POINT('Ctrl Pts',(-12.849217951159,-18.7291026886552,
12.));
#181830=CARTESIAN_POINT('Ctrl Pts',(-12.8536791086315,-18.7376585820851,
12.));
#181831=CARTESIAN_POINT('Ctrl Pts',(-12.8582113455645,-18.7464259171248,
12.));
#181832=CARTESIAN_POINT('Ctrl Pts',(-12.8628118054172,-18.7554020493888,
12.));
#181833=CARTESIAN_POINT('Ctrl Pts',(-12.8674777239656,-18.7645844169568,
12.));
#181834=CARTESIAN_POINT('Ctrl Pts',(-12.8722064211814,-18.7739705329028,
12.));
#181835=CARTESIAN_POINT('Ctrl Pts',(-12.8769952998097,-18.7835579840481,
12.));
#181836=CARTESIAN_POINT('Ctrl Pts',(-12.8818418427474,-18.7933444285867,
12.));
#181837=CARTESIAN_POINT('Ctrl Pts',(-12.8867436109543,-18.8033275941939,
12.));
#181838=CARTESIAN_POINT('Ctrl Pts',(-12.8916982409931,-18.8135052757815,
12.));
#181839=CARTESIAN_POINT('Ctrl Pts',(-12.8967034410752,-18.8238753319124,
12.));
#181840=CARTESIAN_POINT('Ctrl Pts',(-12.9017569871738,-18.834435681259,
12.));
#181841=CARTESIAN_POINT('Ctrl Pts',(-12.9068567191856,-18.8451842990986,
12.));
#181842=CARTESIAN_POINT('Ctrl Pts',(-12.9120005369066,-18.8561192136201,
12.));
#181843=CARTESIAN_POINT('Ctrl Pts',(-12.9171863977047,-18.8672385038328,
12.));
#181844=CARTESIAN_POINT('Ctrl Pts',(-12.9224123144982,-18.8785402977528,
12.));
#181845=CARTESIAN_POINT('Ctrl Pts',(-12.9276763536373,-18.8900227704888,
12.));
#181846=CARTESIAN_POINT('Ctrl Pts',(-12.9329766328184,-18.9016841423402,
12.));
#181847=CARTESIAN_POINT('Ctrl Pts',(-12.9383113190375,-18.9135226769466,
12.));
#181848=CARTESIAN_POINT('Ctrl Pts',(-12.9436786266106,-18.9255366795196,
12.));
#181849=CARTESIAN_POINT('Ctrl Pts',(-12.9490768151821,-18.9377244950435,
12.));
#181850=CARTESIAN_POINT('Ctrl Pts',(-12.9545041877377,-18.9500845064714,
12.));
#181851=CARTESIAN_POINT('Ctrl Pts',(-12.9599590886318,-18.9626151329226,
12.));
#181852=CARTESIAN_POINT('Ctrl Pts',(-12.9654399021868,-18.9753148284473,
12.));
#181853=CARTESIAN_POINT('Ctrl Pts',(-12.9709450512747,-18.9881820807585,
12.));
#181854=CARTESIAN_POINT('Ctrl Pts',(-12.9764729959206,-19.0012154099792,
12.));
#181855=CARTESIAN_POINT('Ctrl Pts',(-12.9820222318716,-19.014413367335,
12.));
#181856=CARTESIAN_POINT('Ctrl Pts',(-12.9875912893003,-19.0277745339908,
12.));
#181857=CARTESIAN_POINT('Ctrl Pts',(-12.9931787316514,-19.0412975200398,
12.));
#181858=CARTESIAN_POINT('Ctrl Pts',(-12.9987831544502,-19.0549809634354,
12.));
#181859=CARTESIAN_POINT('Ctrl Pts',(-13.0044031841382,-19.0688235289437,
12.));
#181860=CARTESIAN_POINT('Ctrl Pts',(-13.0100374768788,-19.0828239070484,
12.));
#181861=CARTESIAN_POINT('Ctrl Pts',(-13.0156847176097,-19.0969808131228,
12.));
#181862=CARTESIAN_POINT('Ctrl Pts',(-13.0213436191328,-19.111292986631,
12.));
#181863=CARTESIAN_POINT('Ctrl Pts',(-13.0270129211976,-19.1257591903099,
12.));
#181864=CARTESIAN_POINT('Ctrl Pts',(-13.0326913895838,-19.1403782093386,
12.));
#181865=CARTESIAN_POINT('Ctrl Pts',(-13.0383778152068,-19.155148850523,
12.));
#181866=CARTESIAN_POINT('Ctrl Pts',(-13.0440710133772,-19.1700699416622,
12.));
#181867=CARTESIAN_POINT('Ctrl Pts',(-13.0497698230441,-19.1851403308825,
12.));
#181868=CARTESIAN_POINT('Ctrl Pts',(-13.0554731060538,-19.2003588859772,
12.));
#181869=CARTESIAN_POINT('Ctrl Pts',(-13.0611797463915,-19.2157244937142,
12.));
#181870=CARTESIAN_POINT('Ctrl Pts',(-13.0668886494795,-19.2312360592033,
12.));
#181871=CARTESIAN_POINT('Ctrl Pts',(-13.0725987415859,-19.2468925053989,
12.));
#181872=CARTESIAN_POINT('Ctrl Pts',(-13.0783089692118,-19.2626927725596,
12.));
#181873=CARTESIAN_POINT('Ctrl Pts',(-13.0840182984949,-19.2786358177198,
12.));
#181874=CARTESIAN_POINT('Ctrl Pts',(-13.0897257145969,-19.2947206141247,
12.));
#181875=CARTESIAN_POINT('Ctrl Pts',(-13.0954302211479,-19.310946150736,
12.));
#181876=CARTESIAN_POINT('Ctrl Pts',(-13.1011308397591,-19.3273114318269,
12.));
#181877=CARTESIAN_POINT('Ctrl Pts',(-13.1068266095186,-19.3438154765395,
12.));
#181878=CARTESIAN_POINT('Ctrl Pts',(-13.1125165865022,-19.3604573184515,
12.));
#181879=CARTESIAN_POINT('Ctrl Pts',(-13.118199843271,-19.3772360051091,
12.));
#181880=CARTESIAN_POINT('Ctrl Pts',(-13.1238754684177,-19.3941505976263,
12.));
#181881=CARTESIAN_POINT('Ctrl Pts',(-13.1295425661634,-19.4112001703557,
12.));
#181882=CARTESIAN_POINT('Ctrl Pts',(-13.1352002559438,-19.4283838105262,
12.));
#181883=CARTESIAN_POINT('Ctrl Pts',(-13.1408476720061,-19.4457006178876,
12.));
#181884=CARTESIAN_POINT('Ctrl Pts',(-13.1464839629971,-19.4631497043258,
12.));
#181885=CARTESIAN_POINT('Ctrl Pts',(-13.1521082915853,-19.4807301935268,
12.));
#181886=CARTESIAN_POINT('Ctrl Pts',(-13.1577198341245,-19.4984412207081,
12.));
#181887=CARTESIAN_POINT('Ctrl Pts',(-13.1633177803101,-19.5162819323213,
12.));
#181888=CARTESIAN_POINT('Ctrl Pts',(-13.1689013328431,-19.5342514857562,
12.));
#181889=CARTESIAN_POINT('Ctrl Pts',(-13.1744697070911,-19.5523490490244,
12.));
#181890=CARTESIAN_POINT('Ctrl Pts',(-13.1800221307673,-19.5705738004667,
12.));
#181891=CARTESIAN_POINT('Ctrl Pts',(-13.1855578436471,-19.5889249285338,
12.));
#181892=CARTESIAN_POINT('Ctrl Pts',(-13.1910760972814,-19.6074016315414,
12.));
#181893=CARTESIAN_POINT('Ctrl Pts',(-13.1965761547151,-19.6260031174244,
12.));
#181894=CARTESIAN_POINT('Ctrl Pts',(-13.2020572902065,-19.6447286034772,
12.));
#181895=CARTESIAN_POINT('Ctrl Pts',(-13.2075187889529,-19.6635773160936,
12.));
#181896=CARTESIAN_POINT('Ctrl Pts',(-13.2129599468485,-19.6825484905823,
12.));
#181897=CARTESIAN_POINT('Ctrl Pts',(-13.2183800702436,-19.7016413709685,
12.));
#181898=CARTESIAN_POINT('Ctrl Pts',(-13.2237784757066,-19.7208552097868,
12.));
#181899=CARTESIAN_POINT('Ctrl Pts',(-13.2291544897899,-19.7401892678697,
12.));
#181900=CARTESIAN_POINT('Ctrl Pts',(-13.2345074487963,-19.7596428141168,
12.));
#181901=CARTESIAN_POINT('Ctrl Pts',(-13.2398366985675,-19.7792151253289,
12.));
#181902=CARTESIAN_POINT('Ctrl Pts',(-13.2451415942805,-19.7989054860495,
12.));
#181903=CARTESIAN_POINT('Ctrl Pts',(-13.2504215002457,-19.8187131883917,
12.));
#181904=CARTESIAN_POINT('Ctrl Pts',(-13.2556757897086,-19.8386375318634,
12.));
#181905=CARTESIAN_POINT('Ctrl Pts',(-13.2609038446529,-19.8586778231715,
12.));
#181906=CARTESIAN_POINT('Ctrl Pts',(-13.2661050556132,-19.8788333760577,
12.));
#181907=CARTESIAN_POINT('Ctrl Pts',(-13.271278821502,-19.8991035111745,
12.));
#181908=CARTESIAN_POINT('Ctrl Pts',(-13.2764245494357,-19.9194875559422,
12.));
#181909=CARTESIAN_POINT('Ctrl Pts',(-13.2815416545663,-19.9399848444019,
12.));
#181910=CARTESIAN_POINT('Ctrl Pts',(-13.286629559915,-19.9605947170586,
12.));
#181911=CARTESIAN_POINT('Ctrl Pts',(-13.2916876962094,-19.981316520717,
12.));
#181912=CARTESIAN_POINT('Ctrl Pts',(-13.2967155017306,-20.0021496083738,
12.));
#181913=CARTESIAN_POINT('Ctrl Pts',(-13.3017124221637,-20.0230933391038,
12.));
#181914=CARTESIAN_POINT('Ctrl Pts',(-13.3066779104515,-20.0441470779345,
12.));
#181915=CARTESIAN_POINT('Ctrl Pts',(-13.3116114266515,-20.0653101957188,
12.));
#181916=CARTESIAN_POINT('Ctrl Pts',(-13.3165124377963,-20.0865820689882,
12.));
#181917=CARTESIAN_POINT('Ctrl Pts',(-13.3213804177587,-20.1079620798375,
12.));
#181918=CARTESIAN_POINT('Ctrl Pts',(-13.3262148471226,-20.1294496158402,
12.));
#181919=CARTESIAN_POINT('Ctrl Pts',(-13.3310152130564,-20.1510440699474,
12.));
#181920=CARTESIAN_POINT('Ctrl Pts',(-13.3357810091903,-20.1727448403817,
12.));
#181921=CARTESIAN_POINT('Ctrl Pts',(-13.3405117354971,-20.1945513305235,
12.));
#181922=CARTESIAN_POINT('Ctrl Pts',(-13.3452068981766,-20.216462948786,
12.));
#181923=CARTESIAN_POINT('Ctrl Pts',(-13.3498660095386,-20.2384791085359,
12.));
#181924=CARTESIAN_POINT('Ctrl Pts',(-13.3544885878889,-20.2605992280122,
12.));
#181925=CARTESIAN_POINT('Ctrl Pts',(-13.3590741574195,-20.2828227302339,
12.));
#181926=CARTESIAN_POINT('Ctrl Pts',(-13.3636222481016,-20.3051490429048,
12.));
#181927=CARTESIAN_POINT('Ctrl Pts',(-13.3681323955826,-20.3275775983029,
12.));
#181928=CARTESIAN_POINT('Ctrl Pts',(-13.3726041410867,-20.3501078331814,
12.));
#181929=CARTESIAN_POINT('Ctrl Pts',(-13.3770370313188,-20.3727391887184,
12.));
#181930=CARTESIAN_POINT('Ctrl Pts',(-13.3814306183719,-20.3954711104502,
12.));
#181931=CARTESIAN_POINT('Ctrl Pts',(-13.3857844596387,-20.4183030482002,
12.));
#181932=CARTESIAN_POINT('Ctrl Pts',(-13.3900981177255,-20.4412344560007,
12.));
#181933=CARTESIAN_POINT('Ctrl Pts',(-13.3943711603739,-20.4642647920037,
12.));
#181934=CARTESIAN_POINT('Ctrl Pts',(-13.3986031603716,-20.487393518404,
12.));
#181935=CARTESIAN_POINT('Ctrl Pts',(-13.4027936954529,-20.5106201013753,
12.));
#181936=CARTESIAN_POINT('Ctrl Pts',(-13.4069423482076,-20.5339440109956,
12.));
#181937=CARTESIAN_POINT('Ctrl Pts',(-13.4110487059912,-20.5573647211639,
12.));
#181938=CARTESIAN_POINT('Ctrl Pts',(-13.4151123608411,-20.5808817095155,
12.));
#181939=CARTESIAN_POINT('Ctrl Pts',(-13.4191329093933,-20.6044944573153,
12.));
#181940=CARTESIAN_POINT('Ctrl Pts',(-13.4231099528179,-20.6282024494237,
12.));
#181941=CARTESIAN_POINT('Ctrl Pts',(-13.4270430967652,-20.6520051742869,
12.));
#181942=CARTESIAN_POINT('Ctrl Pts',(-13.4309319513119,-20.6759021239103,
12.));
#181943=CARTESIAN_POINT('Ctrl Pts',(-13.4347761309154,-20.6998927938288,
12.));
#181944=CARTESIAN_POINT('Ctrl Pts',(-13.4385752543663,-20.7239766830675,
12.));
#181945=CARTESIAN_POINT('Ctrl Pts',(-13.4423289447561,-20.7481532941013,
12.));
#181946=CARTESIAN_POINT('Ctrl Pts',(-13.4460368293688,-20.7724221327608,
12.));
#181947=CARTESIAN_POINT('Ctrl Pts',(-13.4496985395637,-20.7967827081227,
12.));
#181948=CARTESIAN_POINT('Ctrl Pts',(-13.4533137106667,-20.821234532398,
12.));
#181949=CARTESIAN_POINT('Ctrl Pts',(-13.4568819818631,-20.8457771208082,
12.));
#181950=CARTESIAN_POINT('Ctrl Pts',(-13.4604029960983,-20.8704099914641,
12.));
#181951=CARTESIAN_POINT('Ctrl Pts',(-13.4638763999726,-20.8951326652158,
12.));
#181952=CARTESIAN_POINT('Ctrl Pts',(-13.4673018437718,-20.9199446657584,
12.));
#181953=CARTESIAN_POINT('Ctrl Pts',(-13.4706789815167,-20.9448455197557,
12.));
#181954=CARTESIAN_POINT('Ctrl Pts',(-13.4740074710087,-20.9698347569476,
12.));
#181955=CARTESIAN_POINT('Ctrl Pts',(-13.4772869738879,-20.9949119102592,
12.));
#181956=CARTESIAN_POINT('Ctrl Pts',(-13.4805171556822,-21.0200765158885,
12.));
#181957=CARTESIAN_POINT('Ctrl Pts',(-13.4836976858912,-21.0453281134247,
12.));
#181958=CARTESIAN_POINT('Ctrl Pts',(-13.4868282377192,-21.0706662455202,
12.));
#181959=CARTESIAN_POINT('Ctrl Pts',(-13.4899084877718,-21.0960904575048,
12.));
#181960=CARTESIAN_POINT('Ctrl Pts',(-13.4929381157778,-21.1216002970209,
12.));
#181961=CARTESIAN_POINT('Ctrl Pts',(-13.4959168042934,-21.1471953136209,
12.));
#181962=CARTESIAN_POINT('Ctrl Pts',(-13.4988442384491,-21.1728750584173,
12.));
#181963=CARTESIAN_POINT('Ctrl Pts',(-13.5017201056088,-21.1986390835825,
12.));
#181964=CARTESIAN_POINT('Ctrl Pts',(-13.5045440957404,-21.224486942933,
12.));
#181965=CARTESIAN_POINT('Ctrl Pts',(-13.5073159019454,-21.2504181927429,
12.));
#181966=CARTESIAN_POINT('Ctrl Pts',(-13.5100352209207,-21.2764323924442,
12.));
#181967=CARTESIAN_POINT('Ctrl Pts',(-13.5127017534972,-21.3025291054236,
12.));
#181968=CARTESIAN_POINT('Ctrl Pts',(-13.5153152050554,-21.328707899634,
12.));
#181969=CARTESIAN_POINT('Ctrl Pts',(-13.5178752862461,-21.3549683486219,
12.));
#181970=CARTESIAN_POINT('Ctrl Pts',(-13.5203817122497,-21.3813100304967,
12.));
#181971=CARTESIAN_POINT('Ctrl Pts',(-13.5228342013508,-21.4077325259318,
12.));
#181972=CARTESIAN_POINT('Ctrl Pts',(-13.5252324737795,-21.4342354165253,
12.));
#181973=CARTESIAN_POINT('Ctrl Pts',(-13.5275762503553,-21.4608182828695,
12.));
#181974=CARTESIAN_POINT('Ctrl Pts',(-13.5298652514357,-21.487480703047,
12.));
#181975=CARTESIAN_POINT('Ctrl Pts',(-13.5320991952145,-21.5142222501671,
12.));
#181976=CARTESIAN_POINT('Ctrl Pts',(-13.5342777983225,-21.5410424932511,
12.));
#181977=CARTESIAN_POINT('Ctrl Pts',(-13.5364007790292,-21.5679410019011,
12.));
#181978=CARTESIAN_POINT('Ctrl Pts',(-13.5384678597206,-21.5949173499022,
12.));
#181979=CARTESIAN_POINT('Ctrl Pts',(-13.5404787697798,-21.6219711193951,
12.));
#181980=CARTESIAN_POINT('Ctrl Pts',(-13.5424332480698,-21.6491019044647,
12.));
#181981=CARTESIAN_POINT('Ctrl Pts',(-13.5443310461516,-21.676309315769,
12.));
#181982=CARTESIAN_POINT('Ctrl Pts',(-13.546171929503,-21.7035929822939,
12.));
#181983=CARTESIAN_POINT('Ctrl Pts',(-13.5479556704457,-21.730952541226,
12.));
#181984=CARTESIAN_POINT('Ctrl Pts',(-13.5496820422187,-21.7583876294532,
12.));
#181985=CARTESIAN_POINT('Ctrl Pts',(-13.5513508127232,-21.7858978745848,
12.));
#181986=CARTESIAN_POINT('Ctrl Pts',(-13.5529617381569,-21.8134828857963,
12.));
#181987=CARTESIAN_POINT('Ctrl Pts',(-13.5545145573049,-21.841142245609,
12.));
#181988=CARTESIAN_POINT('Ctrl Pts',(-13.5560089839426,-21.8688754989401,
12.));
#181989=CARTESIAN_POINT('Ctrl Pts',(-13.5574447178485,-21.8966821688876,
12.));
#181990=CARTESIAN_POINT('Ctrl Pts',(-13.5588214586672,-21.9245617765827,
12.));
#181991=CARTESIAN_POINT('Ctrl Pts',(-13.5601389185315,-21.9525138592862,
12.));
#181992=CARTESIAN_POINT('Ctrl Pts',(-13.5613968357589,-21.9805379899192,
12.));
#181993=CARTESIAN_POINT('Ctrl Pts',(-13.5625949868313,-22.0086337943431,
12.));
#181994=CARTESIAN_POINT('Ctrl Pts',(-13.5637332022393,-22.0368009736227,
12.));
#181995=CARTESIAN_POINT('Ctrl Pts',(-13.5648113688895,-22.0650393089492,
12.));
#181996=CARTESIAN_POINT('Ctrl Pts',(-13.5658294169107,-22.0933486464442,
12.));
#181997=CARTESIAN_POINT('Ctrl Pts',(-13.5667873105179,-22.1217288871823,
12.));
#181998=CARTESIAN_POINT('Ctrl Pts',(-13.5675054918922,-22.1444897575076,
12.));
#181999=CARTESIAN_POINT('Ctrl Pts',(-13.5680170531724,-22.1615922804939,
12.));
#182000=CARTESIAN_POINT('Ctrl Pts',(-13.5683460612913,-22.1730081264583,
12.));
#182001=CARTESIAN_POINT('Ctrl Pts',(-13.5685075571671,-22.1787195904339,
12.));
#182002=CARTESIAN_POINT('',(-12.4230808101438,-22.8400320311648,12.));
#182003=CARTESIAN_POINT('Origin',(0.,0.,12.));
#182004=CARTESIAN_POINT('',(-9.71462809124917,-20.353053841303,12.));
#182005=CARTESIAN_POINT('Ctrl Pts',(-12.4230808101438,-22.8400320311648,
12.));
#182006=CARTESIAN_POINT('Ctrl Pts',(-12.4182152851867,-22.8370364396497,
12.));
#182007=CARTESIAN_POINT('Ctrl Pts',(-12.4084933766366,-22.8310435872852,
12.));
#182008=CARTESIAN_POINT('Ctrl Pts',(-12.393937937903,-22.8220493007353,
12.));
#182009=CARTESIAN_POINT('Ctrl Pts',(-12.3745855366772,-22.8100469022632,
12.));
#182010=CARTESIAN_POINT('Ctrl Pts',(-12.3504864740361,-22.7950272216959,
12.));
#182011=CARTESIAN_POINT('Ctrl Pts',(-12.3264788926108,-22.7799908974947,
12.));
#182012=CARTESIAN_POINT('Ctrl Pts',(-12.3025628601812,-22.7649380101154,
12.));
#182013=CARTESIAN_POINT('Ctrl Pts',(-12.2787384750747,-22.7498686970096,
12.));
#182014=CARTESIAN_POINT('Ctrl Pts',(-12.2550058702389,-22.7347831655251,
12.));
#182015=CARTESIAN_POINT('Ctrl Pts',(-12.2313652198047,-22.7196817119299,
12.));
#182016=CARTESIAN_POINT('Ctrl Pts',(-12.2078167360267,-22.7045647168659,
12.));
#182017=CARTESIAN_POINT('Ctrl Pts',(-12.1843606579246,-22.6894326204959,
12.));
#182018=CARTESIAN_POINT('Ctrl Pts',(-12.1609972423089,-22.6742859034891,
12.));
#182019=CARTESIAN_POINT('Ctrl Pts',(-12.1377267537141,-22.6591250653942,
12.));
#182020=CARTESIAN_POINT('Ctrl Pts',(-12.1145494550384,-22.6439506046611,
12.));
#182021=CARTESIAN_POINT('Ctrl Pts',(-12.0914655972828,-22.628762996708,
12.));
#182022=CARTESIAN_POINT('Ctrl Pts',(-12.0684754113869,-22.613562676493,
12.));
#182023=CARTESIAN_POINT('Ctrl Pts',(-12.0455791139135,-22.5983500505675,
12.));
#182024=CARTESIAN_POINT('Ctrl Pts',(-12.0227769113132,-22.5831255061306,
12.));
#182025=CARTESIAN_POINT('Ctrl Pts',(-12.0000690046697,-22.5678894211194,
12.));
#182026=CARTESIAN_POINT('Ctrl Pts',(-11.9774555943496,-22.5526421741159,
12.));
#182027=CARTESIAN_POINT('Ctrl Pts',(-11.9549368843996,-22.5373841537299,
12.));
#182028=CARTESIAN_POINT('Ctrl Pts',(-11.9325130877801,-22.5221157697869,
12.));
#182029=CARTESIAN_POINT('Ctrl Pts',(-11.9101844254555,-22.5068374513958,
12.));
#182030=CARTESIAN_POINT('Ctrl Pts',(-11.8879511239941,-22.4915496418472,
12.));
#182031=CARTESIAN_POINT('Ctrl Pts',(-11.8658134137018,-22.4762527946694,
12.));
#182032=CARTESIAN_POINT('Ctrl Pts',(-11.8437715264487,-22.4609473690469,
12.));
#182033=CARTESIAN_POINT('Ctrl Pts',(-11.8218256937889,-22.4456338258738,
12.));
#182034=CARTESIAN_POINT('Ctrl Pts',(-11.7999761445175,-22.4303126226468,
12.));
#182035=CARTESIAN_POINT('Ctrl Pts',(-11.7782231042041,-22.4149842125018,
12.));
#182036=CARTESIAN_POINT('Ctrl Pts',(-11.7565667964765,-22.39964904692,12.));
#182037=CARTESIAN_POINT('Ctrl Pts',(-11.7350074437961,-22.3843075773905,
12.));
#182038=CARTESIAN_POINT('Ctrl Pts',(-11.7135452684532,-22.3689602575492,
12.));
#182039=CARTESIAN_POINT('Ctrl Pts',(-11.6921804934056,-22.3536075450028,
12.));
#182040=CARTESIAN_POINT('Ctrl Pts',(-11.6709133432986,-22.3382499035618,
12.));
#182041=CARTESIAN_POINT('Ctrl Pts',(-11.6497440449858,-22.3228878043976,
12.));
#182042=CARTESIAN_POINT('Ctrl Pts',(-11.6286728270011,-22.3075217249049,
12.));
#182043=CARTESIAN_POINT('Ctrl Pts',(-11.6076999192359,-22.2921521480357,
12.));
#182044=CARTESIAN_POINT('Ctrl Pts',(-11.5868255525189,-22.2767795614349,
12.));
#182045=CARTESIAN_POINT('Ctrl Pts',(-11.5660499582403,-22.2614044566898,
12.));
#182046=CARTESIAN_POINT('Ctrl Pts',(-11.545373367912,-22.2460273284653,
12.));
#182047=CARTESIAN_POINT('Ctrl Pts',(-11.5247960128476,-22.2306486738899,
12.));
#182048=CARTESIAN_POINT('Ctrl Pts',(-11.504318124424,-22.215268993102,12.));
#182049=CARTESIAN_POINT('Ctrl Pts',(-11.4839399342589,-22.1998887896435,
12.));
#182050=CARTESIAN_POINT('Ctrl Pts',(-11.463661674411,-22.1845085709169,
12.));
#182051=CARTESIAN_POINT('Ctrl Pts',(-11.443483577557,-22.1691288486096,
12.));
#182052=CARTESIAN_POINT('Ctrl Pts',(-11.4234058771742,-22.1537501391486,
12.));
#182053=CARTESIAN_POINT('Ctrl Pts',(-11.4034288076909,-22.1383729640963,
12.));
#182054=CARTESIAN_POINT('Ctrl Pts',(-11.3835526044256,-22.1229978500185,
12.));
#182055=CARTESIAN_POINT('Ctrl Pts',(-11.3637775035367,-22.1076253283978,
12.));
#182056=CARTESIAN_POINT('Ctrl Pts',(-11.3441037419553,-22.0922559355293,
12.));
#182057=CARTESIAN_POINT('Ctrl Pts',(-11.3245315573168,-22.0768902124267,
12.));
#182058=CARTESIAN_POINT('Ctrl Pts',(-11.3050611878771,-22.0615287047179,
12.));
#182059=CARTESIAN_POINT('Ctrl Pts',(-11.2856928724374,-22.046171962566,
12.));
#182060=CARTESIAN_POINT('Ctrl Pts',(-11.2664268504207,-22.0308205408351,
12.));
#182061=CARTESIAN_POINT('Ctrl Pts',(-11.2472633619276,-22.0154749992364,
12.));
#182062=CARTESIAN_POINT('Ctrl Pts',(-11.2282026477897,-22.0001359024839,
12.));
#182063=CARTESIAN_POINT('Ctrl Pts',(-11.2092449496125,-21.9848038204439,
12.));
#182064=CARTESIAN_POINT('Ctrl Pts',(-11.190390509811,-21.9694793282913,
12.));
#182065=CARTESIAN_POINT('Ctrl Pts',(-11.1716395716375,-21.9541630066504,
12.));
#182066=CARTESIAN_POINT('Ctrl Pts',(-11.1529923792002,-21.9388554416437,
12.));
#182067=CARTESIAN_POINT('Ctrl Pts',(-11.134449177474,-21.9235572249518,
12.));
#182068=CARTESIAN_POINT('Ctrl Pts',(-11.1160102123024,-21.9082689538687,
12.));
#182069=CARTESIAN_POINT('Ctrl Pts',(-11.0976757303944,-21.8929912313608,
12.));
#182070=CARTESIAN_POINT('Ctrl Pts',(-11.0794459793058,-21.8777246661191,
12.));
#182071=CARTESIAN_POINT('Ctrl Pts',(-11.0613212074364,-21.8624698726319,
12.));
#182072=CARTESIAN_POINT('Ctrl Pts',(-11.0433016640808,-21.8472274713103,
12.));
#182073=CARTESIAN_POINT('Ctrl Pts',(-11.0253875994598,-21.8319980886033,
12.));
#182074=CARTESIAN_POINT('Ctrl Pts',(-11.0075792647477,-21.8167823571168,
12.));
#182075=CARTESIAN_POINT('Ctrl Pts',(-10.9898769120913,-21.8015809157302,
12.));
#182076=CARTESIAN_POINT('Ctrl Pts',(-10.9722807946157,-21.7863944097143,
12.));
#182077=CARTESIAN_POINT('Ctrl Pts',(-10.9547911664457,-21.7712234908468,
12.));
#182078=CARTESIAN_POINT('Ctrl Pts',(-10.9374082827446,-21.7560688175252,
12.));
#182079=CARTESIAN_POINT('Ctrl Pts',(-10.9201323997386,-21.74093105488,12.));
#182080=CARTESIAN_POINT('Ctrl Pts',(-10.9029637747341,-21.7258108748874,
12.));
#182081=CARTESIAN_POINT('Ctrl Pts',(-10.8859026661292,-21.7107089564822,
12.));
#182082=CARTESIAN_POINT('Ctrl Pts',(-10.8689493334093,-21.6956259856667,
12.));
#182083=CARTESIAN_POINT('Ctrl Pts',(-10.8521040371832,-21.6805626556461,
12.));
#182084=CARTESIAN_POINT('Ctrl Pts',(-10.835367039227,-21.6655196669727,
12.));
#182085=CARTESIAN_POINT('Ctrl Pts',(-10.8187386025135,-21.6504977276864,
12.));
#182086=CARTESIAN_POINT('Ctrl Pts',(-10.802218991237,-21.6354975534557,
12.));
#182087=CARTESIAN_POINT('Ctrl Pts',(-10.7858084708262,-21.6205198677176,
12.));
#182088=CARTESIAN_POINT('Ctrl Pts',(-10.7695073079554,-21.6055654018179,
12.));
#182089=CARTESIAN_POINT('Ctrl Pts',(-10.7533157705943,-21.5906348951745,
12.));
#182090=CARTESIAN_POINT('Ctrl Pts',(-10.7372341280468,-21.5757290954372,
12.));
#182091=CARTESIAN_POINT('Ctrl Pts',(-10.7212626509816,-21.5608487586467,
12.));
#182092=CARTESIAN_POINT('Ctrl Pts',(-10.7054016114571,-21.5459946493955,
12.));
#182093=CARTESIAN_POINT('Ctrl Pts',(-10.689651282929,-21.531167540981,12.));
#182094=CARTESIAN_POINT('Ctrl Pts',(-10.6740119402835,-21.5163682155805,
12.));
#182095=CARTESIAN_POINT('Ctrl Pts',(-10.6584838598941,-21.5015974644454,
12.));
#182096=CARTESIAN_POINT('Ctrl Pts',(-10.6430673196609,-21.4868560880893,
12.));
#182097=CARTESIAN_POINT('Ctrl Pts',(-10.6277625990457,-21.4721448964766,
12.));
#182098=CARTESIAN_POINT('Ctrl Pts',(-10.612569979096,-21.4574647092093,
12.));
#182099=CARTESIAN_POINT('Ctrl Pts',(-10.597489742462,-21.4428163557137,
12.));
#182100=CARTESIAN_POINT('Ctrl Pts',(-10.582522173457,-21.4282006754624,
12.));
#182101=CARTESIAN_POINT('Ctrl Pts',(-10.5676675581106,-21.4136185181974,
12.));
#182102=CARTESIAN_POINT('Ctrl Pts',(-10.5529261842107,-21.3990707441495,
12.));
#182103=CARTESIAN_POINT('Ctrl Pts',(-10.5382983413422,-21.3845582242604,
12.));
#182104=CARTESIAN_POINT('Ctrl Pts',(-10.523784320906,-21.3700818403942,
12.));
#182105=CARTESIAN_POINT('Ctrl Pts',(-10.509384416169,-21.3556424855822,
12.));
#182106=CARTESIAN_POINT('Ctrl Pts',(-10.4950989223341,-21.3412410642912,
12.));
#182107=CARTESIAN_POINT('Ctrl Pts',(-10.4809281365933,-21.3268784926823,
12.));
#182108=CARTESIAN_POINT('Ctrl Pts',(-10.4668723581768,-21.312555698873,
12.));
#182109=CARTESIAN_POINT('Ctrl Pts',(-10.452931888387,-21.2982736231924,
12.));
#182110=CARTESIAN_POINT('Ctrl Pts',(-10.4391070306385,-21.2840332184471,
12.));
#182111=CARTESIAN_POINT('Ctrl Pts',(-10.4253980905394,-21.2698354502391,
12.));
#182112=CARTESIAN_POINT('Ctrl Pts',(-10.4118053759584,-21.2556812972741,
12.));
#182113=CARTESIAN_POINT('Ctrl Pts',(-10.3983291970846,-21.2415717516713,
12.));
#182114=CARTESIAN_POINT('Ctrl Pts',(-10.384969866479,-21.2275078192708,
12.));
#182115=CARTESIAN_POINT('Ctrl Pts',(-10.3717276991137,-21.2134905199359,
12.));
#182116=CARTESIAN_POINT('Ctrl Pts',(-10.3586030124595,-21.1995208879205,
12.));
#182117=CARTESIAN_POINT('Ctrl Pts',(-10.3455961265706,-21.1855999722427,
12.));
#182118=CARTESIAN_POINT('Ctrl Pts',(-10.3327073641574,-21.1717288370512,
12.));
#182119=CARTESIAN_POINT('Ctrl Pts',(-10.3199370506541,-21.1579085619959,
12.));
#182120=CARTESIAN_POINT('Ctrl Pts',(-10.307285514268,-21.1441402425831,
12.));
#182121=CARTESIAN_POINT('Ctrl Pts',(-10.2947530860714,-21.130424990599,
12.));
#182122=CARTESIAN_POINT('Ctrl Pts',(-10.2823401001067,-21.1167639345623,
12.));
#182123=CARTESIAN_POINT('Ctrl Pts',(-10.2700468934743,-21.1031582201625,
12.));
#182124=CARTESIAN_POINT('Ctrl Pts',(-10.2578738064183,-21.0896090107066,
12.));
#182125=CARTESIAN_POINT('Ctrl Pts',(-10.2458211823915,-21.0761174875448,
12.));
#182126=CARTESIAN_POINT('Ctrl Pts',(-10.233889368157,-21.0626848505665,
12.));
#182127=CARTESIAN_POINT('Ctrl Pts',(-10.2220787139157,-21.0493123187483,
12.));
#182128=CARTESIAN_POINT('Ctrl Pts',(-10.2103895734124,-21.0360011306814,
12.));
#182129=CARTESIAN_POINT('Ctrl Pts',(-10.1988223040425,-21.0227525451107,
12.));
#182130=CARTESIAN_POINT('Ctrl Pts',(-10.1873772669358,-21.0095678414486,
12.));
#182131=CARTESIAN_POINT('Ctrl Pts',(-10.1760548270765,-20.9964483203685,
12.));
#182132=CARTESIAN_POINT('Ctrl Pts',(-10.1648553534567,-20.9833953044736,
12.));
#182133=CARTESIAN_POINT('Ctrl Pts',(-10.1537792192065,-20.970410138937,
12.));
#182134=CARTESIAN_POINT('Ctrl Pts',(-10.1428268017257,-20.9574941921591,
12.));
#182135=CARTESIAN_POINT('Ctrl Pts',(-10.1319984827909,-20.944648856393,
12.));
#182136=CARTESIAN_POINT('Ctrl Pts',(-10.1212946487057,-20.931875548473,
12.));
#182137=CARTESIAN_POINT('Ctrl Pts',(-10.1107156904836,-20.9191757106266,
12.));
#182138=CARTESIAN_POINT('Ctrl Pts',(-10.1002620040076,-20.9065508112556,
12.));
#182139=CARTESIAN_POINT('Ctrl Pts',(-10.0899339901916,-20.8940023457371,
12.));
#182140=CARTESIAN_POINT('Ctrl Pts',(-10.0797320551154,-20.8815318371844,
12.));
#182141=CARTESIAN_POINT('Ctrl Pts',(-10.0696566102219,-20.8691408373705,
12.));
#182142=CARTESIAN_POINT('Ctrl Pts',(-10.0597080725375,-20.856830927732,
12.));
#182143=CARTESIAN_POINT('Ctrl Pts',(-10.0498868648733,-20.8446037203402,
12.));
#182144=CARTESIAN_POINT('Ctrl Pts',(-10.0401934160234,-20.8324608588906,
12.));
#182145=CARTESIAN_POINT('Ctrl Pts',(-10.0306281609435,-20.8204040196599,
12.));
#182146=CARTESIAN_POINT('Ctrl Pts',(-10.0211915410095,-20.8084349126885,
12.));
#182147=CARTESIAN_POINT('Ctrl Pts',(-10.0118840042786,-20.7965552829907,
12.));
#182148=CARTESIAN_POINT('Ctrl Pts',(-10.0027060057389,-20.7847669117568,
12.));
#182149=CARTESIAN_POINT('Ctrl Pts',(-9.99365800754638,-20.7730716175417,
12.));
#182150=CARTESIAN_POINT('Ctrl Pts',(-9.98474047926846,-20.7614712574989,
12.));
#182151=CARTESIAN_POINT('Ctrl Pts',(-9.97595389823461,-20.7499677289625,
12.));
#182152=CARTESIAN_POINT('Ctrl Pts',(-9.96729874986199,-20.7385629709795,
12.));
#182153=CARTESIAN_POINT('Ctrl Pts',(-9.95877552798403,-20.7272589658752,
12.));
#182154=CARTESIAN_POINT('Ctrl Pts',(-9.95038473514962,-20.716057740758,
12.));
#182155=CARTESIAN_POINT('Ctrl Pts',(-9.94212688298251,-20.7049613692237,
12.));
#182156=CARTESIAN_POINT('Ctrl Pts',(-9.93400249259737,-20.6939719732485,
12.));
#182157=CARTESIAN_POINT('Ctrl Pts',(-9.92601209498751,-20.6830917250255,
12.));
#182158=CARTESIAN_POINT('Ctrl Pts',(-9.91815623141285,-20.6723228488261,
12.));
#182159=CARTESIAN_POINT('Ctrl Pts',(-9.91043545377005,-20.6616676228315,
12.));
#182160=CARTESIAN_POINT('Ctrl Pts',(-9.90285032516696,-20.6511283817415,
12.));
#182161=CARTESIAN_POINT('Ctrl Pts',(-9.89540142049124,-20.6407075193977,
12.));
#182162=CARTESIAN_POINT('Ctrl Pts',(-9.88808932697305,-20.6304074914086,
12.));
#182163=CARTESIAN_POINT('Ctrl Pts',(-9.88091464472669,-20.6202308177472,
12.));
#182164=CARTESIAN_POINT('Ctrl Pts',(-9.87387798732944,-20.6101800854491,
12.));
#182165=CARTESIAN_POINT('Ctrl Pts',(-9.86697998242612,-20.6002579513696,
12.));
#182166=CARTESIAN_POINT('Ctrl Pts',(-9.8602212723275,-20.5904671449754,
12.));
#182167=CARTESIAN_POINT('Ctrl Pts',(-9.85360251457004,-20.580810471002,
12.));
#182168=CARTESIAN_POINT('Ctrl Pts',(-9.84712438256308,-20.5712908125145,
12.));
#182169=CARTESIAN_POINT('Ctrl Pts',(-9.84078756677589,-20.5619111362406,
12.));
#182170=CARTESIAN_POINT('Ctrl Pts',(-9.83459277585321,-20.5526744976461,
12.));
#182171=CARTESIAN_POINT('Ctrl Pts',(-9.82854073773858,-20.5435840460717,
12.));
#182172=CARTESIAN_POINT('Ctrl Pts',(-9.82263220080328,-20.534643029951,
12.));
#182173=CARTESIAN_POINT('Ctrl Pts',(-9.81686793455918,-20.5258548000625,
12.));
#182174=CARTESIAN_POINT('Ctrl Pts',(-9.81124873025278,-20.5172228122839,
12.));
#182175=CARTESIAN_POINT('Ctrl Pts',(-9.80577540161103,-20.5087506310507,
12.));
#182176=CARTESIAN_POINT('Ctrl Pts',(-9.80044878520968,-20.500441931211,
12.));
#182177=CARTESIAN_POINT('Ctrl Pts',(-9.79526974288344,-20.4923005087945,
12.));
#182178=CARTESIAN_POINT('Ctrl Pts',(-9.7902391649866,-20.4843302955329,
12.));
#182179=CARTESIAN_POINT('Ctrl Pts',(-9.78535797314162,-20.4765353711585,
12.));
#182180=CARTESIAN_POINT('Ctrl Pts',(-9.78062712373313,-20.4689199790668,
12.));
#182181=CARTESIAN_POINT('Ctrl Pts',(-9.77604760815523,-20.4614885274973,
12.));
#182182=CARTESIAN_POINT('Ctrl Pts',(-9.7716204510407,-20.4542455817527,
12.));
#182183=CARTESIAN_POINT('Ctrl Pts',(-9.76734670980897,-20.447195862298,
12.));
#182184=CARTESIAN_POINT('Ctrl Pts',(-9.76322747195502,-20.4403442329401,
12.));
#182185=CARTESIAN_POINT('Ctrl Pts',(-9.7592638628993,-20.4336957355474,
12.));
#182186=CARTESIAN_POINT('Ctrl Pts',(-9.75545705902416,-20.4272556476629,
12.));
#182187=CARTESIAN_POINT('Ctrl Pts',(-9.75180829786433,-20.4210295275818,
12.));
#182188=CARTESIAN_POINT('Ctrl Pts',(-9.74831889242175,-20.4150232777393,
12.));
#182189=CARTESIAN_POINT('Ctrl Pts',(-9.74499021838537,-20.4092430879861,
12.));
#182190=CARTESIAN_POINT('Ctrl Pts',(-9.74182369656273,-20.4036953576549,
12.));
#182191=CARTESIAN_POINT('Ctrl Pts',(-9.73882077613206,-20.3983866213331,
12.));
#182192=CARTESIAN_POINT('Ctrl Pts',(-9.7359829201425,-20.3933234845646,
12.));
#182193=CARTESIAN_POINT('Ctrl Pts',(-9.73331167102812,-20.3885129129912,
12.));
#182194=CARTESIAN_POINT('Ctrl Pts',(-9.73080870123726,-20.3839624556742,
12.));
#182195=CARTESIAN_POINT('Ctrl Pts',(-9.72847589116533,-20.3796805893304,
12.));
#182196=CARTESIAN_POINT('Ctrl Pts',(-9.72631531732871,-20.3756766651952,
12.));
#182197=CARTESIAN_POINT('Ctrl Pts',(-9.72432910043193,-20.371960235676,
12.));
#182198=CARTESIAN_POINT('Ctrl Pts',(-9.72251930722504,-20.3685406190576,
12.));
#182199=CARTESIAN_POINT('Ctrl Pts',(-9.72088778381102,-20.3654261611055,
12.));
#182200=CARTESIAN_POINT('Ctrl Pts',(-9.71943648548115,-20.362625691398,
12.));
#182201=CARTESIAN_POINT('Ctrl Pts',(-9.71816778327999,-20.3601498764344,
12.));
#182202=CARTESIAN_POINT('Ctrl Pts',(-9.71708493723062,-20.3580133103357,
12.));
#182203=CARTESIAN_POINT('Ctrl Pts',(-9.71619192554147,-20.3562337557875,
12.));
#182204=CARTESIAN_POINT('Ctrl Pts',(-9.71549257088175,-20.3548282742361,
12.));
#182205=CARTESIAN_POINT('Ctrl Pts',(-9.71498978052101,-20.3538098605706,
12.));
#182206=CARTESIAN_POINT('Ctrl Pts',(-9.71474590350792,-20.3533097561886,
12.));
#182207=CARTESIAN_POINT('Ctrl Pts',(-9.71465227853122,-20.3531126095522,
12.));
#182208=CARTESIAN_POINT('Ctrl Pts',(-9.71462954053074,-20.353060251684,
12.));
#182209=CARTESIAN_POINT('Ctrl Pts',(-9.71462809124917,-20.353053841303,
12.));
#182210=CARTESIAN_POINT('',(-9.47413589477549,-19.84920021178,12.));
#182211=CARTESIAN_POINT('',(-4.63060338698782,-9.70154690100589,12.));
#182212=CARTESIAN_POINT('',(-8.81783521984851,-19.6085639972844,12.));
#182213=CARTESIAN_POINT('Origin',(-9.02290115519382,-20.0645771135003,12.));
#182214=CARTESIAN_POINT('',(-7.63019749246979,-20.1004996511507,12.));
#182215=CARTESIAN_POINT('Origin',(-3.26562511982935E-13,-7.08841632778409E-13,
12.));
#182216=CARTESIAN_POINT('',(-7.33627833380047,-20.7347298079577,12.));
#182217=CARTESIAN_POINT('Origin',(-7.80764394578304,-20.56795313141,12.));
#182218=CARTESIAN_POINT('',(-7.52250298901266,-21.2610617890679,12.));
#182219=CARTESIAN_POINT('',(-3.76125149450632,-10.6305308945339,12.));
#182220=CARTESIAN_POINT('',(-7.36589684767345,-24.9347862158358,12.));
#182221=CARTESIAN_POINT('Ctrl Pts',(-7.52250298901266,-21.2610617890679,
12.));
#182222=CARTESIAN_POINT('Ctrl Pts',(-7.52250649703992,-21.2610673466883,
12.));
#182223=CARTESIAN_POINT('Ctrl Pts',(-7.52252744144958,-21.261120447486,
12.));
#182224=CARTESIAN_POINT('Ctrl Pts',(-7.52260064231736,-21.2613260540651,
12.));
#182225=CARTESIAN_POINT('Ctrl Pts',(-7.52278182242728,-21.261852128355,
12.));
#182226=CARTESIAN_POINT('Ctrl Pts',(-7.52314642316203,-21.262927782038,
12.));
#182227=CARTESIAN_POINT('Ctrl Pts',(-7.52364573027521,-21.2644161259965,
12.));
#182228=CARTESIAN_POINT('Ctrl Pts',(-7.52427261074264,-21.266305915706,
12.));
#182229=CARTESIAN_POINT('Ctrl Pts',(-7.52501770333522,-21.2685823838672,
12.));
#182230=CARTESIAN_POINT('Ctrl Pts',(-7.52587126095544,-21.2712301573465,
12.));
#182231=CARTESIAN_POINT('Ctrl Pts',(-7.52682526918561,-21.2742366113578,
12.));
#182232=CARTESIAN_POINT('Ctrl Pts',(-7.52787386225344,-21.2775925269651,
12.));
#182233=CARTESIAN_POINT('Ctrl Pts',(-7.52901217930407,-21.2812902781143,
12.));
#182234=CARTESIAN_POINT('Ctrl Pts',(-7.53023562438221,-21.2853226580658,
12.));
#182235=CARTESIAN_POINT('Ctrl Pts',(-7.53153906987847,-21.2896816163843,
12.));
#182236=CARTESIAN_POINT('Ctrl Pts',(-7.53291726078527,-21.2943588989331,
12.));
#182237=CARTESIAN_POINT('Ctrl Pts',(-7.53436505309949,-21.2993464250717,
12.));
#182238=CARTESIAN_POINT('Ctrl Pts',(-7.53587778251743,-21.3046368712156,
12.));
#182239=CARTESIAN_POINT('Ctrl Pts',(-7.5374512936462,-21.3102237167729,
12.));
#182240=CARTESIAN_POINT('Ctrl Pts',(-7.53908175169899,-21.3161009456256,
12.));
#182241=CARTESIAN_POINT('Ctrl Pts',(-7.5407655203828,-21.3222628524165,
12.));
#182242=CARTESIAN_POINT('Ctrl Pts',(-7.54249900377032,-21.328703791771,
12.));
#182243=CARTESIAN_POINT('Ctrl Pts',(-7.54427868151269,-21.3354182340149,
12.));
#182244=CARTESIAN_POINT('Ctrl Pts',(-7.54610114948351,-21.3424008295038,
12.));
#182245=CARTESIAN_POINT('Ctrl Pts',(-7.54796316246327,-21.349646476153,
12.));
#182246=CARTESIAN_POINT('Ctrl Pts',(-7.54986166521307,-21.3571503685853,
12.));
#182247=CARTESIAN_POINT('Ctrl Pts',(-7.55179375777442,-21.3649079431864,
12.));
#182248=CARTESIAN_POINT('Ctrl Pts',(-7.55375667080032,-21.3729148390244,
12.));
#182249=CARTESIAN_POINT('Ctrl Pts',(-7.55574773403508,-21.3811668478933,
12.));
#182250=CARTESIAN_POINT('Ctrl Pts',(-7.55776435731422,-21.3896598842119,
12.));
#182251=CARTESIAN_POINT('Ctrl Pts',(-7.55980403700615,-21.3983899952988,
12.));
#182252=CARTESIAN_POINT('Ctrl Pts',(-7.56186435703622,-21.4073533630364,
12.));
#182253=CARTESIAN_POINT('Ctrl Pts',(-7.56394299313683,-21.4165463106252,
12.));
#182254=CARTESIAN_POINT('Ctrl Pts',(-7.56603771218706,-21.4259653015732,
12.));
#182255=CARTESIAN_POINT('Ctrl Pts',(-7.56814636360842,-21.435606926151,
12.));
#182256=CARTESIAN_POINT('Ctrl Pts',(-7.5702668726117,-21.445467890751,12.));
#182257=CARTESIAN_POINT('Ctrl Pts',(-7.57239723223521,-21.4555450053147,
12.));
#182258=CARTESIAN_POINT('Ctrl Pts',(-7.57453549743435,-21.4658351740135,
12.));
#182259=CARTESIAN_POINT('Ctrl Pts',(-7.57667978403003,-21.4763353936766,
12.));
#182260=CARTESIAN_POINT('Ctrl Pts',(-7.57882826679131,-21.4870427508193,
12.));
#182261=CARTESIAN_POINT('Ctrl Pts',(-7.5809791779073,-21.4979544192739,
12.));
#182262=CARTESIAN_POINT('Ctrl Pts',(-7.58313080519159,-21.5090676573866,
12.));
#182263=CARTESIAN_POINT('Ctrl Pts',(-7.58528148919114,-21.5203798035294,
12.));
#182264=CARTESIAN_POINT('Ctrl Pts',(-7.58742962034834,-21.5318882716735,
12.));
#182265=CARTESIAN_POINT('Ctrl Pts',(-7.58957363620026,-21.5435905470113,
12.));
#182266=CARTESIAN_POINT('Ctrl Pts',(-7.59171201844793,-21.5554841813465,
12.));
#182267=CARTESIAN_POINT('Ctrl Pts',(-7.5938432912493,-21.5675667904728,
12.));
#182268=CARTESIAN_POINT('Ctrl Pts',(-7.59596601973589,-21.5798360518978,
12.));
#182269=CARTESIAN_POINT('Ctrl Pts',(-7.59807880846193,-21.5922897024466,
12.));
#182270=CARTESIAN_POINT('Ctrl Pts',(-7.60018029988238,-21.6049255358842,
12.));
#182271=CARTESIAN_POINT('Ctrl Pts',(-7.60226917285432,-21.6177414005991,
12.));
#182272=CARTESIAN_POINT('Ctrl Pts',(-7.604344141183,-21.6307351973823,12.));
#182273=CARTESIAN_POINT('Ctrl Pts',(-7.60640395216359,-21.6439048771743,
12.));
#182274=CARTESIAN_POINT('Ctrl Pts',(-7.60844738512872,-21.6572484388079,
12.));
#182275=CARTESIAN_POINT('Ctrl Pts',(-7.6104732500095,-21.6707639267573,
12.));
#182276=CARTESIAN_POINT('Ctrl Pts',(-7.61248038630265,-21.6844494295813,
12.));
#182277=CARTESIAN_POINT('Ctrl Pts',(-7.61446766202787,-21.6983030783321,
12.));
#182278=CARTESIAN_POINT('Ctrl Pts',(-7.61643397270425,-21.7123230449835,
12.));
#182279=CARTESIAN_POINT('Ctrl Pts',(-7.61837824030542,-21.7265075407977,
12.));
#182280=CARTESIAN_POINT('Ctrl Pts',(-7.62029941230855,-21.7408548148657,
12.));
#182281=CARTESIAN_POINT('Ctrl Pts',(-7.62219646084226,-21.7553631528329,
12.));
#182282=CARTESIAN_POINT('Ctrl Pts',(-7.62406838181164,-21.7700308755583,
12.));
#182283=CARTESIAN_POINT('Ctrl Pts',(-7.62591419404521,-21.7848563378022,
12.));
#182284=CARTESIAN_POINT('Ctrl Pts',(-7.62773293842409,-21.7998379268583,
12.));
#182285=CARTESIAN_POINT('Ctrl Pts',(-7.62952367718151,-21.8149740615093,
12.));
#182286=CARTESIAN_POINT('Ctrl Pts',(-7.6312854932304,-21.8302631910197,
12.));
#182287=CARTESIAN_POINT('Ctrl Pts',(-7.63301748948936,-21.8457037941084,
12.));
#182288=CARTESIAN_POINT('Ctrl Pts',(-7.63471878821204,-21.8612943779086,
12.));
#182289=CARTESIAN_POINT('Ctrl Pts',(-7.63638853033368,-21.8770334769492,
12.));
#182290=CARTESIAN_POINT('Ctrl Pts',(-7.63802587492008,-21.8929196523511,
12.));
#182291=CARTESIAN_POINT('Ctrl Pts',(-7.63962999860917,-21.9089514909873,
12.));
#182292=CARTESIAN_POINT('Ctrl Pts',(-7.6412000950654,-21.9251276046546,
12.));
#182293=CARTESIAN_POINT('Ctrl Pts',(-7.64273537442707,-21.9414466292074,
12.));
#182294=CARTESIAN_POINT('Ctrl Pts',(-7.64423506279154,-21.9579072237653,
12.));
#182295=CARTESIAN_POINT('Ctrl Pts',(-7.64569840177359,-21.97450807008,12.));
#182296=CARTESIAN_POINT('Ctrl Pts',(-7.64712464805258,-21.9912478718542,
12.));
#182297=CARTESIAN_POINT('Ctrl Pts',(-7.64851307293346,-22.0081253540773,
12.));
#182298=CARTESIAN_POINT('Ctrl Pts',(-7.64986296190157,-22.0251392623209,
12.));
#182299=CARTESIAN_POINT('Ctrl Pts',(-7.65117361421347,-22.0422883621176,
12.));
#182300=CARTESIAN_POINT('Ctrl Pts',(-7.65244434253104,-22.0595714384432,
12.));
#182301=CARTESIAN_POINT('Ctrl Pts',(-7.65367447254945,-22.0769872951596,
12.));
#182302=CARTESIAN_POINT('Ctrl Pts',(-7.65486334263651,-22.094534754469,
12.));
#182303=CARTESIAN_POINT('Ctrl Pts',(-7.65601030346819,-22.1122126563327,
12.));
#182304=CARTESIAN_POINT('Ctrl Pts',(-7.65711471769407,-22.1300198579671,
12.));
#182305=CARTESIAN_POINT('Ctrl Pts',(-7.65817595963351,-22.1479552334206,
12.));
#182306=CARTESIAN_POINT('Ctrl Pts',(-7.65919341496926,-22.1660176731174,
12.));
#182307=CARTESIAN_POINT('Ctrl Pts',(-7.66016648045008,-22.1842060834092,
12.));
#182308=CARTESIAN_POINT('Ctrl Pts',(-7.66109456359292,-22.2025193860972,
12.));
#182309=CARTESIAN_POINT('Ctrl Pts',(-7.66197708240436,-22.2209565180098,
12.));
#182310=CARTESIAN_POINT('Ctrl Pts',(-7.66281346512546,-22.239516430656,
12.));
#182311=CARTESIAN_POINT('Ctrl Pts',(-7.66360314997662,-22.2581980898487,
12.));
#182312=CARTESIAN_POINT('Ctrl Pts',(-7.66434558490973,-22.2770004753332,
12.));
#182313=CARTESIAN_POINT('Ctrl Pts',(-7.66504022736263,-22.2959225803925,
12.));
#182314=CARTESIAN_POINT('Ctrl Pts',(-7.66568654402442,-22.3149634114823,
12.));
#182315=CARTESIAN_POINT('Ctrl Pts',(-7.66628401061906,-22.3341219879454,
12.));
#182316=CARTESIAN_POINT('Ctrl Pts',(-7.66683211169134,-22.3533973417013,
12.));
#182317=CARTESIAN_POINT('Ctrl Pts',(-7.66733034039887,-22.3727885169361,
12.));
#182318=CARTESIAN_POINT('Ctrl Pts',(-7.6677781983082,-22.3922945697782,
12.));
#182319=CARTESIAN_POINT('Ctrl Pts',(-7.66817519519682,-22.411914567977,
12.));
#182320=CARTESIAN_POINT('Ctrl Pts',(-7.66852084886746,-22.4316475906616,
12.));
#182321=CARTESIAN_POINT('Ctrl Pts',(-7.6688146849666,-22.4514927280862,
12.));
#182322=CARTESIAN_POINT('Ctrl Pts',(-7.66905623680836,-22.47144908137,12.));
#182323=CARTESIAN_POINT('Ctrl Pts',(-7.66924504520302,-22.4915157622308,
12.));
#182324=CARTESIAN_POINT('Ctrl Pts',(-7.66938065829083,-22.5116918927023,
12.));
#182325=CARTESIAN_POINT('Ctrl Pts',(-7.66946263138116,-22.5319766049191,
12.));
#182326=CARTESIAN_POINT('Ctrl Pts',(-7.66949052679672,-22.5523690409109,
12.));
#182327=CARTESIAN_POINT('Ctrl Pts',(-7.66946391372299,-22.5728683523828,
12.));
#182328=CARTESIAN_POINT('Ctrl Pts',(-7.66938236806241,-22.5934737004955,
12.));
#182329=CARTESIAN_POINT('Ctrl Pts',(-7.66924547229435,-22.6141842556248,
12.));
#182330=CARTESIAN_POINT('Ctrl Pts',(-7.66905281533745,-22.6349991971547,
12.));
#182331=CARTESIAN_POINT('Ctrl Pts',(-7.66880399241354,-22.6559177133133,
12.));
#182332=CARTESIAN_POINT('Ctrl Pts',(-7.66849860491763,-22.6769390009889,
12.));
#182333=CARTESIAN_POINT('Ctrl Pts',(-7.66813626029277,-22.6980622655446,
12.));
#182334=CARTESIAN_POINT('Ctrl Pts',(-7.6677165719101,-22.7192867206242,
12.));
#182335=CARTESIAN_POINT('Ctrl Pts',(-7.66723915895413,-22.7406115879508,
12.));
#182336=CARTESIAN_POINT('Ctrl Pts',(-7.66670364630273,-22.7620360971839,
12.));
#182337=CARTESIAN_POINT('Ctrl Pts',(-7.66610966441259,-22.7835594857697,
12.));
#182338=CARTESIAN_POINT('Ctrl Pts',(-7.66545684920988,-22.8051809987833,
12.));
#182339=CARTESIAN_POINT('Ctrl Pts',(-7.66474484198553,-22.8268998887678,
12.));
#182340=CARTESIAN_POINT('Ctrl Pts',(-7.66397328929805,-22.8487154155569,
12.));
#182341=CARTESIAN_POINT('Ctrl Pts',(-7.66314184287334,-22.870626846128,
12.));
#182342=CARTESIAN_POINT('Ctrl Pts',(-7.66225015950148,-22.8926334544879,
12.));
#182343=CARTESIAN_POINT('Ctrl Pts',(-7.661297900941,-22.9147345215418,12.));
#182344=CARTESIAN_POINT('Ctrl Pts',(-7.66028473382777,-22.9369293349592,
12.));
#182345=CARTESIAN_POINT('Ctrl Pts',(-7.65921032958912,-22.9592171890332,
12.));
#182346=CARTESIAN_POINT('Ctrl Pts',(-7.65807436436453,-22.9815973845301,
12.));
#182347=CARTESIAN_POINT('Ctrl Pts',(-7.6568765189133,-23.004069228582,12.));
#182348=CARTESIAN_POINT('Ctrl Pts',(-7.65561647852555,-23.0266320345792,
12.));
#182349=CARTESIAN_POINT('Ctrl Pts',(-7.65429393293955,-23.049285122053,
12.));
#182350=CARTESIAN_POINT('Ctrl Pts',(-7.65290857626357,-23.072027816555,
12.));
#182351=CARTESIAN_POINT('Ctrl Pts',(-7.65146010690465,-23.0948594495246,
12.));
#182352=CARTESIAN_POINT('Ctrl Pts',(-7.64994822749845,-23.1177793581674,
12.));
#182353=CARTESIAN_POINT('Ctrl Pts',(-7.64837264482929,-23.1407868853815,
12.));
#182354=CARTESIAN_POINT('Ctrl Pts',(-7.64673306975797,-23.1638813796691,
12.));
#182355=CARTESIAN_POINT('Ctrl Pts',(-7.64502921715483,-23.1870621950452,
12.));
#182356=CARTESIAN_POINT('Ctrl Pts',(-7.64326080583684,-23.2103286909399,
12.));
#182357=CARTESIAN_POINT('Ctrl Pts',(-7.64142755851508,-23.2336802320912,
12.));
#182358=CARTESIAN_POINT('Ctrl Pts',(-7.63952920172837,-23.2571161884487,
12.));
#182359=CARTESIAN_POINT('Ctrl Pts',(-7.63756546576375,-23.2806359350853,
12.));
#182360=CARTESIAN_POINT('Ctrl Pts',(-7.63553608458784,-23.3042388521021,
12.));
#182361=CARTESIAN_POINT('Ctrl Pts',(-7.63344079578163,-23.3279243245241,
12.));
#182362=CARTESIAN_POINT('Ctrl Pts',(-7.63127934048139,-23.3516917421973,
12.));
#182363=CARTESIAN_POINT('Ctrl Pts',(-7.62905146332598,-23.3755404996638,
12.));
#182364=CARTESIAN_POINT('Ctrl Pts',(-7.62675691240335,-23.3994699961122,
12.));
#182365=CARTESIAN_POINT('Ctrl Pts',(-7.62439543920055,-23.4234796353544,
12.));
#182366=CARTESIAN_POINT('Ctrl Pts',(-7.62196679855957,-23.4475688257854,
12.));
#182367=CARTESIAN_POINT('Ctrl Pts',(-7.61947074863978,-23.4717369803438,
12.));
#182368=CARTESIAN_POINT('Ctrl Pts',(-7.61690705088319,-23.4959835164608,
12.));
#182369=CARTESIAN_POINT('Ctrl Pts',(-7.61427546999299,-23.5203078560128,
12.));
#182370=CARTESIAN_POINT('Ctrl Pts',(-7.61157577385372,-23.5447094252028,
12.));
#182371=CARTESIAN_POINT('Ctrl Pts',(-7.608807733446,-23.5691876544243,12.));
#182372=CARTESIAN_POINT('Ctrl Pts',(-7.60597112277094,-23.5937419781244,
12.));
#182373=CARTESIAN_POINT('Ctrl Pts',(-7.60306571877806,-23.6183718346576,
12.));
#182374=CARTESIAN_POINT('Ctrl Pts',(-7.6000913013013,-23.6430766661419,
12.));
#182375=CARTESIAN_POINT('Ctrl Pts',(-7.59704765299572,-23.6678559182876,
12.));
#182376=CARTESIAN_POINT('Ctrl Pts',(-7.59393455934042,-23.6927090405067,
12.));
#182377=CARTESIAN_POINT('Ctrl Pts',(-7.59075180865327,-23.7176354860457,
12.));
#182378=CARTESIAN_POINT('Ctrl Pts',(-7.58749919210832,-23.7426347121006,
12.));
#182379=CARTESIAN_POINT('Ctrl Pts',(-7.58417650376272,-23.7677061799376,
12.));
#182380=CARTESIAN_POINT('Ctrl Pts',(-7.58078354058212,-23.7928493549908,
12.));
#182381=CARTESIAN_POINT('Ctrl Pts',(-7.57732010249066,-23.8180637069977,
12.));
#182382=CARTESIAN_POINT('Ctrl Pts',(-7.57378599219817,-23.8433487096134,
12.));
#182383=CARTESIAN_POINT('Ctrl Pts',(-7.57018101500711,-23.8687038399597,
12.));
#182384=CARTESIAN_POINT('Ctrl Pts',(-7.56650497863792,-23.8941285782003,
12.));
#182385=CARTESIAN_POINT('Ctrl Pts',(-7.56275769304773,-23.9196224070759,
12.));
#182386=CARTESIAN_POINT('Ctrl Pts',(-7.55893897027683,-23.9451848115,12.));
#182387=CARTESIAN_POINT('Ctrl Pts',(-7.55504862424812,-23.9708152779884,
12.));
#182388=CARTESIAN_POINT('Ctrl Pts',(-7.55108647097441,-23.9965132953185,
12.));
#182389=CARTESIAN_POINT('Ctrl Pts',(-7.5470523288591,-24.022278355453,12.));
#182390=CARTESIAN_POINT('Ctrl Pts',(-7.54294601896145,-24.0481099543353,
12.));
#182391=CARTESIAN_POINT('Ctrl Pts',(-7.53876736531014,-24.0740075927985,
12.));
#182392=CARTESIAN_POINT('Ctrl Pts',(-7.53451619514649,-24.0999707772642,
12.));
#182393=CARTESIAN_POINT('Ctrl Pts',(-7.53019233935502,-24.1259990209207,
12.));
#182394=CARTESIAN_POINT('Ctrl Pts',(-7.52579563201424,-24.1520918425364,
12.));
#182395=CARTESIAN_POINT('Ctrl Pts',(-7.52132590953802,-24.1782487641594,
12.));
#182396=CARTESIAN_POINT('Ctrl Pts',(-7.51678300997949,-24.2044693092349,
12.));
#182397=CARTESIAN_POINT('Ctrl Pts',(-7.51216677222181,-24.2307530003887,
12.));
#182398=CARTESIAN_POINT('Ctrl Pts',(-7.50747703535134,-24.2570993577034,
12.));
#182399=CARTESIAN_POINT('Ctrl Pts',(-7.50271363765152,-24.2835078958973,
12.));
#182400=CARTESIAN_POINT('Ctrl Pts',(-7.49787641695439,-24.3099781253355,
12.));
#182401=CARTESIAN_POINT('Ctrl Pts',(-7.49296521252421,-24.3365095573685,
12.));
#182402=CARTESIAN_POINT('Ctrl Pts',(-7.48797986651909,-24.3631017084524,
12.));
#182403=CARTESIAN_POINT('Ctrl Pts',(-7.48292022569301,-24.3897541049254,
12.));
#182404=CARTESIAN_POINT('Ctrl Pts',(-7.47778614286565,-24.4164662871163,
12.));
#182405=CARTESIAN_POINT('Ctrl Pts',(-7.47257747883246,-24.443237814649,
12.));
#182406=CARTESIAN_POINT('Ctrl Pts',(-7.46729410308787,-24.4700682684524,
12.));
#182407=CARTESIAN_POINT('Ctrl Pts',(-7.46193588961464,-24.4969572391483,
12.));
#182408=CARTESIAN_POINT('Ctrl Pts',(-7.45650271335862,-24.5239043173072,
12.));
#182409=CARTESIAN_POINT('Ctrl Pts',(-7.4509944465116,-24.5509090831559,
12.));
#182410=CARTESIAN_POINT('Ctrl Pts',(-7.44541095473135,-24.577971096086,
12.));
#182411=CARTESIAN_POINT('Ctrl Pts',(-7.43975209375504,-24.6050898852368,
12.));
#182412=CARTESIAN_POINT('Ctrl Pts',(-7.43401770489524,-24.6322649369517,
12.));
#182413=CARTESIAN_POINT('Ctrl Pts',(-7.42820762159126,-24.6594957128756,
12.));
#182414=CARTESIAN_POINT('Ctrl Pts',(-7.42232167766266,-24.6867816727192,
12.));
#182415=CARTESIAN_POINT('Ctrl Pts',(-7.41635971481674,-24.7141222950051,
12.));
#182416=CARTESIAN_POINT('Ctrl Pts',(-7.41032159082382,-24.7415170994784,
12.));
#182417=CARTESIAN_POINT('Ctrl Pts',(-7.40420718661603,-24.7689656668983,
12.));
#182418=CARTESIAN_POINT('Ctrl Pts',(-7.39801641583013,-24.7964676646431,
12.));
#182419=CARTESIAN_POINT('Ctrl Pts',(-7.39174922585809,-24.8240228520893,
12.));
#182420=CARTESIAN_POINT('Ctrl Pts',(-7.38540558903621,-24.8516310625176,
12.));
#182421=CARTESIAN_POINT('Ctrl Pts',(-7.3789854964027,-24.8792921911115,
12.));
#182422=CARTESIAN_POINT('Ctrl Pts',(-7.37378825961676,-24.901463382605,
12.));
#182423=CARTESIAN_POINT('Ctrl Pts',(-7.36985593120091,-24.9181155530543,
12.));
#182424=CARTESIAN_POINT('Ctrl Pts',(-7.36721909028843,-24.9292275670674,
12.));
#182425=CARTESIAN_POINT('Ctrl Pts',(-7.36589684767345,-24.9347862158358,
12.));
#182426=CARTESIAN_POINT('',(-6.088339316177,-25.2771067246846,12.));
#182427=CARTESIAN_POINT('Origin',(0.,0.,12.));
#182428=CARTESIAN_POINT('',(-4.11585220600463,-22.1738711152697,12.));
#182429=CARTESIAN_POINT('Ctrl Pts',(-6.088339316177,-25.2771067246846,12.));
#182430=CARTESIAN_POINT('Ctrl Pts',(-6.08441489609794,-25.2729539149517,
12.));
#182431=CARTESIAN_POINT('Ctrl Pts',(-6.07657531787491,-25.2646490489922,
12.));
#182432=CARTESIAN_POINT('Ctrl Pts',(-6.06484373634547,-25.2521940105705,
12.));
#182433=CARTESIAN_POINT('Ctrl Pts',(-6.04925720151219,-25.2355918139032,
12.));
#182434=CARTESIAN_POINT('Ctrl Pts',(-6.02986667389998,-25.21484662016,12.));
#182435=CARTESIAN_POINT('Ctrl Pts',(-6.01056881804614,-25.1941090269819,
12.));
#182436=CARTESIAN_POINT('Ctrl Pts',(-5.99136367859755,-25.1733791296259,
12.));
#182437=CARTESIAN_POINT('Ctrl Pts',(-5.97225131495618,-25.1526570863092,
12.));
#182438=CARTESIAN_POINT('Ctrl Pts',(-5.95323180187379,-25.1319431317237,
12.));
#182439=CARTESIAN_POINT('Ctrl Pts',(-5.93430523086836,-25.1112375971106,
12.));
#182440=CARTESIAN_POINT('Ctrl Pts',(-5.91547170844448,-25.0905409050773,
12.));
#182441=CARTESIAN_POINT('Ctrl Pts',(-5.89673135155515,-25.0698535426514,
12.));
#182442=CARTESIAN_POINT('Ctrl Pts',(-5.87808428385367,-25.049176040591,
12.));
#182443=CARTESIAN_POINT('Ctrl Pts',(-5.85953063156827,-25.0285089498899,
12.));
#182444=CARTESIAN_POINT('Ctrl Pts',(-5.84107051963072,-25.0078528200564,
12.));
#182445=CARTESIAN_POINT('Ctrl Pts',(-5.822704067442,-24.9872081752734,12.));
#182446=CARTESIAN_POINT('Ctrl Pts',(-5.80443138549727,-24.9665754954496,
12.));
#182447=CARTESIAN_POINT('Ctrl Pts',(-5.78625257775682,-24.945955229334,
12.));
#182448=CARTESIAN_POINT('Ctrl Pts',(-5.76816774342221,-24.9253478043656,
12.));
#182449=CARTESIAN_POINT('Ctrl Pts',(-5.75017697890805,-24.904753637648,
12.));
#182450=CARTESIAN_POINT('Ctrl Pts',(-5.73228037976928,-24.884173146722,
12.));
#182451=CARTESIAN_POINT('Ctrl Pts',(-5.71447804252028,-24.8636067597669,
12.));
#182452=CARTESIAN_POINT('Ctrl Pts',(-5.69677006679445,-24.8430549277621,
12.));
#182453=CARTESIAN_POINT('Ctrl Pts',(-5.67915655496543,-24.8225181223845,
12.));
#182454=CARTESIAN_POINT('Ctrl Pts',(-5.66163761114922,-24.8019968304605,
12.));
#182455=CARTESIAN_POINT('Ctrl Pts',(-5.64421334042262,-24.781491549672,
12.));
#182456=CARTESIAN_POINT('Ctrl Pts',(-5.62688384790924,-24.7610027835697,
12.));
#182457=CARTESIAN_POINT('Ctrl Pts',(-5.60964923798492,-24.7405310372739,
12.));
#182458=CARTESIAN_POINT('Ctrl Pts',(-5.59250961323988,-24.7200768119088,
12.));
#182459=CARTESIAN_POINT('Ctrl Pts',(-5.57546507427756,-24.6996406035517,
12.));
#182460=CARTESIAN_POINT('Ctrl Pts',(-5.55851572025377,-24.6792229061794,
12.));
#182461=CARTESIAN_POINT('Ctrl Pts',(-5.54166164919584,-24.6588242134738,
12.));
#182462=CARTESIAN_POINT('Ctrl Pts',(-5.52490295840993,-24.6384450211467,
12.));
#182463=CARTESIAN_POINT('Ctrl Pts',(-5.50823974481963,-24.6180858289179,
12.));
#182464=CARTESIAN_POINT('Ctrl Pts',(-5.49167210537248,-24.5977471429364,
12.));
#182465=CARTESIAN_POINT('Ctrl Pts',(-5.4752001372442,-24.5774294770329,
12.));
#182466=CARTESIAN_POINT('Ctrl Pts',(-5.45882393762262,-24.5571333514842,
12.));
#182467=CARTESIAN_POINT('Ctrl Pts',(-5.44254360356881,-24.5368592922863,
12.));
#182468=CARTESIAN_POINT('Ctrl Pts',(-5.4263592318342,-24.5166078302108,
12.));
#182469=CARTESIAN_POINT('Ctrl Pts',(-5.41027091869242,-24.496379499983,
12.));
#182470=CARTESIAN_POINT('Ctrl Pts',(-5.39427875973825,-24.4761748393321,
12.));
#182471=CARTESIAN_POINT('Ctrl Pts',(-5.37838284973696,-24.4559943883157,
12.));
#182472=CARTESIAN_POINT('Ctrl Pts',(-5.36258328273628,-24.435838689915,
12.));
#182473=CARTESIAN_POINT('Ctrl Pts',(-5.34688015213538,-24.4157082904614,
12.));
#182474=CARTESIAN_POINT('Ctrl Pts',(-5.33127355076035,-24.3956037401293,
12.));
#182475=CARTESIAN_POINT('Ctrl Pts',(-5.31576357092527,-24.3755255933917,
12.));
#182476=CARTESIAN_POINT('Ctrl Pts',(-5.30035030449064,-24.3554744095075,
12.));
#182477=CARTESIAN_POINT('Ctrl Pts',(-5.28503384290649,-24.3354507529414,
12.));
#182478=CARTESIAN_POINT('Ctrl Pts',(-5.269814277188,-24.3154551932221,12.));
#182479=CARTESIAN_POINT('Ctrl Pts',(-5.25469169788857,-24.2954883048447,
12.));
#182480=CARTESIAN_POINT('Ctrl Pts',(-5.2396661950629,-24.2755506671525,
12.));
#182481=CARTESIAN_POINT('Ctrl Pts',(-5.22473785822443,-24.2556428642294,
12.));
#182482=CARTESIAN_POINT('Ctrl Pts',(-5.20990677629177,-24.2357654847766,
12.));
#182483=CARTESIAN_POINT('Ctrl Pts',(-5.19517303753648,-24.2159191220171,
12.));
#182484=CARTESIAN_POINT('Ctrl Pts',(-5.180536729614,-24.1961043738756,12.));
#182485=CARTESIAN_POINT('Ctrl Pts',(-5.16599793957987,-24.1763218431344,
12.));
#182486=CARTESIAN_POINT('Ctrl Pts',(-5.1515567539008,-24.1565721375971,
12.));
#182487=CARTESIAN_POINT('Ctrl Pts',(-5.13721325845746,-24.1368558702443,
12.));
#182488=CARTESIAN_POINT('Ctrl Pts',(-5.12296753853858,-24.117173659394,
12.));
#182489=CARTESIAN_POINT('Ctrl Pts',(-5.10881967883126,-24.0975261288444,
12.));
#182490=CARTESIAN_POINT('Ctrl Pts',(-5.09476976342618,-24.0779139079264,
12.));
#182491=CARTESIAN_POINT('Ctrl Pts',(-5.08081787581271,-24.0583376315636,
12.));
#182492=CARTESIAN_POINT('Ctrl Pts',(-5.0669640988664,-24.0387979403268,
12.));
#182493=CARTESIAN_POINT('Ctrl Pts',(-5.05320851483069,-24.0192954804896,
12.));
#182494=CARTESIAN_POINT('Ctrl Pts',(-5.03955120528528,-23.9998309040747,
12.));
#182495=CARTESIAN_POINT('Ctrl Pts',(-5.02599225112462,-23.9804048689228,
12.));
#182496=CARTESIAN_POINT('Ctrl Pts',(-5.01253173257459,-23.9610180388271,
12.));
#182497=CARTESIAN_POINT('Ctrl Pts',(-4.9991697291931,-23.9416710836529,
12.));
#182498=CARTESIAN_POINT('Ctrl Pts',(-4.98590631986534,-23.9223646794591,
12.));
#182499=CARTESIAN_POINT('Ctrl Pts',(-4.9727415827923,-23.9030995086164,
12.));
#182500=CARTESIAN_POINT('Ctrl Pts',(-4.95967559546566,-23.883876259922,
12.));
#182501=CARTESIAN_POINT('Ctrl Pts',(-4.94670843465869,-23.8646956287172,
12.));
#182502=CARTESIAN_POINT('Ctrl Pts',(-4.93384017643442,-23.8455583170062,
12.));
#182503=CARTESIAN_POINT('Ctrl Pts',(-4.92107089613977,-23.8264650335721,
12.));
#182504=CARTESIAN_POINT('Ctrl Pts',(-4.90840066839348,-23.8074164940897,
12.));
#182505=CARTESIAN_POINT('Ctrl Pts',(-4.89582956706772,-23.7884134212381,
12.));
#182506=CARTESIAN_POINT('Ctrl Pts',(-4.88335766525566,-23.7694565448044,
12.));
#182507=CARTESIAN_POINT('Ctrl Pts',(-4.87098503527144,-23.7505466018239,
12.));
#182508=CARTESIAN_POINT('Ctrl Pts',(-4.85871174865492,-23.7316843367308,
12.));
#182509=CARTESIAN_POINT('Ctrl Pts',(-4.84653787616424,-23.7128705015014,
12.));
#182510=CARTESIAN_POINT('Ctrl Pts',(-4.83446348776268,-23.6941058557971,
12.));
#182511=CARTESIAN_POINT('Ctrl Pts',(-4.82248865259571,-23.6753911671023,
12.));
#182512=CARTESIAN_POINT('Ctrl Pts',(-4.81061343896443,-23.6567272108631,
12.));
#182513=CARTESIAN_POINT('Ctrl Pts',(-4.79883791433231,-23.6381147706581,
12.));
#182514=CARTESIAN_POINT('Ctrl Pts',(-4.78716214532105,-23.6195546383625,
12.));
#182515=CARTESIAN_POINT('Ctrl Pts',(-4.77558619769876,-23.6010476143099,
12.));
#182516=CARTESIAN_POINT('Ctrl Pts',(-4.76411013636252,-23.5825945074535,
12.));
#182517=CARTESIAN_POINT('Ctrl Pts',(-4.75273402530616,-23.564196135517,
12.));
#182518=CARTESIAN_POINT('Ctrl Pts',(-4.74145792760699,-23.5458533251715,
12.));
#182519=CARTESIAN_POINT('Ctrl Pts',(-4.73028190543032,-23.5275669122378,
12.));
#182520=CARTESIAN_POINT('Ctrl Pts',(-4.71920602001905,-23.5093377418784,
12.));
#182521=CARTESIAN_POINT('Ctrl Pts',(-4.70823033167821,-23.491166668789,
12.));
#182522=CARTESIAN_POINT('Ctrl Pts',(-4.69735489975024,-23.4730545573849,
12.));
#182523=CARTESIAN_POINT('Ctrl Pts',(-4.68657978258298,-23.4550022819852,
12.));
#182524=CARTESIAN_POINT('Ctrl Pts',(-4.67590503753051,-23.4370107270444,
12.));
#182525=CARTESIAN_POINT('Ctrl Pts',(-4.66533072094664,-23.4190807873798,
12.));
#182526=CARTESIAN_POINT('Ctrl Pts',(-4.65485688816923,-23.4012133683957,
12.));
#182527=CARTESIAN_POINT('Ctrl Pts',(-4.64448359349936,-23.383409386307,
12.));
#182528=CARTESIAN_POINT('Ctrl Pts',(-4.63421089016555,-23.3656697683496,
12.));
#182529=CARTESIAN_POINT('Ctrl Pts',(-4.62403883030825,-23.3479954530281,
12.));
#182530=CARTESIAN_POINT('Ctrl Pts',(-4.61396746497849,-23.3303873903947,
12.));
#182531=CARTESIAN_POINT('Ctrl Pts',(-4.60399684412176,-23.3128465423119,
12.));
#182532=CARTESIAN_POINT('Ctrl Pts',(-4.5941270165575,-23.295373882719,12.));
#182533=CARTESIAN_POINT('Ctrl Pts',(-4.58435802994675,-23.2779703978868,
12.));
#182534=CARTESIAN_POINT('Ctrl Pts',(-4.57468993076071,-23.2606370866854,
12.));
#182535=CARTESIAN_POINT('Ctrl Pts',(-4.56512276427812,-23.2433749609117,
12.));
#182536=CARTESIAN_POINT('Ctrl Pts',(-4.55565657456957,-23.2261850456055,
12.));
#182537=CARTESIAN_POINT('Ctrl Pts',(-4.54629140447543,-23.2090683793627,
12.));
#182538=CARTESIAN_POINT('Ctrl Pts',(-4.53702729557586,-23.1920260146474,
12.));
#182539=CARTESIAN_POINT('Ctrl Pts',(-4.52786428815049,-23.1750590180923,
12.));
#182540=CARTESIAN_POINT('Ctrl Pts',(-4.51880242116786,-23.1581684708778,
12.));
#182541=CARTESIAN_POINT('Ctrl Pts',(-4.50984173227088,-23.1413554691136,
12.));
#182542=CARTESIAN_POINT('Ctrl Pts',(-4.50098225775179,-23.1246211242117,
12.));
#182543=CARTESIAN_POINT('Ctrl Pts',(-4.49222403252202,-23.1079665632629,
12.));
#182544=CARTESIAN_POINT('Ctrl Pts',(-4.48356709006757,-23.0913929293909,
12.));
#182545=CARTESIAN_POINT('Ctrl Pts',(-4.47501146242822,-23.0749013821867,
12.));
#182546=CARTESIAN_POINT('Ctrl Pts',(-4.46655718018206,-23.0584930981723,
12.));
#182547=CARTESIAN_POINT('Ctrl Pts',(-4.45820427241677,-23.0421692712466,
12.));
#182548=CARTESIAN_POINT('Ctrl Pts',(-4.44995276669699,-23.0259311131395,
12.));
#182549=CARTESIAN_POINT('Ctrl Pts',(-4.44180268901667,-23.0097798538399,
12.));
#182550=CARTESIAN_POINT('Ctrl Pts',(-4.43375406376906,-22.9937167421009,
12.));
#182551=CARTESIAN_POINT('Ctrl Pts',(-4.42580691372772,-22.9777430460021,
12.));
#182552=CARTESIAN_POINT('Ctrl Pts',(-4.41796126001311,-22.9618600534866,
12.));
#182553=CARTESIAN_POINT('Ctrl Pts',(-4.41021712205549,-22.9460690729093,
12.));
#182554=CARTESIAN_POINT('Ctrl Pts',(-4.40257451754308,-22.9303714335549,
12.));
#182555=CARTESIAN_POINT('Ctrl Pts',(-4.39503346238455,-22.9147684862425,
12.));
#182556=CARTESIAN_POINT('Ctrl Pts',(-4.38759397068393,-22.8992616040108,
12.));
#182557=CARTESIAN_POINT('Ctrl Pts',(-4.38025605470091,-22.8838521827702,
12.));
#182558=CARTESIAN_POINT('Ctrl Pts',(-4.37301972480753,-22.8685416419725,
12.));
#182559=CARTESIAN_POINT('Ctrl Pts',(-4.36588498943011,-22.8533314252419,
12.));
#182560=CARTESIAN_POINT('Ctrl Pts',(-4.3588518550056,-22.838223001118,12.));
#182561=CARTESIAN_POINT('Ctrl Pts',(-4.35192032594802,-22.8232178638873,
12.));
#182562=CARTESIAN_POINT('Ctrl Pts',(-4.34509040460066,-22.808317534379,
12.));
#182563=CARTESIAN_POINT('Ctrl Pts',(-4.33836209118444,-22.7935235607807,
12.));
#182564=CARTESIAN_POINT('Ctrl Pts',(-4.33173538373183,-22.7788375194081,
12.));
#182565=CARTESIAN_POINT('Ctrl Pts',(-4.32521027803748,-22.764261015648,
12.));
#182566=CARTESIAN_POINT('Ctrl Pts',(-4.31878676761231,-22.7497956849852,
12.));
#182567=CARTESIAN_POINT('Ctrl Pts',(-4.31246484362551,-22.7354431939926,
12.));
#182568=CARTESIAN_POINT('Ctrl Pts',(-4.30624449484075,-22.7212052413384,
12.));
#182569=CARTESIAN_POINT('Ctrl Pts',(-4.30012570754067,-22.707083558756,
12.));
#182570=CARTESIAN_POINT('Ctrl Pts',(-4.29410846547062,-22.6930799122545,
12.));
#182571=CARTESIAN_POINT('Ctrl Pts',(-4.28819274977767,-22.6791961033536,
12.));
#182572=CARTESIAN_POINT('Ctrl Pts',(-4.2823785389406,-22.665433970311,12.));
#182573=CARTESIAN_POINT('Ctrl Pts',(-4.27666580869118,-22.6517953893303,
12.));
#182574=CARTESIAN_POINT('Ctrl Pts',(-4.27105453193,-22.6382822758171,12.));
#182575=CARTESIAN_POINT('Ctrl Pts',(-4.26554467865572,-22.6248965859975,
12.));
#182576=CARTESIAN_POINT('Ctrl Pts',(-4.26013621588304,-22.611640318482,
12.));
#182577=CARTESIAN_POINT('Ctrl Pts',(-4.25482910755486,-22.5985155158637,
12.));
#182578=CARTESIAN_POINT('Ctrl Pts',(-4.24962331444186,-22.5855242662479,
12.));
#182579=CARTESIAN_POINT('Ctrl Pts',(-4.2445187940486,-22.5726687049922,
12.));
#182580=CARTESIAN_POINT('Ctrl Pts',(-4.23951550052527,-22.559951016643,
12.));
#182581=CARTESIAN_POINT('Ctrl Pts',(-4.23461338456714,-22.5473734368086,
12.));
#182582=CARTESIAN_POINT('Ctrl Pts',(-4.22981239330732,-22.5349382540587,
12.));
#182583=CARTESIAN_POINT('Ctrl Pts',(-4.22511247020041,-22.5226478117885,
12.));
#182584=CARTESIAN_POINT('Ctrl Pts',(-4.22051355490198,-22.5105045108882,
12.));
#182585=CARTESIAN_POINT('Ctrl Pts',(-4.21601558313909,-22.4985108124229,
12.));
#182586=CARTESIAN_POINT('Ctrl Pts',(-4.21161848657429,-22.4866692403147,
12.));
#182587=CARTESIAN_POINT('Ctrl Pts',(-4.20732219265649,-22.4749823839915,
12.));
#182588=CARTESIAN_POINT('Ctrl Pts',(-4.20312662448172,-22.4634529011433,
12.));
#182589=CARTESIAN_POINT('Ctrl Pts',(-4.19903170066356,-22.4520835205419,
12.));
#182590=CARTESIAN_POINT('Ctrl Pts',(-4.19503733518862,-22.4408770448917,
12.));
#182591=CARTESIAN_POINT('Ctrl Pts',(-4.19114343726943,-22.4298363535421,
12.));
#182592=CARTESIAN_POINT('Ctrl Pts',(-4.18734991117722,-22.4189644056115,
12.));
#182593=CARTESIAN_POINT('Ctrl Pts',(-4.18365665600851,-22.4082642454453,
12.));
#182594=CARTESIAN_POINT('Ctrl Pts',(-4.18006356544883,-22.3977390078075,
12.));
#182595=CARTESIAN_POINT('Ctrl Pts',(-4.17657052752826,-22.3873919231334,
12.));
#182596=CARTESIAN_POINT('Ctrl Pts',(-4.17317742436146,-22.3772263228617,
12.));
#182597=CARTESIAN_POINT('Ctrl Pts',(-4.16988413199458,-22.36724564276,12.));
#182598=CARTESIAN_POINT('Ctrl Pts',(-4.16669052026601,-22.3574534257396,
12.));
#182599=CARTESIAN_POINT('Ctrl Pts',(-4.16359645263189,-22.3478533253889,
12.));
#182600=CARTESIAN_POINT('Ctrl Pts',(-4.16060178604165,-22.3384491078602,
12.));
#182601=CARTESIAN_POINT('Ctrl Pts',(-4.15770637047891,-22.3292446628959,
12.));
#182602=CARTESIAN_POINT('Ctrl Pts',(-4.15491004835282,-22.320244018698,
12.));
#182603=CARTESIAN_POINT('Ctrl Pts',(-4.15221265396991,-22.3114513545185,
12.));
#182604=CARTESIAN_POINT('Ctrl Pts',(-4.14961401285523,-22.3028710166933,
12.));
#182605=CARTESIAN_POINT('Ctrl Pts',(-4.14711394168557,-22.2945075198467,
12.));
#182606=CARTESIAN_POINT('Ctrl Pts',(-4.14471224859296,-22.2863655389166,
12.));
#182607=CARTESIAN_POINT('Ctrl Pts',(-4.14240873321985,-22.2784499072027,
12.));
#182608=CARTESIAN_POINT('Ctrl Pts',(-4.14020318715992,-22.2707656042457,
12.));
#182609=CARTESIAN_POINT('Ctrl Pts',(-4.13809539255423,-22.2633177913972,
12.));
#182610=CARTESIAN_POINT('Ctrl Pts',(-4.13608511977226,-22.2561118708421,
12.));
#182611=CARTESIAN_POINT('Ctrl Pts',(-4.13417212558811,-22.249153531779,
12.));
#182612=CARTESIAN_POINT('Ctrl Pts',(-4.13235615060161,-22.2424488153523,
12.));
#182613=CARTESIAN_POINT('Ctrl Pts',(-4.13063692157499,-22.2360040565533,
12.));
#182614=CARTESIAN_POINT('Ctrl Pts',(-4.1290141546338,-22.2298258043947,
12.));
#182615=CARTESIAN_POINT('Ctrl Pts',(-4.12748755830105,-22.2239207458781,
12.));
#182616=CARTESIAN_POINT('Ctrl Pts',(-4.12605683613308,-22.2182956401341,
12.));
#182617=CARTESIAN_POINT('Ctrl Pts',(-4.12472167516608,-22.2129576146671,
12.));
#182618=CARTESIAN_POINT('Ctrl Pts',(-4.12348173702024,-22.2079143941719,
12.));
#182619=CARTESIAN_POINT('Ctrl Pts',(-4.12233664408228,-22.2031746532106,
12.));
#182620=CARTESIAN_POINT('Ctrl Pts',(-4.12128598183523,-22.1987479618246,
12.));
#182621=CARTESIAN_POINT('Ctrl Pts',(-4.12032932637737,-22.1946440958098,
12.));
#182622=CARTESIAN_POINT('Ctrl Pts',(-4.11946626228637,-22.1908725908525,
12.));
#182623=CARTESIAN_POINT('Ctrl Pts',(-4.11869641271774,-22.1874419861496,
12.));
#182624=CARTESIAN_POINT('Ctrl Pts',(-4.11801938107481,-22.1843613164855,
12.));
#182625=CARTESIAN_POINT('Ctrl Pts',(-4.11743469691757,-22.1816414985788,
12.));
#182626=CARTESIAN_POINT('Ctrl Pts',(-4.11694173195005,-22.179297473024,
12.));
#182627=CARTESIAN_POINT('Ctrl Pts',(-4.11653973150519,-22.177347426894,
12.));
#182628=CARTESIAN_POINT('Ctrl Pts',(-4.11622797217069,-22.1758088296598,
12.));
#182629=CARTESIAN_POINT('Ctrl Pts',(-4.11600589882846,-22.1746949858775,
12.));
#182630=CARTESIAN_POINT('Ctrl Pts',(-4.11589976826167,-22.1741488021234,
12.));
#182631=CARTESIAN_POINT('Ctrl Pts',(-4.11586035878288,-22.1739341411687,
12.));
#182632=CARTESIAN_POINT('Ctrl Pts',(-4.11585194677443,-22.173877682324,
12.));
#182633=CARTESIAN_POINT('Ctrl Pts',(-4.11585220600463,-22.1738711152697,
12.));
#182634=CARTESIAN_POINT('',(-4.0139614976743,-21.624941921198,12.));
#182635=CARTESIAN_POINT('',(-1.96187429785751,-10.5694630535049,12.));
#182636=CARTESIAN_POINT('',(-3.4423049612042,-21.2226420728916,12.));
#182637=CARTESIAN_POINT('Origin',(-3.52235856495314,-21.7161918885402,12.));
#182638=CARTESIAN_POINT('',(-2.16781269186829,-21.3904321633055,12.));
#182639=CARTESIAN_POINT('Origin',(-1.31973449697531E-13,-7.6920903736728E-13,
12.));
#182640=CARTESIAN_POINT('',(-1.71975774210843,-21.9269795755927,12.));
#182641=CARTESIAN_POINT('Origin',(-2.21822694051639,-21.88788407408,12.));
#182642=CARTESIAN_POINT('',(-1.76341220531181,-22.4835757167854,12.));
#182643=CARTESIAN_POINT('',(-0.881706102655891,-11.2417878583927,12.));
#182644=CARTESIAN_POINT('',(-0.661312440730913,-25.991588367311,12.));
#182645=CARTESIAN_POINT('Ctrl Pts',(-1.76341220531181,-22.4835757167854,
12.));
#182646=CARTESIAN_POINT('Ctrl Pts',(-1.76341415538792,-22.4835819929788,
12.));
#182647=CARTESIAN_POINT('Ctrl Pts',(-1.76342064263638,-22.4836387052228,
12.));
#182648=CARTESIAN_POINT('Ctrl Pts',(-1.7634381343466,-22.4838562517064,
12.));
#182649=CARTESIAN_POINT('Ctrl Pts',(-1.76347698284863,-22.4844112933125,
12.));
#182650=CARTESIAN_POINT('Ctrl Pts',(-1.7635507604555,-22.4855446605991,
12.));
#182651=CARTESIAN_POINT('Ctrl Pts',(-1.76364784232926,-22.4871115206572,
12.));
#182652=CARTESIAN_POINT('Ctrl Pts',(-1.76376424879469,-22.4890991659479,
12.));
#182653=CARTESIAN_POINT('Ctrl Pts',(-1.76389475965715,-22.4914909094908,
12.));
#182654=CARTESIAN_POINT('Ctrl Pts',(-1.76403393880317,-22.4942693792449,
12.));
#182655=CARTESIAN_POINT('Ctrl Pts',(-1.76417731243484,-22.4974203063191,
12.));
#182656=CARTESIAN_POINT('Ctrl Pts',(-1.76432160068739,-22.5009332677316,
12.));
#182657=CARTESIAN_POINT('Ctrl Pts',(-1.76446408210366,-22.5047996391978,
12.));
#182658=CARTESIAN_POINT('Ctrl Pts',(-1.76460218257314,-22.5090112700212,
12.));
#182659=CARTESIAN_POINT('Ctrl Pts',(-1.7647330328115,-22.5135590569554,
12.));
#182660=CARTESIAN_POINT('Ctrl Pts',(-1.76485369319896,-22.5184336670207,
12.));
#182661=CARTESIAN_POINT('Ctrl Pts',(-1.76496128643376,-22.5236259635515,
12.));
#182662=CARTESIAN_POINT('Ctrl Pts',(-1.7650532026276,-22.529127665298,12.));
#182663=CARTESIAN_POINT('Ctrl Pts',(-1.76512711563255,-22.5349313983571,
12.));
#182664=CARTESIAN_POINT('Ctrl Pts',(-1.76518087841494,-22.5410303590892,
12.));
#182665=CARTESIAN_POINT('Ctrl Pts',(-1.76521245524048,-22.5474180954006,
12.));
#182666=CARTESIAN_POINT('Ctrl Pts',(-1.76521983384063,-22.5540882235837,
12.));
#182667=CARTESIAN_POINT('Ctrl Pts',(-1.76520104500451,-22.5610344912501,
12.));
#182668=CARTESIAN_POINT('Ctrl Pts',(-1.76515418518832,-22.5682508499874,
12.));
#182669=CARTESIAN_POINT('Ctrl Pts',(-1.76507744026747,-22.5757315316353,
12.));
#182670=CARTESIAN_POINT('Ctrl Pts',(-1.76496910283089,-22.5834711038022,
12.));
#182671=CARTESIAN_POINT('Ctrl Pts',(-1.76482755288412,-22.5914644078106,
12.));
#182672=CARTESIAN_POINT('Ctrl Pts',(-1.76465124413558,-22.5997065145638,
12.));
#182673=CARTESIAN_POINT('Ctrl Pts',(-1.76443868648017,-22.6081926681343,
12.));
#182674=CARTESIAN_POINT('Ctrl Pts',(-1.7641884354374,-22.6169182517694,
12.));
#182675=CARTESIAN_POINT('Ctrl Pts',(-1.76389909571404,-22.6258787994848,
12.));
#182676=CARTESIAN_POINT('Ctrl Pts',(-1.76356932176274,-22.6350699979359,
12.));
#182677=CARTESIAN_POINT('Ctrl Pts',(-1.76319782013917,-22.6444876940423,
12.));
#182678=CARTESIAN_POINT('Ctrl Pts',(-1.76278334912562,-22.654127893841,
12.));
#182679=CARTESIAN_POINT('Ctrl Pts',(-1.7623247139257,-22.6639867471753,
12.));
#182680=CARTESIAN_POINT('Ctrl Pts',(-1.76182076289527,-22.67406053567,12.));
#182681=CARTESIAN_POINT('Ctrl Pts',(-1.76127038310615,-22.684345658525,
12.));
#182682=CARTESIAN_POINT('Ctrl Pts',(-1.76067249704888,-22.6948386219851,
12.));
#182683=CARTESIAN_POINT('Ctrl Pts',(-1.76002606202402,-22.7055360375485,
12.));
#182684=CARTESIAN_POINT('Ctrl Pts',(-1.75933006905926,-22.7164346186006,
12.));
#182685=CARTESIAN_POINT('Ctrl Pts',(-1.75858354204634,-22.72753117773,12.));
#182686=CARTESIAN_POINT('Ctrl Pts',(-1.75778553673245,-22.7388226235559,
12.));
#182687=CARTESIAN_POINT('Ctrl Pts',(-1.75693513908908,-22.750305955645,
12.));
#182688=CARTESIAN_POINT('Ctrl Pts',(-1.75603146371642,-22.7619782595013,
12.));
#182689=CARTESIAN_POINT('Ctrl Pts',(-1.75507365227133,-22.7738367016118,
12.));
#182690=CARTESIAN_POINT('Ctrl Pts',(-1.75406087182937,-22.7858785242361,
12.));
#182691=CARTESIAN_POINT('Ctrl Pts',(-1.75299231391467,-22.7981010424314,
12.));
#182692=CARTESIAN_POINT('Ctrl Pts',(-1.75186719365593,-22.8105016414713,
12.));
#182693=CARTESIAN_POINT('Ctrl Pts',(-1.75068474890884,-22.8230777741284,
12.));
#182694=CARTESIAN_POINT('Ctrl Pts',(-1.74944423940117,-22.8358269579853,
12.));
#182695=CARTESIAN_POINT('Ctrl Pts',(-1.74814494588494,-22.8487467728076,
12.));
#182696=CARTESIAN_POINT('Ctrl Pts',(-1.74678616930666,-22.8618348580235,
12.));
#182697=CARTESIAN_POINT('Ctrl Pts',(-1.74536722998202,-22.8750889101696,
12.));
#182698=CARTESIAN_POINT('Ctrl Pts',(-1.74388746677703,-22.888506680335,
12.));
#182699=CARTESIAN_POINT('Ctrl Pts',(-1.74234623630081,-22.9020859716141,
12.));
#182700=CARTESIAN_POINT('Ctrl Pts',(-1.74074291231059,-22.9158246373363,
12.));
#182701=CARTESIAN_POINT('Ctrl Pts',(-1.73907688511667,-22.9297205792586,
12.));
#182702=CARTESIAN_POINT('Ctrl Pts',(-1.7373475610004,-22.9437717457826,
12.));
#182703=CARTESIAN_POINT('Ctrl Pts',(-1.7355543616277,-22.9579761301063,
12.));
#182704=CARTESIAN_POINT('Ctrl Pts',(-1.73369672350816,-22.9723317685688,
12.));
#182705=CARTESIAN_POINT('Ctrl Pts',(-1.73177409750192,-22.9868367391978,
12.));
#182706=CARTESIAN_POINT('Ctrl Pts',(-1.72978594832137,-23.001489160189,
12.));
#182707=CARTESIAN_POINT('Ctrl Pts',(-1.7277317540471,-23.0162871884168,
12.));
#182708=CARTESIAN_POINT('Ctrl Pts',(-1.72561100564047,-23.0312290178883,
12.));
#182709=CARTESIAN_POINT('Ctrl Pts',(-1.72342320653748,-23.0463128785531,
12.));
#182710=CARTESIAN_POINT('Ctrl Pts',(-1.72116787225993,-23.0615370351562,
12.));
#182711=CARTESIAN_POINT('Ctrl Pts',(-1.71884453003028,-23.0768997860709,
12.));
#182712=CARTESIAN_POINT('Ctrl Pts',(-1.71645271839298,-23.0923994621213,
12.));
#182713=CARTESIAN_POINT('Ctrl Pts',(-1.71399198684705,-23.1080344254286,
12.));
#182714=CARTESIAN_POINT('Ctrl Pts',(-1.71146189552175,-23.1238030684925,
12.));
#182715=CARTESIAN_POINT('Ctrl Pts',(-1.70886201485453,-23.1397038132356,
12.));
#182716=CARTESIAN_POINT('Ctrl Pts',(-1.70619192527853,-23.1557351100614,
12.));
#182717=CARTESIAN_POINT('Ctrl Pts',(-1.70345121691277,-23.1718954368751,
12.));
#182718=CARTESIAN_POINT('Ctrl Pts',(-1.70063948927011,-23.1881832981851,
12.));
#182719=CARTESIAN_POINT('Ctrl Pts',(-1.69775635099444,-23.2045972243767,
12.));
#182720=CARTESIAN_POINT('Ctrl Pts',(-1.69480141959954,-23.2211357709374,
12.));
#182721=CARTESIAN_POINT('Ctrl Pts',(-1.69177432121712,-23.2377975177013,
12.));
#182722=CARTESIAN_POINT('Ctrl Pts',(-1.68867469034897,-23.2545810680537,
12.));
#182723=CARTESIAN_POINT('Ctrl Pts',(-1.68550216963259,-23.2714850482246,
12.));
#182724=CARTESIAN_POINT('Ctrl Pts',(-1.68225640962169,-23.2885081066951,
12.));
#182725=CARTESIAN_POINT('Ctrl Pts',(-1.67893706857118,-23.3056489135611,
12.));
#182726=CARTESIAN_POINT('Ctrl Pts',(-1.67554381222995,-23.3229061599145,
12.));
#182727=CARTESIAN_POINT('Ctrl Pts',(-1.67207631363923,-23.3402785571865,
12.));
#182728=CARTESIAN_POINT('Ctrl Pts',(-1.66853425293997,-23.3577648365744,
12.));
#182729=CARTESIAN_POINT('Ctrl Pts',(-1.66491731718878,-23.3753637485545,
12.));
#182730=CARTESIAN_POINT('Ctrl Pts',(-1.66122520018012,-23.3930740623619,
12.));
#182731=CARTESIAN_POINT('Ctrl Pts',(-1.65745760227506,-23.4108945654805,
12.));
#182732=CARTESIAN_POINT('Ctrl Pts',(-1.65361423023729,-23.4288240631043,
12.));
#182733=CARTESIAN_POINT('Ctrl Pts',(-1.64969479707341,-23.4468613776574,
12.));
#182734=CARTESIAN_POINT('Ctrl Pts',(-1.64569902187612,-23.4650053483932,
12.));
#182735=CARTESIAN_POINT('Ctrl Pts',(-1.64162662967529,-23.4832548309645,
12.));
#182736=CARTESIAN_POINT('Ctrl Pts',(-1.63747735129475,-23.5016086970003,
12.));
#182737=CARTESIAN_POINT('Ctrl Pts',(-1.63325092321727,-23.5200658336612,
12.));
#182738=CARTESIAN_POINT('Ctrl Pts',(-1.62894708745224,-23.538625143226,
12.));
#182739=CARTESIAN_POINT('Ctrl Pts',(-1.62456559140065,-23.5572855427601,
12.));
#182740=CARTESIAN_POINT('Ctrl Pts',(-1.62010618772867,-23.57604596376,12.));
#182741=CARTESIAN_POINT('Ctrl Pts',(-1.61556863424699,-23.5949053517997,
12.));
#182742=CARTESIAN_POINT('Ctrl Pts',(-1.61095269379779,-23.6138626661653,
12.));
#182743=CARTESIAN_POINT('Ctrl Pts',(-1.60625813414674,-23.6329168794929,
12.));
#182744=CARTESIAN_POINT('Ctrl Pts',(-1.60148472786596,-23.6520669774876,
12.));
#182745=CARTESIAN_POINT('Ctrl Pts',(-1.59663225222464,-23.671311958631,
12.));
#182746=CARTESIAN_POINT('Ctrl Pts',(-1.59170048908634,-23.6906508338833,
12.));
#182747=CARTESIAN_POINT('Ctrl Pts',(-1.58668922481222,-23.710082626383,
12.));
#182748=CARTESIAN_POINT('Ctrl Pts',(-1.58159825017359,-23.72960637113,12.));
#182749=CARTESIAN_POINT('Ctrl Pts',(-1.57642736025247,-23.749221114736,
12.));
#182750=CARTESIAN_POINT('Ctrl Pts',(-1.57117635434409,-23.7689259151862,
12.));
#182751=CARTESIAN_POINT('Ctrl Pts',(-1.56584503586844,-23.7887198415878,
12.));
#182752=CARTESIAN_POINT('Ctrl Pts',(-1.56043321228635,-23.8086019739194,
12.));
#182753=CARTESIAN_POINT('Ctrl Pts',(-1.55494069502636,-23.8285714027636,
12.));
#182754=CARTESIAN_POINT('Ctrl Pts',(-1.54936729940542,-23.8486272290705,
12.));
#182755=CARTESIAN_POINT('Ctrl Pts',(-1.54371284453991,-23.8687685639642,
12.));
#182756=CARTESIAN_POINT('Ctrl Pts',(-1.53797715326759,-23.8889945285318,
12.));
#182757=CARTESIAN_POINT('Ctrl Pts',(-1.53216005207464,-23.9093042536119,
12.));
#182758=CARTESIAN_POINT('Ctrl Pts',(-1.52626137103033,-23.9296968795757,
12.));
#182759=CARTESIAN_POINT('Ctrl Pts',(-1.52028094372793,-23.9501715561033,
12.));
#182760=CARTESIAN_POINT('Ctrl Pts',(-1.51421860720615,-23.970727442014,
12.));
#182761=CARTESIAN_POINT('Ctrl Pts',(-1.50807420187695,-23.9913637050927,
12.));
#182762=CARTESIAN_POINT('Ctrl Pts',(-1.501847571461,-24.0120795219086,12.));
#182763=CARTESIAN_POINT('Ctrl Pts',(-1.49553856292802,-24.0328740776331,
12.));
#182764=CARTESIAN_POINT('Ctrl Pts',(-1.48914702644888,-24.0537465658429,
12.));
#182765=CARTESIAN_POINT('Ctrl Pts',(-1.48267281533684,-24.0746961883528,
12.));
#182766=CARTESIAN_POINT('Ctrl Pts',(-1.47611578597743,-24.0957221550778,
12.));
#182767=CARTESIAN_POINT('Ctrl Pts',(-1.46947579776992,-24.1168236838824,
12.));
#182768=CARTESIAN_POINT('Ctrl Pts',(-1.46275271307399,-24.1380000004272,
12.));
#182769=CARTESIAN_POINT('Ctrl Pts',(-1.45594639716319,-24.1592503380107,
12.));
#182770=CARTESIAN_POINT('Ctrl Pts',(-1.44905671818729,-24.1805739374038,
12.));
#182771=CARTESIAN_POINT('Ctrl Pts',(-1.44208354711083,-24.201970046722,
12.));
#182772=CARTESIAN_POINT('Ctrl Pts',(-1.43502675765509,-24.2234379212984,
12.));
#182773=CARTESIAN_POINT('Ctrl Pts',(-1.42788622624855,-24.2449768235488,
12.));
#182774=CARTESIAN_POINT('Ctrl Pts',(-1.42066183198254,-24.2665860228356,
12.));
#182775=CARTESIAN_POINT('Ctrl Pts',(-1.41335345657684,-24.288264795321,
12.));
#182776=CARTESIAN_POINT('Ctrl Pts',(-1.40596098434338,-24.3100124238311,
12.));
#182777=CARTESIAN_POINT('Ctrl Pts',(-1.39848430212808,-24.3318281977643,
12.));
#182778=CARTESIAN_POINT('Ctrl Pts',(-1.39092329926389,-24.3537114129875,
12.));
#182779=CARTESIAN_POINT('Ctrl Pts',(-1.38327786753,-24.3756613717299,12.));
#182780=CARTESIAN_POINT('Ctrl Pts',(-1.3755479011161,-24.3976773824732,
12.));
#182781=CARTESIAN_POINT('Ctrl Pts',(-1.36773329659957,-24.4197587598337,
12.));
#182782=CARTESIAN_POINT('Ctrl Pts',(-1.35983395290628,-24.4419048244523,
12.));
#182783=CARTESIAN_POINT('Ctrl Pts',(-1.35184977125649,-24.4641149028892,
12.));
#182784=CARTESIAN_POINT('Ctrl Pts',(-1.34378065512339,-24.4863883275134,
12.));
#182785=CARTESIAN_POINT('Ctrl Pts',(-1.33562651019687,-24.5087244363856,
12.));
#182786=CARTESIAN_POINT('Ctrl Pts',(-1.32738724435327,-24.5311225731435,
12.));
#182787=CARTESIAN_POINT('Ctrl Pts',(-1.31906276763669,-24.5535820868674,
12.));
#182788=CARTESIAN_POINT('Ctrl Pts',(-1.31065299222023,-24.5761023320183,
12.));
#182789=CARTESIAN_POINT('Ctrl Pts',(-1.30215783236363,-24.5986826684027,
12.));
#182790=CARTESIAN_POINT('Ctrl Pts',(-1.29357720438108,-24.6213224611229,
12.));
#182791=CARTESIAN_POINT('Ctrl Pts',(-1.28491102661515,-24.6440210805278,
12.));
#182792=CARTESIAN_POINT('Ctrl Pts',(-1.27615921941643,-24.6667779021559,
12.));
#182793=CARTESIAN_POINT('Ctrl Pts',(-1.26732170513501,-24.6895923066836,
12.));
#182794=CARTESIAN_POINT('Ctrl Pts',(-1.25839840807419,-24.7124636797894,
12.));
#182795=CARTESIAN_POINT('Ctrl Pts',(-1.24938925444327,-24.7353914120011,
12.));
#182796=CARTESIAN_POINT('Ctrl Pts',(-1.2402941723199,-24.7583748985438,
12.));
#182797=CARTESIAN_POINT('Ctrl Pts',(-1.23111309161845,-24.7814135391799,
12.));
#182798=CARTESIAN_POINT('Ctrl Pts',(-1.22184594406529,-24.8045067380536,
12.));
#182799=CARTESIAN_POINT('Ctrl Pts',(-1.21249266318209,-24.8276539035092,
12.));
#182800=CARTESIAN_POINT('Ctrl Pts',(-1.20305318426021,-24.8508544481974,
12.));
#182801=CARTESIAN_POINT('Ctrl Pts',(-1.19352744434065,-24.8741077892075,
12.));
#182802=CARTESIAN_POINT('Ctrl Pts',(-1.18391538220104,-24.8974133481829,
12.));
#182803=CARTESIAN_POINT('Ctrl Pts',(-1.17421693835042,-24.9207705514448,
12.));
#182804=CARTESIAN_POINT('Ctrl Pts',(-1.16443205502851,-24.9441788300932,
12.));
#182805=CARTESIAN_POINT('Ctrl Pts',(-1.1545606762189,-24.9676376201502,
12.));
#182806=CARTESIAN_POINT('Ctrl Pts',(-1.14460274758202,-24.9911463621433,
12.));
#182807=CARTESIAN_POINT('Ctrl Pts',(-1.13455821638531,-25.0147045006196,
12.));
#182808=CARTESIAN_POINT('Ctrl Pts',(-1.12442703144453,-25.0383114836899,
12.));
#182809=CARTESIAN_POINT('Ctrl Pts',(-1.1142091430689,-25.0619667625336,
12.));
#182810=CARTESIAN_POINT('Ctrl Pts',(-1.10390450301746,-25.0856697909679,
12.));
#182811=CARTESIAN_POINT('Ctrl Pts',(-1.09351306445309,-25.1094200248446,
12.));
#182812=CARTESIAN_POINT('Ctrl Pts',(-1.08303478197189,-25.1332169227413,
12.));
#182813=CARTESIAN_POINT('Ctrl Pts',(-1.07246961165477,-25.157059946931,
12.));
#182814=CARTESIAN_POINT('Ctrl Pts',(-1.06181751111769,-25.1809485642192,
12.));
#182815=CARTESIAN_POINT('Ctrl Pts',(-1.05107843957933,-25.2048822469028,
12.));
#182816=CARTESIAN_POINT('Ctrl Pts',(-1.04025235791508,-25.2288604735086,
12.));
#182817=CARTESIAN_POINT('Ctrl Pts',(-1.02933922876807,-25.2528827300422,
12.));
#182818=CARTESIAN_POINT('Ctrl Pts',(-1.01833901642238,-25.276948508726,
12.));
#182819=CARTESIAN_POINT('Ctrl Pts',(-1.00725168656897,-25.3010573055548,
12.));
#182820=CARTESIAN_POINT('Ctrl Pts',(-0.996077206120636,-25.3252086182968,
12.));
#182821=CARTESIAN_POINT('Ctrl Pts',(-0.984815543003984,-25.3494019441441,
12.));
#182822=CARTESIAN_POINT('Ctrl Pts',(-0.973466666000176,-25.3736367778845,
12.));
#182823=CARTESIAN_POINT('Ctrl Pts',(-0.962030544503155,-25.3979126089163,
12.));
#182824=CARTESIAN_POINT('Ctrl Pts',(-0.950507148597481,-25.4222289223167,
12.));
#182825=CARTESIAN_POINT('Ctrl Pts',(-0.938896449496205,-25.4465852044849,
12.));
#182826=CARTESIAN_POINT('Ctrl Pts',(-0.927198419886107,-25.4709809475009,
12.));
#182827=CARTESIAN_POINT('Ctrl Pts',(-0.915413034335626,-25.4954156541795,
12.));
#182828=CARTESIAN_POINT('Ctrl Pts',(-0.903540269651119,-25.5198888424194,
12.));
#182829=CARTESIAN_POINT('Ctrl Pts',(-0.891580105349052,-25.5444000508211,
12.));
#182830=CARTESIAN_POINT('Ctrl Pts',(-0.879532523834307,-25.5689488408156,
12.));
#182831=CARTESIAN_POINT('Ctrl Pts',(-0.867397509338443,-25.5935347843585,
12.));
#182832=CARTESIAN_POINT('Ctrl Pts',(-0.85517504703656,-25.6181574536049,
12.));
#182833=CARTESIAN_POINT('Ctrl Pts',(-0.842865122120771,-25.6428164100055,
12.));
#182834=CARTESIAN_POINT('Ctrl Pts',(-0.830467718864218,-25.6675111931952,
12.));
#182835=CARTESIAN_POINT('Ctrl Pts',(-0.817982819787476,-25.6922413110194,
12.));
#182836=CARTESIAN_POINT('Ctrl Pts',(-0.805410404554365,-25.7170062262525,
12.));
#182837=CARTESIAN_POINT('Ctrl Pts',(-0.792750451616139,-25.7418053757746,
12.));
#182838=CARTESIAN_POINT('Ctrl Pts',(-0.780002940291976,-25.7666381946955,
12.));
#182839=CARTESIAN_POINT('Ctrl Pts',(-0.76716785265118,-25.7915041383376,
12.));
#182840=CARTESIAN_POINT('Ctrl Pts',(-0.754245175609535,-25.8164027059984,
12.));
#182841=CARTESIAN_POINT('Ctrl Pts',(-0.741234902663818,-25.8413334619055,
12.));
#182842=CARTESIAN_POINT('Ctrl Pts',(-0.728137036482348,-25.8662960624185,
12.));
#182843=CARTESIAN_POINT('Ctrl Pts',(-0.714951588527651,-25.891290261497,
12.));
#182844=CARTESIAN_POINT('Ctrl Pts',(-0.701678575228768,-25.9163158909426,
12.));
#182845=CARTESIAN_POINT('Ctrl Pts',(-0.688318015057743,-25.9413728471909,
12.));
#182846=CARTESIAN_POINT('Ctrl Pts',(-0.677559543209739,-25.9614434297919,
12.));
#182847=CARTESIAN_POINT('Ctrl Pts',(-0.669451306780837,-25.9765104298071,
12.));
#182848=CARTESIAN_POINT('Ctrl Pts',(-0.664028313187638,-25.9865613464773,
12.));
#182849=CARTESIAN_POINT('Ctrl Pts',(-0.661312440730913,-25.991588367311,
12.));
#182850=CARTESIAN_POINT('',(0.66131244073089,-25.991588367311,12.));
#182851=CARTESIAN_POINT('Origin',(0.,0.,12.));
#182852=CARTESIAN_POINT('',(1.76341220531179,-22.4835757167854,12.));
#182853=CARTESIAN_POINT('Ctrl Pts',(0.66131244073089,-25.991588367311,12.));
#182854=CARTESIAN_POINT('Ctrl Pts',(0.664028313188911,-25.9865613464809,
12.));
#182855=CARTESIAN_POINT('Ctrl Pts',(0.669451306784414,-25.9765104298171,
12.));
#182856=CARTESIAN_POINT('Ctrl Pts',(0.677559543215902,-25.9614434298092,
12.));
#182857=CARTESIAN_POINT('Ctrl Pts',(0.688318015065675,-25.941372847213,
12.));
#182858=CARTESIAN_POINT('Ctrl Pts',(0.701678575236601,-25.9163158909645,
12.));
#182859=CARTESIAN_POINT('Ctrl Pts',(0.714951588533752,-25.8912902615141,
12.));
#182860=CARTESIAN_POINT('Ctrl Pts',(0.728137036485876,-25.8662960624285,
12.));
#182861=CARTESIAN_POINT('Ctrl Pts',(0.741234902664695,-25.841333461908,
12.));
#182862=CARTESIAN_POINT('Ctrl Pts',(0.754245175608287,-25.816402705995,
12.));
#182863=CARTESIAN_POINT('Ctrl Pts',(0.767167852648638,-25.7915041383304,
12.));
#182864=CARTESIAN_POINT('Ctrl Pts',(0.780002940289024,-25.7666381946871,
12.));
#182865=CARTESIAN_POINT('Ctrl Pts',(0.792750451613533,-25.7418053757671,
12.));
#182866=CARTESIAN_POINT('Ctrl Pts',(0.805410404552592,-25.7170062262474,
12.));
#182867=CARTESIAN_POINT('Ctrl Pts',(0.817982819786718,-25.6922413110172,
12.));
#182868=CARTESIAN_POINT('Ctrl Pts',(0.830467718864366,-25.6675111931957,
12.));
#182869=CARTESIAN_POINT('Ctrl Pts',(0.842865122121542,-25.6428164100078,
12.));
#182870=CARTESIAN_POINT('Ctrl Pts',(0.855175047037614,-25.618157453608,
12.));
#182871=CARTESIAN_POINT('Ctrl Pts',(0.867397509339468,-25.5935347843616,
12.));
#182872=CARTESIAN_POINT('Ctrl Pts',(0.879532523835088,-25.568948840818,
12.));
#182873=CARTESIAN_POINT('Ctrl Pts',(0.891580105349464,-25.5444000508223,
12.));
#182874=CARTESIAN_POINT('Ctrl Pts',(0.903540269651152,-25.5198888424195,
12.));
#182875=CARTESIAN_POINT('Ctrl Pts',(0.915413034335331,-25.4954156541787,
12.));
#182876=CARTESIAN_POINT('Ctrl Pts',(0.927198419885603,-25.4709809474996,
12.));
#182877=CARTESIAN_POINT('Ctrl Pts',(0.938896449495631,-25.4465852044835,
12.));
#182878=CARTESIAN_POINT('Ctrl Pts',(0.950507148596967,-25.4222289223155,
12.));
#182879=CARTESIAN_POINT('Ctrl Pts',(0.962030544502801,-25.3979126089155,
12.));
#182880=CARTESIAN_POINT('Ctrl Pts',(0.973466666000047,-25.3736367778842,
12.));
#182881=CARTESIAN_POINT('Ctrl Pts',(0.984815543004088,-25.3494019441444,
12.));
#182882=CARTESIAN_POINT('Ctrl Pts',(0.996077206120918,-25.3252086182976,
12.));
#182883=CARTESIAN_POINT('Ctrl Pts',(1.00725168656933,-25.3010573055557,
12.));
#182884=CARTESIAN_POINT('Ctrl Pts',(1.01833901642272,-25.2769485087268,
12.));
#182885=CARTESIAN_POINT('Ctrl Pts',(1.0293392287683,-25.2528827300427,12.));
#182886=CARTESIAN_POINT('Ctrl Pts',(1.04025235791514,-25.2288604735087,
12.));
#182887=CARTESIAN_POINT('Ctrl Pts',(1.05107843957925,-25.2048822469027,
12.));
#182888=CARTESIAN_POINT('Ctrl Pts',(1.06181751111754,-25.1809485642191,
12.));
#182889=CARTESIAN_POINT('Ctrl Pts',(1.07246961165459,-25.1570599469311,
12.));
#182890=CARTESIAN_POINT('Ctrl Pts',(1.08303478197174,-25.1332169227415,
12.));
#182891=CARTESIAN_POINT('Ctrl Pts',(1.09351306445299,-25.1094200248448,
12.));
#182892=CARTESIAN_POINT('Ctrl Pts',(1.1039045030174,-25.085669790968,12.));
#182893=CARTESIAN_POINT('Ctrl Pts',(1.1142091430689,-25.0619667625336,12.));
#182894=CARTESIAN_POINT('Ctrl Pts',(1.12442703144455,-25.0383114836898,
12.));
#182895=CARTESIAN_POINT('Ctrl Pts',(1.13455821638535,-25.0147045006193,
12.));
#182896=CARTESIAN_POINT('Ctrl Pts',(1.14460274758206,-24.9911463621431,
12.));
#182897=CARTESIAN_POINT('Ctrl Pts',(1.15456067621894,-24.9676376201501,
12.));
#182898=CARTESIAN_POINT('Ctrl Pts',(1.16443205502852,-24.9441788300932,
12.));
#182899=CARTESIAN_POINT('Ctrl Pts',(1.17421693835039,-24.9207705514449,
12.));
#182900=CARTESIAN_POINT('Ctrl Pts',(1.18391538220098,-24.8974133481829,
12.));
#182901=CARTESIAN_POINT('Ctrl Pts',(1.19352744434059,-24.8741077892074,
12.));
#182902=CARTESIAN_POINT('Ctrl Pts',(1.20305318426015,-24.8508544481973,
12.));
#182903=CARTESIAN_POINT('Ctrl Pts',(1.21249266318205,-24.8276539035092,
12.));
#182904=CARTESIAN_POINT('Ctrl Pts',(1.22184594406526,-24.8045067380536,
12.));
#182905=CARTESIAN_POINT('Ctrl Pts',(1.23111309161843,-24.78141353918,12.));
#182906=CARTESIAN_POINT('Ctrl Pts',(1.24029417231987,-24.7583748985439,
12.));
#182907=CARTESIAN_POINT('Ctrl Pts',(1.24938925444323,-24.7353914120012,
12.));
#182908=CARTESIAN_POINT('Ctrl Pts',(1.25839840807414,-24.7124636797895,
12.));
#182909=CARTESIAN_POINT('Ctrl Pts',(1.26732170513497,-24.6895923066837,
12.));
#182910=CARTESIAN_POINT('Ctrl Pts',(1.2761592194164,-24.666777902156,12.));
#182911=CARTESIAN_POINT('Ctrl Pts',(1.28491102661513,-24.6440210805278,
12.));
#182912=CARTESIAN_POINT('Ctrl Pts',(1.29357720438107,-24.6213224611228,
12.));
#182913=CARTESIAN_POINT('Ctrl Pts',(1.30215783236363,-24.5986826684025,
12.));
#182914=CARTESIAN_POINT('Ctrl Pts',(1.31065299222023,-24.576102332018,12.));
#182915=CARTESIAN_POINT('Ctrl Pts',(1.31906276763669,-24.5535820868671,
12.));
#182916=CARTESIAN_POINT('Ctrl Pts',(1.32738724435326,-24.5311225731434,
12.));
#182917=CARTESIAN_POINT('Ctrl Pts',(1.33562651019684,-24.5087244363856,
12.));
#182918=CARTESIAN_POINT('Ctrl Pts',(1.34378065512335,-24.4863883275135,
12.));
#182919=CARTESIAN_POINT('Ctrl Pts',(1.35184977125644,-24.4641149028894,
12.));
#182920=CARTESIAN_POINT('Ctrl Pts',(1.35983395290624,-24.4419048244524,
12.));
#182921=CARTESIAN_POINT('Ctrl Pts',(1.36773329659954,-24.4197587598337,
12.));
#182922=CARTESIAN_POINT('Ctrl Pts',(1.37554790111607,-24.3976773824731,
12.));
#182923=CARTESIAN_POINT('Ctrl Pts',(1.38327786752998,-24.37566137173,12.));
#182924=CARTESIAN_POINT('Ctrl Pts',(1.3909232992639,-24.3537114129877,12.));
#182925=CARTESIAN_POINT('Ctrl Pts',(1.3984843021281,-24.3318281977647,12.));
#182926=CARTESIAN_POINT('Ctrl Pts',(1.4059609843434,-24.3100124238316,12.));
#182927=CARTESIAN_POINT('Ctrl Pts',(1.41335345657684,-24.2882647953214,
12.));
#182928=CARTESIAN_POINT('Ctrl Pts',(1.42066183198252,-24.2665860228357,
12.));
#182929=CARTESIAN_POINT('Ctrl Pts',(1.42788622624851,-24.2449768235485,
12.));
#182930=CARTESIAN_POINT('Ctrl Pts',(1.43502675765502,-24.2234379212978,
12.));
#182931=CARTESIAN_POINT('Ctrl Pts',(1.44208354711074,-24.2019700467214,
12.));
#182932=CARTESIAN_POINT('Ctrl Pts',(1.4490567181872,-24.1805739374033,12.));
#182933=CARTESIAN_POINT('Ctrl Pts',(1.45594639716314,-24.1592503380105,
12.));
#182934=CARTESIAN_POINT('Ctrl Pts',(1.46275271307398,-24.1380000004272,
12.));
#182935=CARTESIAN_POINT('Ctrl Pts',(1.46947579776991,-24.1168236838827,
12.));
#182936=CARTESIAN_POINT('Ctrl Pts',(1.47611578597741,-24.0957221550782,
12.));
#182937=CARTESIAN_POINT('Ctrl Pts',(1.4826728153368,-24.074696188353,12.));
#182938=CARTESIAN_POINT('Ctrl Pts',(1.48914702644883,-24.053746565843,12.));
#182939=CARTESIAN_POINT('Ctrl Pts',(1.49553856292798,-24.0328740776331,
12.));
#182940=CARTESIAN_POINT('Ctrl Pts',(1.50184757146099,-24.0120795219086,
12.));
#182941=CARTESIAN_POINT('Ctrl Pts',(1.50807420187702,-23.991363705093,12.));
#182942=CARTESIAN_POINT('Ctrl Pts',(1.51421860720628,-23.9707274420145,
12.));
#182943=CARTESIAN_POINT('Ctrl Pts',(1.52028094372806,-23.9501715561038,
12.));
#182944=CARTESIAN_POINT('Ctrl Pts',(1.52626137103039,-23.9296968795761,
12.));
#182945=CARTESIAN_POINT('Ctrl Pts',(1.53216005207462,-23.9093042536119,
12.));
#182946=CARTESIAN_POINT('Ctrl Pts',(1.53797715326748,-23.8889945285313,
12.));
#182947=CARTESIAN_POINT('Ctrl Pts',(1.54371284453977,-23.8687685639635,
12.));
#182948=CARTESIAN_POINT('Ctrl Pts',(1.5493672994053,-23.8486272290698,12.));
#182949=CARTESIAN_POINT('Ctrl Pts',(1.55494069502627,-23.8285714027631,
12.));
#182950=CARTESIAN_POINT('Ctrl Pts',(1.56043321228631,-23.8086019739192,
12.));
#182951=CARTESIAN_POINT('Ctrl Pts',(1.56584503586844,-23.788719841588,12.));
#182952=CARTESIAN_POINT('Ctrl Pts',(1.57117635434412,-23.7689259151869,
12.));
#182953=CARTESIAN_POINT('Ctrl Pts',(1.57642736025251,-23.7492211147369,
12.));
#182954=CARTESIAN_POINT('Ctrl Pts',(1.58159825017362,-23.7296063711308,
12.));
#182955=CARTESIAN_POINT('Ctrl Pts',(1.58668922481222,-23.7100826263835,
12.));
#182956=CARTESIAN_POINT('Ctrl Pts',(1.59170048908631,-23.6906508338833,
12.));
#182957=CARTESIAN_POINT('Ctrl Pts',(1.59663225222458,-23.6713119586302,
12.));
#182958=CARTESIAN_POINT('Ctrl Pts',(1.60148472786588,-23.6520669774863,
12.));
#182959=CARTESIAN_POINT('Ctrl Pts',(1.60625813414666,-23.6329168794916,
12.));
#182960=CARTESIAN_POINT('Ctrl Pts',(1.61095269379773,-23.6138626661644,
12.));
#182961=CARTESIAN_POINT('Ctrl Pts',(1.61556863424697,-23.5949053517996,
12.));
#182962=CARTESIAN_POINT('Ctrl Pts',(1.62010618772869,-23.5760459637608,
12.));
#182963=CARTESIAN_POINT('Ctrl Pts',(1.62456559140071,-23.5572855427617,
12.));
#182964=CARTESIAN_POINT('Ctrl Pts',(1.62894708745231,-23.5386251432278,
12.));
#182965=CARTESIAN_POINT('Ctrl Pts',(1.63325092321731,-23.5200658336624,
12.));
#182966=CARTESIAN_POINT('Ctrl Pts',(1.63747735129474,-23.5016086970006,
12.));
#182967=CARTESIAN_POINT('Ctrl Pts',(1.64162662967524,-23.4832548309638,
12.));
#182968=CARTESIAN_POINT('Ctrl Pts',(1.64569902187608,-23.4650053483919,
12.));
#182969=CARTESIAN_POINT('Ctrl Pts',(1.64969479707339,-23.446861377656,12.));
#182970=CARTESIAN_POINT('Ctrl Pts',(1.6536142302373,-23.4288240631034,12.));
#182971=CARTESIAN_POINT('Ctrl Pts',(1.65745760227507,-23.4108945654803,
12.));
#182972=CARTESIAN_POINT('Ctrl Pts',(1.66122520018008,-23.3930740623622,
12.));
#182973=CARTESIAN_POINT('Ctrl Pts',(1.66491731718864,-23.375363748555,12.));
#182974=CARTESIAN_POINT('Ctrl Pts',(1.66853425293977,-23.3577648365747,
12.));
#182975=CARTESIAN_POINT('Ctrl Pts',(1.67207631363905,-23.3402785571866,
12.));
#182976=CARTESIAN_POINT('Ctrl Pts',(1.67554381222987,-23.3229061599145,
12.));
#182977=CARTESIAN_POINT('Ctrl Pts',(1.67893706857123,-23.3056489135611,
12.));
#182978=CARTESIAN_POINT('Ctrl Pts',(1.68225640962181,-23.2885081066949,
12.));
#182979=CARTESIAN_POINT('Ctrl Pts',(1.68550216963274,-23.2714850482245,
12.));
#182980=CARTESIAN_POINT('Ctrl Pts',(1.6886746903491,-23.2545810680536,12.));
#182981=CARTESIAN_POINT('Ctrl Pts',(1.69177432121716,-23.2377975177014,
12.));
#182982=CARTESIAN_POINT('Ctrl Pts',(1.69480141959945,-23.2211357709374,
12.));
#182983=CARTESIAN_POINT('Ctrl Pts',(1.69775635099425,-23.2045972243765,
12.));
#182984=CARTESIAN_POINT('Ctrl Pts',(1.70063948926987,-23.1881832981848,
12.));
#182985=CARTESIAN_POINT('Ctrl Pts',(1.70345121691259,-23.1718954368749,
12.));
#182986=CARTESIAN_POINT('Ctrl Pts',(1.70619192527846,-23.1557351100613,
12.));
#182987=CARTESIAN_POINT('Ctrl Pts',(1.70886201485459,-23.1397038132358,
12.));
#182988=CARTESIAN_POINT('Ctrl Pts',(1.71146189552192,-23.1238030684929,
12.));
#182989=CARTESIAN_POINT('Ctrl Pts',(1.71399198684724,-23.1080344254291,
12.));
#182990=CARTESIAN_POINT('Ctrl Pts',(1.71645271839311,-23.0923994621216,
12.));
#182991=CARTESIAN_POINT('Ctrl Pts',(1.71884453003027,-23.0768997860709,
12.));
#182992=CARTESIAN_POINT('Ctrl Pts',(1.7211678722598,-23.061537035156,12.));
#182993=CARTESIAN_POINT('Ctrl Pts',(1.72342320653731,-23.0463128785528,
12.));
#182994=CARTESIAN_POINT('Ctrl Pts',(1.72561100564033,-23.031229017888,12.));
#182995=CARTESIAN_POINT('Ctrl Pts',(1.72773175404702,-23.0162871884167,
12.));
#182996=CARTESIAN_POINT('Ctrl Pts',(1.72978594832137,-23.0014891601891,
12.));
#182997=CARTESIAN_POINT('Ctrl Pts',(1.73177409750193,-22.9868367391978,
12.));
#182998=CARTESIAN_POINT('Ctrl Pts',(1.73369672350817,-22.9723317685688,
12.));
#182999=CARTESIAN_POINT('Ctrl Pts',(1.73555436162771,-22.9579761301062,
12.));
#183000=CARTESIAN_POINT('Ctrl Pts',(1.73734756100038,-22.9437717457825,
12.));
#183001=CARTESIAN_POINT('Ctrl Pts',(1.73907688511664,-22.9297205792587,
12.));
#183002=CARTESIAN_POINT('Ctrl Pts',(1.74074291231056,-22.9158246373365,
12.));
#183003=CARTESIAN_POINT('Ctrl Pts',(1.74234623630079,-22.9020859716144,
12.));
#183004=CARTESIAN_POINT('Ctrl Pts',(1.74388746677702,-22.8885066803351,
12.));
#183005=CARTESIAN_POINT('Ctrl Pts',(1.74536722998199,-22.8750889101696,
12.));
#183006=CARTESIAN_POINT('Ctrl Pts',(1.74678616930663,-22.8618348580234,
12.));
#183007=CARTESIAN_POINT('Ctrl Pts',(1.74814494588491,-22.8487467728075,
12.));
#183008=CARTESIAN_POINT('Ctrl Pts',(1.74944423940117,-22.8358269579854,
12.));
#183009=CARTESIAN_POINT('Ctrl Pts',(1.75068474890883,-22.8230777741285,
12.));
#183010=CARTESIAN_POINT('Ctrl Pts',(1.75186719365589,-22.8105016414712,
12.));
#183011=CARTESIAN_POINT('Ctrl Pts',(1.75299231391461,-22.7981010424312,
12.));
#183012=CARTESIAN_POINT('Ctrl Pts',(1.75406087182929,-22.7858785242358,
12.));
#183013=CARTESIAN_POINT('Ctrl Pts',(1.75507365227127,-22.7738367016115,
12.));
#183014=CARTESIAN_POINT('Ctrl Pts',(1.7560314637164,-22.7619782595013,12.));
#183015=CARTESIAN_POINT('Ctrl Pts',(1.75693513908911,-22.7503059556455,
12.));
#183016=CARTESIAN_POINT('Ctrl Pts',(1.75778553673249,-22.7388226235565,
12.));
#183017=CARTESIAN_POINT('Ctrl Pts',(1.75858354204634,-22.7275311777305,
12.));
#183018=CARTESIAN_POINT('Ctrl Pts',(1.75933006905924,-22.7164346186007,
12.));
#183019=CARTESIAN_POINT('Ctrl Pts',(1.76002606202398,-22.7055360375481,
12.));
#183020=CARTESIAN_POINT('Ctrl Pts',(1.76067249704884,-22.6948386219843,
12.));
#183021=CARTESIAN_POINT('Ctrl Pts',(1.76127038310612,-22.6843456585245,
12.));
#183022=CARTESIAN_POINT('Ctrl Pts',(1.76182076289525,-22.6740605356699,
12.));
#183023=CARTESIAN_POINT('Ctrl Pts',(1.76232471392567,-22.6639867471756,
12.));
#183024=CARTESIAN_POINT('Ctrl Pts',(1.76278334912559,-22.6541278938413,
12.));
#183025=CARTESIAN_POINT('Ctrl Pts',(1.76319782013913,-22.6444876940425,
12.));
#183026=CARTESIAN_POINT('Ctrl Pts',(1.76356932176272,-22.635069997936,12.));
#183027=CARTESIAN_POINT('Ctrl Pts',(1.76389909571402,-22.6258787994847,
12.));
#183028=CARTESIAN_POINT('Ctrl Pts',(1.76418843543739,-22.6169182517693,
12.));
#183029=CARTESIAN_POINT('Ctrl Pts',(1.76443868648015,-22.6081926681342,
12.));
#183030=CARTESIAN_POINT('Ctrl Pts',(1.76465124413556,-22.5997065145638,
12.));
#183031=CARTESIAN_POINT('Ctrl Pts',(1.76482755288411,-22.5914644078106,
12.));
#183032=CARTESIAN_POINT('Ctrl Pts',(1.76496910283088,-22.5834711038024,
12.));
#183033=CARTESIAN_POINT('Ctrl Pts',(1.76507744026747,-22.5757315316355,
12.));
#183034=CARTESIAN_POINT('Ctrl Pts',(1.76515418518829,-22.5682508499873,
12.));
#183035=CARTESIAN_POINT('Ctrl Pts',(1.76520104500449,-22.5610344912501,
12.));
#183036=CARTESIAN_POINT('Ctrl Pts',(1.76521983384062,-22.5540882235837,
12.));
#183037=CARTESIAN_POINT('Ctrl Pts',(1.76521245524047,-22.5474180954006,
12.));
#183038=CARTESIAN_POINT('Ctrl Pts',(1.76518087841492,-22.5410303590891,
12.));
#183039=CARTESIAN_POINT('Ctrl Pts',(1.7651271156325,-22.5349313983571,12.));
#183040=CARTESIAN_POINT('Ctrl Pts',(1.76505320262751,-22.529127665298,12.));
#183041=CARTESIAN_POINT('Ctrl Pts',(1.76496128643369,-22.5236259635515,
12.));
#183042=CARTESIAN_POINT('Ctrl Pts',(1.76485369319896,-22.5184336670207,
12.));
#183043=CARTESIAN_POINT('Ctrl Pts',(1.76473303281158,-22.5135590569554,
12.));
#183044=CARTESIAN_POINT('Ctrl Pts',(1.76460218257323,-22.5090112700212,
12.));
#183045=CARTESIAN_POINT('Ctrl Pts',(1.76446408210366,-22.5047996391978,
12.));
#183046=CARTESIAN_POINT('Ctrl Pts',(1.76432160068725,-22.5009332677316,
12.));
#183047=CARTESIAN_POINT('Ctrl Pts',(1.76417731243462,-22.4974203063191,
12.));
#183048=CARTESIAN_POINT('Ctrl Pts',(1.764033938803,-22.4942693792449,12.));
#183049=CARTESIAN_POINT('Ctrl Pts',(1.76389475965723,-22.4914909094908,
12.));
#183050=CARTESIAN_POINT('Ctrl Pts',(1.76376424879504,-22.4890991659478,
12.));
#183051=CARTESIAN_POINT('Ctrl Pts',(1.76364784232963,-22.4871115206571,
12.));
#183052=CARTESIAN_POINT('Ctrl Pts',(1.76355076045546,-22.4855446605991,
12.));
#183053=CARTESIAN_POINT('Ctrl Pts',(1.76347698284791,-22.4844112933129,
12.));
#183054=CARTESIAN_POINT('Ctrl Pts',(1.76343813434565,-22.483856251707,12.));
#183055=CARTESIAN_POINT('Ctrl Pts',(1.7634206426357,-22.4836387052232,12.));
#183056=CARTESIAN_POINT('Ctrl Pts',(1.76341415538764,-22.483581992979,12.));
#183057=CARTESIAN_POINT('Ctrl Pts',(1.76341220531179,-22.4835757167854,
12.));
#183058=CARTESIAN_POINT('',(1.71975774210841,-21.9269795755927,12.));
#183059=CARTESIAN_POINT('',(0.840553282521226,-10.7170877657712,12.));
#183060=CARTESIAN_POINT('',(2.16781269186827,-21.3904321633055,12.));
#183061=CARTESIAN_POINT('Origin',(2.21822694051637,-21.8878840740801,12.));
#183062=CARTESIAN_POINT('',(3.44230496120418,-21.2226420728916,12.));
#183063=CARTESIAN_POINT('Origin',(7.16093850883225E-14,-7.7715611723761E-13,
12.));
#183064=CARTESIAN_POINT('',(4.01396149767428,-21.624941921198,12.));
#183065=CARTESIAN_POINT('Origin',(3.52235856495312,-21.7161918885403,12.));
#183066=CARTESIAN_POINT('',(4.11585220600461,-22.1738711152697,12.));
#183067=CARTESIAN_POINT('',(2.05792610300232,-11.0869355576349,12.));
#183068=CARTESIAN_POINT('',(6.08833931617698,-25.2771067246846,12.));
#183069=CARTESIAN_POINT('Ctrl Pts',(4.11585220600461,-22.1738711152697,
12.));
#183070=CARTESIAN_POINT('Ctrl Pts',(4.11585194677412,-22.1738776823239,
12.));
#183071=CARTESIAN_POINT('Ctrl Pts',(4.1158603587821,-22.1739341411684,12.));
#183072=CARTESIAN_POINT('Ctrl Pts',(4.11589976826061,-22.174148802123,12.));
#183073=CARTESIAN_POINT('Ctrl Pts',(4.11600589882767,-22.1746949858773,
12.));
#183074=CARTESIAN_POINT('Ctrl Pts',(4.11622797217066,-22.1758088296598,
12.));
#183075=CARTESIAN_POINT('Ctrl Pts',(4.11653973150558,-22.177347426894,12.));
#183076=CARTESIAN_POINT('Ctrl Pts',(4.11694173195041,-22.179297473024,12.));
#183077=CARTESIAN_POINT('Ctrl Pts',(4.11743469691765,-22.1816414985788,
12.));
#183078=CARTESIAN_POINT('Ctrl Pts',(4.11801938107464,-22.1843613164855,
12.));
#183079=CARTESIAN_POINT('Ctrl Pts',(4.11869641271752,-22.1874419861496,
12.));
#183080=CARTESIAN_POINT('Ctrl Pts',(4.11946626228623,-22.1908725908525,
12.));
#183081=CARTESIAN_POINT('Ctrl Pts',(4.12032932637738,-22.1946440958098,
12.));
#183082=CARTESIAN_POINT('Ctrl Pts',(4.12128598183533,-22.1987479618246,
12.));
#183083=CARTESIAN_POINT('Ctrl Pts',(4.12233664408237,-22.2031746532106,
12.));
#183084=CARTESIAN_POINT('Ctrl Pts',(4.12348173702024,-22.2079143941719,
12.));
#183085=CARTESIAN_POINT('Ctrl Pts',(4.12472167516602,-22.2129576146671,
12.));
#183086=CARTESIAN_POINT('Ctrl Pts',(4.12605683613299,-22.2182956401341,
12.));
#183087=CARTESIAN_POINT('Ctrl Pts',(4.12748755830099,-22.2239207458781,
12.));
#183088=CARTESIAN_POINT('Ctrl Pts',(4.12901415463378,-22.2298258043947,
12.));
#183089=CARTESIAN_POINT('Ctrl Pts',(4.13063692157499,-22.2360040565534,
12.));
#183090=CARTESIAN_POINT('Ctrl Pts',(4.1323561506016,-22.2424488153523,12.));
#183091=CARTESIAN_POINT('Ctrl Pts',(4.13417212558808,-22.2491535317789,
12.));
#183092=CARTESIAN_POINT('Ctrl Pts',(4.13608511977226,-22.2561118708422,
12.));
#183093=CARTESIAN_POINT('Ctrl Pts',(4.13809539255418,-22.263317791397,12.));
#183094=CARTESIAN_POINT('Ctrl Pts',(4.14020318715987,-22.2707656042456,
12.));
#183095=CARTESIAN_POINT('Ctrl Pts',(4.14240873321982,-22.2784499072026,
12.));
#183096=CARTESIAN_POINT('Ctrl Pts',(4.14471224859295,-22.2863655389167,
12.));
#183097=CARTESIAN_POINT('Ctrl Pts',(4.14711394168559,-22.2945075198468,
12.));
#183098=CARTESIAN_POINT('Ctrl Pts',(4.14961401285525,-22.3028710166935,
12.));
#183099=CARTESIAN_POINT('Ctrl Pts',(4.15221265396992,-22.3114513545186,
12.));
#183100=CARTESIAN_POINT('Ctrl Pts',(4.15491004835278,-22.3202440186979,
12.));
#183101=CARTESIAN_POINT('Ctrl Pts',(4.15770637047882,-22.3292446628957,
12.));
#183102=CARTESIAN_POINT('Ctrl Pts',(4.16060178604153,-22.3384491078599,
12.));
#183103=CARTESIAN_POINT('Ctrl Pts',(4.1635964526318,-22.3478533253886,12.));
#183104=CARTESIAN_POINT('Ctrl Pts',(4.16669052026602,-22.3574534257397,
12.));
#183105=CARTESIAN_POINT('Ctrl Pts',(4.16988413199469,-22.3672456427605,
12.));
#183106=CARTESIAN_POINT('Ctrl Pts',(4.17317742436162,-22.3772263228624,
12.));
#183107=CARTESIAN_POINT('Ctrl Pts',(4.17657052752834,-22.3873919231339,
12.));
#183108=CARTESIAN_POINT('Ctrl Pts',(4.18006356544879,-22.3977390078074,
12.));
#183109=CARTESIAN_POINT('Ctrl Pts',(4.18365665600839,-22.4082642454448,
12.));
#183110=CARTESIAN_POINT('Ctrl Pts',(4.18734991117707,-22.4189644056109,
12.));
#183111=CARTESIAN_POINT('Ctrl Pts',(4.19114343726932,-22.4298363535416,
12.));
#183112=CARTESIAN_POINT('Ctrl Pts',(4.1950373351886,-22.4408770448917,12.));
#183113=CARTESIAN_POINT('Ctrl Pts',(4.19903170066358,-22.4520835205422,
12.));
#183114=CARTESIAN_POINT('Ctrl Pts',(4.20312662448174,-22.4634529011437,
12.));
#183115=CARTESIAN_POINT('Ctrl Pts',(4.20732219265648,-22.4749823839917,
12.));
#183116=CARTESIAN_POINT('Ctrl Pts',(4.21161848657428,-22.4866692403147,
12.));
#183117=CARTESIAN_POINT('Ctrl Pts',(4.21601558313906,-22.4985108124228,
12.));
#183118=CARTESIAN_POINT('Ctrl Pts',(4.22051355490196,-22.5105045108881,
12.));
#183119=CARTESIAN_POINT('Ctrl Pts',(4.22511247020041,-22.5226478117886,
12.));
#183120=CARTESIAN_POINT('Ctrl Pts',(4.22981239330733,-22.5349382540588,
12.));
#183121=CARTESIAN_POINT('Ctrl Pts',(4.23461338456712,-22.5473734368086,
12.));
#183122=CARTESIAN_POINT('Ctrl Pts',(4.23951550052522,-22.5599510166429,
12.));
#183123=CARTESIAN_POINT('Ctrl Pts',(4.24451879404851,-22.572668704992,12.));
#183124=CARTESIAN_POINT('Ctrl Pts',(4.24962331444177,-22.5855242662477,
12.));
#183125=CARTESIAN_POINT('Ctrl Pts',(4.25482910755481,-22.5985155158636,
12.));
#183126=CARTESIAN_POINT('Ctrl Pts',(4.26013621588305,-22.6116403184821,
12.));
#183127=CARTESIAN_POINT('Ctrl Pts',(4.26554467865576,-22.6248965859977,
12.));
#183128=CARTESIAN_POINT('Ctrl Pts',(4.27105453193004,-22.6382822758172,
12.));
#183129=CARTESIAN_POINT('Ctrl Pts',(4.2766658086912,-22.6517953893303,12.));
#183130=CARTESIAN_POINT('Ctrl Pts',(4.28237853894058,-22.6654339703109,
12.));
#183131=CARTESIAN_POINT('Ctrl Pts',(4.28819274977763,-22.6791961033538,
12.));
#183132=CARTESIAN_POINT('Ctrl Pts',(4.29410846547056,-22.6930799122548,
12.));
#183133=CARTESIAN_POINT('Ctrl Pts',(4.3001257075406,-22.7070835587564,12.));
#183134=CARTESIAN_POINT('Ctrl Pts',(4.30624449484069,-22.7212052413386,
12.));
#183135=CARTESIAN_POINT('Ctrl Pts',(4.31246484362549,-22.7354431939926,
12.));
#183136=CARTESIAN_POINT('Ctrl Pts',(4.31878676761235,-22.7497956849848,
12.));
#183137=CARTESIAN_POINT('Ctrl Pts',(4.32521027803754,-22.7642610156475,
12.));
#183138=CARTESIAN_POINT('Ctrl Pts',(4.33173538373189,-22.7788375194076,
12.));
#183139=CARTESIAN_POINT('Ctrl Pts',(4.33836209118446,-22.7935235607806,
12.));
#183140=CARTESIAN_POINT('Ctrl Pts',(4.34509040460062,-22.8083175343791,
12.));
#183141=CARTESIAN_POINT('Ctrl Pts',(4.3519203259479,-22.8232178638876,12.));
#183142=CARTESIAN_POINT('Ctrl Pts',(4.35885185500546,-22.8382230011184,
12.));
#183143=CARTESIAN_POINT('Ctrl Pts',(4.36588498942997,-22.8533314252422,
12.));
#183144=CARTESIAN_POINT('Ctrl Pts',(4.37301972480745,-22.8685416419725,
12.));
#183145=CARTESIAN_POINT('Ctrl Pts',(4.38025605470092,-22.8838521827701,
12.));
#183146=CARTESIAN_POINT('Ctrl Pts',(4.38759397068405,-22.8992616040108,
12.));
#183147=CARTESIAN_POINT('Ctrl Pts',(4.39503346238473,-22.9147684862426,
12.));
#183148=CARTESIAN_POINT('Ctrl Pts',(4.40257451754323,-22.930371433555,12.));
#183149=CARTESIAN_POINT('Ctrl Pts',(4.41021712205553,-22.9460690729093,
12.));
#183150=CARTESIAN_POINT('Ctrl Pts',(4.41796126001302,-22.9618600534866,
12.));
#183151=CARTESIAN_POINT('Ctrl Pts',(4.42580691372751,-22.977743046002,12.));
#183152=CARTESIAN_POINT('Ctrl Pts',(4.43375406376879,-22.9937167421006,
12.));
#183153=CARTESIAN_POINT('Ctrl Pts',(4.44180268901643,-23.0097798538395,
12.));
#183154=CARTESIAN_POINT('Ctrl Pts',(4.44995276669686,-23.0259311131392,
12.));
#183155=CARTESIAN_POINT('Ctrl Pts',(4.45820427241683,-23.0421692712467,
12.));
#183156=CARTESIAN_POINT('Ctrl Pts',(4.4665571801823,-23.0584930981732,12.));
#183157=CARTESIAN_POINT('Ctrl Pts',(4.47501146242856,-23.0749013821881,
12.));
#183158=CARTESIAN_POINT('Ctrl Pts',(4.48356709006788,-23.0913929293922,
12.));
#183159=CARTESIAN_POINT('Ctrl Pts',(4.49222403252216,-23.1079665632636,
12.));
#183160=CARTESIAN_POINT('Ctrl Pts',(4.50098225775171,-23.1246211242115,
12.));
#183161=CARTESIAN_POINT('Ctrl Pts',(4.5098417322706,-23.1413554691123,12.));
#183162=CARTESIAN_POINT('Ctrl Pts',(4.51880242116748,-23.1581684708761,
12.));
#183163=CARTESIAN_POINT('Ctrl Pts',(4.52786428815014,-23.1750590180908,
12.));
#183164=CARTESIAN_POINT('Ctrl Pts',(4.53702729557566,-23.1920260146465,
12.));
#183165=CARTESIAN_POINT('Ctrl Pts',(4.54629140447544,-23.2090683793629,
12.));
#183166=CARTESIAN_POINT('Ctrl Pts',(4.55565657456975,-23.2261850456064,
12.));
#183167=CARTESIAN_POINT('Ctrl Pts',(4.56512276427839,-23.2433749609131,
12.));
#183168=CARTESIAN_POINT('Ctrl Pts',(4.57468993076097,-23.2606370866866,
12.));
#183169=CARTESIAN_POINT('Ctrl Pts',(4.5843580299469,-23.2779703978876,12.));
#183170=CARTESIAN_POINT('Ctrl Pts',(4.5941270165575,-23.2953738827191,12.));
#183171=CARTESIAN_POINT('Ctrl Pts',(4.60399684412163,-23.3128465423115,
12.));
#183172=CARTESIAN_POINT('Ctrl Pts',(4.6139674649783,-23.3303873903938,12.));
#183173=CARTESIAN_POINT('Ctrl Pts',(4.62403883030805,-23.3479954530272,
12.));
#183174=CARTESIAN_POINT('Ctrl Pts',(4.63421089016541,-23.3656697683489,
12.));
#183175=CARTESIAN_POINT('Ctrl Pts',(4.6444835934993,-23.3834093863068,12.));
#183176=CARTESIAN_POINT('Ctrl Pts',(4.65485688816924,-23.4012133683959,
12.));
#183177=CARTESIAN_POINT('Ctrl Pts',(4.6653307209467,-23.4190807873803,12.));
#183178=CARTESIAN_POINT('Ctrl Pts',(4.67590503753058,-23.4370107270451,
12.));
#183179=CARTESIAN_POINT('Ctrl Pts',(4.68657978258303,-23.455002281986,12.));
#183180=CARTESIAN_POINT('Ctrl Pts',(4.69735489975024,-23.4730545573853,
12.));
#183181=CARTESIAN_POINT('Ctrl Pts',(4.70823033167818,-23.491166668789,12.));
#183182=CARTESIAN_POINT('Ctrl Pts',(4.71920602001901,-23.509337741878,12.));
#183183=CARTESIAN_POINT('Ctrl Pts',(4.73028190543029,-23.5275669122372,
12.));
#183184=CARTESIAN_POINT('Ctrl Pts',(4.74145792760698,-23.545853325171,12.));
#183185=CARTESIAN_POINT('Ctrl Pts',(4.75273402530617,-23.5641961355168,
12.));
#183186=CARTESIAN_POINT('Ctrl Pts',(4.76411013636251,-23.5825945074535,
12.));
#183187=CARTESIAN_POINT('Ctrl Pts',(4.77558619769872,-23.6010476143099,
12.));
#183188=CARTESIAN_POINT('Ctrl Pts',(4.78716214532097,-23.6195546383624,
12.));
#183189=CARTESIAN_POINT('Ctrl Pts',(4.7988379143322,-23.6381147706579,12.));
#183190=CARTESIAN_POINT('Ctrl Pts',(4.81061343896432,-23.6567272108628,
12.));
#183191=CARTESIAN_POINT('Ctrl Pts',(4.82248865259562,-23.675391167102,12.));
#183192=CARTESIAN_POINT('Ctrl Pts',(4.83446348776265,-23.6941058557971,
12.));
#183193=CARTESIAN_POINT('Ctrl Pts',(4.84653787616425,-23.7128705015017,
12.));
#183194=CARTESIAN_POINT('Ctrl Pts',(4.85871174865499,-23.7316843367313,
12.));
#183195=CARTESIAN_POINT('Ctrl Pts',(4.87098503527152,-23.7505466018245,
12.));
#183196=CARTESIAN_POINT('Ctrl Pts',(4.88335766525573,-23.7694565448049,
12.));
#183197=CARTESIAN_POINT('Ctrl Pts',(4.89582956706775,-23.7884134212384,
12.));
#183198=CARTESIAN_POINT('Ctrl Pts',(4.90840066839344,-23.8074164940896,
12.));
#183199=CARTESIAN_POINT('Ctrl Pts',(4.92107089613968,-23.8264650335717,
12.));
#183200=CARTESIAN_POINT('Ctrl Pts',(4.93384017643432,-23.8455583170057,
12.));
#183201=CARTESIAN_POINT('Ctrl Pts',(4.9467084346586,-23.8646956287168,12.));
#183202=CARTESIAN_POINT('Ctrl Pts',(4.9596755954656,-23.8838762599218,12.));
#183203=CARTESIAN_POINT('Ctrl Pts',(4.97274158279226,-23.9030995086163,
12.));
#183204=CARTESIAN_POINT('Ctrl Pts',(4.98590631986532,-23.9223646794592,
12.));
#183205=CARTESIAN_POINT('Ctrl Pts',(4.99916972919306,-23.9416710836529,
12.));
#183206=CARTESIAN_POINT('Ctrl Pts',(5.01253173257452,-23.9610180388271,
12.));
#183207=CARTESIAN_POINT('Ctrl Pts',(5.02599225112454,-23.9804048689227,
12.));
#183208=CARTESIAN_POINT('Ctrl Pts',(5.03955120528521,-23.9998309040746,
12.));
#183209=CARTESIAN_POINT('Ctrl Pts',(5.05320851483065,-24.0192954804896,
12.));
#183210=CARTESIAN_POINT('Ctrl Pts',(5.06696409886641,-24.0387979403268,
12.));
#183211=CARTESIAN_POINT('Ctrl Pts',(5.08081787581276,-24.0583376315638,
12.));
#183212=CARTESIAN_POINT('Ctrl Pts',(5.09476976342625,-24.0779139079266,
12.));
#183213=CARTESIAN_POINT('Ctrl Pts',(5.10881967883132,-24.0975261288446,
12.));
#183214=CARTESIAN_POINT('Ctrl Pts',(5.12296753853859,-24.117173659394,12.));
#183215=CARTESIAN_POINT('Ctrl Pts',(5.13721325845744,-24.1368558702443,
12.));
#183216=CARTESIAN_POINT('Ctrl Pts',(5.15155675390075,-24.1565721375971,
12.));
#183217=CARTESIAN_POINT('Ctrl Pts',(5.16599793957979,-24.1763218431343,
12.));
#183218=CARTESIAN_POINT('Ctrl Pts',(5.18053672961392,-24.1961043738754,
12.));
#183219=CARTESIAN_POINT('Ctrl Pts',(5.19517303753642,-24.215919122017,12.));
#183220=CARTESIAN_POINT('Ctrl Pts',(5.20990677629173,-24.2357654847765,
12.));
#183221=CARTESIAN_POINT('Ctrl Pts',(5.22473785822441,-24.2556428642294,
12.));
#183222=CARTESIAN_POINT('Ctrl Pts',(5.23966619506289,-24.2755506671526,
12.));
#183223=CARTESIAN_POINT('Ctrl Pts',(5.25469169788855,-24.2954883048448,
12.));
#183224=CARTESIAN_POINT('Ctrl Pts',(5.26981427718796,-24.3154551932222,
12.));
#183225=CARTESIAN_POINT('Ctrl Pts',(5.28503384290644,-24.3354507529415,
12.));
#183226=CARTESIAN_POINT('Ctrl Pts',(5.30035030449058,-24.3554744095075,
12.));
#183227=CARTESIAN_POINT('Ctrl Pts',(5.31576357092524,-24.3755255933917,
12.));
#183228=CARTESIAN_POINT('Ctrl Pts',(5.33127355076036,-24.3956037401293,
12.));
#183229=CARTESIAN_POINT('Ctrl Pts',(5.34688015213546,-24.4157082904615,
12.));
#183230=CARTESIAN_POINT('Ctrl Pts',(5.36258328273639,-24.4358386899152,
12.));
#183231=CARTESIAN_POINT('Ctrl Pts',(5.37838284973706,-24.4559943883159,
12.));
#183232=CARTESIAN_POINT('Ctrl Pts',(5.3942787597383,-24.4761748393322,12.));
#183233=CARTESIAN_POINT('Ctrl Pts',(5.41027091869242,-24.4963794999831,
12.));
#183234=CARTESIAN_POINT('Ctrl Pts',(5.42635923183411,-24.5166078302107,
12.));
#183235=CARTESIAN_POINT('Ctrl Pts',(5.44254360356865,-24.5368592922861,
12.));
#183236=CARTESIAN_POINT('Ctrl Pts',(5.45882393762244,-24.5571333514841,
12.));
#183237=CARTESIAN_POINT('Ctrl Pts',(5.47520013724403,-24.5774294770329,
12.));
#183238=CARTESIAN_POINT('Ctrl Pts',(5.49167210537235,-24.5977471429365,
12.));
#183239=CARTESIAN_POINT('Ctrl Pts',(5.50823974481959,-24.618085828918,12.));
#183240=CARTESIAN_POINT('Ctrl Pts',(5.52490295840996,-24.6384450211466,
12.));
#183241=CARTESIAN_POINT('Ctrl Pts',(5.54166164919592,-24.6588242134733,
12.));
#183242=CARTESIAN_POINT('Ctrl Pts',(5.55851572025389,-24.6792229061785,
12.));
#183243=CARTESIAN_POINT('Ctrl Pts',(5.57546507427766,-24.6996406035507,
12.));
#183244=CARTESIAN_POINT('Ctrl Pts',(5.59250961323995,-24.7200768119079,
12.));
#183245=CARTESIAN_POINT('Ctrl Pts',(5.60964923798494,-24.7405310372736,
12.));
#183246=CARTESIAN_POINT('Ctrl Pts',(5.62688384790918,-24.76100278357,12.));
#183247=CARTESIAN_POINT('Ctrl Pts',(5.64421334042247,-24.7814915496728,
12.));
#183248=CARTESIAN_POINT('Ctrl Pts',(5.66163761114903,-24.8019968304618,
12.));
#183249=CARTESIAN_POINT('Ctrl Pts',(5.67915655496524,-24.822518122386,12.));
#183250=CARTESIAN_POINT('Ctrl Pts',(5.69677006679429,-24.8430549277634,
12.));
#183251=CARTESIAN_POINT('Ctrl Pts',(5.71447804252019,-24.8636067597677,
12.));
#183252=CARTESIAN_POINT('Ctrl Pts',(5.73228037976926,-24.8841731467219,
12.));
#183253=CARTESIAN_POINT('Ctrl Pts',(5.75017697890812,-24.9047536376467,
12.));
#183254=CARTESIAN_POINT('Ctrl Pts',(5.76816774342236,-24.9253478043632,
12.));
#183255=CARTESIAN_POINT('Ctrl Pts',(5.78625257775702,-24.9459552293308,
12.));
#183256=CARTESIAN_POINT('Ctrl Pts',(5.80443138549747,-24.9665754954463,
12.));
#183257=CARTESIAN_POINT('Ctrl Pts',(5.82270406744213,-24.9872081752709,
12.));
#183258=CARTESIAN_POINT('Ctrl Pts',(5.84107051963073,-25.0078528200558,
12.));
#183259=CARTESIAN_POINT('Ctrl Pts',(5.8595306315681,-25.0285089498922,12.));
#183260=CARTESIAN_POINT('Ctrl Pts',(5.87808428385329,-25.0491760405965,
12.));
#183261=CARTESIAN_POINT('Ctrl Pts',(5.89673135155458,-25.0698535426593,
12.));
#183262=CARTESIAN_POINT('Ctrl Pts',(5.91547170844382,-25.0905409050863,
12.));
#183263=CARTESIAN_POINT('Ctrl Pts',(5.93430523086776,-25.1112375971182,
12.));
#183264=CARTESIAN_POINT('Ctrl Pts',(5.95323180187347,-25.1319431317273,
12.));
#183265=CARTESIAN_POINT('Ctrl Pts',(5.97225131495636,-25.1526570863065,
12.));
#183266=CARTESIAN_POINT('Ctrl Pts',(5.99136367859838,-25.1733791296154,
12.));
#183267=CARTESIAN_POINT('Ctrl Pts',(6.0105688180476,-25.1941090269638,12.));
#183268=CARTESIAN_POINT('Ctrl Pts',(6.02986667390187,-25.2148466201368,
12.));
#183269=CARTESIAN_POINT('Ctrl Pts',(6.04925720151412,-25.2355918138798,
12.));
#183270=CARTESIAN_POINT('Ctrl Pts',(6.06484373634696,-25.2521940105523,
12.));
#183271=CARTESIAN_POINT('Ctrl Pts',(6.07657531787577,-25.2646490489816,
12.));
#183272=CARTESIAN_POINT('Ctrl Pts',(6.08441489609824,-25.2729539149479,
12.));
#183273=CARTESIAN_POINT('Ctrl Pts',(6.08833931617698,-25.2771067246846,
12.));
#183274=CARTESIAN_POINT('',(7.36589684767343,-24.9347862158358,12.));
#183275=CARTESIAN_POINT('Origin',(0.,0.,12.));
#183276=CARTESIAN_POINT('',(7.52250298901263,-21.2610617890679,12.));
#183277=CARTESIAN_POINT('Ctrl Pts',(7.36589684767343,-24.9347862158358,
12.));
#183278=CARTESIAN_POINT('Ctrl Pts',(7.36721909029059,-24.9292275670705,
12.));
#183279=CARTESIAN_POINT('Ctrl Pts',(7.36985593120695,-24.9181155530631,
12.));
#183280=CARTESIAN_POINT('Ctrl Pts',(7.37378825962717,-24.9014633826201,
12.));
#183281=CARTESIAN_POINT('Ctrl Pts',(7.37898549641609,-24.8792921911309,
12.));
#183282=CARTESIAN_POINT('Ctrl Pts',(7.38540558904945,-24.8516310625367,
12.));
#183283=CARTESIAN_POINT('Ctrl Pts',(7.3917492258684,-24.8240228521042,12.));
#183284=CARTESIAN_POINT('Ctrl Pts',(7.39801641583612,-24.7964676646518,
12.));
#183285=CARTESIAN_POINT('Ctrl Pts',(7.40420718661754,-24.7689656669005,
12.));
#183286=CARTESIAN_POINT('Ctrl Pts',(7.41032159082172,-24.7415170994754,
12.));
#183287=CARTESIAN_POINT('Ctrl Pts',(7.41635971481242,-24.7141222949988,
12.));
#183288=CARTESIAN_POINT('Ctrl Pts',(7.42232167765762,-24.6867816727118,
12.));
#183289=CARTESIAN_POINT('Ctrl Pts',(7.4282076215868,-24.659495712869,12.));
#183290=CARTESIAN_POINT('Ctrl Pts',(7.4340177048922,-24.6322649369472,12.));
#183291=CARTESIAN_POINT('Ctrl Pts',(7.43975209375374,-24.6050898852349,
12.));
#183292=CARTESIAN_POINT('Ctrl Pts',(7.44541095473162,-24.5779710960865,
12.));
#183293=CARTESIAN_POINT('Ctrl Pts',(7.45099444651295,-24.550909083158,12.));
#183294=CARTESIAN_POINT('Ctrl Pts',(7.45650271336044,-24.52390431731,12.));
#183295=CARTESIAN_POINT('Ctrl Pts',(7.46193588961641,-24.4969572391509,
12.));
#183296=CARTESIAN_POINT('Ctrl Pts',(7.46729410308922,-24.4700682684544,
12.));
#183297=CARTESIAN_POINT('Ctrl Pts',(7.47257747883318,-24.4432378146501,
12.));
#183298=CARTESIAN_POINT('Ctrl Pts',(7.47778614286572,-24.4164662871165,
12.));
#183299=CARTESIAN_POINT('Ctrl Pts',(7.48292022569253,-24.3897541049248,
12.));
#183300=CARTESIAN_POINT('Ctrl Pts',(7.48797986651827,-24.3631017084513,
12.));
#183301=CARTESIAN_POINT('Ctrl Pts',(7.49296521252329,-24.3365095573673,
12.));
#183302=CARTESIAN_POINT('Ctrl Pts',(7.49787641695358,-24.3099781253345,
12.));
#183303=CARTESIAN_POINT('Ctrl Pts',(7.50271363765098,-24.2835078958966,
12.));
#183304=CARTESIAN_POINT('Ctrl Pts',(7.50747703535114,-24.2570993577032,
12.));
#183305=CARTESIAN_POINT('Ctrl Pts',(7.51216677222198,-24.230753000389,12.));
#183306=CARTESIAN_POINT('Ctrl Pts',(7.51678300997997,-24.2044693092356,
12.));
#183307=CARTESIAN_POINT('Ctrl Pts',(7.52132590953862,-24.1782487641602,
12.));
#183308=CARTESIAN_POINT('Ctrl Pts',(7.52579563201478,-24.152091842537,12.));
#183309=CARTESIAN_POINT('Ctrl Pts',(7.53019233935536,-24.1259990209211,
12.));
#183310=CARTESIAN_POINT('Ctrl Pts',(7.53451619514658,-24.0999707772643,
12.));
#183311=CARTESIAN_POINT('Ctrl Pts',(7.53876736531004,-24.0740075927984,
12.));
#183312=CARTESIAN_POINT('Ctrl Pts',(7.54294601896127,-24.0481099543353,
12.));
#183313=CARTESIAN_POINT('Ctrl Pts',(7.54705232885894,-24.0222783554531,
12.));
#183314=CARTESIAN_POINT('Ctrl Pts',(7.55108647097431,-23.9965132953187,
12.));
#183315=CARTESIAN_POINT('Ctrl Pts',(7.55504862424807,-23.9708152779886,
12.));
#183316=CARTESIAN_POINT('Ctrl Pts',(7.55893897027679,-23.9451848115002,
12.));
#183317=CARTESIAN_POINT('Ctrl Pts',(7.56275769304772,-23.9196224070759,
12.));
#183318=CARTESIAN_POINT('Ctrl Pts',(7.5665049786379,-23.8941285782002,12.));
#183319=CARTESIAN_POINT('Ctrl Pts',(7.57018101500708,-23.8687038399595,
12.));
#183320=CARTESIAN_POINT('Ctrl Pts',(7.57378599219813,-23.8433487096132,
12.));
#183321=CARTESIAN_POINT('Ctrl Pts',(7.57732010249065,-23.8180637069976,
12.));
#183322=CARTESIAN_POINT('Ctrl Pts',(7.58078354058212,-23.7928493549908,
12.));
#183323=CARTESIAN_POINT('Ctrl Pts',(7.5841765037627,-23.7677061799376,12.));
#183324=CARTESIAN_POINT('Ctrl Pts',(7.58749919210825,-23.7426347121006,
12.));
#183325=CARTESIAN_POINT('Ctrl Pts',(7.5907518086532,-23.7176354860457,12.));
#183326=CARTESIAN_POINT('Ctrl Pts',(7.59393455934034,-23.6927090405066,
12.));
#183327=CARTESIAN_POINT('Ctrl Pts',(7.59704765299566,-23.6678559182875,
12.));
#183328=CARTESIAN_POINT('Ctrl Pts',(7.60009130130125,-23.6430766661418,
12.));
#183329=CARTESIAN_POINT('Ctrl Pts',(7.60306571877805,-23.6183718346576,
12.));
#183330=CARTESIAN_POINT('Ctrl Pts',(7.60597112277093,-23.5937419781245,
12.));
#183331=CARTESIAN_POINT('Ctrl Pts',(7.60880773344599,-23.5691876544244,
12.));
#183332=CARTESIAN_POINT('Ctrl Pts',(7.61157577385371,-23.544709425203,12.));
#183333=CARTESIAN_POINT('Ctrl Pts',(7.61427546999297,-23.5203078560129,
12.));
#183334=CARTESIAN_POINT('Ctrl Pts',(7.61690705088318,-23.4959835164609,
12.));
#183335=CARTESIAN_POINT('Ctrl Pts',(7.61947074863976,-23.4717369803438,
12.));
#183336=CARTESIAN_POINT('Ctrl Pts',(7.62196679855954,-23.4475688257854,
12.));
#183337=CARTESIAN_POINT('Ctrl Pts',(7.62439543920049,-23.4234796353542,
12.));
#183338=CARTESIAN_POINT('Ctrl Pts',(7.62675691240328,-23.399469996112,12.));
#183339=CARTESIAN_POINT('Ctrl Pts',(7.62905146332592,-23.3755404996636,
12.));
#183340=CARTESIAN_POINT('Ctrl Pts',(7.63127934048136,-23.3516917421972,
12.));
#183341=CARTESIAN_POINT('Ctrl Pts',(7.63344079578161,-23.3279243245241,
12.));
#183342=CARTESIAN_POINT('Ctrl Pts',(7.63553608458782,-23.3042388521022,
12.));
#183343=CARTESIAN_POINT('Ctrl Pts',(7.63756546576373,-23.2806359350855,
12.));
#183344=CARTESIAN_POINT('Ctrl Pts',(7.63952920172834,-23.2571161884488,
12.));
#183345=CARTESIAN_POINT('Ctrl Pts',(7.64142755851504,-23.2336802320912,
12.));
#183346=CARTESIAN_POINT('Ctrl Pts',(7.64326080583679,-23.2103286909398,
12.));
#183347=CARTESIAN_POINT('Ctrl Pts',(7.64502921715482,-23.1870621950452,
12.));
#183348=CARTESIAN_POINT('Ctrl Pts',(7.64673306975804,-23.1638813796694,
12.));
#183349=CARTESIAN_POINT('Ctrl Pts',(7.64837264482942,-23.1407868853819,
12.));
#183350=CARTESIAN_POINT('Ctrl Pts',(7.64994822749859,-23.1177793581679,
12.));
#183351=CARTESIAN_POINT('Ctrl Pts',(7.65146010690475,-23.094859449525,12.));
#183352=CARTESIAN_POINT('Ctrl Pts',(7.65290857626357,-23.072027816555,12.));
#183353=CARTESIAN_POINT('Ctrl Pts',(7.65429393293945,-23.0492851220528,
12.));
#183354=CARTESIAN_POINT('Ctrl Pts',(7.65561647852533,-23.0266320345787,
12.));
#183355=CARTESIAN_POINT('Ctrl Pts',(7.65687651891303,-23.0040692285814,
12.));
#183356=CARTESIAN_POINT('Ctrl Pts',(7.65807436436431,-22.9815973845296,
12.));
#183357=CARTESIAN_POINT('Ctrl Pts',(7.65921032958901,-22.959217189033,12.));
#183358=CARTESIAN_POINT('Ctrl Pts',(7.66028473382777,-22.9369293349593,
12.));
#183359=CARTESIAN_POINT('Ctrl Pts',(7.66129790094107,-22.9147345215421,
12.));
#183360=CARTESIAN_POINT('Ctrl Pts',(7.66225015950155,-22.8926334544883,
12.));
#183361=CARTESIAN_POINT('Ctrl Pts',(7.66314184287336,-22.8706268461283,
12.));
#183362=CARTESIAN_POINT('Ctrl Pts',(7.66397328929802,-22.848715415557,12.));
#183363=CARTESIAN_POINT('Ctrl Pts',(7.66474484198548,-22.8268998887678,
12.));
#183364=CARTESIAN_POINT('Ctrl Pts',(7.66545684920986,-22.8051809987833,
12.));
#183365=CARTESIAN_POINT('Ctrl Pts',(7.66610966441272,-22.7835594857699,
12.));
#183366=CARTESIAN_POINT('Ctrl Pts',(7.66670364630298,-22.7620360971843,
12.));
#183367=CARTESIAN_POINT('Ctrl Pts',(7.66723915895439,-22.7406115879513,
12.));
#183368=CARTESIAN_POINT('Ctrl Pts',(7.66771657191027,-22.7192867206245,
12.));
#183369=CARTESIAN_POINT('Ctrl Pts',(7.66813626029274,-22.6980622655446,
12.));
#183370=CARTESIAN_POINT('Ctrl Pts',(7.66849860491742,-22.6769390009885,
12.));
#183371=CARTESIAN_POINT('Ctrl Pts',(7.66880399241322,-22.6559177133127,
12.));
#183372=CARTESIAN_POINT('Ctrl Pts',(7.66905281533714,-22.6349991971541,
12.));
#183373=CARTESIAN_POINT('Ctrl Pts',(7.66924547229413,-22.6141842556243,
12.));
#183374=CARTESIAN_POINT('Ctrl Pts',(7.66938236806232,-22.5934737004953,
12.));
#183375=CARTESIAN_POINT('Ctrl Pts',(7.66946391372305,-22.5728683523831,
12.));
#183376=CARTESIAN_POINT('Ctrl Pts',(7.66949052679692,-22.5523690409116,
12.));
#183377=CARTESIAN_POINT('Ctrl Pts',(7.66946263138143,-22.53197660492,12.));
#183378=CARTESIAN_POINT('Ctrl Pts',(7.66938065829107,-22.5116918927032,
12.));
#183379=CARTESIAN_POINT('Ctrl Pts',(7.66924504520314,-22.4915157622312,
12.));
#183380=CARTESIAN_POINT('Ctrl Pts',(7.6690562368083,-22.47144908137,12.));
#183381=CARTESIAN_POINT('Ctrl Pts',(7.66881468496634,-22.4514927280855,
12.));
#183382=CARTESIAN_POINT('Ctrl Pts',(7.66852084886703,-22.4316475906603,
12.));
#183383=CARTESIAN_POINT('Ctrl Pts',(7.66817519519639,-22.4119145679758,
12.));
#183384=CARTESIAN_POINT('Ctrl Pts',(7.66777819830789,-22.3922945697773,
12.));
#183385=CARTESIAN_POINT('Ctrl Pts',(7.66733034039882,-22.372788516936,12.));
#183386=CARTESIAN_POINT('Ctrl Pts',(7.66683211169157,-22.3533973417021,
12.));
#183387=CARTESIAN_POINT('Ctrl Pts',(7.66628401061951,-22.3341219879469,
12.));
#183388=CARTESIAN_POINT('Ctrl Pts',(7.66568654402493,-22.314963411484,12.));
#183389=CARTESIAN_POINT('Ctrl Pts',(7.66504022736298,-22.2959225803937,
12.));
#183390=CARTESIAN_POINT('Ctrl Pts',(7.66434558490978,-22.2770004753335,
12.));
#183391=CARTESIAN_POINT('Ctrl Pts',(7.6636031499764,-22.258198089848,12.));
#183392=CARTESIAN_POINT('Ctrl Pts',(7.66281346512508,-22.2395164306547,
12.));
#183393=CARTESIAN_POINT('Ctrl Pts',(7.66197708240399,-22.2209565180085,
12.));
#183394=CARTESIAN_POINT('Ctrl Pts',(7.6610945635927,-22.2025193860964,12.));
#183395=CARTESIAN_POINT('Ctrl Pts',(7.66016648045004,-22.1842060834091,
12.));
#183396=CARTESIAN_POINT('Ctrl Pts',(7.6591934149693,-22.1660176731178,12.));
#183397=CARTESIAN_POINT('Ctrl Pts',(7.65817595963348,-22.1479552334211,
12.));
#183398=CARTESIAN_POINT('Ctrl Pts',(7.65711471769396,-22.1300198579675,
12.));
#183399=CARTESIAN_POINT('Ctrl Pts',(7.65601030346806,-22.1122126563329,
12.));
#183400=CARTESIAN_POINT('Ctrl Pts',(7.65486334263643,-22.094534754469,12.));
#183401=CARTESIAN_POINT('Ctrl Pts',(7.65367447254949,-22.0769872951596,
12.));
#183402=CARTESIAN_POINT('Ctrl Pts',(7.65244434253112,-22.0595714384431,
12.));
#183403=CARTESIAN_POINT('Ctrl Pts',(7.65117361421358,-22.0422883621174,
12.));
#183404=CARTESIAN_POINT('Ctrl Pts',(7.64986296190168,-22.0251392623209,
12.));
#183405=CARTESIAN_POINT('Ctrl Pts',(7.64851307293351,-22.0081253540774,
12.));
#183406=CARTESIAN_POINT('Ctrl Pts',(7.64712464805249,-21.9912478718542,
12.));
#183407=CARTESIAN_POINT('Ctrl Pts',(7.64569840177335,-21.9745080700798,
12.));
#183408=CARTESIAN_POINT('Ctrl Pts',(7.64423506279122,-21.9579072237651,
12.));
#183409=CARTESIAN_POINT('Ctrl Pts',(7.64273537442681,-21.9414466292072,
12.));
#183410=CARTESIAN_POINT('Ctrl Pts',(7.64120009506531,-21.9251276046546,
12.));
#183411=CARTESIAN_POINT('Ctrl Pts',(7.63962999860926,-21.9089514909874,
12.));
#183412=CARTESIAN_POINT('Ctrl Pts',(7.63802587492034,-21.8929196523514,
12.));
#183413=CARTESIAN_POINT('Ctrl Pts',(7.63638853033399,-21.8770334769496,
12.));
#183414=CARTESIAN_POINT('Ctrl Pts',(7.63471878821225,-21.8612943779089,
12.));
#183415=CARTESIAN_POINT('Ctrl Pts',(7.63301748948935,-21.8457037941084,
12.));
#183416=CARTESIAN_POINT('Ctrl Pts',(7.63128549323022,-21.8302631910195,
12.));
#183417=CARTESIAN_POINT('Ctrl Pts',(7.62952367718126,-21.814974061509,12.));
#183418=CARTESIAN_POINT('Ctrl Pts',(7.62773293842388,-21.799837926858,12.));
#183419=CARTESIAN_POINT('Ctrl Pts',(7.62591419404512,-21.7848563378021,
12.));
#183420=CARTESIAN_POINT('Ctrl Pts',(7.62406838181165,-21.7700308755584,
12.));
#183421=CARTESIAN_POINT('Ctrl Pts',(7.62219646084228,-21.7553631528328,
12.));
#183422=CARTESIAN_POINT('Ctrl Pts',(7.62029941230854,-21.7408548148656,
12.));
#183423=CARTESIAN_POINT('Ctrl Pts',(7.61837824030537,-21.7265075407975,
12.));
#183424=CARTESIAN_POINT('Ctrl Pts',(7.6164339727042,-21.7123230449834,12.));
#183425=CARTESIAN_POINT('Ctrl Pts',(7.61446766202786,-21.6983030783322,
12.));
#183426=CARTESIAN_POINT('Ctrl Pts',(7.61248038630268,-21.6844494295815,
12.));
#183427=CARTESIAN_POINT('Ctrl Pts',(7.61047325000955,-21.6707639267576,
12.));
#183428=CARTESIAN_POINT('Ctrl Pts',(7.60844738512873,-21.6572484388081,
12.));
#183429=CARTESIAN_POINT('Ctrl Pts',(7.60640395216356,-21.6439048771743,
12.));
#183430=CARTESIAN_POINT('Ctrl Pts',(7.60434414118295,-21.6307351973822,
12.));
#183431=CARTESIAN_POINT('Ctrl Pts',(7.60226917285428,-21.617741400599,12.));
#183432=CARTESIAN_POINT('Ctrl Pts',(7.6001802998824,-21.6049255358843,12.));
#183433=CARTESIAN_POINT('Ctrl Pts',(7.59807880846194,-21.5922897024466,
12.));
#183434=CARTESIAN_POINT('Ctrl Pts',(7.59596601973583,-21.5798360518978,
12.));
#183435=CARTESIAN_POINT('Ctrl Pts',(7.59384329124918,-21.5675667904726,
12.));
#183436=CARTESIAN_POINT('Ctrl Pts',(7.59171201844776,-21.5554841813462,
12.));
#183437=CARTESIAN_POINT('Ctrl Pts',(7.58957363620013,-21.543590547011,12.));
#183438=CARTESIAN_POINT('Ctrl Pts',(7.58742962034833,-21.5318882716736,
12.));
#183439=CARTESIAN_POINT('Ctrl Pts',(7.58528148919129,-21.5203798035299,
12.));
#183440=CARTESIAN_POINT('Ctrl Pts',(7.58313080519179,-21.5090676573873,
12.));
#183441=CARTESIAN_POINT('Ctrl Pts',(7.58097917790743,-21.4979544192744,
12.));
#183442=CARTESIAN_POINT('Ctrl Pts',(7.57882826679131,-21.4870427508194,
12.));
#183443=CARTESIAN_POINT('Ctrl Pts',(7.57667978402986,-21.4763353936762,
12.));
#183444=CARTESIAN_POINT('Ctrl Pts',(7.57453549743411,-21.4658351740128,
12.));
#183445=CARTESIAN_POINT('Ctrl Pts',(7.57239723223505,-21.4555450053142,
12.));
#183446=CARTESIAN_POINT('Ctrl Pts',(7.57026687261165,-21.4454678907509,
12.));
#183447=CARTESIAN_POINT('Ctrl Pts',(7.56814636360847,-21.4356069261513,
12.));
#183448=CARTESIAN_POINT('Ctrl Pts',(7.56603771218711,-21.4259653015736,
12.));
#183449=CARTESIAN_POINT('Ctrl Pts',(7.56394299313684,-21.4165463106254,
12.));
#183450=CARTESIAN_POINT('Ctrl Pts',(7.56186435703621,-21.4073533630365,
12.));
#183451=CARTESIAN_POINT('Ctrl Pts',(7.5598040370061,-21.3983899952987,12.));
#183452=CARTESIAN_POINT('Ctrl Pts',(7.55776435731416,-21.3896598842117,
12.));
#183453=CARTESIAN_POINT('Ctrl Pts',(7.55574773403502,-21.3811668478932,
12.));
#183454=CARTESIAN_POINT('Ctrl Pts',(7.55375667080028,-21.3729148390243,
12.));
#183455=CARTESIAN_POINT('Ctrl Pts',(7.55179375777443,-21.3649079431865,
12.));
#183456=CARTESIAN_POINT('Ctrl Pts',(7.54986166521309,-21.3571503685855,
12.));
#183457=CARTESIAN_POINT('Ctrl Pts',(7.5479631624633,-21.3496464761531,12.));
#183458=CARTESIAN_POINT('Ctrl Pts',(7.54610114948346,-21.3424008295038,
12.));
#183459=CARTESIAN_POINT('Ctrl Pts',(7.54427868151267,-21.3354182340149,
12.));
#183460=CARTESIAN_POINT('Ctrl Pts',(7.5424990037703,-21.328703791771,12.));
#183461=CARTESIAN_POINT('Ctrl Pts',(7.54076552038278,-21.3222628524165,
12.));
#183462=CARTESIAN_POINT('Ctrl Pts',(7.53908175169898,-21.3161009456256,
12.));
#183463=CARTESIAN_POINT('Ctrl Pts',(7.53745129364615,-21.310223716773,12.));
#183464=CARTESIAN_POINT('Ctrl Pts',(7.53587778251735,-21.3046368712157,
12.));
#183465=CARTESIAN_POINT('Ctrl Pts',(7.53436505309942,-21.2993464250717,
12.));
#183466=CARTESIAN_POINT('Ctrl Pts',(7.53291726078526,-21.2943588989331,
12.));
#183467=CARTESIAN_POINT('Ctrl Pts',(7.53153906987855,-21.2896816163842,
12.));
#183468=CARTESIAN_POINT('Ctrl Pts',(7.53023562438229,-21.2853226580657,
12.));
#183469=CARTESIAN_POINT('Ctrl Pts',(7.52901217930407,-21.2812902781143,
12.));
#183470=CARTESIAN_POINT('Ctrl Pts',(7.52787386225332,-21.2775925269652,
12.));
#183471=CARTESIAN_POINT('Ctrl Pts',(7.5268252691854,-21.2742366113579,12.));
#183472=CARTESIAN_POINT('Ctrl Pts',(7.52587126095529,-21.2712301573466,
12.));
#183473=CARTESIAN_POINT('Ctrl Pts',(7.5250177033353,-21.2685823838671,12.));
#183474=CARTESIAN_POINT('Ctrl Pts',(7.52427261074297,-21.2663059157058,
12.));
#183475=CARTESIAN_POINT('Ctrl Pts',(7.52364573027552,-21.2644161259962,
12.));
#183476=CARTESIAN_POINT('Ctrl Pts',(7.52314642316199,-21.262927782038,12.));
#183477=CARTESIAN_POINT('Ctrl Pts',(7.52278182242669,-21.2618521283555,
12.));
#183478=CARTESIAN_POINT('Ctrl Pts',(7.5226006423166,-21.261326054066,12.));
#183479=CARTESIAN_POINT('Ctrl Pts',(7.52252744144903,-21.2611204474866,
12.));
#183480=CARTESIAN_POINT('Ctrl Pts',(7.52250649703969,-21.2610673466886,
12.));
#183481=CARTESIAN_POINT('Ctrl Pts',(7.52250298901263,-21.2610617890679,
12.));
#183482=CARTESIAN_POINT('',(7.33627833380045,-20.7347298079577,12.));
#183483=CARTESIAN_POINT('',(3.58569854577611,-10.1343606576251,12.));
#183484=CARTESIAN_POINT('',(7.63019749246977,-20.1004996511507,12.));
#183485=CARTESIAN_POINT('Origin',(7.80764394578302,-20.56795313141,12.));
#183486=CARTESIAN_POINT('',(8.81783521984849,-19.6085639972844,12.));
#183487=CARTESIAN_POINT('Origin',(2.70312158620511E-13,-7.32141292029404E-13,
12.));
#183488=CARTESIAN_POINT('',(9.47413589477548,-19.84920021178,12.));
#183489=CARTESIAN_POINT('Origin',(9.02290115519381,-20.0645771135004,12.));
#183490=CARTESIAN_POINT('',(9.71462809124915,-20.353053841303,12.));
#183491=CARTESIAN_POINT('',(4.85731404562459,-10.1765269206515,12.));
#183492=CARTESIAN_POINT('',(12.4230808101438,-22.8400320311649,12.));
#183493=CARTESIAN_POINT('Ctrl Pts',(9.71462809124915,-20.353053841303,12.));
#183494=CARTESIAN_POINT('Ctrl Pts',(9.71462954053041,-20.353060251684,12.));
#183495=CARTESIAN_POINT('Ctrl Pts',(9.71465227853041,-20.3531126095522,
12.));
#183496=CARTESIAN_POINT('Ctrl Pts',(9.7147459035068,-20.3533097561886,12.));
#183497=CARTESIAN_POINT('Ctrl Pts',(9.7149897805202,-20.3538098605706,12.));
#183498=CARTESIAN_POINT('Ctrl Pts',(9.71549257088172,-20.3548282742361,
12.));
#183499=CARTESIAN_POINT('Ctrl Pts',(9.71619192554185,-20.3562337557875,
12.));
#183500=CARTESIAN_POINT('Ctrl Pts',(9.71708493723096,-20.3580133103356,
12.));
#183501=CARTESIAN_POINT('Ctrl Pts',(9.71816778328006,-20.3601498764344,
12.));
#183502=CARTESIAN_POINT('Ctrl Pts',(9.71943648548099,-20.3626256913981,
12.));
#183503=CARTESIAN_POINT('Ctrl Pts',(9.7208877838108,-20.3654261611056,12.));
#183504=CARTESIAN_POINT('Ctrl Pts',(9.72251930722489,-20.3685406190576,
12.));
#183505=CARTESIAN_POINT('Ctrl Pts',(9.72432910043194,-20.371960235676,12.));
#183506=CARTESIAN_POINT('Ctrl Pts',(9.7263153173288,-20.3756766651951,12.));
#183507=CARTESIAN_POINT('Ctrl Pts',(9.72847589116541,-20.3796805893304,
12.));
#183508=CARTESIAN_POINT('Ctrl Pts',(9.73080870123726,-20.3839624556742,
12.));
#183509=CARTESIAN_POINT('Ctrl Pts',(9.73331167102807,-20.3885129129912,
12.));
#183510=CARTESIAN_POINT('Ctrl Pts',(9.73598292014242,-20.3933234845647,
12.));
#183511=CARTESIAN_POINT('Ctrl Pts',(9.738820776132,-20.3983866213331,12.));
#183512=CARTESIAN_POINT('Ctrl Pts',(9.74182369656271,-20.4036953576549,
12.));
#183513=CARTESIAN_POINT('Ctrl Pts',(9.74499021838537,-20.4092430879861,
12.));
#183514=CARTESIAN_POINT('Ctrl Pts',(9.74831889242173,-20.4150232777393,
12.));
#183515=CARTESIAN_POINT('Ctrl Pts',(9.75180829786429,-20.4210295275817,
12.));
#183516=CARTESIAN_POINT('Ctrl Pts',(9.75545705902417,-20.4272556476629,
12.));
#183517=CARTESIAN_POINT('Ctrl Pts',(9.75926386289922,-20.4336957355473,
12.));
#183518=CARTESIAN_POINT('Ctrl Pts',(9.76322747195494,-20.44034423294,12.));
#183519=CARTESIAN_POINT('Ctrl Pts',(9.76734670980891,-20.447195862298,12.));
#183520=CARTESIAN_POINT('Ctrl Pts',(9.77162045104069,-20.4542455817527,
12.));
#183521=CARTESIAN_POINT('Ctrl Pts',(9.77604760815528,-20.4614885274975,
12.));
#183522=CARTESIAN_POINT('Ctrl Pts',(9.7806271237332,-20.4689199790669,12.));
#183523=CARTESIAN_POINT('Ctrl Pts',(9.78535797314166,-20.4765353711586,
12.));
#183524=CARTESIAN_POINT('Ctrl Pts',(9.79023916498655,-20.4843302955329,
12.));
#183525=CARTESIAN_POINT('Ctrl Pts',(9.7952697428833,-20.4923005087943,12.));
#183526=CARTESIAN_POINT('Ctrl Pts',(9.80044878520948,-20.5004419312107,
12.));
#183527=CARTESIAN_POINT('Ctrl Pts',(9.80577540161087,-20.5087506310505,
12.));
#183528=CARTESIAN_POINT('Ctrl Pts',(9.81124873025281,-20.517222812284,12.));
#183529=CARTESIAN_POINT('Ctrl Pts',(9.81686793455942,-20.5258548000629,
12.));
#183530=CARTESIAN_POINT('Ctrl Pts',(9.82263220080362,-20.5346430299517,
12.));
#183531=CARTESIAN_POINT('Ctrl Pts',(9.82854073773876,-20.5435840460721,
12.));
#183532=CARTESIAN_POINT('Ctrl Pts',(9.83459277585315,-20.552674497646,12.));
#183533=CARTESIAN_POINT('Ctrl Pts',(9.84078756677565,-20.5619111362402,
12.));
#183534=CARTESIAN_POINT('Ctrl Pts',(9.84712438256277,-20.5712908125139,
12.));
#183535=CARTESIAN_POINT('Ctrl Pts',(9.8536025145698,-20.5808104710015,12.));
#183536=CARTESIAN_POINT('Ctrl Pts',(9.86022127232747,-20.5904671449754,
12.));
#183537=CARTESIAN_POINT('Ctrl Pts',(9.86697998242622,-20.6002579513699,
12.));
#183538=CARTESIAN_POINT('Ctrl Pts',(9.87387798732955,-20.6101800854494,
12.));
#183539=CARTESIAN_POINT('Ctrl Pts',(9.88091464472675,-20.6202308177475,
12.));
#183540=CARTESIAN_POINT('Ctrl Pts',(9.88808932697305,-20.6304074914087,
12.));
#183541=CARTESIAN_POINT('Ctrl Pts',(9.89540142049119,-20.6407075193976,
12.));
#183542=CARTESIAN_POINT('Ctrl Pts',(9.90285032516692,-20.6511283817414,
12.));
#183543=CARTESIAN_POINT('Ctrl Pts',(9.91043545377007,-20.6616676228315,
12.));
#183544=CARTESIAN_POINT('Ctrl Pts',(9.91815623141288,-20.6723228488263,
12.));
#183545=CARTESIAN_POINT('Ctrl Pts',(9.92601209498748,-20.6830917250255,
12.));
#183546=CARTESIAN_POINT('Ctrl Pts',(9.93400249259729,-20.6939719732484,
12.));
#183547=CARTESIAN_POINT('Ctrl Pts',(9.94212688298236,-20.7049613692234,
12.));
#183548=CARTESIAN_POINT('Ctrl Pts',(9.95038473514948,-20.7160577407579,
12.));
#183549=CARTESIAN_POINT('Ctrl Pts',(9.95877552798397,-20.7272589658751,
12.));
#183550=CARTESIAN_POINT('Ctrl Pts',(9.96729874986201,-20.7385629709795,
12.));
#183551=CARTESIAN_POINT('Ctrl Pts',(9.97595389823469,-20.7499677289627,
12.));
#183552=CARTESIAN_POINT('Ctrl Pts',(9.98474047926852,-20.761471257499,12.));
#183553=CARTESIAN_POINT('Ctrl Pts',(9.9936580075464,-20.7730716175417,12.));
#183554=CARTESIAN_POINT('Ctrl Pts',(10.0027060057389,-20.7847669117568,
12.));
#183555=CARTESIAN_POINT('Ctrl Pts',(10.0118840042786,-20.7965552829908,
12.));
#183556=CARTESIAN_POINT('Ctrl Pts',(10.0211915410095,-20.8084349126888,
12.));
#183557=CARTESIAN_POINT('Ctrl Pts',(10.0306281609435,-20.8204040196602,
12.));
#183558=CARTESIAN_POINT('Ctrl Pts',(10.0401934160234,-20.8324608588909,
12.));
#183559=CARTESIAN_POINT('Ctrl Pts',(10.0498868648733,-20.8446037203402,
12.));
#183560=CARTESIAN_POINT('Ctrl Pts',(10.0597080725375,-20.8568309277316,
12.));
#183561=CARTESIAN_POINT('Ctrl Pts',(10.0696566102218,-20.86914083737,12.));
#183562=CARTESIAN_POINT('Ctrl Pts',(10.0797320551154,-20.881531837184,12.));
#183563=CARTESIAN_POINT('Ctrl Pts',(10.0899339901915,-20.894002345737,12.));
#183564=CARTESIAN_POINT('Ctrl Pts',(10.1002620040076,-20.9065508112557,
12.));
#183565=CARTESIAN_POINT('Ctrl Pts',(10.1107156904836,-20.919175710627,12.));
#183566=CARTESIAN_POINT('Ctrl Pts',(10.1212946487057,-20.9318755484734,
12.));
#183567=CARTESIAN_POINT('Ctrl Pts',(10.1319984827908,-20.9446488563933,
12.));
#183568=CARTESIAN_POINT('Ctrl Pts',(10.1428268017256,-20.9574941921591,
12.));
#183569=CARTESIAN_POINT('Ctrl Pts',(10.1537792192065,-20.9704101389369,
12.));
#183570=CARTESIAN_POINT('Ctrl Pts',(10.1648553534568,-20.9833953044736,
12.));
#183571=CARTESIAN_POINT('Ctrl Pts',(10.1760548270767,-20.9964483203686,
12.));
#183572=CARTESIAN_POINT('Ctrl Pts',(10.187377266936,-21.0095678414486,12.));
#183573=CARTESIAN_POINT('Ctrl Pts',(10.1988223040425,-21.0227525451107,
12.));
#183574=CARTESIAN_POINT('Ctrl Pts',(10.2103895734123,-21.0360011306815,
12.));
#183575=CARTESIAN_POINT('Ctrl Pts',(10.2220787139154,-21.0493123187483,
12.));
#183576=CARTESIAN_POINT('Ctrl Pts',(10.2338893681567,-21.0626848505663,
12.));
#183577=CARTESIAN_POINT('Ctrl Pts',(10.2458211823912,-21.0761174875445,
12.));
#183578=CARTESIAN_POINT('Ctrl Pts',(10.2578738064181,-21.0896090107063,
12.));
#183579=CARTESIAN_POINT('Ctrl Pts',(10.2700468934744,-21.1031582201627,
12.));
#183580=CARTESIAN_POINT('Ctrl Pts',(10.2823401001072,-21.1167639345631,
12.));
#183581=CARTESIAN_POINT('Ctrl Pts',(10.2947530860721,-21.1304249906002,
12.));
#183582=CARTESIAN_POINT('Ctrl Pts',(10.3072855142687,-21.1441402425843,
12.));
#183583=CARTESIAN_POINT('Ctrl Pts',(10.3199370506544,-21.1579085619965,
12.));
#183584=CARTESIAN_POINT('Ctrl Pts',(10.3327073641572,-21.1717288370509,
12.));
#183585=CARTESIAN_POINT('Ctrl Pts',(10.34559612657,-21.1855999722416,12.));
#183586=CARTESIAN_POINT('Ctrl Pts',(10.3586030124587,-21.199520887919,12.));
#183587=CARTESIAN_POINT('Ctrl Pts',(10.371727699113,-21.2134905199345,12.));
#183588=CARTESIAN_POINT('Ctrl Pts',(10.3849698664786,-21.22750781927,12.));
#183589=CARTESIAN_POINT('Ctrl Pts',(10.3983291970846,-21.2415717516714,
12.));
#183590=CARTESIAN_POINT('Ctrl Pts',(10.4118053759588,-21.255681297275,12.));
#183591=CARTESIAN_POINT('Ctrl Pts',(10.42539809054,-21.2698354502403,12.));
#183592=CARTESIAN_POINT('Ctrl Pts',(10.4391070306391,-21.2840332184483,
12.));
#183593=CARTESIAN_POINT('Ctrl Pts',(10.4529318883874,-21.2982736231931,
12.));
#183594=CARTESIAN_POINT('Ctrl Pts',(10.4668723581768,-21.3125556988731,
12.));
#183595=CARTESIAN_POINT('Ctrl Pts',(10.4809281365931,-21.3268784926819,
12.));
#183596=CARTESIAN_POINT('Ctrl Pts',(10.4950989223336,-21.3412410642904,
12.));
#183597=CARTESIAN_POINT('Ctrl Pts',(10.5093844161685,-21.3556424855814,
12.));
#183598=CARTESIAN_POINT('Ctrl Pts',(10.5237843209057,-21.3700818403936,
12.));
#183599=CARTESIAN_POINT('Ctrl Pts',(10.5382983413421,-21.3845582242602,
12.));
#183600=CARTESIAN_POINT('Ctrl Pts',(10.5529261842108,-21.3990707441497,
12.));
#183601=CARTESIAN_POINT('Ctrl Pts',(10.5676675581108,-21.4136185181979,
12.));
#183602=CARTESIAN_POINT('Ctrl Pts',(10.5825221734573,-21.4282006754631,
12.));
#183603=CARTESIAN_POINT('Ctrl Pts',(10.5974897424622,-21.4428163557144,
12.));
#183604=CARTESIAN_POINT('Ctrl Pts',(10.6125699790961,-21.4574647092097,
12.));
#183605=CARTESIAN_POINT('Ctrl Pts',(10.6277625990456,-21.4721448964766,
12.));
#183606=CARTESIAN_POINT('Ctrl Pts',(10.6430673196607,-21.4868560880889,
12.));
#183607=CARTESIAN_POINT('Ctrl Pts',(10.6584838598939,-21.5015974644449,
12.));
#183608=CARTESIAN_POINT('Ctrl Pts',(10.6740119402834,-21.51636821558,12.));
#183609=CARTESIAN_POINT('Ctrl Pts',(10.689651282929,-21.5311675409807,12.));
#183610=CARTESIAN_POINT('Ctrl Pts',(10.7054016114571,-21.5459946493955,
12.));
#183611=CARTESIAN_POINT('Ctrl Pts',(10.7212626509816,-21.5608487586468,
12.));
#183612=CARTESIAN_POINT('Ctrl Pts',(10.7372341280467,-21.5757290954371,
12.));
#183613=CARTESIAN_POINT('Ctrl Pts',(10.7533157705941,-21.5906348951743,
12.));
#183614=CARTESIAN_POINT('Ctrl Pts',(10.7695073079552,-21.6055654018176,
12.));
#183615=CARTESIAN_POINT('Ctrl Pts',(10.7858084708261,-21.6205198677173,
12.));
#183616=CARTESIAN_POINT('Ctrl Pts',(10.8022189912369,-21.6354975534557,
12.));
#183617=CARTESIAN_POINT('Ctrl Pts',(10.8187386025136,-21.6504977276866,
12.));
#183618=CARTESIAN_POINT('Ctrl Pts',(10.8353670392272,-21.6655196669732,
12.));
#183619=CARTESIAN_POINT('Ctrl Pts',(10.8521040371835,-21.6805626556467,
12.));
#183620=CARTESIAN_POINT('Ctrl Pts',(10.8689493334095,-21.6956259856672,
12.));
#183621=CARTESIAN_POINT('Ctrl Pts',(10.8859026661293,-21.7107089564825,
12.));
#183622=CARTESIAN_POINT('Ctrl Pts',(10.902963774734,-21.7258108748873,12.));
#183623=CARTESIAN_POINT('Ctrl Pts',(10.9201323997384,-21.7409310548797,
12.));
#183624=CARTESIAN_POINT('Ctrl Pts',(10.9374082827444,-21.7560688175247,
12.));
#183625=CARTESIAN_POINT('Ctrl Pts',(10.9547911664455,-21.7712234908464,
12.));
#183626=CARTESIAN_POINT('Ctrl Pts',(10.9722807946155,-21.7863944097141,
12.));
#183627=CARTESIAN_POINT('Ctrl Pts',(10.9898769120912,-21.8015809157301,
12.));
#183628=CARTESIAN_POINT('Ctrl Pts',(11.0075792647477,-21.8167823571168,
12.));
#183629=CARTESIAN_POINT('Ctrl Pts',(11.0253875994598,-21.8319980886033,
12.));
#183630=CARTESIAN_POINT('Ctrl Pts',(11.0433016640807,-21.8472274713103,
12.));
#183631=CARTESIAN_POINT('Ctrl Pts',(11.0613212074363,-21.8624698726318,
12.));
#183632=CARTESIAN_POINT('Ctrl Pts',(11.0794459793057,-21.877724666119,12.));
#183633=CARTESIAN_POINT('Ctrl Pts',(11.0976757303944,-21.8929912313608,
12.));
#183634=CARTESIAN_POINT('Ctrl Pts',(11.1160102123024,-21.9082689538688,
12.));
#183635=CARTESIAN_POINT('Ctrl Pts',(11.1344491774741,-21.923557224952,12.));
#183636=CARTESIAN_POINT('Ctrl Pts',(11.1529923792003,-21.9388554416439,
12.));
#183637=CARTESIAN_POINT('Ctrl Pts',(11.1716395716376,-21.9541630066506,
12.));
#183638=CARTESIAN_POINT('Ctrl Pts',(11.190390509811,-21.9694793282914,12.));
#183639=CARTESIAN_POINT('Ctrl Pts',(11.2092449496125,-21.9848038204439,
12.));
#183640=CARTESIAN_POINT('Ctrl Pts',(11.2282026477896,-22.0001359024839,
12.));
#183641=CARTESIAN_POINT('Ctrl Pts',(11.2472633619275,-22.0154749992363,
12.));
#183642=CARTESIAN_POINT('Ctrl Pts',(11.2664268504206,-22.030820540835,12.));
#183643=CARTESIAN_POINT('Ctrl Pts',(11.2856928724374,-22.046171962566,12.));
#183644=CARTESIAN_POINT('Ctrl Pts',(11.3050611878771,-22.0615287047179,
12.));
#183645=CARTESIAN_POINT('Ctrl Pts',(11.3245315573168,-22.0768902124267,
12.));
#183646=CARTESIAN_POINT('Ctrl Pts',(11.3441037419553,-22.0922559355294,
12.));
#183647=CARTESIAN_POINT('Ctrl Pts',(11.3637775035367,-22.1076253283979,
12.));
#183648=CARTESIAN_POINT('Ctrl Pts',(11.3835526044256,-22.1229978500186,
12.));
#183649=CARTESIAN_POINT('Ctrl Pts',(11.4034288076908,-22.1383729640964,
12.));
#183650=CARTESIAN_POINT('Ctrl Pts',(11.4234058771742,-22.1537501391487,
12.));
#183651=CARTESIAN_POINT('Ctrl Pts',(11.443483577557,-22.1691288486096,12.));
#183652=CARTESIAN_POINT('Ctrl Pts',(11.463661674411,-22.184508570917,12.));
#183653=CARTESIAN_POINT('Ctrl Pts',(11.483939934259,-22.1998887896436,12.));
#183654=CARTESIAN_POINT('Ctrl Pts',(11.5043181244242,-22.2152689931022,
12.));
#183655=CARTESIAN_POINT('Ctrl Pts',(11.5247960128477,-22.2306486738901,
12.));
#183656=CARTESIAN_POINT('Ctrl Pts',(11.5453733679121,-22.2460273284654,
12.));
#183657=CARTESIAN_POINT('Ctrl Pts',(11.5660499582403,-22.2614044566898,
12.));
#183658=CARTESIAN_POINT('Ctrl Pts',(11.5868255525188,-22.2767795614348,
12.));
#183659=CARTESIAN_POINT('Ctrl Pts',(11.6076999192357,-22.2921521480356,
12.));
#183660=CARTESIAN_POINT('Ctrl Pts',(11.6286728270009,-22.3075217249049,
12.));
#183661=CARTESIAN_POINT('Ctrl Pts',(11.6497440449857,-22.3228878043976,
12.));
#183662=CARTESIAN_POINT('Ctrl Pts',(11.6709133432985,-22.3382499035619,
12.));
#183663=CARTESIAN_POINT('Ctrl Pts',(11.6921804934056,-22.3536075450029,
12.));
#183664=CARTESIAN_POINT('Ctrl Pts',(11.7135452684532,-22.3689602575491,
12.));
#183665=CARTESIAN_POINT('Ctrl Pts',(11.7350074437961,-22.3843075773899,
12.));
#183666=CARTESIAN_POINT('Ctrl Pts',(11.7565667964764,-22.3996490469191,
12.));
#183667=CARTESIAN_POINT('Ctrl Pts',(11.7782231042039,-22.4149842125008,
12.));
#183668=CARTESIAN_POINT('Ctrl Pts',(11.7999761445173,-22.430312622646,12.));
#183669=CARTESIAN_POINT('Ctrl Pts',(11.8218256937889,-22.4456338258735,
12.));
#183670=CARTESIAN_POINT('Ctrl Pts',(11.8437715264487,-22.4609473690472,
12.));
#183671=CARTESIAN_POINT('Ctrl Pts',(11.8658134137019,-22.4762527946702,
12.));
#183672=CARTESIAN_POINT('Ctrl Pts',(11.8879511239942,-22.4915496418485,
12.));
#183673=CARTESIAN_POINT('Ctrl Pts',(11.9101844254557,-22.5068374513973,
12.));
#183674=CARTESIAN_POINT('Ctrl Pts',(11.9325130877803,-22.5221157697883,
12.));
#183675=CARTESIAN_POINT('Ctrl Pts',(11.9549368843997,-22.5373841537307,
12.));
#183676=CARTESIAN_POINT('Ctrl Pts',(11.9774555943496,-22.5526421741158,
12.));
#183677=CARTESIAN_POINT('Ctrl Pts',(12.0000690046694,-22.5678894211181,
12.));
#183678=CARTESIAN_POINT('Ctrl Pts',(12.0227769113127,-22.5831255061282,
12.));
#183679=CARTESIAN_POINT('Ctrl Pts',(12.0455791139128,-22.5983500505644,
12.));
#183680=CARTESIAN_POINT('Ctrl Pts',(12.0684754113862,-22.6135626764898,
12.));
#183681=CARTESIAN_POINT('Ctrl Pts',(12.0914655972823,-22.6287629967056,
12.));
#183682=CARTESIAN_POINT('Ctrl Pts',(12.1145494550383,-22.6439506046605,
12.));
#183683=CARTESIAN_POINT('Ctrl Pts',(12.1377267537145,-22.6591250653965,
12.));
#183684=CARTESIAN_POINT('Ctrl Pts',(12.1609972423099,-22.6742859034944,
12.));
#183685=CARTESIAN_POINT('Ctrl Pts',(12.1843606579261,-22.6894326205037,
12.));
#183686=CARTESIAN_POINT('Ctrl Pts',(12.2078167360284,-22.7045647168747,
12.));
#183687=CARTESIAN_POINT('Ctrl Pts',(12.2313652198061,-22.7196817119374,
12.));
#183688=CARTESIAN_POINT('Ctrl Pts',(12.2550058702395,-22.7347831655287,
12.));
#183689=CARTESIAN_POINT('Ctrl Pts',(12.2787384750742,-22.7498686970069,
12.));
#183690=CARTESIAN_POINT('Ctrl Pts',(12.3025628601792,-22.764938010105,12.));
#183691=CARTESIAN_POINT('Ctrl Pts',(12.3264788926075,-22.7799908974768,
12.));
#183692=CARTESIAN_POINT('Ctrl Pts',(12.3504864740319,-22.795027221673,12.));
#183693=CARTESIAN_POINT('Ctrl Pts',(12.374585536673,-22.81004690224,12.));
#183694=CARTESIAN_POINT('Ctrl Pts',(12.3939379378998,-22.8220493007173,
12.));
#183695=CARTESIAN_POINT('Ctrl Pts',(12.4084933766346,-22.8310435872748,
12.));
#183696=CARTESIAN_POINT('Ctrl Pts',(12.418215285186,-22.8370364396459,12.));
#183697=CARTESIAN_POINT('Ctrl Pts',(12.4230808101438,-22.8400320311649,
12.));
#183698=CARTESIAN_POINT('',(13.5685075571671,-22.178719590434,12.));
#183699=CARTESIAN_POINT('Origin',(0.,0.,12.));
#183700=CARTESIAN_POINT('',(12.7689476255362,-18.5896416359912,12.));
#183701=CARTESIAN_POINT('Ctrl Pts',(13.5685075571671,-22.178719590434,12.));
#183702=CARTESIAN_POINT('Ctrl Pts',(13.5683460612942,-22.1730081264608,
12.));
#183703=CARTESIAN_POINT('Ctrl Pts',(13.5680170531805,-22.1615922805008,
12.));
#183704=CARTESIAN_POINT('Ctrl Pts',(13.5675054919061,-22.1444897575194,
12.));
#183705=CARTESIAN_POINT('Ctrl Pts',(13.5667873105359,-22.1217288871975,
12.));
#183706=CARTESIAN_POINT('Ctrl Pts',(13.5658294169284,-22.0933486464593,
12.));
#183707=CARTESIAN_POINT('Ctrl Pts',(13.5648113689033,-22.065039308961,12.));
#183708=CARTESIAN_POINT('Ctrl Pts',(13.5637332022473,-22.0368009736295,
12.));
#183709=CARTESIAN_POINT('Ctrl Pts',(13.5625949868333,-22.0086337943449,
12.));
#183710=CARTESIAN_POINT('Ctrl Pts',(13.5613968357561,-21.9805379899168,
12.));
#183711=CARTESIAN_POINT('Ctrl Pts',(13.5601389185257,-21.9525138592813,
12.));
#183712=CARTESIAN_POINT('Ctrl Pts',(13.5588214586604,-21.9245617765769,
12.));
#183713=CARTESIAN_POINT('Ctrl Pts',(13.5574447178424,-21.8966821688824,
12.));
#183714=CARTESIAN_POINT('Ctrl Pts',(13.5560089839385,-21.8688754989365,
12.));
#183715=CARTESIAN_POINT('Ctrl Pts',(13.5545145573031,-21.8411422456075,
12.));
#183716=CARTESIAN_POINT('Ctrl Pts',(13.5529617381573,-21.8134828857967,
12.));
#183717=CARTESIAN_POINT('Ctrl Pts',(13.551350812725,-21.7858978745865,12.));
#183718=CARTESIAN_POINT('Ctrl Pts',(13.5496820422211,-21.7583876294554,
12.));
#183719=CARTESIAN_POINT('Ctrl Pts',(13.5479556704481,-21.7309525412281,
12.));
#183720=CARTESIAN_POINT('Ctrl Pts',(13.5461719295048,-21.7035929822955,
12.));
#183721=CARTESIAN_POINT('Ctrl Pts',(13.5443310461526,-21.6763093157699,
12.));
#183722=CARTESIAN_POINT('Ctrl Pts',(13.5424332480699,-21.6491019044648,
12.));
#183723=CARTESIAN_POINT('Ctrl Pts',(13.5404787697791,-21.6219711193946,
12.));
#183724=CARTESIAN_POINT('Ctrl Pts',(13.5384678597195,-21.5949173499013,
12.));
#183725=CARTESIAN_POINT('Ctrl Pts',(13.536400779028,-21.5679410019002,12.));
#183726=CARTESIAN_POINT('Ctrl Pts',(13.5342777983214,-21.5410424932503,
12.));
#183727=CARTESIAN_POINT('Ctrl Pts',(13.5320991952138,-21.5142222501666,
12.));
#183728=CARTESIAN_POINT('Ctrl Pts',(13.5298652514355,-21.4874807030468,
12.));
#183729=CARTESIAN_POINT('Ctrl Pts',(13.5275762503555,-21.4608182828697,
12.));
#183730=CARTESIAN_POINT('Ctrl Pts',(13.5252324737801,-21.4342354165259,
12.));
#183731=CARTESIAN_POINT('Ctrl Pts',(13.5228342013516,-21.4077325259324,
12.));
#183732=CARTESIAN_POINT('Ctrl Pts',(13.5203817122503,-21.3813100304973,
12.));
#183733=CARTESIAN_POINT('Ctrl Pts',(13.5178752862466,-21.3549683486222,
12.));
#183734=CARTESIAN_POINT('Ctrl Pts',(13.5153152050555,-21.3287078996341,
12.));
#183735=CARTESIAN_POINT('Ctrl Pts',(13.5127017534971,-21.3025291054235,
12.));
#183736=CARTESIAN_POINT('Ctrl Pts',(13.5100352209205,-21.2764323924442,
12.));
#183737=CARTESIAN_POINT('Ctrl Pts',(13.5073159019452,-21.250418192743,12.));
#183738=CARTESIAN_POINT('Ctrl Pts',(13.5045440957404,-21.2244869429332,
12.));
#183739=CARTESIAN_POINT('Ctrl Pts',(13.5017201056088,-21.1986390835828,
12.));
#183740=CARTESIAN_POINT('Ctrl Pts',(13.4988442384491,-21.1728750584175,
12.));
#183741=CARTESIAN_POINT('Ctrl Pts',(13.4959168042934,-21.1471953136209,
12.));
#183742=CARTESIAN_POINT('Ctrl Pts',(13.4929381157778,-21.1216002970207,
12.));
#183743=CARTESIAN_POINT('Ctrl Pts',(13.4899084877717,-21.0960904575046,
12.));
#183744=CARTESIAN_POINT('Ctrl Pts',(13.4868282377191,-21.0706662455199,
12.));
#183745=CARTESIAN_POINT('Ctrl Pts',(13.4836976858912,-21.0453281134245,
12.));
#183746=CARTESIAN_POINT('Ctrl Pts',(13.4805171556822,-21.0200765158884,
12.));
#183747=CARTESIAN_POINT('Ctrl Pts',(13.4772869738878,-20.9949119102592,
12.));
#183748=CARTESIAN_POINT('Ctrl Pts',(13.4740074710086,-20.9698347569477,
12.));
#183749=CARTESIAN_POINT('Ctrl Pts',(13.4706789815166,-20.9448455197557,
12.));
#183750=CARTESIAN_POINT('Ctrl Pts',(13.4673018437717,-20.9199446657583,
12.));
#183751=CARTESIAN_POINT('Ctrl Pts',(13.4638763999725,-20.8951326652158,
12.));
#183752=CARTESIAN_POINT('Ctrl Pts',(13.4604029960983,-20.8704099914641,
12.));
#183753=CARTESIAN_POINT('Ctrl Pts',(13.4568819818631,-20.8457771208083,
12.));
#183754=CARTESIAN_POINT('Ctrl Pts',(13.4533137106667,-20.821234532398,12.));
#183755=CARTESIAN_POINT('Ctrl Pts',(13.4496985395637,-20.7967827081228,
12.));
#183756=CARTESIAN_POINT('Ctrl Pts',(13.4460368293689,-20.7724221327609,
12.));
#183757=CARTESIAN_POINT('Ctrl Pts',(13.4423289447561,-20.7481532941014,
12.));
#183758=CARTESIAN_POINT('Ctrl Pts',(13.4385752543663,-20.7239766830676,
12.));
#183759=CARTESIAN_POINT('Ctrl Pts',(13.4347761309154,-20.6998927938288,
12.));
#183760=CARTESIAN_POINT('Ctrl Pts',(13.4309319513119,-20.6759021239102,
12.));
#183761=CARTESIAN_POINT('Ctrl Pts',(13.427043096765,-20.6520051742868,12.));
#183762=CARTESIAN_POINT('Ctrl Pts',(13.4231099528178,-20.6282024494234,
12.));
#183763=CARTESIAN_POINT('Ctrl Pts',(13.4191329093931,-20.6044944573151,
12.));
#183764=CARTESIAN_POINT('Ctrl Pts',(13.415112360841,-20.5808817095155,12.));
#183765=CARTESIAN_POINT('Ctrl Pts',(13.4110487059912,-20.557364721164,12.));
#183766=CARTESIAN_POINT('Ctrl Pts',(13.4069423482076,-20.5339440109958,
12.));
#183767=CARTESIAN_POINT('Ctrl Pts',(13.4027936954529,-20.5106201013755,
12.));
#183768=CARTESIAN_POINT('Ctrl Pts',(13.3986031603716,-20.4873935184041,
12.));
#183769=CARTESIAN_POINT('Ctrl Pts',(13.3943711603739,-20.4642647920038,
12.));
#183770=CARTESIAN_POINT('Ctrl Pts',(13.3900981177254,-20.4412344560007,
12.));
#183771=CARTESIAN_POINT('Ctrl Pts',(13.3857844596387,-20.4183030482002,
12.));
#183772=CARTESIAN_POINT('Ctrl Pts',(13.3814306183721,-20.3954711104505,
12.));
#183773=CARTESIAN_POINT('Ctrl Pts',(13.377037031319,-20.3727391887187,12.));
#183774=CARTESIAN_POINT('Ctrl Pts',(13.3726041410869,-20.3501078331818,
12.));
#183775=CARTESIAN_POINT('Ctrl Pts',(13.3681323955828,-20.3275775983032,
12.));
#183776=CARTESIAN_POINT('Ctrl Pts',(13.3636222481016,-20.3051490429049,
12.));
#183777=CARTESIAN_POINT('Ctrl Pts',(13.3590741574194,-20.2828227302337,
12.));
#183778=CARTESIAN_POINT('Ctrl Pts',(13.3544885878886,-20.2605992280117,
12.));
#183779=CARTESIAN_POINT('Ctrl Pts',(13.3498660095381,-20.2384791085354,
12.));
#183780=CARTESIAN_POINT('Ctrl Pts',(13.3452068981762,-20.2164629487855,
12.));
#183781=CARTESIAN_POINT('Ctrl Pts',(13.3405117354969,-20.1945513305233,
12.));
#183782=CARTESIAN_POINT('Ctrl Pts',(13.3357810091903,-20.1727448403818,
12.));
#183783=CARTESIAN_POINT('Ctrl Pts',(13.3310152130565,-20.1510440699477,
12.));
#183784=CARTESIAN_POINT('Ctrl Pts',(13.3262148471228,-20.1294496158405,
12.));
#183785=CARTESIAN_POINT('Ctrl Pts',(13.3213804177588,-20.1079620798377,
12.));
#183786=CARTESIAN_POINT('Ctrl Pts',(13.3165124377962,-20.0865820689884,
12.));
#183787=CARTESIAN_POINT('Ctrl Pts',(13.3116114266514,-20.0653101957188,
12.));
#183788=CARTESIAN_POINT('Ctrl Pts',(13.3066779104515,-20.0441470779345,
12.));
#183789=CARTESIAN_POINT('Ctrl Pts',(13.3017124221639,-20.023093339104,12.));
#183790=CARTESIAN_POINT('Ctrl Pts',(13.296715501731,-20.0021496083742,12.));
#183791=CARTESIAN_POINT('Ctrl Pts',(13.2916876962098,-19.9813165207174,
12.));
#183792=CARTESIAN_POINT('Ctrl Pts',(13.2866295599152,-19.9605947170589,
12.));
#183793=CARTESIAN_POINT('Ctrl Pts',(13.2815416545662,-19.939984844402,12.));
#183794=CARTESIAN_POINT('Ctrl Pts',(13.2764245494354,-19.9194875559419,
12.));
#183795=CARTESIAN_POINT('Ctrl Pts',(13.2712788215015,-19.8991035111739,
12.));
#183796=CARTESIAN_POINT('Ctrl Pts',(13.2661050556128,-19.8788333760571,
12.));
#183797=CARTESIAN_POINT('Ctrl Pts',(13.2609038446525,-19.8586778231711,
12.));
#183798=CARTESIAN_POINT('Ctrl Pts',(13.2556757897085,-19.8386375318632,
12.));
#183799=CARTESIAN_POINT('Ctrl Pts',(13.2504215002458,-19.8187131883919,
12.));
#183800=CARTESIAN_POINT('Ctrl Pts',(13.2451415942809,-19.7989054860501,
12.));
#183801=CARTESIAN_POINT('Ctrl Pts',(13.239836698568,-19.7792151253297,12.));
#183802=CARTESIAN_POINT('Ctrl Pts',(13.2345074487968,-19.7596428141176,
12.));
#183803=CARTESIAN_POINT('Ctrl Pts',(13.2291544897902,-19.7401892678701,
12.));
#183804=CARTESIAN_POINT('Ctrl Pts',(13.2237784757065,-19.7208552097867,
12.));
#183805=CARTESIAN_POINT('Ctrl Pts',(13.2183800702431,-19.7016413709678,
12.));
#183806=CARTESIAN_POINT('Ctrl Pts',(13.2129599468478,-19.6825484905812,
12.));
#183807=CARTESIAN_POINT('Ctrl Pts',(13.2075187889522,-19.6635773160924,
12.));
#183808=CARTESIAN_POINT('Ctrl Pts',(13.202057290206,-19.6447286034764,12.));
#183809=CARTESIAN_POINT('Ctrl Pts',(13.196576154715,-19.6260031174244,12.));
#183810=CARTESIAN_POINT('Ctrl Pts',(13.1910760972818,-19.6074016315421,
12.));
#183811=CARTESIAN_POINT('Ctrl Pts',(13.1855578436479,-19.5889249285352,
12.));
#183812=CARTESIAN_POINT('Ctrl Pts',(13.1800221307682,-19.5705738004682,
12.));
#183813=CARTESIAN_POINT('Ctrl Pts',(13.1744697070918,-19.5523490490254,
12.));
#183814=CARTESIAN_POINT('Ctrl Pts',(13.1689013328432,-19.5342514857564,
12.));
#183815=CARTESIAN_POINT('Ctrl Pts',(13.1633177803097,-19.5162819323207,
12.));
#183816=CARTESIAN_POINT('Ctrl Pts',(13.1577198341238,-19.498441220707,12.));
#183817=CARTESIAN_POINT('Ctrl Pts',(13.1521082915846,-19.4807301935256,
12.));
#183818=CARTESIAN_POINT('Ctrl Pts',(13.1464839629966,-19.463149704325,12.));
#183819=CARTESIAN_POINT('Ctrl Pts',(13.140847672006,-19.4457006178875,12.));
#183820=CARTESIAN_POINT('Ctrl Pts',(13.1352002559439,-19.4283838105265,
12.));
#183821=CARTESIAN_POINT('Ctrl Pts',(13.1295425661635,-19.4112001703561,
12.));
#183822=CARTESIAN_POINT('Ctrl Pts',(13.1238754684177,-19.3941505976267,
12.));
#183823=CARTESIAN_POINT('Ctrl Pts',(13.118199843271,-19.3772360051093,12.));
#183824=CARTESIAN_POINT('Ctrl Pts',(13.1125165865021,-19.3604573184516,
12.));
#183825=CARTESIAN_POINT('Ctrl Pts',(13.1068266095186,-19.3438154765395,
12.));
#183826=CARTESIAN_POINT('Ctrl Pts',(13.1011308397591,-19.3273114318268,
12.));
#183827=CARTESIAN_POINT('Ctrl Pts',(13.095430221148,-19.3109461507358,12.));
#183828=CARTESIAN_POINT('Ctrl Pts',(13.0897257145969,-19.2947206141246,
12.));
#183829=CARTESIAN_POINT('Ctrl Pts',(13.0840182984949,-19.2786358177198,
12.));
#183830=CARTESIAN_POINT('Ctrl Pts',(13.0783089692117,-19.2626927725596,
12.));
#183831=CARTESIAN_POINT('Ctrl Pts',(13.0725987415856,-19.2468925053988,
12.));
#183832=CARTESIAN_POINT('Ctrl Pts',(13.0668886494791,-19.2312360592031,
12.));
#183833=CARTESIAN_POINT('Ctrl Pts',(13.0611797463912,-19.2157244937141,
12.));
#183834=CARTESIAN_POINT('Ctrl Pts',(13.0554731060537,-19.2003588859771,
12.));
#183835=CARTESIAN_POINT('Ctrl Pts',(13.0497698230442,-19.1851403308826,
12.));
#183836=CARTESIAN_POINT('Ctrl Pts',(13.0440710133775,-19.1700699416625,
12.));
#183837=CARTESIAN_POINT('Ctrl Pts',(13.0383778152072,-19.1551488505233,
12.));
#183838=CARTESIAN_POINT('Ctrl Pts',(13.0326913895841,-19.1403782093389,
12.));
#183839=CARTESIAN_POINT('Ctrl Pts',(13.0270129211976,-19.1257591903099,
12.));
#183840=CARTESIAN_POINT('Ctrl Pts',(13.0213436191326,-19.1112929866308,
12.));
#183841=CARTESIAN_POINT('Ctrl Pts',(13.0156847176093,-19.0969808131226,
12.));
#183842=CARTESIAN_POINT('Ctrl Pts',(13.0100374768785,-19.0828239070482,
12.));
#183843=CARTESIAN_POINT('Ctrl Pts',(13.0044031841381,-19.0688235289437,
12.));
#183844=CARTESIAN_POINT('Ctrl Pts',(12.9987831544502,-19.0549809634355,
12.));
#183845=CARTESIAN_POINT('Ctrl Pts',(12.9931787316514,-19.0412975200398,
12.));
#183846=CARTESIAN_POINT('Ctrl Pts',(12.9875912893003,-19.0277745339908,
12.));
#183847=CARTESIAN_POINT('Ctrl Pts',(12.9820222318715,-19.0144133673348,
12.));
#183848=CARTESIAN_POINT('Ctrl Pts',(12.9764729959205,-19.0012154099791,
12.));
#183849=CARTESIAN_POINT('Ctrl Pts',(12.9709450512747,-18.9881820807586,
12.));
#183850=CARTESIAN_POINT('Ctrl Pts',(12.9654399021869,-18.9753148284475,
12.));
#183851=CARTESIAN_POINT('Ctrl Pts',(12.9599590886319,-18.9626151329229,
12.));
#183852=CARTESIAN_POINT('Ctrl Pts',(12.9545041877377,-18.9500845064715,
12.));
#183853=CARTESIAN_POINT('Ctrl Pts',(12.9490768151821,-18.9377244950435,
12.));
#183854=CARTESIAN_POINT('Ctrl Pts',(12.9436786266105,-18.9255366795195,
12.));
#183855=CARTESIAN_POINT('Ctrl Pts',(12.9383113190374,-18.9135226769466,
12.));
#183856=CARTESIAN_POINT('Ctrl Pts',(12.9329766328184,-18.9016841423403,
12.));
#183857=CARTESIAN_POINT('Ctrl Pts',(12.9276763536373,-18.8900227704889,
12.));
#183858=CARTESIAN_POINT('Ctrl Pts',(12.9224123144981,-18.8785402977528,
12.));
#183859=CARTESIAN_POINT('Ctrl Pts',(12.9171863977045,-18.8672385038326,
12.));
#183860=CARTESIAN_POINT('Ctrl Pts',(12.9120005369063,-18.8561192136198,
12.));
#183861=CARTESIAN_POINT('Ctrl Pts',(12.9068567191854,-18.8451842990984,
12.));
#183862=CARTESIAN_POINT('Ctrl Pts',(12.9017569871738,-18.8344356812591,
12.));
#183863=CARTESIAN_POINT('Ctrl Pts',(12.8967034410754,-18.8238753319129,
12.));
#183864=CARTESIAN_POINT('Ctrl Pts',(12.8916982409935,-18.813505275782,12.));
#183865=CARTESIAN_POINT('Ctrl Pts',(12.8867436109546,-18.8033275941943,
12.));
#183866=CARTESIAN_POINT('Ctrl Pts',(12.8818418427475,-18.7933444285868,
12.));
#183867=CARTESIAN_POINT('Ctrl Pts',(12.8769952998095,-18.7835579840477,
12.));
#183868=CARTESIAN_POINT('Ctrl Pts',(12.872206421181,-18.7739705329022,12.));
#183869=CARTESIAN_POINT('Ctrl Pts',(12.8674777239653,-18.7645844169564,
12.));
#183870=CARTESIAN_POINT('Ctrl Pts',(12.8628118054171,-18.7554020493887,
12.));
#183871=CARTESIAN_POINT('Ctrl Pts',(12.8582113455646,-18.7464259171251,
12.));
#183872=CARTESIAN_POINT('Ctrl Pts',(12.8536791086316,-18.7376585820854,
12.));
#183873=CARTESIAN_POINT('Ctrl Pts',(12.8492179511591,-18.7291026886554,
12.));
#183874=CARTESIAN_POINT('Ctrl Pts',(12.8448308329494,-18.7207609737702,
12.));
#183875=CARTESIAN_POINT('Ctrl Pts',(12.8405208263431,-18.7126362754445,
12.));
#183876=CARTESIAN_POINT('Ctrl Pts',(12.8362911280361,-18.7047315436294,
12.));
#183877=CARTESIAN_POINT('Ctrl Pts',(12.8321450599789,-18.6970498410172,
12.));
#183878=CARTESIAN_POINT('Ctrl Pts',(12.8280860635231,-18.6895943376172,
12.));
#183879=CARTESIAN_POINT('Ctrl Pts',(12.8241176980017,-18.6823683094139,
12.));
#183880=CARTESIAN_POINT('Ctrl Pts',(12.8202436318474,-18.6753751301092,
12.));
#183881=CARTESIAN_POINT('Ctrl Pts',(12.8164676687362,-18.66861829528,12.));
#183882=CARTESIAN_POINT('Ctrl Pts',(12.8127937909631,-18.6621014624746,
12.));
#183883=CARTESIAN_POINT('Ctrl Pts',(12.8092261933858,-18.6558284825773,
12.));
#183884=CARTESIAN_POINT('Ctrl Pts',(12.805769331162,-18.6498034438987,12.));
#183885=CARTESIAN_POINT('Ctrl Pts',(12.8024278770152,-18.6440306327456,
12.));
#183886=CARTESIAN_POINT('Ctrl Pts',(12.7992066625264,-18.63851447924,12.));
#183887=CARTESIAN_POINT('Ctrl Pts',(12.796110622225,-18.6332595057006,12.));
#183888=CARTESIAN_POINT('Ctrl Pts',(12.7931447451555,-18.6282702819371,
12.));
#183889=CARTESIAN_POINT('Ctrl Pts',(12.7903142925234,-18.6235516265575,
12.));
#183890=CARTESIAN_POINT('Ctrl Pts',(12.7876249657834,-18.6191087624752,
12.));
#183891=CARTESIAN_POINT('Ctrl Pts',(12.7850831657901,-18.6149475565188,
12.));
#183892=CARTESIAN_POINT('Ctrl Pts',(12.7826959526924,-18.611074482622,12.));
#183893=CARTESIAN_POINT('Ctrl Pts',(12.7804705387658,-18.6074961535723,
12.));
#183894=CARTESIAN_POINT('Ctrl Pts',(12.7784139605066,-18.6042190183704,
12.));
#183895=CARTESIAN_POINT('Ctrl Pts',(12.7765325225081,-18.6012488486709,
12.));
#183896=CARTESIAN_POINT('Ctrl Pts',(12.7748328937638,-18.598591752595,12.));
#183897=CARTESIAN_POINT('Ctrl Pts',(12.7733231262108,-18.5962551167772,
12.));
#183898=CARTESIAN_POINT('Ctrl Pts',(12.7720142287172,-18.5942490615407,
12.));
#183899=CARTESIAN_POINT('Ctrl Pts',(12.7709195951156,-18.5925859134579,
12.));
#183900=CARTESIAN_POINT('Ctrl Pts',(12.7700520897173,-18.5912775137806,
12.));
#183901=CARTESIAN_POINT('Ctrl Pts',(12.7694215127918,-18.5903328777227,
12.));
#183902=CARTESIAN_POINT('Ctrl Pts',(12.769110348199,-18.589871621843,12.));
#183903=CARTESIAN_POINT('Ctrl Pts',(12.768986426692,-18.5896919669165,12.));
#183904=CARTESIAN_POINT('Ctrl Pts',(12.7689524524483,-18.5896460962964,
12.));
#183905=CARTESIAN_POINT('Ctrl Pts',(12.7689476255362,-18.5896416359912,
12.));
#183906=CARTESIAN_POINT('',(12.4528436808172,-18.1294424696716,12.));
#183907=CARTESIAN_POINT('',(6.08648437878337,-8.86099361848466,12.));
#183908=CARTESIAN_POINT('',(12.572596943457,-17.4407513054162,12.));
#183909=CARTESIAN_POINT('Origin',(12.8649829188862,-17.846350172984,12.));
#183910=CARTESIAN_POINT('',(13.5924445804218,-16.6581946899465,12.));
#183911=CARTESIAN_POINT('Origin',(4.50593605254674E-13,-6.37232247690087E-13,
12.));
#183912=CARTESIAN_POINT('',(14.2886635873976,-16.7207683102834,12.));
#183913=CARTESIAN_POINT('Origin',(13.9085479427572,-17.0455945664569,12.));
#183914=CARTESIAN_POINT('',(14.6513681262571,-17.1452095830633,12.));
#183915=CARTESIAN_POINT('',(7.32568406312854,-8.57260479153162,12.));
#183916=CARTESIAN_POINT('',(17.9112098770111,-18.8464468996588,12.));
#183917=CARTESIAN_POINT('Ctrl Pts',(14.6513681262571,-17.1452095830633,
12.));
#183918=CARTESIAN_POINT('Ctrl Pts',(14.6513711852839,-17.1452153999142,
12.));
#183919=CARTESIAN_POINT('Ctrl Pts',(14.6514066997188,-17.1452600887039,
12.));
#183920=CARTESIAN_POINT('Ctrl Pts',(14.6515481598057,-17.1454262858045,
12.));
#183921=CARTESIAN_POINT('Ctrl Pts',(14.65191316345,-17.1458462295273,12.));
#183922=CARTESIAN_POINT('Ctrl Pts',(14.6526624064978,-17.1466998098673,
12.));
#183923=CARTESIAN_POINT('Ctrl Pts',(14.6537016966188,-17.1478763944909,
12.));
#183924=CARTESIAN_POINT('Ctrl Pts',(14.6550248622813,-17.1493641837556,
12.));
#183925=CARTESIAN_POINT('Ctrl Pts',(14.6566237952435,-17.1511476869495,
12.));
#183926=CARTESIAN_POINT('Ctrl Pts',(14.65849005553,-17.1532107762719,12.));
#183927=CARTESIAN_POINT('Ctrl Pts',(14.660616716964,-17.1555401986403,12.));
#183928=CARTESIAN_POINT('Ctrl Pts',(14.662998728599,-17.1581262646789,12.));
#183929=CARTESIAN_POINT('Ctrl Pts',(14.6656319165057,-17.1609609517369,
12.));
#183930=CARTESIAN_POINT('Ctrl Pts',(14.6685123374424,-17.1640366762304,
12.));
#183931=CARTESIAN_POINT('Ctrl Pts',(14.6716355833321,-17.1673449723019,
12.));
#183932=CARTESIAN_POINT('Ctrl Pts',(14.6749971333867,-17.1708771619129,
12.));
#183933=CARTESIAN_POINT('Ctrl Pts',(14.6785925615676,-17.1746247499057,
12.));
#183934=CARTESIAN_POINT('Ctrl Pts',(14.6824178576166,-17.1785800350827,
12.));
#183935=CARTESIAN_POINT('Ctrl Pts',(14.6864694522319,-17.182736158472,12.));
#183936=CARTESIAN_POINT('Ctrl Pts',(14.6907440526957,-17.1870867909918,
12.));
#183937=CARTESIAN_POINT('Ctrl Pts',(14.6952385361706,-17.1916259308416,
12.));
#183938=CARTESIAN_POINT('Ctrl Pts',(14.699949811582,-17.1963476411694,12.));
#183939=CARTESIAN_POINT('Ctrl Pts',(14.7048748502662,-17.2012461084268,
12.));
#183940=CARTESIAN_POINT('Ctrl Pts',(14.7100107213586,-17.2063157097316,
12.));
#183941=CARTESIAN_POINT('Ctrl Pts',(14.7153546289338,-17.2115510835988,
12.));
#183942=CARTESIAN_POINT('Ctrl Pts',(14.7209039390325,-17.2169471814255,
12.));
#183943=CARTESIAN_POINT('Ctrl Pts',(14.7266561494282,-17.2224992099666,
12.));
#183944=CARTESIAN_POINT('Ctrl Pts',(14.7326088681163,-17.2282025904314,
12.));
#183945=CARTESIAN_POINT('Ctrl Pts',(14.7387597858117,-17.2340529062078,
12.));
#183946=CARTESIAN_POINT('Ctrl Pts',(14.7451066593793,-17.2400458713566,
12.));
#183947=CARTESIAN_POINT('Ctrl Pts',(14.7516473175124,-17.2461773413289,
12.));
#183948=CARTESIAN_POINT('Ctrl Pts',(14.7583796616617,-17.2524433146837,
12.));
#183949=CARTESIAN_POINT('Ctrl Pts',(14.7653016697589,-17.2588399401464,
12.));
#183950=CARTESIAN_POINT('Ctrl Pts',(14.7724113956728,-17.2653635155317,
12.));
#183951=CARTESIAN_POINT('Ctrl Pts',(14.7797069617802,-17.2720104735192,
12.));
#183952=CARTESIAN_POINT('Ctrl Pts',(14.787186553128,-17.278777370485,12.));
#183953=CARTESIAN_POINT('Ctrl Pts',(14.7948484105252,-17.28566087332,12.));
#183954=CARTESIAN_POINT('Ctrl Pts',(14.8026908254281,-17.2926577496519,
12.));
#183955=CARTESIAN_POINT('Ctrl Pts',(14.8107121391038,-17.2997648661483,
12.));
#183956=CARTESIAN_POINT('Ctrl Pts',(14.8189107410161,-17.3069791853705,
12.));
#183957=CARTESIAN_POINT('Ctrl Pts',(14.8272850675375,-17.3142977632656,
12.));
#183958=CARTESIAN_POINT('Ctrl Pts',(14.8358336004193,-17.3217177462096,
12.));
#183959=CARTESIAN_POINT('Ctrl Pts',(14.8445548643504,-17.3292363662601,
12.));
#183960=CARTESIAN_POINT('Ctrl Pts',(14.8534474245433,-17.336850936485,12.));
#183961=CARTESIAN_POINT('Ctrl Pts',(14.8625098843419,-17.3445588463477,
12.));
#183962=CARTESIAN_POINT('Ctrl Pts',(14.8717408826957,-17.3523575568648,
12.));
#183963=CARTESIAN_POINT('Ctrl Pts',(14.8811390927424,-17.3602445978163,
12.));
#183964=CARTESIAN_POINT('Ctrl Pts',(14.8907032205789,-17.3682175653236,
12.));
#183965=CARTESIAN_POINT('Ctrl Pts',(14.9004320039609,-17.3762741193075,
12.));
#183966=CARTESIAN_POINT('Ctrl Pts',(14.9103242110057,-17.3844119809823,
12.));
#183967=CARTESIAN_POINT('Ctrl Pts',(14.9203786389343,-17.3926289303987,
12.));
#183968=CARTESIAN_POINT('Ctrl Pts',(14.9305941128758,-17.400922804075,12.));
#183969=CARTESIAN_POINT('Ctrl Pts',(14.940969484645,-17.4092914926072,12.));
#183970=CARTESIAN_POINT('Ctrl Pts',(14.9515036315142,-17.4177329382827,
12.));
#183971=CARTESIAN_POINT('Ctrl Pts',(14.9621954549825,-17.4262451327088,
12.));
#183972=CARTESIAN_POINT('Ctrl Pts',(14.973043879945,-17.4348261151395,12.));
#183973=CARTESIAN_POINT('Ctrl Pts',(14.9840478538357,-17.4434739707773,
12.));
#183974=CARTESIAN_POINT('Ctrl Pts',(14.9952063457779,-17.4521868291005,
12.));
#183975=CARTESIAN_POINT('Ctrl Pts',(15.0065183456922,-17.4609628621419,
12.));
#183976=CARTESIAN_POINT('Ctrl Pts',(15.0179828635087,-17.4698002829357,
12.));
#183977=CARTESIAN_POINT('Ctrl Pts',(15.029598928488,-17.4786973441417,12.));
#183978=CARTESIAN_POINT('Ctrl Pts',(15.0413655884993,-17.4876523366178,
12.));
#183979=CARTESIAN_POINT('Ctrl Pts',(15.0532819093085,-17.4966635880246,
12.));
#183980=CARTESIAN_POINT('Ctrl Pts',(15.0653469738307,-17.5057294613877,
12.));
#183981=CARTESIAN_POINT('Ctrl Pts',(15.0775598815749,-17.5148483539687,
12.));
#183982=CARTESIAN_POINT('Ctrl Pts',(15.0899197481082,-17.5240186961791,
12.));
#183983=CARTESIAN_POINT('Ctrl Pts',(15.1024257045033,-17.5332389504829,
12.));
#183984=CARTESIAN_POINT('Ctrl Pts',(15.1150768967728,-17.5425076102963,
12.));
#183985=CARTESIAN_POINT('Ctrl Pts',(15.1278724853138,-17.5518231989117,
12.));
#183986=CARTESIAN_POINT('Ctrl Pts',(15.1408116444876,-17.5611842686192,
12.));
#183987=CARTESIAN_POINT('Ctrl Pts',(15.1538935621714,-17.5705893998029,
12.));
#183988=CARTESIAN_POINT('Ctrl Pts',(15.1671174393137,-17.580037200054,12.));
#183989=CARTESIAN_POINT('Ctrl Pts',(15.1804824894605,-17.5895263032595,
12.));
#183990=CARTESIAN_POINT('Ctrl Pts',(15.1939879383268,-17.5990553687599,
12.));
#183991=CARTESIAN_POINT('Ctrl Pts',(15.2076330234686,-17.60862308065,12.));
#183992=CARTESIAN_POINT('Ctrl Pts',(15.2214169939199,-17.6182281470468,
12.));
#183993=CARTESIAN_POINT('Ctrl Pts',(15.2353391098366,-17.6278692993764,
12.));
#183994=CARTESIAN_POINT('Ctrl Pts',(15.2493986421092,-17.6375452916369,
12.));
#183995=CARTESIAN_POINT('Ctrl Pts',(15.2635948720292,-17.6472548997328,
12.));
#183996=CARTESIAN_POINT('Ctrl Pts',(15.2779270910239,-17.6569969209,12.));
#183997=CARTESIAN_POINT('Ctrl Pts',(15.2923946003598,-17.6667701731041,
12.));
#183998=CARTESIAN_POINT('Ctrl Pts',(15.30699671085,-17.676573494456,12.));
#183999=CARTESIAN_POINT('Ctrl Pts',(15.3217327425338,-17.6864057426052,
12.));
#184000=CARTESIAN_POINT('Ctrl Pts',(15.3366020244066,-17.6962657941983,
12.));
#184001=CARTESIAN_POINT('Ctrl Pts',(15.351603894206,-17.7061525444042,12.));
#184002=CARTESIAN_POINT('Ctrl Pts',(15.3667376981699,-17.7160649064206,
12.));
#184003=CARTESIAN_POINT('Ctrl Pts',(15.3820027907966,-17.7260018109924,
12.));
#184004=CARTESIAN_POINT('Ctrl Pts',(15.3973985345802,-17.735962205915,12.));
#184005=CARTESIAN_POINT('Ctrl Pts',(15.4129242997837,-17.7459450555813,
12.));
#184006=CARTESIAN_POINT('Ctrl Pts',(15.4285794642667,-17.7559493405881,
12.));
#184007=CARTESIAN_POINT('Ctrl Pts',(15.4443634132869,-17.7659740573265,
12.));
#184008=CARTESIAN_POINT('Ctrl Pts',(15.4602755393017,-17.7760182175815,
12.));
#184009=CARTESIAN_POINT('Ctrl Pts',(15.4763152417497,-17.786080848122,12.));
#184010=CARTESIAN_POINT('Ctrl Pts',(15.4924819268517,-17.7961609903148,
12.));
#184011=CARTESIAN_POINT('Ctrl Pts',(15.5087750074718,-17.8062576997952,
12.));
#184012=CARTESIAN_POINT('Ctrl Pts',(15.5251939029552,-17.8163700461256,
12.));
#184013=CARTESIAN_POINT('Ctrl Pts',(15.541738038964,-17.8264971124607,12.));
#184014=CARTESIAN_POINT('Ctrl Pts',(15.5584068472982,-17.8366379952085,
12.));
#184015=CARTESIAN_POINT('Ctrl Pts',(15.5751997657162,-17.8467918036987,
12.));
#184016=CARTESIAN_POINT('Ctrl Pts',(15.5921162378192,-17.8569576599006,
12.));
#184017=CARTESIAN_POINT('Ctrl Pts',(15.609155712921,-17.8671346981394,12.));
#184018=CARTESIAN_POINT('Ctrl Pts',(15.6263176459108,-17.8773220648125,
12.));
#184019=CARTESIAN_POINT('Ctrl Pts',(15.6436014971084,-17.8875189181091,
12.));
#184020=CARTESIAN_POINT('Ctrl Pts',(15.661006732103,-17.897724427724,12.));
#184021=CARTESIAN_POINT('Ctrl Pts',(15.678532821646,-17.9079377746111,12.));
#184022=CARTESIAN_POINT('Ctrl Pts',(15.6961792415522,-17.9181581507455,
12.));
#184023=CARTESIAN_POINT('Ctrl Pts',(15.7139454725838,-17.9283847588836,
12.));
#184024=CARTESIAN_POINT('Ctrl Pts',(15.7318310003335,-17.9386168123262,
12.));
#184025=CARTESIAN_POINT('Ctrl Pts',(15.749835315086,-17.9488535346781,12.));
#184026=CARTESIAN_POINT('Ctrl Pts',(15.7679579117077,-17.9590941596242,
12.));
#184027=CARTESIAN_POINT('Ctrl Pts',(15.7861982895724,-17.9693379307303,
12.));
#184028=CARTESIAN_POINT('Ctrl Pts',(15.8045559524676,-17.9795841012386,
12.));
#184029=CARTESIAN_POINT('Ctrl Pts',(15.8230304084962,-17.9898319338665,
12.));
#184030=CARTESIAN_POINT('Ctrl Pts',(15.8416211699679,-18.0000807006052,
12.));
#184031=CARTESIAN_POINT('Ctrl Pts',(15.8603277532831,-18.0103296825205,
12.));
#184032=CARTESIAN_POINT('Ctrl Pts',(15.8791496788682,-18.0205781695769,
12.));
#184033=CARTESIAN_POINT('Ctrl Pts',(15.8980864711042,-18.0308254604636,
12.));
#184034=CARTESIAN_POINT('Ctrl Pts',(15.9171376582436,-18.0410708624209,
12.));
#184035=CARTESIAN_POINT('Ctrl Pts',(15.9363027723244,-18.0513136910691,
12.));
#184036=CARTESIAN_POINT('Ctrl Pts',(15.9555813490644,-18.061553270236,12.));
#184037=CARTESIAN_POINT('Ctrl Pts',(15.9749729277846,-18.0717889317958,
12.));
#184038=CARTESIAN_POINT('Ctrl Pts',(15.9944770513613,-18.0820200155236,
12.));
#184039=CARTESIAN_POINT('Ctrl Pts',(16.014093266161,-18.0922458689462,12.));
#184040=CARTESIAN_POINT('Ctrl Pts',(16.0338211219693,-18.1024658471966,
12.));
#184041=CARTESIAN_POINT('Ctrl Pts',(16.0536601719125,-18.112679312869,12.));
#184042=CARTESIAN_POINT('Ctrl Pts',(16.0736099723668,-18.1228856358751,
12.));
#184043=CARTESIAN_POINT('Ctrl Pts',(16.0936700829112,-18.1330841933105,
12.));
#184044=CARTESIAN_POINT('Ctrl Pts',(16.1138400662794,-18.1432743693235,
12.));
#184045=CARTESIAN_POINT('Ctrl Pts',(16.1341194882988,-18.1534555549853,
12.));
#184046=CARTESIAN_POINT('Ctrl Pts',(16.154507917826,-18.1636271481615,12.));
#184047=CARTESIAN_POINT('Ctrl Pts',(16.1750049266671,-18.1737885533849,
12.));
#184048=CARTESIAN_POINT('Ctrl Pts',(16.1956100895073,-18.1839391817331,
12.));
#184049=CARTESIAN_POINT('Ctrl Pts',(16.2163229838875,-18.1940784507229,
12.));
#184050=CARTESIAN_POINT('Ctrl Pts',(16.2371431901638,-18.2042057842035,
12.));
#184051=CARTESIAN_POINT('Ctrl Pts',(16.2580702914615,-18.2143206122529,
12.));
#184052=CARTESIAN_POINT('Ctrl Pts',(16.2791038736223,-18.2244223710746,
12.));
#184053=CARTESIAN_POINT('Ctrl Pts',(16.3002435251378,-18.2345105028982,
12.));
#184054=CARTESIAN_POINT('Ctrl Pts',(16.3214888370987,-18.2445844558742,
12.));
#184055=CARTESIAN_POINT('Ctrl Pts',(16.3428394031589,-18.2546436839608,
12.));
#184056=CARTESIAN_POINT('Ctrl Pts',(16.3642948194868,-18.2646876468169,
12.));
#184057=CARTESIAN_POINT('Ctrl Pts',(16.385854684708,-18.2747158096934,12.));
#184058=CARTESIAN_POINT('Ctrl Pts',(16.4075185998454,-18.2847276433309,
12.));
#184059=CARTESIAN_POINT('Ctrl Pts',(16.4292861682378,-18.294722623851,12.));
#184060=CARTESIAN_POINT('Ctrl Pts',(16.4511569955233,-18.304700232686,12.));
#184061=CARTESIAN_POINT('Ctrl Pts',(16.4731306896441,-18.3146599565231,
12.));
#184062=CARTESIAN_POINT('Ctrl Pts',(16.4952068608345,-18.3246012872469,
12.));
#184063=CARTESIAN_POINT('Ctrl Pts',(16.5173851216045,-18.3345237218864,
12.));
#184064=CARTESIAN_POINT('Ctrl Pts',(16.5396650867139,-18.34442676256,12.));
#184065=CARTESIAN_POINT('Ctrl Pts',(16.5620463731413,-18.354309916433,12.));
#184066=CARTESIAN_POINT('Ctrl Pts',(16.5845286000217,-18.3641726955889,
12.));
#184067=CARTESIAN_POINT('Ctrl Pts',(16.607111388571,-18.3740146168879,12.));
#184068=CARTESIAN_POINT('Ctrl Pts',(16.6297943620056,-18.3838352018327,
12.));
#184069=CARTESIAN_POINT('Ctrl Pts',(16.6525771454513,-18.3936339764332,
12.));
#184070=CARTESIAN_POINT('Ctrl Pts',(16.6754593658513,-18.403410471079,12.));
#184071=CARTESIAN_POINT('Ctrl Pts',(16.698440651849,-18.413164220399,12.));
#184072=CARTESIAN_POINT('Ctrl Pts',(16.7215206338818,-18.4228947633187,
12.));
#184073=CARTESIAN_POINT('Ctrl Pts',(16.7446989442882,-18.4326016431392,
12.));
#184074=CARTESIAN_POINT('Ctrl Pts',(16.7679752173992,-18.44228440761,12.));
#184075=CARTESIAN_POINT('Ctrl Pts',(16.791349089629,-18.4519426090124,12.));
#184076=CARTESIAN_POINT('Ctrl Pts',(16.8148201995472,-18.4615758042305,
12.));
#184077=CARTESIAN_POINT('Ctrl Pts',(16.8383881879709,-18.4711835548623,
12.));
#184078=CARTESIAN_POINT('Ctrl Pts',(16.8620526977171,-18.4807654268771,
12.));
#184079=CARTESIAN_POINT('Ctrl Pts',(16.8858133733088,-18.4903209902227,
12.));
#184080=CARTESIAN_POINT('Ctrl Pts',(16.9096698606943,-18.499849818462,12.));
#184081=CARTESIAN_POINT('Ctrl Pts',(16.9336218069353,-18.5093514883835,
12.));
#184082=CARTESIAN_POINT('Ctrl Pts',(16.9576688599339,-18.5188255796659,
12.));
#184083=CARTESIAN_POINT('Ctrl Pts',(16.981810668038,-18.5282716744197,12.));
#184084=CARTESIAN_POINT('Ctrl Pts',(17.0060468805097,-18.5376893576961,
12.));
#184085=CARTESIAN_POINT('Ctrl Pts',(17.0303771481738,-18.547078218209,12.));
#184086=CARTESIAN_POINT('Ctrl Pts',(17.0548011239751,-18.556437848963,12.));
#184087=CARTESIAN_POINT('Ctrl Pts',(17.0793184636079,-18.5657678479789,
12.));
#184088=CARTESIAN_POINT('Ctrl Pts',(17.1039288260001,-18.5750678188542,
12.));
#184089=CARTESIAN_POINT('Ctrl Pts',(17.1286318741183,-18.5843373717247,
12.));
#184090=CARTESIAN_POINT('Ctrl Pts',(17.1534272741643,-18.5935761222825,
12.));
#184091=CARTESIAN_POINT('Ctrl Pts',(17.1783146940127,-18.6027836898817,
12.));
#184092=CARTESIAN_POINT('Ctrl Pts',(17.2032938019284,-18.6119596959949,
12.));
#184093=CARTESIAN_POINT('Ctrl Pts',(17.2283642650517,-18.6211037624038,
12.));
#184094=CARTESIAN_POINT('Ctrl Pts',(17.2535257482187,-18.6302155097943,
12.));
#184095=CARTESIAN_POINT('Ctrl Pts',(17.2787779120213,-18.6392945554748,
12.));
#184096=CARTESIAN_POINT('Ctrl Pts',(17.3041204135074,-18.6483405141865,
12.));
#184097=CARTESIAN_POINT('Ctrl Pts',(17.3295529098618,-18.6573530024033,
12.));
#184098=CARTESIAN_POINT('Ctrl Pts',(17.3550750612443,-18.6663316416582,
12.));
#184099=CARTESIAN_POINT('Ctrl Pts',(17.3806865340747,-18.6752760624052,
12.));
#184100=CARTESIAN_POINT('Ctrl Pts',(17.4063870038562,-18.6841859073471,
12.));
#184101=CARTESIAN_POINT('Ctrl Pts',(17.4321761588142,-18.6930608357409,
12.));
#184102=CARTESIAN_POINT('Ctrl Pts',(17.4580537012753,-18.70190052503,12.));
#184103=CARTESIAN_POINT('Ctrl Pts',(17.4840193397162,-18.7107046613912,
12.));
#184104=CARTESIAN_POINT('Ctrl Pts',(17.5100727820876,-18.7194729318098,
12.));
#184105=CARTESIAN_POINT('Ctrl Pts',(17.5362137287593,-18.7282050157138,
12.));
#184106=CARTESIAN_POINT('Ctrl Pts',(17.5624418653245,-18.7369005764553,
12.));
#184107=CARTESIAN_POINT('Ctrl Pts',(17.5887568561371,-18.7455592536688,
12.));
#184108=CARTESIAN_POINT('Ctrl Pts',(17.6151583357012,-18.7541806530984,
12.));
#184109=CARTESIAN_POINT('Ctrl Pts',(17.6416459210681,-18.762764361321,12.));
#184110=CARTESIAN_POINT('Ctrl Pts',(17.6682192274236,-18.7713099642754,
12.));
#184111=CARTESIAN_POINT('Ctrl Pts',(17.6948778823014,-18.7798170641374,
12.));
#184112=CARTESIAN_POINT('Ctrl Pts',(17.7216215409035,-18.788285297605,12.));
#184113=CARTESIAN_POINT('Ctrl Pts',(17.7484498996905,-18.7967143519419,
12.));
#184114=CARTESIAN_POINT('Ctrl Pts',(17.7753627137853,-18.8051039860448,
12.));
#184115=CARTESIAN_POINT('Ctrl Pts',(17.8023598011057,-18.8134540340417,
12.));
#184116=CARTESIAN_POINT('Ctrl Pts',(17.8294410311006,-18.8217643886157,
12.));
#184117=CARTESIAN_POINT('Ctrl Pts',(17.856606317477,-18.8300349895974,12.));
#184118=CARTESIAN_POINT('Ctrl Pts',(17.8784057509355,-18.8366196462581,
12.));
#184119=CARTESIAN_POINT('Ctrl Pts',(17.8947931177807,-18.8415402351786,
12.));
#184120=CARTESIAN_POINT('Ctrl Pts',(17.9057348246595,-18.8448126709692,
12.));
#184121=CARTESIAN_POINT('Ctrl Pts',(17.9112098770111,-18.8464468996588,
12.));
#184122=CARTESIAN_POINT('',(18.8464468996588,-17.9112098770111,12.));
#184123=CARTESIAN_POINT('Origin',(0.,0.,12.));
#184124=CARTESIAN_POINT('',(17.1452095830632,-14.6513681262571,12.));
#184125=CARTESIAN_POINT('Ctrl Pts',(18.8464468996588,-17.9112098770111,
12.));
#184126=CARTESIAN_POINT('Ctrl Pts',(18.8448126709726,-17.9057348246611,
12.));
#184127=CARTESIAN_POINT('Ctrl Pts',(18.8415402351882,-17.8947931177853,
12.));
#184128=CARTESIAN_POINT('Ctrl Pts',(18.8366196462746,-17.8784057509434,
12.));
#184129=CARTESIAN_POINT('Ctrl Pts',(18.8300349896187,-17.8566063174871,
12.));
#184130=CARTESIAN_POINT('Ctrl Pts',(18.8217643886368,-17.8294410311105,
12.));
#184131=CARTESIAN_POINT('Ctrl Pts',(18.8134540340581,-17.8023598011135,
12.));
#184132=CARTESIAN_POINT('Ctrl Pts',(18.8051039860543,-17.7753627137898,
12.));
#184133=CARTESIAN_POINT('Ctrl Pts',(18.7967143519444,-17.7484498996916,
12.));
#184134=CARTESIAN_POINT('Ctrl Pts',(18.7882852976016,-17.7216215409019,
12.));
#184135=CARTESIAN_POINT('Ctrl Pts',(18.7798170641305,-17.6948778822982,
12.));
#184136=CARTESIAN_POINT('Ctrl Pts',(18.7713099642673,-17.6682192274197,
12.));
#184137=CARTESIAN_POINT('Ctrl Pts',(18.7627643613139,-17.6416459210646,
12.));
#184138=CARTESIAN_POINT('Ctrl Pts',(18.7541806530935,-17.6151583356989,
12.));
#184139=CARTESIAN_POINT('Ctrl Pts',(18.7455592536667,-17.5887568561361,
12.));
#184140=CARTESIAN_POINT('Ctrl Pts',(18.7369005764558,-17.5624418653248,
12.));
#184141=CARTESIAN_POINT('Ctrl Pts',(18.728205015716,-17.5362137287604,12.));
#184142=CARTESIAN_POINT('Ctrl Pts',(18.7194729318127,-17.5100727820891,
12.));
#184143=CARTESIAN_POINT('Ctrl Pts',(18.7107046613941,-17.4840193397176,
12.));
#184144=CARTESIAN_POINT('Ctrl Pts',(18.7019005250322,-17.4580537012764,
12.));
#184145=CARTESIAN_POINT('Ctrl Pts',(18.6930608357421,-17.4321761588148,
12.));
#184146=CARTESIAN_POINT('Ctrl Pts',(18.6841859073472,-17.4063870038563,
12.));
#184147=CARTESIAN_POINT('Ctrl Pts',(18.6752760624045,-17.3806865340744,
12.));
#184148=CARTESIAN_POINT('Ctrl Pts',(18.6663316416569,-17.3550750612438,
12.));
#184149=CARTESIAN_POINT('Ctrl Pts',(18.6573530024019,-17.3295529098612,
12.));
#184150=CARTESIAN_POINT('Ctrl Pts',(18.6483405141853,-17.3041204135069,
12.));
#184151=CARTESIAN_POINT('Ctrl Pts',(18.639294555474,-17.278777912021,12.));
#184152=CARTESIAN_POINT('Ctrl Pts',(18.630215509794,-17.2535257482186,12.));
#184153=CARTESIAN_POINT('Ctrl Pts',(18.6211037624041,-17.2283642650519,
12.));
#184154=CARTESIAN_POINT('Ctrl Pts',(18.6119596959957,-17.2032938019288,
12.));
#184155=CARTESIAN_POINT('Ctrl Pts',(18.6027836898826,-17.1783146940131,
12.));
#184156=CARTESIAN_POINT('Ctrl Pts',(18.5935761222833,-17.1534272741646,
12.));
#184157=CARTESIAN_POINT('Ctrl Pts',(18.5843373717253,-17.1286318741185,
12.));
#184158=CARTESIAN_POINT('Ctrl Pts',(18.5750678188543,-17.1039288260002,
12.));
#184159=CARTESIAN_POINT('Ctrl Pts',(18.5657678479788,-17.0793184636079,
12.));
#184160=CARTESIAN_POINT('Ctrl Pts',(18.5564378489628,-17.0548011239751,
12.));
#184161=CARTESIAN_POINT('Ctrl Pts',(18.5470782182089,-17.030377148174,12.));
#184162=CARTESIAN_POINT('Ctrl Pts',(18.5376893576961,-17.0060468805099,
12.));
#184163=CARTESIAN_POINT('Ctrl Pts',(18.5282716744198,-16.9818106680382,
12.));
#184164=CARTESIAN_POINT('Ctrl Pts',(18.518825579666,-16.957668859934,12.));
#184165=CARTESIAN_POINT('Ctrl Pts',(18.5093514883835,-16.9336218069353,
12.));
#184166=CARTESIAN_POINT('Ctrl Pts',(18.4998498184619,-16.9096698606942,
12.));
#184167=CARTESIAN_POINT('Ctrl Pts',(18.4903209902226,-16.8858133733086,
12.));
#184168=CARTESIAN_POINT('Ctrl Pts',(18.4807654268769,-16.8620526977169,
12.));
#184169=CARTESIAN_POINT('Ctrl Pts',(18.4711835548622,-16.8383881879707,
12.));
#184170=CARTESIAN_POINT('Ctrl Pts',(18.4615758042305,-16.8148201995472,
12.));
#184171=CARTESIAN_POINT('Ctrl Pts',(18.4519426090124,-16.791349089629,12.));
#184172=CARTESIAN_POINT('Ctrl Pts',(18.4422844076099,-16.7679752173992,
12.));
#184173=CARTESIAN_POINT('Ctrl Pts',(18.4326016431392,-16.7446989442882,
12.));
#184174=CARTESIAN_POINT('Ctrl Pts',(18.4228947633186,-16.7215206338818,
12.));
#184175=CARTESIAN_POINT('Ctrl Pts',(18.4131642203989,-16.698440651849,12.));
#184176=CARTESIAN_POINT('Ctrl Pts',(18.4034104710789,-16.6754593658513,
12.));
#184177=CARTESIAN_POINT('Ctrl Pts',(18.3936339764332,-16.6525771454513,
12.));
#184178=CARTESIAN_POINT('Ctrl Pts',(18.3838352018327,-16.6297943620056,
12.));
#184179=CARTESIAN_POINT('Ctrl Pts',(18.3740146168879,-16.6071113885711,
12.));
#184180=CARTESIAN_POINT('Ctrl Pts',(18.364172695589,-16.5845286000218,12.));
#184181=CARTESIAN_POINT('Ctrl Pts',(18.3543099164331,-16.5620463731414,
12.));
#184182=CARTESIAN_POINT('Ctrl Pts',(18.3444267625601,-16.5396650867139,
12.));
#184183=CARTESIAN_POINT('Ctrl Pts',(18.3345237218864,-16.5173851216045,
12.));
#184184=CARTESIAN_POINT('Ctrl Pts',(18.3246012872468,-16.4952068608344,
12.));
#184185=CARTESIAN_POINT('Ctrl Pts',(18.3146599565229,-16.4731306896439,
12.));
#184186=CARTESIAN_POINT('Ctrl Pts',(18.3047002326858,-16.4511569955231,
12.));
#184187=CARTESIAN_POINT('Ctrl Pts',(18.2947226238509,-16.4292861682377,
12.));
#184188=CARTESIAN_POINT('Ctrl Pts',(18.2847276433308,-16.4075185998454,
12.));
#184189=CARTESIAN_POINT('Ctrl Pts',(18.2747158096934,-16.385854684708,12.));
#184190=CARTESIAN_POINT('Ctrl Pts',(18.2646876468169,-16.3642948194869,
12.));
#184191=CARTESIAN_POINT('Ctrl Pts',(18.2546436839609,-16.342839403159,12.));
#184192=CARTESIAN_POINT('Ctrl Pts',(18.2445844558742,-16.3214888370988,
12.));
#184193=CARTESIAN_POINT('Ctrl Pts',(18.2345105028981,-16.3002435251378,
12.));
#184194=CARTESIAN_POINT('Ctrl Pts',(18.2244223710745,-16.2791038736223,
12.));
#184195=CARTESIAN_POINT('Ctrl Pts',(18.214320612253,-16.2580702914615,12.));
#184196=CARTESIAN_POINT('Ctrl Pts',(18.2042057842037,-16.237143190164,12.));
#184197=CARTESIAN_POINT('Ctrl Pts',(18.1940784507232,-16.2163229838878,
12.));
#184198=CARTESIAN_POINT('Ctrl Pts',(18.1839391817335,-16.1956100895076,
12.));
#184199=CARTESIAN_POINT('Ctrl Pts',(18.1737885533852,-16.1750049266673,
12.));
#184200=CARTESIAN_POINT('Ctrl Pts',(18.1636271481616,-16.1545079178261,
12.));
#184201=CARTESIAN_POINT('Ctrl Pts',(18.153455554985,-16.1341194882987,12.));
#184202=CARTESIAN_POINT('Ctrl Pts',(18.1432743693231,-16.113840066279,12.));
#184203=CARTESIAN_POINT('Ctrl Pts',(18.1330841933099,-16.0936700829108,
12.));
#184204=CARTESIAN_POINT('Ctrl Pts',(18.1228856358746,-16.0736099723664,
12.));
#184205=CARTESIAN_POINT('Ctrl Pts',(18.1126793128688,-16.0536601719124,
12.));
#184206=CARTESIAN_POINT('Ctrl Pts',(18.1024658471966,-16.0338211219694,
12.));
#184207=CARTESIAN_POINT('Ctrl Pts',(18.0922458689464,-16.0140932661612,
12.));
#184208=CARTESIAN_POINT('Ctrl Pts',(18.0820200155239,-15.9944770513616,
12.));
#184209=CARTESIAN_POINT('Ctrl Pts',(18.071788931796,-15.9749729277848,12.));
#184210=CARTESIAN_POINT('Ctrl Pts',(18.061553270236,-15.9555813490645,12.));
#184211=CARTESIAN_POINT('Ctrl Pts',(18.0513136910691,-15.9363027723244,
12.));
#184212=CARTESIAN_POINT('Ctrl Pts',(18.0410708624208,-15.9171376582436,
12.));
#184213=CARTESIAN_POINT('Ctrl Pts',(18.0308254604638,-15.8980864711043,
12.));
#184214=CARTESIAN_POINT('Ctrl Pts',(18.0205781695773,-15.8791496788685,
12.));
#184215=CARTESIAN_POINT('Ctrl Pts',(18.010329682521,-15.8603277532834,12.));
#184216=CARTESIAN_POINT('Ctrl Pts',(18.0000807006055,-15.8416211699682,
12.));
#184217=CARTESIAN_POINT('Ctrl Pts',(17.9898319338664,-15.8230304084963,
12.));
#184218=CARTESIAN_POINT('Ctrl Pts',(17.9795841012383,-15.8045559524674,
12.));
#184219=CARTESIAN_POINT('Ctrl Pts',(17.9693379307297,-15.786198289572,12.));
#184220=CARTESIAN_POINT('Ctrl Pts',(17.9590941596236,-15.7679579117072,
12.));
#184221=CARTESIAN_POINT('Ctrl Pts',(17.9488535346776,-15.7498353150856,
12.));
#184222=CARTESIAN_POINT('Ctrl Pts',(17.9386168123261,-15.7318310003334,
12.));
#184223=CARTESIAN_POINT('Ctrl Pts',(17.9283847588837,-15.713945472584,12.));
#184224=CARTESIAN_POINT('Ctrl Pts',(17.918158150746,-15.6961792415526,12.));
#184225=CARTESIAN_POINT('Ctrl Pts',(17.9079377746118,-15.6785328216467,
12.));
#184226=CARTESIAN_POINT('Ctrl Pts',(17.8977244277247,-15.6610067321036,
12.));
#184227=CARTESIAN_POINT('Ctrl Pts',(17.8875189181095,-15.6436014971088,
12.));
#184228=CARTESIAN_POINT('Ctrl Pts',(17.8773220648125,-15.6263176459107,
12.));
#184229=CARTESIAN_POINT('Ctrl Pts',(17.8671346981388,-15.6091557129205,
12.));
#184230=CARTESIAN_POINT('Ctrl Pts',(17.8569576598996,-15.5921162378183,
12.));
#184231=CARTESIAN_POINT('Ctrl Pts',(17.8467918036976,-15.5751997657153,
12.));
#184232=CARTESIAN_POINT('Ctrl Pts',(17.8366379952078,-15.5584068472976,
12.));
#184233=CARTESIAN_POINT('Ctrl Pts',(17.8264971124606,-15.5417380389639,
12.));
#184234=CARTESIAN_POINT('Ctrl Pts',(17.8163700461263,-15.5251939029558,
12.));
#184235=CARTESIAN_POINT('Ctrl Pts',(17.8062576997964,-15.5087750074728,
12.));
#184236=CARTESIAN_POINT('Ctrl Pts',(17.7961609903161,-15.4924819268529,
12.));
#184237=CARTESIAN_POINT('Ctrl Pts',(17.7860808481229,-15.4763152417506,
12.));
#184238=CARTESIAN_POINT('Ctrl Pts',(17.7760182175817,-15.4602755393019,
12.));
#184239=CARTESIAN_POINT('Ctrl Pts',(17.765974057326,-15.4443634132865,12.));
#184240=CARTESIAN_POINT('Ctrl Pts',(17.7559493405871,-15.4285794642658,
12.));
#184241=CARTESIAN_POINT('Ctrl Pts',(17.7459450555803,-15.4129242997828,
12.));
#184242=CARTESIAN_POINT('Ctrl Pts',(17.7359622059143,-15.3973985345796,
12.));
#184243=CARTESIAN_POINT('Ctrl Pts',(17.7260018109923,-15.3820027907965,
12.));
#184244=CARTESIAN_POINT('Ctrl Pts',(17.7160649064208,-15.3667376981702,
12.));
#184245=CARTESIAN_POINT('Ctrl Pts',(17.7061525444044,-15.3516038942064,
12.));
#184246=CARTESIAN_POINT('Ctrl Pts',(17.6962657941984,-15.3366020244069,
12.));
#184247=CARTESIAN_POINT('Ctrl Pts',(17.6864057426052,-15.3217327425341,
12.));
#184248=CARTESIAN_POINT('Ctrl Pts',(17.6765734944559,-15.3069967108501,
12.));
#184249=CARTESIAN_POINT('Ctrl Pts',(17.6667701731041,-15.2923946003598,
12.));
#184250=CARTESIAN_POINT('Ctrl Pts',(17.6569969209,-15.2779270910238,12.));
#184251=CARTESIAN_POINT('Ctrl Pts',(17.6472548997329,-15.263594872029,12.));
#184252=CARTESIAN_POINT('Ctrl Pts',(17.637545291637,-15.2493986421091,12.));
#184253=CARTESIAN_POINT('Ctrl Pts',(17.6278692993765,-15.2353391098367,
12.));
#184254=CARTESIAN_POINT('Ctrl Pts',(17.6182281470467,-15.22141699392,12.));
#184255=CARTESIAN_POINT('Ctrl Pts',(17.6086230806497,-15.2076330234686,
12.));
#184256=CARTESIAN_POINT('Ctrl Pts',(17.5990553687595,-15.1939879383268,
12.));
#184257=CARTESIAN_POINT('Ctrl Pts',(17.5895263032592,-15.1804824894605,
12.));
#184258=CARTESIAN_POINT('Ctrl Pts',(17.5800372000539,-15.1671174393136,
12.));
#184259=CARTESIAN_POINT('Ctrl Pts',(17.570589399803,-15.1538935621715,12.));
#184260=CARTESIAN_POINT('Ctrl Pts',(17.5611842686196,-15.1408116444877,
12.));
#184261=CARTESIAN_POINT('Ctrl Pts',(17.5518231989122,-15.127872485314,12.));
#184262=CARTESIAN_POINT('Ctrl Pts',(17.5425076102966,-15.1150768967729,
12.));
#184263=CARTESIAN_POINT('Ctrl Pts',(17.5332389504829,-15.1024257045033,
12.));
#184264=CARTESIAN_POINT('Ctrl Pts',(17.5240186961788,-15.0899197481082,
12.));
#184265=CARTESIAN_POINT('Ctrl Pts',(17.5148483539683,-15.0775598815748,
12.));
#184266=CARTESIAN_POINT('Ctrl Pts',(17.5057294613874,-15.0653469738306,
12.));
#184267=CARTESIAN_POINT('Ctrl Pts',(17.4966635880245,-15.0532819093085,
12.));
#184268=CARTESIAN_POINT('Ctrl Pts',(17.4876523366178,-15.0413655884993,
12.));
#184269=CARTESIAN_POINT('Ctrl Pts',(17.4786973441417,-15.029598928488,12.));
#184270=CARTESIAN_POINT('Ctrl Pts',(17.4698002829357,-15.0179828635086,
12.));
#184271=CARTESIAN_POINT('Ctrl Pts',(17.4609628621418,-15.0065183456921,
12.));
#184272=CARTESIAN_POINT('Ctrl Pts',(17.4521868291004,-14.9952063457778,
12.));
#184273=CARTESIAN_POINT('Ctrl Pts',(17.4434739707773,-14.9840478538358,
12.));
#184274=CARTESIAN_POINT('Ctrl Pts',(17.4348261151396,-14.9730438799452,
12.));
#184275=CARTESIAN_POINT('Ctrl Pts',(17.426245132709,-14.9621954549827,12.));
#184276=CARTESIAN_POINT('Ctrl Pts',(17.4177329382828,-14.9515036315143,
12.));
#184277=CARTESIAN_POINT('Ctrl Pts',(17.4092914926071,-14.940969484645,12.));
#184278=CARTESIAN_POINT('Ctrl Pts',(17.4009228040749,-14.9305941128757,
12.));
#184279=CARTESIAN_POINT('Ctrl Pts',(17.3926289303986,-14.9203786389342,
12.));
#184280=CARTESIAN_POINT('Ctrl Pts',(17.3844119809824,-14.9103242110057,
12.));
#184281=CARTESIAN_POINT('Ctrl Pts',(17.3762741193076,-14.900432003961,12.));
#184282=CARTESIAN_POINT('Ctrl Pts',(17.3682175653235,-14.8907032205788,
12.));
#184283=CARTESIAN_POINT('Ctrl Pts',(17.3602445978161,-14.8811390927423,
12.));
#184284=CARTESIAN_POINT('Ctrl Pts',(17.3523575568645,-14.8717408826956,
12.));
#184285=CARTESIAN_POINT('Ctrl Pts',(17.3445588463474,-14.8625098843417,
12.));
#184286=CARTESIAN_POINT('Ctrl Pts',(17.336850936485,-14.8534474245434,12.));
#184287=CARTESIAN_POINT('Ctrl Pts',(17.3292363662605,-14.8445548643508,
12.));
#184288=CARTESIAN_POINT('Ctrl Pts',(17.3217177462101,-14.8358336004197,
12.));
#184289=CARTESIAN_POINT('Ctrl Pts',(17.3142977632659,-14.8272850675379,
12.));
#184290=CARTESIAN_POINT('Ctrl Pts',(17.3069791853706,-14.8189107410162,
12.));
#184291=CARTESIAN_POINT('Ctrl Pts',(17.299764866148,-14.8107121391035,12.));
#184292=CARTESIAN_POINT('Ctrl Pts',(17.2926577496513,-14.8026908254276,
12.));
#184293=CARTESIAN_POINT('Ctrl Pts',(17.2856608733196,-14.7948484105249,
12.));
#184294=CARTESIAN_POINT('Ctrl Pts',(17.2787773704849,-14.787186553128,12.));
#184295=CARTESIAN_POINT('Ctrl Pts',(17.2720104735194,-14.7797069617804,
12.));
#184296=CARTESIAN_POINT('Ctrl Pts',(17.2653635155319,-14.7724113956731,
12.));
#184297=CARTESIAN_POINT('Ctrl Pts',(17.2588399401465,-14.7653016697591,
12.));
#184298=CARTESIAN_POINT('Ctrl Pts',(17.2524433146837,-14.7583796616617,
12.));
#184299=CARTESIAN_POINT('Ctrl Pts',(17.2461773413288,-14.7516473175124,
12.));
#184300=CARTESIAN_POINT('Ctrl Pts',(17.2400458713565,-14.7451066593792,
12.));
#184301=CARTESIAN_POINT('Ctrl Pts',(17.2340529062076,-14.7387597858117,
12.));
#184302=CARTESIAN_POINT('Ctrl Pts',(17.2282025904314,-14.7326088681163,
12.));
#184303=CARTESIAN_POINT('Ctrl Pts',(17.2224992099667,-14.7266561494282,
12.));
#184304=CARTESIAN_POINT('Ctrl Pts',(17.2169471814256,-14.7209039390327,
12.));
#184305=CARTESIAN_POINT('Ctrl Pts',(17.2115510835989,-14.7153546289339,
12.));
#184306=CARTESIAN_POINT('Ctrl Pts',(17.2063157097315,-14.7100107213586,
12.));
#184307=CARTESIAN_POINT('Ctrl Pts',(17.2012461084268,-14.7048748502663,
12.));
#184308=CARTESIAN_POINT('Ctrl Pts',(17.1963476411694,-14.699949811582,12.));
#184309=CARTESIAN_POINT('Ctrl Pts',(17.1916259308415,-14.6952385361706,
12.));
#184310=CARTESIAN_POINT('Ctrl Pts',(17.1870867909918,-14.6907440526958,
12.));
#184311=CARTESIAN_POINT('Ctrl Pts',(17.182736158472,-14.686469452232,12.));
#184312=CARTESIAN_POINT('Ctrl Pts',(17.1785800350826,-14.6824178576167,
12.));
#184313=CARTESIAN_POINT('Ctrl Pts',(17.1746247499057,-14.6785925615677,
12.));
#184314=CARTESIAN_POINT('Ctrl Pts',(17.1708771619129,-14.6749971333867,
12.));
#184315=CARTESIAN_POINT('Ctrl Pts',(17.167344972302,-14.671635583332,12.));
#184316=CARTESIAN_POINT('Ctrl Pts',(17.1640366762305,-14.6685123374423,
12.));
#184317=CARTESIAN_POINT('Ctrl Pts',(17.1609609517369,-14.6656319165057,
12.));
#184318=CARTESIAN_POINT('Ctrl Pts',(17.1581262646789,-14.6629987285992,
12.));
#184319=CARTESIAN_POINT('Ctrl Pts',(17.1555401986401,-14.6606167169642,
12.));
#184320=CARTESIAN_POINT('Ctrl Pts',(17.1532107762718,-14.6584900555302,
12.));
#184321=CARTESIAN_POINT('Ctrl Pts',(17.1511476869496,-14.6566237952435,
12.));
#184322=CARTESIAN_POINT('Ctrl Pts',(17.1493641837558,-14.655024862281,12.));
#184323=CARTESIAN_POINT('Ctrl Pts',(17.147876394491,-14.6537016966184,12.));
#184324=CARTESIAN_POINT('Ctrl Pts',(17.1466998098673,-14.6526624064978,
12.));
#184325=CARTESIAN_POINT('Ctrl Pts',(17.1458462295271,-14.6519131634508,
12.));
#184326=CARTESIAN_POINT('Ctrl Pts',(17.1454262858043,-14.6515481598068,
12.));
#184327=CARTESIAN_POINT('Ctrl Pts',(17.1452600887037,-14.6514066997196,
12.));
#184328=CARTESIAN_POINT('Ctrl Pts',(17.1452153999142,-14.6513711852843,
12.));
#184329=CARTESIAN_POINT('Ctrl Pts',(17.1452095830632,-14.6513681262571,
12.));
#184330=CARTESIAN_POINT('',(16.7207683102834,-14.2886635873976,12.));
#184331=CARTESIAN_POINT('',(8.17248635976757,-6.98376450772884,12.));
#184332=CARTESIAN_POINT('',(16.6581946899465,-13.5924445804218,12.));
#184333=CARTESIAN_POINT('Origin',(17.0455945664569,-13.9085479427572,12.));
#184334=CARTESIAN_POINT('',(17.4407513054162,-12.572596943457,12.));
#184335=CARTESIAN_POINT('Origin',(6.00167842331873E-13,-4.9889687874677E-13,
12.));
#184336=CARTESIAN_POINT('',(18.1294424696716,-12.4528436808172,12.));
#184337=CARTESIAN_POINT('Origin',(17.846350172984,-12.8649829188862,12.));
#184338=CARTESIAN_POINT('',(18.5896416359912,-12.7689476255363,12.));
#184339=CARTESIAN_POINT('',(9.29482081799561,-6.38447381276812,12.));
#184340=CARTESIAN_POINT('',(22.1787195904339,-13.5685075571671,12.));
#184341=CARTESIAN_POINT('Ctrl Pts',(18.5896416359912,-12.7689476255363,
12.));
#184342=CARTESIAN_POINT('Ctrl Pts',(18.5896460962961,-12.7689524524484,
12.));
#184343=CARTESIAN_POINT('Ctrl Pts',(18.5896919669158,-12.7689864266924,
12.));
#184344=CARTESIAN_POINT('Ctrl Pts',(18.589871621842,-12.7691103481996,12.));
#184345=CARTESIAN_POINT('Ctrl Pts',(18.590332877722,-12.7694215127923,12.));
#184346=CARTESIAN_POINT('Ctrl Pts',(18.5912775137806,-12.7700520897174,
12.));
#184347=CARTESIAN_POINT('Ctrl Pts',(18.5925859134582,-12.7709195951153,
12.));
#184348=CARTESIAN_POINT('Ctrl Pts',(18.5942490615409,-12.7720142287169,
12.));
#184349=CARTESIAN_POINT('Ctrl Pts',(18.5962551167772,-12.7733231262107,
12.));
#184350=CARTESIAN_POINT('Ctrl Pts',(18.5985917525949,-12.7748328937639,
12.));
#184351=CARTESIAN_POINT('Ctrl Pts',(18.6012488486708,-12.7765325225082,
12.));
#184352=CARTESIAN_POINT('Ctrl Pts',(18.6042190183703,-12.7784139605067,
12.));
#184353=CARTESIAN_POINT('Ctrl Pts',(18.6074961535723,-12.7804705387658,
12.));
#184354=CARTESIAN_POINT('Ctrl Pts',(18.611074482622,-12.7826959526924,12.));
#184355=CARTESIAN_POINT('Ctrl Pts',(18.6149475565189,-12.78508316579,12.));
#184356=CARTESIAN_POINT('Ctrl Pts',(18.6191087624752,-12.7876249657834,
12.));
#184357=CARTESIAN_POINT('Ctrl Pts',(18.6235516265575,-12.7903142925234,
12.));
#184358=CARTESIAN_POINT('Ctrl Pts',(18.6282702819371,-12.7931447451556,
12.));
#184359=CARTESIAN_POINT('Ctrl Pts',(18.6332595057005,-12.7961106222251,
12.));
#184360=CARTESIAN_POINT('Ctrl Pts',(18.63851447924,-12.7992066625264,12.));
#184361=CARTESIAN_POINT('Ctrl Pts',(18.6440306327457,-12.8024278770153,
12.));
#184362=CARTESIAN_POINT('Ctrl Pts',(18.6498034438986,-12.805769331162,12.));
#184363=CARTESIAN_POINT('Ctrl Pts',(18.6558284825772,-12.8092261933858,
12.));
#184364=CARTESIAN_POINT('Ctrl Pts',(18.6621014624746,-12.8127937909632,
12.));
#184365=CARTESIAN_POINT('Ctrl Pts',(18.6686182952798,-12.8164676687361,
12.));
#184366=CARTESIAN_POINT('Ctrl Pts',(18.6753751301091,-12.8202436318473,
12.));
#184367=CARTESIAN_POINT('Ctrl Pts',(18.6823683094139,-12.8241176980016,
12.));
#184368=CARTESIAN_POINT('Ctrl Pts',(18.6895943376172,-12.8280860635231,
12.));
#184369=CARTESIAN_POINT('Ctrl Pts',(18.6970498410173,-12.832145059979,12.));
#184370=CARTESIAN_POINT('Ctrl Pts',(18.7047315436296,-12.8362911280362,
12.));
#184371=CARTESIAN_POINT('Ctrl Pts',(18.7126362754446,-12.8405208263432,
12.));
#184372=CARTESIAN_POINT('Ctrl Pts',(18.7207609737701,-12.8448308329494,
12.));
#184373=CARTESIAN_POINT('Ctrl Pts',(18.7291026886552,-12.849217951159,12.));
#184374=CARTESIAN_POINT('Ctrl Pts',(18.7376585820851,-12.8536791086315,
12.));
#184375=CARTESIAN_POINT('Ctrl Pts',(18.7464259171248,-12.8582113455644,
12.));
#184376=CARTESIAN_POINT('Ctrl Pts',(18.7554020493888,-12.8628118054172,
12.));
#184377=CARTESIAN_POINT('Ctrl Pts',(18.7645844169568,-12.8674777239656,
12.));
#184378=CARTESIAN_POINT('Ctrl Pts',(18.7739705329028,-12.8722064211814,
12.));
#184379=CARTESIAN_POINT('Ctrl Pts',(18.7835579840481,-12.8769952998097,
12.));
#184380=CARTESIAN_POINT('Ctrl Pts',(18.7933444285867,-12.8818418427474,
12.));
#184381=CARTESIAN_POINT('Ctrl Pts',(18.8033275941939,-12.8867436109543,
12.));
#184382=CARTESIAN_POINT('Ctrl Pts',(18.8135052757815,-12.8916982409931,
12.));
#184383=CARTESIAN_POINT('Ctrl Pts',(18.8238753319124,-12.8967034410752,
12.));
#184384=CARTESIAN_POINT('Ctrl Pts',(18.834435681259,-12.9017569871738,12.));
#184385=CARTESIAN_POINT('Ctrl Pts',(18.8451842990986,-12.9068567191856,
12.));
#184386=CARTESIAN_POINT('Ctrl Pts',(18.8561192136201,-12.9120005369066,
12.));
#184387=CARTESIAN_POINT('Ctrl Pts',(18.8672385038328,-12.9171863977047,
12.));
#184388=CARTESIAN_POINT('Ctrl Pts',(18.8785402977528,-12.9224123144982,
12.));
#184389=CARTESIAN_POINT('Ctrl Pts',(18.8900227704888,-12.9276763536372,
12.));
#184390=CARTESIAN_POINT('Ctrl Pts',(18.9016841423402,-12.9329766328184,
12.));
#184391=CARTESIAN_POINT('Ctrl Pts',(18.9135226769466,-12.9383113190375,
12.));
#184392=CARTESIAN_POINT('Ctrl Pts',(18.9255366795196,-12.9436786266106,
12.));
#184393=CARTESIAN_POINT('Ctrl Pts',(18.9377244950435,-12.9490768151821,
12.));
#184394=CARTESIAN_POINT('Ctrl Pts',(18.9500845064714,-12.9545041877377,
12.));
#184395=CARTESIAN_POINT('Ctrl Pts',(18.9626151329226,-12.9599590886318,
12.));
#184396=CARTESIAN_POINT('Ctrl Pts',(18.9753148284473,-12.9654399021868,
12.));
#184397=CARTESIAN_POINT('Ctrl Pts',(18.9881820807585,-12.9709450512747,
12.));
#184398=CARTESIAN_POINT('Ctrl Pts',(19.0012154099792,-12.9764729959206,
12.));
#184399=CARTESIAN_POINT('Ctrl Pts',(19.014413367335,-12.9820222318716,12.));
#184400=CARTESIAN_POINT('Ctrl Pts',(19.0277745339908,-12.9875912893003,
12.));
#184401=CARTESIAN_POINT('Ctrl Pts',(19.0412975200398,-12.9931787316514,
12.));
#184402=CARTESIAN_POINT('Ctrl Pts',(19.0549809634354,-12.9987831544502,
12.));
#184403=CARTESIAN_POINT('Ctrl Pts',(19.0688235289437,-13.0044031841382,
12.));
#184404=CARTESIAN_POINT('Ctrl Pts',(19.0828239070484,-13.0100374768788,
12.));
#184405=CARTESIAN_POINT('Ctrl Pts',(19.0969808131228,-13.0156847176097,
12.));
#184406=CARTESIAN_POINT('Ctrl Pts',(19.111292986631,-13.0213436191328,12.));
#184407=CARTESIAN_POINT('Ctrl Pts',(19.1257591903099,-13.0270129211976,
12.));
#184408=CARTESIAN_POINT('Ctrl Pts',(19.1403782093386,-13.0326913895838,
12.));
#184409=CARTESIAN_POINT('Ctrl Pts',(19.155148850523,-13.0383778152068,12.));
#184410=CARTESIAN_POINT('Ctrl Pts',(19.1700699416622,-13.0440710133772,
12.));
#184411=CARTESIAN_POINT('Ctrl Pts',(19.1851403308825,-13.0497698230441,
12.));
#184412=CARTESIAN_POINT('Ctrl Pts',(19.2003588859772,-13.0554731060538,
12.));
#184413=CARTESIAN_POINT('Ctrl Pts',(19.2157244937142,-13.0611797463915,
12.));
#184414=CARTESIAN_POINT('Ctrl Pts',(19.2312360592033,-13.0668886494795,
12.));
#184415=CARTESIAN_POINT('Ctrl Pts',(19.2468925053989,-13.0725987415859,
12.));
#184416=CARTESIAN_POINT('Ctrl Pts',(19.2626927725596,-13.0783089692118,
12.));
#184417=CARTESIAN_POINT('Ctrl Pts',(19.2786358177198,-13.0840182984949,
12.));
#184418=CARTESIAN_POINT('Ctrl Pts',(19.2947206141247,-13.0897257145969,
12.));
#184419=CARTESIAN_POINT('Ctrl Pts',(19.310946150736,-13.0954302211479,12.));
#184420=CARTESIAN_POINT('Ctrl Pts',(19.3273114318269,-13.1011308397591,
12.));
#184421=CARTESIAN_POINT('Ctrl Pts',(19.3438154765395,-13.1068266095186,
12.));
#184422=CARTESIAN_POINT('Ctrl Pts',(19.3604573184515,-13.1125165865022,
12.));
#184423=CARTESIAN_POINT('Ctrl Pts',(19.3772360051091,-13.118199843271,12.));
#184424=CARTESIAN_POINT('Ctrl Pts',(19.3941505976263,-13.1238754684177,
12.));
#184425=CARTESIAN_POINT('Ctrl Pts',(19.4112001703557,-13.1295425661634,
12.));
#184426=CARTESIAN_POINT('Ctrl Pts',(19.4283838105262,-13.1352002559438,
12.));
#184427=CARTESIAN_POINT('Ctrl Pts',(19.4457006178876,-13.1408476720061,
12.));
#184428=CARTESIAN_POINT('Ctrl Pts',(19.4631497043258,-13.1464839629971,
12.));
#184429=CARTESIAN_POINT('Ctrl Pts',(19.4807301935268,-13.1521082915853,
12.));
#184430=CARTESIAN_POINT('Ctrl Pts',(19.4984412207082,-13.1577198341245,
12.));
#184431=CARTESIAN_POINT('Ctrl Pts',(19.5162819323213,-13.1633177803101,
12.));
#184432=CARTESIAN_POINT('Ctrl Pts',(19.5342514857562,-13.168901332843,12.));
#184433=CARTESIAN_POINT('Ctrl Pts',(19.5523490490244,-13.1744697070911,
12.));
#184434=CARTESIAN_POINT('Ctrl Pts',(19.5705738004667,-13.1800221307673,
12.));
#184435=CARTESIAN_POINT('Ctrl Pts',(19.5889249285338,-13.1855578436471,
12.));
#184436=CARTESIAN_POINT('Ctrl Pts',(19.6074016315414,-13.1910760972814,
12.));
#184437=CARTESIAN_POINT('Ctrl Pts',(19.6260031174244,-13.1965761547151,
12.));
#184438=CARTESIAN_POINT('Ctrl Pts',(19.6447286034772,-13.2020572902065,
12.));
#184439=CARTESIAN_POINT('Ctrl Pts',(19.6635773160936,-13.2075187889529,
12.));
#184440=CARTESIAN_POINT('Ctrl Pts',(19.6825484905823,-13.2129599468485,
12.));
#184441=CARTESIAN_POINT('Ctrl Pts',(19.7016413709685,-13.2183800702436,
12.));
#184442=CARTESIAN_POINT('Ctrl Pts',(19.7208552097868,-13.2237784757065,
12.));
#184443=CARTESIAN_POINT('Ctrl Pts',(19.7401892678697,-13.2291544897899,
12.));
#184444=CARTESIAN_POINT('Ctrl Pts',(19.7596428141168,-13.2345074487963,
12.));
#184445=CARTESIAN_POINT('Ctrl Pts',(19.7792151253289,-13.2398366985675,
12.));
#184446=CARTESIAN_POINT('Ctrl Pts',(19.7989054860495,-13.2451415942805,
12.));
#184447=CARTESIAN_POINT('Ctrl Pts',(19.8187131883917,-13.2504215002457,
12.));
#184448=CARTESIAN_POINT('Ctrl Pts',(19.8386375318634,-13.2556757897086,
12.));
#184449=CARTESIAN_POINT('Ctrl Pts',(19.8586778231715,-13.2609038446529,
12.));
#184450=CARTESIAN_POINT('Ctrl Pts',(19.8788333760577,-13.2661050556132,
12.));
#184451=CARTESIAN_POINT('Ctrl Pts',(19.8991035111745,-13.271278821502,12.));
#184452=CARTESIAN_POINT('Ctrl Pts',(19.9194875559422,-13.2764245494357,
12.));
#184453=CARTESIAN_POINT('Ctrl Pts',(19.9399848444019,-13.2815416545663,
12.));
#184454=CARTESIAN_POINT('Ctrl Pts',(19.9605947170586,-13.286629559915,12.));
#184455=CARTESIAN_POINT('Ctrl Pts',(19.981316520717,-13.2916876962094,12.));
#184456=CARTESIAN_POINT('Ctrl Pts',(20.0021496083738,-13.2967155017306,
12.));
#184457=CARTESIAN_POINT('Ctrl Pts',(20.0230933391038,-13.3017124221637,
12.));
#184458=CARTESIAN_POINT('Ctrl Pts',(20.0441470779345,-13.3066779104515,
12.));
#184459=CARTESIAN_POINT('Ctrl Pts',(20.0653101957188,-13.3116114266515,
12.));
#184460=CARTESIAN_POINT('Ctrl Pts',(20.0865820689882,-13.3165124377963,
12.));
#184461=CARTESIAN_POINT('Ctrl Pts',(20.1079620798375,-13.3213804177587,
12.));
#184462=CARTESIAN_POINT('Ctrl Pts',(20.1294496158402,-13.3262148471226,
12.));
#184463=CARTESIAN_POINT('Ctrl Pts',(20.1510440699474,-13.3310152130564,
12.));
#184464=CARTESIAN_POINT('Ctrl Pts',(20.1727448403817,-13.3357810091903,
12.));
#184465=CARTESIAN_POINT('Ctrl Pts',(20.1945513305235,-13.3405117354971,
12.));
#184466=CARTESIAN_POINT('Ctrl Pts',(20.216462948786,-13.3452068981766,12.));
#184467=CARTESIAN_POINT('Ctrl Pts',(20.2384791085359,-13.3498660095386,
12.));
#184468=CARTESIAN_POINT('Ctrl Pts',(20.2605992280122,-13.3544885878889,
12.));
#184469=CARTESIAN_POINT('Ctrl Pts',(20.2828227302339,-13.3590741574195,
12.));
#184470=CARTESIAN_POINT('Ctrl Pts',(20.3051490429048,-13.3636222481016,
12.));
#184471=CARTESIAN_POINT('Ctrl Pts',(20.3275775983029,-13.3681323955826,
12.));
#184472=CARTESIAN_POINT('Ctrl Pts',(20.3501078331814,-13.3726041410867,
12.));
#184473=CARTESIAN_POINT('Ctrl Pts',(20.3727391887184,-13.3770370313188,
12.));
#184474=CARTESIAN_POINT('Ctrl Pts',(20.3954711104502,-13.3814306183719,
12.));
#184475=CARTESIAN_POINT('Ctrl Pts',(20.4183030482002,-13.3857844596387,
12.));
#184476=CARTESIAN_POINT('Ctrl Pts',(20.4412344560008,-13.3900981177255,
12.));
#184477=CARTESIAN_POINT('Ctrl Pts',(20.4642647920038,-13.3943711603739,
12.));
#184478=CARTESIAN_POINT('Ctrl Pts',(20.487393518404,-13.3986031603716,12.));
#184479=CARTESIAN_POINT('Ctrl Pts',(20.5106201013753,-13.4027936954529,
12.));
#184480=CARTESIAN_POINT('Ctrl Pts',(20.5339440109956,-13.4069423482076,
12.));
#184481=CARTESIAN_POINT('Ctrl Pts',(20.5573647211639,-13.4110487059912,
12.));
#184482=CARTESIAN_POINT('Ctrl Pts',(20.5808817095155,-13.4151123608411,
12.));
#184483=CARTESIAN_POINT('Ctrl Pts',(20.6044944573153,-13.4191329093933,
12.));
#184484=CARTESIAN_POINT('Ctrl Pts',(20.6282024494237,-13.4231099528179,
12.));
#184485=CARTESIAN_POINT('Ctrl Pts',(20.6520051742869,-13.4270430967651,
12.));
#184486=CARTESIAN_POINT('Ctrl Pts',(20.6759021239103,-13.4309319513119,
12.));
#184487=CARTESIAN_POINT('Ctrl Pts',(20.6998927938288,-13.4347761309154,
12.));
#184488=CARTESIAN_POINT('Ctrl Pts',(20.7239766830675,-13.4385752543663,
12.));
#184489=CARTESIAN_POINT('Ctrl Pts',(20.7481532941013,-13.4423289447561,
12.));
#184490=CARTESIAN_POINT('Ctrl Pts',(20.7724221327608,-13.4460368293688,
12.));
#184491=CARTESIAN_POINT('Ctrl Pts',(20.7967827081227,-13.4496985395637,
12.));
#184492=CARTESIAN_POINT('Ctrl Pts',(20.821234532398,-13.4533137106667,12.));
#184493=CARTESIAN_POINT('Ctrl Pts',(20.8457771208082,-13.4568819818631,
12.));
#184494=CARTESIAN_POINT('Ctrl Pts',(20.8704099914641,-13.4604029960983,
12.));
#184495=CARTESIAN_POINT('Ctrl Pts',(20.8951326652158,-13.4638763999725,
12.));
#184496=CARTESIAN_POINT('Ctrl Pts',(20.9199446657584,-13.4673018437718,
12.));
#184497=CARTESIAN_POINT('Ctrl Pts',(20.9448455197557,-13.4706789815166,
12.));
#184498=CARTESIAN_POINT('Ctrl Pts',(20.9698347569476,-13.4740074710087,
12.));
#184499=CARTESIAN_POINT('Ctrl Pts',(20.9949119102592,-13.4772869738879,
12.));
#184500=CARTESIAN_POINT('Ctrl Pts',(21.0200765158885,-13.4805171556822,
12.));
#184501=CARTESIAN_POINT('Ctrl Pts',(21.0453281134247,-13.4836976858912,
12.));
#184502=CARTESIAN_POINT('Ctrl Pts',(21.0706662455202,-13.4868282377192,
12.));
#184503=CARTESIAN_POINT('Ctrl Pts',(21.0960904575048,-13.4899084877718,
12.));
#184504=CARTESIAN_POINT('Ctrl Pts',(21.1216002970209,-13.4929381157778,
12.));
#184505=CARTESIAN_POINT('Ctrl Pts',(21.1471953136209,-13.4959168042934,
12.));
#184506=CARTESIAN_POINT('Ctrl Pts',(21.1728750584173,-13.4988442384491,
12.));
#184507=CARTESIAN_POINT('Ctrl Pts',(21.1986390835825,-13.5017201056088,
12.));
#184508=CARTESIAN_POINT('Ctrl Pts',(21.224486942933,-13.5045440957404,12.));
#184509=CARTESIAN_POINT('Ctrl Pts',(21.2504181927429,-13.5073159019454,
12.));
#184510=CARTESIAN_POINT('Ctrl Pts',(21.2764323924442,-13.5100352209207,
12.));
#184511=CARTESIAN_POINT('Ctrl Pts',(21.3025291054236,-13.5127017534972,
12.));
#184512=CARTESIAN_POINT('Ctrl Pts',(21.328707899634,-13.5153152050554,12.));
#184513=CARTESIAN_POINT('Ctrl Pts',(21.3549683486219,-13.5178752862461,
12.));
#184514=CARTESIAN_POINT('Ctrl Pts',(21.3813100304967,-13.5203817122497,
12.));
#184515=CARTESIAN_POINT('Ctrl Pts',(21.4077325259318,-13.5228342013508,
12.));
#184516=CARTESIAN_POINT('Ctrl Pts',(21.4342354165254,-13.5252324737795,
12.));
#184517=CARTESIAN_POINT('Ctrl Pts',(21.4608182828695,-13.5275762503553,
12.));
#184518=CARTESIAN_POINT('Ctrl Pts',(21.487480703047,-13.5298652514357,12.));
#184519=CARTESIAN_POINT('Ctrl Pts',(21.5142222501671,-13.5320991952145,
12.));
#184520=CARTESIAN_POINT('Ctrl Pts',(21.5410424932511,-13.5342777983225,
12.));
#184521=CARTESIAN_POINT('Ctrl Pts',(21.5679410019011,-13.5364007790292,
12.));
#184522=CARTESIAN_POINT('Ctrl Pts',(21.5949173499022,-13.5384678597206,
12.));
#184523=CARTESIAN_POINT('Ctrl Pts',(21.6219711193951,-13.5404787697798,
12.));
#184524=CARTESIAN_POINT('Ctrl Pts',(21.6491019044647,-13.5424332480698,
12.));
#184525=CARTESIAN_POINT('Ctrl Pts',(21.676309315769,-13.5443310461516,12.));
#184526=CARTESIAN_POINT('Ctrl Pts',(21.7035929822939,-13.546171929503,12.));
#184527=CARTESIAN_POINT('Ctrl Pts',(21.730952541226,-13.5479556704457,12.));
#184528=CARTESIAN_POINT('Ctrl Pts',(21.7583876294532,-13.5496820422186,
12.));
#184529=CARTESIAN_POINT('Ctrl Pts',(21.7858978745848,-13.5513508127232,
12.));
#184530=CARTESIAN_POINT('Ctrl Pts',(21.8134828857963,-13.5529617381569,
12.));
#184531=CARTESIAN_POINT('Ctrl Pts',(21.841142245609,-13.5545145573048,12.));
#184532=CARTESIAN_POINT('Ctrl Pts',(21.8688754989401,-13.5560089839426,
12.));
#184533=CARTESIAN_POINT('Ctrl Pts',(21.8966821688876,-13.5574447178485,
12.));
#184534=CARTESIAN_POINT('Ctrl Pts',(21.9245617765827,-13.5588214586672,
12.));
#184535=CARTESIAN_POINT('Ctrl Pts',(21.9525138592862,-13.5601389185315,
12.));
#184536=CARTESIAN_POINT('Ctrl Pts',(21.9805379899192,-13.5613968357589,
12.));
#184537=CARTESIAN_POINT('Ctrl Pts',(22.0086337943431,-13.5625949868313,
12.));
#184538=CARTESIAN_POINT('Ctrl Pts',(22.0368009736227,-13.5637332022393,
12.));
#184539=CARTESIAN_POINT('Ctrl Pts',(22.0650393089492,-13.5648113688895,
12.));
#184540=CARTESIAN_POINT('Ctrl Pts',(22.0933486464442,-13.5658294169106,
12.));
#184541=CARTESIAN_POINT('Ctrl Pts',(22.1217288871823,-13.5667873105179,
12.));
#184542=CARTESIAN_POINT('Ctrl Pts',(22.1444897575076,-13.5675054918922,
12.));
#184543=CARTESIAN_POINT('Ctrl Pts',(22.1615922804939,-13.5680170531724,
12.));
#184544=CARTESIAN_POINT('Ctrl Pts',(22.1730081264583,-13.5683460612913,
12.));
#184545=CARTESIAN_POINT('Ctrl Pts',(22.1787195904339,-13.5685075571671,
12.));
#184546=CARTESIAN_POINT('',(22.8400320311648,-12.4230808101438,12.));
#184547=CARTESIAN_POINT('Origin',(0.,0.,12.));
#184548=CARTESIAN_POINT('',(20.353053841303,-9.71462809124917,12.));
#184549=CARTESIAN_POINT('Ctrl Pts',(22.8400320311648,-12.4230808101438,
12.));
#184550=CARTESIAN_POINT('Ctrl Pts',(22.8370364396497,-12.4182152851867,
12.));
#184551=CARTESIAN_POINT('Ctrl Pts',(22.8310435872852,-12.4084933766366,
12.));
#184552=CARTESIAN_POINT('Ctrl Pts',(22.8220493007353,-12.393937937903,12.));
#184553=CARTESIAN_POINT('Ctrl Pts',(22.8100469022632,-12.3745855366772,
12.));
#184554=CARTESIAN_POINT('Ctrl Pts',(22.7950272216959,-12.3504864740361,
12.));
#184555=CARTESIAN_POINT('Ctrl Pts',(22.7799908974947,-12.3264788926108,
12.));
#184556=CARTESIAN_POINT('Ctrl Pts',(22.7649380101154,-12.3025628601812,
12.));
#184557=CARTESIAN_POINT('Ctrl Pts',(22.7498686970096,-12.2787384750747,
12.));
#184558=CARTESIAN_POINT('Ctrl Pts',(22.7347831655251,-12.2550058702389,
12.));
#184559=CARTESIAN_POINT('Ctrl Pts',(22.7196817119299,-12.2313652198047,
12.));
#184560=CARTESIAN_POINT('Ctrl Pts',(22.7045647168659,-12.2078167360267,
12.));
#184561=CARTESIAN_POINT('Ctrl Pts',(22.6894326204959,-12.1843606579246,
12.));
#184562=CARTESIAN_POINT('Ctrl Pts',(22.6742859034891,-12.1609972423089,
12.));
#184563=CARTESIAN_POINT('Ctrl Pts',(22.6591250653942,-12.1377267537141,
12.));
#184564=CARTESIAN_POINT('Ctrl Pts',(22.6439506046611,-12.1145494550384,
12.));
#184565=CARTESIAN_POINT('Ctrl Pts',(22.628762996708,-12.0914655972828,12.));
#184566=CARTESIAN_POINT('Ctrl Pts',(22.613562676493,-12.0684754113869,12.));
#184567=CARTESIAN_POINT('Ctrl Pts',(22.5983500505675,-12.0455791139135,
12.));
#184568=CARTESIAN_POINT('Ctrl Pts',(22.5831255061306,-12.0227769113132,
12.));
#184569=CARTESIAN_POINT('Ctrl Pts',(22.5678894211194,-12.0000690046697,
12.));
#184570=CARTESIAN_POINT('Ctrl Pts',(22.5526421741159,-11.9774555943496,
12.));
#184571=CARTESIAN_POINT('Ctrl Pts',(22.5373841537299,-11.9549368843996,
12.));
#184572=CARTESIAN_POINT('Ctrl Pts',(22.5221157697869,-11.9325130877801,
12.));
#184573=CARTESIAN_POINT('Ctrl Pts',(22.5068374513958,-11.9101844254555,
12.));
#184574=CARTESIAN_POINT('Ctrl Pts',(22.4915496418472,-11.8879511239941,
12.));
#184575=CARTESIAN_POINT('Ctrl Pts',(22.4762527946694,-11.8658134137018,
12.));
#184576=CARTESIAN_POINT('Ctrl Pts',(22.4609473690469,-11.8437715264487,
12.));
#184577=CARTESIAN_POINT('Ctrl Pts',(22.4456338258738,-11.8218256937889,
12.));
#184578=CARTESIAN_POINT('Ctrl Pts',(22.4303126226468,-11.7999761445175,
12.));
#184579=CARTESIAN_POINT('Ctrl Pts',(22.4149842125018,-11.7782231042041,
12.));
#184580=CARTESIAN_POINT('Ctrl Pts',(22.39964904692,-11.7565667964765,12.));
#184581=CARTESIAN_POINT('Ctrl Pts',(22.3843075773905,-11.7350074437961,
12.));
#184582=CARTESIAN_POINT('Ctrl Pts',(22.3689602575492,-11.7135452684532,
12.));
#184583=CARTESIAN_POINT('Ctrl Pts',(22.3536075450028,-11.6921804934056,
12.));
#184584=CARTESIAN_POINT('Ctrl Pts',(22.3382499035618,-11.6709133432986,
12.));
#184585=CARTESIAN_POINT('Ctrl Pts',(22.3228878043976,-11.6497440449858,
12.));
#184586=CARTESIAN_POINT('Ctrl Pts',(22.3075217249049,-11.6286728270011,
12.));
#184587=CARTESIAN_POINT('Ctrl Pts',(22.2921521480357,-11.6076999192359,
12.));
#184588=CARTESIAN_POINT('Ctrl Pts',(22.2767795614349,-11.5868255525189,
12.));
#184589=CARTESIAN_POINT('Ctrl Pts',(22.2614044566898,-11.5660499582403,
12.));
#184590=CARTESIAN_POINT('Ctrl Pts',(22.2460273284653,-11.545373367912,12.));
#184591=CARTESIAN_POINT('Ctrl Pts',(22.2306486738899,-11.5247960128476,
12.));
#184592=CARTESIAN_POINT('Ctrl Pts',(22.215268993102,-11.504318124424,12.));
#184593=CARTESIAN_POINT('Ctrl Pts',(22.1998887896435,-11.4839399342589,
12.));
#184594=CARTESIAN_POINT('Ctrl Pts',(22.1845085709169,-11.463661674411,12.));
#184595=CARTESIAN_POINT('Ctrl Pts',(22.1691288486096,-11.443483577557,12.));
#184596=CARTESIAN_POINT('Ctrl Pts',(22.1537501391486,-11.4234058771742,
12.));
#184597=CARTESIAN_POINT('Ctrl Pts',(22.1383729640963,-11.4034288076909,
12.));
#184598=CARTESIAN_POINT('Ctrl Pts',(22.1229978500185,-11.3835526044256,
12.));
#184599=CARTESIAN_POINT('Ctrl Pts',(22.1076253283978,-11.3637775035367,
12.));
#184600=CARTESIAN_POINT('Ctrl Pts',(22.0922559355293,-11.3441037419553,
12.));
#184601=CARTESIAN_POINT('Ctrl Pts',(22.0768902124267,-11.3245315573168,
12.));
#184602=CARTESIAN_POINT('Ctrl Pts',(22.0615287047179,-11.3050611878771,
12.));
#184603=CARTESIAN_POINT('Ctrl Pts',(22.046171962566,-11.2856928724374,12.));
#184604=CARTESIAN_POINT('Ctrl Pts',(22.0308205408351,-11.2664268504207,
12.));
#184605=CARTESIAN_POINT('Ctrl Pts',(22.0154749992364,-11.2472633619276,
12.));
#184606=CARTESIAN_POINT('Ctrl Pts',(22.0001359024839,-11.2282026477897,
12.));
#184607=CARTESIAN_POINT('Ctrl Pts',(21.9848038204439,-11.2092449496125,
12.));
#184608=CARTESIAN_POINT('Ctrl Pts',(21.9694793282913,-11.190390509811,12.));
#184609=CARTESIAN_POINT('Ctrl Pts',(21.9541630066504,-11.1716395716375,
12.));
#184610=CARTESIAN_POINT('Ctrl Pts',(21.9388554416437,-11.1529923792002,
12.));
#184611=CARTESIAN_POINT('Ctrl Pts',(21.9235572249518,-11.134449177474,12.));
#184612=CARTESIAN_POINT('Ctrl Pts',(21.9082689538687,-11.1160102123024,
12.));
#184613=CARTESIAN_POINT('Ctrl Pts',(21.8929912313608,-11.0976757303944,
12.));
#184614=CARTESIAN_POINT('Ctrl Pts',(21.8777246661191,-11.0794459793058,
12.));
#184615=CARTESIAN_POINT('Ctrl Pts',(21.8624698726319,-11.0613212074364,
12.));
#184616=CARTESIAN_POINT('Ctrl Pts',(21.8472274713103,-11.0433016640808,
12.));
#184617=CARTESIAN_POINT('Ctrl Pts',(21.8319980886033,-11.0253875994598,
12.));
#184618=CARTESIAN_POINT('Ctrl Pts',(21.8167823571168,-11.0075792647477,
12.));
#184619=CARTESIAN_POINT('Ctrl Pts',(21.8015809157302,-10.9898769120913,
12.));
#184620=CARTESIAN_POINT('Ctrl Pts',(21.7863944097143,-10.9722807946157,
12.));
#184621=CARTESIAN_POINT('Ctrl Pts',(21.7712234908468,-10.9547911664457,
12.));
#184622=CARTESIAN_POINT('Ctrl Pts',(21.7560688175252,-10.9374082827446,
12.));
#184623=CARTESIAN_POINT('Ctrl Pts',(21.74093105488,-10.9201323997386,12.));
#184624=CARTESIAN_POINT('Ctrl Pts',(21.7258108748874,-10.9029637747341,
12.));
#184625=CARTESIAN_POINT('Ctrl Pts',(21.7107089564822,-10.8859026661292,
12.));
#184626=CARTESIAN_POINT('Ctrl Pts',(21.6956259856667,-10.8689493334093,
12.));
#184627=CARTESIAN_POINT('Ctrl Pts',(21.6805626556461,-10.8521040371832,
12.));
#184628=CARTESIAN_POINT('Ctrl Pts',(21.6655196669727,-10.835367039227,12.));
#184629=CARTESIAN_POINT('Ctrl Pts',(21.6504977276864,-10.8187386025135,
12.));
#184630=CARTESIAN_POINT('Ctrl Pts',(21.6354975534557,-10.802218991237,12.));
#184631=CARTESIAN_POINT('Ctrl Pts',(21.6205198677176,-10.7858084708262,
12.));
#184632=CARTESIAN_POINT('Ctrl Pts',(21.6055654018179,-10.7695073079554,
12.));
#184633=CARTESIAN_POINT('Ctrl Pts',(21.5906348951745,-10.7533157705943,
12.));
#184634=CARTESIAN_POINT('Ctrl Pts',(21.5757290954372,-10.7372341280468,
12.));
#184635=CARTESIAN_POINT('Ctrl Pts',(21.5608487586467,-10.7212626509816,
12.));
#184636=CARTESIAN_POINT('Ctrl Pts',(21.5459946493955,-10.7054016114571,
12.));
#184637=CARTESIAN_POINT('Ctrl Pts',(21.531167540981,-10.689651282929,12.));
#184638=CARTESIAN_POINT('Ctrl Pts',(21.5163682155805,-10.6740119402835,
12.));
#184639=CARTESIAN_POINT('Ctrl Pts',(21.5015974644454,-10.6584838598941,
12.));
#184640=CARTESIAN_POINT('Ctrl Pts',(21.4868560880893,-10.6430673196609,
12.));
#184641=CARTESIAN_POINT('Ctrl Pts',(21.4721448964766,-10.6277625990457,
12.));
#184642=CARTESIAN_POINT('Ctrl Pts',(21.4574647092093,-10.612569979096,12.));
#184643=CARTESIAN_POINT('Ctrl Pts',(21.4428163557137,-10.597489742462,12.));
#184644=CARTESIAN_POINT('Ctrl Pts',(21.4282006754624,-10.582522173457,12.));
#184645=CARTESIAN_POINT('Ctrl Pts',(21.4136185181974,-10.5676675581106,
12.));
#184646=CARTESIAN_POINT('Ctrl Pts',(21.3990707441495,-10.5529261842107,
12.));
#184647=CARTESIAN_POINT('Ctrl Pts',(21.3845582242604,-10.5382983413422,
12.));
#184648=CARTESIAN_POINT('Ctrl Pts',(21.3700818403942,-10.523784320906,12.));
#184649=CARTESIAN_POINT('Ctrl Pts',(21.3556424855822,-10.509384416169,12.));
#184650=CARTESIAN_POINT('Ctrl Pts',(21.3412410642912,-10.4950989223341,
12.));
#184651=CARTESIAN_POINT('Ctrl Pts',(21.3268784926823,-10.4809281365933,
12.));
#184652=CARTESIAN_POINT('Ctrl Pts',(21.312555698873,-10.4668723581768,12.));
#184653=CARTESIAN_POINT('Ctrl Pts',(21.2982736231924,-10.452931888387,12.));
#184654=CARTESIAN_POINT('Ctrl Pts',(21.2840332184471,-10.4391070306385,
12.));
#184655=CARTESIAN_POINT('Ctrl Pts',(21.2698354502391,-10.4253980905394,
12.));
#184656=CARTESIAN_POINT('Ctrl Pts',(21.2556812972741,-10.4118053759584,
12.));
#184657=CARTESIAN_POINT('Ctrl Pts',(21.2415717516713,-10.3983291970846,
12.));
#184658=CARTESIAN_POINT('Ctrl Pts',(21.2275078192708,-10.384969866479,12.));
#184659=CARTESIAN_POINT('Ctrl Pts',(21.2134905199359,-10.3717276991137,
12.));
#184660=CARTESIAN_POINT('Ctrl Pts',(21.1995208879205,-10.3586030124595,
12.));
#184661=CARTESIAN_POINT('Ctrl Pts',(21.1855999722427,-10.3455961265706,
12.));
#184662=CARTESIAN_POINT('Ctrl Pts',(21.1717288370512,-10.3327073641574,
12.));
#184663=CARTESIAN_POINT('Ctrl Pts',(21.1579085619959,-10.3199370506541,
12.));
#184664=CARTESIAN_POINT('Ctrl Pts',(21.1441402425831,-10.307285514268,12.));
#184665=CARTESIAN_POINT('Ctrl Pts',(21.130424990599,-10.2947530860714,12.));
#184666=CARTESIAN_POINT('Ctrl Pts',(21.1167639345623,-10.2823401001067,
12.));
#184667=CARTESIAN_POINT('Ctrl Pts',(21.1031582201625,-10.2700468934743,
12.));
#184668=CARTESIAN_POINT('Ctrl Pts',(21.0896090107066,-10.2578738064183,
12.));
#184669=CARTESIAN_POINT('Ctrl Pts',(21.0761174875448,-10.2458211823915,
12.));
#184670=CARTESIAN_POINT('Ctrl Pts',(21.0626848505665,-10.233889368157,12.));
#184671=CARTESIAN_POINT('Ctrl Pts',(21.0493123187483,-10.2220787139157,
12.));
#184672=CARTESIAN_POINT('Ctrl Pts',(21.0360011306814,-10.2103895734124,
12.));
#184673=CARTESIAN_POINT('Ctrl Pts',(21.0227525451107,-10.1988223040425,
12.));
#184674=CARTESIAN_POINT('Ctrl Pts',(21.0095678414486,-10.1873772669358,
12.));
#184675=CARTESIAN_POINT('Ctrl Pts',(20.9964483203685,-10.1760548270765,
12.));
#184676=CARTESIAN_POINT('Ctrl Pts',(20.9833953044736,-10.1648553534567,
12.));
#184677=CARTESIAN_POINT('Ctrl Pts',(20.970410138937,-10.1537792192065,12.));
#184678=CARTESIAN_POINT('Ctrl Pts',(20.9574941921591,-10.1428268017257,
12.));
#184679=CARTESIAN_POINT('Ctrl Pts',(20.944648856393,-10.1319984827909,12.));
#184680=CARTESIAN_POINT('Ctrl Pts',(20.931875548473,-10.1212946487057,12.));
#184681=CARTESIAN_POINT('Ctrl Pts',(20.9191757106266,-10.1107156904836,
12.));
#184682=CARTESIAN_POINT('Ctrl Pts',(20.9065508112556,-10.1002620040076,
12.));
#184683=CARTESIAN_POINT('Ctrl Pts',(20.8940023457371,-10.0899339901916,
12.));
#184684=CARTESIAN_POINT('Ctrl Pts',(20.8815318371844,-10.0797320551154,
12.));
#184685=CARTESIAN_POINT('Ctrl Pts',(20.8691408373705,-10.0696566102219,
12.));
#184686=CARTESIAN_POINT('Ctrl Pts',(20.856830927732,-10.0597080725375,12.));
#184687=CARTESIAN_POINT('Ctrl Pts',(20.8446037203402,-10.0498868648733,
12.));
#184688=CARTESIAN_POINT('Ctrl Pts',(20.8324608588906,-10.0401934160234,
12.));
#184689=CARTESIAN_POINT('Ctrl Pts',(20.8204040196599,-10.0306281609435,
12.));
#184690=CARTESIAN_POINT('Ctrl Pts',(20.8084349126885,-10.0211915410095,
12.));
#184691=CARTESIAN_POINT('Ctrl Pts',(20.7965552829907,-10.0118840042786,
12.));
#184692=CARTESIAN_POINT('Ctrl Pts',(20.7847669117568,-10.0027060057389,
12.));
#184693=CARTESIAN_POINT('Ctrl Pts',(20.7730716175417,-9.99365800754638,
12.));
#184694=CARTESIAN_POINT('Ctrl Pts',(20.7614712574989,-9.98474047926846,
12.));
#184695=CARTESIAN_POINT('Ctrl Pts',(20.7499677289625,-9.97595389823461,
12.));
#184696=CARTESIAN_POINT('Ctrl Pts',(20.7385629709795,-9.96729874986199,
12.));
#184697=CARTESIAN_POINT('Ctrl Pts',(20.7272589658752,-9.95877552798403,
12.));
#184698=CARTESIAN_POINT('Ctrl Pts',(20.716057740758,-9.95038473514962,12.));
#184699=CARTESIAN_POINT('Ctrl Pts',(20.7049613692237,-9.94212688298251,
12.));
#184700=CARTESIAN_POINT('Ctrl Pts',(20.6939719732485,-9.93400249259737,
12.));
#184701=CARTESIAN_POINT('Ctrl Pts',(20.6830917250255,-9.92601209498751,
12.));
#184702=CARTESIAN_POINT('Ctrl Pts',(20.6723228488261,-9.91815623141285,
12.));
#184703=CARTESIAN_POINT('Ctrl Pts',(20.6616676228315,-9.91043545377005,
12.));
#184704=CARTESIAN_POINT('Ctrl Pts',(20.6511283817415,-9.90285032516696,
12.));
#184705=CARTESIAN_POINT('Ctrl Pts',(20.6407075193977,-9.89540142049124,
12.));
#184706=CARTESIAN_POINT('Ctrl Pts',(20.6304074914086,-9.88808932697305,
12.));
#184707=CARTESIAN_POINT('Ctrl Pts',(20.6202308177472,-9.88091464472669,
12.));
#184708=CARTESIAN_POINT('Ctrl Pts',(20.6101800854491,-9.87387798732944,
12.));
#184709=CARTESIAN_POINT('Ctrl Pts',(20.6002579513696,-9.86697998242612,
12.));
#184710=CARTESIAN_POINT('Ctrl Pts',(20.5904671449754,-9.8602212723275,12.));
#184711=CARTESIAN_POINT('Ctrl Pts',(20.580810471002,-9.85360251457004,12.));
#184712=CARTESIAN_POINT('Ctrl Pts',(20.5712908125145,-9.84712438256308,
12.));
#184713=CARTESIAN_POINT('Ctrl Pts',(20.5619111362406,-9.84078756677589,
12.));
#184714=CARTESIAN_POINT('Ctrl Pts',(20.5526744976461,-9.83459277585321,
12.));
#184715=CARTESIAN_POINT('Ctrl Pts',(20.5435840460717,-9.82854073773858,
12.));
#184716=CARTESIAN_POINT('Ctrl Pts',(20.534643029951,-9.82263220080328,12.));
#184717=CARTESIAN_POINT('Ctrl Pts',(20.5258548000625,-9.81686793455918,
12.));
#184718=CARTESIAN_POINT('Ctrl Pts',(20.5172228122839,-9.81124873025278,
12.));
#184719=CARTESIAN_POINT('Ctrl Pts',(20.5087506310507,-9.80577540161103,
12.));
#184720=CARTESIAN_POINT('Ctrl Pts',(20.500441931211,-9.80044878520968,12.));
#184721=CARTESIAN_POINT('Ctrl Pts',(20.4923005087945,-9.79526974288344,
12.));
#184722=CARTESIAN_POINT('Ctrl Pts',(20.4843302955329,-9.7902391649866,12.));
#184723=CARTESIAN_POINT('Ctrl Pts',(20.4765353711585,-9.78535797314162,
12.));
#184724=CARTESIAN_POINT('Ctrl Pts',(20.4689199790668,-9.78062712373313,
12.));
#184725=CARTESIAN_POINT('Ctrl Pts',(20.4614885274973,-9.77604760815523,
12.));
#184726=CARTESIAN_POINT('Ctrl Pts',(20.4542455817527,-9.7716204510407,12.));
#184727=CARTESIAN_POINT('Ctrl Pts',(20.447195862298,-9.76734670980897,12.));
#184728=CARTESIAN_POINT('Ctrl Pts',(20.4403442329401,-9.76322747195502,
12.));
#184729=CARTESIAN_POINT('Ctrl Pts',(20.4336957355474,-9.7592638628993,12.));
#184730=CARTESIAN_POINT('Ctrl Pts',(20.4272556476629,-9.75545705902416,
12.));
#184731=CARTESIAN_POINT('Ctrl Pts',(20.4210295275818,-9.75180829786433,
12.));
#184732=CARTESIAN_POINT('Ctrl Pts',(20.4150232777393,-9.74831889242175,
12.));
#184733=CARTESIAN_POINT('Ctrl Pts',(20.4092430879861,-9.74499021838537,
12.));
#184734=CARTESIAN_POINT('Ctrl Pts',(20.4036953576549,-9.74182369656273,
12.));
#184735=CARTESIAN_POINT('Ctrl Pts',(20.3983866213331,-9.73882077613206,
12.));
#184736=CARTESIAN_POINT('Ctrl Pts',(20.3933234845646,-9.7359829201425,12.));
#184737=CARTESIAN_POINT('Ctrl Pts',(20.3885129129912,-9.73331167102812,
12.));
#184738=CARTESIAN_POINT('Ctrl Pts',(20.3839624556742,-9.73080870123726,
12.));
#184739=CARTESIAN_POINT('Ctrl Pts',(20.3796805893304,-9.72847589116533,
12.));
#184740=CARTESIAN_POINT('Ctrl Pts',(20.3756766651952,-9.72631531732871,
12.));
#184741=CARTESIAN_POINT('Ctrl Pts',(20.371960235676,-9.72432910043193,12.));
#184742=CARTESIAN_POINT('Ctrl Pts',(20.3685406190576,-9.72251930722504,
12.));
#184743=CARTESIAN_POINT('Ctrl Pts',(20.3654261611055,-9.72088778381102,
12.));
#184744=CARTESIAN_POINT('Ctrl Pts',(20.362625691398,-9.71943648548115,12.));
#184745=CARTESIAN_POINT('Ctrl Pts',(20.3601498764344,-9.71816778327999,
12.));
#184746=CARTESIAN_POINT('Ctrl Pts',(20.3580133103357,-9.71708493723062,
12.));
#184747=CARTESIAN_POINT('Ctrl Pts',(20.3562337557875,-9.71619192554147,
12.));
#184748=CARTESIAN_POINT('Ctrl Pts',(20.3548282742361,-9.71549257088175,
12.));
#184749=CARTESIAN_POINT('Ctrl Pts',(20.3538098605706,-9.71498978052101,
12.));
#184750=CARTESIAN_POINT('Ctrl Pts',(20.3533097561886,-9.71474590350792,
12.));
#184751=CARTESIAN_POINT('Ctrl Pts',(20.3531126095522,-9.71465227853122,
12.));
#184752=CARTESIAN_POINT('Ctrl Pts',(20.353060251684,-9.71462954053074,12.));
#184753=CARTESIAN_POINT('Ctrl Pts',(20.353053841303,-9.71462809124917,12.));
#184754=CARTESIAN_POINT('',(19.84920021178,-9.47413589477549,12.));
#184755=CARTESIAN_POINT('',(9.70154690100589,-4.63060338698782,12.));
#184756=CARTESIAN_POINT('',(19.6085639972844,-8.81783521984851,12.));
#184757=CARTESIAN_POINT('Origin',(20.0645771135003,-9.02290115519382,12.));
#184758=CARTESIAN_POINT('',(20.1004996511507,-7.63019749246979,12.));
#184759=CARTESIAN_POINT('Origin',(7.08841632778409E-13,-3.26562511982935E-13,
12.));
#184760=CARTESIAN_POINT('',(20.7347298079577,-7.33627833380047,12.));
#184761=CARTESIAN_POINT('Origin',(20.56795313141,-7.80764394578304,12.));
#184762=CARTESIAN_POINT('',(21.2610617890679,-7.52250298901266,12.));
#184763=CARTESIAN_POINT('',(10.6305308945339,-3.76125149450632,12.));
#184764=CARTESIAN_POINT('',(24.9347862158358,-7.36589684767345,12.));
#184765=CARTESIAN_POINT('Ctrl Pts',(21.2610617890679,-7.52250298901266,
12.));
#184766=CARTESIAN_POINT('Ctrl Pts',(21.2610673466883,-7.52250649703992,
12.));
#184767=CARTESIAN_POINT('Ctrl Pts',(21.261120447486,-7.52252744144958,12.));
#184768=CARTESIAN_POINT('Ctrl Pts',(21.2613260540651,-7.52260064231736,
12.));
#184769=CARTESIAN_POINT('Ctrl Pts',(21.261852128355,-7.52278182242728,12.));
#184770=CARTESIAN_POINT('Ctrl Pts',(21.262927782038,-7.52314642316203,12.));
#184771=CARTESIAN_POINT('Ctrl Pts',(21.2644161259965,-7.52364573027521,
12.));
#184772=CARTESIAN_POINT('Ctrl Pts',(21.266305915706,-7.52427261074264,12.));
#184773=CARTESIAN_POINT('Ctrl Pts',(21.2685823838672,-7.52501770333522,
12.));
#184774=CARTESIAN_POINT('Ctrl Pts',(21.2712301573465,-7.52587126095544,
12.));
#184775=CARTESIAN_POINT('Ctrl Pts',(21.2742366113578,-7.52682526918561,
12.));
#184776=CARTESIAN_POINT('Ctrl Pts',(21.2775925269651,-7.52787386225344,
12.));
#184777=CARTESIAN_POINT('Ctrl Pts',(21.2812902781143,-7.52901217930407,
12.));
#184778=CARTESIAN_POINT('Ctrl Pts',(21.2853226580658,-7.53023562438221,
12.));
#184779=CARTESIAN_POINT('Ctrl Pts',(21.2896816163843,-7.53153906987847,
12.));
#184780=CARTESIAN_POINT('Ctrl Pts',(21.2943588989331,-7.53291726078527,
12.));
#184781=CARTESIAN_POINT('Ctrl Pts',(21.2993464250717,-7.53436505309949,
12.));
#184782=CARTESIAN_POINT('Ctrl Pts',(21.3046368712156,-7.53587778251743,
12.));
#184783=CARTESIAN_POINT('Ctrl Pts',(21.3102237167729,-7.5374512936462,12.));
#184784=CARTESIAN_POINT('Ctrl Pts',(21.3161009456256,-7.53908175169899,
12.));
#184785=CARTESIAN_POINT('Ctrl Pts',(21.3222628524165,-7.5407655203828,12.));
#184786=CARTESIAN_POINT('Ctrl Pts',(21.328703791771,-7.54249900377032,12.));
#184787=CARTESIAN_POINT('Ctrl Pts',(21.3354182340149,-7.54427868151269,
12.));
#184788=CARTESIAN_POINT('Ctrl Pts',(21.3424008295038,-7.54610114948351,
12.));
#184789=CARTESIAN_POINT('Ctrl Pts',(21.349646476153,-7.54796316246327,12.));
#184790=CARTESIAN_POINT('Ctrl Pts',(21.3571503685853,-7.54986166521307,
12.));
#184791=CARTESIAN_POINT('Ctrl Pts',(21.3649079431864,-7.55179375777442,
12.));
#184792=CARTESIAN_POINT('Ctrl Pts',(21.3729148390244,-7.55375667080032,
12.));
#184793=CARTESIAN_POINT('Ctrl Pts',(21.3811668478933,-7.55574773403508,
12.));
#184794=CARTESIAN_POINT('Ctrl Pts',(21.3896598842119,-7.55776435731422,
12.));
#184795=CARTESIAN_POINT('Ctrl Pts',(21.3983899952988,-7.55980403700615,
12.));
#184796=CARTESIAN_POINT('Ctrl Pts',(21.4073533630364,-7.56186435703622,
12.));
#184797=CARTESIAN_POINT('Ctrl Pts',(21.4165463106252,-7.56394299313683,
12.));
#184798=CARTESIAN_POINT('Ctrl Pts',(21.4259653015732,-7.56603771218706,
12.));
#184799=CARTESIAN_POINT('Ctrl Pts',(21.435606926151,-7.56814636360842,12.));
#184800=CARTESIAN_POINT('Ctrl Pts',(21.445467890751,-7.5702668726117,12.));
#184801=CARTESIAN_POINT('Ctrl Pts',(21.4555450053147,-7.57239723223521,
12.));
#184802=CARTESIAN_POINT('Ctrl Pts',(21.4658351740135,-7.57453549743435,
12.));
#184803=CARTESIAN_POINT('Ctrl Pts',(21.4763353936766,-7.57667978403003,
12.));
#184804=CARTESIAN_POINT('Ctrl Pts',(21.4870427508193,-7.57882826679131,
12.));
#184805=CARTESIAN_POINT('Ctrl Pts',(21.4979544192739,-7.5809791779073,12.));
#184806=CARTESIAN_POINT('Ctrl Pts',(21.5090676573866,-7.58313080519159,
12.));
#184807=CARTESIAN_POINT('Ctrl Pts',(21.5203798035294,-7.58528148919114,
12.));
#184808=CARTESIAN_POINT('Ctrl Pts',(21.5318882716735,-7.58742962034834,
12.));
#184809=CARTESIAN_POINT('Ctrl Pts',(21.5435905470113,-7.58957363620026,
12.));
#184810=CARTESIAN_POINT('Ctrl Pts',(21.5554841813465,-7.59171201844793,
12.));
#184811=CARTESIAN_POINT('Ctrl Pts',(21.5675667904728,-7.5938432912493,12.));
#184812=CARTESIAN_POINT('Ctrl Pts',(21.5798360518978,-7.59596601973589,
12.));
#184813=CARTESIAN_POINT('Ctrl Pts',(21.5922897024466,-7.59807880846193,
12.));
#184814=CARTESIAN_POINT('Ctrl Pts',(21.6049255358842,-7.60018029988238,
12.));
#184815=CARTESIAN_POINT('Ctrl Pts',(21.6177414005991,-7.60226917285432,
12.));
#184816=CARTESIAN_POINT('Ctrl Pts',(21.6307351973823,-7.604344141183,12.));
#184817=CARTESIAN_POINT('Ctrl Pts',(21.6439048771743,-7.60640395216359,
12.));
#184818=CARTESIAN_POINT('Ctrl Pts',(21.6572484388079,-7.60844738512872,
12.));
#184819=CARTESIAN_POINT('Ctrl Pts',(21.6707639267573,-7.6104732500095,12.));
#184820=CARTESIAN_POINT('Ctrl Pts',(21.6844494295813,-7.61248038630265,
12.));
#184821=CARTESIAN_POINT('Ctrl Pts',(21.6983030783321,-7.61446766202787,
12.));
#184822=CARTESIAN_POINT('Ctrl Pts',(21.7123230449835,-7.61643397270425,
12.));
#184823=CARTESIAN_POINT('Ctrl Pts',(21.7265075407977,-7.61837824030542,
12.));
#184824=CARTESIAN_POINT('Ctrl Pts',(21.7408548148657,-7.62029941230855,
12.));
#184825=CARTESIAN_POINT('Ctrl Pts',(21.7553631528329,-7.62219646084226,
12.));
#184826=CARTESIAN_POINT('Ctrl Pts',(21.7700308755583,-7.62406838181164,
12.));
#184827=CARTESIAN_POINT('Ctrl Pts',(21.7848563378022,-7.62591419404521,
12.));
#184828=CARTESIAN_POINT('Ctrl Pts',(21.7998379268583,-7.62773293842409,
12.));
#184829=CARTESIAN_POINT('Ctrl Pts',(21.8149740615093,-7.62952367718151,
12.));
#184830=CARTESIAN_POINT('Ctrl Pts',(21.8302631910197,-7.6312854932304,12.));
#184831=CARTESIAN_POINT('Ctrl Pts',(21.8457037941084,-7.63301748948936,
12.));
#184832=CARTESIAN_POINT('Ctrl Pts',(21.8612943779086,-7.63471878821204,
12.));
#184833=CARTESIAN_POINT('Ctrl Pts',(21.8770334769492,-7.63638853033368,
12.));
#184834=CARTESIAN_POINT('Ctrl Pts',(21.8929196523511,-7.63802587492008,
12.));
#184835=CARTESIAN_POINT('Ctrl Pts',(21.9089514909873,-7.63962999860917,
12.));
#184836=CARTESIAN_POINT('Ctrl Pts',(21.9251276046546,-7.6412000950654,12.));
#184837=CARTESIAN_POINT('Ctrl Pts',(21.9414466292074,-7.64273537442707,
12.));
#184838=CARTESIAN_POINT('Ctrl Pts',(21.9579072237653,-7.64423506279154,
12.));
#184839=CARTESIAN_POINT('Ctrl Pts',(21.97450807008,-7.64569840177359,12.));
#184840=CARTESIAN_POINT('Ctrl Pts',(21.9912478718542,-7.64712464805258,
12.));
#184841=CARTESIAN_POINT('Ctrl Pts',(22.0081253540773,-7.64851307293346,
12.));
#184842=CARTESIAN_POINT('Ctrl Pts',(22.0251392623209,-7.64986296190157,
12.));
#184843=CARTESIAN_POINT('Ctrl Pts',(22.0422883621176,-7.65117361421347,
12.));
#184844=CARTESIAN_POINT('Ctrl Pts',(22.0595714384432,-7.65244434253104,
12.));
#184845=CARTESIAN_POINT('Ctrl Pts',(22.0769872951596,-7.65367447254945,
12.));
#184846=CARTESIAN_POINT('Ctrl Pts',(22.094534754469,-7.65486334263651,12.));
#184847=CARTESIAN_POINT('Ctrl Pts',(22.1122126563327,-7.65601030346819,
12.));
#184848=CARTESIAN_POINT('Ctrl Pts',(22.1300198579671,-7.65711471769407,
12.));
#184849=CARTESIAN_POINT('Ctrl Pts',(22.1479552334206,-7.65817595963351,
12.));
#184850=CARTESIAN_POINT('Ctrl Pts',(22.1660176731174,-7.65919341496926,
12.));
#184851=CARTESIAN_POINT('Ctrl Pts',(22.1842060834092,-7.66016648045008,
12.));
#184852=CARTESIAN_POINT('Ctrl Pts',(22.2025193860972,-7.66109456359292,
12.));
#184853=CARTESIAN_POINT('Ctrl Pts',(22.2209565180098,-7.66197708240436,
12.));
#184854=CARTESIAN_POINT('Ctrl Pts',(22.239516430656,-7.66281346512546,12.));
#184855=CARTESIAN_POINT('Ctrl Pts',(22.2581980898487,-7.66360314997662,
12.));
#184856=CARTESIAN_POINT('Ctrl Pts',(22.2770004753332,-7.66434558490973,
12.));
#184857=CARTESIAN_POINT('Ctrl Pts',(22.2959225803925,-7.66504022736263,
12.));
#184858=CARTESIAN_POINT('Ctrl Pts',(22.3149634114823,-7.66568654402442,
12.));
#184859=CARTESIAN_POINT('Ctrl Pts',(22.3341219879454,-7.66628401061906,
12.));
#184860=CARTESIAN_POINT('Ctrl Pts',(22.3533973417013,-7.66683211169134,
12.));
#184861=CARTESIAN_POINT('Ctrl Pts',(22.3727885169361,-7.66733034039887,
12.));
#184862=CARTESIAN_POINT('Ctrl Pts',(22.3922945697782,-7.6677781983082,12.));
#184863=CARTESIAN_POINT('Ctrl Pts',(22.411914567977,-7.66817519519682,12.));
#184864=CARTESIAN_POINT('Ctrl Pts',(22.4316475906616,-7.66852084886746,
12.));
#184865=CARTESIAN_POINT('Ctrl Pts',(22.4514927280862,-7.6688146849666,12.));
#184866=CARTESIAN_POINT('Ctrl Pts',(22.47144908137,-7.66905623680836,12.));
#184867=CARTESIAN_POINT('Ctrl Pts',(22.4915157622308,-7.66924504520302,
12.));
#184868=CARTESIAN_POINT('Ctrl Pts',(22.5116918927023,-7.66938065829083,
12.));
#184869=CARTESIAN_POINT('Ctrl Pts',(22.5319766049191,-7.66946263138116,
12.));
#184870=CARTESIAN_POINT('Ctrl Pts',(22.5523690409109,-7.66949052679672,
12.));
#184871=CARTESIAN_POINT('Ctrl Pts',(22.5728683523828,-7.66946391372299,
12.));
#184872=CARTESIAN_POINT('Ctrl Pts',(22.5934737004955,-7.66938236806241,
12.));
#184873=CARTESIAN_POINT('Ctrl Pts',(22.6141842556248,-7.66924547229435,
12.));
#184874=CARTESIAN_POINT('Ctrl Pts',(22.6349991971547,-7.66905281533745,
12.));
#184875=CARTESIAN_POINT('Ctrl Pts',(22.6559177133133,-7.66880399241354,
12.));
#184876=CARTESIAN_POINT('Ctrl Pts',(22.6769390009889,-7.66849860491763,
12.));
#184877=CARTESIAN_POINT('Ctrl Pts',(22.6980622655446,-7.66813626029277,
12.));
#184878=CARTESIAN_POINT('Ctrl Pts',(22.7192867206242,-7.6677165719101,12.));
#184879=CARTESIAN_POINT('Ctrl Pts',(22.7406115879508,-7.66723915895413,
12.));
#184880=CARTESIAN_POINT('Ctrl Pts',(22.7620360971839,-7.66670364630273,
12.));
#184881=CARTESIAN_POINT('Ctrl Pts',(22.7835594857697,-7.66610966441259,
12.));
#184882=CARTESIAN_POINT('Ctrl Pts',(22.8051809987833,-7.66545684920988,
12.));
#184883=CARTESIAN_POINT('Ctrl Pts',(22.8268998887678,-7.66474484198553,
12.));
#184884=CARTESIAN_POINT('Ctrl Pts',(22.8487154155569,-7.66397328929805,
12.));
#184885=CARTESIAN_POINT('Ctrl Pts',(22.870626846128,-7.66314184287334,12.));
#184886=CARTESIAN_POINT('Ctrl Pts',(22.8926334544879,-7.66225015950148,
12.));
#184887=CARTESIAN_POINT('Ctrl Pts',(22.9147345215418,-7.661297900941,12.));
#184888=CARTESIAN_POINT('Ctrl Pts',(22.9369293349592,-7.66028473382777,
12.));
#184889=CARTESIAN_POINT('Ctrl Pts',(22.9592171890332,-7.65921032958912,
12.));
#184890=CARTESIAN_POINT('Ctrl Pts',(22.9815973845301,-7.65807436436453,
12.));
#184891=CARTESIAN_POINT('Ctrl Pts',(23.004069228582,-7.6568765189133,12.));
#184892=CARTESIAN_POINT('Ctrl Pts',(23.0266320345792,-7.65561647852555,
12.));
#184893=CARTESIAN_POINT('Ctrl Pts',(23.049285122053,-7.65429393293955,12.));
#184894=CARTESIAN_POINT('Ctrl Pts',(23.072027816555,-7.65290857626357,12.));
#184895=CARTESIAN_POINT('Ctrl Pts',(23.0948594495246,-7.65146010690465,
12.));
#184896=CARTESIAN_POINT('Ctrl Pts',(23.1177793581674,-7.64994822749845,
12.));
#184897=CARTESIAN_POINT('Ctrl Pts',(23.1407868853815,-7.64837264482929,
12.));
#184898=CARTESIAN_POINT('Ctrl Pts',(23.1638813796691,-7.64673306975797,
12.));
#184899=CARTESIAN_POINT('Ctrl Pts',(23.1870621950452,-7.64502921715483,
12.));
#184900=CARTESIAN_POINT('Ctrl Pts',(23.2103286909399,-7.64326080583684,
12.));
#184901=CARTESIAN_POINT('Ctrl Pts',(23.2336802320912,-7.64142755851508,
12.));
#184902=CARTESIAN_POINT('Ctrl Pts',(23.2571161884487,-7.63952920172837,
12.));
#184903=CARTESIAN_POINT('Ctrl Pts',(23.2806359350853,-7.63756546576375,
12.));
#184904=CARTESIAN_POINT('Ctrl Pts',(23.3042388521021,-7.63553608458784,
12.));
#184905=CARTESIAN_POINT('Ctrl Pts',(23.3279243245241,-7.63344079578163,
12.));
#184906=CARTESIAN_POINT('Ctrl Pts',(23.3516917421973,-7.63127934048139,
12.));
#184907=CARTESIAN_POINT('Ctrl Pts',(23.3755404996638,-7.62905146332598,
12.));
#184908=CARTESIAN_POINT('Ctrl Pts',(23.3994699961122,-7.62675691240335,
12.));
#184909=CARTESIAN_POINT('Ctrl Pts',(23.4234796353544,-7.62439543920055,
12.));
#184910=CARTESIAN_POINT('Ctrl Pts',(23.4475688257854,-7.62196679855957,
12.));
#184911=CARTESIAN_POINT('Ctrl Pts',(23.4717369803438,-7.61947074863978,
12.));
#184912=CARTESIAN_POINT('Ctrl Pts',(23.4959835164608,-7.61690705088319,
12.));
#184913=CARTESIAN_POINT('Ctrl Pts',(23.5203078560128,-7.61427546999299,
12.));
#184914=CARTESIAN_POINT('Ctrl Pts',(23.5447094252028,-7.61157577385372,
12.));
#184915=CARTESIAN_POINT('Ctrl Pts',(23.5691876544243,-7.608807733446,12.));
#184916=CARTESIAN_POINT('Ctrl Pts',(23.5937419781244,-7.60597112277094,
12.));
#184917=CARTESIAN_POINT('Ctrl Pts',(23.6183718346576,-7.60306571877806,
12.));
#184918=CARTESIAN_POINT('Ctrl Pts',(23.6430766661419,-7.6000913013013,12.));
#184919=CARTESIAN_POINT('Ctrl Pts',(23.6678559182876,-7.59704765299572,
12.));
#184920=CARTESIAN_POINT('Ctrl Pts',(23.6927090405067,-7.59393455934042,
12.));
#184921=CARTESIAN_POINT('Ctrl Pts',(23.7176354860457,-7.59075180865327,
12.));
#184922=CARTESIAN_POINT('Ctrl Pts',(23.7426347121006,-7.58749919210832,
12.));
#184923=CARTESIAN_POINT('Ctrl Pts',(23.7677061799376,-7.58417650376272,
12.));
#184924=CARTESIAN_POINT('Ctrl Pts',(23.7928493549908,-7.58078354058212,
12.));
#184925=CARTESIAN_POINT('Ctrl Pts',(23.8180637069977,-7.57732010249066,
12.));
#184926=CARTESIAN_POINT('Ctrl Pts',(23.8433487096134,-7.57378599219817,
12.));
#184927=CARTESIAN_POINT('Ctrl Pts',(23.8687038399597,-7.57018101500711,
12.));
#184928=CARTESIAN_POINT('Ctrl Pts',(23.8941285782003,-7.56650497863792,
12.));
#184929=CARTESIAN_POINT('Ctrl Pts',(23.9196224070759,-7.56275769304773,
12.));
#184930=CARTESIAN_POINT('Ctrl Pts',(23.9451848115,-7.55893897027683,12.));
#184931=CARTESIAN_POINT('Ctrl Pts',(23.9708152779884,-7.55504862424812,
12.));
#184932=CARTESIAN_POINT('Ctrl Pts',(23.9965132953185,-7.55108647097441,
12.));
#184933=CARTESIAN_POINT('Ctrl Pts',(24.022278355453,-7.5470523288591,12.));
#184934=CARTESIAN_POINT('Ctrl Pts',(24.0481099543353,-7.54294601896145,
12.));
#184935=CARTESIAN_POINT('Ctrl Pts',(24.0740075927985,-7.53876736531014,
12.));
#184936=CARTESIAN_POINT('Ctrl Pts',(24.0999707772642,-7.53451619514649,
12.));
#184937=CARTESIAN_POINT('Ctrl Pts',(24.1259990209207,-7.53019233935502,
12.));
#184938=CARTESIAN_POINT('Ctrl Pts',(24.1520918425364,-7.52579563201424,
12.));
#184939=CARTESIAN_POINT('Ctrl Pts',(24.1782487641594,-7.52132590953802,
12.));
#184940=CARTESIAN_POINT('Ctrl Pts',(24.2044693092349,-7.51678300997949,
12.));
#184941=CARTESIAN_POINT('Ctrl Pts',(24.2307530003887,-7.51216677222181,
12.));
#184942=CARTESIAN_POINT('Ctrl Pts',(24.2570993577034,-7.50747703535134,
12.));
#184943=CARTESIAN_POINT('Ctrl Pts',(24.2835078958973,-7.50271363765152,
12.));
#184944=CARTESIAN_POINT('Ctrl Pts',(24.3099781253355,-7.49787641695439,
12.));
#184945=CARTESIAN_POINT('Ctrl Pts',(24.3365095573685,-7.49296521252421,
12.));
#184946=CARTESIAN_POINT('Ctrl Pts',(24.3631017084524,-7.48797986651909,
12.));
#184947=CARTESIAN_POINT('Ctrl Pts',(24.3897541049254,-7.48292022569301,
12.));
#184948=CARTESIAN_POINT('Ctrl Pts',(24.4164662871163,-7.47778614286565,
12.));
#184949=CARTESIAN_POINT('Ctrl Pts',(24.443237814649,-7.47257747883246,12.));
#184950=CARTESIAN_POINT('Ctrl Pts',(24.4700682684524,-7.46729410308787,
12.));
#184951=CARTESIAN_POINT('Ctrl Pts',(24.4969572391483,-7.46193588961464,
12.));
#184952=CARTESIAN_POINT('Ctrl Pts',(24.5239043173072,-7.45650271335862,
12.));
#184953=CARTESIAN_POINT('Ctrl Pts',(24.5509090831559,-7.4509944465116,12.));
#184954=CARTESIAN_POINT('Ctrl Pts',(24.577971096086,-7.44541095473135,12.));
#184955=CARTESIAN_POINT('Ctrl Pts',(24.6050898852368,-7.43975209375504,
12.));
#184956=CARTESIAN_POINT('Ctrl Pts',(24.6322649369517,-7.43401770489524,
12.));
#184957=CARTESIAN_POINT('Ctrl Pts',(24.6594957128756,-7.42820762159126,
12.));
#184958=CARTESIAN_POINT('Ctrl Pts',(24.6867816727192,-7.42232167766266,
12.));
#184959=CARTESIAN_POINT('Ctrl Pts',(24.7141222950051,-7.41635971481674,
12.));
#184960=CARTESIAN_POINT('Ctrl Pts',(24.7415170994784,-7.41032159082382,
12.));
#184961=CARTESIAN_POINT('Ctrl Pts',(24.7689656668983,-7.40420718661603,
12.));
#184962=CARTESIAN_POINT('Ctrl Pts',(24.7964676646431,-7.39801641583013,
12.));
#184963=CARTESIAN_POINT('Ctrl Pts',(24.8240228520893,-7.39174922585809,
12.));
#184964=CARTESIAN_POINT('Ctrl Pts',(24.8516310625176,-7.38540558903621,
12.));
#184965=CARTESIAN_POINT('Ctrl Pts',(24.8792921911115,-7.3789854964027,12.));
#184966=CARTESIAN_POINT('Ctrl Pts',(24.901463382605,-7.37378825961676,12.));
#184967=CARTESIAN_POINT('Ctrl Pts',(24.9181155530543,-7.36985593120091,
12.));
#184968=CARTESIAN_POINT('Ctrl Pts',(24.9292275670674,-7.36721909028843,
12.));
#184969=CARTESIAN_POINT('Ctrl Pts',(24.9347862158358,-7.36589684767345,
12.));
#184970=CARTESIAN_POINT('',(25.2771067246846,-6.088339316177,12.));
#184971=CARTESIAN_POINT('Origin',(0.,0.,12.));
#184972=CARTESIAN_POINT('',(22.1738711152697,-4.11585220600463,12.));
#184973=CARTESIAN_POINT('Ctrl Pts',(25.2771067246846,-6.088339316177,12.));
#184974=CARTESIAN_POINT('Ctrl Pts',(25.2729539149517,-6.08441489609794,
12.));
#184975=CARTESIAN_POINT('Ctrl Pts',(25.2646490489922,-6.07657531787491,
12.));
#184976=CARTESIAN_POINT('Ctrl Pts',(25.2521940105705,-6.06484373634547,
12.));
#184977=CARTESIAN_POINT('Ctrl Pts',(25.2355918139032,-6.04925720151219,
12.));
#184978=CARTESIAN_POINT('Ctrl Pts',(25.21484662016,-6.02986667389998,12.));
#184979=CARTESIAN_POINT('Ctrl Pts',(25.1941090269819,-6.01056881804614,
12.));
#184980=CARTESIAN_POINT('Ctrl Pts',(25.1733791296259,-5.99136367859755,
12.));
#184981=CARTESIAN_POINT('Ctrl Pts',(25.1526570863092,-5.97225131495618,
12.));
#184982=CARTESIAN_POINT('Ctrl Pts',(25.1319431317237,-5.95323180187379,
12.));
#184983=CARTESIAN_POINT('Ctrl Pts',(25.1112375971106,-5.93430523086836,
12.));
#184984=CARTESIAN_POINT('Ctrl Pts',(25.0905409050773,-5.91547170844448,
12.));
#184985=CARTESIAN_POINT('Ctrl Pts',(25.0698535426514,-5.89673135155515,
12.));
#184986=CARTESIAN_POINT('Ctrl Pts',(25.049176040591,-5.87808428385367,12.));
#184987=CARTESIAN_POINT('Ctrl Pts',(25.0285089498899,-5.85953063156827,
12.));
#184988=CARTESIAN_POINT('Ctrl Pts',(25.0078528200564,-5.84107051963072,
12.));
#184989=CARTESIAN_POINT('Ctrl Pts',(24.9872081752734,-5.822704067442,12.));
#184990=CARTESIAN_POINT('Ctrl Pts',(24.9665754954496,-5.80443138549727,
12.));
#184991=CARTESIAN_POINT('Ctrl Pts',(24.945955229334,-5.78625257775682,12.));
#184992=CARTESIAN_POINT('Ctrl Pts',(24.9253478043656,-5.76816774342221,
12.));
#184993=CARTESIAN_POINT('Ctrl Pts',(24.904753637648,-5.75017697890805,12.));
#184994=CARTESIAN_POINT('Ctrl Pts',(24.884173146722,-5.73228037976928,12.));
#184995=CARTESIAN_POINT('Ctrl Pts',(24.8636067597669,-5.71447804252028,
12.));
#184996=CARTESIAN_POINT('Ctrl Pts',(24.8430549277621,-5.69677006679445,
12.));
#184997=CARTESIAN_POINT('Ctrl Pts',(24.8225181223845,-5.67915655496543,
12.));
#184998=CARTESIAN_POINT('Ctrl Pts',(24.8019968304605,-5.66163761114922,
12.));
#184999=CARTESIAN_POINT('Ctrl Pts',(24.781491549672,-5.64421334042262,12.));
#185000=CARTESIAN_POINT('Ctrl Pts',(24.7610027835697,-5.62688384790924,
12.));
#185001=CARTESIAN_POINT('Ctrl Pts',(24.7405310372739,-5.60964923798492,
12.));
#185002=CARTESIAN_POINT('Ctrl Pts',(24.7200768119088,-5.59250961323988,
12.));
#185003=CARTESIAN_POINT('Ctrl Pts',(24.6996406035517,-5.57546507427756,
12.));
#185004=CARTESIAN_POINT('Ctrl Pts',(24.6792229061794,-5.55851572025377,
12.));
#185005=CARTESIAN_POINT('Ctrl Pts',(24.6588242134738,-5.54166164919584,
12.));
#185006=CARTESIAN_POINT('Ctrl Pts',(24.6384450211467,-5.52490295840993,
12.));
#185007=CARTESIAN_POINT('Ctrl Pts',(24.6180858289179,-5.50823974481963,
12.));
#185008=CARTESIAN_POINT('Ctrl Pts',(24.5977471429364,-5.49167210537248,
12.));
#185009=CARTESIAN_POINT('Ctrl Pts',(24.5774294770329,-5.4752001372442,12.));
#185010=CARTESIAN_POINT('Ctrl Pts',(24.5571333514842,-5.45882393762263,
12.));
#185011=CARTESIAN_POINT('Ctrl Pts',(24.5368592922863,-5.44254360356881,
12.));
#185012=CARTESIAN_POINT('Ctrl Pts',(24.5166078302108,-5.4263592318342,12.));
#185013=CARTESIAN_POINT('Ctrl Pts',(24.496379499983,-5.41027091869242,12.));
#185014=CARTESIAN_POINT('Ctrl Pts',(24.4761748393321,-5.39427875973825,
12.));
#185015=CARTESIAN_POINT('Ctrl Pts',(24.4559943883157,-5.37838284973696,
12.));
#185016=CARTESIAN_POINT('Ctrl Pts',(24.435838689915,-5.36258328273628,12.));
#185017=CARTESIAN_POINT('Ctrl Pts',(24.4157082904614,-5.34688015213538,
12.));
#185018=CARTESIAN_POINT('Ctrl Pts',(24.3956037401293,-5.33127355076035,
12.));
#185019=CARTESIAN_POINT('Ctrl Pts',(24.3755255933917,-5.31576357092527,
12.));
#185020=CARTESIAN_POINT('Ctrl Pts',(24.3554744095075,-5.30035030449065,
12.));
#185021=CARTESIAN_POINT('Ctrl Pts',(24.3354507529414,-5.28503384290649,
12.));
#185022=CARTESIAN_POINT('Ctrl Pts',(24.3154551932221,-5.269814277188,12.));
#185023=CARTESIAN_POINT('Ctrl Pts',(24.2954883048447,-5.25469169788858,
12.));
#185024=CARTESIAN_POINT('Ctrl Pts',(24.2755506671525,-5.2396661950629,12.));
#185025=CARTESIAN_POINT('Ctrl Pts',(24.2556428642294,-5.22473785822443,
12.));
#185026=CARTESIAN_POINT('Ctrl Pts',(24.2357654847766,-5.20990677629177,
12.));
#185027=CARTESIAN_POINT('Ctrl Pts',(24.2159191220171,-5.19517303753648,
12.));
#185028=CARTESIAN_POINT('Ctrl Pts',(24.1961043738755,-5.180536729614,12.));
#185029=CARTESIAN_POINT('Ctrl Pts',(24.1763218431344,-5.16599793957987,
12.));
#185030=CARTESIAN_POINT('Ctrl Pts',(24.1565721375971,-5.1515567539008,12.));
#185031=CARTESIAN_POINT('Ctrl Pts',(24.1368558702443,-5.13721325845746,
12.));
#185032=CARTESIAN_POINT('Ctrl Pts',(24.117173659394,-5.12296753853858,12.));
#185033=CARTESIAN_POINT('Ctrl Pts',(24.0975261288444,-5.10881967883126,
12.));
#185034=CARTESIAN_POINT('Ctrl Pts',(24.0779139079264,-5.09476976342618,
12.));
#185035=CARTESIAN_POINT('Ctrl Pts',(24.0583376315636,-5.08081787581271,
12.));
#185036=CARTESIAN_POINT('Ctrl Pts',(24.0387979403268,-5.0669640988664,12.));
#185037=CARTESIAN_POINT('Ctrl Pts',(24.0192954804896,-5.05320851483069,
12.));
#185038=CARTESIAN_POINT('Ctrl Pts',(23.9998309040747,-5.03955120528528,
12.));
#185039=CARTESIAN_POINT('Ctrl Pts',(23.9804048689228,-5.02599225112462,
12.));
#185040=CARTESIAN_POINT('Ctrl Pts',(23.9610180388271,-5.01253173257459,
12.));
#185041=CARTESIAN_POINT('Ctrl Pts',(23.9416710836528,-4.9991697291931,12.));
#185042=CARTESIAN_POINT('Ctrl Pts',(23.9223646794591,-4.98590631986534,
12.));
#185043=CARTESIAN_POINT('Ctrl Pts',(23.9030995086164,-4.9727415827923,12.));
#185044=CARTESIAN_POINT('Ctrl Pts',(23.883876259922,-4.95967559546566,12.));
#185045=CARTESIAN_POINT('Ctrl Pts',(23.8646956287172,-4.94670843465869,
12.));
#185046=CARTESIAN_POINT('Ctrl Pts',(23.8455583170062,-4.93384017643443,
12.));
#185047=CARTESIAN_POINT('Ctrl Pts',(23.8264650335721,-4.92107089613978,
12.));
#185048=CARTESIAN_POINT('Ctrl Pts',(23.8074164940897,-4.90840066839348,
12.));
#185049=CARTESIAN_POINT('Ctrl Pts',(23.7884134212381,-4.89582956706772,
12.));
#185050=CARTESIAN_POINT('Ctrl Pts',(23.7694565448044,-4.88335766525566,
12.));
#185051=CARTESIAN_POINT('Ctrl Pts',(23.7505466018239,-4.87098503527144,
12.));
#185052=CARTESIAN_POINT('Ctrl Pts',(23.7316843367308,-4.85871174865493,
12.));
#185053=CARTESIAN_POINT('Ctrl Pts',(23.7128705015014,-4.84653787616424,
12.));
#185054=CARTESIAN_POINT('Ctrl Pts',(23.6941058557971,-4.83446348776268,
12.));
#185055=CARTESIAN_POINT('Ctrl Pts',(23.6753911671023,-4.82248865259571,
12.));
#185056=CARTESIAN_POINT('Ctrl Pts',(23.6567272108631,-4.81061343896443,
12.));
#185057=CARTESIAN_POINT('Ctrl Pts',(23.6381147706581,-4.79883791433231,
12.));
#185058=CARTESIAN_POINT('Ctrl Pts',(23.6195546383625,-4.78716214532105,
12.));
#185059=CARTESIAN_POINT('Ctrl Pts',(23.6010476143099,-4.77558619769876,
12.));
#185060=CARTESIAN_POINT('Ctrl Pts',(23.5825945074535,-4.76411013636252,
12.));
#185061=CARTESIAN_POINT('Ctrl Pts',(23.564196135517,-4.75273402530616,12.));
#185062=CARTESIAN_POINT('Ctrl Pts',(23.5458533251715,-4.74145792760699,
12.));
#185063=CARTESIAN_POINT('Ctrl Pts',(23.5275669122378,-4.73028190543032,
12.));
#185064=CARTESIAN_POINT('Ctrl Pts',(23.5093377418784,-4.71920602001905,
12.));
#185065=CARTESIAN_POINT('Ctrl Pts',(23.491166668789,-4.70823033167821,12.));
#185066=CARTESIAN_POINT('Ctrl Pts',(23.4730545573849,-4.69735489975024,
12.));
#185067=CARTESIAN_POINT('Ctrl Pts',(23.4550022819852,-4.68657978258298,
12.));
#185068=CARTESIAN_POINT('Ctrl Pts',(23.4370107270444,-4.67590503753051,
12.));
#185069=CARTESIAN_POINT('Ctrl Pts',(23.4190807873798,-4.66533072094664,
12.));
#185070=CARTESIAN_POINT('Ctrl Pts',(23.4012133683957,-4.65485688816923,
12.));
#185071=CARTESIAN_POINT('Ctrl Pts',(23.383409386307,-4.64448359349936,12.));
#185072=CARTESIAN_POINT('Ctrl Pts',(23.3656697683496,-4.63421089016556,
12.));
#185073=CARTESIAN_POINT('Ctrl Pts',(23.3479954530281,-4.62403883030825,
12.));
#185074=CARTESIAN_POINT('Ctrl Pts',(23.3303873903947,-4.6139674649785,12.));
#185075=CARTESIAN_POINT('Ctrl Pts',(23.3128465423119,-4.60399684412176,
12.));
#185076=CARTESIAN_POINT('Ctrl Pts',(23.295373882719,-4.59412701655751,12.));
#185077=CARTESIAN_POINT('Ctrl Pts',(23.2779703978868,-4.58435802994675,
12.));
#185078=CARTESIAN_POINT('Ctrl Pts',(23.2606370866853,-4.57468993076071,
12.));
#185079=CARTESIAN_POINT('Ctrl Pts',(23.2433749609117,-4.56512276427812,
12.));
#185080=CARTESIAN_POINT('Ctrl Pts',(23.2261850456054,-4.55565657456957,
12.));
#185081=CARTESIAN_POINT('Ctrl Pts',(23.2090683793627,-4.54629140447543,
12.));
#185082=CARTESIAN_POINT('Ctrl Pts',(23.1920260146474,-4.53702729557586,
12.));
#185083=CARTESIAN_POINT('Ctrl Pts',(23.1750590180923,-4.52786428815049,
12.));
#185084=CARTESIAN_POINT('Ctrl Pts',(23.1581684708778,-4.51880242116786,
12.));
#185085=CARTESIAN_POINT('Ctrl Pts',(23.1413554691136,-4.50984173227088,
12.));
#185086=CARTESIAN_POINT('Ctrl Pts',(23.1246211242117,-4.5009822577518,12.));
#185087=CARTESIAN_POINT('Ctrl Pts',(23.1079665632629,-4.49222403252202,
12.));
#185088=CARTESIAN_POINT('Ctrl Pts',(23.0913929293909,-4.48356709006757,
12.));
#185089=CARTESIAN_POINT('Ctrl Pts',(23.0749013821867,-4.47501146242822,
12.));
#185090=CARTESIAN_POINT('Ctrl Pts',(23.0584930981723,-4.46655718018206,
12.));
#185091=CARTESIAN_POINT('Ctrl Pts',(23.0421692712466,-4.45820427241678,
12.));
#185092=CARTESIAN_POINT('Ctrl Pts',(23.0259311131395,-4.44995276669699,
12.));
#185093=CARTESIAN_POINT('Ctrl Pts',(23.0097798538399,-4.44180268901667,
12.));
#185094=CARTESIAN_POINT('Ctrl Pts',(22.9937167421009,-4.43375406376906,
12.));
#185095=CARTESIAN_POINT('Ctrl Pts',(22.9777430460021,-4.42580691372772,
12.));
#185096=CARTESIAN_POINT('Ctrl Pts',(22.9618600534866,-4.41796126001311,
12.));
#185097=CARTESIAN_POINT('Ctrl Pts',(22.9460690729092,-4.41021712205549,
12.));
#185098=CARTESIAN_POINT('Ctrl Pts',(22.9303714335549,-4.40257451754309,
12.));
#185099=CARTESIAN_POINT('Ctrl Pts',(22.9147684862425,-4.39503346238455,
12.));
#185100=CARTESIAN_POINT('Ctrl Pts',(22.8992616040108,-4.38759397068393,
12.));
#185101=CARTESIAN_POINT('Ctrl Pts',(22.8838521827702,-4.38025605470091,
12.));
#185102=CARTESIAN_POINT('Ctrl Pts',(22.8685416419725,-4.37301972480753,
12.));
#185103=CARTESIAN_POINT('Ctrl Pts',(22.8533314252419,-4.36588498943011,
12.));
#185104=CARTESIAN_POINT('Ctrl Pts',(22.838223001118,-4.3588518550056,12.));
#185105=CARTESIAN_POINT('Ctrl Pts',(22.8232178638873,-4.35192032594802,
12.));
#185106=CARTESIAN_POINT('Ctrl Pts',(22.808317534379,-4.34509040460066,12.));
#185107=CARTESIAN_POINT('Ctrl Pts',(22.7935235607807,-4.33836209118444,
12.));
#185108=CARTESIAN_POINT('Ctrl Pts',(22.7788375194081,-4.33173538373183,
12.));
#185109=CARTESIAN_POINT('Ctrl Pts',(22.764261015648,-4.32521027803748,12.));
#185110=CARTESIAN_POINT('Ctrl Pts',(22.7497956849852,-4.31878676761231,
12.));
#185111=CARTESIAN_POINT('Ctrl Pts',(22.7354431939926,-4.31246484362551,
12.));
#185112=CARTESIAN_POINT('Ctrl Pts',(22.7212052413384,-4.30624449484075,
12.));
#185113=CARTESIAN_POINT('Ctrl Pts',(22.707083558756,-4.30012570754067,12.));
#185114=CARTESIAN_POINT('Ctrl Pts',(22.6930799122545,-4.29410846547062,
12.));
#185115=CARTESIAN_POINT('Ctrl Pts',(22.6791961033536,-4.28819274977767,
12.));
#185116=CARTESIAN_POINT('Ctrl Pts',(22.665433970311,-4.2823785389406,12.));
#185117=CARTESIAN_POINT('Ctrl Pts',(22.6517953893303,-4.27666580869118,
12.));
#185118=CARTESIAN_POINT('Ctrl Pts',(22.6382822758171,-4.27105453193,12.));
#185119=CARTESIAN_POINT('Ctrl Pts',(22.6248965859975,-4.26554467865572,
12.));
#185120=CARTESIAN_POINT('Ctrl Pts',(22.611640318482,-4.26013621588304,12.));
#185121=CARTESIAN_POINT('Ctrl Pts',(22.5985155158637,-4.25482910755486,
12.));
#185122=CARTESIAN_POINT('Ctrl Pts',(22.5855242662479,-4.24962331444186,
12.));
#185123=CARTESIAN_POINT('Ctrl Pts',(22.5726687049922,-4.2445187940486,12.));
#185124=CARTESIAN_POINT('Ctrl Pts',(22.559951016643,-4.23951550052527,12.));
#185125=CARTESIAN_POINT('Ctrl Pts',(22.5473734368086,-4.23461338456714,
12.));
#185126=CARTESIAN_POINT('Ctrl Pts',(22.5349382540587,-4.22981239330733,
12.));
#185127=CARTESIAN_POINT('Ctrl Pts',(22.5226478117885,-4.22511247020041,
12.));
#185128=CARTESIAN_POINT('Ctrl Pts',(22.5105045108882,-4.22051355490198,
12.));
#185129=CARTESIAN_POINT('Ctrl Pts',(22.4985108124229,-4.21601558313909,
12.));
#185130=CARTESIAN_POINT('Ctrl Pts',(22.4866692403147,-4.21161848657429,
12.));
#185131=CARTESIAN_POINT('Ctrl Pts',(22.4749823839915,-4.20732219265649,
12.));
#185132=CARTESIAN_POINT('Ctrl Pts',(22.4634529011433,-4.20312662448172,
12.));
#185133=CARTESIAN_POINT('Ctrl Pts',(22.4520835205419,-4.19903170066356,
12.));
#185134=CARTESIAN_POINT('Ctrl Pts',(22.4408770448917,-4.19503733518862,
12.));
#185135=CARTESIAN_POINT('Ctrl Pts',(22.4298363535421,-4.19114343726943,
12.));
#185136=CARTESIAN_POINT('Ctrl Pts',(22.4189644056115,-4.18734991117722,
12.));
#185137=CARTESIAN_POINT('Ctrl Pts',(22.4082642454453,-4.18365665600852,
12.));
#185138=CARTESIAN_POINT('Ctrl Pts',(22.3977390078075,-4.18006356544883,
12.));
#185139=CARTESIAN_POINT('Ctrl Pts',(22.3873919231334,-4.17657052752826,
12.));
#185140=CARTESIAN_POINT('Ctrl Pts',(22.3772263228617,-4.17317742436146,
12.));
#185141=CARTESIAN_POINT('Ctrl Pts',(22.3672456427599,-4.16988413199458,
12.));
#185142=CARTESIAN_POINT('Ctrl Pts',(22.3574534257396,-4.16669052026601,
12.));
#185143=CARTESIAN_POINT('Ctrl Pts',(22.3478533253889,-4.16359645263189,
12.));
#185144=CARTESIAN_POINT('Ctrl Pts',(22.3384491078602,-4.16060178604165,
12.));
#185145=CARTESIAN_POINT('Ctrl Pts',(22.3292446628959,-4.15770637047891,
12.));
#185146=CARTESIAN_POINT('Ctrl Pts',(22.3202440186979,-4.15491004835282,
12.));
#185147=CARTESIAN_POINT('Ctrl Pts',(22.3114513545185,-4.15221265396991,
12.));
#185148=CARTESIAN_POINT('Ctrl Pts',(22.3028710166933,-4.14961401285523,
12.));
#185149=CARTESIAN_POINT('Ctrl Pts',(22.2945075198467,-4.14711394168557,
12.));
#185150=CARTESIAN_POINT('Ctrl Pts',(22.2863655389166,-4.14471224859297,
12.));
#185151=CARTESIAN_POINT('Ctrl Pts',(22.2784499072027,-4.14240873321985,
12.));
#185152=CARTESIAN_POINT('Ctrl Pts',(22.2707656042457,-4.14020318715992,
12.));
#185153=CARTESIAN_POINT('Ctrl Pts',(22.2633177913972,-4.13809539255423,
12.));
#185154=CARTESIAN_POINT('Ctrl Pts',(22.2561118708421,-4.13608511977227,
12.));
#185155=CARTESIAN_POINT('Ctrl Pts',(22.249153531779,-4.13417212558811,12.));
#185156=CARTESIAN_POINT('Ctrl Pts',(22.2424488153523,-4.13235615060161,
12.));
#185157=CARTESIAN_POINT('Ctrl Pts',(22.2360040565533,-4.13063692157499,
12.));
#185158=CARTESIAN_POINT('Ctrl Pts',(22.2298258043947,-4.1290141546338,12.));
#185159=CARTESIAN_POINT('Ctrl Pts',(22.2239207458781,-4.12748755830105,
12.));
#185160=CARTESIAN_POINT('Ctrl Pts',(22.2182956401341,-4.12605683613308,
12.));
#185161=CARTESIAN_POINT('Ctrl Pts',(22.2129576146671,-4.12472167516608,
12.));
#185162=CARTESIAN_POINT('Ctrl Pts',(22.2079143941719,-4.12348173702024,
12.));
#185163=CARTESIAN_POINT('Ctrl Pts',(22.2031746532106,-4.12233664408228,
12.));
#185164=CARTESIAN_POINT('Ctrl Pts',(22.1987479618246,-4.12128598183523,
12.));
#185165=CARTESIAN_POINT('Ctrl Pts',(22.1946440958098,-4.12032932637738,
12.));
#185166=CARTESIAN_POINT('Ctrl Pts',(22.1908725908525,-4.11946626228637,
12.));
#185167=CARTESIAN_POINT('Ctrl Pts',(22.1874419861496,-4.11869641271775,
12.));
#185168=CARTESIAN_POINT('Ctrl Pts',(22.1843613164855,-4.11801938107481,
12.));
#185169=CARTESIAN_POINT('Ctrl Pts',(22.1816414985788,-4.11743469691757,
12.));
#185170=CARTESIAN_POINT('Ctrl Pts',(22.179297473024,-4.11694173195005,12.));
#185171=CARTESIAN_POINT('Ctrl Pts',(22.177347426894,-4.11653973150519,12.));
#185172=CARTESIAN_POINT('Ctrl Pts',(22.1758088296598,-4.1162279721707,12.));
#185173=CARTESIAN_POINT('Ctrl Pts',(22.1746949858775,-4.11600589882846,
12.));
#185174=CARTESIAN_POINT('Ctrl Pts',(22.1741488021234,-4.11589976826168,
12.));
#185175=CARTESIAN_POINT('Ctrl Pts',(22.1739341411687,-4.11586035878288,
12.));
#185176=CARTESIAN_POINT('Ctrl Pts',(22.173877682324,-4.11585194677443,12.));
#185177=CARTESIAN_POINT('Ctrl Pts',(22.1738711152697,-4.11585220600463,
12.));
#185178=CARTESIAN_POINT('',(21.624941921198,-4.0139614976743,12.));
#185179=CARTESIAN_POINT('',(10.5694630535049,-1.96187429785751,12.));
#185180=CARTESIAN_POINT('',(21.2226420728916,-3.4423049612042,12.));
#185181=CARTESIAN_POINT('Origin',(21.7161918885402,-3.52235856495314,12.));
#185182=CARTESIAN_POINT('',(21.3904321633055,-2.1678126918683,12.));
#185183=CARTESIAN_POINT('Origin',(7.6920903736728E-13,-1.31973449697531E-13,
12.));
#185184=CARTESIAN_POINT('',(21.9269795755927,-1.71975774210843,12.));
#185185=CARTESIAN_POINT('Origin',(21.88788407408,-2.2182269405164,12.));
#185186=CARTESIAN_POINT('',(11.2417878583927,-0.881706102655892,12.));
#185187=CARTESIAN_POINT('Origin',(21.88788407408,-2.2182269405164,0.));
#185188=CARTESIAN_POINT('',(21.3904321633055,-2.1678126918683,0.));
#185189=CARTESIAN_POINT('',(21.9269795755927,-1.71975774210843,0.));
#185190=CARTESIAN_POINT('Origin',(21.88788407408,-2.2182269405164,0.));
#185191=CARTESIAN_POINT('',(21.9269795755927,-1.71975774210843,0.));
#185192=CARTESIAN_POINT('',(21.3904321633055,-2.1678126918683,0.));
#185193=CARTESIAN_POINT('Origin',(22.4835757167854,-1.76341220531181,0.));
#185194=CARTESIAN_POINT('',(22.4835757167854,-1.76341220531181,0.));
#185195=CARTESIAN_POINT('',(11.2417878583927,-0.881706102655892,0.));
#185196=CARTESIAN_POINT('',(22.4835757167854,-1.76341220531181,0.));
#185197=CARTESIAN_POINT('Origin',(21.7161918885402,-3.52235856495314,0.));
#185198=CARTESIAN_POINT('',(21.624941921198,-4.0139614976743,0.));
#185199=CARTESIAN_POINT('',(21.2226420728916,-3.4423049612042,0.));
#185200=CARTESIAN_POINT('Origin',(21.7161918885402,-3.52235856495314,0.));
#185201=CARTESIAN_POINT('',(21.2226420728916,-3.4423049612042,0.));
#185202=CARTESIAN_POINT('',(21.624941921198,-4.0139614976743,0.));
#185203=CARTESIAN_POINT('Origin',(7.6920903736728E-13,-1.31973449697531E-13,
0.));
#185204=CARTESIAN_POINT('Origin',(7.6920903736728E-13,-1.31973449697531E-13,
0.));
#185205=CARTESIAN_POINT('Origin',(20.56795313141,-7.80764394578304,0.));
#185206=CARTESIAN_POINT('',(20.1004996511507,-7.63019749246979,0.));
#185207=CARTESIAN_POINT('',(20.7347298079577,-7.33627833380047,0.));
#185208=CARTESIAN_POINT('Origin',(20.56795313141,-7.80764394578304,0.));
#185209=CARTESIAN_POINT('',(20.7347298079577,-7.33627833380047,0.));
#185210=CARTESIAN_POINT('',(20.1004996511507,-7.63019749246979,0.));
#185211=CARTESIAN_POINT('Origin',(21.2610617890679,-7.52250298901266,0.));
#185212=CARTESIAN_POINT('',(21.2610617890679,-7.52250298901266,0.));
#185213=CARTESIAN_POINT('',(10.6305308945339,-3.76125149450632,0.));
#185214=CARTESIAN_POINT('',(21.2610617890679,-7.52250298901266,0.));
#185215=CARTESIAN_POINT('Origin',(20.0645771135003,-9.02290115519382,0.));
#185216=CARTESIAN_POINT('',(19.84920021178,-9.47413589477549,0.));
#185217=CARTESIAN_POINT('',(19.6085639972844,-8.81783521984851,0.));
#185218=CARTESIAN_POINT('Origin',(20.0645771135003,-9.02290115519382,0.));
#185219=CARTESIAN_POINT('',(19.6085639972844,-8.81783521984851,0.));
#185220=CARTESIAN_POINT('',(19.84920021178,-9.47413589477549,0.));
#185221=CARTESIAN_POINT('Origin',(7.08841632778409E-13,-3.26562511982935E-13,
0.));
#185222=CARTESIAN_POINT('Origin',(7.08841632778409E-13,-3.26562511982935E-13,
0.));
#185223=CARTESIAN_POINT('Origin',(17.846350172984,-12.8649829188862,0.));
#185224=CARTESIAN_POINT('',(17.4407513054162,-12.572596943457,0.));
#185225=CARTESIAN_POINT('',(18.1294424696716,-12.4528436808172,0.));
#185226=CARTESIAN_POINT('Origin',(17.846350172984,-12.8649829188862,0.));
#185227=CARTESIAN_POINT('',(18.1294424696716,-12.4528436808172,0.));
#185228=CARTESIAN_POINT('',(17.4407513054162,-12.572596943457,0.));
#185229=CARTESIAN_POINT('Origin',(18.5896416359912,-12.7689476255363,0.));
#185230=CARTESIAN_POINT('',(18.5896416359912,-12.7689476255363,0.));
#185231=CARTESIAN_POINT('',(9.29482081799561,-6.38447381276812,0.));
#185232=CARTESIAN_POINT('',(18.5896416359912,-12.7689476255363,0.));
#185233=CARTESIAN_POINT('Origin',(17.0455945664569,-13.9085479427572,0.));
#185234=CARTESIAN_POINT('',(16.7207683102834,-14.2886635873976,0.));
#185235=CARTESIAN_POINT('',(16.6581946899465,-13.5924445804218,0.));
#185236=CARTESIAN_POINT('Origin',(17.0455945664569,-13.9085479427572,0.));
#185237=CARTESIAN_POINT('',(16.6581946899465,-13.5924445804218,0.));
#185238=CARTESIAN_POINT('',(16.7207683102834,-14.2886635873976,0.));
#185239=CARTESIAN_POINT('Origin',(6.00167842331873E-13,-4.9889687874677E-13,
0.));
#185240=CARTESIAN_POINT('Origin',(6.00167842331873E-13,-4.9889687874677E-13,
0.));
#185241=CARTESIAN_POINT('Origin',(13.9085479427572,-17.0455945664569,0.));
#185242=CARTESIAN_POINT('',(13.5924445804218,-16.6581946899465,0.));
#185243=CARTESIAN_POINT('',(14.2886635873976,-16.7207683102834,0.));
#185244=CARTESIAN_POINT('Origin',(13.9085479427572,-17.0455945664569,0.));
#185245=CARTESIAN_POINT('',(14.2886635873976,-16.7207683102834,0.));
#185246=CARTESIAN_POINT('',(13.5924445804218,-16.6581946899465,0.));
#185247=CARTESIAN_POINT('Origin',(14.6513681262571,-17.1452095830633,0.));
#185248=CARTESIAN_POINT('',(14.6513681262571,-17.1452095830633,0.));
#185249=CARTESIAN_POINT('',(7.32568406312854,-8.57260479153162,0.));
#185250=CARTESIAN_POINT('',(14.6513681262571,-17.1452095830633,0.));
#185251=CARTESIAN_POINT('Origin',(12.8649829188862,-17.846350172984,0.));
#185252=CARTESIAN_POINT('',(12.4528436808172,-18.1294424696716,0.));
#185253=CARTESIAN_POINT('',(12.572596943457,-17.4407513054162,0.));
#185254=CARTESIAN_POINT('Origin',(12.8649829188862,-17.846350172984,0.));
#185255=CARTESIAN_POINT('',(12.572596943457,-17.4407513054162,0.));
#185256=CARTESIAN_POINT('',(12.4528436808172,-18.1294424696716,0.));
#185257=CARTESIAN_POINT('Origin',(4.50593605254674E-13,-6.37232247690087E-13,
0.));
#185258=CARTESIAN_POINT('Origin',(4.50593605254674E-13,-6.37232247690087E-13,
0.));
#185259=CARTESIAN_POINT('Origin',(9.02290115519381,-20.0645771135004,0.));
#185260=CARTESIAN_POINT('',(8.81783521984849,-19.6085639972844,0.));
#185261=CARTESIAN_POINT('',(9.47413589477548,-19.84920021178,0.));
#185262=CARTESIAN_POINT('Origin',(9.02290115519381,-20.0645771135004,0.));
#185263=CARTESIAN_POINT('',(9.47413589477547,-19.84920021178,0.));
#185264=CARTESIAN_POINT('',(8.81783521984849,-19.6085639972844,0.));
#185265=CARTESIAN_POINT('Origin',(9.71462809124915,-20.353053841303,0.));
#185266=CARTESIAN_POINT('',(9.71462809124915,-20.353053841303,0.));
#185267=CARTESIAN_POINT('',(4.85731404562459,-10.1765269206515,0.));
#185268=CARTESIAN_POINT('',(9.71462809124915,-20.353053841303,0.));
#185269=CARTESIAN_POINT('Origin',(7.80764394578302,-20.56795313141,0.));
#185270=CARTESIAN_POINT('',(7.33627833380045,-20.7347298079577,0.));
#185271=CARTESIAN_POINT('',(7.63019749246977,-20.1004996511507,0.));
#185272=CARTESIAN_POINT('Origin',(7.80764394578302,-20.56795313141,0.));
#185273=CARTESIAN_POINT('',(7.63019749246977,-20.1004996511507,0.));
#185274=CARTESIAN_POINT('',(7.33627833380045,-20.7347298079577,0.));
#185275=CARTESIAN_POINT('Origin',(2.70312158620511E-13,-7.32141292029404E-13,
0.));
#185276=CARTESIAN_POINT('Origin',(2.70312158620511E-13,-7.32141292029404E-13,
0.));
#185277=CARTESIAN_POINT('Origin',(3.52235856495312,-21.7161918885403,0.));
#185278=CARTESIAN_POINT('',(3.44230496120418,-21.2226420728916,0.));
#185279=CARTESIAN_POINT('',(4.01396149767428,-21.624941921198,0.));
#185280=CARTESIAN_POINT('Origin',(3.52235856495312,-21.7161918885403,0.));
#185281=CARTESIAN_POINT('',(4.01396149767428,-21.624941921198,0.));
#185282=CARTESIAN_POINT('',(3.44230496120418,-21.2226420728916,0.));
#185283=CARTESIAN_POINT('Origin',(4.11585220600461,-22.1738711152697,0.));
#185284=CARTESIAN_POINT('',(4.11585220600461,-22.1738711152697,0.));
#185285=CARTESIAN_POINT('',(2.05792610300232,-11.0869355576349,0.));
#185286=CARTESIAN_POINT('',(4.11585220600461,-22.1738711152697,0.));
#185287=CARTESIAN_POINT('Origin',(2.21822694051637,-21.8878840740801,0.));
#185288=CARTESIAN_POINT('',(1.71975774210841,-21.9269795755927,0.));
#185289=CARTESIAN_POINT('',(2.16781269186827,-21.3904321633055,0.));
#185290=CARTESIAN_POINT('Origin',(2.21822694051637,-21.8878840740801,0.));
#185291=CARTESIAN_POINT('',(2.16781269186827,-21.3904321633055,0.));
#185292=CARTESIAN_POINT('',(1.71975774210841,-21.9269795755927,0.));
#185293=CARTESIAN_POINT('Origin',(7.16093850883225E-14,-7.7715611723761E-13,
0.));
#185294=CARTESIAN_POINT('Origin',(7.16093850883225E-14,-7.7715611723761E-13,
0.));
#185295=CARTESIAN_POINT('Origin',(-2.21822694051639,-21.88788407408,0.));
#185296=CARTESIAN_POINT('',(-2.16781269186829,-21.3904321633055,0.));
#185297=CARTESIAN_POINT('',(-1.71975774210843,-21.9269795755927,0.));
#185298=CARTESIAN_POINT('Origin',(-2.21822694051639,-21.88788407408,0.));
#185299=CARTESIAN_POINT('',(-1.71975774210843,-21.9269795755927,0.));
#185300=CARTESIAN_POINT('',(-2.16781269186829,-21.3904321633055,0.));
#185301=CARTESIAN_POINT('Origin',(-1.76341220531181,-22.4835757167854,0.));
#185302=CARTESIAN_POINT('',(-1.76341220531181,-22.4835757167854,0.));
#185303=CARTESIAN_POINT('',(-0.881706102655891,-11.2417878583927,0.));
#185304=CARTESIAN_POINT('',(-1.76341220531181,-22.4835757167854,0.));
#185305=CARTESIAN_POINT('Origin',(-3.52235856495314,-21.7161918885402,0.));
#185306=CARTESIAN_POINT('',(-4.0139614976743,-21.624941921198,0.));
#185307=CARTESIAN_POINT('',(-3.4423049612042,-21.2226420728916,0.));
#185308=CARTESIAN_POINT('Origin',(-3.52235856495314,-21.7161918885402,0.));
#185309=CARTESIAN_POINT('',(-3.4423049612042,-21.2226420728916,0.));
#185310=CARTESIAN_POINT('',(-4.0139614976743,-21.624941921198,0.));
#185311=CARTESIAN_POINT('Origin',(-1.31973449697531E-13,-7.6920903736728E-13,
0.));
#185312=CARTESIAN_POINT('Origin',(-1.31973449697531E-13,-7.6920903736728E-13,
0.));
#185313=CARTESIAN_POINT('Origin',(-7.80764394578304,-20.56795313141,0.));
#185314=CARTESIAN_POINT('',(-7.63019749246979,-20.1004996511507,0.));
#185315=CARTESIAN_POINT('',(-7.33627833380047,-20.7347298079577,0.));
#185316=CARTESIAN_POINT('Origin',(-7.80764394578304,-20.56795313141,0.));
#185317=CARTESIAN_POINT('',(-7.33627833380047,-20.7347298079577,0.));
#185318=CARTESIAN_POINT('',(-7.63019749246979,-20.1004996511507,0.));
#185319=CARTESIAN_POINT('Origin',(-7.52250298901266,-21.2610617890679,0.));
#185320=CARTESIAN_POINT('',(-7.52250298901266,-21.2610617890679,0.));
#185321=CARTESIAN_POINT('',(-3.76125149450632,-10.6305308945339,0.));
#185322=CARTESIAN_POINT('',(-7.52250298901266,-21.2610617890679,0.));
#185323=CARTESIAN_POINT('Origin',(-9.02290115519382,-20.0645771135003,0.));
#185324=CARTESIAN_POINT('',(-9.47413589477549,-19.84920021178,0.));
#185325=CARTESIAN_POINT('',(-8.81783521984851,-19.6085639972844,0.));
#185326=CARTESIAN_POINT('Origin',(-9.02290115519382,-20.0645771135003,0.));
#185327=CARTESIAN_POINT('',(-8.81783521984851,-19.6085639972844,0.));
#185328=CARTESIAN_POINT('',(-9.47413589477549,-19.84920021178,0.));
#185329=CARTESIAN_POINT('Origin',(-3.26562511982935E-13,-7.08841632778409E-13,
0.));
#185330=CARTESIAN_POINT('Origin',(-3.26562511982935E-13,-7.08841632778409E-13,
0.));
#185331=CARTESIAN_POINT('Origin',(-12.8649829188863,-17.846350172984,0.));
#185332=CARTESIAN_POINT('',(-12.572596943457,-17.4407513054161,0.));
#185333=CARTESIAN_POINT('',(-12.4528436808172,-18.1294424696716,0.));
#185334=CARTESIAN_POINT('Origin',(-12.8649829188863,-17.846350172984,0.));
#185335=CARTESIAN_POINT('',(-12.4528436808172,-18.1294424696716,0.));
#185336=CARTESIAN_POINT('',(-12.572596943457,-17.4407513054161,0.));
#185337=CARTESIAN_POINT('Origin',(-12.7689476255363,-18.5896416359912,0.));
#185338=CARTESIAN_POINT('',(-12.7689476255363,-18.5896416359912,0.));
#185339=CARTESIAN_POINT('',(-6.38447381276812,-9.29482081799561,0.));
#185340=CARTESIAN_POINT('',(-12.7689476255363,-18.5896416359912,0.));
#185341=CARTESIAN_POINT('Origin',(-13.9085479427572,-17.0455945664569,0.));
#185342=CARTESIAN_POINT('',(-14.2886635873976,-16.7207683102834,0.));
#185343=CARTESIAN_POINT('',(-13.5924445804218,-16.6581946899465,0.));
#185344=CARTESIAN_POINT('Origin',(-13.9085479427572,-17.0455945664569,0.));
#185345=CARTESIAN_POINT('',(-13.5924445804218,-16.6581946899465,0.));
#185346=CARTESIAN_POINT('',(-14.2886635873976,-16.7207683102834,0.));
#185347=CARTESIAN_POINT('Origin',(-4.9889687874677E-13,-6.00167842331873E-13,
0.));
#185348=CARTESIAN_POINT('Origin',(-4.9889687874677E-13,-6.00167842331873E-13,
0.));
#185349=CARTESIAN_POINT('Origin',(-17.0455945664569,-13.9085479427572,0.));
#185350=CARTESIAN_POINT('',(-16.6581946899465,-13.5924445804218,0.));
#185351=CARTESIAN_POINT('',(-16.7207683102834,-14.2886635873976,0.));
#185352=CARTESIAN_POINT('Origin',(-17.0455945664569,-13.9085479427572,0.));
#185353=CARTESIAN_POINT('',(-16.7207683102834,-14.2886635873976,0.));
#185354=CARTESIAN_POINT('',(-16.6581946899465,-13.5924445804218,0.));
#185355=CARTESIAN_POINT('Origin',(-17.1452095830633,-14.6513681262571,0.));
#185356=CARTESIAN_POINT('',(-17.1452095830633,-14.6513681262571,0.));
#185357=CARTESIAN_POINT('',(-8.57260479153162,-7.32568406312855,0.));
#185358=CARTESIAN_POINT('',(-17.1452095830633,-14.6513681262571,0.));
#185359=CARTESIAN_POINT('Origin',(-17.846350172984,-12.8649829188862,0.));
#185360=CARTESIAN_POINT('',(-18.1294424696716,-12.4528436808172,0.));
#185361=CARTESIAN_POINT('',(-17.4407513054162,-12.572596943457,0.));
#185362=CARTESIAN_POINT('Origin',(-17.846350172984,-12.8649829188862,0.));
#185363=CARTESIAN_POINT('',(-17.4407513054162,-12.572596943457,0.));
#185364=CARTESIAN_POINT('',(-18.1294424696716,-12.4528436808172,0.));
#185365=CARTESIAN_POINT('Origin',(-6.37232247690086E-13,-4.50593605254675E-13,
0.));
#185366=CARTESIAN_POINT('Origin',(-6.37232247690086E-13,-4.50593605254675E-13,
0.));
#185367=CARTESIAN_POINT('Origin',(-20.0645771135004,-9.0229011551938,0.));
#185368=CARTESIAN_POINT('',(-19.6085639972844,-8.81783521984849,0.));
#185369=CARTESIAN_POINT('',(-19.84920021178,-9.47413589477548,0.));
#185370=CARTESIAN_POINT('Origin',(-20.0645771135004,-9.0229011551938,0.));
#185371=CARTESIAN_POINT('',(-19.84920021178,-9.47413589477547,0.));
#185372=CARTESIAN_POINT('',(-19.6085639972844,-8.81783521984849,0.));
#185373=CARTESIAN_POINT('Origin',(-20.353053841303,-9.71462809124915,0.));
#185374=CARTESIAN_POINT('',(-20.353053841303,-9.71462809124915,0.));
#185375=CARTESIAN_POINT('',(-10.1765269206515,-4.85731404562459,0.));
#185376=CARTESIAN_POINT('',(-20.353053841303,-9.71462809124915,0.));
#185377=CARTESIAN_POINT('Origin',(-20.56795313141,-7.80764394578302,0.));
#185378=CARTESIAN_POINT('',(-20.7347298079577,-7.33627833380045,0.));
#185379=CARTESIAN_POINT('',(-20.1004996511507,-7.63019749246977,0.));
#185380=CARTESIAN_POINT('Origin',(-20.56795313141,-7.80764394578302,0.));
#185381=CARTESIAN_POINT('',(-20.1004996511507,-7.63019749246977,0.));
#185382=CARTESIAN_POINT('',(-20.7347298079577,-7.33627833380045,0.));
#185383=CARTESIAN_POINT('Origin',(-7.32141292029404E-13,-2.70312158620511E-13,
0.));
#185384=CARTESIAN_POINT('Origin',(-7.32141292029404E-13,-2.70312158620511E-13,
0.));
#185385=CARTESIAN_POINT('Origin',(-21.7161918885403,-3.52235856495312,0.));
#185386=CARTESIAN_POINT('',(-21.2226420728916,-3.44230496120418,0.));
#185387=CARTESIAN_POINT('',(-21.624941921198,-4.01396149767428,0.));
#185388=CARTESIAN_POINT('Origin',(-21.7161918885403,-3.52235856495312,0.));
#185389=CARTESIAN_POINT('',(-21.624941921198,-4.01396149767428,0.));
#185390=CARTESIAN_POINT('',(-21.2226420728916,-3.44230496120418,0.));
#185391=CARTESIAN_POINT('Origin',(-22.1738711152697,-4.11585220600461,0.));
#185392=CARTESIAN_POINT('',(-22.1738711152697,-4.11585220600461,0.));
#185393=CARTESIAN_POINT('',(-11.0869355576349,-2.05792610300232,0.));
#185394=CARTESIAN_POINT('',(-22.1738711152697,-4.11585220600461,0.));
#185395=CARTESIAN_POINT('Origin',(-21.8878840740801,-2.21822694051637,0.));
#185396=CARTESIAN_POINT('',(-21.9269795755927,-1.71975774210841,0.));
#185397=CARTESIAN_POINT('',(-21.3904321633055,-2.16781269186828,0.));
#185398=CARTESIAN_POINT('Origin',(-21.8878840740801,-2.21822694051637,0.));
#185399=CARTESIAN_POINT('',(-21.3904321633055,-2.16781269186827,0.));
#185400=CARTESIAN_POINT('',(-21.9269795755927,-1.71975774210841,0.));
#185401=CARTESIAN_POINT('Origin',(-7.7715611723761E-13,-7.16093850883225E-14,
0.));
#185402=CARTESIAN_POINT('Origin',(-7.7715611723761E-13,-7.16093850883225E-14,
0.));
#185403=CARTESIAN_POINT('Origin',(-21.8878840740801,2.21822694051638,0.));
#185404=CARTESIAN_POINT('',(-21.3904321633055,2.16781269186828,0.));
#185405=CARTESIAN_POINT('',(-21.9269795755927,1.71975774210842,0.));
#185406=CARTESIAN_POINT('Origin',(-21.8878840740801,2.21822694051638,0.));
#185407=CARTESIAN_POINT('',(-21.9269795755927,1.71975774210842,0.));
#185408=CARTESIAN_POINT('',(-21.3904321633055,2.16781269186828,0.));
#185409=CARTESIAN_POINT('Origin',(-22.4835757167854,1.7634122053118,0.));
#185410=CARTESIAN_POINT('',(-22.4835757167854,1.7634122053118,0.));
#185411=CARTESIAN_POINT('',(-11.2417878583927,0.881706102655883,0.));
#185412=CARTESIAN_POINT('',(-22.4835757167854,1.7634122053118,0.));
#185413=CARTESIAN_POINT('Origin',(-21.7161918885402,3.52235856495312,0.));
#185414=CARTESIAN_POINT('',(-21.624941921198,4.01396149767429,0.));
#185415=CARTESIAN_POINT('',(-21.2226420728916,3.44230496120419,0.));
#185416=CARTESIAN_POINT('Origin',(-21.7161918885402,3.52235856495312,0.));
#185417=CARTESIAN_POINT('',(-21.2226420728916,3.44230496120419,0.));
#185418=CARTESIAN_POINT('',(-21.624941921198,4.01396149767429,0.));
#185419=CARTESIAN_POINT('Origin',(-7.6920903736728E-13,1.31973449697531E-13,
0.));
#185420=CARTESIAN_POINT('Origin',(-7.6920903736728E-13,1.31973449697531E-13,
0.));
#185421=CARTESIAN_POINT('Origin',(-20.56795313141,7.80764394578303,0.));
#185422=CARTESIAN_POINT('',(-20.1004996511507,7.63019749246978,0.));
#185423=CARTESIAN_POINT('',(-20.7347298079577,7.33627833380047,0.));
#185424=CARTESIAN_POINT('Origin',(-20.56795313141,7.80764394578303,0.));
#185425=CARTESIAN_POINT('',(-20.7347298079577,7.33627833380047,0.));
#185426=CARTESIAN_POINT('',(-20.1004996511507,7.63019749246978,0.));
#185427=CARTESIAN_POINT('Origin',(-21.2610617890679,7.52250298901265,0.));
#185428=CARTESIAN_POINT('',(-21.2610617890679,7.52250298901265,0.));
#185429=CARTESIAN_POINT('',(-10.6305308945339,3.76125149450631,0.));
#185430=CARTESIAN_POINT('',(-21.2610617890679,7.52250298901265,0.));
#185431=CARTESIAN_POINT('Origin',(-20.0645771135003,9.02290115519382,0.));
#185432=CARTESIAN_POINT('',(-19.84920021178,9.47413589477549,0.));
#185433=CARTESIAN_POINT('',(-19.6085639972844,8.81783521984851,0.));
#185434=CARTESIAN_POINT('Origin',(-20.0645771135003,9.02290115519382,0.));
#185435=CARTESIAN_POINT('',(-19.6085639972844,8.81783521984851,0.));
#185436=CARTESIAN_POINT('',(-19.84920021178,9.47413589477549,0.));
#185437=CARTESIAN_POINT('Origin',(-7.08841632778408E-13,3.26562511982935E-13,
0.));
#185438=CARTESIAN_POINT('Origin',(-7.08841632778408E-13,3.26562511982935E-13,
0.));
#185439=CARTESIAN_POINT('Origin',(-17.846350172984,12.8649829188862,0.));
#185440=CARTESIAN_POINT('',(-17.4407513054162,12.572596943457,0.));
#185441=CARTESIAN_POINT('',(-18.1294424696716,12.4528436808172,0.));
#185442=CARTESIAN_POINT('Origin',(-17.846350172984,12.8649829188862,0.));
#185443=CARTESIAN_POINT('',(-18.1294424696716,12.4528436808172,0.));
#185444=CARTESIAN_POINT('',(-17.4407513054162,12.572596943457,0.));
#185445=CARTESIAN_POINT('Origin',(-18.5896416359912,12.7689476255363,0.));
#185446=CARTESIAN_POINT('',(-18.5896416359912,12.7689476255363,0.));
#185447=CARTESIAN_POINT('',(-9.29482081799561,6.38447381276812,0.));
#185448=CARTESIAN_POINT('',(-18.5896416359912,12.7689476255363,0.));
#185449=CARTESIAN_POINT('Origin',(-17.0455945664569,13.9085479427572,0.));
#185450=CARTESIAN_POINT('',(-16.7207683102834,14.2886635873976,0.));
#185451=CARTESIAN_POINT('',(-16.6581946899465,13.5924445804218,0.));
#185452=CARTESIAN_POINT('Origin',(-17.0455945664569,13.9085479427572,0.));
#185453=CARTESIAN_POINT('',(-16.6581946899465,13.5924445804218,0.));
#185454=CARTESIAN_POINT('',(-16.7207683102834,14.2886635873976,0.));
#185455=CARTESIAN_POINT('Origin',(-6.00167842331873E-13,4.9889687874677E-13,
0.));
#185456=CARTESIAN_POINT('Origin',(-6.00167842331873E-13,4.9889687874677E-13,
0.));
#185457=CARTESIAN_POINT('Origin',(-13.9085479427572,17.0455945664569,0.));
#185458=CARTESIAN_POINT('',(-13.5924445804218,16.6581946899465,0.));
#185459=CARTESIAN_POINT('',(-14.2886635873976,16.7207683102834,0.));
#185460=CARTESIAN_POINT('Origin',(-13.9085479427572,17.0455945664569,0.));
#185461=CARTESIAN_POINT('',(-14.2886635873976,16.7207683102834,0.));
#185462=CARTESIAN_POINT('',(-13.5924445804218,16.6581946899465,0.));
#185463=CARTESIAN_POINT('Origin',(-14.6513681262571,17.1452095830633,0.));
#185464=CARTESIAN_POINT('',(-14.6513681262571,17.1452095830633,0.));
#185465=CARTESIAN_POINT('',(-7.32568406312854,8.57260479153162,0.));
#185466=CARTESIAN_POINT('',(-14.6513681262571,17.1452095830633,0.));
#185467=CARTESIAN_POINT('Origin',(-12.8649829188862,17.846350172984,0.));
#185468=CARTESIAN_POINT('',(-12.4528436808172,18.1294424696716,0.));
#185469=CARTESIAN_POINT('',(-12.572596943457,17.4407513054162,0.));
#185470=CARTESIAN_POINT('Origin',(-12.8649829188862,17.846350172984,0.));
#185471=CARTESIAN_POINT('',(-12.572596943457,17.4407513054162,0.));
#185472=CARTESIAN_POINT('',(-12.4528436808172,18.1294424696716,0.));
#185473=CARTESIAN_POINT('Origin',(-4.50593605254675E-13,6.37232247690086E-13,
0.));
#185474=CARTESIAN_POINT('Origin',(-4.50593605254675E-13,6.37232247690086E-13,
0.));
#185475=CARTESIAN_POINT('Origin',(-9.02290115519381,20.0645771135003,0.));
#185476=CARTESIAN_POINT('',(-8.8178352198485,19.6085639972844,0.));
#185477=CARTESIAN_POINT('',(-9.47413589477548,19.84920021178,0.));
#185478=CARTESIAN_POINT('Origin',(-9.02290115519381,20.0645771135003,0.));
#185479=CARTESIAN_POINT('',(-9.47413589477548,19.84920021178,0.));
#185480=CARTESIAN_POINT('',(-8.8178352198485,19.6085639972844,0.));
#185481=CARTESIAN_POINT('Origin',(-9.71462809124916,20.353053841303,0.));
#185482=CARTESIAN_POINT('',(-9.71462809124916,20.353053841303,0.));
#185483=CARTESIAN_POINT('',(-4.85731404562459,10.1765269206515,0.));
#185484=CARTESIAN_POINT('',(-9.71462809124916,20.353053841303,0.));
#185485=CARTESIAN_POINT('Origin',(-7.80764394578302,20.56795313141,0.));
#185486=CARTESIAN_POINT('',(-7.33627833380046,20.7347298079577,0.));
#185487=CARTESIAN_POINT('',(-7.63019749246977,20.1004996511507,0.));
#185488=CARTESIAN_POINT('Origin',(-7.80764394578302,20.56795313141,0.));
#185489=CARTESIAN_POINT('',(-7.63019749246977,20.1004996511507,0.));
#185490=CARTESIAN_POINT('',(-7.33627833380046,20.7347298079577,0.));
#185491=CARTESIAN_POINT('Origin',(-2.70312158620511E-13,7.32141292029404E-13,
0.));
#185492=CARTESIAN_POINT('Origin',(-2.70312158620511E-13,7.32141292029404E-13,
0.));
#185493=CARTESIAN_POINT('Origin',(-3.52235856495312,21.7161918885402,0.));
#185494=CARTESIAN_POINT('',(-3.44230496120418,21.2226420728916,0.));
#185495=CARTESIAN_POINT('',(-4.01396149767428,21.624941921198,0.));
#185496=CARTESIAN_POINT('Origin',(-3.52235856495312,21.7161918885402,0.));
#185497=CARTESIAN_POINT('',(-4.01396149767428,21.624941921198,0.));
#185498=CARTESIAN_POINT('',(-3.44230496120418,21.2226420728916,0.));
#185499=CARTESIAN_POINT('Origin',(-4.11585220600461,22.1738711152697,0.));
#185500=CARTESIAN_POINT('',(-4.11585220600461,22.1738711152697,0.));
#185501=CARTESIAN_POINT('',(-2.05792610300232,11.0869355576349,0.));
#185502=CARTESIAN_POINT('',(-4.11585220600461,22.1738711152697,0.));
#185503=CARTESIAN_POINT('Origin',(-2.21822694051637,21.8878840740801,0.));
#185504=CARTESIAN_POINT('',(-1.71975774210841,21.9269795755927,0.));
#185505=CARTESIAN_POINT('',(-2.16781269186828,21.3904321633055,0.));
#185506=CARTESIAN_POINT('Origin',(-2.21822694051637,21.8878840740801,0.));
#185507=CARTESIAN_POINT('',(-2.16781269186828,21.3904321633055,0.));
#185508=CARTESIAN_POINT('',(-1.71975774210841,21.9269795755927,0.));
#185509=CARTESIAN_POINT('Origin',(-7.16093850883226E-14,7.7715611723761E-13,
0.));
#185510=CARTESIAN_POINT('Origin',(-7.16093850883226E-14,7.7715611723761E-13,
0.));
#185511=CARTESIAN_POINT('Origin',(2.21822694051638,21.8878840740801,0.));
#185512=CARTESIAN_POINT('',(2.16781269186828,21.3904321633055,0.));
#185513=CARTESIAN_POINT('',(1.71975774210842,21.9269795755927,0.));
#185514=CARTESIAN_POINT('Origin',(2.21822694051638,21.8878840740801,0.));
#185515=CARTESIAN_POINT('',(1.71975774210842,21.9269795755927,0.));
#185516=CARTESIAN_POINT('',(2.16781269186828,21.3904321633055,0.));
#185517=CARTESIAN_POINT('Origin',(1.7634122053118,22.4835757167854,0.));
#185518=CARTESIAN_POINT('',(1.7634122053118,22.4835757167854,0.));
#185519=CARTESIAN_POINT('',(0.881706102655883,11.2417878583927,0.));
#185520=CARTESIAN_POINT('',(1.7634122053118,22.4835757167854,0.));
#185521=CARTESIAN_POINT('Origin',(3.52235856495312,21.7161918885402,0.));
#185522=CARTESIAN_POINT('',(4.01396149767429,21.624941921198,0.));
#185523=CARTESIAN_POINT('',(3.44230496120419,21.2226420728916,0.));
#185524=CARTESIAN_POINT('Origin',(3.52235856495312,21.7161918885402,0.));
#185525=CARTESIAN_POINT('',(3.44230496120419,21.2226420728916,0.));
#185526=CARTESIAN_POINT('',(4.01396149767429,21.624941921198,0.));
#185527=CARTESIAN_POINT('Origin',(1.31973449697531E-13,7.6920903736728E-13,
0.));
#185528=CARTESIAN_POINT('Origin',(1.31973449697531E-13,7.6920903736728E-13,
0.));
#185529=CARTESIAN_POINT('Origin',(7.80764394578303,20.56795313141,0.));
#185530=CARTESIAN_POINT('',(7.63019749246978,20.1004996511507,0.));
#185531=CARTESIAN_POINT('',(7.33627833380047,20.7347298079577,0.));
#185532=CARTESIAN_POINT('Origin',(7.80764394578303,20.56795313141,0.));
#185533=CARTESIAN_POINT('',(7.33627833380046,20.7347298079577,0.));
#185534=CARTESIAN_POINT('',(7.63019749246978,20.1004996511507,0.));
#185535=CARTESIAN_POINT('Origin',(7.52250298901265,21.2610617890679,0.));
#185536=CARTESIAN_POINT('',(7.52250298901265,21.2610617890679,0.));
#185537=CARTESIAN_POINT('',(3.76125149450631,10.6305308945339,0.));
#185538=CARTESIAN_POINT('',(7.52250298901265,21.2610617890679,0.));
#185539=CARTESIAN_POINT('Origin',(9.02290115519382,20.0645771135003,0.));
#185540=CARTESIAN_POINT('',(9.47413589477549,19.84920021178,0.));
#185541=CARTESIAN_POINT('',(8.8178352198485,19.6085639972844,0.));
#185542=CARTESIAN_POINT('Origin',(9.02290115519382,20.0645771135003,0.));
#185543=CARTESIAN_POINT('',(8.8178352198485,19.6085639972844,0.));
#185544=CARTESIAN_POINT('',(9.47413589477549,19.84920021178,0.));
#185545=CARTESIAN_POINT('Origin',(3.26562511982935E-13,7.08841632778409E-13,
0.));
#185546=CARTESIAN_POINT('Origin',(3.26562511982935E-13,7.08841632778409E-13,
0.));
#185547=CARTESIAN_POINT('Origin',(12.8649829188862,17.846350172984,0.));
#185548=CARTESIAN_POINT('',(12.572596943457,17.4407513054162,0.));
#185549=CARTESIAN_POINT('',(12.4528436808172,18.1294424696716,0.));
#185550=CARTESIAN_POINT('Origin',(12.8649829188862,17.846350172984,0.));
#185551=CARTESIAN_POINT('',(12.4528436808172,18.1294424696716,0.));
#185552=CARTESIAN_POINT('',(12.572596943457,17.4407513054162,0.));
#185553=CARTESIAN_POINT('Origin',(12.7689476255363,18.5896416359912,0.));
#185554=CARTESIAN_POINT('',(12.7689476255363,18.5896416359912,0.));
#185555=CARTESIAN_POINT('',(6.38447381276812,9.29482081799561,0.));
#185556=CARTESIAN_POINT('',(12.7689476255363,18.5896416359912,0.));
#185557=CARTESIAN_POINT('Origin',(13.9085479427572,17.0455945664569,0.));
#185558=CARTESIAN_POINT('',(14.2886635873976,16.7207683102834,0.));
#185559=CARTESIAN_POINT('',(13.5924445804218,16.6581946899465,0.));
#185560=CARTESIAN_POINT('Origin',(13.9085479427572,17.0455945664569,0.));
#185561=CARTESIAN_POINT('',(13.5924445804218,16.6581946899465,0.));
#185562=CARTESIAN_POINT('',(14.2886635873976,16.7207683102834,0.));
#185563=CARTESIAN_POINT('Origin',(4.9889687874677E-13,6.00167842331873E-13,
0.));
#185564=CARTESIAN_POINT('Origin',(4.9889687874677E-13,6.00167842331873E-13,
0.));
#185565=CARTESIAN_POINT('Origin',(17.0455945664569,13.9085479427572,0.));
#185566=CARTESIAN_POINT('',(16.6581946899465,13.5924445804218,0.));
#185567=CARTESIAN_POINT('',(16.7207683102834,14.2886635873976,0.));
#185568=CARTESIAN_POINT('Origin',(17.0455945664569,13.9085479427572,0.));
#185569=CARTESIAN_POINT('',(16.7207683102834,14.2886635873976,0.));
#185570=CARTESIAN_POINT('',(16.6581946899465,13.5924445804218,0.));
#185571=CARTESIAN_POINT('Origin',(17.1452095830633,14.6513681262571,0.));
#185572=CARTESIAN_POINT('',(17.1452095830633,14.6513681262571,0.));
#185573=CARTESIAN_POINT('',(8.57260479153162,7.32568406312855,0.));
#185574=CARTESIAN_POINT('',(17.1452095830633,14.6513681262571,0.));
#185575=CARTESIAN_POINT('Origin',(17.846350172984,12.8649829188862,0.));
#185576=CARTESIAN_POINT('',(18.1294424696716,12.4528436808172,0.));
#185577=CARTESIAN_POINT('',(17.4407513054162,12.572596943457,0.));
#185578=CARTESIAN_POINT('Origin',(17.846350172984,12.8649829188862,0.));
#185579=CARTESIAN_POINT('',(17.4407513054162,12.572596943457,0.));
#185580=CARTESIAN_POINT('',(18.1294424696716,12.4528436808172,0.));
#185581=CARTESIAN_POINT('Origin',(6.37232247690086E-13,4.50593605254675E-13,
0.));
#185582=CARTESIAN_POINT('Origin',(6.37232247690086E-13,4.50593605254675E-13,
0.));
#185583=CARTESIAN_POINT('Origin',(20.0645771135003,9.02290115519381,0.));
#185584=CARTESIAN_POINT('',(19.6085639972844,8.8178352198485,0.));
#185585=CARTESIAN_POINT('',(19.84920021178,9.47413589477548,0.));
#185586=CARTESIAN_POINT('Origin',(20.0645771135003,9.02290115519381,0.));
#185587=CARTESIAN_POINT('',(19.84920021178,9.47413589477548,0.));
#185588=CARTESIAN_POINT('',(19.6085639972844,8.8178352198485,0.));
#185589=CARTESIAN_POINT('Origin',(20.353053841303,9.71462809124916,0.));
#185590=CARTESIAN_POINT('',(20.353053841303,9.71462809124916,0.));
#185591=CARTESIAN_POINT('',(10.1765269206515,4.85731404562459,0.));
#185592=CARTESIAN_POINT('',(20.353053841303,9.71462809124916,0.));
#185593=CARTESIAN_POINT('Origin',(20.56795313141,7.80764394578302,0.));
#185594=CARTESIAN_POINT('',(20.7347298079577,7.33627833380046,0.));
#185595=CARTESIAN_POINT('',(20.1004996511507,7.63019749246977,0.));
#185596=CARTESIAN_POINT('Origin',(20.56795313141,7.80764394578302,0.));
#185597=CARTESIAN_POINT('',(20.1004996511507,7.63019749246977,0.));
#185598=CARTESIAN_POINT('',(20.7347298079577,7.33627833380046,0.));
#185599=CARTESIAN_POINT('Origin',(7.32141292029404E-13,2.70312158620511E-13,
0.));
#185600=CARTESIAN_POINT('Origin',(7.32141292029404E-13,2.70312158620511E-13,
0.));
#185601=CARTESIAN_POINT('Origin',(21.1389261070099,-3.92374859571502,0.));
#185602=CARTESIAN_POINT('',(22.1738711152697,-4.11585220600463,0.));
#185603=CARTESIAN_POINT('',(22.1738711152697,-4.11585220600463,0.));
#185604=CARTESIAN_POINT('',(10.5694630535049,-1.96187429785751,0.));
#185605=CARTESIAN_POINT('Ctrl Pts',(25.991588367311,-0.661312440730916,
0.));
#185606=CARTESIAN_POINT('Ctrl Pts',(25.991588367311,-0.661312440730916,
12.));
#185607=CARTESIAN_POINT('Ctrl Pts',(25.9865613464773,-0.66402831318764,
0.));
#185608=CARTESIAN_POINT('Ctrl Pts',(25.9865613464773,-0.66402831318764,
12.));
#185609=CARTESIAN_POINT('Ctrl Pts',(25.9765104298071,-0.669451306780839,
0.));
#185610=CARTESIAN_POINT('Ctrl Pts',(25.9765104298071,-0.669451306780839,
12.));
#185611=CARTESIAN_POINT('Ctrl Pts',(25.9614434297919,-0.67755954320974,
0.));
#185612=CARTESIAN_POINT('Ctrl Pts',(25.9614434297919,-0.67755954320974,
12.));
#185613=CARTESIAN_POINT('Ctrl Pts',(25.9413728471909,-0.688318015057744,
0.));
#185614=CARTESIAN_POINT('Ctrl Pts',(25.9413728471909,-0.688318015057744,
12.));
#185615=CARTESIAN_POINT('Ctrl Pts',(25.9163158909426,-0.701678575228769,
0.));
#185616=CARTESIAN_POINT('Ctrl Pts',(25.9163158909426,-0.701678575228769,
12.));
#185617=CARTESIAN_POINT('Ctrl Pts',(25.8912902614969,-0.714951588527653,
0.));
#185618=CARTESIAN_POINT('Ctrl Pts',(25.8912902614969,-0.714951588527653,
12.));
#185619=CARTESIAN_POINT('Ctrl Pts',(25.8662960624185,-0.728137036482349,
0.));
#185620=CARTESIAN_POINT('Ctrl Pts',(25.8662960624185,-0.728137036482349,
12.));
#185621=CARTESIAN_POINT('Ctrl Pts',(25.8413334619054,-0.74123490266382,
0.));
#185622=CARTESIAN_POINT('Ctrl Pts',(25.8413334619054,-0.74123490266382,
12.));
#185623=CARTESIAN_POINT('Ctrl Pts',(25.8164027059984,-0.754245175609537,
0.));
#185624=CARTESIAN_POINT('Ctrl Pts',(25.8164027059984,-0.754245175609537,
12.));
#185625=CARTESIAN_POINT('Ctrl Pts',(25.7915041383376,-0.767167852651183,
0.));
#185626=CARTESIAN_POINT('Ctrl Pts',(25.7915041383376,-0.767167852651183,
12.));
#185627=CARTESIAN_POINT('Ctrl Pts',(25.7666381946955,-0.780002940291977,
0.));
#185628=CARTESIAN_POINT('Ctrl Pts',(25.7666381946955,-0.780002940291977,
12.));
#185629=CARTESIAN_POINT('Ctrl Pts',(25.7418053757746,-0.79275045161614,
0.));
#185630=CARTESIAN_POINT('Ctrl Pts',(25.7418053757746,-0.79275045161614,
12.));
#185631=CARTESIAN_POINT('Ctrl Pts',(25.7170062262525,-0.805410404554366,
0.));
#185632=CARTESIAN_POINT('Ctrl Pts',(25.7170062262525,-0.805410404554366,
12.));
#185633=CARTESIAN_POINT('Ctrl Pts',(25.6922413110194,-0.817982819787478,
0.));
#185634=CARTESIAN_POINT('Ctrl Pts',(25.6922413110194,-0.817982819787478,
12.));
#185635=CARTESIAN_POINT('Ctrl Pts',(25.6675111931952,-0.830467718864221,
0.));
#185636=CARTESIAN_POINT('Ctrl Pts',(25.6675111931952,-0.830467718864221,
12.));
#185637=CARTESIAN_POINT('Ctrl Pts',(25.6428164100055,-0.842865122120773,
0.));
#185638=CARTESIAN_POINT('Ctrl Pts',(25.6428164100055,-0.842865122120773,
12.));
#185639=CARTESIAN_POINT('Ctrl Pts',(25.6181574536049,-0.855175047036563,
0.));
#185640=CARTESIAN_POINT('Ctrl Pts',(25.6181574536049,-0.855175047036563,
12.));
#185641=CARTESIAN_POINT('Ctrl Pts',(25.5935347843585,-0.867397509338443,
0.));
#185642=CARTESIAN_POINT('Ctrl Pts',(25.5935347843585,-0.867397509338443,
12.));
#185643=CARTESIAN_POINT('Ctrl Pts',(25.5689488408156,-0.879532523834308,
0.));
#185644=CARTESIAN_POINT('Ctrl Pts',(25.5689488408156,-0.879532523834308,
12.));
#185645=CARTESIAN_POINT('Ctrl Pts',(25.5444000508211,-0.891580105349052,
0.));
#185646=CARTESIAN_POINT('Ctrl Pts',(25.5444000508211,-0.891580105349052,
12.));
#185647=CARTESIAN_POINT('Ctrl Pts',(25.5198888424194,-0.903540269651121,
0.));
#185648=CARTESIAN_POINT('Ctrl Pts',(25.5198888424194,-0.903540269651121,
12.));
#185649=CARTESIAN_POINT('Ctrl Pts',(25.4954156541795,-0.915413034335626,
0.));
#185650=CARTESIAN_POINT('Ctrl Pts',(25.4954156541795,-0.915413034335626,
12.));
#185651=CARTESIAN_POINT('Ctrl Pts',(25.4709809475009,-0.927198419886108,
0.));
#185652=CARTESIAN_POINT('Ctrl Pts',(25.4709809475009,-0.927198419886108,
12.));
#185653=CARTESIAN_POINT('Ctrl Pts',(25.4465852044849,-0.938896449496205,
0.));
#185654=CARTESIAN_POINT('Ctrl Pts',(25.4465852044849,-0.938896449496205,
12.));
#185655=CARTESIAN_POINT('Ctrl Pts',(25.4222289223167,-0.950507148597483,
0.));
#185656=CARTESIAN_POINT('Ctrl Pts',(25.4222289223167,-0.950507148597483,
12.));
#185657=CARTESIAN_POINT('Ctrl Pts',(25.3979126089163,-0.962030544503156,
0.));
#185658=CARTESIAN_POINT('Ctrl Pts',(25.3979126089163,-0.962030544503156,
12.));
#185659=CARTESIAN_POINT('Ctrl Pts',(25.3736367778845,-0.973466666000178,
0.));
#185660=CARTESIAN_POINT('Ctrl Pts',(25.3736367778845,-0.973466666000178,
12.));
#185661=CARTESIAN_POINT('Ctrl Pts',(25.3494019441441,-0.984815543003986,
0.));
#185662=CARTESIAN_POINT('Ctrl Pts',(25.3494019441441,-0.984815543003986,
12.));
#185663=CARTESIAN_POINT('Ctrl Pts',(25.3252086182968,-0.996077206120637,
0.));
#185664=CARTESIAN_POINT('Ctrl Pts',(25.3252086182968,-0.996077206120637,
12.));
#185665=CARTESIAN_POINT('Ctrl Pts',(25.3010573055547,-1.00725168656897,
0.));
#185666=CARTESIAN_POINT('Ctrl Pts',(25.3010573055547,-1.00725168656897,
12.));
#185667=CARTESIAN_POINT('Ctrl Pts',(25.276948508726,-1.01833901642238,0.));
#185668=CARTESIAN_POINT('Ctrl Pts',(25.276948508726,-1.01833901642238,12.));
#185669=CARTESIAN_POINT('Ctrl Pts',(25.2528827300422,-1.02933922876807,
0.));
#185670=CARTESIAN_POINT('Ctrl Pts',(25.2528827300422,-1.02933922876807,
12.));
#185671=CARTESIAN_POINT('Ctrl Pts',(25.2288604735086,-1.04025235791508,
0.));
#185672=CARTESIAN_POINT('Ctrl Pts',(25.2288604735086,-1.04025235791508,
12.));
#185673=CARTESIAN_POINT('Ctrl Pts',(25.2048822469028,-1.05107843957933,
0.));
#185674=CARTESIAN_POINT('Ctrl Pts',(25.2048822469028,-1.05107843957933,
12.));
#185675=CARTESIAN_POINT('Ctrl Pts',(25.1809485642192,-1.06181751111769,
0.));
#185676=CARTESIAN_POINT('Ctrl Pts',(25.1809485642192,-1.06181751111769,
12.));
#185677=CARTESIAN_POINT('Ctrl Pts',(25.157059946931,-1.07246961165477,0.));
#185678=CARTESIAN_POINT('Ctrl Pts',(25.157059946931,-1.07246961165477,12.));
#185679=CARTESIAN_POINT('Ctrl Pts',(25.1332169227413,-1.08303478197189,
0.));
#185680=CARTESIAN_POINT('Ctrl Pts',(25.1332169227413,-1.08303478197189,
12.));
#185681=CARTESIAN_POINT('Ctrl Pts',(25.1094200248446,-1.09351306445309,
0.));
#185682=CARTESIAN_POINT('Ctrl Pts',(25.1094200248446,-1.09351306445309,
12.));
#185683=CARTESIAN_POINT('Ctrl Pts',(25.0856697909679,-1.10390450301747,
0.));
#185684=CARTESIAN_POINT('Ctrl Pts',(25.0856697909679,-1.10390450301747,
12.));
#185685=CARTESIAN_POINT('Ctrl Pts',(25.0619667625336,-1.11420914306891,
0.));
#185686=CARTESIAN_POINT('Ctrl Pts',(25.0619667625336,-1.11420914306891,
12.));
#185687=CARTESIAN_POINT('Ctrl Pts',(25.0383114836899,-1.12442703144453,
0.));
#185688=CARTESIAN_POINT('Ctrl Pts',(25.0383114836899,-1.12442703144453,
12.));
#185689=CARTESIAN_POINT('Ctrl Pts',(25.0147045006195,-1.13455821638531,
0.));
#185690=CARTESIAN_POINT('Ctrl Pts',(25.0147045006195,-1.13455821638531,
12.));
#185691=CARTESIAN_POINT('Ctrl Pts',(24.9911463621433,-1.14460274758202,
0.));
#185692=CARTESIAN_POINT('Ctrl Pts',(24.9911463621433,-1.14460274758202,
12.));
#185693=CARTESIAN_POINT('Ctrl Pts',(24.9676376201502,-1.15456067621891,
0.));
#185694=CARTESIAN_POINT('Ctrl Pts',(24.9676376201502,-1.15456067621891,
12.));
#185695=CARTESIAN_POINT('Ctrl Pts',(24.9441788300932,-1.16443205502851,
0.));
#185696=CARTESIAN_POINT('Ctrl Pts',(24.9441788300932,-1.16443205502851,
12.));
#185697=CARTESIAN_POINT('Ctrl Pts',(24.9207705514448,-1.17421693835042,
0.));
#185698=CARTESIAN_POINT('Ctrl Pts',(24.9207705514448,-1.17421693835042,
12.));
#185699=CARTESIAN_POINT('Ctrl Pts',(24.8974133481829,-1.18391538220104,
0.));
#185700=CARTESIAN_POINT('Ctrl Pts',(24.8974133481829,-1.18391538220104,
12.));
#185701=CARTESIAN_POINT('Ctrl Pts',(24.8741077892075,-1.19352744434066,
0.));
#185702=CARTESIAN_POINT('Ctrl Pts',(24.8741077892075,-1.19352744434066,
12.));
#185703=CARTESIAN_POINT('Ctrl Pts',(24.8508544481974,-1.20305318426021,
0.));
#185704=CARTESIAN_POINT('Ctrl Pts',(24.8508544481974,-1.20305318426021,
12.));
#185705=CARTESIAN_POINT('Ctrl Pts',(24.8276539035092,-1.21249266318209,
0.));
#185706=CARTESIAN_POINT('Ctrl Pts',(24.8276539035092,-1.21249266318209,
12.));
#185707=CARTESIAN_POINT('Ctrl Pts',(24.8045067380536,-1.22184594406529,
0.));
#185708=CARTESIAN_POINT('Ctrl Pts',(24.8045067380536,-1.22184594406529,
12.));
#185709=CARTESIAN_POINT('Ctrl Pts',(24.7814135391799,-1.23111309161845,
0.));
#185710=CARTESIAN_POINT('Ctrl Pts',(24.7814135391799,-1.23111309161845,
12.));
#185711=CARTESIAN_POINT('Ctrl Pts',(24.7583748985438,-1.2402941723199,0.));
#185712=CARTESIAN_POINT('Ctrl Pts',(24.7583748985438,-1.2402941723199,12.));
#185713=CARTESIAN_POINT('Ctrl Pts',(24.7353914120011,-1.24938925444327,
0.));
#185714=CARTESIAN_POINT('Ctrl Pts',(24.7353914120011,-1.24938925444327,
12.));
#185715=CARTESIAN_POINT('Ctrl Pts',(24.7124636797894,-1.25839840807419,
0.));
#185716=CARTESIAN_POINT('Ctrl Pts',(24.7124636797894,-1.25839840807419,
12.));
#185717=CARTESIAN_POINT('Ctrl Pts',(24.6895923066836,-1.26732170513501,
0.));
#185718=CARTESIAN_POINT('Ctrl Pts',(24.6895923066836,-1.26732170513501,
12.));
#185719=CARTESIAN_POINT('Ctrl Pts',(24.6667779021559,-1.27615921941643,
0.));
#185720=CARTESIAN_POINT('Ctrl Pts',(24.6667779021559,-1.27615921941643,
12.));
#185721=CARTESIAN_POINT('Ctrl Pts',(24.6440210805278,-1.28491102661515,
0.));
#185722=CARTESIAN_POINT('Ctrl Pts',(24.6440210805278,-1.28491102661515,
12.));
#185723=CARTESIAN_POINT('Ctrl Pts',(24.6213224611229,-1.29357720438108,
0.));
#185724=CARTESIAN_POINT('Ctrl Pts',(24.6213224611229,-1.29357720438108,
12.));
#185725=CARTESIAN_POINT('Ctrl Pts',(24.5986826684027,-1.30215783236363,
0.));
#185726=CARTESIAN_POINT('Ctrl Pts',(24.5986826684027,-1.30215783236363,
12.));
#185727=CARTESIAN_POINT('Ctrl Pts',(24.5761023320183,-1.31065299222023,
0.));
#185728=CARTESIAN_POINT('Ctrl Pts',(24.5761023320183,-1.31065299222023,
12.));
#185729=CARTESIAN_POINT('Ctrl Pts',(24.5535820868674,-1.31906276763669,
0.));
#185730=CARTESIAN_POINT('Ctrl Pts',(24.5535820868674,-1.31906276763669,
12.));
#185731=CARTESIAN_POINT('Ctrl Pts',(24.5311225731435,-1.32738724435327,
0.));
#185732=CARTESIAN_POINT('Ctrl Pts',(24.5311225731435,-1.32738724435327,
12.));
#185733=CARTESIAN_POINT('Ctrl Pts',(24.5087244363856,-1.33562651019687,
0.));
#185734=CARTESIAN_POINT('Ctrl Pts',(24.5087244363856,-1.33562651019687,
12.));
#185735=CARTESIAN_POINT('Ctrl Pts',(24.4863883275134,-1.34378065512339,
0.));
#185736=CARTESIAN_POINT('Ctrl Pts',(24.4863883275134,-1.34378065512339,
12.));
#185737=CARTESIAN_POINT('Ctrl Pts',(24.4641149028892,-1.35184977125649,
0.));
#185738=CARTESIAN_POINT('Ctrl Pts',(24.4641149028892,-1.35184977125649,
12.));
#185739=CARTESIAN_POINT('Ctrl Pts',(24.4419048244523,-1.35983395290629,
0.));
#185740=CARTESIAN_POINT('Ctrl Pts',(24.4419048244523,-1.35983395290629,
12.));
#185741=CARTESIAN_POINT('Ctrl Pts',(24.4197587598337,-1.36773329659958,
0.));
#185742=CARTESIAN_POINT('Ctrl Pts',(24.4197587598337,-1.36773329659958,
12.));
#185743=CARTESIAN_POINT('Ctrl Pts',(24.3976773824732,-1.37554790111611,
0.));
#185744=CARTESIAN_POINT('Ctrl Pts',(24.3976773824732,-1.37554790111611,
12.));
#185745=CARTESIAN_POINT('Ctrl Pts',(24.3756613717299,-1.38327786753,0.));
#185746=CARTESIAN_POINT('Ctrl Pts',(24.3756613717299,-1.38327786753,12.));
#185747=CARTESIAN_POINT('Ctrl Pts',(24.3537114129875,-1.3909232992639,0.));
#185748=CARTESIAN_POINT('Ctrl Pts',(24.3537114129875,-1.3909232992639,12.));
#185749=CARTESIAN_POINT('Ctrl Pts',(24.3318281977643,-1.39848430212808,
0.));
#185750=CARTESIAN_POINT('Ctrl Pts',(24.3318281977643,-1.39848430212808,
12.));
#185751=CARTESIAN_POINT('Ctrl Pts',(24.3100124238311,-1.40596098434339,
0.));
#185752=CARTESIAN_POINT('Ctrl Pts',(24.3100124238311,-1.40596098434339,
12.));
#185753=CARTESIAN_POINT('Ctrl Pts',(24.288264795321,-1.41335345657684,0.));
#185754=CARTESIAN_POINT('Ctrl Pts',(24.288264795321,-1.41335345657684,12.));
#185755=CARTESIAN_POINT('Ctrl Pts',(24.2665860228356,-1.42066183198254,
0.));
#185756=CARTESIAN_POINT('Ctrl Pts',(24.2665860228356,-1.42066183198254,
12.));
#185757=CARTESIAN_POINT('Ctrl Pts',(24.2449768235488,-1.42788622624855,
0.));
#185758=CARTESIAN_POINT('Ctrl Pts',(24.2449768235488,-1.42788622624855,
12.));
#185759=CARTESIAN_POINT('Ctrl Pts',(24.2234379212984,-1.4350267576551,0.));
#185760=CARTESIAN_POINT('Ctrl Pts',(24.2234379212984,-1.4350267576551,12.));
#185761=CARTESIAN_POINT('Ctrl Pts',(24.201970046722,-1.44208354711083,0.));
#185762=CARTESIAN_POINT('Ctrl Pts',(24.201970046722,-1.44208354711083,12.));
#185763=CARTESIAN_POINT('Ctrl Pts',(24.1805739374038,-1.44905671818729,
0.));
#185764=CARTESIAN_POINT('Ctrl Pts',(24.1805739374038,-1.44905671818729,
12.));
#185765=CARTESIAN_POINT('Ctrl Pts',(24.1592503380107,-1.45594639716319,
0.));
#185766=CARTESIAN_POINT('Ctrl Pts',(24.1592503380107,-1.45594639716319,
12.));
#185767=CARTESIAN_POINT('Ctrl Pts',(24.1380000004272,-1.46275271307399,
0.));
#185768=CARTESIAN_POINT('Ctrl Pts',(24.1380000004272,-1.46275271307399,
12.));
#185769=CARTESIAN_POINT('Ctrl Pts',(24.1168236838824,-1.46947579776993,
0.));
#185770=CARTESIAN_POINT('Ctrl Pts',(24.1168236838824,-1.46947579776993,
12.));
#185771=CARTESIAN_POINT('Ctrl Pts',(24.0957221550778,-1.47611578597743,
0.));
#185772=CARTESIAN_POINT('Ctrl Pts',(24.0957221550778,-1.47611578597743,
12.));
#185773=CARTESIAN_POINT('Ctrl Pts',(24.0746961883528,-1.48267281533684,
0.));
#185774=CARTESIAN_POINT('Ctrl Pts',(24.0746961883528,-1.48267281533684,
12.));
#185775=CARTESIAN_POINT('Ctrl Pts',(24.0537465658429,-1.48914702644889,
0.));
#185776=CARTESIAN_POINT('Ctrl Pts',(24.0537465658429,-1.48914702644889,
12.));
#185777=CARTESIAN_POINT('Ctrl Pts',(24.0328740776331,-1.49553856292802,
0.));
#185778=CARTESIAN_POINT('Ctrl Pts',(24.0328740776331,-1.49553856292802,
12.));
#185779=CARTESIAN_POINT('Ctrl Pts',(24.0120795219086,-1.501847571461,0.));
#185780=CARTESIAN_POINT('Ctrl Pts',(24.0120795219086,-1.501847571461,12.));
#185781=CARTESIAN_POINT('Ctrl Pts',(23.9913637050927,-1.50807420187695,
0.));
#185782=CARTESIAN_POINT('Ctrl Pts',(23.9913637050927,-1.50807420187695,
12.));
#185783=CARTESIAN_POINT('Ctrl Pts',(23.970727442014,-1.51421860720616,0.));
#185784=CARTESIAN_POINT('Ctrl Pts',(23.970727442014,-1.51421860720616,12.));
#185785=CARTESIAN_POINT('Ctrl Pts',(23.9501715561033,-1.52028094372793,
0.));
#185786=CARTESIAN_POINT('Ctrl Pts',(23.9501715561033,-1.52028094372793,
12.));
#185787=CARTESIAN_POINT('Ctrl Pts',(23.9296968795757,-1.52626137103033,
0.));
#185788=CARTESIAN_POINT('Ctrl Pts',(23.9296968795757,-1.52626137103033,
12.));
#185789=CARTESIAN_POINT('Ctrl Pts',(23.9093042536119,-1.53216005207464,
0.));
#185790=CARTESIAN_POINT('Ctrl Pts',(23.9093042536119,-1.53216005207464,
12.));
#185791=CARTESIAN_POINT('Ctrl Pts',(23.8889945285318,-1.53797715326759,
0.));
#185792=CARTESIAN_POINT('Ctrl Pts',(23.8889945285318,-1.53797715326759,
12.));
#185793=CARTESIAN_POINT('Ctrl Pts',(23.8687685639642,-1.54371284453992,
0.));
#185794=CARTESIAN_POINT('Ctrl Pts',(23.8687685639642,-1.54371284453992,
12.));
#185795=CARTESIAN_POINT('Ctrl Pts',(23.8486272290705,-1.54936729940542,
0.));
#185796=CARTESIAN_POINT('Ctrl Pts',(23.8486272290705,-1.54936729940542,
12.));
#185797=CARTESIAN_POINT('Ctrl Pts',(23.8285714027636,-1.55494069502636,
0.));
#185798=CARTESIAN_POINT('Ctrl Pts',(23.8285714027636,-1.55494069502636,
12.));
#185799=CARTESIAN_POINT('Ctrl Pts',(23.8086019739194,-1.56043321228635,
0.));
#185800=CARTESIAN_POINT('Ctrl Pts',(23.8086019739194,-1.56043321228635,
12.));
#185801=CARTESIAN_POINT('Ctrl Pts',(23.7887198415878,-1.56584503586844,
0.));
#185802=CARTESIAN_POINT('Ctrl Pts',(23.7887198415878,-1.56584503586844,
12.));
#185803=CARTESIAN_POINT('Ctrl Pts',(23.7689259151862,-1.57117635434409,
0.));
#185804=CARTESIAN_POINT('Ctrl Pts',(23.7689259151862,-1.57117635434409,
12.));
#185805=CARTESIAN_POINT('Ctrl Pts',(23.749221114736,-1.57642736025247,0.));
#185806=CARTESIAN_POINT('Ctrl Pts',(23.749221114736,-1.57642736025247,12.));
#185807=CARTESIAN_POINT('Ctrl Pts',(23.72960637113,-1.58159825017359,0.));
#185808=CARTESIAN_POINT('Ctrl Pts',(23.72960637113,-1.58159825017359,12.));
#185809=CARTESIAN_POINT('Ctrl Pts',(23.710082626383,-1.58668922481222,0.));
#185810=CARTESIAN_POINT('Ctrl Pts',(23.710082626383,-1.58668922481222,12.));
#185811=CARTESIAN_POINT('Ctrl Pts',(23.6906508338833,-1.59170048908634,
0.));
#185812=CARTESIAN_POINT('Ctrl Pts',(23.6906508338833,-1.59170048908634,
12.));
#185813=CARTESIAN_POINT('Ctrl Pts',(23.671311958631,-1.59663225222464,0.));
#185814=CARTESIAN_POINT('Ctrl Pts',(23.671311958631,-1.59663225222464,12.));
#185815=CARTESIAN_POINT('Ctrl Pts',(23.6520669774876,-1.60148472786596,
0.));
#185816=CARTESIAN_POINT('Ctrl Pts',(23.6520669774876,-1.60148472786596,
12.));
#185817=CARTESIAN_POINT('Ctrl Pts',(23.6329168794929,-1.60625813414674,
0.));
#185818=CARTESIAN_POINT('Ctrl Pts',(23.6329168794929,-1.60625813414674,
12.));
#185819=CARTESIAN_POINT('Ctrl Pts',(23.6138626661653,-1.61095269379779,
0.));
#185820=CARTESIAN_POINT('Ctrl Pts',(23.6138626661653,-1.61095269379779,
12.));
#185821=CARTESIAN_POINT('Ctrl Pts',(23.5949053517997,-1.61556863424699,
0.));
#185822=CARTESIAN_POINT('Ctrl Pts',(23.5949053517997,-1.61556863424699,
12.));
#185823=CARTESIAN_POINT('Ctrl Pts',(23.57604596376,-1.62010618772867,0.));
#185824=CARTESIAN_POINT('Ctrl Pts',(23.57604596376,-1.62010618772867,12.));
#185825=CARTESIAN_POINT('Ctrl Pts',(23.5572855427601,-1.62456559140066,
0.));
#185826=CARTESIAN_POINT('Ctrl Pts',(23.5572855427601,-1.62456559140066,
12.));
#185827=CARTESIAN_POINT('Ctrl Pts',(23.538625143226,-1.62894708745224,0.));
#185828=CARTESIAN_POINT('Ctrl Pts',(23.538625143226,-1.62894708745224,12.));
#185829=CARTESIAN_POINT('Ctrl Pts',(23.5200658336612,-1.63325092321727,
0.));
#185830=CARTESIAN_POINT('Ctrl Pts',(23.5200658336612,-1.63325092321727,
12.));
#185831=CARTESIAN_POINT('Ctrl Pts',(23.5016086970003,-1.63747735129475,
0.));
#185832=CARTESIAN_POINT('Ctrl Pts',(23.5016086970003,-1.63747735129475,
12.));
#185833=CARTESIAN_POINT('Ctrl Pts',(23.4832548309645,-1.64162662967529,
0.));
#185834=CARTESIAN_POINT('Ctrl Pts',(23.4832548309645,-1.64162662967529,
12.));
#185835=CARTESIAN_POINT('Ctrl Pts',(23.4650053483932,-1.64569902187612,
0.));
#185836=CARTESIAN_POINT('Ctrl Pts',(23.4650053483932,-1.64569902187612,
12.));
#185837=CARTESIAN_POINT('Ctrl Pts',(23.4468613776574,-1.64969479707341,
0.));
#185838=CARTESIAN_POINT('Ctrl Pts',(23.4468613776574,-1.64969479707341,
12.));
#185839=CARTESIAN_POINT('Ctrl Pts',(23.4288240631043,-1.6536142302373,0.));
#185840=CARTESIAN_POINT('Ctrl Pts',(23.4288240631043,-1.6536142302373,12.));
#185841=CARTESIAN_POINT('Ctrl Pts',(23.4108945654805,-1.65745760227506,
0.));
#185842=CARTESIAN_POINT('Ctrl Pts',(23.4108945654805,-1.65745760227506,
12.));
#185843=CARTESIAN_POINT('Ctrl Pts',(23.3930740623619,-1.66122520018012,
0.));
#185844=CARTESIAN_POINT('Ctrl Pts',(23.3930740623619,-1.66122520018012,
12.));
#185845=CARTESIAN_POINT('Ctrl Pts',(23.3753637485545,-1.66491731718878,
0.));
#185846=CARTESIAN_POINT('Ctrl Pts',(23.3753637485545,-1.66491731718878,
12.));
#185847=CARTESIAN_POINT('Ctrl Pts',(23.3577648365744,-1.66853425293997,
0.));
#185848=CARTESIAN_POINT('Ctrl Pts',(23.3577648365744,-1.66853425293997,
12.));
#185849=CARTESIAN_POINT('Ctrl Pts',(23.3402785571865,-1.67207631363923,
0.));
#185850=CARTESIAN_POINT('Ctrl Pts',(23.3402785571865,-1.67207631363923,
12.));
#185851=CARTESIAN_POINT('Ctrl Pts',(23.3229061599144,-1.67554381222995,
0.));
#185852=CARTESIAN_POINT('Ctrl Pts',(23.3229061599144,-1.67554381222995,
12.));
#185853=CARTESIAN_POINT('Ctrl Pts',(23.3056489135611,-1.67893706857118,
0.));
#185854=CARTESIAN_POINT('Ctrl Pts',(23.3056489135611,-1.67893706857118,
12.));
#185855=CARTESIAN_POINT('Ctrl Pts',(23.2885081066951,-1.68225640962169,
0.));
#185856=CARTESIAN_POINT('Ctrl Pts',(23.2885081066951,-1.68225640962169,
12.));
#185857=CARTESIAN_POINT('Ctrl Pts',(23.2714850482246,-1.68550216963259,
0.));
#185858=CARTESIAN_POINT('Ctrl Pts',(23.2714850482246,-1.68550216963259,
12.));
#185859=CARTESIAN_POINT('Ctrl Pts',(23.2545810680537,-1.68867469034897,
0.));
#185860=CARTESIAN_POINT('Ctrl Pts',(23.2545810680537,-1.68867469034897,
12.));
#185861=CARTESIAN_POINT('Ctrl Pts',(23.2377975177013,-1.69177432121712,
0.));
#185862=CARTESIAN_POINT('Ctrl Pts',(23.2377975177013,-1.69177432121712,
12.));
#185863=CARTESIAN_POINT('Ctrl Pts',(23.2211357709374,-1.69480141959954,
0.));
#185864=CARTESIAN_POINT('Ctrl Pts',(23.2211357709374,-1.69480141959954,
12.));
#185865=CARTESIAN_POINT('Ctrl Pts',(23.2045972243767,-1.69775635099444,
0.));
#185866=CARTESIAN_POINT('Ctrl Pts',(23.2045972243767,-1.69775635099444,
12.));
#185867=CARTESIAN_POINT('Ctrl Pts',(23.1881832981851,-1.70063948927011,
0.));
#185868=CARTESIAN_POINT('Ctrl Pts',(23.1881832981851,-1.70063948927011,
12.));
#185869=CARTESIAN_POINT('Ctrl Pts',(23.1718954368751,-1.70345121691278,
0.));
#185870=CARTESIAN_POINT('Ctrl Pts',(23.1718954368751,-1.70345121691278,
12.));
#185871=CARTESIAN_POINT('Ctrl Pts',(23.1557351100614,-1.70619192527853,
0.));
#185872=CARTESIAN_POINT('Ctrl Pts',(23.1557351100614,-1.70619192527853,
12.));
#185873=CARTESIAN_POINT('Ctrl Pts',(23.1397038132356,-1.70886201485453,
0.));
#185874=CARTESIAN_POINT('Ctrl Pts',(23.1397038132356,-1.70886201485453,
12.));
#185875=CARTESIAN_POINT('Ctrl Pts',(23.1238030684925,-1.71146189552175,
0.));
#185876=CARTESIAN_POINT('Ctrl Pts',(23.1238030684925,-1.71146189552175,
12.));
#185877=CARTESIAN_POINT('Ctrl Pts',(23.1080344254286,-1.71399198684705,
0.));
#185878=CARTESIAN_POINT('Ctrl Pts',(23.1080344254286,-1.71399198684705,
12.));
#185879=CARTESIAN_POINT('Ctrl Pts',(23.0923994621213,-1.71645271839298,
0.));
#185880=CARTESIAN_POINT('Ctrl Pts',(23.0923994621213,-1.71645271839298,
12.));
#185881=CARTESIAN_POINT('Ctrl Pts',(23.0768997860708,-1.71884453003028,
0.));
#185882=CARTESIAN_POINT('Ctrl Pts',(23.0768997860708,-1.71884453003028,
12.));
#185883=CARTESIAN_POINT('Ctrl Pts',(23.0615370351562,-1.72116787225993,
0.));
#185884=CARTESIAN_POINT('Ctrl Pts',(23.0615370351562,-1.72116787225993,
12.));
#185885=CARTESIAN_POINT('Ctrl Pts',(23.0463128785531,-1.72342320653748,
0.));
#185886=CARTESIAN_POINT('Ctrl Pts',(23.0463128785531,-1.72342320653748,
12.));
#185887=CARTESIAN_POINT('Ctrl Pts',(23.0312290178883,-1.72561100564047,
0.));
#185888=CARTESIAN_POINT('Ctrl Pts',(23.0312290178883,-1.72561100564047,
12.));
#185889=CARTESIAN_POINT('Ctrl Pts',(23.0162871884168,-1.7277317540471,0.));
#185890=CARTESIAN_POINT('Ctrl Pts',(23.0162871884168,-1.7277317540471,12.));
#185891=CARTESIAN_POINT('Ctrl Pts',(23.001489160189,-1.72978594832137,0.));
#185892=CARTESIAN_POINT('Ctrl Pts',(23.001489160189,-1.72978594832137,12.));
#185893=CARTESIAN_POINT('Ctrl Pts',(22.9868367391978,-1.73177409750192,
0.));
#185894=CARTESIAN_POINT('Ctrl Pts',(22.9868367391978,-1.73177409750192,
12.));
#185895=CARTESIAN_POINT('Ctrl Pts',(22.9723317685688,-1.73369672350816,
0.));
#185896=CARTESIAN_POINT('Ctrl Pts',(22.9723317685688,-1.73369672350816,
12.));
#185897=CARTESIAN_POINT('Ctrl Pts',(22.9579761301063,-1.73555436162771,
0.));
#185898=CARTESIAN_POINT('Ctrl Pts',(22.9579761301063,-1.73555436162771,
12.));
#185899=CARTESIAN_POINT('Ctrl Pts',(22.9437717457826,-1.7373475610004,0.));
#185900=CARTESIAN_POINT('Ctrl Pts',(22.9437717457826,-1.7373475610004,12.));
#185901=CARTESIAN_POINT('Ctrl Pts',(22.9297205792586,-1.73907688511667,
0.));
#185902=CARTESIAN_POINT('Ctrl Pts',(22.9297205792586,-1.73907688511667,
12.));
#185903=CARTESIAN_POINT('Ctrl Pts',(22.9158246373363,-1.7407429123106,0.));
#185904=CARTESIAN_POINT('Ctrl Pts',(22.9158246373363,-1.7407429123106,12.));
#185905=CARTESIAN_POINT('Ctrl Pts',(22.9020859716141,-1.74234623630081,
0.));
#185906=CARTESIAN_POINT('Ctrl Pts',(22.9020859716141,-1.74234623630081,
12.));
#185907=CARTESIAN_POINT('Ctrl Pts',(22.888506680335,-1.74388746677704,0.));
#185908=CARTESIAN_POINT('Ctrl Pts',(22.888506680335,-1.74388746677704,12.));
#185909=CARTESIAN_POINT('Ctrl Pts',(22.8750889101696,-1.74536722998202,
0.));
#185910=CARTESIAN_POINT('Ctrl Pts',(22.8750889101696,-1.74536722998202,
12.));
#185911=CARTESIAN_POINT('Ctrl Pts',(22.8618348580235,-1.74678616930666,
0.));
#185912=CARTESIAN_POINT('Ctrl Pts',(22.8618348580235,-1.74678616930666,
12.));
#185913=CARTESIAN_POINT('Ctrl Pts',(22.8487467728076,-1.74814494588494,
0.));
#185914=CARTESIAN_POINT('Ctrl Pts',(22.8487467728076,-1.74814494588494,
12.));
#185915=CARTESIAN_POINT('Ctrl Pts',(22.8358269579853,-1.74944423940117,
0.));
#185916=CARTESIAN_POINT('Ctrl Pts',(22.8358269579853,-1.74944423940117,
12.));
#185917=CARTESIAN_POINT('Ctrl Pts',(22.8230777741284,-1.75068474890884,
0.));
#185918=CARTESIAN_POINT('Ctrl Pts',(22.8230777741284,-1.75068474890884,
12.));
#185919=CARTESIAN_POINT('Ctrl Pts',(22.8105016414713,-1.75186719365593,
0.));
#185920=CARTESIAN_POINT('Ctrl Pts',(22.8105016414713,-1.75186719365593,
12.));
#185921=CARTESIAN_POINT('Ctrl Pts',(22.7981010424314,-1.75299231391468,
0.));
#185922=CARTESIAN_POINT('Ctrl Pts',(22.7981010424314,-1.75299231391468,
12.));
#185923=CARTESIAN_POINT('Ctrl Pts',(22.7858785242361,-1.75406087182937,
0.));
#185924=CARTESIAN_POINT('Ctrl Pts',(22.7858785242361,-1.75406087182937,
12.));
#185925=CARTESIAN_POINT('Ctrl Pts',(22.7738367016118,-1.75507365227133,
0.));
#185926=CARTESIAN_POINT('Ctrl Pts',(22.7738367016118,-1.75507365227133,
12.));
#185927=CARTESIAN_POINT('Ctrl Pts',(22.7619782595013,-1.75603146371642,
0.));
#185928=CARTESIAN_POINT('Ctrl Pts',(22.7619782595013,-1.75603146371642,
12.));
#185929=CARTESIAN_POINT('Ctrl Pts',(22.750305955645,-1.75693513908908,0.));
#185930=CARTESIAN_POINT('Ctrl Pts',(22.750305955645,-1.75693513908908,12.));
#185931=CARTESIAN_POINT('Ctrl Pts',(22.7388226235559,-1.75778553673245,
0.));
#185932=CARTESIAN_POINT('Ctrl Pts',(22.7388226235559,-1.75778553673245,
12.));
#185933=CARTESIAN_POINT('Ctrl Pts',(22.72753117773,-1.75858354204634,0.));
#185934=CARTESIAN_POINT('Ctrl Pts',(22.72753117773,-1.75858354204634,12.));
#185935=CARTESIAN_POINT('Ctrl Pts',(22.7164346186006,-1.75933006905926,
0.));
#185936=CARTESIAN_POINT('Ctrl Pts',(22.7164346186006,-1.75933006905926,
12.));
#185937=CARTESIAN_POINT('Ctrl Pts',(22.7055360375485,-1.76002606202402,
0.));
#185938=CARTESIAN_POINT('Ctrl Pts',(22.7055360375485,-1.76002606202402,
12.));
#185939=CARTESIAN_POINT('Ctrl Pts',(22.6948386219851,-1.76067249704888,
0.));
#185940=CARTESIAN_POINT('Ctrl Pts',(22.6948386219851,-1.76067249704888,
12.));
#185941=CARTESIAN_POINT('Ctrl Pts',(22.684345658525,-1.76127038310615,0.));
#185942=CARTESIAN_POINT('Ctrl Pts',(22.684345658525,-1.76127038310615,12.));
#185943=CARTESIAN_POINT('Ctrl Pts',(22.67406053567,-1.76182076289527,0.));
#185944=CARTESIAN_POINT('Ctrl Pts',(22.67406053567,-1.76182076289527,12.));
#185945=CARTESIAN_POINT('Ctrl Pts',(22.6639867471753,-1.7623247139257,0.));
#185946=CARTESIAN_POINT('Ctrl Pts',(22.6639867471753,-1.7623247139257,12.));
#185947=CARTESIAN_POINT('Ctrl Pts',(22.6541278938409,-1.76278334912562,
0.));
#185948=CARTESIAN_POINT('Ctrl Pts',(22.6541278938409,-1.76278334912562,
12.));
#185949=CARTESIAN_POINT('Ctrl Pts',(22.6444876940423,-1.76319782013917,
0.));
#185950=CARTESIAN_POINT('Ctrl Pts',(22.6444876940423,-1.76319782013917,
12.));
#185951=CARTESIAN_POINT('Ctrl Pts',(22.6350699979359,-1.76356932176274,
0.));
#185952=CARTESIAN_POINT('Ctrl Pts',(22.6350699979359,-1.76356932176274,
12.));
#185953=CARTESIAN_POINT('Ctrl Pts',(22.6258787994848,-1.76389909571404,
0.));
#185954=CARTESIAN_POINT('Ctrl Pts',(22.6258787994848,-1.76389909571404,
12.));
#185955=CARTESIAN_POINT('Ctrl Pts',(22.6169182517694,-1.76418843543741,
0.));
#185956=CARTESIAN_POINT('Ctrl Pts',(22.6169182517694,-1.76418843543741,
12.));
#185957=CARTESIAN_POINT('Ctrl Pts',(22.6081926681343,-1.76443868648017,
0.));
#185958=CARTESIAN_POINT('Ctrl Pts',(22.6081926681343,-1.76443868648017,
12.));
#185959=CARTESIAN_POINT('Ctrl Pts',(22.5997065145638,-1.76465124413558,
0.));
#185960=CARTESIAN_POINT('Ctrl Pts',(22.5997065145638,-1.76465124413558,
12.));
#185961=CARTESIAN_POINT('Ctrl Pts',(22.5914644078105,-1.76482755288412,
0.));
#185962=CARTESIAN_POINT('Ctrl Pts',(22.5914644078105,-1.76482755288412,
12.));
#185963=CARTESIAN_POINT('Ctrl Pts',(22.5834711038022,-1.76496910283089,
0.));
#185964=CARTESIAN_POINT('Ctrl Pts',(22.5834711038022,-1.76496910283089,
12.));
#185965=CARTESIAN_POINT('Ctrl Pts',(22.5757315316353,-1.76507744026747,
0.));
#185966=CARTESIAN_POINT('Ctrl Pts',(22.5757315316353,-1.76507744026747,
12.));
#185967=CARTESIAN_POINT('Ctrl Pts',(22.5682508499873,-1.76515418518832,
0.));
#185968=CARTESIAN_POINT('Ctrl Pts',(22.5682508499873,-1.76515418518832,
12.));
#185969=CARTESIAN_POINT('Ctrl Pts',(22.5610344912501,-1.76520104500451,
0.));
#185970=CARTESIAN_POINT('Ctrl Pts',(22.5610344912501,-1.76520104500451,
12.));
#185971=CARTESIAN_POINT('Ctrl Pts',(22.5540882235837,-1.76521983384064,
0.));
#185972=CARTESIAN_POINT('Ctrl Pts',(22.5540882235837,-1.76521983384064,
12.));
#185973=CARTESIAN_POINT('Ctrl Pts',(22.5474180954006,-1.76521245524048,
0.));
#185974=CARTESIAN_POINT('Ctrl Pts',(22.5474180954006,-1.76521245524048,
12.));
#185975=CARTESIAN_POINT('Ctrl Pts',(22.5410303590892,-1.76518087841494,
0.));
#185976=CARTESIAN_POINT('Ctrl Pts',(22.5410303590892,-1.76518087841494,
12.));
#185977=CARTESIAN_POINT('Ctrl Pts',(22.5349313983571,-1.76512711563255,
0.));
#185978=CARTESIAN_POINT('Ctrl Pts',(22.5349313983571,-1.76512711563255,
12.));
#185979=CARTESIAN_POINT('Ctrl Pts',(22.529127665298,-1.7650532026276,0.));
#185980=CARTESIAN_POINT('Ctrl Pts',(22.529127665298,-1.7650532026276,12.));
#185981=CARTESIAN_POINT('Ctrl Pts',(22.5236259635515,-1.76496128643376,
0.));
#185982=CARTESIAN_POINT('Ctrl Pts',(22.5236259635515,-1.76496128643376,
12.));
#185983=CARTESIAN_POINT('Ctrl Pts',(22.5184336670207,-1.76485369319896,
0.));
#185984=CARTESIAN_POINT('Ctrl Pts',(22.5184336670207,-1.76485369319896,
12.));
#185985=CARTESIAN_POINT('Ctrl Pts',(22.5135590569554,-1.7647330328115,0.));
#185986=CARTESIAN_POINT('Ctrl Pts',(22.5135590569554,-1.7647330328115,12.));
#185987=CARTESIAN_POINT('Ctrl Pts',(22.5090112700212,-1.76460218257314,
0.));
#185988=CARTESIAN_POINT('Ctrl Pts',(22.5090112700212,-1.76460218257314,
12.));
#185989=CARTESIAN_POINT('Ctrl Pts',(22.5047996391978,-1.76446408210366,
0.));
#185990=CARTESIAN_POINT('Ctrl Pts',(22.5047996391978,-1.76446408210366,
12.));
#185991=CARTESIAN_POINT('Ctrl Pts',(22.5009332677316,-1.76432160068739,
0.));
#185992=CARTESIAN_POINT('Ctrl Pts',(22.5009332677316,-1.76432160068739,
12.));
#185993=CARTESIAN_POINT('Ctrl Pts',(22.4974203063191,-1.76417731243484,
0.));
#185994=CARTESIAN_POINT('Ctrl Pts',(22.4974203063191,-1.76417731243484,
12.));
#185995=CARTESIAN_POINT('Ctrl Pts',(22.4942693792449,-1.76403393880317,
0.));
#185996=CARTESIAN_POINT('Ctrl Pts',(22.4942693792449,-1.76403393880317,
12.));
#185997=CARTESIAN_POINT('Ctrl Pts',(22.4914909094908,-1.76389475965715,
0.));
#185998=CARTESIAN_POINT('Ctrl Pts',(22.4914909094908,-1.76389475965715,
12.));
#185999=CARTESIAN_POINT('Ctrl Pts',(22.4890991659479,-1.76376424879469,
0.));
#186000=CARTESIAN_POINT('Ctrl Pts',(22.4890991659479,-1.76376424879469,
12.));
#186001=CARTESIAN_POINT('Ctrl Pts',(22.4871115206572,-1.76364784232927,
0.));
#186002=CARTESIAN_POINT('Ctrl Pts',(22.4871115206572,-1.76364784232927,
12.));
#186003=CARTESIAN_POINT('Ctrl Pts',(22.4855446605991,-1.7635507604555,0.));
#186004=CARTESIAN_POINT('Ctrl Pts',(22.4855446605991,-1.7635507604555,12.));
#186005=CARTESIAN_POINT('Ctrl Pts',(22.4844112933125,-1.76347698284863,
0.));
#186006=CARTESIAN_POINT('Ctrl Pts',(22.4844112933125,-1.76347698284863,
12.));
#186007=CARTESIAN_POINT('Ctrl Pts',(22.4838562517064,-1.7634381343466,0.));
#186008=CARTESIAN_POINT('Ctrl Pts',(22.4838562517064,-1.7634381343466,12.));
#186009=CARTESIAN_POINT('Ctrl Pts',(22.4836387052228,-1.76342064263638,
0.));
#186010=CARTESIAN_POINT('Ctrl Pts',(22.4836387052228,-1.76342064263638,
12.));
#186011=CARTESIAN_POINT('Ctrl Pts',(22.4835819929788,-1.76341415538792,
0.));
#186012=CARTESIAN_POINT('Ctrl Pts',(22.4835819929788,-1.76341415538792,
12.));
#186013=CARTESIAN_POINT('Ctrl Pts',(22.4835757167854,-1.76341220531181,
0.));
#186014=CARTESIAN_POINT('Ctrl Pts',(22.4835757167854,-1.76341220531181,
12.));
#186015=CARTESIAN_POINT('',(25.991588367311,-0.661312440730916,0.));
#186016=CARTESIAN_POINT('Ctrl Pts',(25.991588367311,-0.661312440730916,
0.));
#186017=CARTESIAN_POINT('Ctrl Pts',(25.9865613464773,-0.66402831318764,
0.));
#186018=CARTESIAN_POINT('Ctrl Pts',(25.9765104298071,-0.669451306780839,
0.));
#186019=CARTESIAN_POINT('Ctrl Pts',(25.9614434297919,-0.67755954320974,
0.));
#186020=CARTESIAN_POINT('Ctrl Pts',(25.9413728471909,-0.688318015057744,
0.));
#186021=CARTESIAN_POINT('Ctrl Pts',(25.9163158909426,-0.701678575228769,
0.));
#186022=CARTESIAN_POINT('Ctrl Pts',(25.8912902614969,-0.714951588527653,
0.));
#186023=CARTESIAN_POINT('Ctrl Pts',(25.8662960624185,-0.728137036482349,
0.));
#186024=CARTESIAN_POINT('Ctrl Pts',(25.8413334619054,-0.74123490266382,
0.));
#186025=CARTESIAN_POINT('Ctrl Pts',(25.8164027059984,-0.754245175609537,
0.));
#186026=CARTESIAN_POINT('Ctrl Pts',(25.7915041383376,-0.767167852651183,
0.));
#186027=CARTESIAN_POINT('Ctrl Pts',(25.7666381946955,-0.780002940291977,
0.));
#186028=CARTESIAN_POINT('Ctrl Pts',(25.7418053757746,-0.79275045161614,
0.));
#186029=CARTESIAN_POINT('Ctrl Pts',(25.7170062262525,-0.805410404554366,
0.));
#186030=CARTESIAN_POINT('Ctrl Pts',(25.6922413110194,-0.817982819787478,
0.));
#186031=CARTESIAN_POINT('Ctrl Pts',(25.6675111931952,-0.830467718864221,
0.));
#186032=CARTESIAN_POINT('Ctrl Pts',(25.6428164100055,-0.842865122120773,
0.));
#186033=CARTESIAN_POINT('Ctrl Pts',(25.6181574536049,-0.855175047036563,
0.));
#186034=CARTESIAN_POINT('Ctrl Pts',(25.5935347843585,-0.867397509338443,
0.));
#186035=CARTESIAN_POINT('Ctrl Pts',(25.5689488408156,-0.879532523834308,
0.));
#186036=CARTESIAN_POINT('Ctrl Pts',(25.5444000508211,-0.891580105349052,
0.));
#186037=CARTESIAN_POINT('Ctrl Pts',(25.5198888424194,-0.903540269651121,
0.));
#186038=CARTESIAN_POINT('Ctrl Pts',(25.4954156541795,-0.915413034335626,
0.));
#186039=CARTESIAN_POINT('Ctrl Pts',(25.4709809475009,-0.927198419886108,
0.));
#186040=CARTESIAN_POINT('Ctrl Pts',(25.4465852044849,-0.938896449496205,
0.));
#186041=CARTESIAN_POINT('Ctrl Pts',(25.4222289223167,-0.950507148597483,
0.));
#186042=CARTESIAN_POINT('Ctrl Pts',(25.3979126089163,-0.962030544503156,
0.));
#186043=CARTESIAN_POINT('Ctrl Pts',(25.3736367778845,-0.973466666000178,
0.));
#186044=CARTESIAN_POINT('Ctrl Pts',(25.3494019441441,-0.984815543003986,
0.));
#186045=CARTESIAN_POINT('Ctrl Pts',(25.3252086182968,-0.996077206120637,
0.));
#186046=CARTESIAN_POINT('Ctrl Pts',(25.3010573055547,-1.00725168656897,
0.));
#186047=CARTESIAN_POINT('Ctrl Pts',(25.276948508726,-1.01833901642238,0.));
#186048=CARTESIAN_POINT('Ctrl Pts',(25.2528827300422,-1.02933922876807,
0.));
#186049=CARTESIAN_POINT('Ctrl Pts',(25.2288604735086,-1.04025235791508,
0.));
#186050=CARTESIAN_POINT('Ctrl Pts',(25.2048822469028,-1.05107843957933,
0.));
#186051=CARTESIAN_POINT('Ctrl Pts',(25.1809485642192,-1.06181751111769,
0.));
#186052=CARTESIAN_POINT('Ctrl Pts',(25.157059946931,-1.07246961165477,0.));
#186053=CARTESIAN_POINT('Ctrl Pts',(25.1332169227413,-1.08303478197189,
0.));
#186054=CARTESIAN_POINT('Ctrl Pts',(25.1094200248446,-1.09351306445309,
0.));
#186055=CARTESIAN_POINT('Ctrl Pts',(25.0856697909679,-1.10390450301747,
0.));
#186056=CARTESIAN_POINT('Ctrl Pts',(25.0619667625336,-1.11420914306891,
0.));
#186057=CARTESIAN_POINT('Ctrl Pts',(25.0383114836899,-1.12442703144453,
0.));
#186058=CARTESIAN_POINT('Ctrl Pts',(25.0147045006195,-1.13455821638531,
0.));
#186059=CARTESIAN_POINT('Ctrl Pts',(24.9911463621433,-1.14460274758202,
0.));
#186060=CARTESIAN_POINT('Ctrl Pts',(24.9676376201502,-1.15456067621891,
0.));
#186061=CARTESIAN_POINT('Ctrl Pts',(24.9441788300932,-1.16443205502851,
0.));
#186062=CARTESIAN_POINT('Ctrl Pts',(24.9207705514448,-1.17421693835042,
0.));
#186063=CARTESIAN_POINT('Ctrl Pts',(24.8974133481829,-1.18391538220104,
0.));
#186064=CARTESIAN_POINT('Ctrl Pts',(24.8741077892075,-1.19352744434066,
0.));
#186065=CARTESIAN_POINT('Ctrl Pts',(24.8508544481974,-1.20305318426021,
0.));
#186066=CARTESIAN_POINT('Ctrl Pts',(24.8276539035092,-1.21249266318209,
0.));
#186067=CARTESIAN_POINT('Ctrl Pts',(24.8045067380536,-1.22184594406529,
0.));
#186068=CARTESIAN_POINT('Ctrl Pts',(24.7814135391799,-1.23111309161845,
0.));
#186069=CARTESIAN_POINT('Ctrl Pts',(24.7583748985438,-1.2402941723199,0.));
#186070=CARTESIAN_POINT('Ctrl Pts',(24.7353914120011,-1.24938925444327,
0.));
#186071=CARTESIAN_POINT('Ctrl Pts',(24.7124636797894,-1.25839840807419,
0.));
#186072=CARTESIAN_POINT('Ctrl Pts',(24.6895923066836,-1.26732170513501,
0.));
#186073=CARTESIAN_POINT('Ctrl Pts',(24.6667779021559,-1.27615921941643,
0.));
#186074=CARTESIAN_POINT('Ctrl Pts',(24.6440210805278,-1.28491102661515,
0.));
#186075=CARTESIAN_POINT('Ctrl Pts',(24.6213224611229,-1.29357720438108,
0.));
#186076=CARTESIAN_POINT('Ctrl Pts',(24.5986826684027,-1.30215783236363,
0.));
#186077=CARTESIAN_POINT('Ctrl Pts',(24.5761023320183,-1.31065299222023,
0.));
#186078=CARTESIAN_POINT('Ctrl Pts',(24.5535820868674,-1.31906276763669,
0.));
#186079=CARTESIAN_POINT('Ctrl Pts',(24.5311225731435,-1.32738724435327,
0.));
#186080=CARTESIAN_POINT('Ctrl Pts',(24.5087244363856,-1.33562651019687,
0.));
#186081=CARTESIAN_POINT('Ctrl Pts',(24.4863883275134,-1.34378065512339,
0.));
#186082=CARTESIAN_POINT('Ctrl Pts',(24.4641149028892,-1.35184977125649,
0.));
#186083=CARTESIAN_POINT('Ctrl Pts',(24.4419048244523,-1.35983395290629,
0.));
#186084=CARTESIAN_POINT('Ctrl Pts',(24.4197587598337,-1.36773329659958,
0.));
#186085=CARTESIAN_POINT('Ctrl Pts',(24.3976773824732,-1.37554790111611,
0.));
#186086=CARTESIAN_POINT('Ctrl Pts',(24.3756613717299,-1.38327786753,0.));
#186087=CARTESIAN_POINT('Ctrl Pts',(24.3537114129875,-1.3909232992639,0.));
#186088=CARTESIAN_POINT('Ctrl Pts',(24.3318281977643,-1.39848430212808,
0.));
#186089=CARTESIAN_POINT('Ctrl Pts',(24.3100124238311,-1.40596098434339,
0.));
#186090=CARTESIAN_POINT('Ctrl Pts',(24.288264795321,-1.41335345657684,0.));
#186091=CARTESIAN_POINT('Ctrl Pts',(24.2665860228356,-1.42066183198254,
0.));
#186092=CARTESIAN_POINT('Ctrl Pts',(24.2449768235488,-1.42788622624855,
0.));
#186093=CARTESIAN_POINT('Ctrl Pts',(24.2234379212984,-1.4350267576551,0.));
#186094=CARTESIAN_POINT('Ctrl Pts',(24.201970046722,-1.44208354711083,0.));
#186095=CARTESIAN_POINT('Ctrl Pts',(24.1805739374038,-1.44905671818729,
0.));
#186096=CARTESIAN_POINT('Ctrl Pts',(24.1592503380107,-1.45594639716319,
0.));
#186097=CARTESIAN_POINT('Ctrl Pts',(24.1380000004272,-1.46275271307399,
0.));
#186098=CARTESIAN_POINT('Ctrl Pts',(24.1168236838824,-1.46947579776993,
0.));
#186099=CARTESIAN_POINT('Ctrl Pts',(24.0957221550778,-1.47611578597743,
0.));
#186100=CARTESIAN_POINT('Ctrl Pts',(24.0746961883528,-1.48267281533684,
0.));
#186101=CARTESIAN_POINT('Ctrl Pts',(24.0537465658429,-1.48914702644889,
0.));
#186102=CARTESIAN_POINT('Ctrl Pts',(24.0328740776331,-1.49553856292802,
0.));
#186103=CARTESIAN_POINT('Ctrl Pts',(24.0120795219086,-1.501847571461,0.));
#186104=CARTESIAN_POINT('Ctrl Pts',(23.9913637050927,-1.50807420187695,
0.));
#186105=CARTESIAN_POINT('Ctrl Pts',(23.970727442014,-1.51421860720616,0.));
#186106=CARTESIAN_POINT('Ctrl Pts',(23.9501715561033,-1.52028094372793,
0.));
#186107=CARTESIAN_POINT('Ctrl Pts',(23.9296968795757,-1.52626137103033,
0.));
#186108=CARTESIAN_POINT('Ctrl Pts',(23.9093042536119,-1.53216005207464,
0.));
#186109=CARTESIAN_POINT('Ctrl Pts',(23.8889945285318,-1.53797715326759,
0.));
#186110=CARTESIAN_POINT('Ctrl Pts',(23.8687685639642,-1.54371284453992,
0.));
#186111=CARTESIAN_POINT('Ctrl Pts',(23.8486272290705,-1.54936729940542,
0.));
#186112=CARTESIAN_POINT('Ctrl Pts',(23.8285714027636,-1.55494069502636,
0.));
#186113=CARTESIAN_POINT('Ctrl Pts',(23.8086019739194,-1.56043321228635,
0.));
#186114=CARTESIAN_POINT('Ctrl Pts',(23.7887198415878,-1.56584503586844,
0.));
#186115=CARTESIAN_POINT('Ctrl Pts',(23.7689259151862,-1.57117635434409,
0.));
#186116=CARTESIAN_POINT('Ctrl Pts',(23.749221114736,-1.57642736025247,0.));
#186117=CARTESIAN_POINT('Ctrl Pts',(23.72960637113,-1.58159825017359,0.));
#186118=CARTESIAN_POINT('Ctrl Pts',(23.710082626383,-1.58668922481222,0.));
#186119=CARTESIAN_POINT('Ctrl Pts',(23.6906508338833,-1.59170048908634,
0.));
#186120=CARTESIAN_POINT('Ctrl Pts',(23.671311958631,-1.59663225222464,0.));
#186121=CARTESIAN_POINT('Ctrl Pts',(23.6520669774876,-1.60148472786596,
0.));
#186122=CARTESIAN_POINT('Ctrl Pts',(23.6329168794929,-1.60625813414674,
0.));
#186123=CARTESIAN_POINT('Ctrl Pts',(23.6138626661653,-1.61095269379779,
0.));
#186124=CARTESIAN_POINT('Ctrl Pts',(23.5949053517997,-1.61556863424699,
0.));
#186125=CARTESIAN_POINT('Ctrl Pts',(23.57604596376,-1.62010618772867,0.));
#186126=CARTESIAN_POINT('Ctrl Pts',(23.5572855427601,-1.62456559140066,
0.));
#186127=CARTESIAN_POINT('Ctrl Pts',(23.538625143226,-1.62894708745224,0.));
#186128=CARTESIAN_POINT('Ctrl Pts',(23.5200658336612,-1.63325092321727,
0.));
#186129=CARTESIAN_POINT('Ctrl Pts',(23.5016086970003,-1.63747735129475,
0.));
#186130=CARTESIAN_POINT('Ctrl Pts',(23.4832548309645,-1.64162662967529,
0.));
#186131=CARTESIAN_POINT('Ctrl Pts',(23.4650053483932,-1.64569902187612,
0.));
#186132=CARTESIAN_POINT('Ctrl Pts',(23.4468613776574,-1.64969479707341,
0.));
#186133=CARTESIAN_POINT('Ctrl Pts',(23.4288240631043,-1.6536142302373,0.));
#186134=CARTESIAN_POINT('Ctrl Pts',(23.4108945654805,-1.65745760227506,
0.));
#186135=CARTESIAN_POINT('Ctrl Pts',(23.3930740623619,-1.66122520018012,
0.));
#186136=CARTESIAN_POINT('Ctrl Pts',(23.3753637485545,-1.66491731718878,
0.));
#186137=CARTESIAN_POINT('Ctrl Pts',(23.3577648365744,-1.66853425293997,
0.));
#186138=CARTESIAN_POINT('Ctrl Pts',(23.3402785571865,-1.67207631363923,
0.));
#186139=CARTESIAN_POINT('Ctrl Pts',(23.3229061599144,-1.67554381222995,
0.));
#186140=CARTESIAN_POINT('Ctrl Pts',(23.3056489135611,-1.67893706857118,
0.));
#186141=CARTESIAN_POINT('Ctrl Pts',(23.2885081066951,-1.68225640962169,
0.));
#186142=CARTESIAN_POINT('Ctrl Pts',(23.2714850482246,-1.68550216963259,
0.));
#186143=CARTESIAN_POINT('Ctrl Pts',(23.2545810680537,-1.68867469034897,
0.));
#186144=CARTESIAN_POINT('Ctrl Pts',(23.2377975177013,-1.69177432121712,
0.));
#186145=CARTESIAN_POINT('Ctrl Pts',(23.2211357709374,-1.69480141959954,
0.));
#186146=CARTESIAN_POINT('Ctrl Pts',(23.2045972243767,-1.69775635099444,
0.));
#186147=CARTESIAN_POINT('Ctrl Pts',(23.1881832981851,-1.70063948927011,
0.));
#186148=CARTESIAN_POINT('Ctrl Pts',(23.1718954368751,-1.70345121691278,
0.));
#186149=CARTESIAN_POINT('Ctrl Pts',(23.1557351100614,-1.70619192527853,
0.));
#186150=CARTESIAN_POINT('Ctrl Pts',(23.1397038132356,-1.70886201485453,
0.));
#186151=CARTESIAN_POINT('Ctrl Pts',(23.1238030684925,-1.71146189552175,
0.));
#186152=CARTESIAN_POINT('Ctrl Pts',(23.1080344254286,-1.71399198684705,
0.));
#186153=CARTESIAN_POINT('Ctrl Pts',(23.0923994621213,-1.71645271839298,
0.));
#186154=CARTESIAN_POINT('Ctrl Pts',(23.0768997860708,-1.71884453003028,
0.));
#186155=CARTESIAN_POINT('Ctrl Pts',(23.0615370351562,-1.72116787225993,
0.));
#186156=CARTESIAN_POINT('Ctrl Pts',(23.0463128785531,-1.72342320653748,
0.));
#186157=CARTESIAN_POINT('Ctrl Pts',(23.0312290178883,-1.72561100564047,
0.));
#186158=CARTESIAN_POINT('Ctrl Pts',(23.0162871884168,-1.7277317540471,0.));
#186159=CARTESIAN_POINT('Ctrl Pts',(23.001489160189,-1.72978594832137,0.));
#186160=CARTESIAN_POINT('Ctrl Pts',(22.9868367391978,-1.73177409750192,
0.));
#186161=CARTESIAN_POINT('Ctrl Pts',(22.9723317685688,-1.73369672350816,
0.));
#186162=CARTESIAN_POINT('Ctrl Pts',(22.9579761301063,-1.73555436162771,
0.));
#186163=CARTESIAN_POINT('Ctrl Pts',(22.9437717457826,-1.7373475610004,0.));
#186164=CARTESIAN_POINT('Ctrl Pts',(22.9297205792586,-1.73907688511667,
0.));
#186165=CARTESIAN_POINT('Ctrl Pts',(22.9158246373363,-1.7407429123106,0.));
#186166=CARTESIAN_POINT('Ctrl Pts',(22.9020859716141,-1.74234623630081,
0.));
#186167=CARTESIAN_POINT('Ctrl Pts',(22.888506680335,-1.74388746677704,0.));
#186168=CARTESIAN_POINT('Ctrl Pts',(22.8750889101696,-1.74536722998202,
0.));
#186169=CARTESIAN_POINT('Ctrl Pts',(22.8618348580235,-1.74678616930666,
0.));
#186170=CARTESIAN_POINT('Ctrl Pts',(22.8487467728076,-1.74814494588494,
0.));
#186171=CARTESIAN_POINT('Ctrl Pts',(22.8358269579853,-1.74944423940117,
0.));
#186172=CARTESIAN_POINT('Ctrl Pts',(22.8230777741284,-1.75068474890884,
0.));
#186173=CARTESIAN_POINT('Ctrl Pts',(22.8105016414713,-1.75186719365593,
0.));
#186174=CARTESIAN_POINT('Ctrl Pts',(22.7981010424314,-1.75299231391468,
0.));
#186175=CARTESIAN_POINT('Ctrl Pts',(22.7858785242361,-1.75406087182937,
0.));
#186176=CARTESIAN_POINT('Ctrl Pts',(22.7738367016118,-1.75507365227133,
0.));
#186177=CARTESIAN_POINT('Ctrl Pts',(22.7619782595013,-1.75603146371642,
0.));
#186178=CARTESIAN_POINT('Ctrl Pts',(22.750305955645,-1.75693513908908,0.));
#186179=CARTESIAN_POINT('Ctrl Pts',(22.7388226235559,-1.75778553673245,
0.));
#186180=CARTESIAN_POINT('Ctrl Pts',(22.72753117773,-1.75858354204634,0.));
#186181=CARTESIAN_POINT('Ctrl Pts',(22.7164346186006,-1.75933006905926,
0.));
#186182=CARTESIAN_POINT('Ctrl Pts',(22.7055360375485,-1.76002606202402,
0.));
#186183=CARTESIAN_POINT('Ctrl Pts',(22.6948386219851,-1.76067249704888,
0.));
#186184=CARTESIAN_POINT('Ctrl Pts',(22.684345658525,-1.76127038310615,0.));
#186185=CARTESIAN_POINT('Ctrl Pts',(22.67406053567,-1.76182076289527,0.));
#186186=CARTESIAN_POINT('Ctrl Pts',(22.6639867471753,-1.7623247139257,0.));
#186187=CARTESIAN_POINT('Ctrl Pts',(22.6541278938409,-1.76278334912562,
0.));
#186188=CARTESIAN_POINT('Ctrl Pts',(22.6444876940423,-1.76319782013917,
0.));
#186189=CARTESIAN_POINT('Ctrl Pts',(22.6350699979359,-1.76356932176274,
0.));
#186190=CARTESIAN_POINT('Ctrl Pts',(22.6258787994848,-1.76389909571404,
0.));
#186191=CARTESIAN_POINT('Ctrl Pts',(22.6169182517694,-1.76418843543741,
0.));
#186192=CARTESIAN_POINT('Ctrl Pts',(22.6081926681343,-1.76443868648017,
0.));
#186193=CARTESIAN_POINT('Ctrl Pts',(22.5997065145638,-1.76465124413558,
0.));
#186194=CARTESIAN_POINT('Ctrl Pts',(22.5914644078105,-1.76482755288412,
0.));
#186195=CARTESIAN_POINT('Ctrl Pts',(22.5834711038022,-1.76496910283089,
0.));
#186196=CARTESIAN_POINT('Ctrl Pts',(22.5757315316353,-1.76507744026747,
0.));
#186197=CARTESIAN_POINT('Ctrl Pts',(22.5682508499873,-1.76515418518832,
0.));
#186198=CARTESIAN_POINT('Ctrl Pts',(22.5610344912501,-1.76520104500451,
0.));
#186199=CARTESIAN_POINT('Ctrl Pts',(22.5540882235837,-1.76521983384064,
0.));
#186200=CARTESIAN_POINT('Ctrl Pts',(22.5474180954006,-1.76521245524048,
0.));
#186201=CARTESIAN_POINT('Ctrl Pts',(22.5410303590892,-1.76518087841494,
0.));
#186202=CARTESIAN_POINT('Ctrl Pts',(22.5349313983571,-1.76512711563255,
0.));
#186203=CARTESIAN_POINT('Ctrl Pts',(22.529127665298,-1.7650532026276,0.));
#186204=CARTESIAN_POINT('Ctrl Pts',(22.5236259635515,-1.76496128643376,
0.));
#186205=CARTESIAN_POINT('Ctrl Pts',(22.5184336670207,-1.76485369319896,
0.));
#186206=CARTESIAN_POINT('Ctrl Pts',(22.5135590569554,-1.7647330328115,0.));
#186207=CARTESIAN_POINT('Ctrl Pts',(22.5090112700212,-1.76460218257314,
0.));
#186208=CARTESIAN_POINT('Ctrl Pts',(22.5047996391978,-1.76446408210366,
0.));
#186209=CARTESIAN_POINT('Ctrl Pts',(22.5009332677316,-1.76432160068739,
0.));
#186210=CARTESIAN_POINT('Ctrl Pts',(22.4974203063191,-1.76417731243484,
0.));
#186211=CARTESIAN_POINT('Ctrl Pts',(22.4942693792449,-1.76403393880317,
0.));
#186212=CARTESIAN_POINT('Ctrl Pts',(22.4914909094908,-1.76389475965715,
0.));
#186213=CARTESIAN_POINT('Ctrl Pts',(22.4890991659479,-1.76376424879469,
0.));
#186214=CARTESIAN_POINT('Ctrl Pts',(22.4871115206572,-1.76364784232927,
0.));
#186215=CARTESIAN_POINT('Ctrl Pts',(22.4855446605991,-1.7635507604555,0.));
#186216=CARTESIAN_POINT('Ctrl Pts',(22.4844112933125,-1.76347698284863,
0.));
#186217=CARTESIAN_POINT('Ctrl Pts',(22.4838562517064,-1.7634381343466,0.));
#186218=CARTESIAN_POINT('Ctrl Pts',(22.4836387052228,-1.76342064263638,
0.));
#186219=CARTESIAN_POINT('Ctrl Pts',(22.4835819929788,-1.76341415538792,
0.));
#186220=CARTESIAN_POINT('Ctrl Pts',(22.4835757167854,-1.76341220531181,
0.));
#186221=CARTESIAN_POINT('',(25.991588367311,-0.661312440730916,0.));
#186222=CARTESIAN_POINT('Ctrl Pts',(22.1738711152697,-4.11585220600463,
0.));
#186223=CARTESIAN_POINT('Ctrl Pts',(22.1738711152697,-4.11585220600463,
12.));
#186224=CARTESIAN_POINT('Ctrl Pts',(22.173877682324,-4.11585194677443,0.));
#186225=CARTESIAN_POINT('Ctrl Pts',(22.173877682324,-4.11585194677443,12.));
#186226=CARTESIAN_POINT('Ctrl Pts',(22.1739341411687,-4.11586035878288,
0.));
#186227=CARTESIAN_POINT('Ctrl Pts',(22.1739341411687,-4.11586035878288,
12.));
#186228=CARTESIAN_POINT('Ctrl Pts',(22.1741488021234,-4.11589976826168,
0.));
#186229=CARTESIAN_POINT('Ctrl Pts',(22.1741488021234,-4.11589976826168,
12.));
#186230=CARTESIAN_POINT('Ctrl Pts',(22.1746949858775,-4.11600589882846,
0.));
#186231=CARTESIAN_POINT('Ctrl Pts',(22.1746949858775,-4.11600589882846,
12.));
#186232=CARTESIAN_POINT('Ctrl Pts',(22.1758088296598,-4.1162279721707,0.));
#186233=CARTESIAN_POINT('Ctrl Pts',(22.1758088296598,-4.1162279721707,12.));
#186234=CARTESIAN_POINT('Ctrl Pts',(22.177347426894,-4.11653973150519,0.));
#186235=CARTESIAN_POINT('Ctrl Pts',(22.177347426894,-4.11653973150519,12.));
#186236=CARTESIAN_POINT('Ctrl Pts',(22.179297473024,-4.11694173195005,0.));
#186237=CARTESIAN_POINT('Ctrl Pts',(22.179297473024,-4.11694173195005,12.));
#186238=CARTESIAN_POINT('Ctrl Pts',(22.1816414985788,-4.11743469691757,
0.));
#186239=CARTESIAN_POINT('Ctrl Pts',(22.1816414985788,-4.11743469691757,
12.));
#186240=CARTESIAN_POINT('Ctrl Pts',(22.1843613164855,-4.11801938107481,
0.));
#186241=CARTESIAN_POINT('Ctrl Pts',(22.1843613164855,-4.11801938107481,
12.));
#186242=CARTESIAN_POINT('Ctrl Pts',(22.1874419861496,-4.11869641271775,
0.));
#186243=CARTESIAN_POINT('Ctrl Pts',(22.1874419861496,-4.11869641271775,
12.));
#186244=CARTESIAN_POINT('Ctrl Pts',(22.1908725908525,-4.11946626228637,
0.));
#186245=CARTESIAN_POINT('Ctrl Pts',(22.1908725908525,-4.11946626228637,
12.));
#186246=CARTESIAN_POINT('Ctrl Pts',(22.1946440958098,-4.12032932637738,
0.));
#186247=CARTESIAN_POINT('Ctrl Pts',(22.1946440958098,-4.12032932637738,
12.));
#186248=CARTESIAN_POINT('Ctrl Pts',(22.1987479618246,-4.12128598183523,
0.));
#186249=CARTESIAN_POINT('Ctrl Pts',(22.1987479618246,-4.12128598183523,
12.));
#186250=CARTESIAN_POINT('Ctrl Pts',(22.2031746532106,-4.12233664408228,
0.));
#186251=CARTESIAN_POINT('Ctrl Pts',(22.2031746532106,-4.12233664408228,
12.));
#186252=CARTESIAN_POINT('Ctrl Pts',(22.2079143941719,-4.12348173702024,
0.));
#186253=CARTESIAN_POINT('Ctrl Pts',(22.2079143941719,-4.12348173702024,
12.));
#186254=CARTESIAN_POINT('Ctrl Pts',(22.2129576146671,-4.12472167516608,
0.));
#186255=CARTESIAN_POINT('Ctrl Pts',(22.2129576146671,-4.12472167516608,
12.));
#186256=CARTESIAN_POINT('Ctrl Pts',(22.2182956401341,-4.12605683613308,
0.));
#186257=CARTESIAN_POINT('Ctrl Pts',(22.2182956401341,-4.12605683613308,
12.));
#186258=CARTESIAN_POINT('Ctrl Pts',(22.2239207458781,-4.12748755830105,
0.));
#186259=CARTESIAN_POINT('Ctrl Pts',(22.2239207458781,-4.12748755830105,
12.));
#186260=CARTESIAN_POINT('Ctrl Pts',(22.2298258043947,-4.1290141546338,0.));
#186261=CARTESIAN_POINT('Ctrl Pts',(22.2298258043947,-4.1290141546338,12.));
#186262=CARTESIAN_POINT('Ctrl Pts',(22.2360040565533,-4.13063692157499,
0.));
#186263=CARTESIAN_POINT('Ctrl Pts',(22.2360040565533,-4.13063692157499,
12.));
#186264=CARTESIAN_POINT('Ctrl Pts',(22.2424488153523,-4.13235615060161,
0.));
#186265=CARTESIAN_POINT('Ctrl Pts',(22.2424488153523,-4.13235615060161,
12.));
#186266=CARTESIAN_POINT('Ctrl Pts',(22.249153531779,-4.13417212558811,0.));
#186267=CARTESIAN_POINT('Ctrl Pts',(22.249153531779,-4.13417212558811,12.));
#186268=CARTESIAN_POINT('Ctrl Pts',(22.2561118708421,-4.13608511977227,
0.));
#186269=CARTESIAN_POINT('Ctrl Pts',(22.2561118708421,-4.13608511977227,
12.));
#186270=CARTESIAN_POINT('Ctrl Pts',(22.2633177913972,-4.13809539255423,
0.));
#186271=CARTESIAN_POINT('Ctrl Pts',(22.2633177913972,-4.13809539255423,
12.));
#186272=CARTESIAN_POINT('Ctrl Pts',(22.2707656042457,-4.14020318715992,
0.));
#186273=CARTESIAN_POINT('Ctrl Pts',(22.2707656042457,-4.14020318715992,
12.));
#186274=CARTESIAN_POINT('Ctrl Pts',(22.2784499072027,-4.14240873321985,
0.));
#186275=CARTESIAN_POINT('Ctrl Pts',(22.2784499072027,-4.14240873321985,
12.));
#186276=CARTESIAN_POINT('Ctrl Pts',(22.2863655389166,-4.14471224859297,
0.));
#186277=CARTESIAN_POINT('Ctrl Pts',(22.2863655389166,-4.14471224859297,
12.));
#186278=CARTESIAN_POINT('Ctrl Pts',(22.2945075198467,-4.14711394168557,
0.));
#186279=CARTESIAN_POINT('Ctrl Pts',(22.2945075198467,-4.14711394168557,
12.));
#186280=CARTESIAN_POINT('Ctrl Pts',(22.3028710166933,-4.14961401285523,
0.));
#186281=CARTESIAN_POINT('Ctrl Pts',(22.3028710166933,-4.14961401285523,
12.));
#186282=CARTESIAN_POINT('Ctrl Pts',(22.3114513545185,-4.15221265396991,
0.));
#186283=CARTESIAN_POINT('Ctrl Pts',(22.3114513545185,-4.15221265396991,
12.));
#186284=CARTESIAN_POINT('Ctrl Pts',(22.3202440186979,-4.15491004835282,
0.));
#186285=CARTESIAN_POINT('Ctrl Pts',(22.3202440186979,-4.15491004835282,
12.));
#186286=CARTESIAN_POINT('Ctrl Pts',(22.3292446628959,-4.15770637047891,
0.));
#186287=CARTESIAN_POINT('Ctrl Pts',(22.3292446628959,-4.15770637047891,
12.));
#186288=CARTESIAN_POINT('Ctrl Pts',(22.3384491078602,-4.16060178604165,
0.));
#186289=CARTESIAN_POINT('Ctrl Pts',(22.3384491078602,-4.16060178604165,
12.));
#186290=CARTESIAN_POINT('Ctrl Pts',(22.3478533253889,-4.16359645263189,
0.));
#186291=CARTESIAN_POINT('Ctrl Pts',(22.3478533253889,-4.16359645263189,
12.));
#186292=CARTESIAN_POINT('Ctrl Pts',(22.3574534257396,-4.16669052026601,
0.));
#186293=CARTESIAN_POINT('Ctrl Pts',(22.3574534257396,-4.16669052026601,
12.));
#186294=CARTESIAN_POINT('Ctrl Pts',(22.3672456427599,-4.16988413199458,
0.));
#186295=CARTESIAN_POINT('Ctrl Pts',(22.3672456427599,-4.16988413199458,
12.));
#186296=CARTESIAN_POINT('Ctrl Pts',(22.3772263228617,-4.17317742436146,
0.));
#186297=CARTESIAN_POINT('Ctrl Pts',(22.3772263228617,-4.17317742436146,
12.));
#186298=CARTESIAN_POINT('Ctrl Pts',(22.3873919231334,-4.17657052752826,
0.));
#186299=CARTESIAN_POINT('Ctrl Pts',(22.3873919231334,-4.17657052752826,
12.));
#186300=CARTESIAN_POINT('Ctrl Pts',(22.3977390078075,-4.18006356544883,
0.));
#186301=CARTESIAN_POINT('Ctrl Pts',(22.3977390078075,-4.18006356544883,
12.));
#186302=CARTESIAN_POINT('Ctrl Pts',(22.4082642454453,-4.18365665600852,
0.));
#186303=CARTESIAN_POINT('Ctrl Pts',(22.4082642454453,-4.18365665600852,
12.));
#186304=CARTESIAN_POINT('Ctrl Pts',(22.4189644056115,-4.18734991117722,
0.));
#186305=CARTESIAN_POINT('Ctrl Pts',(22.4189644056115,-4.18734991117722,
12.));
#186306=CARTESIAN_POINT('Ctrl Pts',(22.4298363535421,-4.19114343726943,
0.));
#186307=CARTESIAN_POINT('Ctrl Pts',(22.4298363535421,-4.19114343726943,
12.));
#186308=CARTESIAN_POINT('Ctrl Pts',(22.4408770448917,-4.19503733518862,
0.));
#186309=CARTESIAN_POINT('Ctrl Pts',(22.4408770448917,-4.19503733518862,
12.));
#186310=CARTESIAN_POINT('Ctrl Pts',(22.4520835205419,-4.19903170066356,
0.));
#186311=CARTESIAN_POINT('Ctrl Pts',(22.4520835205419,-4.19903170066356,
12.));
#186312=CARTESIAN_POINT('Ctrl Pts',(22.4634529011433,-4.20312662448172,
0.));
#186313=CARTESIAN_POINT('Ctrl Pts',(22.4634529011433,-4.20312662448172,
12.));
#186314=CARTESIAN_POINT('Ctrl Pts',(22.4749823839915,-4.20732219265649,
0.));
#186315=CARTESIAN_POINT('Ctrl Pts',(22.4749823839915,-4.20732219265649,
12.));
#186316=CARTESIAN_POINT('Ctrl Pts',(22.4866692403147,-4.21161848657429,
0.));
#186317=CARTESIAN_POINT('Ctrl Pts',(22.4866692403147,-4.21161848657429,
12.));
#186318=CARTESIAN_POINT('Ctrl Pts',(22.4985108124229,-4.21601558313909,
0.));
#186319=CARTESIAN_POINT('Ctrl Pts',(22.4985108124229,-4.21601558313909,
12.));
#186320=CARTESIAN_POINT('Ctrl Pts',(22.5105045108882,-4.22051355490198,
0.));
#186321=CARTESIAN_POINT('Ctrl Pts',(22.5105045108882,-4.22051355490198,
12.));
#186322=CARTESIAN_POINT('Ctrl Pts',(22.5226478117885,-4.22511247020041,
0.));
#186323=CARTESIAN_POINT('Ctrl Pts',(22.5226478117885,-4.22511247020041,
12.));
#186324=CARTESIAN_POINT('Ctrl Pts',(22.5349382540587,-4.22981239330733,
0.));
#186325=CARTESIAN_POINT('Ctrl Pts',(22.5349382540587,-4.22981239330733,
12.));
#186326=CARTESIAN_POINT('Ctrl Pts',(22.5473734368086,-4.23461338456714,
0.));
#186327=CARTESIAN_POINT('Ctrl Pts',(22.5473734368086,-4.23461338456714,
12.));
#186328=CARTESIAN_POINT('Ctrl Pts',(22.559951016643,-4.23951550052527,0.));
#186329=CARTESIAN_POINT('Ctrl Pts',(22.559951016643,-4.23951550052527,12.));
#186330=CARTESIAN_POINT('Ctrl Pts',(22.5726687049922,-4.2445187940486,0.));
#186331=CARTESIAN_POINT('Ctrl Pts',(22.5726687049922,-4.2445187940486,12.));
#186332=CARTESIAN_POINT('Ctrl Pts',(22.5855242662479,-4.24962331444186,
0.));
#186333=CARTESIAN_POINT('Ctrl Pts',(22.5855242662479,-4.24962331444186,
12.));
#186334=CARTESIAN_POINT('Ctrl Pts',(22.5985155158637,-4.25482910755486,
0.));
#186335=CARTESIAN_POINT('Ctrl Pts',(22.5985155158637,-4.25482910755486,
12.));
#186336=CARTESIAN_POINT('Ctrl Pts',(22.611640318482,-4.26013621588304,0.));
#186337=CARTESIAN_POINT('Ctrl Pts',(22.611640318482,-4.26013621588304,12.));
#186338=CARTESIAN_POINT('Ctrl Pts',(22.6248965859975,-4.26554467865572,
0.));
#186339=CARTESIAN_POINT('Ctrl Pts',(22.6248965859975,-4.26554467865572,
12.));
#186340=CARTESIAN_POINT('Ctrl Pts',(22.6382822758171,-4.27105453193,0.));
#186341=CARTESIAN_POINT('Ctrl Pts',(22.6382822758171,-4.27105453193,12.));
#186342=CARTESIAN_POINT('Ctrl Pts',(22.6517953893303,-4.27666580869118,
0.));
#186343=CARTESIAN_POINT('Ctrl Pts',(22.6517953893303,-4.27666580869118,
12.));
#186344=CARTESIAN_POINT('Ctrl Pts',(22.665433970311,-4.2823785389406,0.));
#186345=CARTESIAN_POINT('Ctrl Pts',(22.665433970311,-4.2823785389406,12.));
#186346=CARTESIAN_POINT('Ctrl Pts',(22.6791961033536,-4.28819274977767,
0.));
#186347=CARTESIAN_POINT('Ctrl Pts',(22.6791961033536,-4.28819274977767,
12.));
#186348=CARTESIAN_POINT('Ctrl Pts',(22.6930799122545,-4.29410846547062,
0.));
#186349=CARTESIAN_POINT('Ctrl Pts',(22.6930799122545,-4.29410846547062,
12.));
#186350=CARTESIAN_POINT('Ctrl Pts',(22.707083558756,-4.30012570754067,0.));
#186351=CARTESIAN_POINT('Ctrl Pts',(22.707083558756,-4.30012570754067,12.));
#186352=CARTESIAN_POINT('Ctrl Pts',(22.7212052413384,-4.30624449484075,
0.));
#186353=CARTESIAN_POINT('Ctrl Pts',(22.7212052413384,-4.30624449484075,
12.));
#186354=CARTESIAN_POINT('Ctrl Pts',(22.7354431939926,-4.31246484362551,
0.));
#186355=CARTESIAN_POINT('Ctrl Pts',(22.7354431939926,-4.31246484362551,
12.));
#186356=CARTESIAN_POINT('Ctrl Pts',(22.7497956849852,-4.31878676761231,
0.));
#186357=CARTESIAN_POINT('Ctrl Pts',(22.7497956849852,-4.31878676761231,
12.));
#186358=CARTESIAN_POINT('Ctrl Pts',(22.764261015648,-4.32521027803748,0.));
#186359=CARTESIAN_POINT('Ctrl Pts',(22.764261015648,-4.32521027803748,12.));
#186360=CARTESIAN_POINT('Ctrl Pts',(22.7788375194081,-4.33173538373183,
0.));
#186361=CARTESIAN_POINT('Ctrl Pts',(22.7788375194081,-4.33173538373183,
12.));
#186362=CARTESIAN_POINT('Ctrl Pts',(22.7935235607807,-4.33836209118444,
0.));
#186363=CARTESIAN_POINT('Ctrl Pts',(22.7935235607807,-4.33836209118444,
12.));
#186364=CARTESIAN_POINT('Ctrl Pts',(22.808317534379,-4.34509040460066,0.));
#186365=CARTESIAN_POINT('Ctrl Pts',(22.808317534379,-4.34509040460066,12.));
#186366=CARTESIAN_POINT('Ctrl Pts',(22.8232178638873,-4.35192032594802,
0.));
#186367=CARTESIAN_POINT('Ctrl Pts',(22.8232178638873,-4.35192032594802,
12.));
#186368=CARTESIAN_POINT('Ctrl Pts',(22.838223001118,-4.3588518550056,0.));
#186369=CARTESIAN_POINT('Ctrl Pts',(22.838223001118,-4.3588518550056,12.));
#186370=CARTESIAN_POINT('Ctrl Pts',(22.8533314252419,-4.36588498943011,
0.));
#186371=CARTESIAN_POINT('Ctrl Pts',(22.8533314252419,-4.36588498943011,
12.));
#186372=CARTESIAN_POINT('Ctrl Pts',(22.8685416419725,-4.37301972480753,
0.));
#186373=CARTESIAN_POINT('Ctrl Pts',(22.8685416419725,-4.37301972480753,
12.));
#186374=CARTESIAN_POINT('Ctrl Pts',(22.8838521827702,-4.38025605470091,
0.));
#186375=CARTESIAN_POINT('Ctrl Pts',(22.8838521827702,-4.38025605470091,
12.));
#186376=CARTESIAN_POINT('Ctrl Pts',(22.8992616040108,-4.38759397068393,
0.));
#186377=CARTESIAN_POINT('Ctrl Pts',(22.8992616040108,-4.38759397068393,
12.));
#186378=CARTESIAN_POINT('Ctrl Pts',(22.9147684862425,-4.39503346238455,
0.));
#186379=CARTESIAN_POINT('Ctrl Pts',(22.9147684862425,-4.39503346238455,
12.));
#186380=CARTESIAN_POINT('Ctrl Pts',(22.9303714335549,-4.40257451754309,
0.));
#186381=CARTESIAN_POINT('Ctrl Pts',(22.9303714335549,-4.40257451754309,
12.));
#186382=CARTESIAN_POINT('Ctrl Pts',(22.9460690729092,-4.41021712205549,
0.));
#186383=CARTESIAN_POINT('Ctrl Pts',(22.9460690729092,-4.41021712205549,
12.));
#186384=CARTESIAN_POINT('Ctrl Pts',(22.9618600534866,-4.41796126001311,
0.));
#186385=CARTESIAN_POINT('Ctrl Pts',(22.9618600534866,-4.41796126001311,
12.));
#186386=CARTESIAN_POINT('Ctrl Pts',(22.9777430460021,-4.42580691372772,
0.));
#186387=CARTESIAN_POINT('Ctrl Pts',(22.9777430460021,-4.42580691372772,
12.));
#186388=CARTESIAN_POINT('Ctrl Pts',(22.9937167421009,-4.43375406376906,
0.));
#186389=CARTESIAN_POINT('Ctrl Pts',(22.9937167421009,-4.43375406376906,
12.));
#186390=CARTESIAN_POINT('Ctrl Pts',(23.0097798538399,-4.44180268901667,
0.));
#186391=CARTESIAN_POINT('Ctrl Pts',(23.0097798538399,-4.44180268901667,
12.));
#186392=CARTESIAN_POINT('Ctrl Pts',(23.0259311131395,-4.44995276669699,
0.));
#186393=CARTESIAN_POINT('Ctrl Pts',(23.0259311131395,-4.44995276669699,
12.));
#186394=CARTESIAN_POINT('Ctrl Pts',(23.0421692712466,-4.45820427241678,
0.));
#186395=CARTESIAN_POINT('Ctrl Pts',(23.0421692712466,-4.45820427241678,
12.));
#186396=CARTESIAN_POINT('Ctrl Pts',(23.0584930981723,-4.46655718018206,
0.));
#186397=CARTESIAN_POINT('Ctrl Pts',(23.0584930981723,-4.46655718018206,
12.));
#186398=CARTESIAN_POINT('Ctrl Pts',(23.0749013821867,-4.47501146242822,
0.));
#186399=CARTESIAN_POINT('Ctrl Pts',(23.0749013821867,-4.47501146242822,
12.));
#186400=CARTESIAN_POINT('Ctrl Pts',(23.0913929293909,-4.48356709006757,
0.));
#186401=CARTESIAN_POINT('Ctrl Pts',(23.0913929293909,-4.48356709006757,
12.));
#186402=CARTESIAN_POINT('Ctrl Pts',(23.1079665632629,-4.49222403252202,
0.));
#186403=CARTESIAN_POINT('Ctrl Pts',(23.1079665632629,-4.49222403252202,
12.));
#186404=CARTESIAN_POINT('Ctrl Pts',(23.1246211242117,-4.5009822577518,0.));
#186405=CARTESIAN_POINT('Ctrl Pts',(23.1246211242117,-4.5009822577518,12.));
#186406=CARTESIAN_POINT('Ctrl Pts',(23.1413554691136,-4.50984173227088,
0.));
#186407=CARTESIAN_POINT('Ctrl Pts',(23.1413554691136,-4.50984173227088,
12.));
#186408=CARTESIAN_POINT('Ctrl Pts',(23.1581684708778,-4.51880242116786,
0.));
#186409=CARTESIAN_POINT('Ctrl Pts',(23.1581684708778,-4.51880242116786,
12.));
#186410=CARTESIAN_POINT('Ctrl Pts',(23.1750590180923,-4.52786428815049,
0.));
#186411=CARTESIAN_POINT('Ctrl Pts',(23.1750590180923,-4.52786428815049,
12.));
#186412=CARTESIAN_POINT('Ctrl Pts',(23.1920260146474,-4.53702729557586,
0.));
#186413=CARTESIAN_POINT('Ctrl Pts',(23.1920260146474,-4.53702729557586,
12.));
#186414=CARTESIAN_POINT('Ctrl Pts',(23.2090683793627,-4.54629140447543,
0.));
#186415=CARTESIAN_POINT('Ctrl Pts',(23.2090683793627,-4.54629140447543,
12.));
#186416=CARTESIAN_POINT('Ctrl Pts',(23.2261850456054,-4.55565657456957,
0.));
#186417=CARTESIAN_POINT('Ctrl Pts',(23.2261850456054,-4.55565657456957,
12.));
#186418=CARTESIAN_POINT('Ctrl Pts',(23.2433749609117,-4.56512276427812,
0.));
#186419=CARTESIAN_POINT('Ctrl Pts',(23.2433749609117,-4.56512276427812,
12.));
#186420=CARTESIAN_POINT('Ctrl Pts',(23.2606370866853,-4.57468993076071,
0.));
#186421=CARTESIAN_POINT('Ctrl Pts',(23.2606370866853,-4.57468993076071,
12.));
#186422=CARTESIAN_POINT('Ctrl Pts',(23.2779703978868,-4.58435802994675,
0.));
#186423=CARTESIAN_POINT('Ctrl Pts',(23.2779703978868,-4.58435802994675,
12.));
#186424=CARTESIAN_POINT('Ctrl Pts',(23.295373882719,-4.59412701655751,0.));
#186425=CARTESIAN_POINT('Ctrl Pts',(23.295373882719,-4.59412701655751,12.));
#186426=CARTESIAN_POINT('Ctrl Pts',(23.3128465423119,-4.60399684412176,
0.));
#186427=CARTESIAN_POINT('Ctrl Pts',(23.3128465423119,-4.60399684412176,
12.));
#186428=CARTESIAN_POINT('Ctrl Pts',(23.3303873903947,-4.6139674649785,0.));
#186429=CARTESIAN_POINT('Ctrl Pts',(23.3303873903947,-4.6139674649785,12.));
#186430=CARTESIAN_POINT('Ctrl Pts',(23.3479954530281,-4.62403883030825,
0.));
#186431=CARTESIAN_POINT('Ctrl Pts',(23.3479954530281,-4.62403883030825,
12.));
#186432=CARTESIAN_POINT('Ctrl Pts',(23.3656697683496,-4.63421089016556,
0.));
#186433=CARTESIAN_POINT('Ctrl Pts',(23.3656697683496,-4.63421089016556,
12.));
#186434=CARTESIAN_POINT('Ctrl Pts',(23.383409386307,-4.64448359349936,0.));
#186435=CARTESIAN_POINT('Ctrl Pts',(23.383409386307,-4.64448359349936,12.));
#186436=CARTESIAN_POINT('Ctrl Pts',(23.4012133683957,-4.65485688816923,
0.));
#186437=CARTESIAN_POINT('Ctrl Pts',(23.4012133683957,-4.65485688816923,
12.));
#186438=CARTESIAN_POINT('Ctrl Pts',(23.4190807873798,-4.66533072094664,
0.));
#186439=CARTESIAN_POINT('Ctrl Pts',(23.4190807873798,-4.66533072094664,
12.));
#186440=CARTESIAN_POINT('Ctrl Pts',(23.4370107270444,-4.67590503753051,
0.));
#186441=CARTESIAN_POINT('Ctrl Pts',(23.4370107270444,-4.67590503753051,
12.));
#186442=CARTESIAN_POINT('Ctrl Pts',(23.4550022819852,-4.68657978258298,
0.));
#186443=CARTESIAN_POINT('Ctrl Pts',(23.4550022819852,-4.68657978258298,
12.));
#186444=CARTESIAN_POINT('Ctrl Pts',(23.4730545573849,-4.69735489975024,
0.));
#186445=CARTESIAN_POINT('Ctrl Pts',(23.4730545573849,-4.69735489975024,
12.));
#186446=CARTESIAN_POINT('Ctrl Pts',(23.491166668789,-4.70823033167821,0.));
#186447=CARTESIAN_POINT('Ctrl Pts',(23.491166668789,-4.70823033167821,12.));
#186448=CARTESIAN_POINT('Ctrl Pts',(23.5093377418784,-4.71920602001905,
0.));
#186449=CARTESIAN_POINT('Ctrl Pts',(23.5093377418784,-4.71920602001905,
12.));
#186450=CARTESIAN_POINT('Ctrl Pts',(23.5275669122378,-4.73028190543032,
0.));
#186451=CARTESIAN_POINT('Ctrl Pts',(23.5275669122378,-4.73028190543032,
12.));
#186452=CARTESIAN_POINT('Ctrl Pts',(23.5458533251715,-4.74145792760699,
0.));
#186453=CARTESIAN_POINT('Ctrl Pts',(23.5458533251715,-4.74145792760699,
12.));
#186454=CARTESIAN_POINT('Ctrl Pts',(23.564196135517,-4.75273402530616,0.));
#186455=CARTESIAN_POINT('Ctrl Pts',(23.564196135517,-4.75273402530616,12.));
#186456=CARTESIAN_POINT('Ctrl Pts',(23.5825945074535,-4.76411013636252,
0.));
#186457=CARTESIAN_POINT('Ctrl Pts',(23.5825945074535,-4.76411013636252,
12.));
#186458=CARTESIAN_POINT('Ctrl Pts',(23.6010476143099,-4.77558619769876,
0.));
#186459=CARTESIAN_POINT('Ctrl Pts',(23.6010476143099,-4.77558619769876,
12.));
#186460=CARTESIAN_POINT('Ctrl Pts',(23.6195546383625,-4.78716214532105,
0.));
#186461=CARTESIAN_POINT('Ctrl Pts',(23.6195546383625,-4.78716214532105,
12.));
#186462=CARTESIAN_POINT('Ctrl Pts',(23.6381147706581,-4.79883791433231,
0.));
#186463=CARTESIAN_POINT('Ctrl Pts',(23.6381147706581,-4.79883791433231,
12.));
#186464=CARTESIAN_POINT('Ctrl Pts',(23.6567272108631,-4.81061343896443,
0.));
#186465=CARTESIAN_POINT('Ctrl Pts',(23.6567272108631,-4.81061343896443,
12.));
#186466=CARTESIAN_POINT('Ctrl Pts',(23.6753911671023,-4.82248865259571,
0.));
#186467=CARTESIAN_POINT('Ctrl Pts',(23.6753911671023,-4.82248865259571,
12.));
#186468=CARTESIAN_POINT('Ctrl Pts',(23.6941058557971,-4.83446348776268,
0.));
#186469=CARTESIAN_POINT('Ctrl Pts',(23.6941058557971,-4.83446348776268,
12.));
#186470=CARTESIAN_POINT('Ctrl Pts',(23.7128705015014,-4.84653787616424,
0.));
#186471=CARTESIAN_POINT('Ctrl Pts',(23.7128705015014,-4.84653787616424,
12.));
#186472=CARTESIAN_POINT('Ctrl Pts',(23.7316843367308,-4.85871174865493,
0.));
#186473=CARTESIAN_POINT('Ctrl Pts',(23.7316843367308,-4.85871174865493,
12.));
#186474=CARTESIAN_POINT('Ctrl Pts',(23.7505466018239,-4.87098503527144,
0.));
#186475=CARTESIAN_POINT('Ctrl Pts',(23.7505466018239,-4.87098503527144,
12.));
#186476=CARTESIAN_POINT('Ctrl Pts',(23.7694565448044,-4.88335766525566,
0.));
#186477=CARTESIAN_POINT('Ctrl Pts',(23.7694565448044,-4.88335766525566,
12.));
#186478=CARTESIAN_POINT('Ctrl Pts',(23.7884134212381,-4.89582956706772,
0.));
#186479=CARTESIAN_POINT('Ctrl Pts',(23.7884134212381,-4.89582956706772,
12.));
#186480=CARTESIAN_POINT('Ctrl Pts',(23.8074164940897,-4.90840066839348,
0.));
#186481=CARTESIAN_POINT('Ctrl Pts',(23.8074164940897,-4.90840066839348,
12.));
#186482=CARTESIAN_POINT('Ctrl Pts',(23.8264650335721,-4.92107089613978,
0.));
#186483=CARTESIAN_POINT('Ctrl Pts',(23.8264650335721,-4.92107089613978,
12.));
#186484=CARTESIAN_POINT('Ctrl Pts',(23.8455583170062,-4.93384017643443,
0.));
#186485=CARTESIAN_POINT('Ctrl Pts',(23.8455583170062,-4.93384017643443,
12.));
#186486=CARTESIAN_POINT('Ctrl Pts',(23.8646956287172,-4.94670843465869,
0.));
#186487=CARTESIAN_POINT('Ctrl Pts',(23.8646956287172,-4.94670843465869,
12.));
#186488=CARTESIAN_POINT('Ctrl Pts',(23.883876259922,-4.95967559546566,0.));
#186489=CARTESIAN_POINT('Ctrl Pts',(23.883876259922,-4.95967559546566,12.));
#186490=CARTESIAN_POINT('Ctrl Pts',(23.9030995086164,-4.9727415827923,0.));
#186491=CARTESIAN_POINT('Ctrl Pts',(23.9030995086164,-4.9727415827923,12.));
#186492=CARTESIAN_POINT('Ctrl Pts',(23.9223646794591,-4.98590631986534,
0.));
#186493=CARTESIAN_POINT('Ctrl Pts',(23.9223646794591,-4.98590631986534,
12.));
#186494=CARTESIAN_POINT('Ctrl Pts',(23.9416710836528,-4.9991697291931,0.));
#186495=CARTESIAN_POINT('Ctrl Pts',(23.9416710836528,-4.9991697291931,12.));
#186496=CARTESIAN_POINT('Ctrl Pts',(23.9610180388271,-5.01253173257459,
0.));
#186497=CARTESIAN_POINT('Ctrl Pts',(23.9610180388271,-5.01253173257459,
12.));
#186498=CARTESIAN_POINT('Ctrl Pts',(23.9804048689228,-5.02599225112462,
0.));
#186499=CARTESIAN_POINT('Ctrl Pts',(23.9804048689228,-5.02599225112462,
12.));
#186500=CARTESIAN_POINT('Ctrl Pts',(23.9998309040747,-5.03955120528528,
0.));
#186501=CARTESIAN_POINT('Ctrl Pts',(23.9998309040747,-5.03955120528528,
12.));
#186502=CARTESIAN_POINT('Ctrl Pts',(24.0192954804896,-5.05320851483069,
0.));
#186503=CARTESIAN_POINT('Ctrl Pts',(24.0192954804896,-5.05320851483069,
12.));
#186504=CARTESIAN_POINT('Ctrl Pts',(24.0387979403268,-5.0669640988664,0.));
#186505=CARTESIAN_POINT('Ctrl Pts',(24.0387979403268,-5.0669640988664,12.));
#186506=CARTESIAN_POINT('Ctrl Pts',(24.0583376315636,-5.08081787581271,
0.));
#186507=CARTESIAN_POINT('Ctrl Pts',(24.0583376315636,-5.08081787581271,
12.));
#186508=CARTESIAN_POINT('Ctrl Pts',(24.0779139079264,-5.09476976342618,
0.));
#186509=CARTESIAN_POINT('Ctrl Pts',(24.0779139079264,-5.09476976342618,
12.));
#186510=CARTESIAN_POINT('Ctrl Pts',(24.0975261288444,-5.10881967883126,
0.));
#186511=CARTESIAN_POINT('Ctrl Pts',(24.0975261288444,-5.10881967883126,
12.));
#186512=CARTESIAN_POINT('Ctrl Pts',(24.117173659394,-5.12296753853858,0.));
#186513=CARTESIAN_POINT('Ctrl Pts',(24.117173659394,-5.12296753853858,12.));
#186514=CARTESIAN_POINT('Ctrl Pts',(24.1368558702443,-5.13721325845746,
0.));
#186515=CARTESIAN_POINT('Ctrl Pts',(24.1368558702443,-5.13721325845746,
12.));
#186516=CARTESIAN_POINT('Ctrl Pts',(24.1565721375971,-5.1515567539008,0.));
#186517=CARTESIAN_POINT('Ctrl Pts',(24.1565721375971,-5.1515567539008,12.));
#186518=CARTESIAN_POINT('Ctrl Pts',(24.1763218431344,-5.16599793957987,
0.));
#186519=CARTESIAN_POINT('Ctrl Pts',(24.1763218431344,-5.16599793957987,
12.));
#186520=CARTESIAN_POINT('Ctrl Pts',(24.1961043738755,-5.180536729614,0.));
#186521=CARTESIAN_POINT('Ctrl Pts',(24.1961043738755,-5.180536729614,12.));
#186522=CARTESIAN_POINT('Ctrl Pts',(24.2159191220171,-5.19517303753648,
0.));
#186523=CARTESIAN_POINT('Ctrl Pts',(24.2159191220171,-5.19517303753648,
12.));
#186524=CARTESIAN_POINT('Ctrl Pts',(24.2357654847766,-5.20990677629177,
0.));
#186525=CARTESIAN_POINT('Ctrl Pts',(24.2357654847766,-5.20990677629177,
12.));
#186526=CARTESIAN_POINT('Ctrl Pts',(24.2556428642294,-5.22473785822443,
0.));
#186527=CARTESIAN_POINT('Ctrl Pts',(24.2556428642294,-5.22473785822443,
12.));
#186528=CARTESIAN_POINT('Ctrl Pts',(24.2755506671525,-5.2396661950629,0.));
#186529=CARTESIAN_POINT('Ctrl Pts',(24.2755506671525,-5.2396661950629,12.));
#186530=CARTESIAN_POINT('Ctrl Pts',(24.2954883048447,-5.25469169788858,
0.));
#186531=CARTESIAN_POINT('Ctrl Pts',(24.2954883048447,-5.25469169788858,
12.));
#186532=CARTESIAN_POINT('Ctrl Pts',(24.3154551932221,-5.269814277188,0.));
#186533=CARTESIAN_POINT('Ctrl Pts',(24.3154551932221,-5.269814277188,12.));
#186534=CARTESIAN_POINT('Ctrl Pts',(24.3354507529414,-5.28503384290649,
0.));
#186535=CARTESIAN_POINT('Ctrl Pts',(24.3354507529414,-5.28503384290649,
12.));
#186536=CARTESIAN_POINT('Ctrl Pts',(24.3554744095075,-5.30035030449065,
0.));
#186537=CARTESIAN_POINT('Ctrl Pts',(24.3554744095075,-5.30035030449065,
12.));
#186538=CARTESIAN_POINT('Ctrl Pts',(24.3755255933917,-5.31576357092527,
0.));
#186539=CARTESIAN_POINT('Ctrl Pts',(24.3755255933917,-5.31576357092527,
12.));
#186540=CARTESIAN_POINT('Ctrl Pts',(24.3956037401293,-5.33127355076035,
0.));
#186541=CARTESIAN_POINT('Ctrl Pts',(24.3956037401293,-5.33127355076035,
12.));
#186542=CARTESIAN_POINT('Ctrl Pts',(24.4157082904614,-5.34688015213538,
0.));
#186543=CARTESIAN_POINT('Ctrl Pts',(24.4157082904614,-5.34688015213538,
12.));
#186544=CARTESIAN_POINT('Ctrl Pts',(24.435838689915,-5.36258328273628,0.));
#186545=CARTESIAN_POINT('Ctrl Pts',(24.435838689915,-5.36258328273628,12.));
#186546=CARTESIAN_POINT('Ctrl Pts',(24.4559943883157,-5.37838284973696,
0.));
#186547=CARTESIAN_POINT('Ctrl Pts',(24.4559943883157,-5.37838284973696,
12.));
#186548=CARTESIAN_POINT('Ctrl Pts',(24.4761748393321,-5.39427875973825,
0.));
#186549=CARTESIAN_POINT('Ctrl Pts',(24.4761748393321,-5.39427875973825,
12.));
#186550=CARTESIAN_POINT('Ctrl Pts',(24.496379499983,-5.41027091869242,0.));
#186551=CARTESIAN_POINT('Ctrl Pts',(24.496379499983,-5.41027091869242,12.));
#186552=CARTESIAN_POINT('Ctrl Pts',(24.5166078302108,-5.4263592318342,0.));
#186553=CARTESIAN_POINT('Ctrl Pts',(24.5166078302108,-5.4263592318342,12.));
#186554=CARTESIAN_POINT('Ctrl Pts',(24.5368592922863,-5.44254360356881,
0.));
#186555=CARTESIAN_POINT('Ctrl Pts',(24.5368592922863,-5.44254360356881,
12.));
#186556=CARTESIAN_POINT('Ctrl Pts',(24.5571333514842,-5.45882393762263,
0.));
#186557=CARTESIAN_POINT('Ctrl Pts',(24.5571333514842,-5.45882393762263,
12.));
#186558=CARTESIAN_POINT('Ctrl Pts',(24.5774294770329,-5.4752001372442,0.));
#186559=CARTESIAN_POINT('Ctrl Pts',(24.5774294770329,-5.4752001372442,12.));
#186560=CARTESIAN_POINT('Ctrl Pts',(24.5977471429364,-5.49167210537248,
0.));
#186561=CARTESIAN_POINT('Ctrl Pts',(24.5977471429364,-5.49167210537248,
12.));
#186562=CARTESIAN_POINT('Ctrl Pts',(24.6180858289179,-5.50823974481963,
0.));
#186563=CARTESIAN_POINT('Ctrl Pts',(24.6180858289179,-5.50823974481963,
12.));
#186564=CARTESIAN_POINT('Ctrl Pts',(24.6384450211467,-5.52490295840993,
0.));
#186565=CARTESIAN_POINT('Ctrl Pts',(24.6384450211467,-5.52490295840993,
12.));
#186566=CARTESIAN_POINT('Ctrl Pts',(24.6588242134738,-5.54166164919584,
0.));
#186567=CARTESIAN_POINT('Ctrl Pts',(24.6588242134738,-5.54166164919584,
12.));
#186568=CARTESIAN_POINT('Ctrl Pts',(24.6792229061794,-5.55851572025377,
0.));
#186569=CARTESIAN_POINT('Ctrl Pts',(24.6792229061794,-5.55851572025377,
12.));
#186570=CARTESIAN_POINT('Ctrl Pts',(24.6996406035517,-5.57546507427756,
0.));
#186571=CARTESIAN_POINT('Ctrl Pts',(24.6996406035517,-5.57546507427756,
12.));
#186572=CARTESIAN_POINT('Ctrl Pts',(24.7200768119088,-5.59250961323988,
0.));
#186573=CARTESIAN_POINT('Ctrl Pts',(24.7200768119088,-5.59250961323988,
12.));
#186574=CARTESIAN_POINT('Ctrl Pts',(24.7405310372739,-5.60964923798492,
0.));
#186575=CARTESIAN_POINT('Ctrl Pts',(24.7405310372739,-5.60964923798492,
12.));
#186576=CARTESIAN_POINT('Ctrl Pts',(24.7610027835697,-5.62688384790924,
0.));
#186577=CARTESIAN_POINT('Ctrl Pts',(24.7610027835697,-5.62688384790924,
12.));
#186578=CARTESIAN_POINT('Ctrl Pts',(24.781491549672,-5.64421334042262,0.));
#186579=CARTESIAN_POINT('Ctrl Pts',(24.781491549672,-5.64421334042262,12.));
#186580=CARTESIAN_POINT('Ctrl Pts',(24.8019968304605,-5.66163761114922,
0.));
#186581=CARTESIAN_POINT('Ctrl Pts',(24.8019968304605,-5.66163761114922,
12.));
#186582=CARTESIAN_POINT('Ctrl Pts',(24.8225181223845,-5.67915655496543,
0.));
#186583=CARTESIAN_POINT('Ctrl Pts',(24.8225181223845,-5.67915655496543,
12.));
#186584=CARTESIAN_POINT('Ctrl Pts',(24.8430549277621,-5.69677006679445,
0.));
#186585=CARTESIAN_POINT('Ctrl Pts',(24.8430549277621,-5.69677006679445,
12.));
#186586=CARTESIAN_POINT('Ctrl Pts',(24.8636067597669,-5.71447804252028,
0.));
#186587=CARTESIAN_POINT('Ctrl Pts',(24.8636067597669,-5.71447804252028,
12.));
#186588=CARTESIAN_POINT('Ctrl Pts',(24.884173146722,-5.73228037976928,0.));
#186589=CARTESIAN_POINT('Ctrl Pts',(24.884173146722,-5.73228037976928,12.));
#186590=CARTESIAN_POINT('Ctrl Pts',(24.904753637648,-5.75017697890805,0.));
#186591=CARTESIAN_POINT('Ctrl Pts',(24.904753637648,-5.75017697890805,12.));
#186592=CARTESIAN_POINT('Ctrl Pts',(24.9253478043656,-5.76816774342221,
0.));
#186593=CARTESIAN_POINT('Ctrl Pts',(24.9253478043656,-5.76816774342221,
12.));
#186594=CARTESIAN_POINT('Ctrl Pts',(24.945955229334,-5.78625257775682,0.));
#186595=CARTESIAN_POINT('Ctrl Pts',(24.945955229334,-5.78625257775682,12.));
#186596=CARTESIAN_POINT('Ctrl Pts',(24.9665754954496,-5.80443138549727,
0.));
#186597=CARTESIAN_POINT('Ctrl Pts',(24.9665754954496,-5.80443138549727,
12.));
#186598=CARTESIAN_POINT('Ctrl Pts',(24.9872081752734,-5.822704067442,0.));
#186599=CARTESIAN_POINT('Ctrl Pts',(24.9872081752734,-5.822704067442,12.));
#186600=CARTESIAN_POINT('Ctrl Pts',(25.0078528200564,-5.84107051963072,
0.));
#186601=CARTESIAN_POINT('Ctrl Pts',(25.0078528200564,-5.84107051963072,
12.));
#186602=CARTESIAN_POINT('Ctrl Pts',(25.0285089498899,-5.85953063156827,
0.));
#186603=CARTESIAN_POINT('Ctrl Pts',(25.0285089498899,-5.85953063156827,
12.));
#186604=CARTESIAN_POINT('Ctrl Pts',(25.049176040591,-5.87808428385367,0.));
#186605=CARTESIAN_POINT('Ctrl Pts',(25.049176040591,-5.87808428385367,12.));
#186606=CARTESIAN_POINT('Ctrl Pts',(25.0698535426514,-5.89673135155515,
0.));
#186607=CARTESIAN_POINT('Ctrl Pts',(25.0698535426514,-5.89673135155515,
12.));
#186608=CARTESIAN_POINT('Ctrl Pts',(25.0905409050773,-5.91547170844448,
0.));
#186609=CARTESIAN_POINT('Ctrl Pts',(25.0905409050773,-5.91547170844448,
12.));
#186610=CARTESIAN_POINT('Ctrl Pts',(25.1112375971106,-5.93430523086836,
0.));
#186611=CARTESIAN_POINT('Ctrl Pts',(25.1112375971106,-5.93430523086836,
12.));
#186612=CARTESIAN_POINT('Ctrl Pts',(25.1319431317237,-5.95323180187379,
0.));
#186613=CARTESIAN_POINT('Ctrl Pts',(25.1319431317237,-5.95323180187379,
12.));
#186614=CARTESIAN_POINT('Ctrl Pts',(25.1526570863092,-5.97225131495618,
0.));
#186615=CARTESIAN_POINT('Ctrl Pts',(25.1526570863092,-5.97225131495618,
12.));
#186616=CARTESIAN_POINT('Ctrl Pts',(25.1733791296259,-5.99136367859755,
0.));
#186617=CARTESIAN_POINT('Ctrl Pts',(25.1733791296259,-5.99136367859755,
12.));
#186618=CARTESIAN_POINT('Ctrl Pts',(25.1941090269819,-6.01056881804614,
0.));
#186619=CARTESIAN_POINT('Ctrl Pts',(25.1941090269819,-6.01056881804614,
12.));
#186620=CARTESIAN_POINT('Ctrl Pts',(25.21484662016,-6.02986667389998,0.));
#186621=CARTESIAN_POINT('Ctrl Pts',(25.21484662016,-6.02986667389998,12.));
#186622=CARTESIAN_POINT('Ctrl Pts',(25.2355918139032,-6.04925720151219,
0.));
#186623=CARTESIAN_POINT('Ctrl Pts',(25.2355918139032,-6.04925720151219,
12.));
#186624=CARTESIAN_POINT('Ctrl Pts',(25.2521940105705,-6.06484373634547,
0.));
#186625=CARTESIAN_POINT('Ctrl Pts',(25.2521940105705,-6.06484373634547,
12.));
#186626=CARTESIAN_POINT('Ctrl Pts',(25.2646490489922,-6.07657531787491,
0.));
#186627=CARTESIAN_POINT('Ctrl Pts',(25.2646490489922,-6.07657531787491,
12.));
#186628=CARTESIAN_POINT('Ctrl Pts',(25.2729539149517,-6.08441489609794,
0.));
#186629=CARTESIAN_POINT('Ctrl Pts',(25.2729539149517,-6.08441489609794,
12.));
#186630=CARTESIAN_POINT('Ctrl Pts',(25.2771067246846,-6.088339316177,0.));
#186631=CARTESIAN_POINT('Ctrl Pts',(25.2771067246846,-6.088339316177,12.));
#186632=CARTESIAN_POINT('',(25.2771067246846,-6.088339316177,0.));
#186633=CARTESIAN_POINT('Ctrl Pts',(22.1738711152697,-4.11585220600463,
0.));
#186634=CARTESIAN_POINT('Ctrl Pts',(22.173877682324,-4.11585194677443,0.));
#186635=CARTESIAN_POINT('Ctrl Pts',(22.1739341411687,-4.11586035878288,
0.));
#186636=CARTESIAN_POINT('Ctrl Pts',(22.1741488021234,-4.11589976826168,
0.));
#186637=CARTESIAN_POINT('Ctrl Pts',(22.1746949858775,-4.11600589882846,
0.));
#186638=CARTESIAN_POINT('Ctrl Pts',(22.1758088296598,-4.1162279721707,0.));
#186639=CARTESIAN_POINT('Ctrl Pts',(22.177347426894,-4.11653973150519,0.));
#186640=CARTESIAN_POINT('Ctrl Pts',(22.179297473024,-4.11694173195005,0.));
#186641=CARTESIAN_POINT('Ctrl Pts',(22.1816414985788,-4.11743469691757,
0.));
#186642=CARTESIAN_POINT('Ctrl Pts',(22.1843613164855,-4.11801938107481,
0.));
#186643=CARTESIAN_POINT('Ctrl Pts',(22.1874419861496,-4.11869641271775,
0.));
#186644=CARTESIAN_POINT('Ctrl Pts',(22.1908725908525,-4.11946626228637,
0.));
#186645=CARTESIAN_POINT('Ctrl Pts',(22.1946440958098,-4.12032932637738,
0.));
#186646=CARTESIAN_POINT('Ctrl Pts',(22.1987479618246,-4.12128598183523,
0.));
#186647=CARTESIAN_POINT('Ctrl Pts',(22.2031746532106,-4.12233664408228,
0.));
#186648=CARTESIAN_POINT('Ctrl Pts',(22.2079143941719,-4.12348173702024,
0.));
#186649=CARTESIAN_POINT('Ctrl Pts',(22.2129576146671,-4.12472167516608,
0.));
#186650=CARTESIAN_POINT('Ctrl Pts',(22.2182956401341,-4.12605683613308,
0.));
#186651=CARTESIAN_POINT('Ctrl Pts',(22.2239207458781,-4.12748755830105,
0.));
#186652=CARTESIAN_POINT('Ctrl Pts',(22.2298258043947,-4.1290141546338,0.));
#186653=CARTESIAN_POINT('Ctrl Pts',(22.2360040565533,-4.13063692157499,
0.));
#186654=CARTESIAN_POINT('Ctrl Pts',(22.2424488153523,-4.13235615060161,
0.));
#186655=CARTESIAN_POINT('Ctrl Pts',(22.249153531779,-4.13417212558811,0.));
#186656=CARTESIAN_POINT('Ctrl Pts',(22.2561118708421,-4.13608511977227,
0.));
#186657=CARTESIAN_POINT('Ctrl Pts',(22.2633177913972,-4.13809539255423,
0.));
#186658=CARTESIAN_POINT('Ctrl Pts',(22.2707656042457,-4.14020318715992,
0.));
#186659=CARTESIAN_POINT('Ctrl Pts',(22.2784499072027,-4.14240873321985,
0.));
#186660=CARTESIAN_POINT('Ctrl Pts',(22.2863655389166,-4.14471224859297,
0.));
#186661=CARTESIAN_POINT('Ctrl Pts',(22.2945075198467,-4.14711394168557,
0.));
#186662=CARTESIAN_POINT('Ctrl Pts',(22.3028710166933,-4.14961401285523,
0.));
#186663=CARTESIAN_POINT('Ctrl Pts',(22.3114513545185,-4.15221265396991,
0.));
#186664=CARTESIAN_POINT('Ctrl Pts',(22.3202440186979,-4.15491004835282,
0.));
#186665=CARTESIAN_POINT('Ctrl Pts',(22.3292446628959,-4.15770637047891,
0.));
#186666=CARTESIAN_POINT('Ctrl Pts',(22.3384491078602,-4.16060178604165,
0.));
#186667=CARTESIAN_POINT('Ctrl Pts',(22.3478533253889,-4.16359645263189,
0.));
#186668=CARTESIAN_POINT('Ctrl Pts',(22.3574534257396,-4.16669052026601,
0.));
#186669=CARTESIAN_POINT('Ctrl Pts',(22.3672456427599,-4.16988413199458,
0.));
#186670=CARTESIAN_POINT('Ctrl Pts',(22.3772263228617,-4.17317742436146,
0.));
#186671=CARTESIAN_POINT('Ctrl Pts',(22.3873919231334,-4.17657052752826,
0.));
#186672=CARTESIAN_POINT('Ctrl Pts',(22.3977390078075,-4.18006356544883,
0.));
#186673=CARTESIAN_POINT('Ctrl Pts',(22.4082642454453,-4.18365665600852,
0.));
#186674=CARTESIAN_POINT('Ctrl Pts',(22.4189644056115,-4.18734991117722,
0.));
#186675=CARTESIAN_POINT('Ctrl Pts',(22.4298363535421,-4.19114343726943,
0.));
#186676=CARTESIAN_POINT('Ctrl Pts',(22.4408770448917,-4.19503733518862,
0.));
#186677=CARTESIAN_POINT('Ctrl Pts',(22.4520835205419,-4.19903170066356,
0.));
#186678=CARTESIAN_POINT('Ctrl Pts',(22.4634529011433,-4.20312662448172,
0.));
#186679=CARTESIAN_POINT('Ctrl Pts',(22.4749823839915,-4.20732219265649,
0.));
#186680=CARTESIAN_POINT('Ctrl Pts',(22.4866692403147,-4.21161848657429,
0.));
#186681=CARTESIAN_POINT('Ctrl Pts',(22.4985108124229,-4.21601558313909,
0.));
#186682=CARTESIAN_POINT('Ctrl Pts',(22.5105045108882,-4.22051355490198,
0.));
#186683=CARTESIAN_POINT('Ctrl Pts',(22.5226478117885,-4.22511247020041,
0.));
#186684=CARTESIAN_POINT('Ctrl Pts',(22.5349382540587,-4.22981239330733,
0.));
#186685=CARTESIAN_POINT('Ctrl Pts',(22.5473734368086,-4.23461338456714,
0.));
#186686=CARTESIAN_POINT('Ctrl Pts',(22.559951016643,-4.23951550052527,0.));
#186687=CARTESIAN_POINT('Ctrl Pts',(22.5726687049922,-4.2445187940486,0.));
#186688=CARTESIAN_POINT('Ctrl Pts',(22.5855242662479,-4.24962331444186,
0.));
#186689=CARTESIAN_POINT('Ctrl Pts',(22.5985155158637,-4.25482910755486,
0.));
#186690=CARTESIAN_POINT('Ctrl Pts',(22.611640318482,-4.26013621588304,0.));
#186691=CARTESIAN_POINT('Ctrl Pts',(22.6248965859975,-4.26554467865572,
0.));
#186692=CARTESIAN_POINT('Ctrl Pts',(22.6382822758171,-4.27105453193,0.));
#186693=CARTESIAN_POINT('Ctrl Pts',(22.6517953893303,-4.27666580869118,
0.));
#186694=CARTESIAN_POINT('Ctrl Pts',(22.665433970311,-4.2823785389406,0.));
#186695=CARTESIAN_POINT('Ctrl Pts',(22.6791961033536,-4.28819274977767,
0.));
#186696=CARTESIAN_POINT('Ctrl Pts',(22.6930799122545,-4.29410846547062,
0.));
#186697=CARTESIAN_POINT('Ctrl Pts',(22.707083558756,-4.30012570754067,0.));
#186698=CARTESIAN_POINT('Ctrl Pts',(22.7212052413384,-4.30624449484075,
0.));
#186699=CARTESIAN_POINT('Ctrl Pts',(22.7354431939926,-4.31246484362551,
0.));
#186700=CARTESIAN_POINT('Ctrl Pts',(22.7497956849852,-4.31878676761231,
0.));
#186701=CARTESIAN_POINT('Ctrl Pts',(22.764261015648,-4.32521027803748,0.));
#186702=CARTESIAN_POINT('Ctrl Pts',(22.7788375194081,-4.33173538373183,
0.));
#186703=CARTESIAN_POINT('Ctrl Pts',(22.7935235607807,-4.33836209118444,
0.));
#186704=CARTESIAN_POINT('Ctrl Pts',(22.808317534379,-4.34509040460066,0.));
#186705=CARTESIAN_POINT('Ctrl Pts',(22.8232178638873,-4.35192032594802,
0.));
#186706=CARTESIAN_POINT('Ctrl Pts',(22.838223001118,-4.3588518550056,0.));
#186707=CARTESIAN_POINT('Ctrl Pts',(22.8533314252419,-4.36588498943011,
0.));
#186708=CARTESIAN_POINT('Ctrl Pts',(22.8685416419725,-4.37301972480753,
0.));
#186709=CARTESIAN_POINT('Ctrl Pts',(22.8838521827702,-4.38025605470091,
0.));
#186710=CARTESIAN_POINT('Ctrl Pts',(22.8992616040108,-4.38759397068393,
0.));
#186711=CARTESIAN_POINT('Ctrl Pts',(22.9147684862425,-4.39503346238455,
0.));
#186712=CARTESIAN_POINT('Ctrl Pts',(22.9303714335549,-4.40257451754309,
0.));
#186713=CARTESIAN_POINT('Ctrl Pts',(22.9460690729092,-4.41021712205549,
0.));
#186714=CARTESIAN_POINT('Ctrl Pts',(22.9618600534866,-4.41796126001311,
0.));
#186715=CARTESIAN_POINT('Ctrl Pts',(22.9777430460021,-4.42580691372772,
0.));
#186716=CARTESIAN_POINT('Ctrl Pts',(22.9937167421009,-4.43375406376906,
0.));
#186717=CARTESIAN_POINT('Ctrl Pts',(23.0097798538399,-4.44180268901667,
0.));
#186718=CARTESIAN_POINT('Ctrl Pts',(23.0259311131395,-4.44995276669699,
0.));
#186719=CARTESIAN_POINT('Ctrl Pts',(23.0421692712466,-4.45820427241678,
0.));
#186720=CARTESIAN_POINT('Ctrl Pts',(23.0584930981723,-4.46655718018206,
0.));
#186721=CARTESIAN_POINT('Ctrl Pts',(23.0749013821867,-4.47501146242822,
0.));
#186722=CARTESIAN_POINT('Ctrl Pts',(23.0913929293909,-4.48356709006757,
0.));
#186723=CARTESIAN_POINT('Ctrl Pts',(23.1079665632629,-4.49222403252202,
0.));
#186724=CARTESIAN_POINT('Ctrl Pts',(23.1246211242117,-4.5009822577518,0.));
#186725=CARTESIAN_POINT('Ctrl Pts',(23.1413554691136,-4.50984173227088,
0.));
#186726=CARTESIAN_POINT('Ctrl Pts',(23.1581684708778,-4.51880242116786,
0.));
#186727=CARTESIAN_POINT('Ctrl Pts',(23.1750590180923,-4.52786428815049,
0.));
#186728=CARTESIAN_POINT('Ctrl Pts',(23.1920260146474,-4.53702729557586,
0.));
#186729=CARTESIAN_POINT('Ctrl Pts',(23.2090683793627,-4.54629140447543,
0.));
#186730=CARTESIAN_POINT('Ctrl Pts',(23.2261850456054,-4.55565657456957,
0.));
#186731=CARTESIAN_POINT('Ctrl Pts',(23.2433749609117,-4.56512276427812,
0.));
#186732=CARTESIAN_POINT('Ctrl Pts',(23.2606370866853,-4.57468993076071,
0.));
#186733=CARTESIAN_POINT('Ctrl Pts',(23.2779703978868,-4.58435802994675,
0.));
#186734=CARTESIAN_POINT('Ctrl Pts',(23.295373882719,-4.59412701655751,0.));
#186735=CARTESIAN_POINT('Ctrl Pts',(23.3128465423119,-4.60399684412176,
0.));
#186736=CARTESIAN_POINT('Ctrl Pts',(23.3303873903947,-4.6139674649785,0.));
#186737=CARTESIAN_POINT('Ctrl Pts',(23.3479954530281,-4.62403883030825,
0.));
#186738=CARTESIAN_POINT('Ctrl Pts',(23.3656697683496,-4.63421089016556,
0.));
#186739=CARTESIAN_POINT('Ctrl Pts',(23.383409386307,-4.64448359349936,0.));
#186740=CARTESIAN_POINT('Ctrl Pts',(23.4012133683957,-4.65485688816923,
0.));
#186741=CARTESIAN_POINT('Ctrl Pts',(23.4190807873798,-4.66533072094664,
0.));
#186742=CARTESIAN_POINT('Ctrl Pts',(23.4370107270444,-4.67590503753051,
0.));
#186743=CARTESIAN_POINT('Ctrl Pts',(23.4550022819852,-4.68657978258298,
0.));
#186744=CARTESIAN_POINT('Ctrl Pts',(23.4730545573849,-4.69735489975024,
0.));
#186745=CARTESIAN_POINT('Ctrl Pts',(23.491166668789,-4.70823033167821,0.));
#186746=CARTESIAN_POINT('Ctrl Pts',(23.5093377418784,-4.71920602001905,
0.));
#186747=CARTESIAN_POINT('Ctrl Pts',(23.5275669122378,-4.73028190543032,
0.));
#186748=CARTESIAN_POINT('Ctrl Pts',(23.5458533251715,-4.74145792760699,
0.));
#186749=CARTESIAN_POINT('Ctrl Pts',(23.564196135517,-4.75273402530616,0.));
#186750=CARTESIAN_POINT('Ctrl Pts',(23.5825945074535,-4.76411013636252,
0.));
#186751=CARTESIAN_POINT('Ctrl Pts',(23.6010476143099,-4.77558619769876,
0.));
#186752=CARTESIAN_POINT('Ctrl Pts',(23.6195546383625,-4.78716214532105,
0.));
#186753=CARTESIAN_POINT('Ctrl Pts',(23.6381147706581,-4.79883791433231,
0.));
#186754=CARTESIAN_POINT('Ctrl Pts',(23.6567272108631,-4.81061343896443,
0.));
#186755=CARTESIAN_POINT('Ctrl Pts',(23.6753911671023,-4.82248865259571,
0.));
#186756=CARTESIAN_POINT('Ctrl Pts',(23.6941058557971,-4.83446348776268,
0.));
#186757=CARTESIAN_POINT('Ctrl Pts',(23.7128705015014,-4.84653787616424,
0.));
#186758=CARTESIAN_POINT('Ctrl Pts',(23.7316843367308,-4.85871174865493,
0.));
#186759=CARTESIAN_POINT('Ctrl Pts',(23.7505466018239,-4.87098503527144,
0.));
#186760=CARTESIAN_POINT('Ctrl Pts',(23.7694565448044,-4.88335766525566,
0.));
#186761=CARTESIAN_POINT('Ctrl Pts',(23.7884134212381,-4.89582956706772,
0.));
#186762=CARTESIAN_POINT('Ctrl Pts',(23.8074164940897,-4.90840066839348,
0.));
#186763=CARTESIAN_POINT('Ctrl Pts',(23.8264650335721,-4.92107089613978,
0.));
#186764=CARTESIAN_POINT('Ctrl Pts',(23.8455583170062,-4.93384017643443,
0.));
#186765=CARTESIAN_POINT('Ctrl Pts',(23.8646956287172,-4.94670843465869,
0.));
#186766=CARTESIAN_POINT('Ctrl Pts',(23.883876259922,-4.95967559546566,0.));
#186767=CARTESIAN_POINT('Ctrl Pts',(23.9030995086164,-4.9727415827923,0.));
#186768=CARTESIAN_POINT('Ctrl Pts',(23.9223646794591,-4.98590631986534,
0.));
#186769=CARTESIAN_POINT('Ctrl Pts',(23.9416710836528,-4.9991697291931,0.));
#186770=CARTESIAN_POINT('Ctrl Pts',(23.9610180388271,-5.01253173257459,
0.));
#186771=CARTESIAN_POINT('Ctrl Pts',(23.9804048689228,-5.02599225112462,
0.));
#186772=CARTESIAN_POINT('Ctrl Pts',(23.9998309040747,-5.03955120528528,
0.));
#186773=CARTESIAN_POINT('Ctrl Pts',(24.0192954804896,-5.05320851483069,
0.));
#186774=CARTESIAN_POINT('Ctrl Pts',(24.0387979403268,-5.0669640988664,0.));
#186775=CARTESIAN_POINT('Ctrl Pts',(24.0583376315636,-5.08081787581271,
0.));
#186776=CARTESIAN_POINT('Ctrl Pts',(24.0779139079264,-5.09476976342618,
0.));
#186777=CARTESIAN_POINT('Ctrl Pts',(24.0975261288444,-5.10881967883126,
0.));
#186778=CARTESIAN_POINT('Ctrl Pts',(24.117173659394,-5.12296753853858,0.));
#186779=CARTESIAN_POINT('Ctrl Pts',(24.1368558702443,-5.13721325845746,
0.));
#186780=CARTESIAN_POINT('Ctrl Pts',(24.1565721375971,-5.1515567539008,0.));
#186781=CARTESIAN_POINT('Ctrl Pts',(24.1763218431344,-5.16599793957987,
0.));
#186782=CARTESIAN_POINT('Ctrl Pts',(24.1961043738755,-5.180536729614,0.));
#186783=CARTESIAN_POINT('Ctrl Pts',(24.2159191220171,-5.19517303753648,
0.));
#186784=CARTESIAN_POINT('Ctrl Pts',(24.2357654847766,-5.20990677629177,
0.));
#186785=CARTESIAN_POINT('Ctrl Pts',(24.2556428642294,-5.22473785822443,
0.));
#186786=CARTESIAN_POINT('Ctrl Pts',(24.2755506671525,-5.2396661950629,0.));
#186787=CARTESIAN_POINT('Ctrl Pts',(24.2954883048447,-5.25469169788858,
0.));
#186788=CARTESIAN_POINT('Ctrl Pts',(24.3154551932221,-5.269814277188,0.));
#186789=CARTESIAN_POINT('Ctrl Pts',(24.3354507529414,-5.28503384290649,
0.));
#186790=CARTESIAN_POINT('Ctrl Pts',(24.3554744095075,-5.30035030449065,
0.));
#186791=CARTESIAN_POINT('Ctrl Pts',(24.3755255933917,-5.31576357092527,
0.));
#186792=CARTESIAN_POINT('Ctrl Pts',(24.3956037401293,-5.33127355076035,
0.));
#186793=CARTESIAN_POINT('Ctrl Pts',(24.4157082904614,-5.34688015213538,
0.));
#186794=CARTESIAN_POINT('Ctrl Pts',(24.435838689915,-5.36258328273628,0.));
#186795=CARTESIAN_POINT('Ctrl Pts',(24.4559943883157,-5.37838284973696,
0.));
#186796=CARTESIAN_POINT('Ctrl Pts',(24.4761748393321,-5.39427875973825,
0.));
#186797=CARTESIAN_POINT('Ctrl Pts',(24.496379499983,-5.41027091869242,0.));
#186798=CARTESIAN_POINT('Ctrl Pts',(24.5166078302108,-5.4263592318342,0.));
#186799=CARTESIAN_POINT('Ctrl Pts',(24.5368592922863,-5.44254360356881,
0.));
#186800=CARTESIAN_POINT('Ctrl Pts',(24.5571333514842,-5.45882393762263,
0.));
#186801=CARTESIAN_POINT('Ctrl Pts',(24.5774294770329,-5.4752001372442,0.));
#186802=CARTESIAN_POINT('Ctrl Pts',(24.5977471429364,-5.49167210537248,
0.));
#186803=CARTESIAN_POINT('Ctrl Pts',(24.6180858289179,-5.50823974481963,
0.));
#186804=CARTESIAN_POINT('Ctrl Pts',(24.6384450211467,-5.52490295840993,
0.));
#186805=CARTESIAN_POINT('Ctrl Pts',(24.6588242134738,-5.54166164919584,
0.));
#186806=CARTESIAN_POINT('Ctrl Pts',(24.6792229061794,-5.55851572025377,
0.));
#186807=CARTESIAN_POINT('Ctrl Pts',(24.6996406035517,-5.57546507427756,
0.));
#186808=CARTESIAN_POINT('Ctrl Pts',(24.7200768119088,-5.59250961323988,
0.));
#186809=CARTESIAN_POINT('Ctrl Pts',(24.7405310372739,-5.60964923798492,
0.));
#186810=CARTESIAN_POINT('Ctrl Pts',(24.7610027835697,-5.62688384790924,
0.));
#186811=CARTESIAN_POINT('Ctrl Pts',(24.781491549672,-5.64421334042262,0.));
#186812=CARTESIAN_POINT('Ctrl Pts',(24.8019968304605,-5.66163761114922,
0.));
#186813=CARTESIAN_POINT('Ctrl Pts',(24.8225181223845,-5.67915655496543,
0.));
#186814=CARTESIAN_POINT('Ctrl Pts',(24.8430549277621,-5.69677006679445,
0.));
#186815=CARTESIAN_POINT('Ctrl Pts',(24.8636067597669,-5.71447804252028,
0.));
#186816=CARTESIAN_POINT('Ctrl Pts',(24.884173146722,-5.73228037976928,0.));
#186817=CARTESIAN_POINT('Ctrl Pts',(24.904753637648,-5.75017697890805,0.));
#186818=CARTESIAN_POINT('Ctrl Pts',(24.9253478043656,-5.76816774342221,
0.));
#186819=CARTESIAN_POINT('Ctrl Pts',(24.945955229334,-5.78625257775682,0.));
#186820=CARTESIAN_POINT('Ctrl Pts',(24.9665754954496,-5.80443138549727,
0.));
#186821=CARTESIAN_POINT('Ctrl Pts',(24.9872081752734,-5.822704067442,0.));
#186822=CARTESIAN_POINT('Ctrl Pts',(25.0078528200564,-5.84107051963072,
0.));
#186823=CARTESIAN_POINT('Ctrl Pts',(25.0285089498899,-5.85953063156827,
0.));
#186824=CARTESIAN_POINT('Ctrl Pts',(25.049176040591,-5.87808428385367,0.));
#186825=CARTESIAN_POINT('Ctrl Pts',(25.0698535426514,-5.89673135155515,
0.));
#186826=CARTESIAN_POINT('Ctrl Pts',(25.0905409050773,-5.91547170844448,
0.));
#186827=CARTESIAN_POINT('Ctrl Pts',(25.1112375971106,-5.93430523086836,
0.));
#186828=CARTESIAN_POINT('Ctrl Pts',(25.1319431317237,-5.95323180187379,
0.));
#186829=CARTESIAN_POINT('Ctrl Pts',(25.1526570863092,-5.97225131495618,
0.));
#186830=CARTESIAN_POINT('Ctrl Pts',(25.1733791296259,-5.99136367859755,
0.));
#186831=CARTESIAN_POINT('Ctrl Pts',(25.1941090269819,-6.01056881804614,
0.));
#186832=CARTESIAN_POINT('Ctrl Pts',(25.21484662016,-6.02986667389998,0.));
#186833=CARTESIAN_POINT('Ctrl Pts',(25.2355918139032,-6.04925720151219,
0.));
#186834=CARTESIAN_POINT('Ctrl Pts',(25.2521940105705,-6.06484373634547,
0.));
#186835=CARTESIAN_POINT('Ctrl Pts',(25.2646490489922,-6.07657531787491,
0.));
#186836=CARTESIAN_POINT('Ctrl Pts',(25.2729539149517,-6.08441489609794,
0.));
#186837=CARTESIAN_POINT('Ctrl Pts',(25.2771067246846,-6.088339316177,0.));
#186838=CARTESIAN_POINT('',(25.2771067246846,-6.088339316177,0.));
#186839=CARTESIAN_POINT('Origin',(19.4030938020118,-9.26120677397565,0.));
#186840=CARTESIAN_POINT('',(20.353053841303,-9.71462809124917,0.));
#186841=CARTESIAN_POINT('',(20.353053841303,-9.71462809124917,0.));
#186842=CARTESIAN_POINT('',(9.70154690100589,-4.63060338698782,0.));
#186843=CARTESIAN_POINT('Ctrl Pts',(24.9347862158358,-7.36589684767345,
0.));
#186844=CARTESIAN_POINT('Ctrl Pts',(24.9347862158358,-7.36589684767345,
12.));
#186845=CARTESIAN_POINT('Ctrl Pts',(24.9292275670674,-7.36721909028843,
0.));
#186846=CARTESIAN_POINT('Ctrl Pts',(24.9292275670674,-7.36721909028843,
12.));
#186847=CARTESIAN_POINT('Ctrl Pts',(24.9181155530543,-7.36985593120091,
0.));
#186848=CARTESIAN_POINT('Ctrl Pts',(24.9181155530543,-7.36985593120091,
12.));
#186849=CARTESIAN_POINT('Ctrl Pts',(24.901463382605,-7.37378825961676,0.));
#186850=CARTESIAN_POINT('Ctrl Pts',(24.901463382605,-7.37378825961676,12.));
#186851=CARTESIAN_POINT('Ctrl Pts',(24.8792921911115,-7.3789854964027,0.));
#186852=CARTESIAN_POINT('Ctrl Pts',(24.8792921911115,-7.3789854964027,12.));
#186853=CARTESIAN_POINT('Ctrl Pts',(24.8516310625176,-7.38540558903621,
0.));
#186854=CARTESIAN_POINT('Ctrl Pts',(24.8516310625176,-7.38540558903621,
12.));
#186855=CARTESIAN_POINT('Ctrl Pts',(24.8240228520893,-7.39174922585809,
0.));
#186856=CARTESIAN_POINT('Ctrl Pts',(24.8240228520893,-7.39174922585809,
12.));
#186857=CARTESIAN_POINT('Ctrl Pts',(24.7964676646431,-7.39801641583013,
0.));
#186858=CARTESIAN_POINT('Ctrl Pts',(24.7964676646431,-7.39801641583013,
12.));
#186859=CARTESIAN_POINT('Ctrl Pts',(24.7689656668983,-7.40420718661603,
0.));
#186860=CARTESIAN_POINT('Ctrl Pts',(24.7689656668983,-7.40420718661603,
12.));
#186861=CARTESIAN_POINT('Ctrl Pts',(24.7415170994784,-7.41032159082382,
0.));
#186862=CARTESIAN_POINT('Ctrl Pts',(24.7415170994784,-7.41032159082382,
12.));
#186863=CARTESIAN_POINT('Ctrl Pts',(24.7141222950051,-7.41635971481674,
0.));
#186864=CARTESIAN_POINT('Ctrl Pts',(24.7141222950051,-7.41635971481674,
12.));
#186865=CARTESIAN_POINT('Ctrl Pts',(24.6867816727192,-7.42232167766266,
0.));
#186866=CARTESIAN_POINT('Ctrl Pts',(24.6867816727192,-7.42232167766266,
12.));
#186867=CARTESIAN_POINT('Ctrl Pts',(24.6594957128756,-7.42820762159126,
0.));
#186868=CARTESIAN_POINT('Ctrl Pts',(24.6594957128756,-7.42820762159126,
12.));
#186869=CARTESIAN_POINT('Ctrl Pts',(24.6322649369517,-7.43401770489524,
0.));
#186870=CARTESIAN_POINT('Ctrl Pts',(24.6322649369517,-7.43401770489524,
12.));
#186871=CARTESIAN_POINT('Ctrl Pts',(24.6050898852368,-7.43975209375504,
0.));
#186872=CARTESIAN_POINT('Ctrl Pts',(24.6050898852368,-7.43975209375504,
12.));
#186873=CARTESIAN_POINT('Ctrl Pts',(24.577971096086,-7.44541095473135,0.));
#186874=CARTESIAN_POINT('Ctrl Pts',(24.577971096086,-7.44541095473135,12.));
#186875=CARTESIAN_POINT('Ctrl Pts',(24.5509090831559,-7.4509944465116,0.));
#186876=CARTESIAN_POINT('Ctrl Pts',(24.5509090831559,-7.4509944465116,12.));
#186877=CARTESIAN_POINT('Ctrl Pts',(24.5239043173072,-7.45650271335862,
0.));
#186878=CARTESIAN_POINT('Ctrl Pts',(24.5239043173072,-7.45650271335862,
12.));
#186879=CARTESIAN_POINT('Ctrl Pts',(24.4969572391483,-7.46193588961464,
0.));
#186880=CARTESIAN_POINT('Ctrl Pts',(24.4969572391483,-7.46193588961464,
12.));
#186881=CARTESIAN_POINT('Ctrl Pts',(24.4700682684524,-7.46729410308787,
0.));
#186882=CARTESIAN_POINT('Ctrl Pts',(24.4700682684524,-7.46729410308787,
12.));
#186883=CARTESIAN_POINT('Ctrl Pts',(24.443237814649,-7.47257747883246,0.));
#186884=CARTESIAN_POINT('Ctrl Pts',(24.443237814649,-7.47257747883246,12.));
#186885=CARTESIAN_POINT('Ctrl Pts',(24.4164662871163,-7.47778614286565,
0.));
#186886=CARTESIAN_POINT('Ctrl Pts',(24.4164662871163,-7.47778614286565,
12.));
#186887=CARTESIAN_POINT('Ctrl Pts',(24.3897541049254,-7.48292022569301,
0.));
#186888=CARTESIAN_POINT('Ctrl Pts',(24.3897541049254,-7.48292022569301,
12.));
#186889=CARTESIAN_POINT('Ctrl Pts',(24.3631017084524,-7.48797986651909,
0.));
#186890=CARTESIAN_POINT('Ctrl Pts',(24.3631017084524,-7.48797986651909,
12.));
#186891=CARTESIAN_POINT('Ctrl Pts',(24.3365095573685,-7.49296521252421,
0.));
#186892=CARTESIAN_POINT('Ctrl Pts',(24.3365095573685,-7.49296521252421,
12.));
#186893=CARTESIAN_POINT('Ctrl Pts',(24.3099781253355,-7.49787641695439,
0.));
#186894=CARTESIAN_POINT('Ctrl Pts',(24.3099781253355,-7.49787641695439,
12.));
#186895=CARTESIAN_POINT('Ctrl Pts',(24.2835078958973,-7.50271363765152,
0.));
#186896=CARTESIAN_POINT('Ctrl Pts',(24.2835078958973,-7.50271363765152,
12.));
#186897=CARTESIAN_POINT('Ctrl Pts',(24.2570993577034,-7.50747703535134,
0.));
#186898=CARTESIAN_POINT('Ctrl Pts',(24.2570993577034,-7.50747703535134,
12.));
#186899=CARTESIAN_POINT('Ctrl Pts',(24.2307530003887,-7.51216677222181,
0.));
#186900=CARTESIAN_POINT('Ctrl Pts',(24.2307530003887,-7.51216677222181,
12.));
#186901=CARTESIAN_POINT('Ctrl Pts',(24.2044693092349,-7.51678300997949,
0.));
#186902=CARTESIAN_POINT('Ctrl Pts',(24.2044693092349,-7.51678300997949,
12.));
#186903=CARTESIAN_POINT('Ctrl Pts',(24.1782487641594,-7.52132590953802,
0.));
#186904=CARTESIAN_POINT('Ctrl Pts',(24.1782487641594,-7.52132590953802,
12.));
#186905=CARTESIAN_POINT('Ctrl Pts',(24.1520918425364,-7.52579563201424,
0.));
#186906=CARTESIAN_POINT('Ctrl Pts',(24.1520918425364,-7.52579563201424,
12.));
#186907=CARTESIAN_POINT('Ctrl Pts',(24.1259990209207,-7.53019233935502,
0.));
#186908=CARTESIAN_POINT('Ctrl Pts',(24.1259990209207,-7.53019233935502,
12.));
#186909=CARTESIAN_POINT('Ctrl Pts',(24.0999707772642,-7.53451619514649,
0.));
#186910=CARTESIAN_POINT('Ctrl Pts',(24.0999707772642,-7.53451619514649,
12.));
#186911=CARTESIAN_POINT('Ctrl Pts',(24.0740075927985,-7.53876736531014,
0.));
#186912=CARTESIAN_POINT('Ctrl Pts',(24.0740075927985,-7.53876736531014,
12.));
#186913=CARTESIAN_POINT('Ctrl Pts',(24.0481099543353,-7.54294601896145,
0.));
#186914=CARTESIAN_POINT('Ctrl Pts',(24.0481099543353,-7.54294601896145,
12.));
#186915=CARTESIAN_POINT('Ctrl Pts',(24.022278355453,-7.5470523288591,0.));
#186916=CARTESIAN_POINT('Ctrl Pts',(24.022278355453,-7.5470523288591,12.));
#186917=CARTESIAN_POINT('Ctrl Pts',(23.9965132953185,-7.55108647097441,
0.));
#186918=CARTESIAN_POINT('Ctrl Pts',(23.9965132953185,-7.55108647097441,
12.));
#186919=CARTESIAN_POINT('Ctrl Pts',(23.9708152779884,-7.55504862424812,
0.));
#186920=CARTESIAN_POINT('Ctrl Pts',(23.9708152779884,-7.55504862424812,
12.));
#186921=CARTESIAN_POINT('Ctrl Pts',(23.9451848115,-7.55893897027683,0.));
#186922=CARTESIAN_POINT('Ctrl Pts',(23.9451848115,-7.55893897027683,12.));
#186923=CARTESIAN_POINT('Ctrl Pts',(23.9196224070759,-7.56275769304773,
0.));
#186924=CARTESIAN_POINT('Ctrl Pts',(23.9196224070759,-7.56275769304773,
12.));
#186925=CARTESIAN_POINT('Ctrl Pts',(23.8941285782003,-7.56650497863792,
0.));
#186926=CARTESIAN_POINT('Ctrl Pts',(23.8941285782003,-7.56650497863792,
12.));
#186927=CARTESIAN_POINT('Ctrl Pts',(23.8687038399597,-7.57018101500711,
0.));
#186928=CARTESIAN_POINT('Ctrl Pts',(23.8687038399597,-7.57018101500711,
12.));
#186929=CARTESIAN_POINT('Ctrl Pts',(23.8433487096134,-7.57378599219817,
0.));
#186930=CARTESIAN_POINT('Ctrl Pts',(23.8433487096134,-7.57378599219817,
12.));
#186931=CARTESIAN_POINT('Ctrl Pts',(23.8180637069977,-7.57732010249066,
0.));
#186932=CARTESIAN_POINT('Ctrl Pts',(23.8180637069977,-7.57732010249066,
12.));
#186933=CARTESIAN_POINT('Ctrl Pts',(23.7928493549908,-7.58078354058212,
0.));
#186934=CARTESIAN_POINT('Ctrl Pts',(23.7928493549908,-7.58078354058212,
12.));
#186935=CARTESIAN_POINT('Ctrl Pts',(23.7677061799376,-7.58417650376272,
0.));
#186936=CARTESIAN_POINT('Ctrl Pts',(23.7677061799376,-7.58417650376272,
12.));
#186937=CARTESIAN_POINT('Ctrl Pts',(23.7426347121006,-7.58749919210832,
0.));
#186938=CARTESIAN_POINT('Ctrl Pts',(23.7426347121006,-7.58749919210832,
12.));
#186939=CARTESIAN_POINT('Ctrl Pts',(23.7176354860457,-7.59075180865327,
0.));
#186940=CARTESIAN_POINT('Ctrl Pts',(23.7176354860457,-7.59075180865327,
12.));
#186941=CARTESIAN_POINT('Ctrl Pts',(23.6927090405067,-7.59393455934042,
0.));
#186942=CARTESIAN_POINT('Ctrl Pts',(23.6927090405067,-7.59393455934042,
12.));
#186943=CARTESIAN_POINT('Ctrl Pts',(23.6678559182876,-7.59704765299572,
0.));
#186944=CARTESIAN_POINT('Ctrl Pts',(23.6678559182876,-7.59704765299572,
12.));
#186945=CARTESIAN_POINT('Ctrl Pts',(23.6430766661419,-7.6000913013013,0.));
#186946=CARTESIAN_POINT('Ctrl Pts',(23.6430766661419,-7.6000913013013,12.));
#186947=CARTESIAN_POINT('Ctrl Pts',(23.6183718346576,-7.60306571877806,
0.));
#186948=CARTESIAN_POINT('Ctrl Pts',(23.6183718346576,-7.60306571877806,
12.));
#186949=CARTESIAN_POINT('Ctrl Pts',(23.5937419781244,-7.60597112277094,
0.));
#186950=CARTESIAN_POINT('Ctrl Pts',(23.5937419781244,-7.60597112277094,
12.));
#186951=CARTESIAN_POINT('Ctrl Pts',(23.5691876544243,-7.608807733446,0.));
#186952=CARTESIAN_POINT('Ctrl Pts',(23.5691876544243,-7.608807733446,12.));
#186953=CARTESIAN_POINT('Ctrl Pts',(23.5447094252028,-7.61157577385372,
0.));
#186954=CARTESIAN_POINT('Ctrl Pts',(23.5447094252028,-7.61157577385372,
12.));
#186955=CARTESIAN_POINT('Ctrl Pts',(23.5203078560128,-7.61427546999299,
0.));
#186956=CARTESIAN_POINT('Ctrl Pts',(23.5203078560128,-7.61427546999299,
12.));
#186957=CARTESIAN_POINT('Ctrl Pts',(23.4959835164608,-7.61690705088319,
0.));
#186958=CARTESIAN_POINT('Ctrl Pts',(23.4959835164608,-7.61690705088319,
12.));
#186959=CARTESIAN_POINT('Ctrl Pts',(23.4717369803438,-7.61947074863978,
0.));
#186960=CARTESIAN_POINT('Ctrl Pts',(23.4717369803438,-7.61947074863978,
12.));
#186961=CARTESIAN_POINT('Ctrl Pts',(23.4475688257854,-7.62196679855957,
0.));
#186962=CARTESIAN_POINT('Ctrl Pts',(23.4475688257854,-7.62196679855957,
12.));
#186963=CARTESIAN_POINT('Ctrl Pts',(23.4234796353544,-7.62439543920055,
0.));
#186964=CARTESIAN_POINT('Ctrl Pts',(23.4234796353544,-7.62439543920055,
12.));
#186965=CARTESIAN_POINT('Ctrl Pts',(23.3994699961122,-7.62675691240335,
0.));
#186966=CARTESIAN_POINT('Ctrl Pts',(23.3994699961122,-7.62675691240335,
12.));
#186967=CARTESIAN_POINT('Ctrl Pts',(23.3755404996638,-7.62905146332598,
0.));
#186968=CARTESIAN_POINT('Ctrl Pts',(23.3755404996638,-7.62905146332598,
12.));
#186969=CARTESIAN_POINT('Ctrl Pts',(23.3516917421973,-7.63127934048139,
0.));
#186970=CARTESIAN_POINT('Ctrl Pts',(23.3516917421973,-7.63127934048139,
12.));
#186971=CARTESIAN_POINT('Ctrl Pts',(23.3279243245241,-7.63344079578163,
0.));
#186972=CARTESIAN_POINT('Ctrl Pts',(23.3279243245241,-7.63344079578163,
12.));
#186973=CARTESIAN_POINT('Ctrl Pts',(23.3042388521021,-7.63553608458784,
0.));
#186974=CARTESIAN_POINT('Ctrl Pts',(23.3042388521021,-7.63553608458784,
12.));
#186975=CARTESIAN_POINT('Ctrl Pts',(23.2806359350853,-7.63756546576375,
0.));
#186976=CARTESIAN_POINT('Ctrl Pts',(23.2806359350853,-7.63756546576375,
12.));
#186977=CARTESIAN_POINT('Ctrl Pts',(23.2571161884487,-7.63952920172837,
0.));
#186978=CARTESIAN_POINT('Ctrl Pts',(23.2571161884487,-7.63952920172837,
12.));
#186979=CARTESIAN_POINT('Ctrl Pts',(23.2336802320912,-7.64142755851508,
0.));
#186980=CARTESIAN_POINT('Ctrl Pts',(23.2336802320912,-7.64142755851508,
12.));
#186981=CARTESIAN_POINT('Ctrl Pts',(23.2103286909399,-7.64326080583684,
0.));
#186982=CARTESIAN_POINT('Ctrl Pts',(23.2103286909399,-7.64326080583684,
12.));
#186983=CARTESIAN_POINT('Ctrl Pts',(23.1870621950452,-7.64502921715483,
0.));
#186984=CARTESIAN_POINT('Ctrl Pts',(23.1870621950452,-7.64502921715483,
12.));
#186985=CARTESIAN_POINT('Ctrl Pts',(23.1638813796691,-7.64673306975797,
0.));
#186986=CARTESIAN_POINT('Ctrl Pts',(23.1638813796691,-7.64673306975797,
12.));
#186987=CARTESIAN_POINT('Ctrl Pts',(23.1407868853815,-7.64837264482929,
0.));
#186988=CARTESIAN_POINT('Ctrl Pts',(23.1407868853815,-7.64837264482929,
12.));
#186989=CARTESIAN_POINT('Ctrl Pts',(23.1177793581674,-7.64994822749845,
0.));
#186990=CARTESIAN_POINT('Ctrl Pts',(23.1177793581674,-7.64994822749845,
12.));
#186991=CARTESIAN_POINT('Ctrl Pts',(23.0948594495246,-7.65146010690465,
0.));
#186992=CARTESIAN_POINT('Ctrl Pts',(23.0948594495246,-7.65146010690465,
12.));
#186993=CARTESIAN_POINT('Ctrl Pts',(23.072027816555,-7.65290857626357,0.));
#186994=CARTESIAN_POINT('Ctrl Pts',(23.072027816555,-7.65290857626357,12.));
#186995=CARTESIAN_POINT('Ctrl Pts',(23.049285122053,-7.65429393293955,0.));
#186996=CARTESIAN_POINT('Ctrl Pts',(23.049285122053,-7.65429393293955,12.));
#186997=CARTESIAN_POINT('Ctrl Pts',(23.0266320345792,-7.65561647852555,
0.));
#186998=CARTESIAN_POINT('Ctrl Pts',(23.0266320345792,-7.65561647852555,
12.));
#186999=CARTESIAN_POINT('Ctrl Pts',(23.004069228582,-7.6568765189133,0.));
#187000=CARTESIAN_POINT('Ctrl Pts',(23.004069228582,-7.6568765189133,12.));
#187001=CARTESIAN_POINT('Ctrl Pts',(22.9815973845301,-7.65807436436453,
0.));
#187002=CARTESIAN_POINT('Ctrl Pts',(22.9815973845301,-7.65807436436453,
12.));
#187003=CARTESIAN_POINT('Ctrl Pts',(22.9592171890332,-7.65921032958912,
0.));
#187004=CARTESIAN_POINT('Ctrl Pts',(22.9592171890332,-7.65921032958912,
12.));
#187005=CARTESIAN_POINT('Ctrl Pts',(22.9369293349592,-7.66028473382777,
0.));
#187006=CARTESIAN_POINT('Ctrl Pts',(22.9369293349592,-7.66028473382777,
12.));
#187007=CARTESIAN_POINT('Ctrl Pts',(22.9147345215418,-7.661297900941,0.));
#187008=CARTESIAN_POINT('Ctrl Pts',(22.9147345215418,-7.661297900941,12.));
#187009=CARTESIAN_POINT('Ctrl Pts',(22.8926334544879,-7.66225015950148,
0.));
#187010=CARTESIAN_POINT('Ctrl Pts',(22.8926334544879,-7.66225015950148,
12.));
#187011=CARTESIAN_POINT('Ctrl Pts',(22.870626846128,-7.66314184287334,0.));
#187012=CARTESIAN_POINT('Ctrl Pts',(22.870626846128,-7.66314184287334,12.));
#187013=CARTESIAN_POINT('Ctrl Pts',(22.8487154155569,-7.66397328929805,
0.));
#187014=CARTESIAN_POINT('Ctrl Pts',(22.8487154155569,-7.66397328929805,
12.));
#187015=CARTESIAN_POINT('Ctrl Pts',(22.8268998887678,-7.66474484198553,
0.));
#187016=CARTESIAN_POINT('Ctrl Pts',(22.8268998887678,-7.66474484198553,
12.));
#187017=CARTESIAN_POINT('Ctrl Pts',(22.8051809987833,-7.66545684920988,
0.));
#187018=CARTESIAN_POINT('Ctrl Pts',(22.8051809987833,-7.66545684920988,
12.));
#187019=CARTESIAN_POINT('Ctrl Pts',(22.7835594857697,-7.66610966441259,
0.));
#187020=CARTESIAN_POINT('Ctrl Pts',(22.7835594857697,-7.66610966441259,
12.));
#187021=CARTESIAN_POINT('Ctrl Pts',(22.7620360971839,-7.66670364630273,
0.));
#187022=CARTESIAN_POINT('Ctrl Pts',(22.7620360971839,-7.66670364630273,
12.));
#187023=CARTESIAN_POINT('Ctrl Pts',(22.7406115879508,-7.66723915895413,
0.));
#187024=CARTESIAN_POINT('Ctrl Pts',(22.7406115879508,-7.66723915895413,
12.));
#187025=CARTESIAN_POINT('Ctrl Pts',(22.7192867206242,-7.6677165719101,0.));
#187026=CARTESIAN_POINT('Ctrl Pts',(22.7192867206242,-7.6677165719101,12.));
#187027=CARTESIAN_POINT('Ctrl Pts',(22.6980622655446,-7.66813626029277,
0.));
#187028=CARTESIAN_POINT('Ctrl Pts',(22.6980622655446,-7.66813626029277,
12.));
#187029=CARTESIAN_POINT('Ctrl Pts',(22.6769390009889,-7.66849860491763,
0.));
#187030=CARTESIAN_POINT('Ctrl Pts',(22.6769390009889,-7.66849860491763,
12.));
#187031=CARTESIAN_POINT('Ctrl Pts',(22.6559177133133,-7.66880399241354,
0.));
#187032=CARTESIAN_POINT('Ctrl Pts',(22.6559177133133,-7.66880399241354,
12.));
#187033=CARTESIAN_POINT('Ctrl Pts',(22.6349991971547,-7.66905281533745,
0.));
#187034=CARTESIAN_POINT('Ctrl Pts',(22.6349991971547,-7.66905281533745,
12.));
#187035=CARTESIAN_POINT('Ctrl Pts',(22.6141842556248,-7.66924547229435,
0.));
#187036=CARTESIAN_POINT('Ctrl Pts',(22.6141842556248,-7.66924547229435,
12.));
#187037=CARTESIAN_POINT('Ctrl Pts',(22.5934737004955,-7.66938236806241,
0.));
#187038=CARTESIAN_POINT('Ctrl Pts',(22.5934737004955,-7.66938236806241,
12.));
#187039=CARTESIAN_POINT('Ctrl Pts',(22.5728683523828,-7.66946391372299,
0.));
#187040=CARTESIAN_POINT('Ctrl Pts',(22.5728683523828,-7.66946391372299,
12.));
#187041=CARTESIAN_POINT('Ctrl Pts',(22.5523690409109,-7.66949052679672,
0.));
#187042=CARTESIAN_POINT('Ctrl Pts',(22.5523690409109,-7.66949052679672,
12.));
#187043=CARTESIAN_POINT('Ctrl Pts',(22.5319766049191,-7.66946263138116,
0.));
#187044=CARTESIAN_POINT('Ctrl Pts',(22.5319766049191,-7.66946263138116,
12.));
#187045=CARTESIAN_POINT('Ctrl Pts',(22.5116918927023,-7.66938065829083,
0.));
#187046=CARTESIAN_POINT('Ctrl Pts',(22.5116918927023,-7.66938065829083,
12.));
#187047=CARTESIAN_POINT('Ctrl Pts',(22.4915157622308,-7.66924504520302,
0.));
#187048=CARTESIAN_POINT('Ctrl Pts',(22.4915157622308,-7.66924504520302,
12.));
#187049=CARTESIAN_POINT('Ctrl Pts',(22.47144908137,-7.66905623680836,0.));
#187050=CARTESIAN_POINT('Ctrl Pts',(22.47144908137,-7.66905623680836,12.));
#187051=CARTESIAN_POINT('Ctrl Pts',(22.4514927280862,-7.6688146849666,0.));
#187052=CARTESIAN_POINT('Ctrl Pts',(22.4514927280862,-7.6688146849666,12.));
#187053=CARTESIAN_POINT('Ctrl Pts',(22.4316475906616,-7.66852084886746,
0.));
#187054=CARTESIAN_POINT('Ctrl Pts',(22.4316475906616,-7.66852084886746,
12.));
#187055=CARTESIAN_POINT('Ctrl Pts',(22.411914567977,-7.66817519519682,0.));
#187056=CARTESIAN_POINT('Ctrl Pts',(22.411914567977,-7.66817519519682,12.));
#187057=CARTESIAN_POINT('Ctrl Pts',(22.3922945697782,-7.6677781983082,0.));
#187058=CARTESIAN_POINT('Ctrl Pts',(22.3922945697782,-7.6677781983082,12.));
#187059=CARTESIAN_POINT('Ctrl Pts',(22.3727885169361,-7.66733034039887,
0.));
#187060=CARTESIAN_POINT('Ctrl Pts',(22.3727885169361,-7.66733034039887,
12.));
#187061=CARTESIAN_POINT('Ctrl Pts',(22.3533973417013,-7.66683211169134,
0.));
#187062=CARTESIAN_POINT('Ctrl Pts',(22.3533973417013,-7.66683211169134,
12.));
#187063=CARTESIAN_POINT('Ctrl Pts',(22.3341219879454,-7.66628401061906,
0.));
#187064=CARTESIAN_POINT('Ctrl Pts',(22.3341219879454,-7.66628401061906,
12.));
#187065=CARTESIAN_POINT('Ctrl Pts',(22.3149634114823,-7.66568654402442,
0.));
#187066=CARTESIAN_POINT('Ctrl Pts',(22.3149634114823,-7.66568654402442,
12.));
#187067=CARTESIAN_POINT('Ctrl Pts',(22.2959225803925,-7.66504022736263,
0.));
#187068=CARTESIAN_POINT('Ctrl Pts',(22.2959225803925,-7.66504022736263,
12.));
#187069=CARTESIAN_POINT('Ctrl Pts',(22.2770004753332,-7.66434558490973,
0.));
#187070=CARTESIAN_POINT('Ctrl Pts',(22.2770004753332,-7.66434558490973,
12.));
#187071=CARTESIAN_POINT('Ctrl Pts',(22.2581980898487,-7.66360314997662,
0.));
#187072=CARTESIAN_POINT('Ctrl Pts',(22.2581980898487,-7.66360314997662,
12.));
#187073=CARTESIAN_POINT('Ctrl Pts',(22.239516430656,-7.66281346512546,0.));
#187074=CARTESIAN_POINT('Ctrl Pts',(22.239516430656,-7.66281346512546,12.));
#187075=CARTESIAN_POINT('Ctrl Pts',(22.2209565180098,-7.66197708240436,
0.));
#187076=CARTESIAN_POINT('Ctrl Pts',(22.2209565180098,-7.66197708240436,
12.));
#187077=CARTESIAN_POINT('Ctrl Pts',(22.2025193860972,-7.66109456359292,
0.));
#187078=CARTESIAN_POINT('Ctrl Pts',(22.2025193860972,-7.66109456359292,
12.));
#187079=CARTESIAN_POINT('Ctrl Pts',(22.1842060834092,-7.66016648045008,
0.));
#187080=CARTESIAN_POINT('Ctrl Pts',(22.1842060834092,-7.66016648045008,
12.));
#187081=CARTESIAN_POINT('Ctrl Pts',(22.1660176731174,-7.65919341496926,
0.));
#187082=CARTESIAN_POINT('Ctrl Pts',(22.1660176731174,-7.65919341496926,
12.));
#187083=CARTESIAN_POINT('Ctrl Pts',(22.1479552334206,-7.65817595963351,
0.));
#187084=CARTESIAN_POINT('Ctrl Pts',(22.1479552334206,-7.65817595963351,
12.));
#187085=CARTESIAN_POINT('Ctrl Pts',(22.1300198579671,-7.65711471769407,
0.));
#187086=CARTESIAN_POINT('Ctrl Pts',(22.1300198579671,-7.65711471769407,
12.));
#187087=CARTESIAN_POINT('Ctrl Pts',(22.1122126563327,-7.65601030346819,
0.));
#187088=CARTESIAN_POINT('Ctrl Pts',(22.1122126563327,-7.65601030346819,
12.));
#187089=CARTESIAN_POINT('Ctrl Pts',(22.094534754469,-7.65486334263651,0.));
#187090=CARTESIAN_POINT('Ctrl Pts',(22.094534754469,-7.65486334263651,12.));
#187091=CARTESIAN_POINT('Ctrl Pts',(22.0769872951596,-7.65367447254945,
0.));
#187092=CARTESIAN_POINT('Ctrl Pts',(22.0769872951596,-7.65367447254945,
12.));
#187093=CARTESIAN_POINT('Ctrl Pts',(22.0595714384432,-7.65244434253104,
0.));
#187094=CARTESIAN_POINT('Ctrl Pts',(22.0595714384432,-7.65244434253104,
12.));
#187095=CARTESIAN_POINT('Ctrl Pts',(22.0422883621176,-7.65117361421347,
0.));
#187096=CARTESIAN_POINT('Ctrl Pts',(22.0422883621176,-7.65117361421347,
12.));
#187097=CARTESIAN_POINT('Ctrl Pts',(22.0251392623209,-7.64986296190157,
0.));
#187098=CARTESIAN_POINT('Ctrl Pts',(22.0251392623209,-7.64986296190157,
12.));
#187099=CARTESIAN_POINT('Ctrl Pts',(22.0081253540773,-7.64851307293346,
0.));
#187100=CARTESIAN_POINT('Ctrl Pts',(22.0081253540773,-7.64851307293346,
12.));
#187101=CARTESIAN_POINT('Ctrl Pts',(21.9912478718542,-7.64712464805258,
0.));
#187102=CARTESIAN_POINT('Ctrl Pts',(21.9912478718542,-7.64712464805258,
12.));
#187103=CARTESIAN_POINT('Ctrl Pts',(21.97450807008,-7.64569840177359,0.));
#187104=CARTESIAN_POINT('Ctrl Pts',(21.97450807008,-7.64569840177359,12.));
#187105=CARTESIAN_POINT('Ctrl Pts',(21.9579072237653,-7.64423506279154,
0.));
#187106=CARTESIAN_POINT('Ctrl Pts',(21.9579072237653,-7.64423506279154,
12.));
#187107=CARTESIAN_POINT('Ctrl Pts',(21.9414466292074,-7.64273537442707,
0.));
#187108=CARTESIAN_POINT('Ctrl Pts',(21.9414466292074,-7.64273537442707,
12.));
#187109=CARTESIAN_POINT('Ctrl Pts',(21.9251276046546,-7.6412000950654,0.));
#187110=CARTESIAN_POINT('Ctrl Pts',(21.9251276046546,-7.6412000950654,12.));
#187111=CARTESIAN_POINT('Ctrl Pts',(21.9089514909873,-7.63962999860917,
0.));
#187112=CARTESIAN_POINT('Ctrl Pts',(21.9089514909873,-7.63962999860917,
12.));
#187113=CARTESIAN_POINT('Ctrl Pts',(21.8929196523511,-7.63802587492008,
0.));
#187114=CARTESIAN_POINT('Ctrl Pts',(21.8929196523511,-7.63802587492008,
12.));
#187115=CARTESIAN_POINT('Ctrl Pts',(21.8770334769492,-7.63638853033368,
0.));
#187116=CARTESIAN_POINT('Ctrl Pts',(21.8770334769492,-7.63638853033368,
12.));
#187117=CARTESIAN_POINT('Ctrl Pts',(21.8612943779086,-7.63471878821204,
0.));
#187118=CARTESIAN_POINT('Ctrl Pts',(21.8612943779086,-7.63471878821204,
12.));
#187119=CARTESIAN_POINT('Ctrl Pts',(21.8457037941084,-7.63301748948936,
0.));
#187120=CARTESIAN_POINT('Ctrl Pts',(21.8457037941084,-7.63301748948936,
12.));
#187121=CARTESIAN_POINT('Ctrl Pts',(21.8302631910197,-7.6312854932304,0.));
#187122=CARTESIAN_POINT('Ctrl Pts',(21.8302631910197,-7.6312854932304,12.));
#187123=CARTESIAN_POINT('Ctrl Pts',(21.8149740615093,-7.62952367718151,
0.));
#187124=CARTESIAN_POINT('Ctrl Pts',(21.8149740615093,-7.62952367718151,
12.));
#187125=CARTESIAN_POINT('Ctrl Pts',(21.7998379268583,-7.62773293842409,
0.));
#187126=CARTESIAN_POINT('Ctrl Pts',(21.7998379268583,-7.62773293842409,
12.));
#187127=CARTESIAN_POINT('Ctrl Pts',(21.7848563378022,-7.62591419404521,
0.));
#187128=CARTESIAN_POINT('Ctrl Pts',(21.7848563378022,-7.62591419404521,
12.));
#187129=CARTESIAN_POINT('Ctrl Pts',(21.7700308755583,-7.62406838181164,
0.));
#187130=CARTESIAN_POINT('Ctrl Pts',(21.7700308755583,-7.62406838181164,
12.));
#187131=CARTESIAN_POINT('Ctrl Pts',(21.7553631528329,-7.62219646084226,
0.));
#187132=CARTESIAN_POINT('Ctrl Pts',(21.7553631528329,-7.62219646084226,
12.));
#187133=CARTESIAN_POINT('Ctrl Pts',(21.7408548148657,-7.62029941230855,
0.));
#187134=CARTESIAN_POINT('Ctrl Pts',(21.7408548148657,-7.62029941230855,
12.));
#187135=CARTESIAN_POINT('Ctrl Pts',(21.7265075407977,-7.61837824030542,
0.));
#187136=CARTESIAN_POINT('Ctrl Pts',(21.7265075407977,-7.61837824030542,
12.));
#187137=CARTESIAN_POINT('Ctrl Pts',(21.7123230449835,-7.61643397270425,
0.));
#187138=CARTESIAN_POINT('Ctrl Pts',(21.7123230449835,-7.61643397270425,
12.));
#187139=CARTESIAN_POINT('Ctrl Pts',(21.6983030783321,-7.61446766202787,
0.));
#187140=CARTESIAN_POINT('Ctrl Pts',(21.6983030783321,-7.61446766202787,
12.));
#187141=CARTESIAN_POINT('Ctrl Pts',(21.6844494295813,-7.61248038630265,
0.));
#187142=CARTESIAN_POINT('Ctrl Pts',(21.6844494295813,-7.61248038630265,
12.));
#187143=CARTESIAN_POINT('Ctrl Pts',(21.6707639267573,-7.6104732500095,0.));
#187144=CARTESIAN_POINT('Ctrl Pts',(21.6707639267573,-7.6104732500095,12.));
#187145=CARTESIAN_POINT('Ctrl Pts',(21.6572484388079,-7.60844738512872,
0.));
#187146=CARTESIAN_POINT('Ctrl Pts',(21.6572484388079,-7.60844738512872,
12.));
#187147=CARTESIAN_POINT('Ctrl Pts',(21.6439048771743,-7.60640395216359,
0.));
#187148=CARTESIAN_POINT('Ctrl Pts',(21.6439048771743,-7.60640395216359,
12.));
#187149=CARTESIAN_POINT('Ctrl Pts',(21.6307351973823,-7.604344141183,0.));
#187150=CARTESIAN_POINT('Ctrl Pts',(21.6307351973823,-7.604344141183,12.));
#187151=CARTESIAN_POINT('Ctrl Pts',(21.6177414005991,-7.60226917285432,
0.));
#187152=CARTESIAN_POINT('Ctrl Pts',(21.6177414005991,-7.60226917285432,
12.));
#187153=CARTESIAN_POINT('Ctrl Pts',(21.6049255358842,-7.60018029988238,
0.));
#187154=CARTESIAN_POINT('Ctrl Pts',(21.6049255358842,-7.60018029988238,
12.));
#187155=CARTESIAN_POINT('Ctrl Pts',(21.5922897024466,-7.59807880846193,
0.));
#187156=CARTESIAN_POINT('Ctrl Pts',(21.5922897024466,-7.59807880846193,
12.));
#187157=CARTESIAN_POINT('Ctrl Pts',(21.5798360518978,-7.59596601973589,
0.));
#187158=CARTESIAN_POINT('Ctrl Pts',(21.5798360518978,-7.59596601973589,
12.));
#187159=CARTESIAN_POINT('Ctrl Pts',(21.5675667904728,-7.5938432912493,0.));
#187160=CARTESIAN_POINT('Ctrl Pts',(21.5675667904728,-7.5938432912493,12.));
#187161=CARTESIAN_POINT('Ctrl Pts',(21.5554841813465,-7.59171201844793,
0.));
#187162=CARTESIAN_POINT('Ctrl Pts',(21.5554841813465,-7.59171201844793,
12.));
#187163=CARTESIAN_POINT('Ctrl Pts',(21.5435905470113,-7.58957363620026,
0.));
#187164=CARTESIAN_POINT('Ctrl Pts',(21.5435905470113,-7.58957363620026,
12.));
#187165=CARTESIAN_POINT('Ctrl Pts',(21.5318882716735,-7.58742962034834,
0.));
#187166=CARTESIAN_POINT('Ctrl Pts',(21.5318882716735,-7.58742962034834,
12.));
#187167=CARTESIAN_POINT('Ctrl Pts',(21.5203798035294,-7.58528148919114,
0.));
#187168=CARTESIAN_POINT('Ctrl Pts',(21.5203798035294,-7.58528148919114,
12.));
#187169=CARTESIAN_POINT('Ctrl Pts',(21.5090676573866,-7.58313080519159,
0.));
#187170=CARTESIAN_POINT('Ctrl Pts',(21.5090676573866,-7.58313080519159,
12.));
#187171=CARTESIAN_POINT('Ctrl Pts',(21.4979544192739,-7.5809791779073,0.));
#187172=CARTESIAN_POINT('Ctrl Pts',(21.4979544192739,-7.5809791779073,12.));
#187173=CARTESIAN_POINT('Ctrl Pts',(21.4870427508193,-7.57882826679131,
0.));
#187174=CARTESIAN_POINT('Ctrl Pts',(21.4870427508193,-7.57882826679131,
12.));
#187175=CARTESIAN_POINT('Ctrl Pts',(21.4763353936766,-7.57667978403003,
0.));
#187176=CARTESIAN_POINT('Ctrl Pts',(21.4763353936766,-7.57667978403003,
12.));
#187177=CARTESIAN_POINT('Ctrl Pts',(21.4658351740135,-7.57453549743435,
0.));
#187178=CARTESIAN_POINT('Ctrl Pts',(21.4658351740135,-7.57453549743435,
12.));
#187179=CARTESIAN_POINT('Ctrl Pts',(21.4555450053147,-7.57239723223521,
0.));
#187180=CARTESIAN_POINT('Ctrl Pts',(21.4555450053147,-7.57239723223521,
12.));
#187181=CARTESIAN_POINT('Ctrl Pts',(21.445467890751,-7.5702668726117,0.));
#187182=CARTESIAN_POINT('Ctrl Pts',(21.445467890751,-7.5702668726117,12.));
#187183=CARTESIAN_POINT('Ctrl Pts',(21.435606926151,-7.56814636360842,0.));
#187184=CARTESIAN_POINT('Ctrl Pts',(21.435606926151,-7.56814636360842,12.));
#187185=CARTESIAN_POINT('Ctrl Pts',(21.4259653015732,-7.56603771218706,
0.));
#187186=CARTESIAN_POINT('Ctrl Pts',(21.4259653015732,-7.56603771218706,
12.));
#187187=CARTESIAN_POINT('Ctrl Pts',(21.4165463106252,-7.56394299313683,
0.));
#187188=CARTESIAN_POINT('Ctrl Pts',(21.4165463106252,-7.56394299313683,
12.));
#187189=CARTESIAN_POINT('Ctrl Pts',(21.4073533630364,-7.56186435703622,
0.));
#187190=CARTESIAN_POINT('Ctrl Pts',(21.4073533630364,-7.56186435703622,
12.));
#187191=CARTESIAN_POINT('Ctrl Pts',(21.3983899952988,-7.55980403700615,
0.));
#187192=CARTESIAN_POINT('Ctrl Pts',(21.3983899952988,-7.55980403700615,
12.));
#187193=CARTESIAN_POINT('Ctrl Pts',(21.3896598842119,-7.55776435731422,
0.));
#187194=CARTESIAN_POINT('Ctrl Pts',(21.3896598842119,-7.55776435731422,
12.));
#187195=CARTESIAN_POINT('Ctrl Pts',(21.3811668478933,-7.55574773403508,
0.));
#187196=CARTESIAN_POINT('Ctrl Pts',(21.3811668478933,-7.55574773403508,
12.));
#187197=CARTESIAN_POINT('Ctrl Pts',(21.3729148390244,-7.55375667080032,
0.));
#187198=CARTESIAN_POINT('Ctrl Pts',(21.3729148390244,-7.55375667080032,
12.));
#187199=CARTESIAN_POINT('Ctrl Pts',(21.3649079431864,-7.55179375777442,
0.));
#187200=CARTESIAN_POINT('Ctrl Pts',(21.3649079431864,-7.55179375777442,
12.));
#187201=CARTESIAN_POINT('Ctrl Pts',(21.3571503685853,-7.54986166521307,
0.));
#187202=CARTESIAN_POINT('Ctrl Pts',(21.3571503685853,-7.54986166521307,
12.));
#187203=CARTESIAN_POINT('Ctrl Pts',(21.349646476153,-7.54796316246327,0.));
#187204=CARTESIAN_POINT('Ctrl Pts',(21.349646476153,-7.54796316246327,12.));
#187205=CARTESIAN_POINT('Ctrl Pts',(21.3424008295038,-7.54610114948351,
0.));
#187206=CARTESIAN_POINT('Ctrl Pts',(21.3424008295038,-7.54610114948351,
12.));
#187207=CARTESIAN_POINT('Ctrl Pts',(21.3354182340149,-7.54427868151269,
0.));
#187208=CARTESIAN_POINT('Ctrl Pts',(21.3354182340149,-7.54427868151269,
12.));
#187209=CARTESIAN_POINT('Ctrl Pts',(21.328703791771,-7.54249900377032,0.));
#187210=CARTESIAN_POINT('Ctrl Pts',(21.328703791771,-7.54249900377032,12.));
#187211=CARTESIAN_POINT('Ctrl Pts',(21.3222628524165,-7.5407655203828,0.));
#187212=CARTESIAN_POINT('Ctrl Pts',(21.3222628524165,-7.5407655203828,12.));
#187213=CARTESIAN_POINT('Ctrl Pts',(21.3161009456256,-7.53908175169899,
0.));
#187214=CARTESIAN_POINT('Ctrl Pts',(21.3161009456256,-7.53908175169899,
12.));
#187215=CARTESIAN_POINT('Ctrl Pts',(21.3102237167729,-7.5374512936462,0.));
#187216=CARTESIAN_POINT('Ctrl Pts',(21.3102237167729,-7.5374512936462,12.));
#187217=CARTESIAN_POINT('Ctrl Pts',(21.3046368712156,-7.53587778251743,
0.));
#187218=CARTESIAN_POINT('Ctrl Pts',(21.3046368712156,-7.53587778251743,
12.));
#187219=CARTESIAN_POINT('Ctrl Pts',(21.2993464250717,-7.53436505309949,
0.));
#187220=CARTESIAN_POINT('Ctrl Pts',(21.2993464250717,-7.53436505309949,
12.));
#187221=CARTESIAN_POINT('Ctrl Pts',(21.2943588989331,-7.53291726078527,
0.));
#187222=CARTESIAN_POINT('Ctrl Pts',(21.2943588989331,-7.53291726078527,
12.));
#187223=CARTESIAN_POINT('Ctrl Pts',(21.2896816163843,-7.53153906987847,
0.));
#187224=CARTESIAN_POINT('Ctrl Pts',(21.2896816163843,-7.53153906987847,
12.));
#187225=CARTESIAN_POINT('Ctrl Pts',(21.2853226580658,-7.53023562438221,
0.));
#187226=CARTESIAN_POINT('Ctrl Pts',(21.2853226580658,-7.53023562438221,
12.));
#187227=CARTESIAN_POINT('Ctrl Pts',(21.2812902781143,-7.52901217930407,
0.));
#187228=CARTESIAN_POINT('Ctrl Pts',(21.2812902781143,-7.52901217930407,
12.));
#187229=CARTESIAN_POINT('Ctrl Pts',(21.2775925269651,-7.52787386225344,
0.));
#187230=CARTESIAN_POINT('Ctrl Pts',(21.2775925269651,-7.52787386225344,
12.));
#187231=CARTESIAN_POINT('Ctrl Pts',(21.2742366113578,-7.52682526918561,
0.));
#187232=CARTESIAN_POINT('Ctrl Pts',(21.2742366113578,-7.52682526918561,
12.));
#187233=CARTESIAN_POINT('Ctrl Pts',(21.2712301573465,-7.52587126095544,
0.));
#187234=CARTESIAN_POINT('Ctrl Pts',(21.2712301573465,-7.52587126095544,
12.));
#187235=CARTESIAN_POINT('Ctrl Pts',(21.2685823838672,-7.52501770333522,
0.));
#187236=CARTESIAN_POINT('Ctrl Pts',(21.2685823838672,-7.52501770333522,
12.));
#187237=CARTESIAN_POINT('Ctrl Pts',(21.266305915706,-7.52427261074264,0.));
#187238=CARTESIAN_POINT('Ctrl Pts',(21.266305915706,-7.52427261074264,12.));
#187239=CARTESIAN_POINT('Ctrl Pts',(21.2644161259965,-7.52364573027521,
0.));
#187240=CARTESIAN_POINT('Ctrl Pts',(21.2644161259965,-7.52364573027521,
12.));
#187241=CARTESIAN_POINT('Ctrl Pts',(21.262927782038,-7.52314642316203,0.));
#187242=CARTESIAN_POINT('Ctrl Pts',(21.262927782038,-7.52314642316203,12.));
#187243=CARTESIAN_POINT('Ctrl Pts',(21.261852128355,-7.52278182242728,0.));
#187244=CARTESIAN_POINT('Ctrl Pts',(21.261852128355,-7.52278182242728,12.));
#187245=CARTESIAN_POINT('Ctrl Pts',(21.2613260540651,-7.52260064231736,
0.));
#187246=CARTESIAN_POINT('Ctrl Pts',(21.2613260540651,-7.52260064231736,
12.));
#187247=CARTESIAN_POINT('Ctrl Pts',(21.261120447486,-7.52252744144958,0.));
#187248=CARTESIAN_POINT('Ctrl Pts',(21.261120447486,-7.52252744144958,12.));
#187249=CARTESIAN_POINT('Ctrl Pts',(21.2610673466883,-7.52250649703992,
0.));
#187250=CARTESIAN_POINT('Ctrl Pts',(21.2610673466883,-7.52250649703992,
12.));
#187251=CARTESIAN_POINT('Ctrl Pts',(21.2610617890679,-7.52250298901266,
0.));
#187252=CARTESIAN_POINT('Ctrl Pts',(21.2610617890679,-7.52250298901266,
12.));
#187253=CARTESIAN_POINT('',(24.9347862158358,-7.36589684767345,0.));
#187254=CARTESIAN_POINT('Ctrl Pts',(24.9347862158358,-7.36589684767345,
0.));
#187255=CARTESIAN_POINT('Ctrl Pts',(24.9292275670674,-7.36721909028843,
0.));
#187256=CARTESIAN_POINT('Ctrl Pts',(24.9181155530543,-7.36985593120091,
0.));
#187257=CARTESIAN_POINT('Ctrl Pts',(24.901463382605,-7.37378825961676,0.));
#187258=CARTESIAN_POINT('Ctrl Pts',(24.8792921911115,-7.3789854964027,0.));
#187259=CARTESIAN_POINT('Ctrl Pts',(24.8516310625176,-7.38540558903621,
0.));
#187260=CARTESIAN_POINT('Ctrl Pts',(24.8240228520893,-7.39174922585809,
0.));
#187261=CARTESIAN_POINT('Ctrl Pts',(24.7964676646431,-7.39801641583013,
0.));
#187262=CARTESIAN_POINT('Ctrl Pts',(24.7689656668983,-7.40420718661603,
0.));
#187263=CARTESIAN_POINT('Ctrl Pts',(24.7415170994784,-7.41032159082382,
0.));
#187264=CARTESIAN_POINT('Ctrl Pts',(24.7141222950051,-7.41635971481674,
0.));
#187265=CARTESIAN_POINT('Ctrl Pts',(24.6867816727192,-7.42232167766266,
0.));
#187266=CARTESIAN_POINT('Ctrl Pts',(24.6594957128756,-7.42820762159126,
0.));
#187267=CARTESIAN_POINT('Ctrl Pts',(24.6322649369517,-7.43401770489524,
0.));
#187268=CARTESIAN_POINT('Ctrl Pts',(24.6050898852368,-7.43975209375504,
0.));
#187269=CARTESIAN_POINT('Ctrl Pts',(24.577971096086,-7.44541095473135,0.));
#187270=CARTESIAN_POINT('Ctrl Pts',(24.5509090831559,-7.4509944465116,0.));
#187271=CARTESIAN_POINT('Ctrl Pts',(24.5239043173072,-7.45650271335862,
0.));
#187272=CARTESIAN_POINT('Ctrl Pts',(24.4969572391483,-7.46193588961464,
0.));
#187273=CARTESIAN_POINT('Ctrl Pts',(24.4700682684524,-7.46729410308787,
0.));
#187274=CARTESIAN_POINT('Ctrl Pts',(24.443237814649,-7.47257747883246,0.));
#187275=CARTESIAN_POINT('Ctrl Pts',(24.4164662871163,-7.47778614286565,
0.));
#187276=CARTESIAN_POINT('Ctrl Pts',(24.3897541049254,-7.48292022569301,
0.));
#187277=CARTESIAN_POINT('Ctrl Pts',(24.3631017084524,-7.48797986651909,
0.));
#187278=CARTESIAN_POINT('Ctrl Pts',(24.3365095573685,-7.49296521252421,
0.));
#187279=CARTESIAN_POINT('Ctrl Pts',(24.3099781253355,-7.49787641695439,
0.));
#187280=CARTESIAN_POINT('Ctrl Pts',(24.2835078958973,-7.50271363765152,
0.));
#187281=CARTESIAN_POINT('Ctrl Pts',(24.2570993577034,-7.50747703535134,
0.));
#187282=CARTESIAN_POINT('Ctrl Pts',(24.2307530003887,-7.51216677222181,
0.));
#187283=CARTESIAN_POINT('Ctrl Pts',(24.2044693092349,-7.51678300997949,
0.));
#187284=CARTESIAN_POINT('Ctrl Pts',(24.1782487641594,-7.52132590953802,
0.));
#187285=CARTESIAN_POINT('Ctrl Pts',(24.1520918425364,-7.52579563201424,
0.));
#187286=CARTESIAN_POINT('Ctrl Pts',(24.1259990209207,-7.53019233935502,
0.));
#187287=CARTESIAN_POINT('Ctrl Pts',(24.0999707772642,-7.53451619514649,
0.));
#187288=CARTESIAN_POINT('Ctrl Pts',(24.0740075927985,-7.53876736531014,
0.));
#187289=CARTESIAN_POINT('Ctrl Pts',(24.0481099543353,-7.54294601896145,
0.));
#187290=CARTESIAN_POINT('Ctrl Pts',(24.022278355453,-7.5470523288591,0.));
#187291=CARTESIAN_POINT('Ctrl Pts',(23.9965132953185,-7.55108647097441,
0.));
#187292=CARTESIAN_POINT('Ctrl Pts',(23.9708152779884,-7.55504862424812,
0.));
#187293=CARTESIAN_POINT('Ctrl Pts',(23.9451848115,-7.55893897027683,0.));
#187294=CARTESIAN_POINT('Ctrl Pts',(23.9196224070759,-7.56275769304773,
0.));
#187295=CARTESIAN_POINT('Ctrl Pts',(23.8941285782003,-7.56650497863792,
0.));
#187296=CARTESIAN_POINT('Ctrl Pts',(23.8687038399597,-7.57018101500711,
0.));
#187297=CARTESIAN_POINT('Ctrl Pts',(23.8433487096134,-7.57378599219817,
0.));
#187298=CARTESIAN_POINT('Ctrl Pts',(23.8180637069977,-7.57732010249066,
0.));
#187299=CARTESIAN_POINT('Ctrl Pts',(23.7928493549908,-7.58078354058212,
0.));
#187300=CARTESIAN_POINT('Ctrl Pts',(23.7677061799376,-7.58417650376272,
0.));
#187301=CARTESIAN_POINT('Ctrl Pts',(23.7426347121006,-7.58749919210832,
0.));
#187302=CARTESIAN_POINT('Ctrl Pts',(23.7176354860457,-7.59075180865327,
0.));
#187303=CARTESIAN_POINT('Ctrl Pts',(23.6927090405067,-7.59393455934042,
0.));
#187304=CARTESIAN_POINT('Ctrl Pts',(23.6678559182876,-7.59704765299572,
0.));
#187305=CARTESIAN_POINT('Ctrl Pts',(23.6430766661419,-7.6000913013013,0.));
#187306=CARTESIAN_POINT('Ctrl Pts',(23.6183718346576,-7.60306571877806,
0.));
#187307=CARTESIAN_POINT('Ctrl Pts',(23.5937419781244,-7.60597112277094,
0.));
#187308=CARTESIAN_POINT('Ctrl Pts',(23.5691876544243,-7.608807733446,0.));
#187309=CARTESIAN_POINT('Ctrl Pts',(23.5447094252028,-7.61157577385372,
0.));
#187310=CARTESIAN_POINT('Ctrl Pts',(23.5203078560128,-7.61427546999299,
0.));
#187311=CARTESIAN_POINT('Ctrl Pts',(23.4959835164608,-7.61690705088319,
0.));
#187312=CARTESIAN_POINT('Ctrl Pts',(23.4717369803438,-7.61947074863978,
0.));
#187313=CARTESIAN_POINT('Ctrl Pts',(23.4475688257854,-7.62196679855957,
0.));
#187314=CARTESIAN_POINT('Ctrl Pts',(23.4234796353544,-7.62439543920055,
0.));
#187315=CARTESIAN_POINT('Ctrl Pts',(23.3994699961122,-7.62675691240335,
0.));
#187316=CARTESIAN_POINT('Ctrl Pts',(23.3755404996638,-7.62905146332598,
0.));
#187317=CARTESIAN_POINT('Ctrl Pts',(23.3516917421973,-7.63127934048139,
0.));
#187318=CARTESIAN_POINT('Ctrl Pts',(23.3279243245241,-7.63344079578163,
0.));
#187319=CARTESIAN_POINT('Ctrl Pts',(23.3042388521021,-7.63553608458784,
0.));
#187320=CARTESIAN_POINT('Ctrl Pts',(23.2806359350853,-7.63756546576375,
0.));
#187321=CARTESIAN_POINT('Ctrl Pts',(23.2571161884487,-7.63952920172837,
0.));
#187322=CARTESIAN_POINT('Ctrl Pts',(23.2336802320912,-7.64142755851508,
0.));
#187323=CARTESIAN_POINT('Ctrl Pts',(23.2103286909399,-7.64326080583684,
0.));
#187324=CARTESIAN_POINT('Ctrl Pts',(23.1870621950452,-7.64502921715483,
0.));
#187325=CARTESIAN_POINT('Ctrl Pts',(23.1638813796691,-7.64673306975797,
0.));
#187326=CARTESIAN_POINT('Ctrl Pts',(23.1407868853815,-7.64837264482929,
0.));
#187327=CARTESIAN_POINT('Ctrl Pts',(23.1177793581674,-7.64994822749845,
0.));
#187328=CARTESIAN_POINT('Ctrl Pts',(23.0948594495246,-7.65146010690465,
0.));
#187329=CARTESIAN_POINT('Ctrl Pts',(23.072027816555,-7.65290857626357,0.));
#187330=CARTESIAN_POINT('Ctrl Pts',(23.049285122053,-7.65429393293955,0.));
#187331=CARTESIAN_POINT('Ctrl Pts',(23.0266320345792,-7.65561647852555,
0.));
#187332=CARTESIAN_POINT('Ctrl Pts',(23.004069228582,-7.6568765189133,0.));
#187333=CARTESIAN_POINT('Ctrl Pts',(22.9815973845301,-7.65807436436453,
0.));
#187334=CARTESIAN_POINT('Ctrl Pts',(22.9592171890332,-7.65921032958912,
0.));
#187335=CARTESIAN_POINT('Ctrl Pts',(22.9369293349592,-7.66028473382777,
0.));
#187336=CARTESIAN_POINT('Ctrl Pts',(22.9147345215418,-7.661297900941,0.));
#187337=CARTESIAN_POINT('Ctrl Pts',(22.8926334544879,-7.66225015950148,
0.));
#187338=CARTESIAN_POINT('Ctrl Pts',(22.870626846128,-7.66314184287334,0.));
#187339=CARTESIAN_POINT('Ctrl Pts',(22.8487154155569,-7.66397328929805,
0.));
#187340=CARTESIAN_POINT('Ctrl Pts',(22.8268998887678,-7.66474484198553,
0.));
#187341=CARTESIAN_POINT('Ctrl Pts',(22.8051809987833,-7.66545684920988,
0.));
#187342=CARTESIAN_POINT('Ctrl Pts',(22.7835594857697,-7.66610966441259,
0.));
#187343=CARTESIAN_POINT('Ctrl Pts',(22.7620360971839,-7.66670364630273,
0.));
#187344=CARTESIAN_POINT('Ctrl Pts',(22.7406115879508,-7.66723915895413,
0.));
#187345=CARTESIAN_POINT('Ctrl Pts',(22.7192867206242,-7.6677165719101,0.));
#187346=CARTESIAN_POINT('Ctrl Pts',(22.6980622655446,-7.66813626029277,
0.));
#187347=CARTESIAN_POINT('Ctrl Pts',(22.6769390009889,-7.66849860491763,
0.));
#187348=CARTESIAN_POINT('Ctrl Pts',(22.6559177133133,-7.66880399241354,
0.));
#187349=CARTESIAN_POINT('Ctrl Pts',(22.6349991971547,-7.66905281533745,
0.));
#187350=CARTESIAN_POINT('Ctrl Pts',(22.6141842556248,-7.66924547229435,
0.));
#187351=CARTESIAN_POINT('Ctrl Pts',(22.5934737004955,-7.66938236806241,
0.));
#187352=CARTESIAN_POINT('Ctrl Pts',(22.5728683523828,-7.66946391372299,
0.));
#187353=CARTESIAN_POINT('Ctrl Pts',(22.5523690409109,-7.66949052679672,
0.));
#187354=CARTESIAN_POINT('Ctrl Pts',(22.5319766049191,-7.66946263138116,
0.));
#187355=CARTESIAN_POINT('Ctrl Pts',(22.5116918927023,-7.66938065829083,
0.));
#187356=CARTESIAN_POINT('Ctrl Pts',(22.4915157622308,-7.66924504520302,
0.));
#187357=CARTESIAN_POINT('Ctrl Pts',(22.47144908137,-7.66905623680836,0.));
#187358=CARTESIAN_POINT('Ctrl Pts',(22.4514927280862,-7.6688146849666,0.));
#187359=CARTESIAN_POINT('Ctrl Pts',(22.4316475906616,-7.66852084886746,
0.));
#187360=CARTESIAN_POINT('Ctrl Pts',(22.411914567977,-7.66817519519682,0.));
#187361=CARTESIAN_POINT('Ctrl Pts',(22.3922945697782,-7.6677781983082,0.));
#187362=CARTESIAN_POINT('Ctrl Pts',(22.3727885169361,-7.66733034039887,
0.));
#187363=CARTESIAN_POINT('Ctrl Pts',(22.3533973417013,-7.66683211169134,
0.));
#187364=CARTESIAN_POINT('Ctrl Pts',(22.3341219879454,-7.66628401061906,
0.));
#187365=CARTESIAN_POINT('Ctrl Pts',(22.3149634114823,-7.66568654402442,
0.));
#187366=CARTESIAN_POINT('Ctrl Pts',(22.2959225803925,-7.66504022736263,
0.));
#187367=CARTESIAN_POINT('Ctrl Pts',(22.2770004753332,-7.66434558490973,
0.));
#187368=CARTESIAN_POINT('Ctrl Pts',(22.2581980898487,-7.66360314997662,
0.));
#187369=CARTESIAN_POINT('Ctrl Pts',(22.239516430656,-7.66281346512546,0.));
#187370=CARTESIAN_POINT('Ctrl Pts',(22.2209565180098,-7.66197708240436,
0.));
#187371=CARTESIAN_POINT('Ctrl Pts',(22.2025193860972,-7.66109456359292,
0.));
#187372=CARTESIAN_POINT('Ctrl Pts',(22.1842060834092,-7.66016648045008,
0.));
#187373=CARTESIAN_POINT('Ctrl Pts',(22.1660176731174,-7.65919341496926,
0.));
#187374=CARTESIAN_POINT('Ctrl Pts',(22.1479552334206,-7.65817595963351,
0.));
#187375=CARTESIAN_POINT('Ctrl Pts',(22.1300198579671,-7.65711471769407,
0.));
#187376=CARTESIAN_POINT('Ctrl Pts',(22.1122126563327,-7.65601030346819,
0.));
#187377=CARTESIAN_POINT('Ctrl Pts',(22.094534754469,-7.65486334263651,0.));
#187378=CARTESIAN_POINT('Ctrl Pts',(22.0769872951596,-7.65367447254945,
0.));
#187379=CARTESIAN_POINT('Ctrl Pts',(22.0595714384432,-7.65244434253104,
0.));
#187380=CARTESIAN_POINT('Ctrl Pts',(22.0422883621176,-7.65117361421347,
0.));
#187381=CARTESIAN_POINT('Ctrl Pts',(22.0251392623209,-7.64986296190157,
0.));
#187382=CARTESIAN_POINT('Ctrl Pts',(22.0081253540773,-7.64851307293346,
0.));
#187383=CARTESIAN_POINT('Ctrl Pts',(21.9912478718542,-7.64712464805258,
0.));
#187384=CARTESIAN_POINT('Ctrl Pts',(21.97450807008,-7.64569840177359,0.));
#187385=CARTESIAN_POINT('Ctrl Pts',(21.9579072237653,-7.64423506279154,
0.));
#187386=CARTESIAN_POINT('Ctrl Pts',(21.9414466292074,-7.64273537442707,
0.));
#187387=CARTESIAN_POINT('Ctrl Pts',(21.9251276046546,-7.6412000950654,0.));
#187388=CARTESIAN_POINT('Ctrl Pts',(21.9089514909873,-7.63962999860917,
0.));
#187389=CARTESIAN_POINT('Ctrl Pts',(21.8929196523511,-7.63802587492008,
0.));
#187390=CARTESIAN_POINT('Ctrl Pts',(21.8770334769492,-7.63638853033368,
0.));
#187391=CARTESIAN_POINT('Ctrl Pts',(21.8612943779086,-7.63471878821204,
0.));
#187392=CARTESIAN_POINT('Ctrl Pts',(21.8457037941084,-7.63301748948936,
0.));
#187393=CARTESIAN_POINT('Ctrl Pts',(21.8302631910197,-7.6312854932304,0.));
#187394=CARTESIAN_POINT('Ctrl Pts',(21.8149740615093,-7.62952367718151,
0.));
#187395=CARTESIAN_POINT('Ctrl Pts',(21.7998379268583,-7.62773293842409,
0.));
#187396=CARTESIAN_POINT('Ctrl Pts',(21.7848563378022,-7.62591419404521,
0.));
#187397=CARTESIAN_POINT('Ctrl Pts',(21.7700308755583,-7.62406838181164,
0.));
#187398=CARTESIAN_POINT('Ctrl Pts',(21.7553631528329,-7.62219646084226,
0.));
#187399=CARTESIAN_POINT('Ctrl Pts',(21.7408548148657,-7.62029941230855,
0.));
#187400=CARTESIAN_POINT('Ctrl Pts',(21.7265075407977,-7.61837824030542,
0.));
#187401=CARTESIAN_POINT('Ctrl Pts',(21.7123230449835,-7.61643397270425,
0.));
#187402=CARTESIAN_POINT('Ctrl Pts',(21.6983030783321,-7.61446766202787,
0.));
#187403=CARTESIAN_POINT('Ctrl Pts',(21.6844494295813,-7.61248038630265,
0.));
#187404=CARTESIAN_POINT('Ctrl Pts',(21.6707639267573,-7.6104732500095,0.));
#187405=CARTESIAN_POINT('Ctrl Pts',(21.6572484388079,-7.60844738512872,
0.));
#187406=CARTESIAN_POINT('Ctrl Pts',(21.6439048771743,-7.60640395216359,
0.));
#187407=CARTESIAN_POINT('Ctrl Pts',(21.6307351973823,-7.604344141183,0.));
#187408=CARTESIAN_POINT('Ctrl Pts',(21.6177414005991,-7.60226917285432,
0.));
#187409=CARTESIAN_POINT('Ctrl Pts',(21.6049255358842,-7.60018029988238,
0.));
#187410=CARTESIAN_POINT('Ctrl Pts',(21.5922897024466,-7.59807880846193,
0.));
#187411=CARTESIAN_POINT('Ctrl Pts',(21.5798360518978,-7.59596601973589,
0.));
#187412=CARTESIAN_POINT('Ctrl Pts',(21.5675667904728,-7.5938432912493,0.));
#187413=CARTESIAN_POINT('Ctrl Pts',(21.5554841813465,-7.59171201844793,
0.));
#187414=CARTESIAN_POINT('Ctrl Pts',(21.5435905470113,-7.58957363620026,
0.));
#187415=CARTESIAN_POINT('Ctrl Pts',(21.5318882716735,-7.58742962034834,
0.));
#187416=CARTESIAN_POINT('Ctrl Pts',(21.5203798035294,-7.58528148919114,
0.));
#187417=CARTESIAN_POINT('Ctrl Pts',(21.5090676573866,-7.58313080519159,
0.));
#187418=CARTESIAN_POINT('Ctrl Pts',(21.4979544192739,-7.5809791779073,0.));
#187419=CARTESIAN_POINT('Ctrl Pts',(21.4870427508193,-7.57882826679131,
0.));
#187420=CARTESIAN_POINT('Ctrl Pts',(21.4763353936766,-7.57667978403003,
0.));
#187421=CARTESIAN_POINT('Ctrl Pts',(21.4658351740135,-7.57453549743435,
0.));
#187422=CARTESIAN_POINT('Ctrl Pts',(21.4555450053147,-7.57239723223521,
0.));
#187423=CARTESIAN_POINT('Ctrl Pts',(21.445467890751,-7.5702668726117,0.));
#187424=CARTESIAN_POINT('Ctrl Pts',(21.435606926151,-7.56814636360842,0.));
#187425=CARTESIAN_POINT('Ctrl Pts',(21.4259653015732,-7.56603771218706,
0.));
#187426=CARTESIAN_POINT('Ctrl Pts',(21.4165463106252,-7.56394299313683,
0.));
#187427=CARTESIAN_POINT('Ctrl Pts',(21.4073533630364,-7.56186435703622,
0.));
#187428=CARTESIAN_POINT('Ctrl Pts',(21.3983899952988,-7.55980403700615,
0.));
#187429=CARTESIAN_POINT('Ctrl Pts',(21.3896598842119,-7.55776435731422,
0.));
#187430=CARTESIAN_POINT('Ctrl Pts',(21.3811668478933,-7.55574773403508,
0.));
#187431=CARTESIAN_POINT('Ctrl Pts',(21.3729148390244,-7.55375667080032,
0.));
#187432=CARTESIAN_POINT('Ctrl Pts',(21.3649079431864,-7.55179375777442,
0.));
#187433=CARTESIAN_POINT('Ctrl Pts',(21.3571503685853,-7.54986166521307,
0.));
#187434=CARTESIAN_POINT('Ctrl Pts',(21.349646476153,-7.54796316246327,0.));
#187435=CARTESIAN_POINT('Ctrl Pts',(21.3424008295038,-7.54610114948351,
0.));
#187436=CARTESIAN_POINT('Ctrl Pts',(21.3354182340149,-7.54427868151269,
0.));
#187437=CARTESIAN_POINT('Ctrl Pts',(21.328703791771,-7.54249900377032,0.));
#187438=CARTESIAN_POINT('Ctrl Pts',(21.3222628524165,-7.5407655203828,0.));
#187439=CARTESIAN_POINT('Ctrl Pts',(21.3161009456256,-7.53908175169899,
0.));
#187440=CARTESIAN_POINT('Ctrl Pts',(21.3102237167729,-7.5374512936462,0.));
#187441=CARTESIAN_POINT('Ctrl Pts',(21.3046368712156,-7.53587778251743,
0.));
#187442=CARTESIAN_POINT('Ctrl Pts',(21.2993464250717,-7.53436505309949,
0.));
#187443=CARTESIAN_POINT('Ctrl Pts',(21.2943588989331,-7.53291726078527,
0.));
#187444=CARTESIAN_POINT('Ctrl Pts',(21.2896816163843,-7.53153906987847,
0.));
#187445=CARTESIAN_POINT('Ctrl Pts',(21.2853226580658,-7.53023562438221,
0.));
#187446=CARTESIAN_POINT('Ctrl Pts',(21.2812902781143,-7.52901217930407,
0.));
#187447=CARTESIAN_POINT('Ctrl Pts',(21.2775925269651,-7.52787386225344,
0.));
#187448=CARTESIAN_POINT('Ctrl Pts',(21.2742366113578,-7.52682526918561,
0.));
#187449=CARTESIAN_POINT('Ctrl Pts',(21.2712301573465,-7.52587126095544,
0.));
#187450=CARTESIAN_POINT('Ctrl Pts',(21.2685823838672,-7.52501770333522,
0.));
#187451=CARTESIAN_POINT('Ctrl Pts',(21.266305915706,-7.52427261074264,0.));
#187452=CARTESIAN_POINT('Ctrl Pts',(21.2644161259965,-7.52364573027521,
0.));
#187453=CARTESIAN_POINT('Ctrl Pts',(21.262927782038,-7.52314642316203,0.));
#187454=CARTESIAN_POINT('Ctrl Pts',(21.261852128355,-7.52278182242728,0.));
#187455=CARTESIAN_POINT('Ctrl Pts',(21.2613260540651,-7.52260064231736,
0.));
#187456=CARTESIAN_POINT('Ctrl Pts',(21.261120447486,-7.52252744144958,0.));
#187457=CARTESIAN_POINT('Ctrl Pts',(21.2610673466883,-7.52250649703992,
0.));
#187458=CARTESIAN_POINT('Ctrl Pts',(21.2610617890679,-7.52250298901266,
0.));
#187459=CARTESIAN_POINT('',(24.9347862158358,-7.36589684767345,0.));
#187460=CARTESIAN_POINT('Ctrl Pts',(20.353053841303,-9.71462809124917,0.));
#187461=CARTESIAN_POINT('Ctrl Pts',(20.353053841303,-9.71462809124917,12.));
#187462=CARTESIAN_POINT('Ctrl Pts',(20.353060251684,-9.71462954053074,0.));
#187463=CARTESIAN_POINT('Ctrl Pts',(20.353060251684,-9.71462954053074,12.));
#187464=CARTESIAN_POINT('Ctrl Pts',(20.3531126095522,-9.71465227853122,
0.));
#187465=CARTESIAN_POINT('Ctrl Pts',(20.3531126095522,-9.71465227853122,
12.));
#187466=CARTESIAN_POINT('Ctrl Pts',(20.3533097561886,-9.71474590350792,
0.));
#187467=CARTESIAN_POINT('Ctrl Pts',(20.3533097561886,-9.71474590350792,
12.));
#187468=CARTESIAN_POINT('Ctrl Pts',(20.3538098605706,-9.71498978052101,
0.));
#187469=CARTESIAN_POINT('Ctrl Pts',(20.3538098605706,-9.71498978052101,
12.));
#187470=CARTESIAN_POINT('Ctrl Pts',(20.3548282742361,-9.71549257088175,
0.));
#187471=CARTESIAN_POINT('Ctrl Pts',(20.3548282742361,-9.71549257088175,
12.));
#187472=CARTESIAN_POINT('Ctrl Pts',(20.3562337557875,-9.71619192554147,
0.));
#187473=CARTESIAN_POINT('Ctrl Pts',(20.3562337557875,-9.71619192554147,
12.));
#187474=CARTESIAN_POINT('Ctrl Pts',(20.3580133103357,-9.71708493723062,
0.));
#187475=CARTESIAN_POINT('Ctrl Pts',(20.3580133103357,-9.71708493723062,
12.));
#187476=CARTESIAN_POINT('Ctrl Pts',(20.3601498764344,-9.71816778327999,
0.));
#187477=CARTESIAN_POINT('Ctrl Pts',(20.3601498764344,-9.71816778327999,
12.));
#187478=CARTESIAN_POINT('Ctrl Pts',(20.362625691398,-9.71943648548115,0.));
#187479=CARTESIAN_POINT('Ctrl Pts',(20.362625691398,-9.71943648548115,12.));
#187480=CARTESIAN_POINT('Ctrl Pts',(20.3654261611055,-9.72088778381102,
0.));
#187481=CARTESIAN_POINT('Ctrl Pts',(20.3654261611055,-9.72088778381102,
12.));
#187482=CARTESIAN_POINT('Ctrl Pts',(20.3685406190576,-9.72251930722504,
0.));
#187483=CARTESIAN_POINT('Ctrl Pts',(20.3685406190576,-9.72251930722504,
12.));
#187484=CARTESIAN_POINT('Ctrl Pts',(20.371960235676,-9.72432910043193,0.));
#187485=CARTESIAN_POINT('Ctrl Pts',(20.371960235676,-9.72432910043193,12.));
#187486=CARTESIAN_POINT('Ctrl Pts',(20.3756766651952,-9.72631531732871,
0.));
#187487=CARTESIAN_POINT('Ctrl Pts',(20.3756766651952,-9.72631531732871,
12.));
#187488=CARTESIAN_POINT('Ctrl Pts',(20.3796805893304,-9.72847589116533,
0.));
#187489=CARTESIAN_POINT('Ctrl Pts',(20.3796805893304,-9.72847589116533,
12.));
#187490=CARTESIAN_POINT('Ctrl Pts',(20.3839624556742,-9.73080870123726,
0.));
#187491=CARTESIAN_POINT('Ctrl Pts',(20.3839624556742,-9.73080870123726,
12.));
#187492=CARTESIAN_POINT('Ctrl Pts',(20.3885129129912,-9.73331167102812,
0.));
#187493=CARTESIAN_POINT('Ctrl Pts',(20.3885129129912,-9.73331167102812,
12.));
#187494=CARTESIAN_POINT('Ctrl Pts',(20.3933234845646,-9.7359829201425,0.));
#187495=CARTESIAN_POINT('Ctrl Pts',(20.3933234845646,-9.7359829201425,12.));
#187496=CARTESIAN_POINT('Ctrl Pts',(20.3983866213331,-9.73882077613206,
0.));
#187497=CARTESIAN_POINT('Ctrl Pts',(20.3983866213331,-9.73882077613206,
12.));
#187498=CARTESIAN_POINT('Ctrl Pts',(20.4036953576549,-9.74182369656273,
0.));
#187499=CARTESIAN_POINT('Ctrl Pts',(20.4036953576549,-9.74182369656273,
12.));
#187500=CARTESIAN_POINT('Ctrl Pts',(20.4092430879861,-9.74499021838537,
0.));
#187501=CARTESIAN_POINT('Ctrl Pts',(20.4092430879861,-9.74499021838537,
12.));
#187502=CARTESIAN_POINT('Ctrl Pts',(20.4150232777393,-9.74831889242175,
0.));
#187503=CARTESIAN_POINT('Ctrl Pts',(20.4150232777393,-9.74831889242175,
12.));
#187504=CARTESIAN_POINT('Ctrl Pts',(20.4210295275818,-9.75180829786433,
0.));
#187505=CARTESIAN_POINT('Ctrl Pts',(20.4210295275818,-9.75180829786433,
12.));
#187506=CARTESIAN_POINT('Ctrl Pts',(20.4272556476629,-9.75545705902416,
0.));
#187507=CARTESIAN_POINT('Ctrl Pts',(20.4272556476629,-9.75545705902416,
12.));
#187508=CARTESIAN_POINT('Ctrl Pts',(20.4336957355474,-9.7592638628993,0.));
#187509=CARTESIAN_POINT('Ctrl Pts',(20.4336957355474,-9.7592638628993,12.));
#187510=CARTESIAN_POINT('Ctrl Pts',(20.4403442329401,-9.76322747195502,
0.));
#187511=CARTESIAN_POINT('Ctrl Pts',(20.4403442329401,-9.76322747195502,
12.));
#187512=CARTESIAN_POINT('Ctrl Pts',(20.447195862298,-9.76734670980897,0.));
#187513=CARTESIAN_POINT('Ctrl Pts',(20.447195862298,-9.76734670980897,12.));
#187514=CARTESIAN_POINT('Ctrl Pts',(20.4542455817527,-9.7716204510407,0.));
#187515=CARTESIAN_POINT('Ctrl Pts',(20.4542455817527,-9.7716204510407,12.));
#187516=CARTESIAN_POINT('Ctrl Pts',(20.4614885274973,-9.77604760815523,
0.));
#187517=CARTESIAN_POINT('Ctrl Pts',(20.4614885274973,-9.77604760815523,
12.));
#187518=CARTESIAN_POINT('Ctrl Pts',(20.4689199790668,-9.78062712373313,
0.));
#187519=CARTESIAN_POINT('Ctrl Pts',(20.4689199790668,-9.78062712373313,
12.));
#187520=CARTESIAN_POINT('Ctrl Pts',(20.4765353711585,-9.78535797314162,
0.));
#187521=CARTESIAN_POINT('Ctrl Pts',(20.4765353711585,-9.78535797314162,
12.));
#187522=CARTESIAN_POINT('Ctrl Pts',(20.4843302955329,-9.7902391649866,0.));
#187523=CARTESIAN_POINT('Ctrl Pts',(20.4843302955329,-9.7902391649866,12.));
#187524=CARTESIAN_POINT('Ctrl Pts',(20.4923005087945,-9.79526974288344,
0.));
#187525=CARTESIAN_POINT('Ctrl Pts',(20.4923005087945,-9.79526974288344,
12.));
#187526=CARTESIAN_POINT('Ctrl Pts',(20.500441931211,-9.80044878520968,0.));
#187527=CARTESIAN_POINT('Ctrl Pts',(20.500441931211,-9.80044878520968,12.));
#187528=CARTESIAN_POINT('Ctrl Pts',(20.5087506310507,-9.80577540161103,
0.));
#187529=CARTESIAN_POINT('Ctrl Pts',(20.5087506310507,-9.80577540161103,
12.));
#187530=CARTESIAN_POINT('Ctrl Pts',(20.5172228122839,-9.81124873025278,
0.));
#187531=CARTESIAN_POINT('Ctrl Pts',(20.5172228122839,-9.81124873025278,
12.));
#187532=CARTESIAN_POINT('Ctrl Pts',(20.5258548000625,-9.81686793455918,
0.));
#187533=CARTESIAN_POINT('Ctrl Pts',(20.5258548000625,-9.81686793455918,
12.));
#187534=CARTESIAN_POINT('Ctrl Pts',(20.534643029951,-9.82263220080328,0.));
#187535=CARTESIAN_POINT('Ctrl Pts',(20.534643029951,-9.82263220080328,12.));
#187536=CARTESIAN_POINT('Ctrl Pts',(20.5435840460717,-9.82854073773858,
0.));
#187537=CARTESIAN_POINT('Ctrl Pts',(20.5435840460717,-9.82854073773858,
12.));
#187538=CARTESIAN_POINT('Ctrl Pts',(20.5526744976461,-9.83459277585321,
0.));
#187539=CARTESIAN_POINT('Ctrl Pts',(20.5526744976461,-9.83459277585321,
12.));
#187540=CARTESIAN_POINT('Ctrl Pts',(20.5619111362406,-9.84078756677589,
0.));
#187541=CARTESIAN_POINT('Ctrl Pts',(20.5619111362406,-9.84078756677589,
12.));
#187542=CARTESIAN_POINT('Ctrl Pts',(20.5712908125145,-9.84712438256308,
0.));
#187543=CARTESIAN_POINT('Ctrl Pts',(20.5712908125145,-9.84712438256308,
12.));
#187544=CARTESIAN_POINT('Ctrl Pts',(20.580810471002,-9.85360251457004,0.));
#187545=CARTESIAN_POINT('Ctrl Pts',(20.580810471002,-9.85360251457004,12.));
#187546=CARTESIAN_POINT('Ctrl Pts',(20.5904671449754,-9.8602212723275,0.));
#187547=CARTESIAN_POINT('Ctrl Pts',(20.5904671449754,-9.8602212723275,12.));
#187548=CARTESIAN_POINT('Ctrl Pts',(20.6002579513696,-9.86697998242612,
0.));
#187549=CARTESIAN_POINT('Ctrl Pts',(20.6002579513696,-9.86697998242612,
12.));
#187550=CARTESIAN_POINT('Ctrl Pts',(20.6101800854491,-9.87387798732944,
0.));
#187551=CARTESIAN_POINT('Ctrl Pts',(20.6101800854491,-9.87387798732944,
12.));
#187552=CARTESIAN_POINT('Ctrl Pts',(20.6202308177472,-9.88091464472669,
0.));
#187553=CARTESIAN_POINT('Ctrl Pts',(20.6202308177472,-9.88091464472669,
12.));
#187554=CARTESIAN_POINT('Ctrl Pts',(20.6304074914086,-9.88808932697305,
0.));
#187555=CARTESIAN_POINT('Ctrl Pts',(20.6304074914086,-9.88808932697305,
12.));
#187556=CARTESIAN_POINT('Ctrl Pts',(20.6407075193977,-9.89540142049124,
0.));
#187557=CARTESIAN_POINT('Ctrl Pts',(20.6407075193977,-9.89540142049124,
12.));
#187558=CARTESIAN_POINT('Ctrl Pts',(20.6511283817415,-9.90285032516696,
0.));
#187559=CARTESIAN_POINT('Ctrl Pts',(20.6511283817415,-9.90285032516696,
12.));
#187560=CARTESIAN_POINT('Ctrl Pts',(20.6616676228315,-9.91043545377005,
0.));
#187561=CARTESIAN_POINT('Ctrl Pts',(20.6616676228315,-9.91043545377005,
12.));
#187562=CARTESIAN_POINT('Ctrl Pts',(20.6723228488261,-9.91815623141285,
0.));
#187563=CARTESIAN_POINT('Ctrl Pts',(20.6723228488261,-9.91815623141285,
12.));
#187564=CARTESIAN_POINT('Ctrl Pts',(20.6830917250255,-9.92601209498751,
0.));
#187565=CARTESIAN_POINT('Ctrl Pts',(20.6830917250255,-9.92601209498751,
12.));
#187566=CARTESIAN_POINT('Ctrl Pts',(20.6939719732485,-9.93400249259737,
0.));
#187567=CARTESIAN_POINT('Ctrl Pts',(20.6939719732485,-9.93400249259737,
12.));
#187568=CARTESIAN_POINT('Ctrl Pts',(20.7049613692237,-9.94212688298251,
0.));
#187569=CARTESIAN_POINT('Ctrl Pts',(20.7049613692237,-9.94212688298251,
12.));
#187570=CARTESIAN_POINT('Ctrl Pts',(20.716057740758,-9.95038473514962,0.));
#187571=CARTESIAN_POINT('Ctrl Pts',(20.716057740758,-9.95038473514962,12.));
#187572=CARTESIAN_POINT('Ctrl Pts',(20.7272589658752,-9.95877552798403,
0.));
#187573=CARTESIAN_POINT('Ctrl Pts',(20.7272589658752,-9.95877552798403,
12.));
#187574=CARTESIAN_POINT('Ctrl Pts',(20.7385629709795,-9.96729874986199,
0.));
#187575=CARTESIAN_POINT('Ctrl Pts',(20.7385629709795,-9.96729874986199,
12.));
#187576=CARTESIAN_POINT('Ctrl Pts',(20.7499677289625,-9.97595389823461,
0.));
#187577=CARTESIAN_POINT('Ctrl Pts',(20.7499677289625,-9.97595389823461,
12.));
#187578=CARTESIAN_POINT('Ctrl Pts',(20.7614712574989,-9.98474047926846,
0.));
#187579=CARTESIAN_POINT('Ctrl Pts',(20.7614712574989,-9.98474047926846,
12.));
#187580=CARTESIAN_POINT('Ctrl Pts',(20.7730716175417,-9.99365800754638,
0.));
#187581=CARTESIAN_POINT('Ctrl Pts',(20.7730716175417,-9.99365800754638,
12.));
#187582=CARTESIAN_POINT('Ctrl Pts',(20.7847669117568,-10.0027060057389,
0.));
#187583=CARTESIAN_POINT('Ctrl Pts',(20.7847669117568,-10.0027060057389,
12.));
#187584=CARTESIAN_POINT('Ctrl Pts',(20.7965552829907,-10.0118840042786,
0.));
#187585=CARTESIAN_POINT('Ctrl Pts',(20.7965552829907,-10.0118840042786,
12.));
#187586=CARTESIAN_POINT('Ctrl Pts',(20.8084349126885,-10.0211915410095,
0.));
#187587=CARTESIAN_POINT('Ctrl Pts',(20.8084349126885,-10.0211915410095,
12.));
#187588=CARTESIAN_POINT('Ctrl Pts',(20.8204040196599,-10.0306281609435,
0.));
#187589=CARTESIAN_POINT('Ctrl Pts',(20.8204040196599,-10.0306281609435,
12.));
#187590=CARTESIAN_POINT('Ctrl Pts',(20.8324608588906,-10.0401934160234,
0.));
#187591=CARTESIAN_POINT('Ctrl Pts',(20.8324608588906,-10.0401934160234,
12.));
#187592=CARTESIAN_POINT('Ctrl Pts',(20.8446037203402,-10.0498868648733,
0.));
#187593=CARTESIAN_POINT('Ctrl Pts',(20.8446037203402,-10.0498868648733,
12.));
#187594=CARTESIAN_POINT('Ctrl Pts',(20.856830927732,-10.0597080725375,0.));
#187595=CARTESIAN_POINT('Ctrl Pts',(20.856830927732,-10.0597080725375,12.));
#187596=CARTESIAN_POINT('Ctrl Pts',(20.8691408373705,-10.0696566102219,
0.));
#187597=CARTESIAN_POINT('Ctrl Pts',(20.8691408373705,-10.0696566102219,
12.));
#187598=CARTESIAN_POINT('Ctrl Pts',(20.8815318371844,-10.0797320551154,
0.));
#187599=CARTESIAN_POINT('Ctrl Pts',(20.8815318371844,-10.0797320551154,
12.));
#187600=CARTESIAN_POINT('Ctrl Pts',(20.8940023457371,-10.0899339901916,
0.));
#187601=CARTESIAN_POINT('Ctrl Pts',(20.8940023457371,-10.0899339901916,
12.));
#187602=CARTESIAN_POINT('Ctrl Pts',(20.9065508112556,-10.1002620040076,
0.));
#187603=CARTESIAN_POINT('Ctrl Pts',(20.9065508112556,-10.1002620040076,
12.));
#187604=CARTESIAN_POINT('Ctrl Pts',(20.9191757106266,-10.1107156904836,
0.));
#187605=CARTESIAN_POINT('Ctrl Pts',(20.9191757106266,-10.1107156904836,
12.));
#187606=CARTESIAN_POINT('Ctrl Pts',(20.931875548473,-10.1212946487057,0.));
#187607=CARTESIAN_POINT('Ctrl Pts',(20.931875548473,-10.1212946487057,12.));
#187608=CARTESIAN_POINT('Ctrl Pts',(20.944648856393,-10.1319984827909,0.));
#187609=CARTESIAN_POINT('Ctrl Pts',(20.944648856393,-10.1319984827909,12.));
#187610=CARTESIAN_POINT('Ctrl Pts',(20.9574941921591,-10.1428268017257,
0.));
#187611=CARTESIAN_POINT('Ctrl Pts',(20.9574941921591,-10.1428268017257,
12.));
#187612=CARTESIAN_POINT('Ctrl Pts',(20.970410138937,-10.1537792192065,0.));
#187613=CARTESIAN_POINT('Ctrl Pts',(20.970410138937,-10.1537792192065,12.));
#187614=CARTESIAN_POINT('Ctrl Pts',(20.9833953044736,-10.1648553534567,
0.));
#187615=CARTESIAN_POINT('Ctrl Pts',(20.9833953044736,-10.1648553534567,
12.));
#187616=CARTESIAN_POINT('Ctrl Pts',(20.9964483203685,-10.1760548270765,
0.));
#187617=CARTESIAN_POINT('Ctrl Pts',(20.9964483203685,-10.1760548270765,
12.));
#187618=CARTESIAN_POINT('Ctrl Pts',(21.0095678414486,-10.1873772669358,
0.));
#187619=CARTESIAN_POINT('Ctrl Pts',(21.0095678414486,-10.1873772669358,
12.));
#187620=CARTESIAN_POINT('Ctrl Pts',(21.0227525451107,-10.1988223040425,
0.));
#187621=CARTESIAN_POINT('Ctrl Pts',(21.0227525451107,-10.1988223040425,
12.));
#187622=CARTESIAN_POINT('Ctrl Pts',(21.0360011306814,-10.2103895734124,
0.));
#187623=CARTESIAN_POINT('Ctrl Pts',(21.0360011306814,-10.2103895734124,
12.));
#187624=CARTESIAN_POINT('Ctrl Pts',(21.0493123187483,-10.2220787139157,
0.));
#187625=CARTESIAN_POINT('Ctrl Pts',(21.0493123187483,-10.2220787139157,
12.));
#187626=CARTESIAN_POINT('Ctrl Pts',(21.0626848505665,-10.233889368157,0.));
#187627=CARTESIAN_POINT('Ctrl Pts',(21.0626848505665,-10.233889368157,12.));
#187628=CARTESIAN_POINT('Ctrl Pts',(21.0761174875448,-10.2458211823915,
0.));
#187629=CARTESIAN_POINT('Ctrl Pts',(21.0761174875448,-10.2458211823915,
12.));
#187630=CARTESIAN_POINT('Ctrl Pts',(21.0896090107066,-10.2578738064183,
0.));
#187631=CARTESIAN_POINT('Ctrl Pts',(21.0896090107066,-10.2578738064183,
12.));
#187632=CARTESIAN_POINT('Ctrl Pts',(21.1031582201625,-10.2700468934743,
0.));
#187633=CARTESIAN_POINT('Ctrl Pts',(21.1031582201625,-10.2700468934743,
12.));
#187634=CARTESIAN_POINT('Ctrl Pts',(21.1167639345623,-10.2823401001067,
0.));
#187635=CARTESIAN_POINT('Ctrl Pts',(21.1167639345623,-10.2823401001067,
12.));
#187636=CARTESIAN_POINT('Ctrl Pts',(21.130424990599,-10.2947530860714,0.));
#187637=CARTESIAN_POINT('Ctrl Pts',(21.130424990599,-10.2947530860714,12.));
#187638=CARTESIAN_POINT('Ctrl Pts',(21.1441402425831,-10.307285514268,0.));
#187639=CARTESIAN_POINT('Ctrl Pts',(21.1441402425831,-10.307285514268,12.));
#187640=CARTESIAN_POINT('Ctrl Pts',(21.1579085619959,-10.3199370506541,
0.));
#187641=CARTESIAN_POINT('Ctrl Pts',(21.1579085619959,-10.3199370506541,
12.));
#187642=CARTESIAN_POINT('Ctrl Pts',(21.1717288370512,-10.3327073641574,
0.));
#187643=CARTESIAN_POINT('Ctrl Pts',(21.1717288370512,-10.3327073641574,
12.));
#187644=CARTESIAN_POINT('Ctrl Pts',(21.1855999722427,-10.3455961265706,
0.));
#187645=CARTESIAN_POINT('Ctrl Pts',(21.1855999722427,-10.3455961265706,
12.));
#187646=CARTESIAN_POINT('Ctrl Pts',(21.1995208879205,-10.3586030124595,
0.));
#187647=CARTESIAN_POINT('Ctrl Pts',(21.1995208879205,-10.3586030124595,
12.));
#187648=CARTESIAN_POINT('Ctrl Pts',(21.2134905199359,-10.3717276991137,
0.));
#187649=CARTESIAN_POINT('Ctrl Pts',(21.2134905199359,-10.3717276991137,
12.));
#187650=CARTESIAN_POINT('Ctrl Pts',(21.2275078192708,-10.384969866479,0.));
#187651=CARTESIAN_POINT('Ctrl Pts',(21.2275078192708,-10.384969866479,12.));
#187652=CARTESIAN_POINT('Ctrl Pts',(21.2415717516713,-10.3983291970846,
0.));
#187653=CARTESIAN_POINT('Ctrl Pts',(21.2415717516713,-10.3983291970846,
12.));
#187654=CARTESIAN_POINT('Ctrl Pts',(21.2556812972741,-10.4118053759584,
0.));
#187655=CARTESIAN_POINT('Ctrl Pts',(21.2556812972741,-10.4118053759584,
12.));
#187656=CARTESIAN_POINT('Ctrl Pts',(21.2698354502391,-10.4253980905394,
0.));
#187657=CARTESIAN_POINT('Ctrl Pts',(21.2698354502391,-10.4253980905394,
12.));
#187658=CARTESIAN_POINT('Ctrl Pts',(21.2840332184471,-10.4391070306385,
0.));
#187659=CARTESIAN_POINT('Ctrl Pts',(21.2840332184471,-10.4391070306385,
12.));
#187660=CARTESIAN_POINT('Ctrl Pts',(21.2982736231924,-10.452931888387,0.));
#187661=CARTESIAN_POINT('Ctrl Pts',(21.2982736231924,-10.452931888387,12.));
#187662=CARTESIAN_POINT('Ctrl Pts',(21.312555698873,-10.4668723581768,0.));
#187663=CARTESIAN_POINT('Ctrl Pts',(21.312555698873,-10.4668723581768,12.));
#187664=CARTESIAN_POINT('Ctrl Pts',(21.3268784926823,-10.4809281365933,
0.));
#187665=CARTESIAN_POINT('Ctrl Pts',(21.3268784926823,-10.4809281365933,
12.));
#187666=CARTESIAN_POINT('Ctrl Pts',(21.3412410642912,-10.4950989223341,
0.));
#187667=CARTESIAN_POINT('Ctrl Pts',(21.3412410642912,-10.4950989223341,
12.));
#187668=CARTESIAN_POINT('Ctrl Pts',(21.3556424855822,-10.509384416169,0.));
#187669=CARTESIAN_POINT('Ctrl Pts',(21.3556424855822,-10.509384416169,12.));
#187670=CARTESIAN_POINT('Ctrl Pts',(21.3700818403942,-10.523784320906,0.));
#187671=CARTESIAN_POINT('Ctrl Pts',(21.3700818403942,-10.523784320906,12.));
#187672=CARTESIAN_POINT('Ctrl Pts',(21.3845582242604,-10.5382983413422,
0.));
#187673=CARTESIAN_POINT('Ctrl Pts',(21.3845582242604,-10.5382983413422,
12.));
#187674=CARTESIAN_POINT('Ctrl Pts',(21.3990707441495,-10.5529261842107,
0.));
#187675=CARTESIAN_POINT('Ctrl Pts',(21.3990707441495,-10.5529261842107,
12.));
#187676=CARTESIAN_POINT('Ctrl Pts',(21.4136185181974,-10.5676675581106,
0.));
#187677=CARTESIAN_POINT('Ctrl Pts',(21.4136185181974,-10.5676675581106,
12.));
#187678=CARTESIAN_POINT('Ctrl Pts',(21.4282006754624,-10.582522173457,0.));
#187679=CARTESIAN_POINT('Ctrl Pts',(21.4282006754624,-10.582522173457,12.));
#187680=CARTESIAN_POINT('Ctrl Pts',(21.4428163557137,-10.597489742462,0.));
#187681=CARTESIAN_POINT('Ctrl Pts',(21.4428163557137,-10.597489742462,12.));
#187682=CARTESIAN_POINT('Ctrl Pts',(21.4574647092093,-10.612569979096,0.));
#187683=CARTESIAN_POINT('Ctrl Pts',(21.4574647092093,-10.612569979096,12.));
#187684=CARTESIAN_POINT('Ctrl Pts',(21.4721448964766,-10.6277625990457,
0.));
#187685=CARTESIAN_POINT('Ctrl Pts',(21.4721448964766,-10.6277625990457,
12.));
#187686=CARTESIAN_POINT('Ctrl Pts',(21.4868560880893,-10.6430673196609,
0.));
#187687=CARTESIAN_POINT('Ctrl Pts',(21.4868560880893,-10.6430673196609,
12.));
#187688=CARTESIAN_POINT('Ctrl Pts',(21.5015974644454,-10.6584838598941,
0.));
#187689=CARTESIAN_POINT('Ctrl Pts',(21.5015974644454,-10.6584838598941,
12.));
#187690=CARTESIAN_POINT('Ctrl Pts',(21.5163682155805,-10.6740119402835,
0.));
#187691=CARTESIAN_POINT('Ctrl Pts',(21.5163682155805,-10.6740119402835,
12.));
#187692=CARTESIAN_POINT('Ctrl Pts',(21.531167540981,-10.689651282929,0.));
#187693=CARTESIAN_POINT('Ctrl Pts',(21.531167540981,-10.689651282929,12.));
#187694=CARTESIAN_POINT('Ctrl Pts',(21.5459946493955,-10.7054016114571,
0.));
#187695=CARTESIAN_POINT('Ctrl Pts',(21.5459946493955,-10.7054016114571,
12.));
#187696=CARTESIAN_POINT('Ctrl Pts',(21.5608487586467,-10.7212626509816,
0.));
#187697=CARTESIAN_POINT('Ctrl Pts',(21.5608487586467,-10.7212626509816,
12.));
#187698=CARTESIAN_POINT('Ctrl Pts',(21.5757290954372,-10.7372341280468,
0.));
#187699=CARTESIAN_POINT('Ctrl Pts',(21.5757290954372,-10.7372341280468,
12.));
#187700=CARTESIAN_POINT('Ctrl Pts',(21.5906348951745,-10.7533157705943,
0.));
#187701=CARTESIAN_POINT('Ctrl Pts',(21.5906348951745,-10.7533157705943,
12.));
#187702=CARTESIAN_POINT('Ctrl Pts',(21.6055654018179,-10.7695073079554,
0.));
#187703=CARTESIAN_POINT('Ctrl Pts',(21.6055654018179,-10.7695073079554,
12.));
#187704=CARTESIAN_POINT('Ctrl Pts',(21.6205198677176,-10.7858084708262,
0.));
#187705=CARTESIAN_POINT('Ctrl Pts',(21.6205198677176,-10.7858084708262,
12.));
#187706=CARTESIAN_POINT('Ctrl Pts',(21.6354975534557,-10.802218991237,0.));
#187707=CARTESIAN_POINT('Ctrl Pts',(21.6354975534557,-10.802218991237,12.));
#187708=CARTESIAN_POINT('Ctrl Pts',(21.6504977276864,-10.8187386025135,
0.));
#187709=CARTESIAN_POINT('Ctrl Pts',(21.6504977276864,-10.8187386025135,
12.));
#187710=CARTESIAN_POINT('Ctrl Pts',(21.6655196669727,-10.835367039227,0.));
#187711=CARTESIAN_POINT('Ctrl Pts',(21.6655196669727,-10.835367039227,12.));
#187712=CARTESIAN_POINT('Ctrl Pts',(21.6805626556461,-10.8521040371832,
0.));
#187713=CARTESIAN_POINT('Ctrl Pts',(21.6805626556461,-10.8521040371832,
12.));
#187714=CARTESIAN_POINT('Ctrl Pts',(21.6956259856667,-10.8689493334093,
0.));
#187715=CARTESIAN_POINT('Ctrl Pts',(21.6956259856667,-10.8689493334093,
12.));
#187716=CARTESIAN_POINT('Ctrl Pts',(21.7107089564822,-10.8859026661292,
0.));
#187717=CARTESIAN_POINT('Ctrl Pts',(21.7107089564822,-10.8859026661292,
12.));
#187718=CARTESIAN_POINT('Ctrl Pts',(21.7258108748874,-10.9029637747341,
0.));
#187719=CARTESIAN_POINT('Ctrl Pts',(21.7258108748874,-10.9029637747341,
12.));
#187720=CARTESIAN_POINT('Ctrl Pts',(21.74093105488,-10.9201323997386,0.));
#187721=CARTESIAN_POINT('Ctrl Pts',(21.74093105488,-10.9201323997386,12.));
#187722=CARTESIAN_POINT('Ctrl Pts',(21.7560688175252,-10.9374082827446,
0.));
#187723=CARTESIAN_POINT('Ctrl Pts',(21.7560688175252,-10.9374082827446,
12.));
#187724=CARTESIAN_POINT('Ctrl Pts',(21.7712234908468,-10.9547911664457,
0.));
#187725=CARTESIAN_POINT('Ctrl Pts',(21.7712234908468,-10.9547911664457,
12.));
#187726=CARTESIAN_POINT('Ctrl Pts',(21.7863944097143,-10.9722807946157,
0.));
#187727=CARTESIAN_POINT('Ctrl Pts',(21.7863944097143,-10.9722807946157,
12.));
#187728=CARTESIAN_POINT('Ctrl Pts',(21.8015809157302,-10.9898769120913,
0.));
#187729=CARTESIAN_POINT('Ctrl Pts',(21.8015809157302,-10.9898769120913,
12.));
#187730=CARTESIAN_POINT('Ctrl Pts',(21.8167823571168,-11.0075792647477,
0.));
#187731=CARTESIAN_POINT('Ctrl Pts',(21.8167823571168,-11.0075792647477,
12.));
#187732=CARTESIAN_POINT('Ctrl Pts',(21.8319980886033,-11.0253875994598,
0.));
#187733=CARTESIAN_POINT('Ctrl Pts',(21.8319980886033,-11.0253875994598,
12.));
#187734=CARTESIAN_POINT('Ctrl Pts',(21.8472274713103,-11.0433016640808,
0.));
#187735=CARTESIAN_POINT('Ctrl Pts',(21.8472274713103,-11.0433016640808,
12.));
#187736=CARTESIAN_POINT('Ctrl Pts',(21.8624698726319,-11.0613212074364,
0.));
#187737=CARTESIAN_POINT('Ctrl Pts',(21.8624698726319,-11.0613212074364,
12.));
#187738=CARTESIAN_POINT('Ctrl Pts',(21.8777246661191,-11.0794459793058,
0.));
#187739=CARTESIAN_POINT('Ctrl Pts',(21.8777246661191,-11.0794459793058,
12.));
#187740=CARTESIAN_POINT('Ctrl Pts',(21.8929912313608,-11.0976757303944,
0.));
#187741=CARTESIAN_POINT('Ctrl Pts',(21.8929912313608,-11.0976757303944,
12.));
#187742=CARTESIAN_POINT('Ctrl Pts',(21.9082689538687,-11.1160102123024,
0.));
#187743=CARTESIAN_POINT('Ctrl Pts',(21.9082689538687,-11.1160102123024,
12.));
#187744=CARTESIAN_POINT('Ctrl Pts',(21.9235572249518,-11.134449177474,0.));
#187745=CARTESIAN_POINT('Ctrl Pts',(21.9235572249518,-11.134449177474,12.));
#187746=CARTESIAN_POINT('Ctrl Pts',(21.9388554416437,-11.1529923792002,
0.));
#187747=CARTESIAN_POINT('Ctrl Pts',(21.9388554416437,-11.1529923792002,
12.));
#187748=CARTESIAN_POINT('Ctrl Pts',(21.9541630066504,-11.1716395716375,
0.));
#187749=CARTESIAN_POINT('Ctrl Pts',(21.9541630066504,-11.1716395716375,
12.));
#187750=CARTESIAN_POINT('Ctrl Pts',(21.9694793282913,-11.190390509811,0.));
#187751=CARTESIAN_POINT('Ctrl Pts',(21.9694793282913,-11.190390509811,12.));
#187752=CARTESIAN_POINT('Ctrl Pts',(21.9848038204439,-11.2092449496125,
0.));
#187753=CARTESIAN_POINT('Ctrl Pts',(21.9848038204439,-11.2092449496125,
12.));
#187754=CARTESIAN_POINT('Ctrl Pts',(22.0001359024839,-11.2282026477897,
0.));
#187755=CARTESIAN_POINT('Ctrl Pts',(22.0001359024839,-11.2282026477897,
12.));
#187756=CARTESIAN_POINT('Ctrl Pts',(22.0154749992364,-11.2472633619276,
0.));
#187757=CARTESIAN_POINT('Ctrl Pts',(22.0154749992364,-11.2472633619276,
12.));
#187758=CARTESIAN_POINT('Ctrl Pts',(22.0308205408351,-11.2664268504207,
0.));
#187759=CARTESIAN_POINT('Ctrl Pts',(22.0308205408351,-11.2664268504207,
12.));
#187760=CARTESIAN_POINT('Ctrl Pts',(22.046171962566,-11.2856928724374,0.));
#187761=CARTESIAN_POINT('Ctrl Pts',(22.046171962566,-11.2856928724374,12.));
#187762=CARTESIAN_POINT('Ctrl Pts',(22.0615287047179,-11.3050611878771,
0.));
#187763=CARTESIAN_POINT('Ctrl Pts',(22.0615287047179,-11.3050611878771,
12.));
#187764=CARTESIAN_POINT('Ctrl Pts',(22.0768902124267,-11.3245315573168,
0.));
#187765=CARTESIAN_POINT('Ctrl Pts',(22.0768902124267,-11.3245315573168,
12.));
#187766=CARTESIAN_POINT('Ctrl Pts',(22.0922559355293,-11.3441037419553,
0.));
#187767=CARTESIAN_POINT('Ctrl Pts',(22.0922559355293,-11.3441037419553,
12.));
#187768=CARTESIAN_POINT('Ctrl Pts',(22.1076253283978,-11.3637775035367,
0.));
#187769=CARTESIAN_POINT('Ctrl Pts',(22.1076253283978,-11.3637775035367,
12.));
#187770=CARTESIAN_POINT('Ctrl Pts',(22.1229978500185,-11.3835526044256,
0.));
#187771=CARTESIAN_POINT('Ctrl Pts',(22.1229978500185,-11.3835526044256,
12.));
#187772=CARTESIAN_POINT('Ctrl Pts',(22.1383729640963,-11.4034288076909,
0.));
#187773=CARTESIAN_POINT('Ctrl Pts',(22.1383729640963,-11.4034288076909,
12.));
#187774=CARTESIAN_POINT('Ctrl Pts',(22.1537501391486,-11.4234058771742,
0.));
#187775=CARTESIAN_POINT('Ctrl Pts',(22.1537501391486,-11.4234058771742,
12.));
#187776=CARTESIAN_POINT('Ctrl Pts',(22.1691288486096,-11.443483577557,0.));
#187777=CARTESIAN_POINT('Ctrl Pts',(22.1691288486096,-11.443483577557,12.));
#187778=CARTESIAN_POINT('Ctrl Pts',(22.1845085709169,-11.463661674411,0.));
#187779=CARTESIAN_POINT('Ctrl Pts',(22.1845085709169,-11.463661674411,12.));
#187780=CARTESIAN_POINT('Ctrl Pts',(22.1998887896435,-11.4839399342589,
0.));
#187781=CARTESIAN_POINT('Ctrl Pts',(22.1998887896435,-11.4839399342589,
12.));
#187782=CARTESIAN_POINT('Ctrl Pts',(22.215268993102,-11.504318124424,0.));
#187783=CARTESIAN_POINT('Ctrl Pts',(22.215268993102,-11.504318124424,12.));
#187784=CARTESIAN_POINT('Ctrl Pts',(22.2306486738899,-11.5247960128476,
0.));
#187785=CARTESIAN_POINT('Ctrl Pts',(22.2306486738899,-11.5247960128476,
12.));
#187786=CARTESIAN_POINT('Ctrl Pts',(22.2460273284653,-11.545373367912,0.));
#187787=CARTESIAN_POINT('Ctrl Pts',(22.2460273284653,-11.545373367912,12.));
#187788=CARTESIAN_POINT('Ctrl Pts',(22.2614044566898,-11.5660499582403,
0.));
#187789=CARTESIAN_POINT('Ctrl Pts',(22.2614044566898,-11.5660499582403,
12.));
#187790=CARTESIAN_POINT('Ctrl Pts',(22.2767795614349,-11.5868255525189,
0.));
#187791=CARTESIAN_POINT('Ctrl Pts',(22.2767795614349,-11.5868255525189,
12.));
#187792=CARTESIAN_POINT('Ctrl Pts',(22.2921521480357,-11.6076999192359,
0.));
#187793=CARTESIAN_POINT('Ctrl Pts',(22.2921521480357,-11.6076999192359,
12.));
#187794=CARTESIAN_POINT('Ctrl Pts',(22.3075217249049,-11.6286728270011,
0.));
#187795=CARTESIAN_POINT('Ctrl Pts',(22.3075217249049,-11.6286728270011,
12.));
#187796=CARTESIAN_POINT('Ctrl Pts',(22.3228878043976,-11.6497440449858,
0.));
#187797=CARTESIAN_POINT('Ctrl Pts',(22.3228878043976,-11.6497440449858,
12.));
#187798=CARTESIAN_POINT('Ctrl Pts',(22.3382499035618,-11.6709133432986,
0.));
#187799=CARTESIAN_POINT('Ctrl Pts',(22.3382499035618,-11.6709133432986,
12.));
#187800=CARTESIAN_POINT('Ctrl Pts',(22.3536075450028,-11.6921804934056,
0.));
#187801=CARTESIAN_POINT('Ctrl Pts',(22.3536075450028,-11.6921804934056,
12.));
#187802=CARTESIAN_POINT('Ctrl Pts',(22.3689602575492,-11.7135452684532,
0.));
#187803=CARTESIAN_POINT('Ctrl Pts',(22.3689602575492,-11.7135452684532,
12.));
#187804=CARTESIAN_POINT('Ctrl Pts',(22.3843075773905,-11.7350074437961,
0.));
#187805=CARTESIAN_POINT('Ctrl Pts',(22.3843075773905,-11.7350074437961,
12.));
#187806=CARTESIAN_POINT('Ctrl Pts',(22.39964904692,-11.7565667964765,0.));
#187807=CARTESIAN_POINT('Ctrl Pts',(22.39964904692,-11.7565667964765,12.));
#187808=CARTESIAN_POINT('Ctrl Pts',(22.4149842125018,-11.7782231042041,
0.));
#187809=CARTESIAN_POINT('Ctrl Pts',(22.4149842125018,-11.7782231042041,
12.));
#187810=CARTESIAN_POINT('Ctrl Pts',(22.4303126226468,-11.7999761445175,
0.));
#187811=CARTESIAN_POINT('Ctrl Pts',(22.4303126226468,-11.7999761445175,
12.));
#187812=CARTESIAN_POINT('Ctrl Pts',(22.4456338258738,-11.8218256937889,
0.));
#187813=CARTESIAN_POINT('Ctrl Pts',(22.4456338258738,-11.8218256937889,
12.));
#187814=CARTESIAN_POINT('Ctrl Pts',(22.4609473690469,-11.8437715264487,
0.));
#187815=CARTESIAN_POINT('Ctrl Pts',(22.4609473690469,-11.8437715264487,
12.));
#187816=CARTESIAN_POINT('Ctrl Pts',(22.4762527946694,-11.8658134137018,
0.));
#187817=CARTESIAN_POINT('Ctrl Pts',(22.4762527946694,-11.8658134137018,
12.));
#187818=CARTESIAN_POINT('Ctrl Pts',(22.4915496418472,-11.8879511239941,
0.));
#187819=CARTESIAN_POINT('Ctrl Pts',(22.4915496418472,-11.8879511239941,
12.));
#187820=CARTESIAN_POINT('Ctrl Pts',(22.5068374513958,-11.9101844254555,
0.));
#187821=CARTESIAN_POINT('Ctrl Pts',(22.5068374513958,-11.9101844254555,
12.));
#187822=CARTESIAN_POINT('Ctrl Pts',(22.5221157697869,-11.9325130877801,
0.));
#187823=CARTESIAN_POINT('Ctrl Pts',(22.5221157697869,-11.9325130877801,
12.));
#187824=CARTESIAN_POINT('Ctrl Pts',(22.5373841537299,-11.9549368843996,
0.));
#187825=CARTESIAN_POINT('Ctrl Pts',(22.5373841537299,-11.9549368843996,
12.));
#187826=CARTESIAN_POINT('Ctrl Pts',(22.5526421741159,-11.9774555943496,
0.));
#187827=CARTESIAN_POINT('Ctrl Pts',(22.5526421741159,-11.9774555943496,
12.));
#187828=CARTESIAN_POINT('Ctrl Pts',(22.5678894211194,-12.0000690046697,
0.));
#187829=CARTESIAN_POINT('Ctrl Pts',(22.5678894211194,-12.0000690046697,
12.));
#187830=CARTESIAN_POINT('Ctrl Pts',(22.5831255061306,-12.0227769113132,
0.));
#187831=CARTESIAN_POINT('Ctrl Pts',(22.5831255061306,-12.0227769113132,
12.));
#187832=CARTESIAN_POINT('Ctrl Pts',(22.5983500505675,-12.0455791139135,
0.));
#187833=CARTESIAN_POINT('Ctrl Pts',(22.5983500505675,-12.0455791139135,
12.));
#187834=CARTESIAN_POINT('Ctrl Pts',(22.613562676493,-12.0684754113869,0.));
#187835=CARTESIAN_POINT('Ctrl Pts',(22.613562676493,-12.0684754113869,12.));
#187836=CARTESIAN_POINT('Ctrl Pts',(22.628762996708,-12.0914655972828,0.));
#187837=CARTESIAN_POINT('Ctrl Pts',(22.628762996708,-12.0914655972828,12.));
#187838=CARTESIAN_POINT('Ctrl Pts',(22.6439506046611,-12.1145494550384,
0.));
#187839=CARTESIAN_POINT('Ctrl Pts',(22.6439506046611,-12.1145494550384,
12.));
#187840=CARTESIAN_POINT('Ctrl Pts',(22.6591250653942,-12.1377267537141,
0.));
#187841=CARTESIAN_POINT('Ctrl Pts',(22.6591250653942,-12.1377267537141,
12.));
#187842=CARTESIAN_POINT('Ctrl Pts',(22.6742859034891,-12.1609972423089,
0.));
#187843=CARTESIAN_POINT('Ctrl Pts',(22.6742859034891,-12.1609972423089,
12.));
#187844=CARTESIAN_POINT('Ctrl Pts',(22.6894326204959,-12.1843606579246,
0.));
#187845=CARTESIAN_POINT('Ctrl Pts',(22.6894326204959,-12.1843606579246,
12.));
#187846=CARTESIAN_POINT('Ctrl Pts',(22.7045647168659,-12.2078167360267,
0.));
#187847=CARTESIAN_POINT('Ctrl Pts',(22.7045647168659,-12.2078167360267,
12.));
#187848=CARTESIAN_POINT('Ctrl Pts',(22.7196817119299,-12.2313652198047,
0.));
#187849=CARTESIAN_POINT('Ctrl Pts',(22.7196817119299,-12.2313652198047,
12.));
#187850=CARTESIAN_POINT('Ctrl Pts',(22.7347831655251,-12.2550058702389,
0.));
#187851=CARTESIAN_POINT('Ctrl Pts',(22.7347831655251,-12.2550058702389,
12.));
#187852=CARTESIAN_POINT('Ctrl Pts',(22.7498686970096,-12.2787384750747,
0.));
#187853=CARTESIAN_POINT('Ctrl Pts',(22.7498686970096,-12.2787384750747,
12.));
#187854=CARTESIAN_POINT('Ctrl Pts',(22.7649380101154,-12.3025628601812,
0.));
#187855=CARTESIAN_POINT('Ctrl Pts',(22.7649380101154,-12.3025628601812,
12.));
#187856=CARTESIAN_POINT('Ctrl Pts',(22.7799908974947,-12.3264788926108,
0.));
#187857=CARTESIAN_POINT('Ctrl Pts',(22.7799908974947,-12.3264788926108,
12.));
#187858=CARTESIAN_POINT('Ctrl Pts',(22.7950272216959,-12.3504864740361,
0.));
#187859=CARTESIAN_POINT('Ctrl Pts',(22.7950272216959,-12.3504864740361,
12.));
#187860=CARTESIAN_POINT('Ctrl Pts',(22.8100469022632,-12.3745855366772,
0.));
#187861=CARTESIAN_POINT('Ctrl Pts',(22.8100469022632,-12.3745855366772,
12.));
#187862=CARTESIAN_POINT('Ctrl Pts',(22.8220493007353,-12.393937937903,0.));
#187863=CARTESIAN_POINT('Ctrl Pts',(22.8220493007353,-12.393937937903,12.));
#187864=CARTESIAN_POINT('Ctrl Pts',(22.8310435872852,-12.4084933766366,
0.));
#187865=CARTESIAN_POINT('Ctrl Pts',(22.8310435872852,-12.4084933766366,
12.));
#187866=CARTESIAN_POINT('Ctrl Pts',(22.8370364396497,-12.4182152851867,
0.));
#187867=CARTESIAN_POINT('Ctrl Pts',(22.8370364396497,-12.4182152851867,
12.));
#187868=CARTESIAN_POINT('Ctrl Pts',(22.8400320311648,-12.4230808101438,
0.));
#187869=CARTESIAN_POINT('Ctrl Pts',(22.8400320311648,-12.4230808101438,
12.));
#187870=CARTESIAN_POINT('',(22.8400320311648,-12.4230808101438,0.));
#187871=CARTESIAN_POINT('Ctrl Pts',(20.353053841303,-9.71462809124917,0.));
#187872=CARTESIAN_POINT('Ctrl Pts',(20.353060251684,-9.71462954053074,0.));
#187873=CARTESIAN_POINT('Ctrl Pts',(20.3531126095522,-9.71465227853122,
0.));
#187874=CARTESIAN_POINT('Ctrl Pts',(20.3533097561886,-9.71474590350792,
0.));
#187875=CARTESIAN_POINT('Ctrl Pts',(20.3538098605706,-9.71498978052101,
0.));
#187876=CARTESIAN_POINT('Ctrl Pts',(20.3548282742361,-9.71549257088175,
0.));
#187877=CARTESIAN_POINT('Ctrl Pts',(20.3562337557875,-9.71619192554147,
0.));
#187878=CARTESIAN_POINT('Ctrl Pts',(20.3580133103357,-9.71708493723062,
0.));
#187879=CARTESIAN_POINT('Ctrl Pts',(20.3601498764344,-9.71816778327999,
0.));
#187880=CARTESIAN_POINT('Ctrl Pts',(20.362625691398,-9.71943648548115,0.));
#187881=CARTESIAN_POINT('Ctrl Pts',(20.3654261611055,-9.72088778381102,
0.));
#187882=CARTESIAN_POINT('Ctrl Pts',(20.3685406190576,-9.72251930722504,
0.));
#187883=CARTESIAN_POINT('Ctrl Pts',(20.371960235676,-9.72432910043193,0.));
#187884=CARTESIAN_POINT('Ctrl Pts',(20.3756766651952,-9.72631531732871,
0.));
#187885=CARTESIAN_POINT('Ctrl Pts',(20.3796805893304,-9.72847589116533,
0.));
#187886=CARTESIAN_POINT('Ctrl Pts',(20.3839624556742,-9.73080870123726,
0.));
#187887=CARTESIAN_POINT('Ctrl Pts',(20.3885129129912,-9.73331167102812,
0.));
#187888=CARTESIAN_POINT('Ctrl Pts',(20.3933234845646,-9.7359829201425,0.));
#187889=CARTESIAN_POINT('Ctrl Pts',(20.3983866213331,-9.73882077613206,
0.));
#187890=CARTESIAN_POINT('Ctrl Pts',(20.4036953576549,-9.74182369656273,
0.));
#187891=CARTESIAN_POINT('Ctrl Pts',(20.4092430879861,-9.74499021838537,
0.));
#187892=CARTESIAN_POINT('Ctrl Pts',(20.4150232777393,-9.74831889242175,
0.));
#187893=CARTESIAN_POINT('Ctrl Pts',(20.4210295275818,-9.75180829786433,
0.));
#187894=CARTESIAN_POINT('Ctrl Pts',(20.4272556476629,-9.75545705902416,
0.));
#187895=CARTESIAN_POINT('Ctrl Pts',(20.4336957355474,-9.7592638628993,0.));
#187896=CARTESIAN_POINT('Ctrl Pts',(20.4403442329401,-9.76322747195502,
0.));
#187897=CARTESIAN_POINT('Ctrl Pts',(20.447195862298,-9.76734670980897,0.));
#187898=CARTESIAN_POINT('Ctrl Pts',(20.4542455817527,-9.7716204510407,0.));
#187899=CARTESIAN_POINT('Ctrl Pts',(20.4614885274973,-9.77604760815523,
0.));
#187900=CARTESIAN_POINT('Ctrl Pts',(20.4689199790668,-9.78062712373313,
0.));
#187901=CARTESIAN_POINT('Ctrl Pts',(20.4765353711585,-9.78535797314162,
0.));
#187902=CARTESIAN_POINT('Ctrl Pts',(20.4843302955329,-9.7902391649866,0.));
#187903=CARTESIAN_POINT('Ctrl Pts',(20.4923005087945,-9.79526974288344,
0.));
#187904=CARTESIAN_POINT('Ctrl Pts',(20.500441931211,-9.80044878520968,0.));
#187905=CARTESIAN_POINT('Ctrl Pts',(20.5087506310507,-9.80577540161103,
0.));
#187906=CARTESIAN_POINT('Ctrl Pts',(20.5172228122839,-9.81124873025278,
0.));
#187907=CARTESIAN_POINT('Ctrl Pts',(20.5258548000625,-9.81686793455918,
0.));
#187908=CARTESIAN_POINT('Ctrl Pts',(20.534643029951,-9.82263220080328,0.));
#187909=CARTESIAN_POINT('Ctrl Pts',(20.5435840460717,-9.82854073773858,
0.));
#187910=CARTESIAN_POINT('Ctrl Pts',(20.5526744976461,-9.83459277585321,
0.));
#187911=CARTESIAN_POINT('Ctrl Pts',(20.5619111362406,-9.84078756677589,
0.));
#187912=CARTESIAN_POINT('Ctrl Pts',(20.5712908125145,-9.84712438256308,
0.));
#187913=CARTESIAN_POINT('Ctrl Pts',(20.580810471002,-9.85360251457004,0.));
#187914=CARTESIAN_POINT('Ctrl Pts',(20.5904671449754,-9.8602212723275,0.));
#187915=CARTESIAN_POINT('Ctrl Pts',(20.6002579513696,-9.86697998242612,
0.));
#187916=CARTESIAN_POINT('Ctrl Pts',(20.6101800854491,-9.87387798732944,
0.));
#187917=CARTESIAN_POINT('Ctrl Pts',(20.6202308177472,-9.88091464472669,
0.));
#187918=CARTESIAN_POINT('Ctrl Pts',(20.6304074914086,-9.88808932697305,
0.));
#187919=CARTESIAN_POINT('Ctrl Pts',(20.6407075193977,-9.89540142049124,
0.));
#187920=CARTESIAN_POINT('Ctrl Pts',(20.6511283817415,-9.90285032516696,
0.));
#187921=CARTESIAN_POINT('Ctrl Pts',(20.6616676228315,-9.91043545377005,
0.));
#187922=CARTESIAN_POINT('Ctrl Pts',(20.6723228488261,-9.91815623141285,
0.));
#187923=CARTESIAN_POINT('Ctrl Pts',(20.6830917250255,-9.92601209498751,
0.));
#187924=CARTESIAN_POINT('Ctrl Pts',(20.6939719732485,-9.93400249259737,
0.));
#187925=CARTESIAN_POINT('Ctrl Pts',(20.7049613692237,-9.94212688298251,
0.));
#187926=CARTESIAN_POINT('Ctrl Pts',(20.716057740758,-9.95038473514962,0.));
#187927=CARTESIAN_POINT('Ctrl Pts',(20.7272589658752,-9.95877552798403,
0.));
#187928=CARTESIAN_POINT('Ctrl Pts',(20.7385629709795,-9.96729874986199,
0.));
#187929=CARTESIAN_POINT('Ctrl Pts',(20.7499677289625,-9.97595389823461,
0.));
#187930=CARTESIAN_POINT('Ctrl Pts',(20.7614712574989,-9.98474047926846,
0.));
#187931=CARTESIAN_POINT('Ctrl Pts',(20.7730716175417,-9.99365800754638,
0.));
#187932=CARTESIAN_POINT('Ctrl Pts',(20.7847669117568,-10.0027060057389,
0.));
#187933=CARTESIAN_POINT('Ctrl Pts',(20.7965552829907,-10.0118840042786,
0.));
#187934=CARTESIAN_POINT('Ctrl Pts',(20.8084349126885,-10.0211915410095,
0.));
#187935=CARTESIAN_POINT('Ctrl Pts',(20.8204040196599,-10.0306281609435,
0.));
#187936=CARTESIAN_POINT('Ctrl Pts',(20.8324608588906,-10.0401934160234,
0.));
#187937=CARTESIAN_POINT('Ctrl Pts',(20.8446037203402,-10.0498868648733,
0.));
#187938=CARTESIAN_POINT('Ctrl Pts',(20.856830927732,-10.0597080725375,0.));
#187939=CARTESIAN_POINT('Ctrl Pts',(20.8691408373705,-10.0696566102219,
0.));
#187940=CARTESIAN_POINT('Ctrl Pts',(20.8815318371844,-10.0797320551154,
0.));
#187941=CARTESIAN_POINT('Ctrl Pts',(20.8940023457371,-10.0899339901916,
0.));
#187942=CARTESIAN_POINT('Ctrl Pts',(20.9065508112556,-10.1002620040076,
0.));
#187943=CARTESIAN_POINT('Ctrl Pts',(20.9191757106266,-10.1107156904836,
0.));
#187944=CARTESIAN_POINT('Ctrl Pts',(20.931875548473,-10.1212946487057,0.));
#187945=CARTESIAN_POINT('Ctrl Pts',(20.944648856393,-10.1319984827909,0.));
#187946=CARTESIAN_POINT('Ctrl Pts',(20.9574941921591,-10.1428268017257,
0.));
#187947=CARTESIAN_POINT('Ctrl Pts',(20.970410138937,-10.1537792192065,0.));
#187948=CARTESIAN_POINT('Ctrl Pts',(20.9833953044736,-10.1648553534567,
0.));
#187949=CARTESIAN_POINT('Ctrl Pts',(20.9964483203685,-10.1760548270765,
0.));
#187950=CARTESIAN_POINT('Ctrl Pts',(21.0095678414486,-10.1873772669358,
0.));
#187951=CARTESIAN_POINT('Ctrl Pts',(21.0227525451107,-10.1988223040425,
0.));
#187952=CARTESIAN_POINT('Ctrl Pts',(21.0360011306814,-10.2103895734124,
0.));
#187953=CARTESIAN_POINT('Ctrl Pts',(21.0493123187483,-10.2220787139157,
0.));
#187954=CARTESIAN_POINT('Ctrl Pts',(21.0626848505665,-10.233889368157,0.));
#187955=CARTESIAN_POINT('Ctrl Pts',(21.0761174875448,-10.2458211823915,
0.));
#187956=CARTESIAN_POINT('Ctrl Pts',(21.0896090107066,-10.2578738064183,
0.));
#187957=CARTESIAN_POINT('Ctrl Pts',(21.1031582201625,-10.2700468934743,
0.));
#187958=CARTESIAN_POINT('Ctrl Pts',(21.1167639345623,-10.2823401001067,
0.));
#187959=CARTESIAN_POINT('Ctrl Pts',(21.130424990599,-10.2947530860714,0.));
#187960=CARTESIAN_POINT('Ctrl Pts',(21.1441402425831,-10.307285514268,0.));
#187961=CARTESIAN_POINT('Ctrl Pts',(21.1579085619959,-10.3199370506541,
0.));
#187962=CARTESIAN_POINT('Ctrl Pts',(21.1717288370512,-10.3327073641574,
0.));
#187963=CARTESIAN_POINT('Ctrl Pts',(21.1855999722427,-10.3455961265706,
0.));
#187964=CARTESIAN_POINT('Ctrl Pts',(21.1995208879205,-10.3586030124595,
0.));
#187965=CARTESIAN_POINT('Ctrl Pts',(21.2134905199359,-10.3717276991137,
0.));
#187966=CARTESIAN_POINT('Ctrl Pts',(21.2275078192708,-10.384969866479,0.));
#187967=CARTESIAN_POINT('Ctrl Pts',(21.2415717516713,-10.3983291970846,
0.));
#187968=CARTESIAN_POINT('Ctrl Pts',(21.2556812972741,-10.4118053759584,
0.));
#187969=CARTESIAN_POINT('Ctrl Pts',(21.2698354502391,-10.4253980905394,
0.));
#187970=CARTESIAN_POINT('Ctrl Pts',(21.2840332184471,-10.4391070306385,
0.));
#187971=CARTESIAN_POINT('Ctrl Pts',(21.2982736231924,-10.452931888387,0.));
#187972=CARTESIAN_POINT('Ctrl Pts',(21.312555698873,-10.4668723581768,0.));
#187973=CARTESIAN_POINT('Ctrl Pts',(21.3268784926823,-10.4809281365933,
0.));
#187974=CARTESIAN_POINT('Ctrl Pts',(21.3412410642912,-10.4950989223341,
0.));
#187975=CARTESIAN_POINT('Ctrl Pts',(21.3556424855822,-10.509384416169,0.));
#187976=CARTESIAN_POINT('Ctrl Pts',(21.3700818403942,-10.523784320906,0.));
#187977=CARTESIAN_POINT('Ctrl Pts',(21.3845582242604,-10.5382983413422,
0.));
#187978=CARTESIAN_POINT('Ctrl Pts',(21.3990707441495,-10.5529261842107,
0.));
#187979=CARTESIAN_POINT('Ctrl Pts',(21.4136185181974,-10.5676675581106,
0.));
#187980=CARTESIAN_POINT('Ctrl Pts',(21.4282006754624,-10.582522173457,0.));
#187981=CARTESIAN_POINT('Ctrl Pts',(21.4428163557137,-10.597489742462,0.));
#187982=CARTESIAN_POINT('Ctrl Pts',(21.4574647092093,-10.612569979096,0.));
#187983=CARTESIAN_POINT('Ctrl Pts',(21.4721448964766,-10.6277625990457,
0.));
#187984=CARTESIAN_POINT('Ctrl Pts',(21.4868560880893,-10.6430673196609,
0.));
#187985=CARTESIAN_POINT('Ctrl Pts',(21.5015974644454,-10.6584838598941,
0.));
#187986=CARTESIAN_POINT('Ctrl Pts',(21.5163682155805,-10.6740119402835,
0.));
#187987=CARTESIAN_POINT('Ctrl Pts',(21.531167540981,-10.689651282929,0.));
#187988=CARTESIAN_POINT('Ctrl Pts',(21.5459946493955,-10.7054016114571,
0.));
#187989=CARTESIAN_POINT('Ctrl Pts',(21.5608487586467,-10.7212626509816,
0.));
#187990=CARTESIAN_POINT('Ctrl Pts',(21.5757290954372,-10.7372341280468,
0.));
#187991=CARTESIAN_POINT('Ctrl Pts',(21.5906348951745,-10.7533157705943,
0.));
#187992=CARTESIAN_POINT('Ctrl Pts',(21.6055654018179,-10.7695073079554,
0.));
#187993=CARTESIAN_POINT('Ctrl Pts',(21.6205198677176,-10.7858084708262,
0.));
#187994=CARTESIAN_POINT('Ctrl Pts',(21.6354975534557,-10.802218991237,0.));
#187995=CARTESIAN_POINT('Ctrl Pts',(21.6504977276864,-10.8187386025135,
0.));
#187996=CARTESIAN_POINT('Ctrl Pts',(21.6655196669727,-10.835367039227,0.));
#187997=CARTESIAN_POINT('Ctrl Pts',(21.6805626556461,-10.8521040371832,
0.));
#187998=CARTESIAN_POINT('Ctrl Pts',(21.6956259856667,-10.8689493334093,
0.));
#187999=CARTESIAN_POINT('Ctrl Pts',(21.7107089564822,-10.8859026661292,
0.));
#188000=CARTESIAN_POINT('Ctrl Pts',(21.7258108748874,-10.9029637747341,
0.));
#188001=CARTESIAN_POINT('Ctrl Pts',(21.74093105488,-10.9201323997386,0.));
#188002=CARTESIAN_POINT('Ctrl Pts',(21.7560688175252,-10.9374082827446,
0.));
#188003=CARTESIAN_POINT('Ctrl Pts',(21.7712234908468,-10.9547911664457,
0.));
#188004=CARTESIAN_POINT('Ctrl Pts',(21.7863944097143,-10.9722807946157,
0.));
#188005=CARTESIAN_POINT('Ctrl Pts',(21.8015809157302,-10.9898769120913,
0.));
#188006=CARTESIAN_POINT('Ctrl Pts',(21.8167823571168,-11.0075792647477,
0.));
#188007=CARTESIAN_POINT('Ctrl Pts',(21.8319980886033,-11.0253875994598,
0.));
#188008=CARTESIAN_POINT('Ctrl Pts',(21.8472274713103,-11.0433016640808,
0.));
#188009=CARTESIAN_POINT('Ctrl Pts',(21.8624698726319,-11.0613212074364,
0.));
#188010=CARTESIAN_POINT('Ctrl Pts',(21.8777246661191,-11.0794459793058,
0.));
#188011=CARTESIAN_POINT('Ctrl Pts',(21.8929912313608,-11.0976757303944,
0.));
#188012=CARTESIAN_POINT('Ctrl Pts',(21.9082689538687,-11.1160102123024,
0.));
#188013=CARTESIAN_POINT('Ctrl Pts',(21.9235572249518,-11.134449177474,0.));
#188014=CARTESIAN_POINT('Ctrl Pts',(21.9388554416437,-11.1529923792002,
0.));
#188015=CARTESIAN_POINT('Ctrl Pts',(21.9541630066504,-11.1716395716375,
0.));
#188016=CARTESIAN_POINT('Ctrl Pts',(21.9694793282913,-11.190390509811,0.));
#188017=CARTESIAN_POINT('Ctrl Pts',(21.9848038204439,-11.2092449496125,
0.));
#188018=CARTESIAN_POINT('Ctrl Pts',(22.0001359024839,-11.2282026477897,
0.));
#188019=CARTESIAN_POINT('Ctrl Pts',(22.0154749992364,-11.2472633619276,
0.));
#188020=CARTESIAN_POINT('Ctrl Pts',(22.0308205408351,-11.2664268504207,
0.));
#188021=CARTESIAN_POINT('Ctrl Pts',(22.046171962566,-11.2856928724374,0.));
#188022=CARTESIAN_POINT('Ctrl Pts',(22.0615287047179,-11.3050611878771,
0.));
#188023=CARTESIAN_POINT('Ctrl Pts',(22.0768902124267,-11.3245315573168,
0.));
#188024=CARTESIAN_POINT('Ctrl Pts',(22.0922559355293,-11.3441037419553,
0.));
#188025=CARTESIAN_POINT('Ctrl Pts',(22.1076253283978,-11.3637775035367,
0.));
#188026=CARTESIAN_POINT('Ctrl Pts',(22.1229978500185,-11.3835526044256,
0.));
#188027=CARTESIAN_POINT('Ctrl Pts',(22.1383729640963,-11.4034288076909,
0.));
#188028=CARTESIAN_POINT('Ctrl Pts',(22.1537501391486,-11.4234058771742,
0.));
#188029=CARTESIAN_POINT('Ctrl Pts',(22.1691288486096,-11.443483577557,0.));
#188030=CARTESIAN_POINT('Ctrl Pts',(22.1845085709169,-11.463661674411,0.));
#188031=CARTESIAN_POINT('Ctrl Pts',(22.1998887896435,-11.4839399342589,
0.));
#188032=CARTESIAN_POINT('Ctrl Pts',(22.215268993102,-11.504318124424,0.));
#188033=CARTESIAN_POINT('Ctrl Pts',(22.2306486738899,-11.5247960128476,
0.));
#188034=CARTESIAN_POINT('Ctrl Pts',(22.2460273284653,-11.545373367912,0.));
#188035=CARTESIAN_POINT('Ctrl Pts',(22.2614044566898,-11.5660499582403,
0.));
#188036=CARTESIAN_POINT('Ctrl Pts',(22.2767795614349,-11.5868255525189,
0.));
#188037=CARTESIAN_POINT('Ctrl Pts',(22.2921521480357,-11.6076999192359,
0.));
#188038=CARTESIAN_POINT('Ctrl Pts',(22.3075217249049,-11.6286728270011,
0.));
#188039=CARTESIAN_POINT('Ctrl Pts',(22.3228878043976,-11.6497440449858,
0.));
#188040=CARTESIAN_POINT('Ctrl Pts',(22.3382499035618,-11.6709133432986,
0.));
#188041=CARTESIAN_POINT('Ctrl Pts',(22.3536075450028,-11.6921804934056,
0.));
#188042=CARTESIAN_POINT('Ctrl Pts',(22.3689602575492,-11.7135452684532,
0.));
#188043=CARTESIAN_POINT('Ctrl Pts',(22.3843075773905,-11.7350074437961,
0.));
#188044=CARTESIAN_POINT('Ctrl Pts',(22.39964904692,-11.7565667964765,0.));
#188045=CARTESIAN_POINT('Ctrl Pts',(22.4149842125018,-11.7782231042041,
0.));
#188046=CARTESIAN_POINT('Ctrl Pts',(22.4303126226468,-11.7999761445175,
0.));
#188047=CARTESIAN_POINT('Ctrl Pts',(22.4456338258738,-11.8218256937889,
0.));
#188048=CARTESIAN_POINT('Ctrl Pts',(22.4609473690469,-11.8437715264487,
0.));
#188049=CARTESIAN_POINT('Ctrl Pts',(22.4762527946694,-11.8658134137018,
0.));
#188050=CARTESIAN_POINT('Ctrl Pts',(22.4915496418472,-11.8879511239941,
0.));
#188051=CARTESIAN_POINT('Ctrl Pts',(22.5068374513958,-11.9101844254555,
0.));
#188052=CARTESIAN_POINT('Ctrl Pts',(22.5221157697869,-11.9325130877801,
0.));
#188053=CARTESIAN_POINT('Ctrl Pts',(22.5373841537299,-11.9549368843996,
0.));
#188054=CARTESIAN_POINT('Ctrl Pts',(22.5526421741159,-11.9774555943496,
0.));
#188055=CARTESIAN_POINT('Ctrl Pts',(22.5678894211194,-12.0000690046697,
0.));
#188056=CARTESIAN_POINT('Ctrl Pts',(22.5831255061306,-12.0227769113132,
0.));
#188057=CARTESIAN_POINT('Ctrl Pts',(22.5983500505675,-12.0455791139135,
0.));
#188058=CARTESIAN_POINT('Ctrl Pts',(22.613562676493,-12.0684754113869,0.));
#188059=CARTESIAN_POINT('Ctrl Pts',(22.628762996708,-12.0914655972828,0.));
#188060=CARTESIAN_POINT('Ctrl Pts',(22.6439506046611,-12.1145494550384,
0.));
#188061=CARTESIAN_POINT('Ctrl Pts',(22.6591250653942,-12.1377267537141,
0.));
#188062=CARTESIAN_POINT('Ctrl Pts',(22.6742859034891,-12.1609972423089,
0.));
#188063=CARTESIAN_POINT('Ctrl Pts',(22.6894326204959,-12.1843606579246,
0.));
#188064=CARTESIAN_POINT('Ctrl Pts',(22.7045647168659,-12.2078167360267,
0.));
#188065=CARTESIAN_POINT('Ctrl Pts',(22.7196817119299,-12.2313652198047,
0.));
#188066=CARTESIAN_POINT('Ctrl Pts',(22.7347831655251,-12.2550058702389,
0.));
#188067=CARTESIAN_POINT('Ctrl Pts',(22.7498686970096,-12.2787384750747,
0.));
#188068=CARTESIAN_POINT('Ctrl Pts',(22.7649380101154,-12.3025628601812,
0.));
#188069=CARTESIAN_POINT('Ctrl Pts',(22.7799908974947,-12.3264788926108,
0.));
#188070=CARTESIAN_POINT('Ctrl Pts',(22.7950272216959,-12.3504864740361,
0.));
#188071=CARTESIAN_POINT('Ctrl Pts',(22.8100469022632,-12.3745855366772,
0.));
#188072=CARTESIAN_POINT('Ctrl Pts',(22.8220493007353,-12.393937937903,0.));
#188073=CARTESIAN_POINT('Ctrl Pts',(22.8310435872852,-12.4084933766366,
0.));
#188074=CARTESIAN_POINT('Ctrl Pts',(22.8370364396497,-12.4182152851867,
0.));
#188075=CARTESIAN_POINT('Ctrl Pts',(22.8400320311648,-12.4230808101438,
0.));
#188076=CARTESIAN_POINT('',(22.8400320311648,-12.4230808101438,0.));
#188077=CARTESIAN_POINT('Origin',(16.3449727195351,-13.9675290154577,0.));
#188078=CARTESIAN_POINT('',(17.1452095830632,-14.6513681262571,0.));
#188079=CARTESIAN_POINT('',(17.1452095830632,-14.6513681262571,0.));
#188080=CARTESIAN_POINT('',(8.17248635976757,-6.98376450772884,0.));
#188081=CARTESIAN_POINT('Ctrl Pts',(22.1787195904339,-13.5685075571671,
0.));
#188082=CARTESIAN_POINT('Ctrl Pts',(22.1787195904339,-13.5685075571671,
12.));
#188083=CARTESIAN_POINT('Ctrl Pts',(22.1730081264583,-13.5683460612913,
0.));
#188084=CARTESIAN_POINT('Ctrl Pts',(22.1730081264583,-13.5683460612913,
12.));
#188085=CARTESIAN_POINT('Ctrl Pts',(22.1615922804939,-13.5680170531724,
0.));
#188086=CARTESIAN_POINT('Ctrl Pts',(22.1615922804939,-13.5680170531724,
12.));
#188087=CARTESIAN_POINT('Ctrl Pts',(22.1444897575076,-13.5675054918922,
0.));
#188088=CARTESIAN_POINT('Ctrl Pts',(22.1444897575076,-13.5675054918922,
12.));
#188089=CARTESIAN_POINT('Ctrl Pts',(22.1217288871823,-13.5667873105179,
0.));
#188090=CARTESIAN_POINT('Ctrl Pts',(22.1217288871823,-13.5667873105179,
12.));
#188091=CARTESIAN_POINT('Ctrl Pts',(22.0933486464442,-13.5658294169106,
0.));
#188092=CARTESIAN_POINT('Ctrl Pts',(22.0933486464442,-13.5658294169106,
12.));
#188093=CARTESIAN_POINT('Ctrl Pts',(22.0650393089492,-13.5648113688895,
0.));
#188094=CARTESIAN_POINT('Ctrl Pts',(22.0650393089492,-13.5648113688895,
12.));
#188095=CARTESIAN_POINT('Ctrl Pts',(22.0368009736227,-13.5637332022393,
0.));
#188096=CARTESIAN_POINT('Ctrl Pts',(22.0368009736227,-13.5637332022393,
12.));
#188097=CARTESIAN_POINT('Ctrl Pts',(22.0086337943431,-13.5625949868313,
0.));
#188098=CARTESIAN_POINT('Ctrl Pts',(22.0086337943431,-13.5625949868313,
12.));
#188099=CARTESIAN_POINT('Ctrl Pts',(21.9805379899192,-13.5613968357589,
0.));
#188100=CARTESIAN_POINT('Ctrl Pts',(21.9805379899192,-13.5613968357589,
12.));
#188101=CARTESIAN_POINT('Ctrl Pts',(21.9525138592862,-13.5601389185315,
0.));
#188102=CARTESIAN_POINT('Ctrl Pts',(21.9525138592862,-13.5601389185315,
12.));
#188103=CARTESIAN_POINT('Ctrl Pts',(21.9245617765827,-13.5588214586672,
0.));
#188104=CARTESIAN_POINT('Ctrl Pts',(21.9245617765827,-13.5588214586672,
12.));
#188105=CARTESIAN_POINT('Ctrl Pts',(21.8966821688876,-13.5574447178485,
0.));
#188106=CARTESIAN_POINT('Ctrl Pts',(21.8966821688876,-13.5574447178485,
12.));
#188107=CARTESIAN_POINT('Ctrl Pts',(21.8688754989401,-13.5560089839426,
0.));
#188108=CARTESIAN_POINT('Ctrl Pts',(21.8688754989401,-13.5560089839426,
12.));
#188109=CARTESIAN_POINT('Ctrl Pts',(21.841142245609,-13.5545145573048,0.));
#188110=CARTESIAN_POINT('Ctrl Pts',(21.841142245609,-13.5545145573048,12.));
#188111=CARTESIAN_POINT('Ctrl Pts',(21.8134828857963,-13.5529617381569,
0.));
#188112=CARTESIAN_POINT('Ctrl Pts',(21.8134828857963,-13.5529617381569,
12.));
#188113=CARTESIAN_POINT('Ctrl Pts',(21.7858978745848,-13.5513508127232,
0.));
#188114=CARTESIAN_POINT('Ctrl Pts',(21.7858978745848,-13.5513508127232,
12.));
#188115=CARTESIAN_POINT('Ctrl Pts',(21.7583876294532,-13.5496820422186,
0.));
#188116=CARTESIAN_POINT('Ctrl Pts',(21.7583876294532,-13.5496820422186,
12.));
#188117=CARTESIAN_POINT('Ctrl Pts',(21.730952541226,-13.5479556704457,0.));
#188118=CARTESIAN_POINT('Ctrl Pts',(21.730952541226,-13.5479556704457,12.));
#188119=CARTESIAN_POINT('Ctrl Pts',(21.7035929822939,-13.546171929503,0.));
#188120=CARTESIAN_POINT('Ctrl Pts',(21.7035929822939,-13.546171929503,12.));
#188121=CARTESIAN_POINT('Ctrl Pts',(21.676309315769,-13.5443310461516,0.));
#188122=CARTESIAN_POINT('Ctrl Pts',(21.676309315769,-13.5443310461516,12.));
#188123=CARTESIAN_POINT('Ctrl Pts',(21.6491019044647,-13.5424332480698,
0.));
#188124=CARTESIAN_POINT('Ctrl Pts',(21.6491019044647,-13.5424332480698,
12.));
#188125=CARTESIAN_POINT('Ctrl Pts',(21.6219711193951,-13.5404787697798,
0.));
#188126=CARTESIAN_POINT('Ctrl Pts',(21.6219711193951,-13.5404787697798,
12.));
#188127=CARTESIAN_POINT('Ctrl Pts',(21.5949173499022,-13.5384678597206,
0.));
#188128=CARTESIAN_POINT('Ctrl Pts',(21.5949173499022,-13.5384678597206,
12.));
#188129=CARTESIAN_POINT('Ctrl Pts',(21.5679410019011,-13.5364007790292,
0.));
#188130=CARTESIAN_POINT('Ctrl Pts',(21.5679410019011,-13.5364007790292,
12.));
#188131=CARTESIAN_POINT('Ctrl Pts',(21.5410424932511,-13.5342777983225,
0.));
#188132=CARTESIAN_POINT('Ctrl Pts',(21.5410424932511,-13.5342777983225,
12.));
#188133=CARTESIAN_POINT('Ctrl Pts',(21.5142222501671,-13.5320991952145,
0.));
#188134=CARTESIAN_POINT('Ctrl Pts',(21.5142222501671,-13.5320991952145,
12.));
#188135=CARTESIAN_POINT('Ctrl Pts',(21.487480703047,-13.5298652514357,0.));
#188136=CARTESIAN_POINT('Ctrl Pts',(21.487480703047,-13.5298652514357,12.));
#188137=CARTESIAN_POINT('Ctrl Pts',(21.4608182828695,-13.5275762503553,
0.));
#188138=CARTESIAN_POINT('Ctrl Pts',(21.4608182828695,-13.5275762503553,
12.));
#188139=CARTESIAN_POINT('Ctrl Pts',(21.4342354165254,-13.5252324737795,
0.));
#188140=CARTESIAN_POINT('Ctrl Pts',(21.4342354165254,-13.5252324737795,
12.));
#188141=CARTESIAN_POINT('Ctrl Pts',(21.4077325259318,-13.5228342013508,
0.));
#188142=CARTESIAN_POINT('Ctrl Pts',(21.4077325259318,-13.5228342013508,
12.));
#188143=CARTESIAN_POINT('Ctrl Pts',(21.3813100304967,-13.5203817122497,
0.));
#188144=CARTESIAN_POINT('Ctrl Pts',(21.3813100304967,-13.5203817122497,
12.));
#188145=CARTESIAN_POINT('Ctrl Pts',(21.3549683486219,-13.5178752862461,
0.));
#188146=CARTESIAN_POINT('Ctrl Pts',(21.3549683486219,-13.5178752862461,
12.));
#188147=CARTESIAN_POINT('Ctrl Pts',(21.328707899634,-13.5153152050554,0.));
#188148=CARTESIAN_POINT('Ctrl Pts',(21.328707899634,-13.5153152050554,12.));
#188149=CARTESIAN_POINT('Ctrl Pts',(21.3025291054236,-13.5127017534972,
0.));
#188150=CARTESIAN_POINT('Ctrl Pts',(21.3025291054236,-13.5127017534972,
12.));
#188151=CARTESIAN_POINT('Ctrl Pts',(21.2764323924442,-13.5100352209207,
0.));
#188152=CARTESIAN_POINT('Ctrl Pts',(21.2764323924442,-13.5100352209207,
12.));
#188153=CARTESIAN_POINT('Ctrl Pts',(21.2504181927429,-13.5073159019454,
0.));
#188154=CARTESIAN_POINT('Ctrl Pts',(21.2504181927429,-13.5073159019454,
12.));
#188155=CARTESIAN_POINT('Ctrl Pts',(21.224486942933,-13.5045440957404,0.));
#188156=CARTESIAN_POINT('Ctrl Pts',(21.224486942933,-13.5045440957404,12.));
#188157=CARTESIAN_POINT('Ctrl Pts',(21.1986390835825,-13.5017201056088,
0.));
#188158=CARTESIAN_POINT('Ctrl Pts',(21.1986390835825,-13.5017201056088,
12.));
#188159=CARTESIAN_POINT('Ctrl Pts',(21.1728750584173,-13.4988442384491,
0.));
#188160=CARTESIAN_POINT('Ctrl Pts',(21.1728750584173,-13.4988442384491,
12.));
#188161=CARTESIAN_POINT('Ctrl Pts',(21.1471953136209,-13.4959168042934,
0.));
#188162=CARTESIAN_POINT('Ctrl Pts',(21.1471953136209,-13.4959168042934,
12.));
#188163=CARTESIAN_POINT('Ctrl Pts',(21.1216002970209,-13.4929381157778,
0.));
#188164=CARTESIAN_POINT('Ctrl Pts',(21.1216002970209,-13.4929381157778,
12.));
#188165=CARTESIAN_POINT('Ctrl Pts',(21.0960904575048,-13.4899084877718,
0.));
#188166=CARTESIAN_POINT('Ctrl Pts',(21.0960904575048,-13.4899084877718,
12.));
#188167=CARTESIAN_POINT('Ctrl Pts',(21.0706662455202,-13.4868282377192,
0.));
#188168=CARTESIAN_POINT('Ctrl Pts',(21.0706662455202,-13.4868282377192,
12.));
#188169=CARTESIAN_POINT('Ctrl Pts',(21.0453281134247,-13.4836976858912,
0.));
#188170=CARTESIAN_POINT('Ctrl Pts',(21.0453281134247,-13.4836976858912,
12.));
#188171=CARTESIAN_POINT('Ctrl Pts',(21.0200765158885,-13.4805171556822,
0.));
#188172=CARTESIAN_POINT('Ctrl Pts',(21.0200765158885,-13.4805171556822,
12.));
#188173=CARTESIAN_POINT('Ctrl Pts',(20.9949119102592,-13.4772869738879,
0.));
#188174=CARTESIAN_POINT('Ctrl Pts',(20.9949119102592,-13.4772869738879,
12.));
#188175=CARTESIAN_POINT('Ctrl Pts',(20.9698347569476,-13.4740074710087,
0.));
#188176=CARTESIAN_POINT('Ctrl Pts',(20.9698347569476,-13.4740074710087,
12.));
#188177=CARTESIAN_POINT('Ctrl Pts',(20.9448455197557,-13.4706789815166,
0.));
#188178=CARTESIAN_POINT('Ctrl Pts',(20.9448455197557,-13.4706789815166,
12.));
#188179=CARTESIAN_POINT('Ctrl Pts',(20.9199446657584,-13.4673018437718,
0.));
#188180=CARTESIAN_POINT('Ctrl Pts',(20.9199446657584,-13.4673018437718,
12.));
#188181=CARTESIAN_POINT('Ctrl Pts',(20.8951326652158,-13.4638763999725,
0.));
#188182=CARTESIAN_POINT('Ctrl Pts',(20.8951326652158,-13.4638763999725,
12.));
#188183=CARTESIAN_POINT('Ctrl Pts',(20.8704099914641,-13.4604029960983,
0.));
#188184=CARTESIAN_POINT('Ctrl Pts',(20.8704099914641,-13.4604029960983,
12.));
#188185=CARTESIAN_POINT('Ctrl Pts',(20.8457771208082,-13.4568819818631,
0.));
#188186=CARTESIAN_POINT('Ctrl Pts',(20.8457771208082,-13.4568819818631,
12.));
#188187=CARTESIAN_POINT('Ctrl Pts',(20.821234532398,-13.4533137106667,0.));
#188188=CARTESIAN_POINT('Ctrl Pts',(20.821234532398,-13.4533137106667,12.));
#188189=CARTESIAN_POINT('Ctrl Pts',(20.7967827081227,-13.4496985395637,
0.));
#188190=CARTESIAN_POINT('Ctrl Pts',(20.7967827081227,-13.4496985395637,
12.));
#188191=CARTESIAN_POINT('Ctrl Pts',(20.7724221327608,-13.4460368293688,
0.));
#188192=CARTESIAN_POINT('Ctrl Pts',(20.7724221327608,-13.4460368293688,
12.));
#188193=CARTESIAN_POINT('Ctrl Pts',(20.7481532941013,-13.4423289447561,
0.));
#188194=CARTESIAN_POINT('Ctrl Pts',(20.7481532941013,-13.4423289447561,
12.));
#188195=CARTESIAN_POINT('Ctrl Pts',(20.7239766830675,-13.4385752543663,
0.));
#188196=CARTESIAN_POINT('Ctrl Pts',(20.7239766830675,-13.4385752543663,
12.));
#188197=CARTESIAN_POINT('Ctrl Pts',(20.6998927938288,-13.4347761309154,
0.));
#188198=CARTESIAN_POINT('Ctrl Pts',(20.6998927938288,-13.4347761309154,
12.));
#188199=CARTESIAN_POINT('Ctrl Pts',(20.6759021239103,-13.4309319513119,
0.));
#188200=CARTESIAN_POINT('Ctrl Pts',(20.6759021239103,-13.4309319513119,
12.));
#188201=CARTESIAN_POINT('Ctrl Pts',(20.6520051742869,-13.4270430967651,
0.));
#188202=CARTESIAN_POINT('Ctrl Pts',(20.6520051742869,-13.4270430967651,
12.));
#188203=CARTESIAN_POINT('Ctrl Pts',(20.6282024494237,-13.4231099528179,
0.));
#188204=CARTESIAN_POINT('Ctrl Pts',(20.6282024494237,-13.4231099528179,
12.));
#188205=CARTESIAN_POINT('Ctrl Pts',(20.6044944573153,-13.4191329093933,
0.));
#188206=CARTESIAN_POINT('Ctrl Pts',(20.6044944573153,-13.4191329093933,
12.));
#188207=CARTESIAN_POINT('Ctrl Pts',(20.5808817095155,-13.4151123608411,
0.));
#188208=CARTESIAN_POINT('Ctrl Pts',(20.5808817095155,-13.4151123608411,
12.));
#188209=CARTESIAN_POINT('Ctrl Pts',(20.5573647211639,-13.4110487059912,
0.));
#188210=CARTESIAN_POINT('Ctrl Pts',(20.5573647211639,-13.4110487059912,
12.));
#188211=CARTESIAN_POINT('Ctrl Pts',(20.5339440109956,-13.4069423482076,
0.));
#188212=CARTESIAN_POINT('Ctrl Pts',(20.5339440109956,-13.4069423482076,
12.));
#188213=CARTESIAN_POINT('Ctrl Pts',(20.5106201013753,-13.4027936954529,
0.));
#188214=CARTESIAN_POINT('Ctrl Pts',(20.5106201013753,-13.4027936954529,
12.));
#188215=CARTESIAN_POINT('Ctrl Pts',(20.487393518404,-13.3986031603716,0.));
#188216=CARTESIAN_POINT('Ctrl Pts',(20.487393518404,-13.3986031603716,12.));
#188217=CARTESIAN_POINT('Ctrl Pts',(20.4642647920038,-13.3943711603739,
0.));
#188218=CARTESIAN_POINT('Ctrl Pts',(20.4642647920038,-13.3943711603739,
12.));
#188219=CARTESIAN_POINT('Ctrl Pts',(20.4412344560008,-13.3900981177255,
0.));
#188220=CARTESIAN_POINT('Ctrl Pts',(20.4412344560008,-13.3900981177255,
12.));
#188221=CARTESIAN_POINT('Ctrl Pts',(20.4183030482002,-13.3857844596387,
0.));
#188222=CARTESIAN_POINT('Ctrl Pts',(20.4183030482002,-13.3857844596387,
12.));
#188223=CARTESIAN_POINT('Ctrl Pts',(20.3954711104502,-13.3814306183719,
0.));
#188224=CARTESIAN_POINT('Ctrl Pts',(20.3954711104502,-13.3814306183719,
12.));
#188225=CARTESIAN_POINT('Ctrl Pts',(20.3727391887184,-13.3770370313188,
0.));
#188226=CARTESIAN_POINT('Ctrl Pts',(20.3727391887184,-13.3770370313188,
12.));
#188227=CARTESIAN_POINT('Ctrl Pts',(20.3501078331814,-13.3726041410867,
0.));
#188228=CARTESIAN_POINT('Ctrl Pts',(20.3501078331814,-13.3726041410867,
12.));
#188229=CARTESIAN_POINT('Ctrl Pts',(20.3275775983029,-13.3681323955826,
0.));
#188230=CARTESIAN_POINT('Ctrl Pts',(20.3275775983029,-13.3681323955826,
12.));
#188231=CARTESIAN_POINT('Ctrl Pts',(20.3051490429048,-13.3636222481016,
0.));
#188232=CARTESIAN_POINT('Ctrl Pts',(20.3051490429048,-13.3636222481016,
12.));
#188233=CARTESIAN_POINT('Ctrl Pts',(20.2828227302339,-13.3590741574195,
0.));
#188234=CARTESIAN_POINT('Ctrl Pts',(20.2828227302339,-13.3590741574195,
12.));
#188235=CARTESIAN_POINT('Ctrl Pts',(20.2605992280122,-13.3544885878889,
0.));
#188236=CARTESIAN_POINT('Ctrl Pts',(20.2605992280122,-13.3544885878889,
12.));
#188237=CARTESIAN_POINT('Ctrl Pts',(20.2384791085359,-13.3498660095386,
0.));
#188238=CARTESIAN_POINT('Ctrl Pts',(20.2384791085359,-13.3498660095386,
12.));
#188239=CARTESIAN_POINT('Ctrl Pts',(20.216462948786,-13.3452068981766,0.));
#188240=CARTESIAN_POINT('Ctrl Pts',(20.216462948786,-13.3452068981766,12.));
#188241=CARTESIAN_POINT('Ctrl Pts',(20.1945513305235,-13.3405117354971,
0.));
#188242=CARTESIAN_POINT('Ctrl Pts',(20.1945513305235,-13.3405117354971,
12.));
#188243=CARTESIAN_POINT('Ctrl Pts',(20.1727448403817,-13.3357810091903,
0.));
#188244=CARTESIAN_POINT('Ctrl Pts',(20.1727448403817,-13.3357810091903,
12.));
#188245=CARTESIAN_POINT('Ctrl Pts',(20.1510440699474,-13.3310152130564,
0.));
#188246=CARTESIAN_POINT('Ctrl Pts',(20.1510440699474,-13.3310152130564,
12.));
#188247=CARTESIAN_POINT('Ctrl Pts',(20.1294496158402,-13.3262148471226,
0.));
#188248=CARTESIAN_POINT('Ctrl Pts',(20.1294496158402,-13.3262148471226,
12.));
#188249=CARTESIAN_POINT('Ctrl Pts',(20.1079620798375,-13.3213804177587,
0.));
#188250=CARTESIAN_POINT('Ctrl Pts',(20.1079620798375,-13.3213804177587,
12.));
#188251=CARTESIAN_POINT('Ctrl Pts',(20.0865820689882,-13.3165124377963,
0.));
#188252=CARTESIAN_POINT('Ctrl Pts',(20.0865820689882,-13.3165124377963,
12.));
#188253=CARTESIAN_POINT('Ctrl Pts',(20.0653101957188,-13.3116114266515,
0.));
#188254=CARTESIAN_POINT('Ctrl Pts',(20.0653101957188,-13.3116114266515,
12.));
#188255=CARTESIAN_POINT('Ctrl Pts',(20.0441470779345,-13.3066779104515,
0.));
#188256=CARTESIAN_POINT('Ctrl Pts',(20.0441470779345,-13.3066779104515,
12.));
#188257=CARTESIAN_POINT('Ctrl Pts',(20.0230933391038,-13.3017124221637,
0.));
#188258=CARTESIAN_POINT('Ctrl Pts',(20.0230933391038,-13.3017124221637,
12.));
#188259=CARTESIAN_POINT('Ctrl Pts',(20.0021496083738,-13.2967155017306,
0.));
#188260=CARTESIAN_POINT('Ctrl Pts',(20.0021496083738,-13.2967155017306,
12.));
#188261=CARTESIAN_POINT('Ctrl Pts',(19.981316520717,-13.2916876962094,0.));
#188262=CARTESIAN_POINT('Ctrl Pts',(19.981316520717,-13.2916876962094,12.));
#188263=CARTESIAN_POINT('Ctrl Pts',(19.9605947170586,-13.286629559915,0.));
#188264=CARTESIAN_POINT('Ctrl Pts',(19.9605947170586,-13.286629559915,12.));
#188265=CARTESIAN_POINT('Ctrl Pts',(19.9399848444019,-13.2815416545663,
0.));
#188266=CARTESIAN_POINT('Ctrl Pts',(19.9399848444019,-13.2815416545663,
12.));
#188267=CARTESIAN_POINT('Ctrl Pts',(19.9194875559422,-13.2764245494357,
0.));
#188268=CARTESIAN_POINT('Ctrl Pts',(19.9194875559422,-13.2764245494357,
12.));
#188269=CARTESIAN_POINT('Ctrl Pts',(19.8991035111745,-13.271278821502,0.));
#188270=CARTESIAN_POINT('Ctrl Pts',(19.8991035111745,-13.271278821502,12.));
#188271=CARTESIAN_POINT('Ctrl Pts',(19.8788333760577,-13.2661050556132,
0.));
#188272=CARTESIAN_POINT('Ctrl Pts',(19.8788333760577,-13.2661050556132,
12.));
#188273=CARTESIAN_POINT('Ctrl Pts',(19.8586778231715,-13.2609038446529,
0.));
#188274=CARTESIAN_POINT('Ctrl Pts',(19.8586778231715,-13.2609038446529,
12.));
#188275=CARTESIAN_POINT('Ctrl Pts',(19.8386375318634,-13.2556757897086,
0.));
#188276=CARTESIAN_POINT('Ctrl Pts',(19.8386375318634,-13.2556757897086,
12.));
#188277=CARTESIAN_POINT('Ctrl Pts',(19.8187131883917,-13.2504215002457,
0.));
#188278=CARTESIAN_POINT('Ctrl Pts',(19.8187131883917,-13.2504215002457,
12.));
#188279=CARTESIAN_POINT('Ctrl Pts',(19.7989054860495,-13.2451415942805,
0.));
#188280=CARTESIAN_POINT('Ctrl Pts',(19.7989054860495,-13.2451415942805,
12.));
#188281=CARTESIAN_POINT('Ctrl Pts',(19.7792151253289,-13.2398366985675,
0.));
#188282=CARTESIAN_POINT('Ctrl Pts',(19.7792151253289,-13.2398366985675,
12.));
#188283=CARTESIAN_POINT('Ctrl Pts',(19.7596428141168,-13.2345074487963,
0.));
#188284=CARTESIAN_POINT('Ctrl Pts',(19.7596428141168,-13.2345074487963,
12.));
#188285=CARTESIAN_POINT('Ctrl Pts',(19.7401892678697,-13.2291544897899,
0.));
#188286=CARTESIAN_POINT('Ctrl Pts',(19.7401892678697,-13.2291544897899,
12.));
#188287=CARTESIAN_POINT('Ctrl Pts',(19.7208552097868,-13.2237784757065,
0.));
#188288=CARTESIAN_POINT('Ctrl Pts',(19.7208552097868,-13.2237784757065,
12.));
#188289=CARTESIAN_POINT('Ctrl Pts',(19.7016413709685,-13.2183800702436,
0.));
#188290=CARTESIAN_POINT('Ctrl Pts',(19.7016413709685,-13.2183800702436,
12.));
#188291=CARTESIAN_POINT('Ctrl Pts',(19.6825484905823,-13.2129599468485,
0.));
#188292=CARTESIAN_POINT('Ctrl Pts',(19.6825484905823,-13.2129599468485,
12.));
#188293=CARTESIAN_POINT('Ctrl Pts',(19.6635773160936,-13.2075187889529,
0.));
#188294=CARTESIAN_POINT('Ctrl Pts',(19.6635773160936,-13.2075187889529,
12.));
#188295=CARTESIAN_POINT('Ctrl Pts',(19.6447286034772,-13.2020572902065,
0.));
#188296=CARTESIAN_POINT('Ctrl Pts',(19.6447286034772,-13.2020572902065,
12.));
#188297=CARTESIAN_POINT('Ctrl Pts',(19.6260031174244,-13.1965761547151,
0.));
#188298=CARTESIAN_POINT('Ctrl Pts',(19.6260031174244,-13.1965761547151,
12.));
#188299=CARTESIAN_POINT('Ctrl Pts',(19.6074016315414,-13.1910760972814,
0.));
#188300=CARTESIAN_POINT('Ctrl Pts',(19.6074016315414,-13.1910760972814,
12.));
#188301=CARTESIAN_POINT('Ctrl Pts',(19.5889249285338,-13.1855578436471,
0.));
#188302=CARTESIAN_POINT('Ctrl Pts',(19.5889249285338,-13.1855578436471,
12.));
#188303=CARTESIAN_POINT('Ctrl Pts',(19.5705738004667,-13.1800221307673,
0.));
#188304=CARTESIAN_POINT('Ctrl Pts',(19.5705738004667,-13.1800221307673,
12.));
#188305=CARTESIAN_POINT('Ctrl Pts',(19.5523490490244,-13.1744697070911,
0.));
#188306=CARTESIAN_POINT('Ctrl Pts',(19.5523490490244,-13.1744697070911,
12.));
#188307=CARTESIAN_POINT('Ctrl Pts',(19.5342514857562,-13.168901332843,0.));
#188308=CARTESIAN_POINT('Ctrl Pts',(19.5342514857562,-13.168901332843,12.));
#188309=CARTESIAN_POINT('Ctrl Pts',(19.5162819323213,-13.1633177803101,
0.));
#188310=CARTESIAN_POINT('Ctrl Pts',(19.5162819323213,-13.1633177803101,
12.));
#188311=CARTESIAN_POINT('Ctrl Pts',(19.4984412207082,-13.1577198341245,
0.));
#188312=CARTESIAN_POINT('Ctrl Pts',(19.4984412207082,-13.1577198341245,
12.));
#188313=CARTESIAN_POINT('Ctrl Pts',(19.4807301935268,-13.1521082915853,
0.));
#188314=CARTESIAN_POINT('Ctrl Pts',(19.4807301935268,-13.1521082915853,
12.));
#188315=CARTESIAN_POINT('Ctrl Pts',(19.4631497043258,-13.1464839629971,
0.));
#188316=CARTESIAN_POINT('Ctrl Pts',(19.4631497043258,-13.1464839629971,
12.));
#188317=CARTESIAN_POINT('Ctrl Pts',(19.4457006178876,-13.1408476720061,
0.));
#188318=CARTESIAN_POINT('Ctrl Pts',(19.4457006178876,-13.1408476720061,
12.));
#188319=CARTESIAN_POINT('Ctrl Pts',(19.4283838105262,-13.1352002559438,
0.));
#188320=CARTESIAN_POINT('Ctrl Pts',(19.4283838105262,-13.1352002559438,
12.));
#188321=CARTESIAN_POINT('Ctrl Pts',(19.4112001703557,-13.1295425661634,
0.));
#188322=CARTESIAN_POINT('Ctrl Pts',(19.4112001703557,-13.1295425661634,
12.));
#188323=CARTESIAN_POINT('Ctrl Pts',(19.3941505976263,-13.1238754684177,
0.));
#188324=CARTESIAN_POINT('Ctrl Pts',(19.3941505976263,-13.1238754684177,
12.));
#188325=CARTESIAN_POINT('Ctrl Pts',(19.3772360051091,-13.118199843271,0.));
#188326=CARTESIAN_POINT('Ctrl Pts',(19.3772360051091,-13.118199843271,12.));
#188327=CARTESIAN_POINT('Ctrl Pts',(19.3604573184515,-13.1125165865022,
0.));
#188328=CARTESIAN_POINT('Ctrl Pts',(19.3604573184515,-13.1125165865022,
12.));
#188329=CARTESIAN_POINT('Ctrl Pts',(19.3438154765395,-13.1068266095186,
0.));
#188330=CARTESIAN_POINT('Ctrl Pts',(19.3438154765395,-13.1068266095186,
12.));
#188331=CARTESIAN_POINT('Ctrl Pts',(19.3273114318269,-13.1011308397591,
0.));
#188332=CARTESIAN_POINT('Ctrl Pts',(19.3273114318269,-13.1011308397591,
12.));
#188333=CARTESIAN_POINT('Ctrl Pts',(19.310946150736,-13.0954302211479,0.));
#188334=CARTESIAN_POINT('Ctrl Pts',(19.310946150736,-13.0954302211479,12.));
#188335=CARTESIAN_POINT('Ctrl Pts',(19.2947206141247,-13.0897257145969,
0.));
#188336=CARTESIAN_POINT('Ctrl Pts',(19.2947206141247,-13.0897257145969,
12.));
#188337=CARTESIAN_POINT('Ctrl Pts',(19.2786358177198,-13.0840182984949,
0.));
#188338=CARTESIAN_POINT('Ctrl Pts',(19.2786358177198,-13.0840182984949,
12.));
#188339=CARTESIAN_POINT('Ctrl Pts',(19.2626927725596,-13.0783089692118,
0.));
#188340=CARTESIAN_POINT('Ctrl Pts',(19.2626927725596,-13.0783089692118,
12.));
#188341=CARTESIAN_POINT('Ctrl Pts',(19.2468925053989,-13.0725987415859,
0.));
#188342=CARTESIAN_POINT('Ctrl Pts',(19.2468925053989,-13.0725987415859,
12.));
#188343=CARTESIAN_POINT('Ctrl Pts',(19.2312360592033,-13.0668886494795,
0.));
#188344=CARTESIAN_POINT('Ctrl Pts',(19.2312360592033,-13.0668886494795,
12.));
#188345=CARTESIAN_POINT('Ctrl Pts',(19.2157244937142,-13.0611797463915,
0.));
#188346=CARTESIAN_POINT('Ctrl Pts',(19.2157244937142,-13.0611797463915,
12.));
#188347=CARTESIAN_POINT('Ctrl Pts',(19.2003588859772,-13.0554731060538,
0.));
#188348=CARTESIAN_POINT('Ctrl Pts',(19.2003588859772,-13.0554731060538,
12.));
#188349=CARTESIAN_POINT('Ctrl Pts',(19.1851403308825,-13.0497698230441,
0.));
#188350=CARTESIAN_POINT('Ctrl Pts',(19.1851403308825,-13.0497698230441,
12.));
#188351=CARTESIAN_POINT('Ctrl Pts',(19.1700699416622,-13.0440710133772,
0.));
#188352=CARTESIAN_POINT('Ctrl Pts',(19.1700699416622,-13.0440710133772,
12.));
#188353=CARTESIAN_POINT('Ctrl Pts',(19.155148850523,-13.0383778152068,0.));
#188354=CARTESIAN_POINT('Ctrl Pts',(19.155148850523,-13.0383778152068,12.));
#188355=CARTESIAN_POINT('Ctrl Pts',(19.1403782093386,-13.0326913895838,
0.));
#188356=CARTESIAN_POINT('Ctrl Pts',(19.1403782093386,-13.0326913895838,
12.));
#188357=CARTESIAN_POINT('Ctrl Pts',(19.1257591903099,-13.0270129211976,
0.));
#188358=CARTESIAN_POINT('Ctrl Pts',(19.1257591903099,-13.0270129211976,
12.));
#188359=CARTESIAN_POINT('Ctrl Pts',(19.111292986631,-13.0213436191328,0.));
#188360=CARTESIAN_POINT('Ctrl Pts',(19.111292986631,-13.0213436191328,12.));
#188361=CARTESIAN_POINT('Ctrl Pts',(19.0969808131228,-13.0156847176097,
0.));
#188362=CARTESIAN_POINT('Ctrl Pts',(19.0969808131228,-13.0156847176097,
12.));
#188363=CARTESIAN_POINT('Ctrl Pts',(19.0828239070484,-13.0100374768788,
0.));
#188364=CARTESIAN_POINT('Ctrl Pts',(19.0828239070484,-13.0100374768788,
12.));
#188365=CARTESIAN_POINT('Ctrl Pts',(19.0688235289437,-13.0044031841382,
0.));
#188366=CARTESIAN_POINT('Ctrl Pts',(19.0688235289437,-13.0044031841382,
12.));
#188367=CARTESIAN_POINT('Ctrl Pts',(19.0549809634354,-12.9987831544502,
0.));
#188368=CARTESIAN_POINT('Ctrl Pts',(19.0549809634354,-12.9987831544502,
12.));
#188369=CARTESIAN_POINT('Ctrl Pts',(19.0412975200398,-12.9931787316514,
0.));
#188370=CARTESIAN_POINT('Ctrl Pts',(19.0412975200398,-12.9931787316514,
12.));
#188371=CARTESIAN_POINT('Ctrl Pts',(19.0277745339908,-12.9875912893003,
0.));
#188372=CARTESIAN_POINT('Ctrl Pts',(19.0277745339908,-12.9875912893003,
12.));
#188373=CARTESIAN_POINT('Ctrl Pts',(19.014413367335,-12.9820222318716,0.));
#188374=CARTESIAN_POINT('Ctrl Pts',(19.014413367335,-12.9820222318716,12.));
#188375=CARTESIAN_POINT('Ctrl Pts',(19.0012154099792,-12.9764729959206,
0.));
#188376=CARTESIAN_POINT('Ctrl Pts',(19.0012154099792,-12.9764729959206,
12.));
#188377=CARTESIAN_POINT('Ctrl Pts',(18.9881820807585,-12.9709450512747,
0.));
#188378=CARTESIAN_POINT('Ctrl Pts',(18.9881820807585,-12.9709450512747,
12.));
#188379=CARTESIAN_POINT('Ctrl Pts',(18.9753148284473,-12.9654399021868,
0.));
#188380=CARTESIAN_POINT('Ctrl Pts',(18.9753148284473,-12.9654399021868,
12.));
#188381=CARTESIAN_POINT('Ctrl Pts',(18.9626151329226,-12.9599590886318,
0.));
#188382=CARTESIAN_POINT('Ctrl Pts',(18.9626151329226,-12.9599590886318,
12.));
#188383=CARTESIAN_POINT('Ctrl Pts',(18.9500845064714,-12.9545041877377,
0.));
#188384=CARTESIAN_POINT('Ctrl Pts',(18.9500845064714,-12.9545041877377,
12.));
#188385=CARTESIAN_POINT('Ctrl Pts',(18.9377244950435,-12.9490768151821,
0.));
#188386=CARTESIAN_POINT('Ctrl Pts',(18.9377244950435,-12.9490768151821,
12.));
#188387=CARTESIAN_POINT('Ctrl Pts',(18.9255366795196,-12.9436786266106,
0.));
#188388=CARTESIAN_POINT('Ctrl Pts',(18.9255366795196,-12.9436786266106,
12.));
#188389=CARTESIAN_POINT('Ctrl Pts',(18.9135226769466,-12.9383113190375,
0.));
#188390=CARTESIAN_POINT('Ctrl Pts',(18.9135226769466,-12.9383113190375,
12.));
#188391=CARTESIAN_POINT('Ctrl Pts',(18.9016841423402,-12.9329766328184,
0.));
#188392=CARTESIAN_POINT('Ctrl Pts',(18.9016841423402,-12.9329766328184,
12.));
#188393=CARTESIAN_POINT('Ctrl Pts',(18.8900227704888,-12.9276763536372,
0.));
#188394=CARTESIAN_POINT('Ctrl Pts',(18.8900227704888,-12.9276763536372,
12.));
#188395=CARTESIAN_POINT('Ctrl Pts',(18.8785402977528,-12.9224123144982,
0.));
#188396=CARTESIAN_POINT('Ctrl Pts',(18.8785402977528,-12.9224123144982,
12.));
#188397=CARTESIAN_POINT('Ctrl Pts',(18.8672385038328,-12.9171863977047,
0.));
#188398=CARTESIAN_POINT('Ctrl Pts',(18.8672385038328,-12.9171863977047,
12.));
#188399=CARTESIAN_POINT('Ctrl Pts',(18.8561192136201,-12.9120005369066,
0.));
#188400=CARTESIAN_POINT('Ctrl Pts',(18.8561192136201,-12.9120005369066,
12.));
#188401=CARTESIAN_POINT('Ctrl Pts',(18.8451842990986,-12.9068567191856,
0.));
#188402=CARTESIAN_POINT('Ctrl Pts',(18.8451842990986,-12.9068567191856,
12.));
#188403=CARTESIAN_POINT('Ctrl Pts',(18.834435681259,-12.9017569871738,0.));
#188404=CARTESIAN_POINT('Ctrl Pts',(18.834435681259,-12.9017569871738,12.));
#188405=CARTESIAN_POINT('Ctrl Pts',(18.8238753319124,-12.8967034410752,
0.));
#188406=CARTESIAN_POINT('Ctrl Pts',(18.8238753319124,-12.8967034410752,
12.));
#188407=CARTESIAN_POINT('Ctrl Pts',(18.8135052757815,-12.8916982409931,
0.));
#188408=CARTESIAN_POINT('Ctrl Pts',(18.8135052757815,-12.8916982409931,
12.));
#188409=CARTESIAN_POINT('Ctrl Pts',(18.8033275941939,-12.8867436109543,
0.));
#188410=CARTESIAN_POINT('Ctrl Pts',(18.8033275941939,-12.8867436109543,
12.));
#188411=CARTESIAN_POINT('Ctrl Pts',(18.7933444285867,-12.8818418427474,
0.));
#188412=CARTESIAN_POINT('Ctrl Pts',(18.7933444285867,-12.8818418427474,
12.));
#188413=CARTESIAN_POINT('Ctrl Pts',(18.7835579840481,-12.8769952998097,
0.));
#188414=CARTESIAN_POINT('Ctrl Pts',(18.7835579840481,-12.8769952998097,
12.));
#188415=CARTESIAN_POINT('Ctrl Pts',(18.7739705329028,-12.8722064211814,
0.));
#188416=CARTESIAN_POINT('Ctrl Pts',(18.7739705329028,-12.8722064211814,
12.));
#188417=CARTESIAN_POINT('Ctrl Pts',(18.7645844169568,-12.8674777239656,
0.));
#188418=CARTESIAN_POINT('Ctrl Pts',(18.7645844169568,-12.8674777239656,
12.));
#188419=CARTESIAN_POINT('Ctrl Pts',(18.7554020493888,-12.8628118054172,
0.));
#188420=CARTESIAN_POINT('Ctrl Pts',(18.7554020493888,-12.8628118054172,
12.));
#188421=CARTESIAN_POINT('Ctrl Pts',(18.7464259171248,-12.8582113455644,
0.));
#188422=CARTESIAN_POINT('Ctrl Pts',(18.7464259171248,-12.8582113455644,
12.));
#188423=CARTESIAN_POINT('Ctrl Pts',(18.7376585820851,-12.8536791086315,
0.));
#188424=CARTESIAN_POINT('Ctrl Pts',(18.7376585820851,-12.8536791086315,
12.));
#188425=CARTESIAN_POINT('Ctrl Pts',(18.7291026886552,-12.849217951159,0.));
#188426=CARTESIAN_POINT('Ctrl Pts',(18.7291026886552,-12.849217951159,12.));
#188427=CARTESIAN_POINT('Ctrl Pts',(18.7207609737701,-12.8448308329494,
0.));
#188428=CARTESIAN_POINT('Ctrl Pts',(18.7207609737701,-12.8448308329494,
12.));
#188429=CARTESIAN_POINT('Ctrl Pts',(18.7126362754446,-12.8405208263432,
0.));
#188430=CARTESIAN_POINT('Ctrl Pts',(18.7126362754446,-12.8405208263432,
12.));
#188431=CARTESIAN_POINT('Ctrl Pts',(18.7047315436296,-12.8362911280362,
0.));
#188432=CARTESIAN_POINT('Ctrl Pts',(18.7047315436296,-12.8362911280362,
12.));
#188433=CARTESIAN_POINT('Ctrl Pts',(18.6970498410173,-12.832145059979,0.));
#188434=CARTESIAN_POINT('Ctrl Pts',(18.6970498410173,-12.832145059979,12.));
#188435=CARTESIAN_POINT('Ctrl Pts',(18.6895943376172,-12.8280860635231,
0.));
#188436=CARTESIAN_POINT('Ctrl Pts',(18.6895943376172,-12.8280860635231,
12.));
#188437=CARTESIAN_POINT('Ctrl Pts',(18.6823683094139,-12.8241176980016,
0.));
#188438=CARTESIAN_POINT('Ctrl Pts',(18.6823683094139,-12.8241176980016,
12.));
#188439=CARTESIAN_POINT('Ctrl Pts',(18.6753751301091,-12.8202436318473,
0.));
#188440=CARTESIAN_POINT('Ctrl Pts',(18.6753751301091,-12.8202436318473,
12.));
#188441=CARTESIAN_POINT('Ctrl Pts',(18.6686182952798,-12.8164676687361,
0.));
#188442=CARTESIAN_POINT('Ctrl Pts',(18.6686182952798,-12.8164676687361,
12.));
#188443=CARTESIAN_POINT('Ctrl Pts',(18.6621014624746,-12.8127937909632,
0.));
#188444=CARTESIAN_POINT('Ctrl Pts',(18.6621014624746,-12.8127937909632,
12.));
#188445=CARTESIAN_POINT('Ctrl Pts',(18.6558284825772,-12.8092261933858,
0.));
#188446=CARTESIAN_POINT('Ctrl Pts',(18.6558284825772,-12.8092261933858,
12.));
#188447=CARTESIAN_POINT('Ctrl Pts',(18.6498034438986,-12.805769331162,0.));
#188448=CARTESIAN_POINT('Ctrl Pts',(18.6498034438986,-12.805769331162,12.));
#188449=CARTESIAN_POINT('Ctrl Pts',(18.6440306327457,-12.8024278770153,
0.));
#188450=CARTESIAN_POINT('Ctrl Pts',(18.6440306327457,-12.8024278770153,
12.));
#188451=CARTESIAN_POINT('Ctrl Pts',(18.63851447924,-12.7992066625264,0.));
#188452=CARTESIAN_POINT('Ctrl Pts',(18.63851447924,-12.7992066625264,12.));
#188453=CARTESIAN_POINT('Ctrl Pts',(18.6332595057005,-12.7961106222251,
0.));
#188454=CARTESIAN_POINT('Ctrl Pts',(18.6332595057005,-12.7961106222251,
12.));
#188455=CARTESIAN_POINT('Ctrl Pts',(18.6282702819371,-12.7931447451556,
0.));
#188456=CARTESIAN_POINT('Ctrl Pts',(18.6282702819371,-12.7931447451556,
12.));
#188457=CARTESIAN_POINT('Ctrl Pts',(18.6235516265575,-12.7903142925234,
0.));
#188458=CARTESIAN_POINT('Ctrl Pts',(18.6235516265575,-12.7903142925234,
12.));
#188459=CARTESIAN_POINT('Ctrl Pts',(18.6191087624752,-12.7876249657834,
0.));
#188460=CARTESIAN_POINT('Ctrl Pts',(18.6191087624752,-12.7876249657834,
12.));
#188461=CARTESIAN_POINT('Ctrl Pts',(18.6149475565189,-12.78508316579,0.));
#188462=CARTESIAN_POINT('Ctrl Pts',(18.6149475565189,-12.78508316579,12.));
#188463=CARTESIAN_POINT('Ctrl Pts',(18.611074482622,-12.7826959526924,0.));
#188464=CARTESIAN_POINT('Ctrl Pts',(18.611074482622,-12.7826959526924,12.));
#188465=CARTESIAN_POINT('Ctrl Pts',(18.6074961535723,-12.7804705387658,
0.));
#188466=CARTESIAN_POINT('Ctrl Pts',(18.6074961535723,-12.7804705387658,
12.));
#188467=CARTESIAN_POINT('Ctrl Pts',(18.6042190183703,-12.7784139605067,
0.));
#188468=CARTESIAN_POINT('Ctrl Pts',(18.6042190183703,-12.7784139605067,
12.));
#188469=CARTESIAN_POINT('Ctrl Pts',(18.6012488486708,-12.7765325225082,
0.));
#188470=CARTESIAN_POINT('Ctrl Pts',(18.6012488486708,-12.7765325225082,
12.));
#188471=CARTESIAN_POINT('Ctrl Pts',(18.5985917525949,-12.7748328937639,
0.));
#188472=CARTESIAN_POINT('Ctrl Pts',(18.5985917525949,-12.7748328937639,
12.));
#188473=CARTESIAN_POINT('Ctrl Pts',(18.5962551167772,-12.7733231262107,
0.));
#188474=CARTESIAN_POINT('Ctrl Pts',(18.5962551167772,-12.7733231262107,
12.));
#188475=CARTESIAN_POINT('Ctrl Pts',(18.5942490615409,-12.7720142287169,
0.));
#188476=CARTESIAN_POINT('Ctrl Pts',(18.5942490615409,-12.7720142287169,
12.));
#188477=CARTESIAN_POINT('Ctrl Pts',(18.5925859134582,-12.7709195951153,
0.));
#188478=CARTESIAN_POINT('Ctrl Pts',(18.5925859134582,-12.7709195951153,
12.));
#188479=CARTESIAN_POINT('Ctrl Pts',(18.5912775137806,-12.7700520897174,
0.));
#188480=CARTESIAN_POINT('Ctrl Pts',(18.5912775137806,-12.7700520897174,
12.));
#188481=CARTESIAN_POINT('Ctrl Pts',(18.590332877722,-12.7694215127923,0.));
#188482=CARTESIAN_POINT('Ctrl Pts',(18.590332877722,-12.7694215127923,12.));
#188483=CARTESIAN_POINT('Ctrl Pts',(18.589871621842,-12.7691103481996,0.));
#188484=CARTESIAN_POINT('Ctrl Pts',(18.589871621842,-12.7691103481996,12.));
#188485=CARTESIAN_POINT('Ctrl Pts',(18.5896919669158,-12.7689864266924,
0.));
#188486=CARTESIAN_POINT('Ctrl Pts',(18.5896919669158,-12.7689864266924,
12.));
#188487=CARTESIAN_POINT('Ctrl Pts',(18.5896460962961,-12.7689524524484,
0.));
#188488=CARTESIAN_POINT('Ctrl Pts',(18.5896460962961,-12.7689524524484,
12.));
#188489=CARTESIAN_POINT('Ctrl Pts',(18.5896416359912,-12.7689476255363,
0.));
#188490=CARTESIAN_POINT('Ctrl Pts',(18.5896416359912,-12.7689476255363,
12.));
#188491=CARTESIAN_POINT('',(22.1787195904339,-13.5685075571671,0.));
#188492=CARTESIAN_POINT('Ctrl Pts',(22.1787195904339,-13.5685075571671,
0.));
#188493=CARTESIAN_POINT('Ctrl Pts',(22.1730081264583,-13.5683460612913,
0.));
#188494=CARTESIAN_POINT('Ctrl Pts',(22.1615922804939,-13.5680170531724,
0.));
#188495=CARTESIAN_POINT('Ctrl Pts',(22.1444897575076,-13.5675054918922,
0.));
#188496=CARTESIAN_POINT('Ctrl Pts',(22.1217288871823,-13.5667873105179,
0.));
#188497=CARTESIAN_POINT('Ctrl Pts',(22.0933486464442,-13.5658294169106,
0.));
#188498=CARTESIAN_POINT('Ctrl Pts',(22.0650393089492,-13.5648113688895,
0.));
#188499=CARTESIAN_POINT('Ctrl Pts',(22.0368009736227,-13.5637332022393,
0.));
#188500=CARTESIAN_POINT('Ctrl Pts',(22.0086337943431,-13.5625949868313,
0.));
#188501=CARTESIAN_POINT('Ctrl Pts',(21.9805379899192,-13.5613968357589,
0.));
#188502=CARTESIAN_POINT('Ctrl Pts',(21.9525138592862,-13.5601389185315,
0.));
#188503=CARTESIAN_POINT('Ctrl Pts',(21.9245617765827,-13.5588214586672,
0.));
#188504=CARTESIAN_POINT('Ctrl Pts',(21.8966821688876,-13.5574447178485,
0.));
#188505=CARTESIAN_POINT('Ctrl Pts',(21.8688754989401,-13.5560089839426,
0.));
#188506=CARTESIAN_POINT('Ctrl Pts',(21.841142245609,-13.5545145573048,0.));
#188507=CARTESIAN_POINT('Ctrl Pts',(21.8134828857963,-13.5529617381569,
0.));
#188508=CARTESIAN_POINT('Ctrl Pts',(21.7858978745848,-13.5513508127232,
0.));
#188509=CARTESIAN_POINT('Ctrl Pts',(21.7583876294532,-13.5496820422186,
0.));
#188510=CARTESIAN_POINT('Ctrl Pts',(21.730952541226,-13.5479556704457,0.));
#188511=CARTESIAN_POINT('Ctrl Pts',(21.7035929822939,-13.546171929503,0.));
#188512=CARTESIAN_POINT('Ctrl Pts',(21.676309315769,-13.5443310461516,0.));
#188513=CARTESIAN_POINT('Ctrl Pts',(21.6491019044647,-13.5424332480698,
0.));
#188514=CARTESIAN_POINT('Ctrl Pts',(21.6219711193951,-13.5404787697798,
0.));
#188515=CARTESIAN_POINT('Ctrl Pts',(21.5949173499022,-13.5384678597206,
0.));
#188516=CARTESIAN_POINT('Ctrl Pts',(21.5679410019011,-13.5364007790292,
0.));
#188517=CARTESIAN_POINT('Ctrl Pts',(21.5410424932511,-13.5342777983225,
0.));
#188518=CARTESIAN_POINT('Ctrl Pts',(21.5142222501671,-13.5320991952145,
0.));
#188519=CARTESIAN_POINT('Ctrl Pts',(21.487480703047,-13.5298652514357,0.));
#188520=CARTESIAN_POINT('Ctrl Pts',(21.4608182828695,-13.5275762503553,
0.));
#188521=CARTESIAN_POINT('Ctrl Pts',(21.4342354165254,-13.5252324737795,
0.));
#188522=CARTESIAN_POINT('Ctrl Pts',(21.4077325259318,-13.5228342013508,
0.));
#188523=CARTESIAN_POINT('Ctrl Pts',(21.3813100304967,-13.5203817122497,
0.));
#188524=CARTESIAN_POINT('Ctrl Pts',(21.3549683486219,-13.5178752862461,
0.));
#188525=CARTESIAN_POINT('Ctrl Pts',(21.328707899634,-13.5153152050554,0.));
#188526=CARTESIAN_POINT('Ctrl Pts',(21.3025291054236,-13.5127017534972,
0.));
#188527=CARTESIAN_POINT('Ctrl Pts',(21.2764323924442,-13.5100352209207,
0.));
#188528=CARTESIAN_POINT('Ctrl Pts',(21.2504181927429,-13.5073159019454,
0.));
#188529=CARTESIAN_POINT('Ctrl Pts',(21.224486942933,-13.5045440957404,0.));
#188530=CARTESIAN_POINT('Ctrl Pts',(21.1986390835825,-13.5017201056088,
0.));
#188531=CARTESIAN_POINT('Ctrl Pts',(21.1728750584173,-13.4988442384491,
0.));
#188532=CARTESIAN_POINT('Ctrl Pts',(21.1471953136209,-13.4959168042934,
0.));
#188533=CARTESIAN_POINT('Ctrl Pts',(21.1216002970209,-13.4929381157778,
0.));
#188534=CARTESIAN_POINT('Ctrl Pts',(21.0960904575048,-13.4899084877718,
0.));
#188535=CARTESIAN_POINT('Ctrl Pts',(21.0706662455202,-13.4868282377192,
0.));
#188536=CARTESIAN_POINT('Ctrl Pts',(21.0453281134247,-13.4836976858912,
0.));
#188537=CARTESIAN_POINT('Ctrl Pts',(21.0200765158885,-13.4805171556822,
0.));
#188538=CARTESIAN_POINT('Ctrl Pts',(20.9949119102592,-13.4772869738879,
0.));
#188539=CARTESIAN_POINT('Ctrl Pts',(20.9698347569476,-13.4740074710087,
0.));
#188540=CARTESIAN_POINT('Ctrl Pts',(20.9448455197557,-13.4706789815166,
0.));
#188541=CARTESIAN_POINT('Ctrl Pts',(20.9199446657584,-13.4673018437718,
0.));
#188542=CARTESIAN_POINT('Ctrl Pts',(20.8951326652158,-13.4638763999725,
0.));
#188543=CARTESIAN_POINT('Ctrl Pts',(20.8704099914641,-13.4604029960983,
0.));
#188544=CARTESIAN_POINT('Ctrl Pts',(20.8457771208082,-13.4568819818631,
0.));
#188545=CARTESIAN_POINT('Ctrl Pts',(20.821234532398,-13.4533137106667,0.));
#188546=CARTESIAN_POINT('Ctrl Pts',(20.7967827081227,-13.4496985395637,
0.));
#188547=CARTESIAN_POINT('Ctrl Pts',(20.7724221327608,-13.4460368293688,
0.));
#188548=CARTESIAN_POINT('Ctrl Pts',(20.7481532941013,-13.4423289447561,
0.));
#188549=CARTESIAN_POINT('Ctrl Pts',(20.7239766830675,-13.4385752543663,
0.));
#188550=CARTESIAN_POINT('Ctrl Pts',(20.6998927938288,-13.4347761309154,
0.));
#188551=CARTESIAN_POINT('Ctrl Pts',(20.6759021239103,-13.4309319513119,
0.));
#188552=CARTESIAN_POINT('Ctrl Pts',(20.6520051742869,-13.4270430967651,
0.));
#188553=CARTESIAN_POINT('Ctrl Pts',(20.6282024494237,-13.4231099528179,
0.));
#188554=CARTESIAN_POINT('Ctrl Pts',(20.6044944573153,-13.4191329093933,
0.));
#188555=CARTESIAN_POINT('Ctrl Pts',(20.5808817095155,-13.4151123608411,
0.));
#188556=CARTESIAN_POINT('Ctrl Pts',(20.5573647211639,-13.4110487059912,
0.));
#188557=CARTESIAN_POINT('Ctrl Pts',(20.5339440109956,-13.4069423482076,
0.));
#188558=CARTESIAN_POINT('Ctrl Pts',(20.5106201013753,-13.4027936954529,
0.));
#188559=CARTESIAN_POINT('Ctrl Pts',(20.487393518404,-13.3986031603716,0.));
#188560=CARTESIAN_POINT('Ctrl Pts',(20.4642647920038,-13.3943711603739,
0.));
#188561=CARTESIAN_POINT('Ctrl Pts',(20.4412344560008,-13.3900981177255,
0.));
#188562=CARTESIAN_POINT('Ctrl Pts',(20.4183030482002,-13.3857844596387,
0.));
#188563=CARTESIAN_POINT('Ctrl Pts',(20.3954711104502,-13.3814306183719,
0.));
#188564=CARTESIAN_POINT('Ctrl Pts',(20.3727391887184,-13.3770370313188,
0.));
#188565=CARTESIAN_POINT('Ctrl Pts',(20.3501078331814,-13.3726041410867,
0.));
#188566=CARTESIAN_POINT('Ctrl Pts',(20.3275775983029,-13.3681323955826,
0.));
#188567=CARTESIAN_POINT('Ctrl Pts',(20.3051490429048,-13.3636222481016,
0.));
#188568=CARTESIAN_POINT('Ctrl Pts',(20.2828227302339,-13.3590741574195,
0.));
#188569=CARTESIAN_POINT('Ctrl Pts',(20.2605992280122,-13.3544885878889,
0.));
#188570=CARTESIAN_POINT('Ctrl Pts',(20.2384791085359,-13.3498660095386,
0.));
#188571=CARTESIAN_POINT('Ctrl Pts',(20.216462948786,-13.3452068981766,0.));
#188572=CARTESIAN_POINT('Ctrl Pts',(20.1945513305235,-13.3405117354971,
0.));
#188573=CARTESIAN_POINT('Ctrl Pts',(20.1727448403817,-13.3357810091903,
0.));
#188574=CARTESIAN_POINT('Ctrl Pts',(20.1510440699474,-13.3310152130564,
0.));
#188575=CARTESIAN_POINT('Ctrl Pts',(20.1294496158402,-13.3262148471226,
0.));
#188576=CARTESIAN_POINT('Ctrl Pts',(20.1079620798375,-13.3213804177587,
0.));
#188577=CARTESIAN_POINT('Ctrl Pts',(20.0865820689882,-13.3165124377963,
0.));
#188578=CARTESIAN_POINT('Ctrl Pts',(20.0653101957188,-13.3116114266515,
0.));
#188579=CARTESIAN_POINT('Ctrl Pts',(20.0441470779345,-13.3066779104515,
0.));
#188580=CARTESIAN_POINT('Ctrl Pts',(20.0230933391038,-13.3017124221637,
0.));
#188581=CARTESIAN_POINT('Ctrl Pts',(20.0021496083738,-13.2967155017306,
0.));
#188582=CARTESIAN_POINT('Ctrl Pts',(19.981316520717,-13.2916876962094,0.));
#188583=CARTESIAN_POINT('Ctrl Pts',(19.9605947170586,-13.286629559915,0.));
#188584=CARTESIAN_POINT('Ctrl Pts',(19.9399848444019,-13.2815416545663,
0.));
#188585=CARTESIAN_POINT('Ctrl Pts',(19.9194875559422,-13.2764245494357,
0.));
#188586=CARTESIAN_POINT('Ctrl Pts',(19.8991035111745,-13.271278821502,0.));
#188587=CARTESIAN_POINT('Ctrl Pts',(19.8788333760577,-13.2661050556132,
0.));
#188588=CARTESIAN_POINT('Ctrl Pts',(19.8586778231715,-13.2609038446529,
0.));
#188589=CARTESIAN_POINT('Ctrl Pts',(19.8386375318634,-13.2556757897086,
0.));
#188590=CARTESIAN_POINT('Ctrl Pts',(19.8187131883917,-13.2504215002457,
0.));
#188591=CARTESIAN_POINT('Ctrl Pts',(19.7989054860495,-13.2451415942805,
0.));
#188592=CARTESIAN_POINT('Ctrl Pts',(19.7792151253289,-13.2398366985675,
0.));
#188593=CARTESIAN_POINT('Ctrl Pts',(19.7596428141168,-13.2345074487963,
0.));
#188594=CARTESIAN_POINT('Ctrl Pts',(19.7401892678697,-13.2291544897899,
0.));
#188595=CARTESIAN_POINT('Ctrl Pts',(19.7208552097868,-13.2237784757065,
0.));
#188596=CARTESIAN_POINT('Ctrl Pts',(19.7016413709685,-13.2183800702436,
0.));
#188597=CARTESIAN_POINT('Ctrl Pts',(19.6825484905823,-13.2129599468485,
0.));
#188598=CARTESIAN_POINT('Ctrl Pts',(19.6635773160936,-13.2075187889529,
0.));
#188599=CARTESIAN_POINT('Ctrl Pts',(19.6447286034772,-13.2020572902065,
0.));
#188600=CARTESIAN_POINT('Ctrl Pts',(19.6260031174244,-13.1965761547151,
0.));
#188601=CARTESIAN_POINT('Ctrl Pts',(19.6074016315414,-13.1910760972814,
0.));
#188602=CARTESIAN_POINT('Ctrl Pts',(19.5889249285338,-13.1855578436471,
0.));
#188603=CARTESIAN_POINT('Ctrl Pts',(19.5705738004667,-13.1800221307673,
0.));
#188604=CARTESIAN_POINT('Ctrl Pts',(19.5523490490244,-13.1744697070911,
0.));
#188605=CARTESIAN_POINT('Ctrl Pts',(19.5342514857562,-13.168901332843,0.));
#188606=CARTESIAN_POINT('Ctrl Pts',(19.5162819323213,-13.1633177803101,
0.));
#188607=CARTESIAN_POINT('Ctrl Pts',(19.4984412207082,-13.1577198341245,
0.));
#188608=CARTESIAN_POINT('Ctrl Pts',(19.4807301935268,-13.1521082915853,
0.));
#188609=CARTESIAN_POINT('Ctrl Pts',(19.4631497043258,-13.1464839629971,
0.));
#188610=CARTESIAN_POINT('Ctrl Pts',(19.4457006178876,-13.1408476720061,
0.));
#188611=CARTESIAN_POINT('Ctrl Pts',(19.4283838105262,-13.1352002559438,
0.));
#188612=CARTESIAN_POINT('Ctrl Pts',(19.4112001703557,-13.1295425661634,
0.));
#188613=CARTESIAN_POINT('Ctrl Pts',(19.3941505976263,-13.1238754684177,
0.));
#188614=CARTESIAN_POINT('Ctrl Pts',(19.3772360051091,-13.118199843271,0.));
#188615=CARTESIAN_POINT('Ctrl Pts',(19.3604573184515,-13.1125165865022,
0.));
#188616=CARTESIAN_POINT('Ctrl Pts',(19.3438154765395,-13.1068266095186,
0.));
#188617=CARTESIAN_POINT('Ctrl Pts',(19.3273114318269,-13.1011308397591,
0.));
#188618=CARTESIAN_POINT('Ctrl Pts',(19.310946150736,-13.0954302211479,0.));
#188619=CARTESIAN_POINT('Ctrl Pts',(19.2947206141247,-13.0897257145969,
0.));
#188620=CARTESIAN_POINT('Ctrl Pts',(19.2786358177198,-13.0840182984949,
0.));
#188621=CARTESIAN_POINT('Ctrl Pts',(19.2626927725596,-13.0783089692118,
0.));
#188622=CARTESIAN_POINT('Ctrl Pts',(19.2468925053989,-13.0725987415859,
0.));
#188623=CARTESIAN_POINT('Ctrl Pts',(19.2312360592033,-13.0668886494795,
0.));
#188624=CARTESIAN_POINT('Ctrl Pts',(19.2157244937142,-13.0611797463915,
0.));
#188625=CARTESIAN_POINT('Ctrl Pts',(19.2003588859772,-13.0554731060538,
0.));
#188626=CARTESIAN_POINT('Ctrl Pts',(19.1851403308825,-13.0497698230441,
0.));
#188627=CARTESIAN_POINT('Ctrl Pts',(19.1700699416622,-13.0440710133772,
0.));
#188628=CARTESIAN_POINT('Ctrl Pts',(19.155148850523,-13.0383778152068,0.));
#188629=CARTESIAN_POINT('Ctrl Pts',(19.1403782093386,-13.0326913895838,
0.));
#188630=CARTESIAN_POINT('Ctrl Pts',(19.1257591903099,-13.0270129211976,
0.));
#188631=CARTESIAN_POINT('Ctrl Pts',(19.111292986631,-13.0213436191328,0.));
#188632=CARTESIAN_POINT('Ctrl Pts',(19.0969808131228,-13.0156847176097,
0.));
#188633=CARTESIAN_POINT('Ctrl Pts',(19.0828239070484,-13.0100374768788,
0.));
#188634=CARTESIAN_POINT('Ctrl Pts',(19.0688235289437,-13.0044031841382,
0.));
#188635=CARTESIAN_POINT('Ctrl Pts',(19.0549809634354,-12.9987831544502,
0.));
#188636=CARTESIAN_POINT('Ctrl Pts',(19.0412975200398,-12.9931787316514,
0.));
#188637=CARTESIAN_POINT('Ctrl Pts',(19.0277745339908,-12.9875912893003,
0.));
#188638=CARTESIAN_POINT('Ctrl Pts',(19.014413367335,-12.9820222318716,0.));
#188639=CARTESIAN_POINT('Ctrl Pts',(19.0012154099792,-12.9764729959206,
0.));
#188640=CARTESIAN_POINT('Ctrl Pts',(18.9881820807585,-12.9709450512747,
0.));
#188641=CARTESIAN_POINT('Ctrl Pts',(18.9753148284473,-12.9654399021868,
0.));
#188642=CARTESIAN_POINT('Ctrl Pts',(18.9626151329226,-12.9599590886318,
0.));
#188643=CARTESIAN_POINT('Ctrl Pts',(18.9500845064714,-12.9545041877377,
0.));
#188644=CARTESIAN_POINT('Ctrl Pts',(18.9377244950435,-12.9490768151821,
0.));
#188645=CARTESIAN_POINT('Ctrl Pts',(18.9255366795196,-12.9436786266106,
0.));
#188646=CARTESIAN_POINT('Ctrl Pts',(18.9135226769466,-12.9383113190375,
0.));
#188647=CARTESIAN_POINT('Ctrl Pts',(18.9016841423402,-12.9329766328184,
0.));
#188648=CARTESIAN_POINT('Ctrl Pts',(18.8900227704888,-12.9276763536372,
0.));
#188649=CARTESIAN_POINT('Ctrl Pts',(18.8785402977528,-12.9224123144982,
0.));
#188650=CARTESIAN_POINT('Ctrl Pts',(18.8672385038328,-12.9171863977047,
0.));
#188651=CARTESIAN_POINT('Ctrl Pts',(18.8561192136201,-12.9120005369066,
0.));
#188652=CARTESIAN_POINT('Ctrl Pts',(18.8451842990986,-12.9068567191856,
0.));
#188653=CARTESIAN_POINT('Ctrl Pts',(18.834435681259,-12.9017569871738,0.));
#188654=CARTESIAN_POINT('Ctrl Pts',(18.8238753319124,-12.8967034410752,
0.));
#188655=CARTESIAN_POINT('Ctrl Pts',(18.8135052757815,-12.8916982409931,
0.));
#188656=CARTESIAN_POINT('Ctrl Pts',(18.8033275941939,-12.8867436109543,
0.));
#188657=CARTESIAN_POINT('Ctrl Pts',(18.7933444285867,-12.8818418427474,
0.));
#188658=CARTESIAN_POINT('Ctrl Pts',(18.7835579840481,-12.8769952998097,
0.));
#188659=CARTESIAN_POINT('Ctrl Pts',(18.7739705329028,-12.8722064211814,
0.));
#188660=CARTESIAN_POINT('Ctrl Pts',(18.7645844169568,-12.8674777239656,
0.));
#188661=CARTESIAN_POINT('Ctrl Pts',(18.7554020493888,-12.8628118054172,
0.));
#188662=CARTESIAN_POINT('Ctrl Pts',(18.7464259171248,-12.8582113455644,
0.));
#188663=CARTESIAN_POINT('Ctrl Pts',(18.7376585820851,-12.8536791086315,
0.));
#188664=CARTESIAN_POINT('Ctrl Pts',(18.7291026886552,-12.849217951159,0.));
#188665=CARTESIAN_POINT('Ctrl Pts',(18.7207609737701,-12.8448308329494,
0.));
#188666=CARTESIAN_POINT('Ctrl Pts',(18.7126362754446,-12.8405208263432,
0.));
#188667=CARTESIAN_POINT('Ctrl Pts',(18.7047315436296,-12.8362911280362,
0.));
#188668=CARTESIAN_POINT('Ctrl Pts',(18.6970498410173,-12.832145059979,0.));
#188669=CARTESIAN_POINT('Ctrl Pts',(18.6895943376172,-12.8280860635231,
0.));
#188670=CARTESIAN_POINT('Ctrl Pts',(18.6823683094139,-12.8241176980016,
0.));
#188671=CARTESIAN_POINT('Ctrl Pts',(18.6753751301091,-12.8202436318473,
0.));
#188672=CARTESIAN_POINT('Ctrl Pts',(18.6686182952798,-12.8164676687361,
0.));
#188673=CARTESIAN_POINT('Ctrl Pts',(18.6621014624746,-12.8127937909632,
0.));
#188674=CARTESIAN_POINT('Ctrl Pts',(18.6558284825772,-12.8092261933858,
0.));
#188675=CARTESIAN_POINT('Ctrl Pts',(18.6498034438986,-12.805769331162,0.));
#188676=CARTESIAN_POINT('Ctrl Pts',(18.6440306327457,-12.8024278770153,
0.));
#188677=CARTESIAN_POINT('Ctrl Pts',(18.63851447924,-12.7992066625264,0.));
#188678=CARTESIAN_POINT('Ctrl Pts',(18.6332595057005,-12.7961106222251,
0.));
#188679=CARTESIAN_POINT('Ctrl Pts',(18.6282702819371,-12.7931447451556,
0.));
#188680=CARTESIAN_POINT('Ctrl Pts',(18.6235516265575,-12.7903142925234,
0.));
#188681=CARTESIAN_POINT('Ctrl Pts',(18.6191087624752,-12.7876249657834,
0.));
#188682=CARTESIAN_POINT('Ctrl Pts',(18.6149475565189,-12.78508316579,0.));
#188683=CARTESIAN_POINT('Ctrl Pts',(18.611074482622,-12.7826959526924,0.));
#188684=CARTESIAN_POINT('Ctrl Pts',(18.6074961535723,-12.7804705387658,
0.));
#188685=CARTESIAN_POINT('Ctrl Pts',(18.6042190183703,-12.7784139605067,
0.));
#188686=CARTESIAN_POINT('Ctrl Pts',(18.6012488486708,-12.7765325225082,
0.));
#188687=CARTESIAN_POINT('Ctrl Pts',(18.5985917525949,-12.7748328937639,
0.));
#188688=CARTESIAN_POINT('Ctrl Pts',(18.5962551167772,-12.7733231262107,
0.));
#188689=CARTESIAN_POINT('Ctrl Pts',(18.5942490615409,-12.7720142287169,
0.));
#188690=CARTESIAN_POINT('Ctrl Pts',(18.5925859134582,-12.7709195951153,
0.));
#188691=CARTESIAN_POINT('Ctrl Pts',(18.5912775137806,-12.7700520897174,
0.));
#188692=CARTESIAN_POINT('Ctrl Pts',(18.590332877722,-12.7694215127923,0.));
#188693=CARTESIAN_POINT('Ctrl Pts',(18.589871621842,-12.7691103481996,0.));
#188694=CARTESIAN_POINT('Ctrl Pts',(18.5896919669158,-12.7689864266924,
0.));
#188695=CARTESIAN_POINT('Ctrl Pts',(18.5896460962961,-12.7689524524484,
0.));
#188696=CARTESIAN_POINT('Ctrl Pts',(18.5896416359912,-12.7689476255363,
0.));
#188697=CARTESIAN_POINT('',(22.1787195904339,-13.5685075571671,0.));
#188698=CARTESIAN_POINT('Ctrl Pts',(17.1452095830632,-14.6513681262571,
0.));
#188699=CARTESIAN_POINT('Ctrl Pts',(17.1452095830632,-14.6513681262571,
12.));
#188700=CARTESIAN_POINT('Ctrl Pts',(17.1452153999142,-14.6513711852843,
0.));
#188701=CARTESIAN_POINT('Ctrl Pts',(17.1452153999142,-14.6513711852843,
12.));
#188702=CARTESIAN_POINT('Ctrl Pts',(17.1452600887037,-14.6514066997196,
0.));
#188703=CARTESIAN_POINT('Ctrl Pts',(17.1452600887037,-14.6514066997196,
12.));
#188704=CARTESIAN_POINT('Ctrl Pts',(17.1454262858043,-14.6515481598068,
0.));
#188705=CARTESIAN_POINT('Ctrl Pts',(17.1454262858043,-14.6515481598068,
12.));
#188706=CARTESIAN_POINT('Ctrl Pts',(17.1458462295271,-14.6519131634508,
0.));
#188707=CARTESIAN_POINT('Ctrl Pts',(17.1458462295271,-14.6519131634508,
12.));
#188708=CARTESIAN_POINT('Ctrl Pts',(17.1466998098673,-14.6526624064978,
0.));
#188709=CARTESIAN_POINT('Ctrl Pts',(17.1466998098673,-14.6526624064978,
12.));
#188710=CARTESIAN_POINT('Ctrl Pts',(17.147876394491,-14.6537016966184,0.));
#188711=CARTESIAN_POINT('Ctrl Pts',(17.147876394491,-14.6537016966184,12.));
#188712=CARTESIAN_POINT('Ctrl Pts',(17.1493641837558,-14.655024862281,0.));
#188713=CARTESIAN_POINT('Ctrl Pts',(17.1493641837558,-14.655024862281,12.));
#188714=CARTESIAN_POINT('Ctrl Pts',(17.1511476869496,-14.6566237952435,
0.));
#188715=CARTESIAN_POINT('Ctrl Pts',(17.1511476869496,-14.6566237952435,
12.));
#188716=CARTESIAN_POINT('Ctrl Pts',(17.1532107762718,-14.6584900555302,
0.));
#188717=CARTESIAN_POINT('Ctrl Pts',(17.1532107762718,-14.6584900555302,
12.));
#188718=CARTESIAN_POINT('Ctrl Pts',(17.1555401986401,-14.6606167169642,
0.));
#188719=CARTESIAN_POINT('Ctrl Pts',(17.1555401986401,-14.6606167169642,
12.));
#188720=CARTESIAN_POINT('Ctrl Pts',(17.1581262646789,-14.6629987285992,
0.));
#188721=CARTESIAN_POINT('Ctrl Pts',(17.1581262646789,-14.6629987285992,
12.));
#188722=CARTESIAN_POINT('Ctrl Pts',(17.1609609517369,-14.6656319165057,
0.));
#188723=CARTESIAN_POINT('Ctrl Pts',(17.1609609517369,-14.6656319165057,
12.));
#188724=CARTESIAN_POINT('Ctrl Pts',(17.1640366762305,-14.6685123374423,
0.));
#188725=CARTESIAN_POINT('Ctrl Pts',(17.1640366762305,-14.6685123374423,
12.));
#188726=CARTESIAN_POINT('Ctrl Pts',(17.167344972302,-14.671635583332,0.));
#188727=CARTESIAN_POINT('Ctrl Pts',(17.167344972302,-14.671635583332,12.));
#188728=CARTESIAN_POINT('Ctrl Pts',(17.1708771619129,-14.6749971333867,
0.));
#188729=CARTESIAN_POINT('Ctrl Pts',(17.1708771619129,-14.6749971333867,
12.));
#188730=CARTESIAN_POINT('Ctrl Pts',(17.1746247499057,-14.6785925615677,
0.));
#188731=CARTESIAN_POINT('Ctrl Pts',(17.1746247499057,-14.6785925615677,
12.));
#188732=CARTESIAN_POINT('Ctrl Pts',(17.1785800350826,-14.6824178576167,
0.));
#188733=CARTESIAN_POINT('Ctrl Pts',(17.1785800350826,-14.6824178576167,
12.));
#188734=CARTESIAN_POINT('Ctrl Pts',(17.182736158472,-14.686469452232,0.));
#188735=CARTESIAN_POINT('Ctrl Pts',(17.182736158472,-14.686469452232,12.));
#188736=CARTESIAN_POINT('Ctrl Pts',(17.1870867909918,-14.6907440526958,
0.));
#188737=CARTESIAN_POINT('Ctrl Pts',(17.1870867909918,-14.6907440526958,
12.));
#188738=CARTESIAN_POINT('Ctrl Pts',(17.1916259308415,-14.6952385361706,
0.));
#188739=CARTESIAN_POINT('Ctrl Pts',(17.1916259308415,-14.6952385361706,
12.));
#188740=CARTESIAN_POINT('Ctrl Pts',(17.1963476411694,-14.699949811582,0.));
#188741=CARTESIAN_POINT('Ctrl Pts',(17.1963476411694,-14.699949811582,12.));
#188742=CARTESIAN_POINT('Ctrl Pts',(17.2012461084268,-14.7048748502663,
0.));
#188743=CARTESIAN_POINT('Ctrl Pts',(17.2012461084268,-14.7048748502663,
12.));
#188744=CARTESIAN_POINT('Ctrl Pts',(17.2063157097315,-14.7100107213586,
0.));
#188745=CARTESIAN_POINT('Ctrl Pts',(17.2063157097315,-14.7100107213586,
12.));
#188746=CARTESIAN_POINT('Ctrl Pts',(17.2115510835989,-14.7153546289339,
0.));
#188747=CARTESIAN_POINT('Ctrl Pts',(17.2115510835989,-14.7153546289339,
12.));
#188748=CARTESIAN_POINT('Ctrl Pts',(17.2169471814256,-14.7209039390327,
0.));
#188749=CARTESIAN_POINT('Ctrl Pts',(17.2169471814256,-14.7209039390327,
12.));
#188750=CARTESIAN_POINT('Ctrl Pts',(17.2224992099667,-14.7266561494282,
0.));
#188751=CARTESIAN_POINT('Ctrl Pts',(17.2224992099667,-14.7266561494282,
12.));
#188752=CARTESIAN_POINT('Ctrl Pts',(17.2282025904314,-14.7326088681163,
0.));
#188753=CARTESIAN_POINT('Ctrl Pts',(17.2282025904314,-14.7326088681163,
12.));
#188754=CARTESIAN_POINT('Ctrl Pts',(17.2340529062076,-14.7387597858117,
0.));
#188755=CARTESIAN_POINT('Ctrl Pts',(17.2340529062076,-14.7387597858117,
12.));
#188756=CARTESIAN_POINT('Ctrl Pts',(17.2400458713565,-14.7451066593792,
0.));
#188757=CARTESIAN_POINT('Ctrl Pts',(17.2400458713565,-14.7451066593792,
12.));
#188758=CARTESIAN_POINT('Ctrl Pts',(17.2461773413288,-14.7516473175124,
0.));
#188759=CARTESIAN_POINT('Ctrl Pts',(17.2461773413288,-14.7516473175124,
12.));
#188760=CARTESIAN_POINT('Ctrl Pts',(17.2524433146837,-14.7583796616617,
0.));
#188761=CARTESIAN_POINT('Ctrl Pts',(17.2524433146837,-14.7583796616617,
12.));
#188762=CARTESIAN_POINT('Ctrl Pts',(17.2588399401465,-14.7653016697591,
0.));
#188763=CARTESIAN_POINT('Ctrl Pts',(17.2588399401465,-14.7653016697591,
12.));
#188764=CARTESIAN_POINT('Ctrl Pts',(17.2653635155319,-14.7724113956731,
0.));
#188765=CARTESIAN_POINT('Ctrl Pts',(17.2653635155319,-14.7724113956731,
12.));
#188766=CARTESIAN_POINT('Ctrl Pts',(17.2720104735194,-14.7797069617804,
0.));
#188767=CARTESIAN_POINT('Ctrl Pts',(17.2720104735194,-14.7797069617804,
12.));
#188768=CARTESIAN_POINT('Ctrl Pts',(17.2787773704849,-14.787186553128,0.));
#188769=CARTESIAN_POINT('Ctrl Pts',(17.2787773704849,-14.787186553128,12.));
#188770=CARTESIAN_POINT('Ctrl Pts',(17.2856608733196,-14.7948484105249,
0.));
#188771=CARTESIAN_POINT('Ctrl Pts',(17.2856608733196,-14.7948484105249,
12.));
#188772=CARTESIAN_POINT('Ctrl Pts',(17.2926577496513,-14.8026908254276,
0.));
#188773=CARTESIAN_POINT('Ctrl Pts',(17.2926577496513,-14.8026908254276,
12.));
#188774=CARTESIAN_POINT('Ctrl Pts',(17.299764866148,-14.8107121391035,0.));
#188775=CARTESIAN_POINT('Ctrl Pts',(17.299764866148,-14.8107121391035,12.));
#188776=CARTESIAN_POINT('Ctrl Pts',(17.3069791853706,-14.8189107410162,
0.));
#188777=CARTESIAN_POINT('Ctrl Pts',(17.3069791853706,-14.8189107410162,
12.));
#188778=CARTESIAN_POINT('Ctrl Pts',(17.3142977632659,-14.8272850675379,
0.));
#188779=CARTESIAN_POINT('Ctrl Pts',(17.3142977632659,-14.8272850675379,
12.));
#188780=CARTESIAN_POINT('Ctrl Pts',(17.3217177462101,-14.8358336004197,
0.));
#188781=CARTESIAN_POINT('Ctrl Pts',(17.3217177462101,-14.8358336004197,
12.));
#188782=CARTESIAN_POINT('Ctrl Pts',(17.3292363662605,-14.8445548643508,
0.));
#188783=CARTESIAN_POINT('Ctrl Pts',(17.3292363662605,-14.8445548643508,
12.));
#188784=CARTESIAN_POINT('Ctrl Pts',(17.336850936485,-14.8534474245434,0.));
#188785=CARTESIAN_POINT('Ctrl Pts',(17.336850936485,-14.8534474245434,12.));
#188786=CARTESIAN_POINT('Ctrl Pts',(17.3445588463474,-14.8625098843417,
0.));
#188787=CARTESIAN_POINT('Ctrl Pts',(17.3445588463474,-14.8625098843417,
12.));
#188788=CARTESIAN_POINT('Ctrl Pts',(17.3523575568645,-14.8717408826956,
0.));
#188789=CARTESIAN_POINT('Ctrl Pts',(17.3523575568645,-14.8717408826956,
12.));
#188790=CARTESIAN_POINT('Ctrl Pts',(17.3602445978161,-14.8811390927423,
0.));
#188791=CARTESIAN_POINT('Ctrl Pts',(17.3602445978161,-14.8811390927423,
12.));
#188792=CARTESIAN_POINT('Ctrl Pts',(17.3682175653235,-14.8907032205788,
0.));
#188793=CARTESIAN_POINT('Ctrl Pts',(17.3682175653235,-14.8907032205788,
12.));
#188794=CARTESIAN_POINT('Ctrl Pts',(17.3762741193076,-14.900432003961,0.));
#188795=CARTESIAN_POINT('Ctrl Pts',(17.3762741193076,-14.900432003961,12.));
#188796=CARTESIAN_POINT('Ctrl Pts',(17.3844119809824,-14.9103242110057,
0.));
#188797=CARTESIAN_POINT('Ctrl Pts',(17.3844119809824,-14.9103242110057,
12.));
#188798=CARTESIAN_POINT('Ctrl Pts',(17.3926289303986,-14.9203786389342,
0.));
#188799=CARTESIAN_POINT('Ctrl Pts',(17.3926289303986,-14.9203786389342,
12.));
#188800=CARTESIAN_POINT('Ctrl Pts',(17.4009228040749,-14.9305941128757,
0.));
#188801=CARTESIAN_POINT('Ctrl Pts',(17.4009228040749,-14.9305941128757,
12.));
#188802=CARTESIAN_POINT('Ctrl Pts',(17.4092914926071,-14.940969484645,0.));
#188803=CARTESIAN_POINT('Ctrl Pts',(17.4092914926071,-14.940969484645,12.));
#188804=CARTESIAN_POINT('Ctrl Pts',(17.4177329382828,-14.9515036315143,
0.));
#188805=CARTESIAN_POINT('Ctrl Pts',(17.4177329382828,-14.9515036315143,
12.));
#188806=CARTESIAN_POINT('Ctrl Pts',(17.426245132709,-14.9621954549827,0.));
#188807=CARTESIAN_POINT('Ctrl Pts',(17.426245132709,-14.9621954549827,12.));
#188808=CARTESIAN_POINT('Ctrl Pts',(17.4348261151396,-14.9730438799452,
0.));
#188809=CARTESIAN_POINT('Ctrl Pts',(17.4348261151396,-14.9730438799452,
12.));
#188810=CARTESIAN_POINT('Ctrl Pts',(17.4434739707773,-14.9840478538358,
0.));
#188811=CARTESIAN_POINT('Ctrl Pts',(17.4434739707773,-14.9840478538358,
12.));
#188812=CARTESIAN_POINT('Ctrl Pts',(17.4521868291004,-14.9952063457778,
0.));
#188813=CARTESIAN_POINT('Ctrl Pts',(17.4521868291004,-14.9952063457778,
12.));
#188814=CARTESIAN_POINT('Ctrl Pts',(17.4609628621418,-15.0065183456921,
0.));
#188815=CARTESIAN_POINT('Ctrl Pts',(17.4609628621418,-15.0065183456921,
12.));
#188816=CARTESIAN_POINT('Ctrl Pts',(17.4698002829357,-15.0179828635086,
0.));
#188817=CARTESIAN_POINT('Ctrl Pts',(17.4698002829357,-15.0179828635086,
12.));
#188818=CARTESIAN_POINT('Ctrl Pts',(17.4786973441417,-15.029598928488,0.));
#188819=CARTESIAN_POINT('Ctrl Pts',(17.4786973441417,-15.029598928488,12.));
#188820=CARTESIAN_POINT('Ctrl Pts',(17.4876523366178,-15.0413655884993,
0.));
#188821=CARTESIAN_POINT('Ctrl Pts',(17.4876523366178,-15.0413655884993,
12.));
#188822=CARTESIAN_POINT('Ctrl Pts',(17.4966635880245,-15.0532819093085,
0.));
#188823=CARTESIAN_POINT('Ctrl Pts',(17.4966635880245,-15.0532819093085,
12.));
#188824=CARTESIAN_POINT('Ctrl Pts',(17.5057294613874,-15.0653469738306,
0.));
#188825=CARTESIAN_POINT('Ctrl Pts',(17.5057294613874,-15.0653469738306,
12.));
#188826=CARTESIAN_POINT('Ctrl Pts',(17.5148483539683,-15.0775598815748,
0.));
#188827=CARTESIAN_POINT('Ctrl Pts',(17.5148483539683,-15.0775598815748,
12.));
#188828=CARTESIAN_POINT('Ctrl Pts',(17.5240186961788,-15.0899197481082,
0.));
#188829=CARTESIAN_POINT('Ctrl Pts',(17.5240186961788,-15.0899197481082,
12.));
#188830=CARTESIAN_POINT('Ctrl Pts',(17.5332389504829,-15.1024257045033,
0.));
#188831=CARTESIAN_POINT('Ctrl Pts',(17.5332389504829,-15.1024257045033,
12.));
#188832=CARTESIAN_POINT('Ctrl Pts',(17.5425076102966,-15.1150768967729,
0.));
#188833=CARTESIAN_POINT('Ctrl Pts',(17.5425076102966,-15.1150768967729,
12.));
#188834=CARTESIAN_POINT('Ctrl Pts',(17.5518231989122,-15.127872485314,0.));
#188835=CARTESIAN_POINT('Ctrl Pts',(17.5518231989122,-15.127872485314,12.));
#188836=CARTESIAN_POINT('Ctrl Pts',(17.5611842686196,-15.1408116444877,
0.));
#188837=CARTESIAN_POINT('Ctrl Pts',(17.5611842686196,-15.1408116444877,
12.));
#188838=CARTESIAN_POINT('Ctrl Pts',(17.570589399803,-15.1538935621715,0.));
#188839=CARTESIAN_POINT('Ctrl Pts',(17.570589399803,-15.1538935621715,12.));
#188840=CARTESIAN_POINT('Ctrl Pts',(17.5800372000539,-15.1671174393136,
0.));
#188841=CARTESIAN_POINT('Ctrl Pts',(17.5800372000539,-15.1671174393136,
12.));
#188842=CARTESIAN_POINT('Ctrl Pts',(17.5895263032592,-15.1804824894605,
0.));
#188843=CARTESIAN_POINT('Ctrl Pts',(17.5895263032592,-15.1804824894605,
12.));
#188844=CARTESIAN_POINT('Ctrl Pts',(17.5990553687595,-15.1939879383268,
0.));
#188845=CARTESIAN_POINT('Ctrl Pts',(17.5990553687595,-15.1939879383268,
12.));
#188846=CARTESIAN_POINT('Ctrl Pts',(17.6086230806497,-15.2076330234686,
0.));
#188847=CARTESIAN_POINT('Ctrl Pts',(17.6086230806497,-15.2076330234686,
12.));
#188848=CARTESIAN_POINT('Ctrl Pts',(17.6182281470467,-15.22141699392,0.));
#188849=CARTESIAN_POINT('Ctrl Pts',(17.6182281470467,-15.22141699392,12.));
#188850=CARTESIAN_POINT('Ctrl Pts',(17.6278692993765,-15.2353391098367,
0.));
#188851=CARTESIAN_POINT('Ctrl Pts',(17.6278692993765,-15.2353391098367,
12.));
#188852=CARTESIAN_POINT('Ctrl Pts',(17.637545291637,-15.2493986421091,0.));
#188853=CARTESIAN_POINT('Ctrl Pts',(17.637545291637,-15.2493986421091,12.));
#188854=CARTESIAN_POINT('Ctrl Pts',(17.6472548997329,-15.263594872029,0.));
#188855=CARTESIAN_POINT('Ctrl Pts',(17.6472548997329,-15.263594872029,12.));
#188856=CARTESIAN_POINT('Ctrl Pts',(17.6569969209,-15.2779270910238,0.));
#188857=CARTESIAN_POINT('Ctrl Pts',(17.6569969209,-15.2779270910238,12.));
#188858=CARTESIAN_POINT('Ctrl Pts',(17.6667701731041,-15.2923946003598,
0.));
#188859=CARTESIAN_POINT('Ctrl Pts',(17.6667701731041,-15.2923946003598,
12.));
#188860=CARTESIAN_POINT('Ctrl Pts',(17.6765734944559,-15.3069967108501,
0.));
#188861=CARTESIAN_POINT('Ctrl Pts',(17.6765734944559,-15.3069967108501,
12.));
#188862=CARTESIAN_POINT('Ctrl Pts',(17.6864057426052,-15.3217327425341,
0.));
#188863=CARTESIAN_POINT('Ctrl Pts',(17.6864057426052,-15.3217327425341,
12.));
#188864=CARTESIAN_POINT('Ctrl Pts',(17.6962657941984,-15.3366020244069,
0.));
#188865=CARTESIAN_POINT('Ctrl Pts',(17.6962657941984,-15.3366020244069,
12.));
#188866=CARTESIAN_POINT('Ctrl Pts',(17.7061525444044,-15.3516038942064,
0.));
#188867=CARTESIAN_POINT('Ctrl Pts',(17.7061525444044,-15.3516038942064,
12.));
#188868=CARTESIAN_POINT('Ctrl Pts',(17.7160649064208,-15.3667376981702,
0.));
#188869=CARTESIAN_POINT('Ctrl Pts',(17.7160649064208,-15.3667376981702,
12.));
#188870=CARTESIAN_POINT('Ctrl Pts',(17.7260018109923,-15.3820027907965,
0.));
#188871=CARTESIAN_POINT('Ctrl Pts',(17.7260018109923,-15.3820027907965,
12.));
#188872=CARTESIAN_POINT('Ctrl Pts',(17.7359622059143,-15.3973985345796,
0.));
#188873=CARTESIAN_POINT('Ctrl Pts',(17.7359622059143,-15.3973985345796,
12.));
#188874=CARTESIAN_POINT('Ctrl Pts',(17.7459450555803,-15.4129242997828,
0.));
#188875=CARTESIAN_POINT('Ctrl Pts',(17.7459450555803,-15.4129242997828,
12.));
#188876=CARTESIAN_POINT('Ctrl Pts',(17.7559493405871,-15.4285794642658,
0.));
#188877=CARTESIAN_POINT('Ctrl Pts',(17.7559493405871,-15.4285794642658,
12.));
#188878=CARTESIAN_POINT('Ctrl Pts',(17.765974057326,-15.4443634132865,0.));
#188879=CARTESIAN_POINT('Ctrl Pts',(17.765974057326,-15.4443634132865,12.));
#188880=CARTESIAN_POINT('Ctrl Pts',(17.7760182175817,-15.4602755393019,
0.));
#188881=CARTESIAN_POINT('Ctrl Pts',(17.7760182175817,-15.4602755393019,
12.));
#188882=CARTESIAN_POINT('Ctrl Pts',(17.7860808481229,-15.4763152417506,
0.));
#188883=CARTESIAN_POINT('Ctrl Pts',(17.7860808481229,-15.4763152417506,
12.));
#188884=CARTESIAN_POINT('Ctrl Pts',(17.7961609903161,-15.4924819268529,
0.));
#188885=CARTESIAN_POINT('Ctrl Pts',(17.7961609903161,-15.4924819268529,
12.));
#188886=CARTESIAN_POINT('Ctrl Pts',(17.8062576997964,-15.5087750074728,
0.));
#188887=CARTESIAN_POINT('Ctrl Pts',(17.8062576997964,-15.5087750074728,
12.));
#188888=CARTESIAN_POINT('Ctrl Pts',(17.8163700461263,-15.5251939029558,
0.));
#188889=CARTESIAN_POINT('Ctrl Pts',(17.8163700461263,-15.5251939029558,
12.));
#188890=CARTESIAN_POINT('Ctrl Pts',(17.8264971124606,-15.5417380389639,
0.));
#188891=CARTESIAN_POINT('Ctrl Pts',(17.8264971124606,-15.5417380389639,
12.));
#188892=CARTESIAN_POINT('Ctrl Pts',(17.8366379952078,-15.5584068472976,
0.));
#188893=CARTESIAN_POINT('Ctrl Pts',(17.8366379952078,-15.5584068472976,
12.));
#188894=CARTESIAN_POINT('Ctrl Pts',(17.8467918036976,-15.5751997657153,
0.));
#188895=CARTESIAN_POINT('Ctrl Pts',(17.8467918036976,-15.5751997657153,
12.));
#188896=CARTESIAN_POINT('Ctrl Pts',(17.8569576598996,-15.5921162378183,
0.));
#188897=CARTESIAN_POINT('Ctrl Pts',(17.8569576598996,-15.5921162378183,
12.));
#188898=CARTESIAN_POINT('Ctrl Pts',(17.8671346981388,-15.6091557129205,
0.));
#188899=CARTESIAN_POINT('Ctrl Pts',(17.8671346981388,-15.6091557129205,
12.));
#188900=CARTESIAN_POINT('Ctrl Pts',(17.8773220648125,-15.6263176459107,
0.));
#188901=CARTESIAN_POINT('Ctrl Pts',(17.8773220648125,-15.6263176459107,
12.));
#188902=CARTESIAN_POINT('Ctrl Pts',(17.8875189181095,-15.6436014971088,
0.));
#188903=CARTESIAN_POINT('Ctrl Pts',(17.8875189181095,-15.6436014971088,
12.));
#188904=CARTESIAN_POINT('Ctrl Pts',(17.8977244277247,-15.6610067321036,
0.));
#188905=CARTESIAN_POINT('Ctrl Pts',(17.8977244277247,-15.6610067321036,
12.));
#188906=CARTESIAN_POINT('Ctrl Pts',(17.9079377746118,-15.6785328216467,
0.));
#188907=CARTESIAN_POINT('Ctrl Pts',(17.9079377746118,-15.6785328216467,
12.));
#188908=CARTESIAN_POINT('Ctrl Pts',(17.918158150746,-15.6961792415526,0.));
#188909=CARTESIAN_POINT('Ctrl Pts',(17.918158150746,-15.6961792415526,12.));
#188910=CARTESIAN_POINT('Ctrl Pts',(17.9283847588837,-15.713945472584,0.));
#188911=CARTESIAN_POINT('Ctrl Pts',(17.9283847588837,-15.713945472584,12.));
#188912=CARTESIAN_POINT('Ctrl Pts',(17.9386168123261,-15.7318310003334,
0.));
#188913=CARTESIAN_POINT('Ctrl Pts',(17.9386168123261,-15.7318310003334,
12.));
#188914=CARTESIAN_POINT('Ctrl Pts',(17.9488535346776,-15.7498353150856,
0.));
#188915=CARTESIAN_POINT('Ctrl Pts',(17.9488535346776,-15.7498353150856,
12.));
#188916=CARTESIAN_POINT('Ctrl Pts',(17.9590941596236,-15.7679579117072,
0.));
#188917=CARTESIAN_POINT('Ctrl Pts',(17.9590941596236,-15.7679579117072,
12.));
#188918=CARTESIAN_POINT('Ctrl Pts',(17.9693379307297,-15.786198289572,0.));
#188919=CARTESIAN_POINT('Ctrl Pts',(17.9693379307297,-15.786198289572,12.));
#188920=CARTESIAN_POINT('Ctrl Pts',(17.9795841012383,-15.8045559524674,
0.));
#188921=CARTESIAN_POINT('Ctrl Pts',(17.9795841012383,-15.8045559524674,
12.));
#188922=CARTESIAN_POINT('Ctrl Pts',(17.9898319338664,-15.8230304084963,
0.));
#188923=CARTESIAN_POINT('Ctrl Pts',(17.9898319338664,-15.8230304084963,
12.));
#188924=CARTESIAN_POINT('Ctrl Pts',(18.0000807006055,-15.8416211699682,
0.));
#188925=CARTESIAN_POINT('Ctrl Pts',(18.0000807006055,-15.8416211699682,
12.));
#188926=CARTESIAN_POINT('Ctrl Pts',(18.010329682521,-15.8603277532834,0.));
#188927=CARTESIAN_POINT('Ctrl Pts',(18.010329682521,-15.8603277532834,12.));
#188928=CARTESIAN_POINT('Ctrl Pts',(18.0205781695773,-15.8791496788685,
0.));
#188929=CARTESIAN_POINT('Ctrl Pts',(18.0205781695773,-15.8791496788685,
12.));
#188930=CARTESIAN_POINT('Ctrl Pts',(18.0308254604638,-15.8980864711043,
0.));
#188931=CARTESIAN_POINT('Ctrl Pts',(18.0308254604638,-15.8980864711043,
12.));
#188932=CARTESIAN_POINT('Ctrl Pts',(18.0410708624208,-15.9171376582436,
0.));
#188933=CARTESIAN_POINT('Ctrl Pts',(18.0410708624208,-15.9171376582436,
12.));
#188934=CARTESIAN_POINT('Ctrl Pts',(18.0513136910691,-15.9363027723244,
0.));
#188935=CARTESIAN_POINT('Ctrl Pts',(18.0513136910691,-15.9363027723244,
12.));
#188936=CARTESIAN_POINT('Ctrl Pts',(18.061553270236,-15.9555813490645,0.));
#188937=CARTESIAN_POINT('Ctrl Pts',(18.061553270236,-15.9555813490645,12.));
#188938=CARTESIAN_POINT('Ctrl Pts',(18.071788931796,-15.9749729277848,0.));
#188939=CARTESIAN_POINT('Ctrl Pts',(18.071788931796,-15.9749729277848,12.));
#188940=CARTESIAN_POINT('Ctrl Pts',(18.0820200155239,-15.9944770513616,
0.));
#188941=CARTESIAN_POINT('Ctrl Pts',(18.0820200155239,-15.9944770513616,
12.));
#188942=CARTESIAN_POINT('Ctrl Pts',(18.0922458689464,-16.0140932661612,
0.));
#188943=CARTESIAN_POINT('Ctrl Pts',(18.0922458689464,-16.0140932661612,
12.));
#188944=CARTESIAN_POINT('Ctrl Pts',(18.1024658471966,-16.0338211219694,
0.));
#188945=CARTESIAN_POINT('Ctrl Pts',(18.1024658471966,-16.0338211219694,
12.));
#188946=CARTESIAN_POINT('Ctrl Pts',(18.1126793128688,-16.0536601719124,
0.));
#188947=CARTESIAN_POINT('Ctrl Pts',(18.1126793128688,-16.0536601719124,
12.));
#188948=CARTESIAN_POINT('Ctrl Pts',(18.1228856358746,-16.0736099723664,
0.));
#188949=CARTESIAN_POINT('Ctrl Pts',(18.1228856358746,-16.0736099723664,
12.));
#188950=CARTESIAN_POINT('Ctrl Pts',(18.1330841933099,-16.0936700829108,
0.));
#188951=CARTESIAN_POINT('Ctrl Pts',(18.1330841933099,-16.0936700829108,
12.));
#188952=CARTESIAN_POINT('Ctrl Pts',(18.1432743693231,-16.113840066279,0.));
#188953=CARTESIAN_POINT('Ctrl Pts',(18.1432743693231,-16.113840066279,12.));
#188954=CARTESIAN_POINT('Ctrl Pts',(18.153455554985,-16.1341194882987,0.));
#188955=CARTESIAN_POINT('Ctrl Pts',(18.153455554985,-16.1341194882987,12.));
#188956=CARTESIAN_POINT('Ctrl Pts',(18.1636271481616,-16.1545079178261,
0.));
#188957=CARTESIAN_POINT('Ctrl Pts',(18.1636271481616,-16.1545079178261,
12.));
#188958=CARTESIAN_POINT('Ctrl Pts',(18.1737885533852,-16.1750049266673,
0.));
#188959=CARTESIAN_POINT('Ctrl Pts',(18.1737885533852,-16.1750049266673,
12.));
#188960=CARTESIAN_POINT('Ctrl Pts',(18.1839391817335,-16.1956100895076,
0.));
#188961=CARTESIAN_POINT('Ctrl Pts',(18.1839391817335,-16.1956100895076,
12.));
#188962=CARTESIAN_POINT('Ctrl Pts',(18.1940784507232,-16.2163229838878,
0.));
#188963=CARTESIAN_POINT('Ctrl Pts',(18.1940784507232,-16.2163229838878,
12.));
#188964=CARTESIAN_POINT('Ctrl Pts',(18.2042057842037,-16.237143190164,0.));
#188965=CARTESIAN_POINT('Ctrl Pts',(18.2042057842037,-16.237143190164,12.));
#188966=CARTESIAN_POINT('Ctrl Pts',(18.214320612253,-16.2580702914615,0.));
#188967=CARTESIAN_POINT('Ctrl Pts',(18.214320612253,-16.2580702914615,12.));
#188968=CARTESIAN_POINT('Ctrl Pts',(18.2244223710745,-16.2791038736223,
0.));
#188969=CARTESIAN_POINT('Ctrl Pts',(18.2244223710745,-16.2791038736223,
12.));
#188970=CARTESIAN_POINT('Ctrl Pts',(18.2345105028981,-16.3002435251378,
0.));
#188971=CARTESIAN_POINT('Ctrl Pts',(18.2345105028981,-16.3002435251378,
12.));
#188972=CARTESIAN_POINT('Ctrl Pts',(18.2445844558742,-16.3214888370988,
0.));
#188973=CARTESIAN_POINT('Ctrl Pts',(18.2445844558742,-16.3214888370988,
12.));
#188974=CARTESIAN_POINT('Ctrl Pts',(18.2546436839609,-16.342839403159,0.));
#188975=CARTESIAN_POINT('Ctrl Pts',(18.2546436839609,-16.342839403159,12.));
#188976=CARTESIAN_POINT('Ctrl Pts',(18.2646876468169,-16.3642948194869,
0.));
#188977=CARTESIAN_POINT('Ctrl Pts',(18.2646876468169,-16.3642948194869,
12.));
#188978=CARTESIAN_POINT('Ctrl Pts',(18.2747158096934,-16.385854684708,0.));
#188979=CARTESIAN_POINT('Ctrl Pts',(18.2747158096934,-16.385854684708,12.));
#188980=CARTESIAN_POINT('Ctrl Pts',(18.2847276433308,-16.4075185998454,
0.));
#188981=CARTESIAN_POINT('Ctrl Pts',(18.2847276433308,-16.4075185998454,
12.));
#188982=CARTESIAN_POINT('Ctrl Pts',(18.2947226238509,-16.4292861682377,
0.));
#188983=CARTESIAN_POINT('Ctrl Pts',(18.2947226238509,-16.4292861682377,
12.));
#188984=CARTESIAN_POINT('Ctrl Pts',(18.3047002326858,-16.4511569955231,
0.));
#188985=CARTESIAN_POINT('Ctrl Pts',(18.3047002326858,-16.4511569955231,
12.));
#188986=CARTESIAN_POINT('Ctrl Pts',(18.3146599565229,-16.4731306896439,
0.));
#188987=CARTESIAN_POINT('Ctrl Pts',(18.3146599565229,-16.4731306896439,
12.));
#188988=CARTESIAN_POINT('Ctrl Pts',(18.3246012872468,-16.4952068608344,
0.));
#188989=CARTESIAN_POINT('Ctrl Pts',(18.3246012872468,-16.4952068608344,
12.));
#188990=CARTESIAN_POINT('Ctrl Pts',(18.3345237218864,-16.5173851216045,
0.));
#188991=CARTESIAN_POINT('Ctrl Pts',(18.3345237218864,-16.5173851216045,
12.));
#188992=CARTESIAN_POINT('Ctrl Pts',(18.3444267625601,-16.5396650867139,
0.));
#188993=CARTESIAN_POINT('Ctrl Pts',(18.3444267625601,-16.5396650867139,
12.));
#188994=CARTESIAN_POINT('Ctrl Pts',(18.3543099164331,-16.5620463731414,
0.));
#188995=CARTESIAN_POINT('Ctrl Pts',(18.3543099164331,-16.5620463731414,
12.));
#188996=CARTESIAN_POINT('Ctrl Pts',(18.364172695589,-16.5845286000218,0.));
#188997=CARTESIAN_POINT('Ctrl Pts',(18.364172695589,-16.5845286000218,12.));
#188998=CARTESIAN_POINT('Ctrl Pts',(18.3740146168879,-16.6071113885711,
0.));
#188999=CARTESIAN_POINT('Ctrl Pts',(18.3740146168879,-16.6071113885711,
12.));
#189000=CARTESIAN_POINT('Ctrl Pts',(18.3838352018327,-16.6297943620056,
0.));
#189001=CARTESIAN_POINT('Ctrl Pts',(18.3838352018327,-16.6297943620056,
12.));
#189002=CARTESIAN_POINT('Ctrl Pts',(18.3936339764332,-16.6525771454513,
0.));
#189003=CARTESIAN_POINT('Ctrl Pts',(18.3936339764332,-16.6525771454513,
12.));
#189004=CARTESIAN_POINT('Ctrl Pts',(18.4034104710789,-16.6754593658513,
0.));
#189005=CARTESIAN_POINT('Ctrl Pts',(18.4034104710789,-16.6754593658513,
12.));
#189006=CARTESIAN_POINT('Ctrl Pts',(18.4131642203989,-16.698440651849,0.));
#189007=CARTESIAN_POINT('Ctrl Pts',(18.4131642203989,-16.698440651849,12.));
#189008=CARTESIAN_POINT('Ctrl Pts',(18.4228947633186,-16.7215206338818,
0.));
#189009=CARTESIAN_POINT('Ctrl Pts',(18.4228947633186,-16.7215206338818,
12.));
#189010=CARTESIAN_POINT('Ctrl Pts',(18.4326016431392,-16.7446989442882,
0.));
#189011=CARTESIAN_POINT('Ctrl Pts',(18.4326016431392,-16.7446989442882,
12.));
#189012=CARTESIAN_POINT('Ctrl Pts',(18.4422844076099,-16.7679752173992,
0.));
#189013=CARTESIAN_POINT('Ctrl Pts',(18.4422844076099,-16.7679752173992,
12.));
#189014=CARTESIAN_POINT('Ctrl Pts',(18.4519426090124,-16.791349089629,0.));
#189015=CARTESIAN_POINT('Ctrl Pts',(18.4519426090124,-16.791349089629,12.));
#189016=CARTESIAN_POINT('Ctrl Pts',(18.4615758042305,-16.8148201995472,
0.));
#189017=CARTESIAN_POINT('Ctrl Pts',(18.4615758042305,-16.8148201995472,
12.));
#189018=CARTESIAN_POINT('Ctrl Pts',(18.4711835548622,-16.8383881879707,
0.));
#189019=CARTESIAN_POINT('Ctrl Pts',(18.4711835548622,-16.8383881879707,
12.));
#189020=CARTESIAN_POINT('Ctrl Pts',(18.4807654268769,-16.8620526977169,
0.));
#189021=CARTESIAN_POINT('Ctrl Pts',(18.4807654268769,-16.8620526977169,
12.));
#189022=CARTESIAN_POINT('Ctrl Pts',(18.4903209902226,-16.8858133733086,
0.));
#189023=CARTESIAN_POINT('Ctrl Pts',(18.4903209902226,-16.8858133733086,
12.));
#189024=CARTESIAN_POINT('Ctrl Pts',(18.4998498184619,-16.9096698606942,
0.));
#189025=CARTESIAN_POINT('Ctrl Pts',(18.4998498184619,-16.9096698606942,
12.));
#189026=CARTESIAN_POINT('Ctrl Pts',(18.5093514883835,-16.9336218069353,
0.));
#189027=CARTESIAN_POINT('Ctrl Pts',(18.5093514883835,-16.9336218069353,
12.));
#189028=CARTESIAN_POINT('Ctrl Pts',(18.518825579666,-16.957668859934,0.));
#189029=CARTESIAN_POINT('Ctrl Pts',(18.518825579666,-16.957668859934,12.));
#189030=CARTESIAN_POINT('Ctrl Pts',(18.5282716744198,-16.9818106680382,
0.));
#189031=CARTESIAN_POINT('Ctrl Pts',(18.5282716744198,-16.9818106680382,
12.));
#189032=CARTESIAN_POINT('Ctrl Pts',(18.5376893576961,-17.0060468805099,
0.));
#189033=CARTESIAN_POINT('Ctrl Pts',(18.5376893576961,-17.0060468805099,
12.));
#189034=CARTESIAN_POINT('Ctrl Pts',(18.5470782182089,-17.030377148174,0.));
#189035=CARTESIAN_POINT('Ctrl Pts',(18.5470782182089,-17.030377148174,12.));
#189036=CARTESIAN_POINT('Ctrl Pts',(18.5564378489628,-17.0548011239751,
0.));
#189037=CARTESIAN_POINT('Ctrl Pts',(18.5564378489628,-17.0548011239751,
12.));
#189038=CARTESIAN_POINT('Ctrl Pts',(18.5657678479788,-17.0793184636079,
0.));
#189039=CARTESIAN_POINT('Ctrl Pts',(18.5657678479788,-17.0793184636079,
12.));
#189040=CARTESIAN_POINT('Ctrl Pts',(18.5750678188543,-17.1039288260002,
0.));
#189041=CARTESIAN_POINT('Ctrl Pts',(18.5750678188543,-17.1039288260002,
12.));
#189042=CARTESIAN_POINT('Ctrl Pts',(18.5843373717253,-17.1286318741185,
0.));
#189043=CARTESIAN_POINT('Ctrl Pts',(18.5843373717253,-17.1286318741185,
12.));
#189044=CARTESIAN_POINT('Ctrl Pts',(18.5935761222833,-17.1534272741646,
0.));
#189045=CARTESIAN_POINT('Ctrl Pts',(18.5935761222833,-17.1534272741646,
12.));
#189046=CARTESIAN_POINT('Ctrl Pts',(18.6027836898826,-17.1783146940131,
0.));
#189047=CARTESIAN_POINT('Ctrl Pts',(18.6027836898826,-17.1783146940131,
12.));
#189048=CARTESIAN_POINT('Ctrl Pts',(18.6119596959957,-17.2032938019288,
0.));
#189049=CARTESIAN_POINT('Ctrl Pts',(18.6119596959957,-17.2032938019288,
12.));
#189050=CARTESIAN_POINT('Ctrl Pts',(18.6211037624041,-17.2283642650519,
0.));
#189051=CARTESIAN_POINT('Ctrl Pts',(18.6211037624041,-17.2283642650519,
12.));
#189052=CARTESIAN_POINT('Ctrl Pts',(18.630215509794,-17.2535257482186,0.));
#189053=CARTESIAN_POINT('Ctrl Pts',(18.630215509794,-17.2535257482186,12.));
#189054=CARTESIAN_POINT('Ctrl Pts',(18.639294555474,-17.278777912021,0.));
#189055=CARTESIAN_POINT('Ctrl Pts',(18.639294555474,-17.278777912021,12.));
#189056=CARTESIAN_POINT('Ctrl Pts',(18.6483405141853,-17.3041204135069,
0.));
#189057=CARTESIAN_POINT('Ctrl Pts',(18.6483405141853,-17.3041204135069,
12.));
#189058=CARTESIAN_POINT('Ctrl Pts',(18.6573530024019,-17.3295529098612,
0.));
#189059=CARTESIAN_POINT('Ctrl Pts',(18.6573530024019,-17.3295529098612,
12.));
#189060=CARTESIAN_POINT('Ctrl Pts',(18.6663316416569,-17.3550750612438,
0.));
#189061=CARTESIAN_POINT('Ctrl Pts',(18.6663316416569,-17.3550750612438,
12.));
#189062=CARTESIAN_POINT('Ctrl Pts',(18.6752760624045,-17.3806865340744,
0.));
#189063=CARTESIAN_POINT('Ctrl Pts',(18.6752760624045,-17.3806865340744,
12.));
#189064=CARTESIAN_POINT('Ctrl Pts',(18.6841859073472,-17.4063870038563,
0.));
#189065=CARTESIAN_POINT('Ctrl Pts',(18.6841859073472,-17.4063870038563,
12.));
#189066=CARTESIAN_POINT('Ctrl Pts',(18.6930608357421,-17.4321761588148,
0.));
#189067=CARTESIAN_POINT('Ctrl Pts',(18.6930608357421,-17.4321761588148,
12.));
#189068=CARTESIAN_POINT('Ctrl Pts',(18.7019005250322,-17.4580537012764,
0.));
#189069=CARTESIAN_POINT('Ctrl Pts',(18.7019005250322,-17.4580537012764,
12.));
#189070=CARTESIAN_POINT('Ctrl Pts',(18.7107046613941,-17.4840193397176,
0.));
#189071=CARTESIAN_POINT('Ctrl Pts',(18.7107046613941,-17.4840193397176,
12.));
#189072=CARTESIAN_POINT('Ctrl Pts',(18.7194729318127,-17.5100727820891,
0.));
#189073=CARTESIAN_POINT('Ctrl Pts',(18.7194729318127,-17.5100727820891,
12.));
#189074=CARTESIAN_POINT('Ctrl Pts',(18.728205015716,-17.5362137287604,0.));
#189075=CARTESIAN_POINT('Ctrl Pts',(18.728205015716,-17.5362137287604,12.));
#189076=CARTESIAN_POINT('Ctrl Pts',(18.7369005764558,-17.5624418653248,
0.));
#189077=CARTESIAN_POINT('Ctrl Pts',(18.7369005764558,-17.5624418653248,
12.));
#189078=CARTESIAN_POINT('Ctrl Pts',(18.7455592536667,-17.5887568561361,
0.));
#189079=CARTESIAN_POINT('Ctrl Pts',(18.7455592536667,-17.5887568561361,
12.));
#189080=CARTESIAN_POINT('Ctrl Pts',(18.7541806530935,-17.6151583356989,
0.));
#189081=CARTESIAN_POINT('Ctrl Pts',(18.7541806530935,-17.6151583356989,
12.));
#189082=CARTESIAN_POINT('Ctrl Pts',(18.7627643613139,-17.6416459210646,
0.));
#189083=CARTESIAN_POINT('Ctrl Pts',(18.7627643613139,-17.6416459210646,
12.));
#189084=CARTESIAN_POINT('Ctrl Pts',(18.7713099642673,-17.6682192274197,
0.));
#189085=CARTESIAN_POINT('Ctrl Pts',(18.7713099642673,-17.6682192274197,
12.));
#189086=CARTESIAN_POINT('Ctrl Pts',(18.7798170641305,-17.6948778822982,
0.));
#189087=CARTESIAN_POINT('Ctrl Pts',(18.7798170641305,-17.6948778822982,
12.));
#189088=CARTESIAN_POINT('Ctrl Pts',(18.7882852976016,-17.7216215409019,
0.));
#189089=CARTESIAN_POINT('Ctrl Pts',(18.7882852976016,-17.7216215409019,
12.));
#189090=CARTESIAN_POINT('Ctrl Pts',(18.7967143519444,-17.7484498996916,
0.));
#189091=CARTESIAN_POINT('Ctrl Pts',(18.7967143519444,-17.7484498996916,
12.));
#189092=CARTESIAN_POINT('Ctrl Pts',(18.8051039860543,-17.7753627137898,
0.));
#189093=CARTESIAN_POINT('Ctrl Pts',(18.8051039860543,-17.7753627137898,
12.));
#189094=CARTESIAN_POINT('Ctrl Pts',(18.8134540340581,-17.8023598011135,
0.));
#189095=CARTESIAN_POINT('Ctrl Pts',(18.8134540340581,-17.8023598011135,
12.));
#189096=CARTESIAN_POINT('Ctrl Pts',(18.8217643886368,-17.8294410311105,
0.));
#189097=CARTESIAN_POINT('Ctrl Pts',(18.8217643886368,-17.8294410311105,
12.));
#189098=CARTESIAN_POINT('Ctrl Pts',(18.8300349896187,-17.8566063174871,
0.));
#189099=CARTESIAN_POINT('Ctrl Pts',(18.8300349896187,-17.8566063174871,
12.));
#189100=CARTESIAN_POINT('Ctrl Pts',(18.8366196462746,-17.8784057509434,
0.));
#189101=CARTESIAN_POINT('Ctrl Pts',(18.8366196462746,-17.8784057509434,
12.));
#189102=CARTESIAN_POINT('Ctrl Pts',(18.8415402351882,-17.8947931177853,
0.));
#189103=CARTESIAN_POINT('Ctrl Pts',(18.8415402351882,-17.8947931177853,
12.));
#189104=CARTESIAN_POINT('Ctrl Pts',(18.8448126709726,-17.9057348246611,
0.));
#189105=CARTESIAN_POINT('Ctrl Pts',(18.8448126709726,-17.9057348246611,
12.));
#189106=CARTESIAN_POINT('Ctrl Pts',(18.8464468996588,-17.9112098770111,
0.));
#189107=CARTESIAN_POINT('Ctrl Pts',(18.8464468996588,-17.9112098770111,
12.));
#189108=CARTESIAN_POINT('',(18.8464468996588,-17.9112098770111,0.));
#189109=CARTESIAN_POINT('Ctrl Pts',(17.1452095830632,-14.6513681262571,
0.));
#189110=CARTESIAN_POINT('Ctrl Pts',(17.1452153999142,-14.6513711852843,
0.));
#189111=CARTESIAN_POINT('Ctrl Pts',(17.1452600887037,-14.6514066997196,
0.));
#189112=CARTESIAN_POINT('Ctrl Pts',(17.1454262858043,-14.6515481598068,
0.));
#189113=CARTESIAN_POINT('Ctrl Pts',(17.1458462295271,-14.6519131634508,
0.));
#189114=CARTESIAN_POINT('Ctrl Pts',(17.1466998098673,-14.6526624064978,
0.));
#189115=CARTESIAN_POINT('Ctrl Pts',(17.147876394491,-14.6537016966184,0.));
#189116=CARTESIAN_POINT('Ctrl Pts',(17.1493641837558,-14.655024862281,0.));
#189117=CARTESIAN_POINT('Ctrl Pts',(17.1511476869496,-14.6566237952435,
0.));
#189118=CARTESIAN_POINT('Ctrl Pts',(17.1532107762718,-14.6584900555302,
0.));
#189119=CARTESIAN_POINT('Ctrl Pts',(17.1555401986401,-14.6606167169642,
0.));
#189120=CARTESIAN_POINT('Ctrl Pts',(17.1581262646789,-14.6629987285992,
0.));
#189121=CARTESIAN_POINT('Ctrl Pts',(17.1609609517369,-14.6656319165057,
0.));
#189122=CARTESIAN_POINT('Ctrl Pts',(17.1640366762305,-14.6685123374423,
0.));
#189123=CARTESIAN_POINT('Ctrl Pts',(17.167344972302,-14.671635583332,0.));
#189124=CARTESIAN_POINT('Ctrl Pts',(17.1708771619129,-14.6749971333867,
0.));
#189125=CARTESIAN_POINT('Ctrl Pts',(17.1746247499057,-14.6785925615677,
0.));
#189126=CARTESIAN_POINT('Ctrl Pts',(17.1785800350826,-14.6824178576167,
0.));
#189127=CARTESIAN_POINT('Ctrl Pts',(17.182736158472,-14.686469452232,0.));
#189128=CARTESIAN_POINT('Ctrl Pts',(17.1870867909918,-14.6907440526958,
0.));
#189129=CARTESIAN_POINT('Ctrl Pts',(17.1916259308415,-14.6952385361706,
0.));
#189130=CARTESIAN_POINT('Ctrl Pts',(17.1963476411694,-14.699949811582,0.));
#189131=CARTESIAN_POINT('Ctrl Pts',(17.2012461084268,-14.7048748502663,
0.));
#189132=CARTESIAN_POINT('Ctrl Pts',(17.2063157097315,-14.7100107213586,
0.));
#189133=CARTESIAN_POINT('Ctrl Pts',(17.2115510835989,-14.7153546289339,
0.));
#189134=CARTESIAN_POINT('Ctrl Pts',(17.2169471814256,-14.7209039390327,
0.));
#189135=CARTESIAN_POINT('Ctrl Pts',(17.2224992099667,-14.7266561494282,
0.));
#189136=CARTESIAN_POINT('Ctrl Pts',(17.2282025904314,-14.7326088681163,
0.));
#189137=CARTESIAN_POINT('Ctrl Pts',(17.2340529062076,-14.7387597858117,
0.));
#189138=CARTESIAN_POINT('Ctrl Pts',(17.2400458713565,-14.7451066593792,
0.));
#189139=CARTESIAN_POINT('Ctrl Pts',(17.2461773413288,-14.7516473175124,
0.));
#189140=CARTESIAN_POINT('Ctrl Pts',(17.2524433146837,-14.7583796616617,
0.));
#189141=CARTESIAN_POINT('Ctrl Pts',(17.2588399401465,-14.7653016697591,
0.));
#189142=CARTESIAN_POINT('Ctrl Pts',(17.2653635155319,-14.7724113956731,
0.));
#189143=CARTESIAN_POINT('Ctrl Pts',(17.2720104735194,-14.7797069617804,
0.));
#189144=CARTESIAN_POINT('Ctrl Pts',(17.2787773704849,-14.787186553128,0.));
#189145=CARTESIAN_POINT('Ctrl Pts',(17.2856608733196,-14.7948484105249,
0.));
#189146=CARTESIAN_POINT('Ctrl Pts',(17.2926577496513,-14.8026908254276,
0.));
#189147=CARTESIAN_POINT('Ctrl Pts',(17.299764866148,-14.8107121391035,0.));
#189148=CARTESIAN_POINT('Ctrl Pts',(17.3069791853706,-14.8189107410162,
0.));
#189149=CARTESIAN_POINT('Ctrl Pts',(17.3142977632659,-14.8272850675379,
0.));
#189150=CARTESIAN_POINT('Ctrl Pts',(17.3217177462101,-14.8358336004197,
0.));
#189151=CARTESIAN_POINT('Ctrl Pts',(17.3292363662605,-14.8445548643508,
0.));
#189152=CARTESIAN_POINT('Ctrl Pts',(17.336850936485,-14.8534474245434,0.));
#189153=CARTESIAN_POINT('Ctrl Pts',(17.3445588463474,-14.8625098843417,
0.));
#189154=CARTESIAN_POINT('Ctrl Pts',(17.3523575568645,-14.8717408826956,
0.));
#189155=CARTESIAN_POINT('Ctrl Pts',(17.3602445978161,-14.8811390927423,
0.));
#189156=CARTESIAN_POINT('Ctrl Pts',(17.3682175653235,-14.8907032205788,
0.));
#189157=CARTESIAN_POINT('Ctrl Pts',(17.3762741193076,-14.900432003961,0.));
#189158=CARTESIAN_POINT('Ctrl Pts',(17.3844119809824,-14.9103242110057,
0.));
#189159=CARTESIAN_POINT('Ctrl Pts',(17.3926289303986,-14.9203786389342,
0.));
#189160=CARTESIAN_POINT('Ctrl Pts',(17.4009228040749,-14.9305941128757,
0.));
#189161=CARTESIAN_POINT('Ctrl Pts',(17.4092914926071,-14.940969484645,0.));
#189162=CARTESIAN_POINT('Ctrl Pts',(17.4177329382828,-14.9515036315143,
0.));
#189163=CARTESIAN_POINT('Ctrl Pts',(17.426245132709,-14.9621954549827,0.));
#189164=CARTESIAN_POINT('Ctrl Pts',(17.4348261151396,-14.9730438799452,
0.));
#189165=CARTESIAN_POINT('Ctrl Pts',(17.4434739707773,-14.9840478538358,
0.));
#189166=CARTESIAN_POINT('Ctrl Pts',(17.4521868291004,-14.9952063457778,
0.));
#189167=CARTESIAN_POINT('Ctrl Pts',(17.4609628621418,-15.0065183456921,
0.));
#189168=CARTESIAN_POINT('Ctrl Pts',(17.4698002829357,-15.0179828635086,
0.));
#189169=CARTESIAN_POINT('Ctrl Pts',(17.4786973441417,-15.029598928488,0.));
#189170=CARTESIAN_POINT('Ctrl Pts',(17.4876523366178,-15.0413655884993,
0.));
#189171=CARTESIAN_POINT('Ctrl Pts',(17.4966635880245,-15.0532819093085,
0.));
#189172=CARTESIAN_POINT('Ctrl Pts',(17.5057294613874,-15.0653469738306,
0.));
#189173=CARTESIAN_POINT('Ctrl Pts',(17.5148483539683,-15.0775598815748,
0.));
#189174=CARTESIAN_POINT('Ctrl Pts',(17.5240186961788,-15.0899197481082,
0.));
#189175=CARTESIAN_POINT('Ctrl Pts',(17.5332389504829,-15.1024257045033,
0.));
#189176=CARTESIAN_POINT('Ctrl Pts',(17.5425076102966,-15.1150768967729,
0.));
#189177=CARTESIAN_POINT('Ctrl Pts',(17.5518231989122,-15.127872485314,0.));
#189178=CARTESIAN_POINT('Ctrl Pts',(17.5611842686196,-15.1408116444877,
0.));
#189179=CARTESIAN_POINT('Ctrl Pts',(17.570589399803,-15.1538935621715,0.));
#189180=CARTESIAN_POINT('Ctrl Pts',(17.5800372000539,-15.1671174393136,
0.));
#189181=CARTESIAN_POINT('Ctrl Pts',(17.5895263032592,-15.1804824894605,
0.));
#189182=CARTESIAN_POINT('Ctrl Pts',(17.5990553687595,-15.1939879383268,
0.));
#189183=CARTESIAN_POINT('Ctrl Pts',(17.6086230806497,-15.2076330234686,
0.));
#189184=CARTESIAN_POINT('Ctrl Pts',(17.6182281470467,-15.22141699392,0.));
#189185=CARTESIAN_POINT('Ctrl Pts',(17.6278692993765,-15.2353391098367,
0.));
#189186=CARTESIAN_POINT('Ctrl Pts',(17.637545291637,-15.2493986421091,0.));
#189187=CARTESIAN_POINT('Ctrl Pts',(17.6472548997329,-15.263594872029,0.));
#189188=CARTESIAN_POINT('Ctrl Pts',(17.6569969209,-15.2779270910238,0.));
#189189=CARTESIAN_POINT('Ctrl Pts',(17.6667701731041,-15.2923946003598,
0.));
#189190=CARTESIAN_POINT('Ctrl Pts',(17.6765734944559,-15.3069967108501,
0.));
#189191=CARTESIAN_POINT('Ctrl Pts',(17.6864057426052,-15.3217327425341,
0.));
#189192=CARTESIAN_POINT('Ctrl Pts',(17.6962657941984,-15.3366020244069,
0.));
#189193=CARTESIAN_POINT('Ctrl Pts',(17.7061525444044,-15.3516038942064,
0.));
#189194=CARTESIAN_POINT('Ctrl Pts',(17.7160649064208,-15.3667376981702,
0.));
#189195=CARTESIAN_POINT('Ctrl Pts',(17.7260018109923,-15.3820027907965,
0.));
#189196=CARTESIAN_POINT('Ctrl Pts',(17.7359622059143,-15.3973985345796,
0.));
#189197=CARTESIAN_POINT('Ctrl Pts',(17.7459450555803,-15.4129242997828,
0.));
#189198=CARTESIAN_POINT('Ctrl Pts',(17.7559493405871,-15.4285794642658,
0.));
#189199=CARTESIAN_POINT('Ctrl Pts',(17.765974057326,-15.4443634132865,0.));
#189200=CARTESIAN_POINT('Ctrl Pts',(17.7760182175817,-15.4602755393019,
0.));
#189201=CARTESIAN_POINT('Ctrl Pts',(17.7860808481229,-15.4763152417506,
0.));
#189202=CARTESIAN_POINT('Ctrl Pts',(17.7961609903161,-15.4924819268529,
0.));
#189203=CARTESIAN_POINT('Ctrl Pts',(17.8062576997964,-15.5087750074728,
0.));
#189204=CARTESIAN_POINT('Ctrl Pts',(17.8163700461263,-15.5251939029558,
0.));
#189205=CARTESIAN_POINT('Ctrl Pts',(17.8264971124606,-15.5417380389639,
0.));
#189206=CARTESIAN_POINT('Ctrl Pts',(17.8366379952078,-15.5584068472976,
0.));
#189207=CARTESIAN_POINT('Ctrl Pts',(17.8467918036976,-15.5751997657153,
0.));
#189208=CARTESIAN_POINT('Ctrl Pts',(17.8569576598996,-15.5921162378183,
0.));
#189209=CARTESIAN_POINT('Ctrl Pts',(17.8671346981388,-15.6091557129205,
0.));
#189210=CARTESIAN_POINT('Ctrl Pts',(17.8773220648125,-15.6263176459107,
0.));
#189211=CARTESIAN_POINT('Ctrl Pts',(17.8875189181095,-15.6436014971088,
0.));
#189212=CARTESIAN_POINT('Ctrl Pts',(17.8977244277247,-15.6610067321036,
0.));
#189213=CARTESIAN_POINT('Ctrl Pts',(17.9079377746118,-15.6785328216467,
0.));
#189214=CARTESIAN_POINT('Ctrl Pts',(17.918158150746,-15.6961792415526,0.));
#189215=CARTESIAN_POINT('Ctrl Pts',(17.9283847588837,-15.713945472584,0.));
#189216=CARTESIAN_POINT('Ctrl Pts',(17.9386168123261,-15.7318310003334,
0.));
#189217=CARTESIAN_POINT('Ctrl Pts',(17.9488535346776,-15.7498353150856,
0.));
#189218=CARTESIAN_POINT('Ctrl Pts',(17.9590941596236,-15.7679579117072,
0.));
#189219=CARTESIAN_POINT('Ctrl Pts',(17.9693379307297,-15.786198289572,0.));
#189220=CARTESIAN_POINT('Ctrl Pts',(17.9795841012383,-15.8045559524674,
0.));
#189221=CARTESIAN_POINT('Ctrl Pts',(17.9898319338664,-15.8230304084963,
0.));
#189222=CARTESIAN_POINT('Ctrl Pts',(18.0000807006055,-15.8416211699682,
0.));
#189223=CARTESIAN_POINT('Ctrl Pts',(18.010329682521,-15.8603277532834,0.));
#189224=CARTESIAN_POINT('Ctrl Pts',(18.0205781695773,-15.8791496788685,
0.));
#189225=CARTESIAN_POINT('Ctrl Pts',(18.0308254604638,-15.8980864711043,
0.));
#189226=CARTESIAN_POINT('Ctrl Pts',(18.0410708624208,-15.9171376582436,
0.));
#189227=CARTESIAN_POINT('Ctrl Pts',(18.0513136910691,-15.9363027723244,
0.));
#189228=CARTESIAN_POINT('Ctrl Pts',(18.061553270236,-15.9555813490645,0.));
#189229=CARTESIAN_POINT('Ctrl Pts',(18.071788931796,-15.9749729277848,0.));
#189230=CARTESIAN_POINT('Ctrl Pts',(18.0820200155239,-15.9944770513616,
0.));
#189231=CARTESIAN_POINT('Ctrl Pts',(18.0922458689464,-16.0140932661612,
0.));
#189232=CARTESIAN_POINT('Ctrl Pts',(18.1024658471966,-16.0338211219694,
0.));
#189233=CARTESIAN_POINT('Ctrl Pts',(18.1126793128688,-16.0536601719124,
0.));
#189234=CARTESIAN_POINT('Ctrl Pts',(18.1228856358746,-16.0736099723664,
0.));
#189235=CARTESIAN_POINT('Ctrl Pts',(18.1330841933099,-16.0936700829108,
0.));
#189236=CARTESIAN_POINT('Ctrl Pts',(18.1432743693231,-16.113840066279,0.));
#189237=CARTESIAN_POINT('Ctrl Pts',(18.153455554985,-16.1341194882987,0.));
#189238=CARTESIAN_POINT('Ctrl Pts',(18.1636271481616,-16.1545079178261,
0.));
#189239=CARTESIAN_POINT('Ctrl Pts',(18.1737885533852,-16.1750049266673,
0.));
#189240=CARTESIAN_POINT('Ctrl Pts',(18.1839391817335,-16.1956100895076,
0.));
#189241=CARTESIAN_POINT('Ctrl Pts',(18.1940784507232,-16.2163229838878,
0.));
#189242=CARTESIAN_POINT('Ctrl Pts',(18.2042057842037,-16.237143190164,0.));
#189243=CARTESIAN_POINT('Ctrl Pts',(18.214320612253,-16.2580702914615,0.));
#189244=CARTESIAN_POINT('Ctrl Pts',(18.2244223710745,-16.2791038736223,
0.));
#189245=CARTESIAN_POINT('Ctrl Pts',(18.2345105028981,-16.3002435251378,
0.));
#189246=CARTESIAN_POINT('Ctrl Pts',(18.2445844558742,-16.3214888370988,
0.));
#189247=CARTESIAN_POINT('Ctrl Pts',(18.2546436839609,-16.342839403159,0.));
#189248=CARTESIAN_POINT('Ctrl Pts',(18.2646876468169,-16.3642948194869,
0.));
#189249=CARTESIAN_POINT('Ctrl Pts',(18.2747158096934,-16.385854684708,0.));
#189250=CARTESIAN_POINT('Ctrl Pts',(18.2847276433308,-16.4075185998454,
0.));
#189251=CARTESIAN_POINT('Ctrl Pts',(18.2947226238509,-16.4292861682377,
0.));
#189252=CARTESIAN_POINT('Ctrl Pts',(18.3047002326858,-16.4511569955231,
0.));
#189253=CARTESIAN_POINT('Ctrl Pts',(18.3146599565229,-16.4731306896439,
0.));
#189254=CARTESIAN_POINT('Ctrl Pts',(18.3246012872468,-16.4952068608344,
0.));
#189255=CARTESIAN_POINT('Ctrl Pts',(18.3345237218864,-16.5173851216045,
0.));
#189256=CARTESIAN_POINT('Ctrl Pts',(18.3444267625601,-16.5396650867139,
0.));
#189257=CARTESIAN_POINT('Ctrl Pts',(18.3543099164331,-16.5620463731414,
0.));
#189258=CARTESIAN_POINT('Ctrl Pts',(18.364172695589,-16.5845286000218,0.));
#189259=CARTESIAN_POINT('Ctrl Pts',(18.3740146168879,-16.6071113885711,
0.));
#189260=CARTESIAN_POINT('Ctrl Pts',(18.3838352018327,-16.6297943620056,
0.));
#189261=CARTESIAN_POINT('Ctrl Pts',(18.3936339764332,-16.6525771454513,
0.));
#189262=CARTESIAN_POINT('Ctrl Pts',(18.4034104710789,-16.6754593658513,
0.));
#189263=CARTESIAN_POINT('Ctrl Pts',(18.4131642203989,-16.698440651849,0.));
#189264=CARTESIAN_POINT('Ctrl Pts',(18.4228947633186,-16.7215206338818,
0.));
#189265=CARTESIAN_POINT('Ctrl Pts',(18.4326016431392,-16.7446989442882,
0.));
#189266=CARTESIAN_POINT('Ctrl Pts',(18.4422844076099,-16.7679752173992,
0.));
#189267=CARTESIAN_POINT('Ctrl Pts',(18.4519426090124,-16.791349089629,0.));
#189268=CARTESIAN_POINT('Ctrl Pts',(18.4615758042305,-16.8148201995472,
0.));
#189269=CARTESIAN_POINT('Ctrl Pts',(18.4711835548622,-16.8383881879707,
0.));
#189270=CARTESIAN_POINT('Ctrl Pts',(18.4807654268769,-16.8620526977169,
0.));
#189271=CARTESIAN_POINT('Ctrl Pts',(18.4903209902226,-16.8858133733086,
0.));
#189272=CARTESIAN_POINT('Ctrl Pts',(18.4998498184619,-16.9096698606942,
0.));
#189273=CARTESIAN_POINT('Ctrl Pts',(18.5093514883835,-16.9336218069353,
0.));
#189274=CARTESIAN_POINT('Ctrl Pts',(18.518825579666,-16.957668859934,0.));
#189275=CARTESIAN_POINT('Ctrl Pts',(18.5282716744198,-16.9818106680382,
0.));
#189276=CARTESIAN_POINT('Ctrl Pts',(18.5376893576961,-17.0060468805099,
0.));
#189277=CARTESIAN_POINT('Ctrl Pts',(18.5470782182089,-17.030377148174,0.));
#189278=CARTESIAN_POINT('Ctrl Pts',(18.5564378489628,-17.0548011239751,
0.));
#189279=CARTESIAN_POINT('Ctrl Pts',(18.5657678479788,-17.0793184636079,
0.));
#189280=CARTESIAN_POINT('Ctrl Pts',(18.5750678188543,-17.1039288260002,
0.));
#189281=CARTESIAN_POINT('Ctrl Pts',(18.5843373717253,-17.1286318741185,
0.));
#189282=CARTESIAN_POINT('Ctrl Pts',(18.5935761222833,-17.1534272741646,
0.));
#189283=CARTESIAN_POINT('Ctrl Pts',(18.6027836898826,-17.1783146940131,
0.));
#189284=CARTESIAN_POINT('Ctrl Pts',(18.6119596959957,-17.2032938019288,
0.));
#189285=CARTESIAN_POINT('Ctrl Pts',(18.6211037624041,-17.2283642650519,
0.));
#189286=CARTESIAN_POINT('Ctrl Pts',(18.630215509794,-17.2535257482186,0.));
#189287=CARTESIAN_POINT('Ctrl Pts',(18.639294555474,-17.278777912021,0.));
#189288=CARTESIAN_POINT('Ctrl Pts',(18.6483405141853,-17.3041204135069,
0.));
#189289=CARTESIAN_POINT('Ctrl Pts',(18.6573530024019,-17.3295529098612,
0.));
#189290=CARTESIAN_POINT('Ctrl Pts',(18.6663316416569,-17.3550750612438,
0.));
#189291=CARTESIAN_POINT('Ctrl Pts',(18.6752760624045,-17.3806865340744,
0.));
#189292=CARTESIAN_POINT('Ctrl Pts',(18.6841859073472,-17.4063870038563,
0.));
#189293=CARTESIAN_POINT('Ctrl Pts',(18.6930608357421,-17.4321761588148,
0.));
#189294=CARTESIAN_POINT('Ctrl Pts',(18.7019005250322,-17.4580537012764,
0.));
#189295=CARTESIAN_POINT('Ctrl Pts',(18.7107046613941,-17.4840193397176,
0.));
#189296=CARTESIAN_POINT('Ctrl Pts',(18.7194729318127,-17.5100727820891,
0.));
#189297=CARTESIAN_POINT('Ctrl Pts',(18.728205015716,-17.5362137287604,0.));
#189298=CARTESIAN_POINT('Ctrl Pts',(18.7369005764558,-17.5624418653248,
0.));
#189299=CARTESIAN_POINT('Ctrl Pts',(18.7455592536667,-17.5887568561361,
0.));
#189300=CARTESIAN_POINT('Ctrl Pts',(18.7541806530935,-17.6151583356989,
0.));
#189301=CARTESIAN_POINT('Ctrl Pts',(18.7627643613139,-17.6416459210646,
0.));
#189302=CARTESIAN_POINT('Ctrl Pts',(18.7713099642673,-17.6682192274197,
0.));
#189303=CARTESIAN_POINT('Ctrl Pts',(18.7798170641305,-17.6948778822982,
0.));
#189304=CARTESIAN_POINT('Ctrl Pts',(18.7882852976016,-17.7216215409019,
0.));
#189305=CARTESIAN_POINT('Ctrl Pts',(18.7967143519444,-17.7484498996916,
0.));
#189306=CARTESIAN_POINT('Ctrl Pts',(18.8051039860543,-17.7753627137898,
0.));
#189307=CARTESIAN_POINT('Ctrl Pts',(18.8134540340581,-17.8023598011135,
0.));
#189308=CARTESIAN_POINT('Ctrl Pts',(18.8217643886368,-17.8294410311105,
0.));
#189309=CARTESIAN_POINT('Ctrl Pts',(18.8300349896187,-17.8566063174871,
0.));
#189310=CARTESIAN_POINT('Ctrl Pts',(18.8366196462746,-17.8784057509434,
0.));
#189311=CARTESIAN_POINT('Ctrl Pts',(18.8415402351882,-17.8947931177853,
0.));
#189312=CARTESIAN_POINT('Ctrl Pts',(18.8448126709726,-17.9057348246611,
0.));
#189313=CARTESIAN_POINT('Ctrl Pts',(18.8464468996588,-17.9112098770111,
0.));
#189314=CARTESIAN_POINT('',(18.8464468996588,-17.9112098770111,0.));
#189315=CARTESIAN_POINT('Origin',(12.1729687575668,-17.7219872369693,0.));
#189316=CARTESIAN_POINT('',(12.7689476255362,-18.5896416359912,0.));
#189317=CARTESIAN_POINT('',(12.7689476255362,-18.5896416359912,0.));
#189318=CARTESIAN_POINT('',(6.08648437878337,-8.86099361848466,0.));
#189319=CARTESIAN_POINT('Ctrl Pts',(17.9112098770111,-18.8464468996588,
0.));
#189320=CARTESIAN_POINT('Ctrl Pts',(17.9112098770111,-18.8464468996588,
12.));
#189321=CARTESIAN_POINT('Ctrl Pts',(17.9057348246595,-18.8448126709692,
0.));
#189322=CARTESIAN_POINT('Ctrl Pts',(17.9057348246595,-18.8448126709692,
12.));
#189323=CARTESIAN_POINT('Ctrl Pts',(17.8947931177807,-18.8415402351786,
0.));
#189324=CARTESIAN_POINT('Ctrl Pts',(17.8947931177807,-18.8415402351786,
12.));
#189325=CARTESIAN_POINT('Ctrl Pts',(17.8784057509355,-18.8366196462581,
0.));
#189326=CARTESIAN_POINT('Ctrl Pts',(17.8784057509355,-18.8366196462581,
12.));
#189327=CARTESIAN_POINT('Ctrl Pts',(17.856606317477,-18.8300349895974,0.));
#189328=CARTESIAN_POINT('Ctrl Pts',(17.856606317477,-18.8300349895974,12.));
#189329=CARTESIAN_POINT('Ctrl Pts',(17.8294410311006,-18.8217643886157,
0.));
#189330=CARTESIAN_POINT('Ctrl Pts',(17.8294410311006,-18.8217643886157,
12.));
#189331=CARTESIAN_POINT('Ctrl Pts',(17.8023598011057,-18.8134540340417,
0.));
#189332=CARTESIAN_POINT('Ctrl Pts',(17.8023598011057,-18.8134540340417,
12.));
#189333=CARTESIAN_POINT('Ctrl Pts',(17.7753627137853,-18.8051039860448,
0.));
#189334=CARTESIAN_POINT('Ctrl Pts',(17.7753627137853,-18.8051039860448,
12.));
#189335=CARTESIAN_POINT('Ctrl Pts',(17.7484498996905,-18.7967143519419,
0.));
#189336=CARTESIAN_POINT('Ctrl Pts',(17.7484498996905,-18.7967143519419,
12.));
#189337=CARTESIAN_POINT('Ctrl Pts',(17.7216215409035,-18.788285297605,0.));
#189338=CARTESIAN_POINT('Ctrl Pts',(17.7216215409035,-18.788285297605,12.));
#189339=CARTESIAN_POINT('Ctrl Pts',(17.6948778823014,-18.7798170641374,
0.));
#189340=CARTESIAN_POINT('Ctrl Pts',(17.6948778823014,-18.7798170641374,
12.));
#189341=CARTESIAN_POINT('Ctrl Pts',(17.6682192274236,-18.7713099642754,
0.));
#189342=CARTESIAN_POINT('Ctrl Pts',(17.6682192274236,-18.7713099642754,
12.));
#189343=CARTESIAN_POINT('Ctrl Pts',(17.6416459210681,-18.762764361321,0.));
#189344=CARTESIAN_POINT('Ctrl Pts',(17.6416459210681,-18.762764361321,12.));
#189345=CARTESIAN_POINT('Ctrl Pts',(17.6151583357012,-18.7541806530984,
0.));
#189346=CARTESIAN_POINT('Ctrl Pts',(17.6151583357012,-18.7541806530984,
12.));
#189347=CARTESIAN_POINT('Ctrl Pts',(17.5887568561371,-18.7455592536688,
0.));
#189348=CARTESIAN_POINT('Ctrl Pts',(17.5887568561371,-18.7455592536688,
12.));
#189349=CARTESIAN_POINT('Ctrl Pts',(17.5624418653245,-18.7369005764553,
0.));
#189350=CARTESIAN_POINT('Ctrl Pts',(17.5624418653245,-18.7369005764553,
12.));
#189351=CARTESIAN_POINT('Ctrl Pts',(17.5362137287593,-18.7282050157138,
0.));
#189352=CARTESIAN_POINT('Ctrl Pts',(17.5362137287593,-18.7282050157138,
12.));
#189353=CARTESIAN_POINT('Ctrl Pts',(17.5100727820876,-18.7194729318098,
0.));
#189354=CARTESIAN_POINT('Ctrl Pts',(17.5100727820876,-18.7194729318098,
12.));
#189355=CARTESIAN_POINT('Ctrl Pts',(17.4840193397162,-18.7107046613912,
0.));
#189356=CARTESIAN_POINT('Ctrl Pts',(17.4840193397162,-18.7107046613912,
12.));
#189357=CARTESIAN_POINT('Ctrl Pts',(17.4580537012753,-18.70190052503,0.));
#189358=CARTESIAN_POINT('Ctrl Pts',(17.4580537012753,-18.70190052503,12.));
#189359=CARTESIAN_POINT('Ctrl Pts',(17.4321761588142,-18.6930608357409,
0.));
#189360=CARTESIAN_POINT('Ctrl Pts',(17.4321761588142,-18.6930608357409,
12.));
#189361=CARTESIAN_POINT('Ctrl Pts',(17.4063870038562,-18.6841859073471,
0.));
#189362=CARTESIAN_POINT('Ctrl Pts',(17.4063870038562,-18.6841859073471,
12.));
#189363=CARTESIAN_POINT('Ctrl Pts',(17.3806865340747,-18.6752760624052,
0.));
#189364=CARTESIAN_POINT('Ctrl Pts',(17.3806865340747,-18.6752760624052,
12.));
#189365=CARTESIAN_POINT('Ctrl Pts',(17.3550750612443,-18.6663316416582,
0.));
#189366=CARTESIAN_POINT('Ctrl Pts',(17.3550750612443,-18.6663316416582,
12.));
#189367=CARTESIAN_POINT('Ctrl Pts',(17.3295529098618,-18.6573530024033,
0.));
#189368=CARTESIAN_POINT('Ctrl Pts',(17.3295529098618,-18.6573530024033,
12.));
#189369=CARTESIAN_POINT('Ctrl Pts',(17.3041204135074,-18.6483405141865,
0.));
#189370=CARTESIAN_POINT('Ctrl Pts',(17.3041204135074,-18.6483405141865,
12.));
#189371=CARTESIAN_POINT('Ctrl Pts',(17.2787779120213,-18.6392945554748,
0.));
#189372=CARTESIAN_POINT('Ctrl Pts',(17.2787779120213,-18.6392945554748,
12.));
#189373=CARTESIAN_POINT('Ctrl Pts',(17.2535257482187,-18.6302155097943,
0.));
#189374=CARTESIAN_POINT('Ctrl Pts',(17.2535257482187,-18.6302155097943,
12.));
#189375=CARTESIAN_POINT('Ctrl Pts',(17.2283642650517,-18.6211037624038,
0.));
#189376=CARTESIAN_POINT('Ctrl Pts',(17.2283642650517,-18.6211037624038,
12.));
#189377=CARTESIAN_POINT('Ctrl Pts',(17.2032938019284,-18.6119596959949,
0.));
#189378=CARTESIAN_POINT('Ctrl Pts',(17.2032938019284,-18.6119596959949,
12.));
#189379=CARTESIAN_POINT('Ctrl Pts',(17.1783146940127,-18.6027836898817,
0.));
#189380=CARTESIAN_POINT('Ctrl Pts',(17.1783146940127,-18.6027836898817,
12.));
#189381=CARTESIAN_POINT('Ctrl Pts',(17.1534272741643,-18.5935761222825,
0.));
#189382=CARTESIAN_POINT('Ctrl Pts',(17.1534272741643,-18.5935761222825,
12.));
#189383=CARTESIAN_POINT('Ctrl Pts',(17.1286318741183,-18.5843373717247,
0.));
#189384=CARTESIAN_POINT('Ctrl Pts',(17.1286318741183,-18.5843373717247,
12.));
#189385=CARTESIAN_POINT('Ctrl Pts',(17.1039288260001,-18.5750678188542,
0.));
#189386=CARTESIAN_POINT('Ctrl Pts',(17.1039288260001,-18.5750678188542,
12.));
#189387=CARTESIAN_POINT('Ctrl Pts',(17.0793184636079,-18.5657678479789,
0.));
#189388=CARTESIAN_POINT('Ctrl Pts',(17.0793184636079,-18.5657678479789,
12.));
#189389=CARTESIAN_POINT('Ctrl Pts',(17.0548011239751,-18.556437848963,0.));
#189390=CARTESIAN_POINT('Ctrl Pts',(17.0548011239751,-18.556437848963,12.));
#189391=CARTESIAN_POINT('Ctrl Pts',(17.0303771481738,-18.547078218209,0.));
#189392=CARTESIAN_POINT('Ctrl Pts',(17.0303771481738,-18.547078218209,12.));
#189393=CARTESIAN_POINT('Ctrl Pts',(17.0060468805097,-18.5376893576961,
0.));
#189394=CARTESIAN_POINT('Ctrl Pts',(17.0060468805097,-18.5376893576961,
12.));
#189395=CARTESIAN_POINT('Ctrl Pts',(16.981810668038,-18.5282716744197,0.));
#189396=CARTESIAN_POINT('Ctrl Pts',(16.981810668038,-18.5282716744197,12.));
#189397=CARTESIAN_POINT('Ctrl Pts',(16.9576688599339,-18.5188255796659,
0.));
#189398=CARTESIAN_POINT('Ctrl Pts',(16.9576688599339,-18.5188255796659,
12.));
#189399=CARTESIAN_POINT('Ctrl Pts',(16.9336218069353,-18.5093514883835,
0.));
#189400=CARTESIAN_POINT('Ctrl Pts',(16.9336218069353,-18.5093514883835,
12.));
#189401=CARTESIAN_POINT('Ctrl Pts',(16.9096698606943,-18.499849818462,0.));
#189402=CARTESIAN_POINT('Ctrl Pts',(16.9096698606943,-18.499849818462,12.));
#189403=CARTESIAN_POINT('Ctrl Pts',(16.8858133733088,-18.4903209902227,
0.));
#189404=CARTESIAN_POINT('Ctrl Pts',(16.8858133733088,-18.4903209902227,
12.));
#189405=CARTESIAN_POINT('Ctrl Pts',(16.8620526977171,-18.4807654268771,
0.));
#189406=CARTESIAN_POINT('Ctrl Pts',(16.8620526977171,-18.4807654268771,
12.));
#189407=CARTESIAN_POINT('Ctrl Pts',(16.8383881879709,-18.4711835548623,
0.));
#189408=CARTESIAN_POINT('Ctrl Pts',(16.8383881879709,-18.4711835548623,
12.));
#189409=CARTESIAN_POINT('Ctrl Pts',(16.8148201995472,-18.4615758042305,
0.));
#189410=CARTESIAN_POINT('Ctrl Pts',(16.8148201995472,-18.4615758042305,
12.));
#189411=CARTESIAN_POINT('Ctrl Pts',(16.791349089629,-18.4519426090124,0.));
#189412=CARTESIAN_POINT('Ctrl Pts',(16.791349089629,-18.4519426090124,12.));
#189413=CARTESIAN_POINT('Ctrl Pts',(16.7679752173992,-18.44228440761,0.));
#189414=CARTESIAN_POINT('Ctrl Pts',(16.7679752173992,-18.44228440761,12.));
#189415=CARTESIAN_POINT('Ctrl Pts',(16.7446989442882,-18.4326016431392,
0.));
#189416=CARTESIAN_POINT('Ctrl Pts',(16.7446989442882,-18.4326016431392,
12.));
#189417=CARTESIAN_POINT('Ctrl Pts',(16.7215206338818,-18.4228947633187,
0.));
#189418=CARTESIAN_POINT('Ctrl Pts',(16.7215206338818,-18.4228947633187,
12.));
#189419=CARTESIAN_POINT('Ctrl Pts',(16.698440651849,-18.413164220399,0.));
#189420=CARTESIAN_POINT('Ctrl Pts',(16.698440651849,-18.413164220399,12.));
#189421=CARTESIAN_POINT('Ctrl Pts',(16.6754593658513,-18.403410471079,0.));
#189422=CARTESIAN_POINT('Ctrl Pts',(16.6754593658513,-18.403410471079,12.));
#189423=CARTESIAN_POINT('Ctrl Pts',(16.6525771454513,-18.3936339764332,
0.));
#189424=CARTESIAN_POINT('Ctrl Pts',(16.6525771454513,-18.3936339764332,
12.));
#189425=CARTESIAN_POINT('Ctrl Pts',(16.6297943620056,-18.3838352018327,
0.));
#189426=CARTESIAN_POINT('Ctrl Pts',(16.6297943620056,-18.3838352018327,
12.));
#189427=CARTESIAN_POINT('Ctrl Pts',(16.607111388571,-18.3740146168879,0.));
#189428=CARTESIAN_POINT('Ctrl Pts',(16.607111388571,-18.3740146168879,12.));
#189429=CARTESIAN_POINT('Ctrl Pts',(16.5845286000217,-18.3641726955889,
0.));
#189430=CARTESIAN_POINT('Ctrl Pts',(16.5845286000217,-18.3641726955889,
12.));
#189431=CARTESIAN_POINT('Ctrl Pts',(16.5620463731413,-18.354309916433,0.));
#189432=CARTESIAN_POINT('Ctrl Pts',(16.5620463731413,-18.354309916433,12.));
#189433=CARTESIAN_POINT('Ctrl Pts',(16.5396650867139,-18.34442676256,0.));
#189434=CARTESIAN_POINT('Ctrl Pts',(16.5396650867139,-18.34442676256,12.));
#189435=CARTESIAN_POINT('Ctrl Pts',(16.5173851216045,-18.3345237218864,
0.));
#189436=CARTESIAN_POINT('Ctrl Pts',(16.5173851216045,-18.3345237218864,
12.));
#189437=CARTESIAN_POINT('Ctrl Pts',(16.4952068608345,-18.3246012872469,
0.));
#189438=CARTESIAN_POINT('Ctrl Pts',(16.4952068608345,-18.3246012872469,
12.));
#189439=CARTESIAN_POINT('Ctrl Pts',(16.4731306896441,-18.3146599565231,
0.));
#189440=CARTESIAN_POINT('Ctrl Pts',(16.4731306896441,-18.3146599565231,
12.));
#189441=CARTESIAN_POINT('Ctrl Pts',(16.4511569955233,-18.304700232686,0.));
#189442=CARTESIAN_POINT('Ctrl Pts',(16.4511569955233,-18.304700232686,12.));
#189443=CARTESIAN_POINT('Ctrl Pts',(16.4292861682378,-18.294722623851,0.));
#189444=CARTESIAN_POINT('Ctrl Pts',(16.4292861682378,-18.294722623851,12.));
#189445=CARTESIAN_POINT('Ctrl Pts',(16.4075185998454,-18.2847276433309,
0.));
#189446=CARTESIAN_POINT('Ctrl Pts',(16.4075185998454,-18.2847276433309,
12.));
#189447=CARTESIAN_POINT('Ctrl Pts',(16.385854684708,-18.2747158096934,0.));
#189448=CARTESIAN_POINT('Ctrl Pts',(16.385854684708,-18.2747158096934,12.));
#189449=CARTESIAN_POINT('Ctrl Pts',(16.3642948194868,-18.2646876468169,
0.));
#189450=CARTESIAN_POINT('Ctrl Pts',(16.3642948194868,-18.2646876468169,
12.));
#189451=CARTESIAN_POINT('Ctrl Pts',(16.3428394031589,-18.2546436839608,
0.));
#189452=CARTESIAN_POINT('Ctrl Pts',(16.3428394031589,-18.2546436839608,
12.));
#189453=CARTESIAN_POINT('Ctrl Pts',(16.3214888370987,-18.2445844558742,
0.));
#189454=CARTESIAN_POINT('Ctrl Pts',(16.3214888370987,-18.2445844558742,
12.));
#189455=CARTESIAN_POINT('Ctrl Pts',(16.3002435251378,-18.2345105028982,
0.));
#189456=CARTESIAN_POINT('Ctrl Pts',(16.3002435251378,-18.2345105028982,
12.));
#189457=CARTESIAN_POINT('Ctrl Pts',(16.2791038736223,-18.2244223710746,
0.));
#189458=CARTESIAN_POINT('Ctrl Pts',(16.2791038736223,-18.2244223710746,
12.));
#189459=CARTESIAN_POINT('Ctrl Pts',(16.2580702914615,-18.2143206122529,
0.));
#189460=CARTESIAN_POINT('Ctrl Pts',(16.2580702914615,-18.2143206122529,
12.));
#189461=CARTESIAN_POINT('Ctrl Pts',(16.2371431901638,-18.2042057842035,
0.));
#189462=CARTESIAN_POINT('Ctrl Pts',(16.2371431901638,-18.2042057842035,
12.));
#189463=CARTESIAN_POINT('Ctrl Pts',(16.2163229838875,-18.1940784507229,
0.));
#189464=CARTESIAN_POINT('Ctrl Pts',(16.2163229838875,-18.1940784507229,
12.));
#189465=CARTESIAN_POINT('Ctrl Pts',(16.1956100895073,-18.1839391817331,
0.));
#189466=CARTESIAN_POINT('Ctrl Pts',(16.1956100895073,-18.1839391817331,
12.));
#189467=CARTESIAN_POINT('Ctrl Pts',(16.1750049266671,-18.1737885533849,
0.));
#189468=CARTESIAN_POINT('Ctrl Pts',(16.1750049266671,-18.1737885533849,
12.));
#189469=CARTESIAN_POINT('Ctrl Pts',(16.154507917826,-18.1636271481615,0.));
#189470=CARTESIAN_POINT('Ctrl Pts',(16.154507917826,-18.1636271481615,12.));
#189471=CARTESIAN_POINT('Ctrl Pts',(16.1341194882988,-18.1534555549853,
0.));
#189472=CARTESIAN_POINT('Ctrl Pts',(16.1341194882988,-18.1534555549853,
12.));
#189473=CARTESIAN_POINT('Ctrl Pts',(16.1138400662794,-18.1432743693235,
0.));
#189474=CARTESIAN_POINT('Ctrl Pts',(16.1138400662794,-18.1432743693235,
12.));
#189475=CARTESIAN_POINT('Ctrl Pts',(16.0936700829112,-18.1330841933105,
0.));
#189476=CARTESIAN_POINT('Ctrl Pts',(16.0936700829112,-18.1330841933105,
12.));
#189477=CARTESIAN_POINT('Ctrl Pts',(16.0736099723668,-18.1228856358751,
0.));
#189478=CARTESIAN_POINT('Ctrl Pts',(16.0736099723668,-18.1228856358751,
12.));
#189479=CARTESIAN_POINT('Ctrl Pts',(16.0536601719125,-18.112679312869,0.));
#189480=CARTESIAN_POINT('Ctrl Pts',(16.0536601719125,-18.112679312869,12.));
#189481=CARTESIAN_POINT('Ctrl Pts',(16.0338211219693,-18.1024658471966,
0.));
#189482=CARTESIAN_POINT('Ctrl Pts',(16.0338211219693,-18.1024658471966,
12.));
#189483=CARTESIAN_POINT('Ctrl Pts',(16.014093266161,-18.0922458689462,0.));
#189484=CARTESIAN_POINT('Ctrl Pts',(16.014093266161,-18.0922458689462,12.));
#189485=CARTESIAN_POINT('Ctrl Pts',(15.9944770513613,-18.0820200155236,
0.));
#189486=CARTESIAN_POINT('Ctrl Pts',(15.9944770513613,-18.0820200155236,
12.));
#189487=CARTESIAN_POINT('Ctrl Pts',(15.9749729277846,-18.0717889317958,
0.));
#189488=CARTESIAN_POINT('Ctrl Pts',(15.9749729277846,-18.0717889317958,
12.));
#189489=CARTESIAN_POINT('Ctrl Pts',(15.9555813490644,-18.061553270236,0.));
#189490=CARTESIAN_POINT('Ctrl Pts',(15.9555813490644,-18.061553270236,12.));
#189491=CARTESIAN_POINT('Ctrl Pts',(15.9363027723244,-18.0513136910691,
0.));
#189492=CARTESIAN_POINT('Ctrl Pts',(15.9363027723244,-18.0513136910691,
12.));
#189493=CARTESIAN_POINT('Ctrl Pts',(15.9171376582436,-18.0410708624209,
0.));
#189494=CARTESIAN_POINT('Ctrl Pts',(15.9171376582436,-18.0410708624209,
12.));
#189495=CARTESIAN_POINT('Ctrl Pts',(15.8980864711042,-18.0308254604636,
0.));
#189496=CARTESIAN_POINT('Ctrl Pts',(15.8980864711042,-18.0308254604636,
12.));
#189497=CARTESIAN_POINT('Ctrl Pts',(15.8791496788682,-18.0205781695769,
0.));
#189498=CARTESIAN_POINT('Ctrl Pts',(15.8791496788682,-18.0205781695769,
12.));
#189499=CARTESIAN_POINT('Ctrl Pts',(15.8603277532831,-18.0103296825205,
0.));
#189500=CARTESIAN_POINT('Ctrl Pts',(15.8603277532831,-18.0103296825205,
12.));
#189501=CARTESIAN_POINT('Ctrl Pts',(15.8416211699679,-18.0000807006052,
0.));
#189502=CARTESIAN_POINT('Ctrl Pts',(15.8416211699679,-18.0000807006052,
12.));
#189503=CARTESIAN_POINT('Ctrl Pts',(15.8230304084962,-17.9898319338665,
0.));
#189504=CARTESIAN_POINT('Ctrl Pts',(15.8230304084962,-17.9898319338665,
12.));
#189505=CARTESIAN_POINT('Ctrl Pts',(15.8045559524676,-17.9795841012386,
0.));
#189506=CARTESIAN_POINT('Ctrl Pts',(15.8045559524676,-17.9795841012386,
12.));
#189507=CARTESIAN_POINT('Ctrl Pts',(15.7861982895724,-17.9693379307303,
0.));
#189508=CARTESIAN_POINT('Ctrl Pts',(15.7861982895724,-17.9693379307303,
12.));
#189509=CARTESIAN_POINT('Ctrl Pts',(15.7679579117077,-17.9590941596242,
0.));
#189510=CARTESIAN_POINT('Ctrl Pts',(15.7679579117077,-17.9590941596242,
12.));
#189511=CARTESIAN_POINT('Ctrl Pts',(15.749835315086,-17.9488535346781,0.));
#189512=CARTESIAN_POINT('Ctrl Pts',(15.749835315086,-17.9488535346781,12.));
#189513=CARTESIAN_POINT('Ctrl Pts',(15.7318310003335,-17.9386168123262,
0.));
#189514=CARTESIAN_POINT('Ctrl Pts',(15.7318310003335,-17.9386168123262,
12.));
#189515=CARTESIAN_POINT('Ctrl Pts',(15.7139454725838,-17.9283847588836,
0.));
#189516=CARTESIAN_POINT('Ctrl Pts',(15.7139454725838,-17.9283847588836,
12.));
#189517=CARTESIAN_POINT('Ctrl Pts',(15.6961792415522,-17.9181581507455,
0.));
#189518=CARTESIAN_POINT('Ctrl Pts',(15.6961792415522,-17.9181581507455,
12.));
#189519=CARTESIAN_POINT('Ctrl Pts',(15.678532821646,-17.9079377746111,0.));
#189520=CARTESIAN_POINT('Ctrl Pts',(15.678532821646,-17.9079377746111,12.));
#189521=CARTESIAN_POINT('Ctrl Pts',(15.661006732103,-17.897724427724,0.));
#189522=CARTESIAN_POINT('Ctrl Pts',(15.661006732103,-17.897724427724,12.));
#189523=CARTESIAN_POINT('Ctrl Pts',(15.6436014971084,-17.8875189181091,
0.));
#189524=CARTESIAN_POINT('Ctrl Pts',(15.6436014971084,-17.8875189181091,
12.));
#189525=CARTESIAN_POINT('Ctrl Pts',(15.6263176459108,-17.8773220648125,
0.));
#189526=CARTESIAN_POINT('Ctrl Pts',(15.6263176459108,-17.8773220648125,
12.));
#189527=CARTESIAN_POINT('Ctrl Pts',(15.609155712921,-17.8671346981394,0.));
#189528=CARTESIAN_POINT('Ctrl Pts',(15.609155712921,-17.8671346981394,12.));
#189529=CARTESIAN_POINT('Ctrl Pts',(15.5921162378192,-17.8569576599006,
0.));
#189530=CARTESIAN_POINT('Ctrl Pts',(15.5921162378192,-17.8569576599006,
12.));
#189531=CARTESIAN_POINT('Ctrl Pts',(15.5751997657162,-17.8467918036987,
0.));
#189532=CARTESIAN_POINT('Ctrl Pts',(15.5751997657162,-17.8467918036987,
12.));
#189533=CARTESIAN_POINT('Ctrl Pts',(15.5584068472982,-17.8366379952085,
0.));
#189534=CARTESIAN_POINT('Ctrl Pts',(15.5584068472982,-17.8366379952085,
12.));
#189535=CARTESIAN_POINT('Ctrl Pts',(15.541738038964,-17.8264971124607,0.));
#189536=CARTESIAN_POINT('Ctrl Pts',(15.541738038964,-17.8264971124607,12.));
#189537=CARTESIAN_POINT('Ctrl Pts',(15.5251939029552,-17.8163700461256,
0.));
#189538=CARTESIAN_POINT('Ctrl Pts',(15.5251939029552,-17.8163700461256,
12.));
#189539=CARTESIAN_POINT('Ctrl Pts',(15.5087750074718,-17.8062576997952,
0.));
#189540=CARTESIAN_POINT('Ctrl Pts',(15.5087750074718,-17.8062576997952,
12.));
#189541=CARTESIAN_POINT('Ctrl Pts',(15.4924819268517,-17.7961609903148,
0.));
#189542=CARTESIAN_POINT('Ctrl Pts',(15.4924819268517,-17.7961609903148,
12.));
#189543=CARTESIAN_POINT('Ctrl Pts',(15.4763152417497,-17.786080848122,0.));
#189544=CARTESIAN_POINT('Ctrl Pts',(15.4763152417497,-17.786080848122,12.));
#189545=CARTESIAN_POINT('Ctrl Pts',(15.4602755393017,-17.7760182175815,
0.));
#189546=CARTESIAN_POINT('Ctrl Pts',(15.4602755393017,-17.7760182175815,
12.));
#189547=CARTESIAN_POINT('Ctrl Pts',(15.4443634132869,-17.7659740573265,
0.));
#189548=CARTESIAN_POINT('Ctrl Pts',(15.4443634132869,-17.7659740573265,
12.));
#189549=CARTESIAN_POINT('Ctrl Pts',(15.4285794642667,-17.7559493405881,
0.));
#189550=CARTESIAN_POINT('Ctrl Pts',(15.4285794642667,-17.7559493405881,
12.));
#189551=CARTESIAN_POINT('Ctrl Pts',(15.4129242997837,-17.7459450555813,
0.));
#189552=CARTESIAN_POINT('Ctrl Pts',(15.4129242997837,-17.7459450555813,
12.));
#189553=CARTESIAN_POINT('Ctrl Pts',(15.3973985345802,-17.735962205915,0.));
#189554=CARTESIAN_POINT('Ctrl Pts',(15.3973985345802,-17.735962205915,12.));
#189555=CARTESIAN_POINT('Ctrl Pts',(15.3820027907966,-17.7260018109924,
0.));
#189556=CARTESIAN_POINT('Ctrl Pts',(15.3820027907966,-17.7260018109924,
12.));
#189557=CARTESIAN_POINT('Ctrl Pts',(15.3667376981699,-17.7160649064206,
0.));
#189558=CARTESIAN_POINT('Ctrl Pts',(15.3667376981699,-17.7160649064206,
12.));
#189559=CARTESIAN_POINT('Ctrl Pts',(15.351603894206,-17.7061525444042,0.));
#189560=CARTESIAN_POINT('Ctrl Pts',(15.351603894206,-17.7061525444042,12.));
#189561=CARTESIAN_POINT('Ctrl Pts',(15.3366020244066,-17.6962657941983,
0.));
#189562=CARTESIAN_POINT('Ctrl Pts',(15.3366020244066,-17.6962657941983,
12.));
#189563=CARTESIAN_POINT('Ctrl Pts',(15.3217327425338,-17.6864057426052,
0.));
#189564=CARTESIAN_POINT('Ctrl Pts',(15.3217327425338,-17.6864057426052,
12.));
#189565=CARTESIAN_POINT('Ctrl Pts',(15.30699671085,-17.676573494456,0.));
#189566=CARTESIAN_POINT('Ctrl Pts',(15.30699671085,-17.676573494456,12.));
#189567=CARTESIAN_POINT('Ctrl Pts',(15.2923946003598,-17.6667701731041,
0.));
#189568=CARTESIAN_POINT('Ctrl Pts',(15.2923946003598,-17.6667701731041,
12.));
#189569=CARTESIAN_POINT('Ctrl Pts',(15.2779270910239,-17.6569969209,0.));
#189570=CARTESIAN_POINT('Ctrl Pts',(15.2779270910239,-17.6569969209,12.));
#189571=CARTESIAN_POINT('Ctrl Pts',(15.2635948720292,-17.6472548997328,
0.));
#189572=CARTESIAN_POINT('Ctrl Pts',(15.2635948720292,-17.6472548997328,
12.));
#189573=CARTESIAN_POINT('Ctrl Pts',(15.2493986421092,-17.6375452916369,
0.));
#189574=CARTESIAN_POINT('Ctrl Pts',(15.2493986421092,-17.6375452916369,
12.));
#189575=CARTESIAN_POINT('Ctrl Pts',(15.2353391098366,-17.6278692993764,
0.));
#189576=CARTESIAN_POINT('Ctrl Pts',(15.2353391098366,-17.6278692993764,
12.));
#189577=CARTESIAN_POINT('Ctrl Pts',(15.2214169939199,-17.6182281470468,
0.));
#189578=CARTESIAN_POINT('Ctrl Pts',(15.2214169939199,-17.6182281470468,
12.));
#189579=CARTESIAN_POINT('Ctrl Pts',(15.2076330234686,-17.60862308065,0.));
#189580=CARTESIAN_POINT('Ctrl Pts',(15.2076330234686,-17.60862308065,12.));
#189581=CARTESIAN_POINT('Ctrl Pts',(15.1939879383268,-17.5990553687599,
0.));
#189582=CARTESIAN_POINT('Ctrl Pts',(15.1939879383268,-17.5990553687599,
12.));
#189583=CARTESIAN_POINT('Ctrl Pts',(15.1804824894605,-17.5895263032595,
0.));
#189584=CARTESIAN_POINT('Ctrl Pts',(15.1804824894605,-17.5895263032595,
12.));
#189585=CARTESIAN_POINT('Ctrl Pts',(15.1671174393137,-17.580037200054,0.));
#189586=CARTESIAN_POINT('Ctrl Pts',(15.1671174393137,-17.580037200054,12.));
#189587=CARTESIAN_POINT('Ctrl Pts',(15.1538935621714,-17.5705893998029,
0.));
#189588=CARTESIAN_POINT('Ctrl Pts',(15.1538935621714,-17.5705893998029,
12.));
#189589=CARTESIAN_POINT('Ctrl Pts',(15.1408116444876,-17.5611842686192,
0.));
#189590=CARTESIAN_POINT('Ctrl Pts',(15.1408116444876,-17.5611842686192,
12.));
#189591=CARTESIAN_POINT('Ctrl Pts',(15.1278724853138,-17.5518231989117,
0.));
#189592=CARTESIAN_POINT('Ctrl Pts',(15.1278724853138,-17.5518231989117,
12.));
#189593=CARTESIAN_POINT('Ctrl Pts',(15.1150768967728,-17.5425076102963,
0.));
#189594=CARTESIAN_POINT('Ctrl Pts',(15.1150768967728,-17.5425076102963,
12.));
#189595=CARTESIAN_POINT('Ctrl Pts',(15.1024257045033,-17.5332389504829,
0.));
#189596=CARTESIAN_POINT('Ctrl Pts',(15.1024257045033,-17.5332389504829,
12.));
#189597=CARTESIAN_POINT('Ctrl Pts',(15.0899197481082,-17.5240186961791,
0.));
#189598=CARTESIAN_POINT('Ctrl Pts',(15.0899197481082,-17.5240186961791,
12.));
#189599=CARTESIAN_POINT('Ctrl Pts',(15.0775598815749,-17.5148483539687,
0.));
#189600=CARTESIAN_POINT('Ctrl Pts',(15.0775598815749,-17.5148483539687,
12.));
#189601=CARTESIAN_POINT('Ctrl Pts',(15.0653469738307,-17.5057294613877,
0.));
#189602=CARTESIAN_POINT('Ctrl Pts',(15.0653469738307,-17.5057294613877,
12.));
#189603=CARTESIAN_POINT('Ctrl Pts',(15.0532819093085,-17.4966635880246,
0.));
#189604=CARTESIAN_POINT('Ctrl Pts',(15.0532819093085,-17.4966635880246,
12.));
#189605=CARTESIAN_POINT('Ctrl Pts',(15.0413655884993,-17.4876523366178,
0.));
#189606=CARTESIAN_POINT('Ctrl Pts',(15.0413655884993,-17.4876523366178,
12.));
#189607=CARTESIAN_POINT('Ctrl Pts',(15.029598928488,-17.4786973441417,0.));
#189608=CARTESIAN_POINT('Ctrl Pts',(15.029598928488,-17.4786973441417,12.));
#189609=CARTESIAN_POINT('Ctrl Pts',(15.0179828635087,-17.4698002829357,
0.));
#189610=CARTESIAN_POINT('Ctrl Pts',(15.0179828635087,-17.4698002829357,
12.));
#189611=CARTESIAN_POINT('Ctrl Pts',(15.0065183456922,-17.4609628621419,
0.));
#189612=CARTESIAN_POINT('Ctrl Pts',(15.0065183456922,-17.4609628621419,
12.));
#189613=CARTESIAN_POINT('Ctrl Pts',(14.9952063457779,-17.4521868291005,
0.));
#189614=CARTESIAN_POINT('Ctrl Pts',(14.9952063457779,-17.4521868291005,
12.));
#189615=CARTESIAN_POINT('Ctrl Pts',(14.9840478538357,-17.4434739707773,
0.));
#189616=CARTESIAN_POINT('Ctrl Pts',(14.9840478538357,-17.4434739707773,
12.));
#189617=CARTESIAN_POINT('Ctrl Pts',(14.973043879945,-17.4348261151395,0.));
#189618=CARTESIAN_POINT('Ctrl Pts',(14.973043879945,-17.4348261151395,12.));
#189619=CARTESIAN_POINT('Ctrl Pts',(14.9621954549825,-17.4262451327088,
0.));
#189620=CARTESIAN_POINT('Ctrl Pts',(14.9621954549825,-17.4262451327088,
12.));
#189621=CARTESIAN_POINT('Ctrl Pts',(14.9515036315142,-17.4177329382827,
0.));
#189622=CARTESIAN_POINT('Ctrl Pts',(14.9515036315142,-17.4177329382827,
12.));
#189623=CARTESIAN_POINT('Ctrl Pts',(14.940969484645,-17.4092914926072,0.));
#189624=CARTESIAN_POINT('Ctrl Pts',(14.940969484645,-17.4092914926072,12.));
#189625=CARTESIAN_POINT('Ctrl Pts',(14.9305941128758,-17.400922804075,0.));
#189626=CARTESIAN_POINT('Ctrl Pts',(14.9305941128758,-17.400922804075,12.));
#189627=CARTESIAN_POINT('Ctrl Pts',(14.9203786389343,-17.3926289303987,
0.));
#189628=CARTESIAN_POINT('Ctrl Pts',(14.9203786389343,-17.3926289303987,
12.));
#189629=CARTESIAN_POINT('Ctrl Pts',(14.9103242110057,-17.3844119809823,
0.));
#189630=CARTESIAN_POINT('Ctrl Pts',(14.9103242110057,-17.3844119809823,
12.));
#189631=CARTESIAN_POINT('Ctrl Pts',(14.9004320039609,-17.3762741193075,
0.));
#189632=CARTESIAN_POINT('Ctrl Pts',(14.9004320039609,-17.3762741193075,
12.));
#189633=CARTESIAN_POINT('Ctrl Pts',(14.8907032205789,-17.3682175653236,
0.));
#189634=CARTESIAN_POINT('Ctrl Pts',(14.8907032205789,-17.3682175653236,
12.));
#189635=CARTESIAN_POINT('Ctrl Pts',(14.8811390927424,-17.3602445978163,
0.));
#189636=CARTESIAN_POINT('Ctrl Pts',(14.8811390927424,-17.3602445978163,
12.));
#189637=CARTESIAN_POINT('Ctrl Pts',(14.8717408826957,-17.3523575568648,
0.));
#189638=CARTESIAN_POINT('Ctrl Pts',(14.8717408826957,-17.3523575568648,
12.));
#189639=CARTESIAN_POINT('Ctrl Pts',(14.8625098843419,-17.3445588463477,
0.));
#189640=CARTESIAN_POINT('Ctrl Pts',(14.8625098843419,-17.3445588463477,
12.));
#189641=CARTESIAN_POINT('Ctrl Pts',(14.8534474245433,-17.336850936485,0.));
#189642=CARTESIAN_POINT('Ctrl Pts',(14.8534474245433,-17.336850936485,12.));
#189643=CARTESIAN_POINT('Ctrl Pts',(14.8445548643504,-17.3292363662601,
0.));
#189644=CARTESIAN_POINT('Ctrl Pts',(14.8445548643504,-17.3292363662601,
12.));
#189645=CARTESIAN_POINT('Ctrl Pts',(14.8358336004193,-17.3217177462096,
0.));
#189646=CARTESIAN_POINT('Ctrl Pts',(14.8358336004193,-17.3217177462096,
12.));
#189647=CARTESIAN_POINT('Ctrl Pts',(14.8272850675375,-17.3142977632656,
0.));
#189648=CARTESIAN_POINT('Ctrl Pts',(14.8272850675375,-17.3142977632656,
12.));
#189649=CARTESIAN_POINT('Ctrl Pts',(14.8189107410161,-17.3069791853705,
0.));
#189650=CARTESIAN_POINT('Ctrl Pts',(14.8189107410161,-17.3069791853705,
12.));
#189651=CARTESIAN_POINT('Ctrl Pts',(14.8107121391038,-17.2997648661483,
0.));
#189652=CARTESIAN_POINT('Ctrl Pts',(14.8107121391038,-17.2997648661483,
12.));
#189653=CARTESIAN_POINT('Ctrl Pts',(14.8026908254281,-17.2926577496519,
0.));
#189654=CARTESIAN_POINT('Ctrl Pts',(14.8026908254281,-17.2926577496519,
12.));
#189655=CARTESIAN_POINT('Ctrl Pts',(14.7948484105252,-17.28566087332,0.));
#189656=CARTESIAN_POINT('Ctrl Pts',(14.7948484105252,-17.28566087332,12.));
#189657=CARTESIAN_POINT('Ctrl Pts',(14.787186553128,-17.278777370485,0.));
#189658=CARTESIAN_POINT('Ctrl Pts',(14.787186553128,-17.278777370485,12.));
#189659=CARTESIAN_POINT('Ctrl Pts',(14.7797069617802,-17.2720104735192,
0.));
#189660=CARTESIAN_POINT('Ctrl Pts',(14.7797069617802,-17.2720104735192,
12.));
#189661=CARTESIAN_POINT('Ctrl Pts',(14.7724113956728,-17.2653635155317,
0.));
#189662=CARTESIAN_POINT('Ctrl Pts',(14.7724113956728,-17.2653635155317,
12.));
#189663=CARTESIAN_POINT('Ctrl Pts',(14.7653016697589,-17.2588399401464,
0.));
#189664=CARTESIAN_POINT('Ctrl Pts',(14.7653016697589,-17.2588399401464,
12.));
#189665=CARTESIAN_POINT('Ctrl Pts',(14.7583796616617,-17.2524433146837,
0.));
#189666=CARTESIAN_POINT('Ctrl Pts',(14.7583796616617,-17.2524433146837,
12.));
#189667=CARTESIAN_POINT('Ctrl Pts',(14.7516473175124,-17.2461773413289,
0.));
#189668=CARTESIAN_POINT('Ctrl Pts',(14.7516473175124,-17.2461773413289,
12.));
#189669=CARTESIAN_POINT('Ctrl Pts',(14.7451066593793,-17.2400458713566,
0.));
#189670=CARTESIAN_POINT('Ctrl Pts',(14.7451066593793,-17.2400458713566,
12.));
#189671=CARTESIAN_POINT('Ctrl Pts',(14.7387597858117,-17.2340529062078,
0.));
#189672=CARTESIAN_POINT('Ctrl Pts',(14.7387597858117,-17.2340529062078,
12.));
#189673=CARTESIAN_POINT('Ctrl Pts',(14.7326088681163,-17.2282025904314,
0.));
#189674=CARTESIAN_POINT('Ctrl Pts',(14.7326088681163,-17.2282025904314,
12.));
#189675=CARTESIAN_POINT('Ctrl Pts',(14.7266561494282,-17.2224992099666,
0.));
#189676=CARTESIAN_POINT('Ctrl Pts',(14.7266561494282,-17.2224992099666,
12.));
#189677=CARTESIAN_POINT('Ctrl Pts',(14.7209039390325,-17.2169471814255,
0.));
#189678=CARTESIAN_POINT('Ctrl Pts',(14.7209039390325,-17.2169471814255,
12.));
#189679=CARTESIAN_POINT('Ctrl Pts',(14.7153546289338,-17.2115510835988,
0.));
#189680=CARTESIAN_POINT('Ctrl Pts',(14.7153546289338,-17.2115510835988,
12.));
#189681=CARTESIAN_POINT('Ctrl Pts',(14.7100107213586,-17.2063157097316,
0.));
#189682=CARTESIAN_POINT('Ctrl Pts',(14.7100107213586,-17.2063157097316,
12.));
#189683=CARTESIAN_POINT('Ctrl Pts',(14.7048748502662,-17.2012461084268,
0.));
#189684=CARTESIAN_POINT('Ctrl Pts',(14.7048748502662,-17.2012461084268,
12.));
#189685=CARTESIAN_POINT('Ctrl Pts',(14.699949811582,-17.1963476411694,0.));
#189686=CARTESIAN_POINT('Ctrl Pts',(14.699949811582,-17.1963476411694,12.));
#189687=CARTESIAN_POINT('Ctrl Pts',(14.6952385361706,-17.1916259308416,
0.));
#189688=CARTESIAN_POINT('Ctrl Pts',(14.6952385361706,-17.1916259308416,
12.));
#189689=CARTESIAN_POINT('Ctrl Pts',(14.6907440526957,-17.1870867909918,
0.));
#189690=CARTESIAN_POINT('Ctrl Pts',(14.6907440526957,-17.1870867909918,
12.));
#189691=CARTESIAN_POINT('Ctrl Pts',(14.6864694522319,-17.182736158472,0.));
#189692=CARTESIAN_POINT('Ctrl Pts',(14.6864694522319,-17.182736158472,12.));
#189693=CARTESIAN_POINT('Ctrl Pts',(14.6824178576166,-17.1785800350827,
0.));
#189694=CARTESIAN_POINT('Ctrl Pts',(14.6824178576166,-17.1785800350827,
12.));
#189695=CARTESIAN_POINT('Ctrl Pts',(14.6785925615676,-17.1746247499057,
0.));
#189696=CARTESIAN_POINT('Ctrl Pts',(14.6785925615676,-17.1746247499057,
12.));
#189697=CARTESIAN_POINT('Ctrl Pts',(14.6749971333867,-17.1708771619129,
0.));
#189698=CARTESIAN_POINT('Ctrl Pts',(14.6749971333867,-17.1708771619129,
12.));
#189699=CARTESIAN_POINT('Ctrl Pts',(14.6716355833321,-17.1673449723019,
0.));
#189700=CARTESIAN_POINT('Ctrl Pts',(14.6716355833321,-17.1673449723019,
12.));
#189701=CARTESIAN_POINT('Ctrl Pts',(14.6685123374424,-17.1640366762304,
0.));
#189702=CARTESIAN_POINT('Ctrl Pts',(14.6685123374424,-17.1640366762304,
12.));
#189703=CARTESIAN_POINT('Ctrl Pts',(14.6656319165057,-17.1609609517369,
0.));
#189704=CARTESIAN_POINT('Ctrl Pts',(14.6656319165057,-17.1609609517369,
12.));
#189705=CARTESIAN_POINT('Ctrl Pts',(14.662998728599,-17.1581262646789,0.));
#189706=CARTESIAN_POINT('Ctrl Pts',(14.662998728599,-17.1581262646789,12.));
#189707=CARTESIAN_POINT('Ctrl Pts',(14.660616716964,-17.1555401986403,0.));
#189708=CARTESIAN_POINT('Ctrl Pts',(14.660616716964,-17.1555401986403,12.));
#189709=CARTESIAN_POINT('Ctrl Pts',(14.65849005553,-17.1532107762719,0.));
#189710=CARTESIAN_POINT('Ctrl Pts',(14.65849005553,-17.1532107762719,12.));
#189711=CARTESIAN_POINT('Ctrl Pts',(14.6566237952435,-17.1511476869495,
0.));
#189712=CARTESIAN_POINT('Ctrl Pts',(14.6566237952435,-17.1511476869495,
12.));
#189713=CARTESIAN_POINT('Ctrl Pts',(14.6550248622813,-17.1493641837556,
0.));
#189714=CARTESIAN_POINT('Ctrl Pts',(14.6550248622813,-17.1493641837556,
12.));
#189715=CARTESIAN_POINT('Ctrl Pts',(14.6537016966188,-17.1478763944909,
0.));
#189716=CARTESIAN_POINT('Ctrl Pts',(14.6537016966188,-17.1478763944909,
12.));
#189717=CARTESIAN_POINT('Ctrl Pts',(14.6526624064978,-17.1466998098673,
0.));
#189718=CARTESIAN_POINT('Ctrl Pts',(14.6526624064978,-17.1466998098673,
12.));
#189719=CARTESIAN_POINT('Ctrl Pts',(14.65191316345,-17.1458462295273,0.));
#189720=CARTESIAN_POINT('Ctrl Pts',(14.65191316345,-17.1458462295273,12.));
#189721=CARTESIAN_POINT('Ctrl Pts',(14.6515481598057,-17.1454262858045,
0.));
#189722=CARTESIAN_POINT('Ctrl Pts',(14.6515481598057,-17.1454262858045,
12.));
#189723=CARTESIAN_POINT('Ctrl Pts',(14.6514066997188,-17.1452600887039,
0.));
#189724=CARTESIAN_POINT('Ctrl Pts',(14.6514066997188,-17.1452600887039,
12.));
#189725=CARTESIAN_POINT('Ctrl Pts',(14.6513711852839,-17.1452153999142,
0.));
#189726=CARTESIAN_POINT('Ctrl Pts',(14.6513711852839,-17.1452153999142,
12.));
#189727=CARTESIAN_POINT('Ctrl Pts',(14.6513681262571,-17.1452095830633,
0.));
#189728=CARTESIAN_POINT('Ctrl Pts',(14.6513681262571,-17.1452095830633,
12.));
#189729=CARTESIAN_POINT('',(17.9112098770111,-18.8464468996588,0.));
#189730=CARTESIAN_POINT('Ctrl Pts',(17.9112098770111,-18.8464468996588,
0.));
#189731=CARTESIAN_POINT('Ctrl Pts',(17.9057348246595,-18.8448126709692,
0.));
#189732=CARTESIAN_POINT('Ctrl Pts',(17.8947931177807,-18.8415402351786,
0.));
#189733=CARTESIAN_POINT('Ctrl Pts',(17.8784057509355,-18.8366196462581,
0.));
#189734=CARTESIAN_POINT('Ctrl Pts',(17.856606317477,-18.8300349895974,0.));
#189735=CARTESIAN_POINT('Ctrl Pts',(17.8294410311006,-18.8217643886157,
0.));
#189736=CARTESIAN_POINT('Ctrl Pts',(17.8023598011057,-18.8134540340417,
0.));
#189737=CARTESIAN_POINT('Ctrl Pts',(17.7753627137853,-18.8051039860448,
0.));
#189738=CARTESIAN_POINT('Ctrl Pts',(17.7484498996905,-18.7967143519419,
0.));
#189739=CARTESIAN_POINT('Ctrl Pts',(17.7216215409035,-18.788285297605,0.));
#189740=CARTESIAN_POINT('Ctrl Pts',(17.6948778823014,-18.7798170641374,
0.));
#189741=CARTESIAN_POINT('Ctrl Pts',(17.6682192274236,-18.7713099642754,
0.));
#189742=CARTESIAN_POINT('Ctrl Pts',(17.6416459210681,-18.762764361321,0.));
#189743=CARTESIAN_POINT('Ctrl Pts',(17.6151583357012,-18.7541806530984,
0.));
#189744=CARTESIAN_POINT('Ctrl Pts',(17.5887568561371,-18.7455592536688,
0.));
#189745=CARTESIAN_POINT('Ctrl Pts',(17.5624418653245,-18.7369005764553,
0.));
#189746=CARTESIAN_POINT('Ctrl Pts',(17.5362137287593,-18.7282050157138,
0.));
#189747=CARTESIAN_POINT('Ctrl Pts',(17.5100727820876,-18.7194729318098,
0.));
#189748=CARTESIAN_POINT('Ctrl Pts',(17.4840193397162,-18.7107046613912,
0.));
#189749=CARTESIAN_POINT('Ctrl Pts',(17.4580537012753,-18.70190052503,0.));
#189750=CARTESIAN_POINT('Ctrl Pts',(17.4321761588142,-18.6930608357409,
0.));
#189751=CARTESIAN_POINT('Ctrl Pts',(17.4063870038562,-18.6841859073471,
0.));
#189752=CARTESIAN_POINT('Ctrl Pts',(17.3806865340747,-18.6752760624052,
0.));
#189753=CARTESIAN_POINT('Ctrl Pts',(17.3550750612443,-18.6663316416582,
0.));
#189754=CARTESIAN_POINT('Ctrl Pts',(17.3295529098618,-18.6573530024033,
0.));
#189755=CARTESIAN_POINT('Ctrl Pts',(17.3041204135074,-18.6483405141865,
0.));
#189756=CARTESIAN_POINT('Ctrl Pts',(17.2787779120213,-18.6392945554748,
0.));
#189757=CARTESIAN_POINT('Ctrl Pts',(17.2535257482187,-18.6302155097943,
0.));
#189758=CARTESIAN_POINT('Ctrl Pts',(17.2283642650517,-18.6211037624038,
0.));
#189759=CARTESIAN_POINT('Ctrl Pts',(17.2032938019284,-18.6119596959949,
0.));
#189760=CARTESIAN_POINT('Ctrl Pts',(17.1783146940127,-18.6027836898817,
0.));
#189761=CARTESIAN_POINT('Ctrl Pts',(17.1534272741643,-18.5935761222825,
0.));
#189762=CARTESIAN_POINT('Ctrl Pts',(17.1286318741183,-18.5843373717247,
0.));
#189763=CARTESIAN_POINT('Ctrl Pts',(17.1039288260001,-18.5750678188542,
0.));
#189764=CARTESIAN_POINT('Ctrl Pts',(17.0793184636079,-18.5657678479789,
0.));
#189765=CARTESIAN_POINT('Ctrl Pts',(17.0548011239751,-18.556437848963,0.));
#189766=CARTESIAN_POINT('Ctrl Pts',(17.0303771481738,-18.547078218209,0.));
#189767=CARTESIAN_POINT('Ctrl Pts',(17.0060468805097,-18.5376893576961,
0.));
#189768=CARTESIAN_POINT('Ctrl Pts',(16.981810668038,-18.5282716744197,0.));
#189769=CARTESIAN_POINT('Ctrl Pts',(16.9576688599339,-18.5188255796659,
0.));
#189770=CARTESIAN_POINT('Ctrl Pts',(16.9336218069353,-18.5093514883835,
0.));
#189771=CARTESIAN_POINT('Ctrl Pts',(16.9096698606943,-18.499849818462,0.));
#189772=CARTESIAN_POINT('Ctrl Pts',(16.8858133733088,-18.4903209902227,
0.));
#189773=CARTESIAN_POINT('Ctrl Pts',(16.8620526977171,-18.4807654268771,
0.));
#189774=CARTESIAN_POINT('Ctrl Pts',(16.8383881879709,-18.4711835548623,
0.));
#189775=CARTESIAN_POINT('Ctrl Pts',(16.8148201995472,-18.4615758042305,
0.));
#189776=CARTESIAN_POINT('Ctrl Pts',(16.791349089629,-18.4519426090124,0.));
#189777=CARTESIAN_POINT('Ctrl Pts',(16.7679752173992,-18.44228440761,0.));
#189778=CARTESIAN_POINT('Ctrl Pts',(16.7446989442882,-18.4326016431392,
0.));
#189779=CARTESIAN_POINT('Ctrl Pts',(16.7215206338818,-18.4228947633187,
0.));
#189780=CARTESIAN_POINT('Ctrl Pts',(16.698440651849,-18.413164220399,0.));
#189781=CARTESIAN_POINT('Ctrl Pts',(16.6754593658513,-18.403410471079,0.));
#189782=CARTESIAN_POINT('Ctrl Pts',(16.6525771454513,-18.3936339764332,
0.));
#189783=CARTESIAN_POINT('Ctrl Pts',(16.6297943620056,-18.3838352018327,
0.));
#189784=CARTESIAN_POINT('Ctrl Pts',(16.607111388571,-18.3740146168879,0.));
#189785=CARTESIAN_POINT('Ctrl Pts',(16.5845286000217,-18.3641726955889,
0.));
#189786=CARTESIAN_POINT('Ctrl Pts',(16.5620463731413,-18.354309916433,0.));
#189787=CARTESIAN_POINT('Ctrl Pts',(16.5396650867139,-18.34442676256,0.));
#189788=CARTESIAN_POINT('Ctrl Pts',(16.5173851216045,-18.3345237218864,
0.));
#189789=CARTESIAN_POINT('Ctrl Pts',(16.4952068608345,-18.3246012872469,
0.));
#189790=CARTESIAN_POINT('Ctrl Pts',(16.4731306896441,-18.3146599565231,
0.));
#189791=CARTESIAN_POINT('Ctrl Pts',(16.4511569955233,-18.304700232686,0.));
#189792=CARTESIAN_POINT('Ctrl Pts',(16.4292861682378,-18.294722623851,0.));
#189793=CARTESIAN_POINT('Ctrl Pts',(16.4075185998454,-18.2847276433309,
0.));
#189794=CARTESIAN_POINT('Ctrl Pts',(16.385854684708,-18.2747158096934,0.));
#189795=CARTESIAN_POINT('Ctrl Pts',(16.3642948194868,-18.2646876468169,
0.));
#189796=CARTESIAN_POINT('Ctrl Pts',(16.3428394031589,-18.2546436839608,
0.));
#189797=CARTESIAN_POINT('Ctrl Pts',(16.3214888370987,-18.2445844558742,
0.));
#189798=CARTESIAN_POINT('Ctrl Pts',(16.3002435251378,-18.2345105028982,
0.));
#189799=CARTESIAN_POINT('Ctrl Pts',(16.2791038736223,-18.2244223710746,
0.));
#189800=CARTESIAN_POINT('Ctrl Pts',(16.2580702914615,-18.2143206122529,
0.));
#189801=CARTESIAN_POINT('Ctrl Pts',(16.2371431901638,-18.2042057842035,
0.));
#189802=CARTESIAN_POINT('Ctrl Pts',(16.2163229838875,-18.1940784507229,
0.));
#189803=CARTESIAN_POINT('Ctrl Pts',(16.1956100895073,-18.1839391817331,
0.));
#189804=CARTESIAN_POINT('Ctrl Pts',(16.1750049266671,-18.1737885533849,
0.));
#189805=CARTESIAN_POINT('Ctrl Pts',(16.154507917826,-18.1636271481615,0.));
#189806=CARTESIAN_POINT('Ctrl Pts',(16.1341194882988,-18.1534555549853,
0.));
#189807=CARTESIAN_POINT('Ctrl Pts',(16.1138400662794,-18.1432743693235,
0.));
#189808=CARTESIAN_POINT('Ctrl Pts',(16.0936700829112,-18.1330841933105,
0.));
#189809=CARTESIAN_POINT('Ctrl Pts',(16.0736099723668,-18.1228856358751,
0.));
#189810=CARTESIAN_POINT('Ctrl Pts',(16.0536601719125,-18.112679312869,0.));
#189811=CARTESIAN_POINT('Ctrl Pts',(16.0338211219693,-18.1024658471966,
0.));
#189812=CARTESIAN_POINT('Ctrl Pts',(16.014093266161,-18.0922458689462,0.));
#189813=CARTESIAN_POINT('Ctrl Pts',(15.9944770513613,-18.0820200155236,
0.));
#189814=CARTESIAN_POINT('Ctrl Pts',(15.9749729277846,-18.0717889317958,
0.));
#189815=CARTESIAN_POINT('Ctrl Pts',(15.9555813490644,-18.061553270236,0.));
#189816=CARTESIAN_POINT('Ctrl Pts',(15.9363027723244,-18.0513136910691,
0.));
#189817=CARTESIAN_POINT('Ctrl Pts',(15.9171376582436,-18.0410708624209,
0.));
#189818=CARTESIAN_POINT('Ctrl Pts',(15.8980864711042,-18.0308254604636,
0.));
#189819=CARTESIAN_POINT('Ctrl Pts',(15.8791496788682,-18.0205781695769,
0.));
#189820=CARTESIAN_POINT('Ctrl Pts',(15.8603277532831,-18.0103296825205,
0.));
#189821=CARTESIAN_POINT('Ctrl Pts',(15.8416211699679,-18.0000807006052,
0.));
#189822=CARTESIAN_POINT('Ctrl Pts',(15.8230304084962,-17.9898319338665,
0.));
#189823=CARTESIAN_POINT('Ctrl Pts',(15.8045559524676,-17.9795841012386,
0.));
#189824=CARTESIAN_POINT('Ctrl Pts',(15.7861982895724,-17.9693379307303,
0.));
#189825=CARTESIAN_POINT('Ctrl Pts',(15.7679579117077,-17.9590941596242,
0.));
#189826=CARTESIAN_POINT('Ctrl Pts',(15.749835315086,-17.9488535346781,0.));
#189827=CARTESIAN_POINT('Ctrl Pts',(15.7318310003335,-17.9386168123262,
0.));
#189828=CARTESIAN_POINT('Ctrl Pts',(15.7139454725838,-17.9283847588836,
0.));
#189829=CARTESIAN_POINT('Ctrl Pts',(15.6961792415522,-17.9181581507455,
0.));
#189830=CARTESIAN_POINT('Ctrl Pts',(15.678532821646,-17.9079377746111,0.));
#189831=CARTESIAN_POINT('Ctrl Pts',(15.661006732103,-17.897724427724,0.));
#189832=CARTESIAN_POINT('Ctrl Pts',(15.6436014971084,-17.8875189181091,
0.));
#189833=CARTESIAN_POINT('Ctrl Pts',(15.6263176459108,-17.8773220648125,
0.));
#189834=CARTESIAN_POINT('Ctrl Pts',(15.609155712921,-17.8671346981394,0.));
#189835=CARTESIAN_POINT('Ctrl Pts',(15.5921162378192,-17.8569576599006,
0.));
#189836=CARTESIAN_POINT('Ctrl Pts',(15.5751997657162,-17.8467918036987,
0.));
#189837=CARTESIAN_POINT('Ctrl Pts',(15.5584068472982,-17.8366379952085,
0.));
#189838=CARTESIAN_POINT('Ctrl Pts',(15.541738038964,-17.8264971124607,0.));
#189839=CARTESIAN_POINT('Ctrl Pts',(15.5251939029552,-17.8163700461256,
0.));
#189840=CARTESIAN_POINT('Ctrl Pts',(15.5087750074718,-17.8062576997952,
0.));
#189841=CARTESIAN_POINT('Ctrl Pts',(15.4924819268517,-17.7961609903148,
0.));
#189842=CARTESIAN_POINT('Ctrl Pts',(15.4763152417497,-17.786080848122,0.));
#189843=CARTESIAN_POINT('Ctrl Pts',(15.4602755393017,-17.7760182175815,
0.));
#189844=CARTESIAN_POINT('Ctrl Pts',(15.4443634132869,-17.7659740573265,
0.));
#189845=CARTESIAN_POINT('Ctrl Pts',(15.4285794642667,-17.7559493405881,
0.));
#189846=CARTESIAN_POINT('Ctrl Pts',(15.4129242997837,-17.7459450555813,
0.));
#189847=CARTESIAN_POINT('Ctrl Pts',(15.3973985345802,-17.735962205915,0.));
#189848=CARTESIAN_POINT('Ctrl Pts',(15.3820027907966,-17.7260018109924,
0.));
#189849=CARTESIAN_POINT('Ctrl Pts',(15.3667376981699,-17.7160649064206,
0.));
#189850=CARTESIAN_POINT('Ctrl Pts',(15.351603894206,-17.7061525444042,0.));
#189851=CARTESIAN_POINT('Ctrl Pts',(15.3366020244066,-17.6962657941983,
0.));
#189852=CARTESIAN_POINT('Ctrl Pts',(15.3217327425338,-17.6864057426052,
0.));
#189853=CARTESIAN_POINT('Ctrl Pts',(15.30699671085,-17.676573494456,0.));
#189854=CARTESIAN_POINT('Ctrl Pts',(15.2923946003598,-17.6667701731041,
0.));
#189855=CARTESIAN_POINT('Ctrl Pts',(15.2779270910239,-17.6569969209,0.));
#189856=CARTESIAN_POINT('Ctrl Pts',(15.2635948720292,-17.6472548997328,
0.));
#189857=CARTESIAN_POINT('Ctrl Pts',(15.2493986421092,-17.6375452916369,
0.));
#189858=CARTESIAN_POINT('Ctrl Pts',(15.2353391098366,-17.6278692993764,
0.));
#189859=CARTESIAN_POINT('Ctrl Pts',(15.2214169939199,-17.6182281470468,
0.));
#189860=CARTESIAN_POINT('Ctrl Pts',(15.2076330234686,-17.60862308065,0.));
#189861=CARTESIAN_POINT('Ctrl Pts',(15.1939879383268,-17.5990553687599,
0.));
#189862=CARTESIAN_POINT('Ctrl Pts',(15.1804824894605,-17.5895263032595,
0.));
#189863=CARTESIAN_POINT('Ctrl Pts',(15.1671174393137,-17.580037200054,0.));
#189864=CARTESIAN_POINT('Ctrl Pts',(15.1538935621714,-17.5705893998029,
0.));
#189865=CARTESIAN_POINT('Ctrl Pts',(15.1408116444876,-17.5611842686192,
0.));
#189866=CARTESIAN_POINT('Ctrl Pts',(15.1278724853138,-17.5518231989117,
0.));
#189867=CARTESIAN_POINT('Ctrl Pts',(15.1150768967728,-17.5425076102963,
0.));
#189868=CARTESIAN_POINT('Ctrl Pts',(15.1024257045033,-17.5332389504829,
0.));
#189869=CARTESIAN_POINT('Ctrl Pts',(15.0899197481082,-17.5240186961791,
0.));
#189870=CARTESIAN_POINT('Ctrl Pts',(15.0775598815749,-17.5148483539687,
0.));
#189871=CARTESIAN_POINT('Ctrl Pts',(15.0653469738307,-17.5057294613877,
0.));
#189872=CARTESIAN_POINT('Ctrl Pts',(15.0532819093085,-17.4966635880246,
0.));
#189873=CARTESIAN_POINT('Ctrl Pts',(15.0413655884993,-17.4876523366178,
0.));
#189874=CARTESIAN_POINT('Ctrl Pts',(15.029598928488,-17.4786973441417,0.));
#189875=CARTESIAN_POINT('Ctrl Pts',(15.0179828635087,-17.4698002829357,
0.));
#189876=CARTESIAN_POINT('Ctrl Pts',(15.0065183456922,-17.4609628621419,
0.));
#189877=CARTESIAN_POINT('Ctrl Pts',(14.9952063457779,-17.4521868291005,
0.));
#189878=CARTESIAN_POINT('Ctrl Pts',(14.9840478538357,-17.4434739707773,
0.));
#189879=CARTESIAN_POINT('Ctrl Pts',(14.973043879945,-17.4348261151395,0.));
#189880=CARTESIAN_POINT('Ctrl Pts',(14.9621954549825,-17.4262451327088,
0.));
#189881=CARTESIAN_POINT('Ctrl Pts',(14.9515036315142,-17.4177329382827,
0.));
#189882=CARTESIAN_POINT('Ctrl Pts',(14.940969484645,-17.4092914926072,0.));
#189883=CARTESIAN_POINT('Ctrl Pts',(14.9305941128758,-17.400922804075,0.));
#189884=CARTESIAN_POINT('Ctrl Pts',(14.9203786389343,-17.3926289303987,
0.));
#189885=CARTESIAN_POINT('Ctrl Pts',(14.9103242110057,-17.3844119809823,
0.));
#189886=CARTESIAN_POINT('Ctrl Pts',(14.9004320039609,-17.3762741193075,
0.));
#189887=CARTESIAN_POINT('Ctrl Pts',(14.8907032205789,-17.3682175653236,
0.));
#189888=CARTESIAN_POINT('Ctrl Pts',(14.8811390927424,-17.3602445978163,
0.));
#189889=CARTESIAN_POINT('Ctrl Pts',(14.8717408826957,-17.3523575568648,
0.));
#189890=CARTESIAN_POINT('Ctrl Pts',(14.8625098843419,-17.3445588463477,
0.));
#189891=CARTESIAN_POINT('Ctrl Pts',(14.8534474245433,-17.336850936485,0.));
#189892=CARTESIAN_POINT('Ctrl Pts',(14.8445548643504,-17.3292363662601,
0.));
#189893=CARTESIAN_POINT('Ctrl Pts',(14.8358336004193,-17.3217177462096,
0.));
#189894=CARTESIAN_POINT('Ctrl Pts',(14.8272850675375,-17.3142977632656,
0.));
#189895=CARTESIAN_POINT('Ctrl Pts',(14.8189107410161,-17.3069791853705,
0.));
#189896=CARTESIAN_POINT('Ctrl Pts',(14.8107121391038,-17.2997648661483,
0.));
#189897=CARTESIAN_POINT('Ctrl Pts',(14.8026908254281,-17.2926577496519,
0.));
#189898=CARTESIAN_POINT('Ctrl Pts',(14.7948484105252,-17.28566087332,0.));
#189899=CARTESIAN_POINT('Ctrl Pts',(14.787186553128,-17.278777370485,0.));
#189900=CARTESIAN_POINT('Ctrl Pts',(14.7797069617802,-17.2720104735192,
0.));
#189901=CARTESIAN_POINT('Ctrl Pts',(14.7724113956728,-17.2653635155317,
0.));
#189902=CARTESIAN_POINT('Ctrl Pts',(14.7653016697589,-17.2588399401464,
0.));
#189903=CARTESIAN_POINT('Ctrl Pts',(14.7583796616617,-17.2524433146837,
0.));
#189904=CARTESIAN_POINT('Ctrl Pts',(14.7516473175124,-17.2461773413289,
0.));
#189905=CARTESIAN_POINT('Ctrl Pts',(14.7451066593793,-17.2400458713566,
0.));
#189906=CARTESIAN_POINT('Ctrl Pts',(14.7387597858117,-17.2340529062078,
0.));
#189907=CARTESIAN_POINT('Ctrl Pts',(14.7326088681163,-17.2282025904314,
0.));
#189908=CARTESIAN_POINT('Ctrl Pts',(14.7266561494282,-17.2224992099666,
0.));
#189909=CARTESIAN_POINT('Ctrl Pts',(14.7209039390325,-17.2169471814255,
0.));
#189910=CARTESIAN_POINT('Ctrl Pts',(14.7153546289338,-17.2115510835988,
0.));
#189911=CARTESIAN_POINT('Ctrl Pts',(14.7100107213586,-17.2063157097316,
0.));
#189912=CARTESIAN_POINT('Ctrl Pts',(14.7048748502662,-17.2012461084268,
0.));
#189913=CARTESIAN_POINT('Ctrl Pts',(14.699949811582,-17.1963476411694,0.));
#189914=CARTESIAN_POINT('Ctrl Pts',(14.6952385361706,-17.1916259308416,
0.));
#189915=CARTESIAN_POINT('Ctrl Pts',(14.6907440526957,-17.1870867909918,
0.));
#189916=CARTESIAN_POINT('Ctrl Pts',(14.6864694522319,-17.182736158472,0.));
#189917=CARTESIAN_POINT('Ctrl Pts',(14.6824178576166,-17.1785800350827,
0.));
#189918=CARTESIAN_POINT('Ctrl Pts',(14.6785925615676,-17.1746247499057,
0.));
#189919=CARTESIAN_POINT('Ctrl Pts',(14.6749971333867,-17.1708771619129,
0.));
#189920=CARTESIAN_POINT('Ctrl Pts',(14.6716355833321,-17.1673449723019,
0.));
#189921=CARTESIAN_POINT('Ctrl Pts',(14.6685123374424,-17.1640366762304,
0.));
#189922=CARTESIAN_POINT('Ctrl Pts',(14.6656319165057,-17.1609609517369,
0.));
#189923=CARTESIAN_POINT('Ctrl Pts',(14.662998728599,-17.1581262646789,0.));
#189924=CARTESIAN_POINT('Ctrl Pts',(14.660616716964,-17.1555401986403,0.));
#189925=CARTESIAN_POINT('Ctrl Pts',(14.65849005553,-17.1532107762719,0.));
#189926=CARTESIAN_POINT('Ctrl Pts',(14.6566237952435,-17.1511476869495,
0.));
#189927=CARTESIAN_POINT('Ctrl Pts',(14.6550248622813,-17.1493641837556,
0.));
#189928=CARTESIAN_POINT('Ctrl Pts',(14.6537016966188,-17.1478763944909,
0.));
#189929=CARTESIAN_POINT('Ctrl Pts',(14.6526624064978,-17.1466998098673,
0.));
#189930=CARTESIAN_POINT('Ctrl Pts',(14.65191316345,-17.1458462295273,0.));
#189931=CARTESIAN_POINT('Ctrl Pts',(14.6515481598057,-17.1454262858045,
0.));
#189932=CARTESIAN_POINT('Ctrl Pts',(14.6514066997188,-17.1452600887039,
0.));
#189933=CARTESIAN_POINT('Ctrl Pts',(14.6513711852839,-17.1452153999142,
0.));
#189934=CARTESIAN_POINT('Ctrl Pts',(14.6513681262571,-17.1452095830633,
0.));
#189935=CARTESIAN_POINT('',(17.9112098770111,-18.8464468996588,0.));
#189936=CARTESIAN_POINT('Ctrl Pts',(12.7689476255362,-18.5896416359912,
0.));
#189937=CARTESIAN_POINT('Ctrl Pts',(12.7689476255362,-18.5896416359912,
12.));
#189938=CARTESIAN_POINT('Ctrl Pts',(12.7689524524483,-18.5896460962964,
0.));
#189939=CARTESIAN_POINT('Ctrl Pts',(12.7689524524483,-18.5896460962964,
12.));
#189940=CARTESIAN_POINT('Ctrl Pts',(12.768986426692,-18.5896919669165,0.));
#189941=CARTESIAN_POINT('Ctrl Pts',(12.768986426692,-18.5896919669165,12.));
#189942=CARTESIAN_POINT('Ctrl Pts',(12.769110348199,-18.589871621843,0.));
#189943=CARTESIAN_POINT('Ctrl Pts',(12.769110348199,-18.589871621843,12.));
#189944=CARTESIAN_POINT('Ctrl Pts',(12.7694215127918,-18.5903328777227,
0.));
#189945=CARTESIAN_POINT('Ctrl Pts',(12.7694215127918,-18.5903328777227,
12.));
#189946=CARTESIAN_POINT('Ctrl Pts',(12.7700520897173,-18.5912775137806,
0.));
#189947=CARTESIAN_POINT('Ctrl Pts',(12.7700520897173,-18.5912775137806,
12.));
#189948=CARTESIAN_POINT('Ctrl Pts',(12.7709195951156,-18.5925859134579,
0.));
#189949=CARTESIAN_POINT('Ctrl Pts',(12.7709195951156,-18.5925859134579,
12.));
#189950=CARTESIAN_POINT('Ctrl Pts',(12.7720142287172,-18.5942490615407,
0.));
#189951=CARTESIAN_POINT('Ctrl Pts',(12.7720142287172,-18.5942490615407,
12.));
#189952=CARTESIAN_POINT('Ctrl Pts',(12.7733231262108,-18.5962551167772,
0.));
#189953=CARTESIAN_POINT('Ctrl Pts',(12.7733231262108,-18.5962551167772,
12.));
#189954=CARTESIAN_POINT('Ctrl Pts',(12.7748328937638,-18.598591752595,0.));
#189955=CARTESIAN_POINT('Ctrl Pts',(12.7748328937638,-18.598591752595,12.));
#189956=CARTESIAN_POINT('Ctrl Pts',(12.7765325225081,-18.6012488486709,
0.));
#189957=CARTESIAN_POINT('Ctrl Pts',(12.7765325225081,-18.6012488486709,
12.));
#189958=CARTESIAN_POINT('Ctrl Pts',(12.7784139605066,-18.6042190183704,
0.));
#189959=CARTESIAN_POINT('Ctrl Pts',(12.7784139605066,-18.6042190183704,
12.));
#189960=CARTESIAN_POINT('Ctrl Pts',(12.7804705387658,-18.6074961535723,
0.));
#189961=CARTESIAN_POINT('Ctrl Pts',(12.7804705387658,-18.6074961535723,
12.));
#189962=CARTESIAN_POINT('Ctrl Pts',(12.7826959526924,-18.611074482622,0.));
#189963=CARTESIAN_POINT('Ctrl Pts',(12.7826959526924,-18.611074482622,12.));
#189964=CARTESIAN_POINT('Ctrl Pts',(12.7850831657901,-18.6149475565188,
0.));
#189965=CARTESIAN_POINT('Ctrl Pts',(12.7850831657901,-18.6149475565188,
12.));
#189966=CARTESIAN_POINT('Ctrl Pts',(12.7876249657834,-18.6191087624752,
0.));
#189967=CARTESIAN_POINT('Ctrl Pts',(12.7876249657834,-18.6191087624752,
12.));
#189968=CARTESIAN_POINT('Ctrl Pts',(12.7903142925234,-18.6235516265575,
0.));
#189969=CARTESIAN_POINT('Ctrl Pts',(12.7903142925234,-18.6235516265575,
12.));
#189970=CARTESIAN_POINT('Ctrl Pts',(12.7931447451555,-18.6282702819371,
0.));
#189971=CARTESIAN_POINT('Ctrl Pts',(12.7931447451555,-18.6282702819371,
12.));
#189972=CARTESIAN_POINT('Ctrl Pts',(12.796110622225,-18.6332595057006,0.));
#189973=CARTESIAN_POINT('Ctrl Pts',(12.796110622225,-18.6332595057006,12.));
#189974=CARTESIAN_POINT('Ctrl Pts',(12.7992066625264,-18.63851447924,0.));
#189975=CARTESIAN_POINT('Ctrl Pts',(12.7992066625264,-18.63851447924,12.));
#189976=CARTESIAN_POINT('Ctrl Pts',(12.8024278770152,-18.6440306327456,
0.));
#189977=CARTESIAN_POINT('Ctrl Pts',(12.8024278770152,-18.6440306327456,
12.));
#189978=CARTESIAN_POINT('Ctrl Pts',(12.805769331162,-18.6498034438987,0.));
#189979=CARTESIAN_POINT('Ctrl Pts',(12.805769331162,-18.6498034438987,12.));
#189980=CARTESIAN_POINT('Ctrl Pts',(12.8092261933858,-18.6558284825773,
0.));
#189981=CARTESIAN_POINT('Ctrl Pts',(12.8092261933858,-18.6558284825773,
12.));
#189982=CARTESIAN_POINT('Ctrl Pts',(12.8127937909631,-18.6621014624746,
0.));
#189983=CARTESIAN_POINT('Ctrl Pts',(12.8127937909631,-18.6621014624746,
12.));
#189984=CARTESIAN_POINT('Ctrl Pts',(12.8164676687362,-18.66861829528,0.));
#189985=CARTESIAN_POINT('Ctrl Pts',(12.8164676687362,-18.66861829528,12.));
#189986=CARTESIAN_POINT('Ctrl Pts',(12.8202436318474,-18.6753751301092,
0.));
#189987=CARTESIAN_POINT('Ctrl Pts',(12.8202436318474,-18.6753751301092,
12.));
#189988=CARTESIAN_POINT('Ctrl Pts',(12.8241176980017,-18.6823683094139,
0.));
#189989=CARTESIAN_POINT('Ctrl Pts',(12.8241176980017,-18.6823683094139,
12.));
#189990=CARTESIAN_POINT('Ctrl Pts',(12.8280860635231,-18.6895943376172,
0.));
#189991=CARTESIAN_POINT('Ctrl Pts',(12.8280860635231,-18.6895943376172,
12.));
#189992=CARTESIAN_POINT('Ctrl Pts',(12.8321450599789,-18.6970498410172,
0.));
#189993=CARTESIAN_POINT('Ctrl Pts',(12.8321450599789,-18.6970498410172,
12.));
#189994=CARTESIAN_POINT('Ctrl Pts',(12.8362911280361,-18.7047315436294,
0.));
#189995=CARTESIAN_POINT('Ctrl Pts',(12.8362911280361,-18.7047315436294,
12.));
#189996=CARTESIAN_POINT('Ctrl Pts',(12.8405208263431,-18.7126362754445,
0.));
#189997=CARTESIAN_POINT('Ctrl Pts',(12.8405208263431,-18.7126362754445,
12.));
#189998=CARTESIAN_POINT('Ctrl Pts',(12.8448308329494,-18.7207609737702,
0.));
#189999=CARTESIAN_POINT('Ctrl Pts',(12.8448308329494,-18.7207609737702,
12.));
#190000=CARTESIAN_POINT('Ctrl Pts',(12.8492179511591,-18.7291026886554,
0.));
#190001=CARTESIAN_POINT('Ctrl Pts',(12.8492179511591,-18.7291026886554,
12.));
#190002=CARTESIAN_POINT('Ctrl Pts',(12.8536791086316,-18.7376585820854,
0.));
#190003=CARTESIAN_POINT('Ctrl Pts',(12.8536791086316,-18.7376585820854,
12.));
#190004=CARTESIAN_POINT('Ctrl Pts',(12.8582113455646,-18.7464259171251,
0.));
#190005=CARTESIAN_POINT('Ctrl Pts',(12.8582113455646,-18.7464259171251,
12.));
#190006=CARTESIAN_POINT('Ctrl Pts',(12.8628118054171,-18.7554020493887,
0.));
#190007=CARTESIAN_POINT('Ctrl Pts',(12.8628118054171,-18.7554020493887,
12.));
#190008=CARTESIAN_POINT('Ctrl Pts',(12.8674777239653,-18.7645844169564,
0.));
#190009=CARTESIAN_POINT('Ctrl Pts',(12.8674777239653,-18.7645844169564,
12.));
#190010=CARTESIAN_POINT('Ctrl Pts',(12.872206421181,-18.7739705329022,0.));
#190011=CARTESIAN_POINT('Ctrl Pts',(12.872206421181,-18.7739705329022,12.));
#190012=CARTESIAN_POINT('Ctrl Pts',(12.8769952998095,-18.7835579840477,
0.));
#190013=CARTESIAN_POINT('Ctrl Pts',(12.8769952998095,-18.7835579840477,
12.));
#190014=CARTESIAN_POINT('Ctrl Pts',(12.8818418427475,-18.7933444285868,
0.));
#190015=CARTESIAN_POINT('Ctrl Pts',(12.8818418427475,-18.7933444285868,
12.));
#190016=CARTESIAN_POINT('Ctrl Pts',(12.8867436109546,-18.8033275941943,
0.));
#190017=CARTESIAN_POINT('Ctrl Pts',(12.8867436109546,-18.8033275941943,
12.));
#190018=CARTESIAN_POINT('Ctrl Pts',(12.8916982409935,-18.813505275782,0.));
#190019=CARTESIAN_POINT('Ctrl Pts',(12.8916982409935,-18.813505275782,12.));
#190020=CARTESIAN_POINT('Ctrl Pts',(12.8967034410754,-18.8238753319129,
0.));
#190021=CARTESIAN_POINT('Ctrl Pts',(12.8967034410754,-18.8238753319129,
12.));
#190022=CARTESIAN_POINT('Ctrl Pts',(12.9017569871738,-18.8344356812591,
0.));
#190023=CARTESIAN_POINT('Ctrl Pts',(12.9017569871738,-18.8344356812591,
12.));
#190024=CARTESIAN_POINT('Ctrl Pts',(12.9068567191854,-18.8451842990984,
0.));
#190025=CARTESIAN_POINT('Ctrl Pts',(12.9068567191854,-18.8451842990984,
12.));
#190026=CARTESIAN_POINT('Ctrl Pts',(12.9120005369063,-18.8561192136198,
0.));
#190027=CARTESIAN_POINT('Ctrl Pts',(12.9120005369063,-18.8561192136198,
12.));
#190028=CARTESIAN_POINT('Ctrl Pts',(12.9171863977045,-18.8672385038326,
0.));
#190029=CARTESIAN_POINT('Ctrl Pts',(12.9171863977045,-18.8672385038326,
12.));
#190030=CARTESIAN_POINT('Ctrl Pts',(12.9224123144981,-18.8785402977528,
0.));
#190031=CARTESIAN_POINT('Ctrl Pts',(12.9224123144981,-18.8785402977528,
12.));
#190032=CARTESIAN_POINT('Ctrl Pts',(12.9276763536373,-18.8900227704889,
0.));
#190033=CARTESIAN_POINT('Ctrl Pts',(12.9276763536373,-18.8900227704889,
12.));
#190034=CARTESIAN_POINT('Ctrl Pts',(12.9329766328184,-18.9016841423403,
0.));
#190035=CARTESIAN_POINT('Ctrl Pts',(12.9329766328184,-18.9016841423403,
12.));
#190036=CARTESIAN_POINT('Ctrl Pts',(12.9383113190374,-18.9135226769466,
0.));
#190037=CARTESIAN_POINT('Ctrl Pts',(12.9383113190374,-18.9135226769466,
12.));
#190038=CARTESIAN_POINT('Ctrl Pts',(12.9436786266105,-18.9255366795195,
0.));
#190039=CARTESIAN_POINT('Ctrl Pts',(12.9436786266105,-18.9255366795195,
12.));
#190040=CARTESIAN_POINT('Ctrl Pts',(12.9490768151821,-18.9377244950435,
0.));
#190041=CARTESIAN_POINT('Ctrl Pts',(12.9490768151821,-18.9377244950435,
12.));
#190042=CARTESIAN_POINT('Ctrl Pts',(12.9545041877377,-18.9500845064715,
0.));
#190043=CARTESIAN_POINT('Ctrl Pts',(12.9545041877377,-18.9500845064715,
12.));
#190044=CARTESIAN_POINT('Ctrl Pts',(12.9599590886319,-18.9626151329229,
0.));
#190045=CARTESIAN_POINT('Ctrl Pts',(12.9599590886319,-18.9626151329229,
12.));
#190046=CARTESIAN_POINT('Ctrl Pts',(12.9654399021869,-18.9753148284475,
0.));
#190047=CARTESIAN_POINT('Ctrl Pts',(12.9654399021869,-18.9753148284475,
12.));
#190048=CARTESIAN_POINT('Ctrl Pts',(12.9709450512747,-18.9881820807586,
0.));
#190049=CARTESIAN_POINT('Ctrl Pts',(12.9709450512747,-18.9881820807586,
12.));
#190050=CARTESIAN_POINT('Ctrl Pts',(12.9764729959205,-19.0012154099791,
0.));
#190051=CARTESIAN_POINT('Ctrl Pts',(12.9764729959205,-19.0012154099791,
12.));
#190052=CARTESIAN_POINT('Ctrl Pts',(12.9820222318715,-19.0144133673348,
0.));
#190053=CARTESIAN_POINT('Ctrl Pts',(12.9820222318715,-19.0144133673348,
12.));
#190054=CARTESIAN_POINT('Ctrl Pts',(12.9875912893003,-19.0277745339908,
0.));
#190055=CARTESIAN_POINT('Ctrl Pts',(12.9875912893003,-19.0277745339908,
12.));
#190056=CARTESIAN_POINT('Ctrl Pts',(12.9931787316514,-19.0412975200398,
0.));
#190057=CARTESIAN_POINT('Ctrl Pts',(12.9931787316514,-19.0412975200398,
12.));
#190058=CARTESIAN_POINT('Ctrl Pts',(12.9987831544502,-19.0549809634355,
0.));
#190059=CARTESIAN_POINT('Ctrl Pts',(12.9987831544502,-19.0549809634355,
12.));
#190060=CARTESIAN_POINT('Ctrl Pts',(13.0044031841381,-19.0688235289437,
0.));
#190061=CARTESIAN_POINT('Ctrl Pts',(13.0044031841381,-19.0688235289437,
12.));
#190062=CARTESIAN_POINT('Ctrl Pts',(13.0100374768785,-19.0828239070482,
0.));
#190063=CARTESIAN_POINT('Ctrl Pts',(13.0100374768785,-19.0828239070482,
12.));
#190064=CARTESIAN_POINT('Ctrl Pts',(13.0156847176093,-19.0969808131226,
0.));
#190065=CARTESIAN_POINT('Ctrl Pts',(13.0156847176093,-19.0969808131226,
12.));
#190066=CARTESIAN_POINT('Ctrl Pts',(13.0213436191326,-19.1112929866308,
0.));
#190067=CARTESIAN_POINT('Ctrl Pts',(13.0213436191326,-19.1112929866308,
12.));
#190068=CARTESIAN_POINT('Ctrl Pts',(13.0270129211976,-19.1257591903099,
0.));
#190069=CARTESIAN_POINT('Ctrl Pts',(13.0270129211976,-19.1257591903099,
12.));
#190070=CARTESIAN_POINT('Ctrl Pts',(13.0326913895841,-19.1403782093389,
0.));
#190071=CARTESIAN_POINT('Ctrl Pts',(13.0326913895841,-19.1403782093389,
12.));
#190072=CARTESIAN_POINT('Ctrl Pts',(13.0383778152072,-19.1551488505233,
0.));
#190073=CARTESIAN_POINT('Ctrl Pts',(13.0383778152072,-19.1551488505233,
12.));
#190074=CARTESIAN_POINT('Ctrl Pts',(13.0440710133775,-19.1700699416625,
0.));
#190075=CARTESIAN_POINT('Ctrl Pts',(13.0440710133775,-19.1700699416625,
12.));
#190076=CARTESIAN_POINT('Ctrl Pts',(13.0497698230442,-19.1851403308826,
0.));
#190077=CARTESIAN_POINT('Ctrl Pts',(13.0497698230442,-19.1851403308826,
12.));
#190078=CARTESIAN_POINT('Ctrl Pts',(13.0554731060537,-19.2003588859771,
0.));
#190079=CARTESIAN_POINT('Ctrl Pts',(13.0554731060537,-19.2003588859771,
12.));
#190080=CARTESIAN_POINT('Ctrl Pts',(13.0611797463912,-19.2157244937141,
0.));
#190081=CARTESIAN_POINT('Ctrl Pts',(13.0611797463912,-19.2157244937141,
12.));
#190082=CARTESIAN_POINT('Ctrl Pts',(13.0668886494791,-19.2312360592031,
0.));
#190083=CARTESIAN_POINT('Ctrl Pts',(13.0668886494791,-19.2312360592031,
12.));
#190084=CARTESIAN_POINT('Ctrl Pts',(13.0725987415856,-19.2468925053988,
0.));
#190085=CARTESIAN_POINT('Ctrl Pts',(13.0725987415856,-19.2468925053988,
12.));
#190086=CARTESIAN_POINT('Ctrl Pts',(13.0783089692117,-19.2626927725596,
0.));
#190087=CARTESIAN_POINT('Ctrl Pts',(13.0783089692117,-19.2626927725596,
12.));
#190088=CARTESIAN_POINT('Ctrl Pts',(13.0840182984949,-19.2786358177198,
0.));
#190089=CARTESIAN_POINT('Ctrl Pts',(13.0840182984949,-19.2786358177198,
12.));
#190090=CARTESIAN_POINT('Ctrl Pts',(13.0897257145969,-19.2947206141246,
0.));
#190091=CARTESIAN_POINT('Ctrl Pts',(13.0897257145969,-19.2947206141246,
12.));
#190092=CARTESIAN_POINT('Ctrl Pts',(13.095430221148,-19.3109461507358,0.));
#190093=CARTESIAN_POINT('Ctrl Pts',(13.095430221148,-19.3109461507358,12.));
#190094=CARTESIAN_POINT('Ctrl Pts',(13.1011308397591,-19.3273114318268,
0.));
#190095=CARTESIAN_POINT('Ctrl Pts',(13.1011308397591,-19.3273114318268,
12.));
#190096=CARTESIAN_POINT('Ctrl Pts',(13.1068266095186,-19.3438154765395,
0.));
#190097=CARTESIAN_POINT('Ctrl Pts',(13.1068266095186,-19.3438154765395,
12.));
#190098=CARTESIAN_POINT('Ctrl Pts',(13.1125165865021,-19.3604573184516,
0.));
#190099=CARTESIAN_POINT('Ctrl Pts',(13.1125165865021,-19.3604573184516,
12.));
#190100=CARTESIAN_POINT('Ctrl Pts',(13.118199843271,-19.3772360051093,0.));
#190101=CARTESIAN_POINT('Ctrl Pts',(13.118199843271,-19.3772360051093,12.));
#190102=CARTESIAN_POINT('Ctrl Pts',(13.1238754684177,-19.3941505976267,
0.));
#190103=CARTESIAN_POINT('Ctrl Pts',(13.1238754684177,-19.3941505976267,
12.));
#190104=CARTESIAN_POINT('Ctrl Pts',(13.1295425661635,-19.4112001703561,
0.));
#190105=CARTESIAN_POINT('Ctrl Pts',(13.1295425661635,-19.4112001703561,
12.));
#190106=CARTESIAN_POINT('Ctrl Pts',(13.1352002559439,-19.4283838105265,
0.));
#190107=CARTESIAN_POINT('Ctrl Pts',(13.1352002559439,-19.4283838105265,
12.));
#190108=CARTESIAN_POINT('Ctrl Pts',(13.140847672006,-19.4457006178875,0.));
#190109=CARTESIAN_POINT('Ctrl Pts',(13.140847672006,-19.4457006178875,12.));
#190110=CARTESIAN_POINT('Ctrl Pts',(13.1464839629966,-19.463149704325,0.));
#190111=CARTESIAN_POINT('Ctrl Pts',(13.1464839629966,-19.463149704325,12.));
#190112=CARTESIAN_POINT('Ctrl Pts',(13.1521082915846,-19.4807301935256,
0.));
#190113=CARTESIAN_POINT('Ctrl Pts',(13.1521082915846,-19.4807301935256,
12.));
#190114=CARTESIAN_POINT('Ctrl Pts',(13.1577198341238,-19.498441220707,0.));
#190115=CARTESIAN_POINT('Ctrl Pts',(13.1577198341238,-19.498441220707,12.));
#190116=CARTESIAN_POINT('Ctrl Pts',(13.1633177803097,-19.5162819323207,
0.));
#190117=CARTESIAN_POINT('Ctrl Pts',(13.1633177803097,-19.5162819323207,
12.));
#190118=CARTESIAN_POINT('Ctrl Pts',(13.1689013328432,-19.5342514857564,
0.));
#190119=CARTESIAN_POINT('Ctrl Pts',(13.1689013328432,-19.5342514857564,
12.));
#190120=CARTESIAN_POINT('Ctrl Pts',(13.1744697070918,-19.5523490490254,
0.));
#190121=CARTESIAN_POINT('Ctrl Pts',(13.1744697070918,-19.5523490490254,
12.));
#190122=CARTESIAN_POINT('Ctrl Pts',(13.1800221307682,-19.5705738004682,
0.));
#190123=CARTESIAN_POINT('Ctrl Pts',(13.1800221307682,-19.5705738004682,
12.));
#190124=CARTESIAN_POINT('Ctrl Pts',(13.1855578436479,-19.5889249285352,
0.));
#190125=CARTESIAN_POINT('Ctrl Pts',(13.1855578436479,-19.5889249285352,
12.));
#190126=CARTESIAN_POINT('Ctrl Pts',(13.1910760972818,-19.6074016315421,
0.));
#190127=CARTESIAN_POINT('Ctrl Pts',(13.1910760972818,-19.6074016315421,
12.));
#190128=CARTESIAN_POINT('Ctrl Pts',(13.196576154715,-19.6260031174244,0.));
#190129=CARTESIAN_POINT('Ctrl Pts',(13.196576154715,-19.6260031174244,12.));
#190130=CARTESIAN_POINT('Ctrl Pts',(13.202057290206,-19.6447286034764,0.));
#190131=CARTESIAN_POINT('Ctrl Pts',(13.202057290206,-19.6447286034764,12.));
#190132=CARTESIAN_POINT('Ctrl Pts',(13.2075187889522,-19.6635773160924,
0.));
#190133=CARTESIAN_POINT('Ctrl Pts',(13.2075187889522,-19.6635773160924,
12.));
#190134=CARTESIAN_POINT('Ctrl Pts',(13.2129599468478,-19.6825484905812,
0.));
#190135=CARTESIAN_POINT('Ctrl Pts',(13.2129599468478,-19.6825484905812,
12.));
#190136=CARTESIAN_POINT('Ctrl Pts',(13.2183800702431,-19.7016413709678,
0.));
#190137=CARTESIAN_POINT('Ctrl Pts',(13.2183800702431,-19.7016413709678,
12.));
#190138=CARTESIAN_POINT('Ctrl Pts',(13.2237784757065,-19.7208552097867,
0.));
#190139=CARTESIAN_POINT('Ctrl Pts',(13.2237784757065,-19.7208552097867,
12.));
#190140=CARTESIAN_POINT('Ctrl Pts',(13.2291544897902,-19.7401892678701,
0.));
#190141=CARTESIAN_POINT('Ctrl Pts',(13.2291544897902,-19.7401892678701,
12.));
#190142=CARTESIAN_POINT('Ctrl Pts',(13.2345074487968,-19.7596428141176,
0.));
#190143=CARTESIAN_POINT('Ctrl Pts',(13.2345074487968,-19.7596428141176,
12.));
#190144=CARTESIAN_POINT('Ctrl Pts',(13.239836698568,-19.7792151253297,0.));
#190145=CARTESIAN_POINT('Ctrl Pts',(13.239836698568,-19.7792151253297,12.));
#190146=CARTESIAN_POINT('Ctrl Pts',(13.2451415942809,-19.7989054860501,
0.));
#190147=CARTESIAN_POINT('Ctrl Pts',(13.2451415942809,-19.7989054860501,
12.));
#190148=CARTESIAN_POINT('Ctrl Pts',(13.2504215002458,-19.8187131883919,
0.));
#190149=CARTESIAN_POINT('Ctrl Pts',(13.2504215002458,-19.8187131883919,
12.));
#190150=CARTESIAN_POINT('Ctrl Pts',(13.2556757897085,-19.8386375318632,
0.));
#190151=CARTESIAN_POINT('Ctrl Pts',(13.2556757897085,-19.8386375318632,
12.));
#190152=CARTESIAN_POINT('Ctrl Pts',(13.2609038446525,-19.8586778231711,
0.));
#190153=CARTESIAN_POINT('Ctrl Pts',(13.2609038446525,-19.8586778231711,
12.));
#190154=CARTESIAN_POINT('Ctrl Pts',(13.2661050556128,-19.8788333760571,
0.));
#190155=CARTESIAN_POINT('Ctrl Pts',(13.2661050556128,-19.8788333760571,
12.));
#190156=CARTESIAN_POINT('Ctrl Pts',(13.2712788215015,-19.8991035111739,
0.));
#190157=CARTESIAN_POINT('Ctrl Pts',(13.2712788215015,-19.8991035111739,
12.));
#190158=CARTESIAN_POINT('Ctrl Pts',(13.2764245494354,-19.9194875559419,
0.));
#190159=CARTESIAN_POINT('Ctrl Pts',(13.2764245494354,-19.9194875559419,
12.));
#190160=CARTESIAN_POINT('Ctrl Pts',(13.2815416545662,-19.939984844402,0.));
#190161=CARTESIAN_POINT('Ctrl Pts',(13.2815416545662,-19.939984844402,12.));
#190162=CARTESIAN_POINT('Ctrl Pts',(13.2866295599152,-19.9605947170589,
0.));
#190163=CARTESIAN_POINT('Ctrl Pts',(13.2866295599152,-19.9605947170589,
12.));
#190164=CARTESIAN_POINT('Ctrl Pts',(13.2916876962098,-19.9813165207174,
0.));
#190165=CARTESIAN_POINT('Ctrl Pts',(13.2916876962098,-19.9813165207174,
12.));
#190166=CARTESIAN_POINT('Ctrl Pts',(13.296715501731,-20.0021496083742,0.));
#190167=CARTESIAN_POINT('Ctrl Pts',(13.296715501731,-20.0021496083742,12.));
#190168=CARTESIAN_POINT('Ctrl Pts',(13.3017124221639,-20.023093339104,0.));
#190169=CARTESIAN_POINT('Ctrl Pts',(13.3017124221639,-20.023093339104,12.));
#190170=CARTESIAN_POINT('Ctrl Pts',(13.3066779104515,-20.0441470779345,
0.));
#190171=CARTESIAN_POINT('Ctrl Pts',(13.3066779104515,-20.0441470779345,
12.));
#190172=CARTESIAN_POINT('Ctrl Pts',(13.3116114266514,-20.0653101957188,
0.));
#190173=CARTESIAN_POINT('Ctrl Pts',(13.3116114266514,-20.0653101957188,
12.));
#190174=CARTESIAN_POINT('Ctrl Pts',(13.3165124377962,-20.0865820689884,
0.));
#190175=CARTESIAN_POINT('Ctrl Pts',(13.3165124377962,-20.0865820689884,
12.));
#190176=CARTESIAN_POINT('Ctrl Pts',(13.3213804177588,-20.1079620798377,
0.));
#190177=CARTESIAN_POINT('Ctrl Pts',(13.3213804177588,-20.1079620798377,
12.));
#190178=CARTESIAN_POINT('Ctrl Pts',(13.3262148471228,-20.1294496158405,
0.));
#190179=CARTESIAN_POINT('Ctrl Pts',(13.3262148471228,-20.1294496158405,
12.));
#190180=CARTESIAN_POINT('Ctrl Pts',(13.3310152130565,-20.1510440699477,
0.));
#190181=CARTESIAN_POINT('Ctrl Pts',(13.3310152130565,-20.1510440699477,
12.));
#190182=CARTESIAN_POINT('Ctrl Pts',(13.3357810091903,-20.1727448403818,
0.));
#190183=CARTESIAN_POINT('Ctrl Pts',(13.3357810091903,-20.1727448403818,
12.));
#190184=CARTESIAN_POINT('Ctrl Pts',(13.3405117354969,-20.1945513305233,
0.));
#190185=CARTESIAN_POINT('Ctrl Pts',(13.3405117354969,-20.1945513305233,
12.));
#190186=CARTESIAN_POINT('Ctrl Pts',(13.3452068981762,-20.2164629487855,
0.));
#190187=CARTESIAN_POINT('Ctrl Pts',(13.3452068981762,-20.2164629487855,
12.));
#190188=CARTESIAN_POINT('Ctrl Pts',(13.3498660095381,-20.2384791085354,
0.));
#190189=CARTESIAN_POINT('Ctrl Pts',(13.3498660095381,-20.2384791085354,
12.));
#190190=CARTESIAN_POINT('Ctrl Pts',(13.3544885878886,-20.2605992280117,
0.));
#190191=CARTESIAN_POINT('Ctrl Pts',(13.3544885878886,-20.2605992280117,
12.));
#190192=CARTESIAN_POINT('Ctrl Pts',(13.3590741574194,-20.2828227302337,
0.));
#190193=CARTESIAN_POINT('Ctrl Pts',(13.3590741574194,-20.2828227302337,
12.));
#190194=CARTESIAN_POINT('Ctrl Pts',(13.3636222481016,-20.3051490429049,
0.));
#190195=CARTESIAN_POINT('Ctrl Pts',(13.3636222481016,-20.3051490429049,
12.));
#190196=CARTESIAN_POINT('Ctrl Pts',(13.3681323955828,-20.3275775983032,
0.));
#190197=CARTESIAN_POINT('Ctrl Pts',(13.3681323955828,-20.3275775983032,
12.));
#190198=CARTESIAN_POINT('Ctrl Pts',(13.3726041410869,-20.3501078331818,
0.));
#190199=CARTESIAN_POINT('Ctrl Pts',(13.3726041410869,-20.3501078331818,
12.));
#190200=CARTESIAN_POINT('Ctrl Pts',(13.377037031319,-20.3727391887187,0.));
#190201=CARTESIAN_POINT('Ctrl Pts',(13.377037031319,-20.3727391887187,12.));
#190202=CARTESIAN_POINT('Ctrl Pts',(13.3814306183721,-20.3954711104505,
0.));
#190203=CARTESIAN_POINT('Ctrl Pts',(13.3814306183721,-20.3954711104505,
12.));
#190204=CARTESIAN_POINT('Ctrl Pts',(13.3857844596387,-20.4183030482002,
0.));
#190205=CARTESIAN_POINT('Ctrl Pts',(13.3857844596387,-20.4183030482002,
12.));
#190206=CARTESIAN_POINT('Ctrl Pts',(13.3900981177254,-20.4412344560007,
0.));
#190207=CARTESIAN_POINT('Ctrl Pts',(13.3900981177254,-20.4412344560007,
12.));
#190208=CARTESIAN_POINT('Ctrl Pts',(13.3943711603739,-20.4642647920038,
0.));
#190209=CARTESIAN_POINT('Ctrl Pts',(13.3943711603739,-20.4642647920038,
12.));
#190210=CARTESIAN_POINT('Ctrl Pts',(13.3986031603716,-20.4873935184041,
0.));
#190211=CARTESIAN_POINT('Ctrl Pts',(13.3986031603716,-20.4873935184041,
12.));
#190212=CARTESIAN_POINT('Ctrl Pts',(13.4027936954529,-20.5106201013755,
0.));
#190213=CARTESIAN_POINT('Ctrl Pts',(13.4027936954529,-20.5106201013755,
12.));
#190214=CARTESIAN_POINT('Ctrl Pts',(13.4069423482076,-20.5339440109958,
0.));
#190215=CARTESIAN_POINT('Ctrl Pts',(13.4069423482076,-20.5339440109958,
12.));
#190216=CARTESIAN_POINT('Ctrl Pts',(13.4110487059912,-20.557364721164,0.));
#190217=CARTESIAN_POINT('Ctrl Pts',(13.4110487059912,-20.557364721164,12.));
#190218=CARTESIAN_POINT('Ctrl Pts',(13.415112360841,-20.5808817095155,0.));
#190219=CARTESIAN_POINT('Ctrl Pts',(13.415112360841,-20.5808817095155,12.));
#190220=CARTESIAN_POINT('Ctrl Pts',(13.4191329093931,-20.6044944573151,
0.));
#190221=CARTESIAN_POINT('Ctrl Pts',(13.4191329093931,-20.6044944573151,
12.));
#190222=CARTESIAN_POINT('Ctrl Pts',(13.4231099528178,-20.6282024494234,
0.));
#190223=CARTESIAN_POINT('Ctrl Pts',(13.4231099528178,-20.6282024494234,
12.));
#190224=CARTESIAN_POINT('Ctrl Pts',(13.427043096765,-20.6520051742868,0.));
#190225=CARTESIAN_POINT('Ctrl Pts',(13.427043096765,-20.6520051742868,12.));
#190226=CARTESIAN_POINT('Ctrl Pts',(13.4309319513119,-20.6759021239102,
0.));
#190227=CARTESIAN_POINT('Ctrl Pts',(13.4309319513119,-20.6759021239102,
12.));
#190228=CARTESIAN_POINT('Ctrl Pts',(13.4347761309154,-20.6998927938288,
0.));
#190229=CARTESIAN_POINT('Ctrl Pts',(13.4347761309154,-20.6998927938288,
12.));
#190230=CARTESIAN_POINT('Ctrl Pts',(13.4385752543663,-20.7239766830676,
0.));
#190231=CARTESIAN_POINT('Ctrl Pts',(13.4385752543663,-20.7239766830676,
12.));
#190232=CARTESIAN_POINT('Ctrl Pts',(13.4423289447561,-20.7481532941014,
0.));
#190233=CARTESIAN_POINT('Ctrl Pts',(13.4423289447561,-20.7481532941014,
12.));
#190234=CARTESIAN_POINT('Ctrl Pts',(13.4460368293689,-20.7724221327609,
0.));
#190235=CARTESIAN_POINT('Ctrl Pts',(13.4460368293689,-20.7724221327609,
12.));
#190236=CARTESIAN_POINT('Ctrl Pts',(13.4496985395637,-20.7967827081228,
0.));
#190237=CARTESIAN_POINT('Ctrl Pts',(13.4496985395637,-20.7967827081228,
12.));
#190238=CARTESIAN_POINT('Ctrl Pts',(13.4533137106667,-20.821234532398,0.));
#190239=CARTESIAN_POINT('Ctrl Pts',(13.4533137106667,-20.821234532398,12.));
#190240=CARTESIAN_POINT('Ctrl Pts',(13.4568819818631,-20.8457771208083,
0.));
#190241=CARTESIAN_POINT('Ctrl Pts',(13.4568819818631,-20.8457771208083,
12.));
#190242=CARTESIAN_POINT('Ctrl Pts',(13.4604029960983,-20.8704099914641,
0.));
#190243=CARTESIAN_POINT('Ctrl Pts',(13.4604029960983,-20.8704099914641,
12.));
#190244=CARTESIAN_POINT('Ctrl Pts',(13.4638763999725,-20.8951326652158,
0.));
#190245=CARTESIAN_POINT('Ctrl Pts',(13.4638763999725,-20.8951326652158,
12.));
#190246=CARTESIAN_POINT('Ctrl Pts',(13.4673018437717,-20.9199446657583,
0.));
#190247=CARTESIAN_POINT('Ctrl Pts',(13.4673018437717,-20.9199446657583,
12.));
#190248=CARTESIAN_POINT('Ctrl Pts',(13.4706789815166,-20.9448455197557,
0.));
#190249=CARTESIAN_POINT('Ctrl Pts',(13.4706789815166,-20.9448455197557,
12.));
#190250=CARTESIAN_POINT('Ctrl Pts',(13.4740074710086,-20.9698347569477,
0.));
#190251=CARTESIAN_POINT('Ctrl Pts',(13.4740074710086,-20.9698347569477,
12.));
#190252=CARTESIAN_POINT('Ctrl Pts',(13.4772869738878,-20.9949119102592,
0.));
#190253=CARTESIAN_POINT('Ctrl Pts',(13.4772869738878,-20.9949119102592,
12.));
#190254=CARTESIAN_POINT('Ctrl Pts',(13.4805171556822,-21.0200765158884,
0.));
#190255=CARTESIAN_POINT('Ctrl Pts',(13.4805171556822,-21.0200765158884,
12.));
#190256=CARTESIAN_POINT('Ctrl Pts',(13.4836976858912,-21.0453281134245,
0.));
#190257=CARTESIAN_POINT('Ctrl Pts',(13.4836976858912,-21.0453281134245,
12.));
#190258=CARTESIAN_POINT('Ctrl Pts',(13.4868282377191,-21.0706662455199,
0.));
#190259=CARTESIAN_POINT('Ctrl Pts',(13.4868282377191,-21.0706662455199,
12.));
#190260=CARTESIAN_POINT('Ctrl Pts',(13.4899084877717,-21.0960904575046,
0.));
#190261=CARTESIAN_POINT('Ctrl Pts',(13.4899084877717,-21.0960904575046,
12.));
#190262=CARTESIAN_POINT('Ctrl Pts',(13.4929381157778,-21.1216002970207,
0.));
#190263=CARTESIAN_POINT('Ctrl Pts',(13.4929381157778,-21.1216002970207,
12.));
#190264=CARTESIAN_POINT('Ctrl Pts',(13.4959168042934,-21.1471953136209,
0.));
#190265=CARTESIAN_POINT('Ctrl Pts',(13.4959168042934,-21.1471953136209,
12.));
#190266=CARTESIAN_POINT('Ctrl Pts',(13.4988442384491,-21.1728750584175,
0.));
#190267=CARTESIAN_POINT('Ctrl Pts',(13.4988442384491,-21.1728750584175,
12.));
#190268=CARTESIAN_POINT('Ctrl Pts',(13.5017201056088,-21.1986390835828,
0.));
#190269=CARTESIAN_POINT('Ctrl Pts',(13.5017201056088,-21.1986390835828,
12.));
#190270=CARTESIAN_POINT('Ctrl Pts',(13.5045440957404,-21.2244869429332,
0.));
#190271=CARTESIAN_POINT('Ctrl Pts',(13.5045440957404,-21.2244869429332,
12.));
#190272=CARTESIAN_POINT('Ctrl Pts',(13.5073159019452,-21.250418192743,0.));
#190273=CARTESIAN_POINT('Ctrl Pts',(13.5073159019452,-21.250418192743,12.));
#190274=CARTESIAN_POINT('Ctrl Pts',(13.5100352209205,-21.2764323924442,
0.));
#190275=CARTESIAN_POINT('Ctrl Pts',(13.5100352209205,-21.2764323924442,
12.));
#190276=CARTESIAN_POINT('Ctrl Pts',(13.5127017534971,-21.3025291054235,
0.));
#190277=CARTESIAN_POINT('Ctrl Pts',(13.5127017534971,-21.3025291054235,
12.));
#190278=CARTESIAN_POINT('Ctrl Pts',(13.5153152050555,-21.3287078996341,
0.));
#190279=CARTESIAN_POINT('Ctrl Pts',(13.5153152050555,-21.3287078996341,
12.));
#190280=CARTESIAN_POINT('Ctrl Pts',(13.5178752862466,-21.3549683486222,
0.));
#190281=CARTESIAN_POINT('Ctrl Pts',(13.5178752862466,-21.3549683486222,
12.));
#190282=CARTESIAN_POINT('Ctrl Pts',(13.5203817122503,-21.3813100304973,
0.));
#190283=CARTESIAN_POINT('Ctrl Pts',(13.5203817122503,-21.3813100304973,
12.));
#190284=CARTESIAN_POINT('Ctrl Pts',(13.5228342013516,-21.4077325259324,
0.));
#190285=CARTESIAN_POINT('Ctrl Pts',(13.5228342013516,-21.4077325259324,
12.));
#190286=CARTESIAN_POINT('Ctrl Pts',(13.5252324737801,-21.4342354165259,
0.));
#190287=CARTESIAN_POINT('Ctrl Pts',(13.5252324737801,-21.4342354165259,
12.));
#190288=CARTESIAN_POINT('Ctrl Pts',(13.5275762503555,-21.4608182828697,
0.));
#190289=CARTESIAN_POINT('Ctrl Pts',(13.5275762503555,-21.4608182828697,
12.));
#190290=CARTESIAN_POINT('Ctrl Pts',(13.5298652514355,-21.4874807030468,
0.));
#190291=CARTESIAN_POINT('Ctrl Pts',(13.5298652514355,-21.4874807030468,
12.));
#190292=CARTESIAN_POINT('Ctrl Pts',(13.5320991952138,-21.5142222501666,
0.));
#190293=CARTESIAN_POINT('Ctrl Pts',(13.5320991952138,-21.5142222501666,
12.));
#190294=CARTESIAN_POINT('Ctrl Pts',(13.5342777983214,-21.5410424932503,
0.));
#190295=CARTESIAN_POINT('Ctrl Pts',(13.5342777983214,-21.5410424932503,
12.));
#190296=CARTESIAN_POINT('Ctrl Pts',(13.536400779028,-21.5679410019002,0.));
#190297=CARTESIAN_POINT('Ctrl Pts',(13.536400779028,-21.5679410019002,12.));
#190298=CARTESIAN_POINT('Ctrl Pts',(13.5384678597195,-21.5949173499013,
0.));
#190299=CARTESIAN_POINT('Ctrl Pts',(13.5384678597195,-21.5949173499013,
12.));
#190300=CARTESIAN_POINT('Ctrl Pts',(13.5404787697791,-21.6219711193946,
0.));
#190301=CARTESIAN_POINT('Ctrl Pts',(13.5404787697791,-21.6219711193946,
12.));
#190302=CARTESIAN_POINT('Ctrl Pts',(13.5424332480699,-21.6491019044648,
0.));
#190303=CARTESIAN_POINT('Ctrl Pts',(13.5424332480699,-21.6491019044648,
12.));
#190304=CARTESIAN_POINT('Ctrl Pts',(13.5443310461526,-21.6763093157699,
0.));
#190305=CARTESIAN_POINT('Ctrl Pts',(13.5443310461526,-21.6763093157699,
12.));
#190306=CARTESIAN_POINT('Ctrl Pts',(13.5461719295048,-21.7035929822955,
0.));
#190307=CARTESIAN_POINT('Ctrl Pts',(13.5461719295048,-21.7035929822955,
12.));
#190308=CARTESIAN_POINT('Ctrl Pts',(13.5479556704481,-21.7309525412281,
0.));
#190309=CARTESIAN_POINT('Ctrl Pts',(13.5479556704481,-21.7309525412281,
12.));
#190310=CARTESIAN_POINT('Ctrl Pts',(13.5496820422211,-21.7583876294554,
0.));
#190311=CARTESIAN_POINT('Ctrl Pts',(13.5496820422211,-21.7583876294554,
12.));
#190312=CARTESIAN_POINT('Ctrl Pts',(13.551350812725,-21.7858978745865,0.));
#190313=CARTESIAN_POINT('Ctrl Pts',(13.551350812725,-21.7858978745865,12.));
#190314=CARTESIAN_POINT('Ctrl Pts',(13.5529617381573,-21.8134828857967,
0.));
#190315=CARTESIAN_POINT('Ctrl Pts',(13.5529617381573,-21.8134828857967,
12.));
#190316=CARTESIAN_POINT('Ctrl Pts',(13.5545145573031,-21.8411422456075,
0.));
#190317=CARTESIAN_POINT('Ctrl Pts',(13.5545145573031,-21.8411422456075,
12.));
#190318=CARTESIAN_POINT('Ctrl Pts',(13.5560089839385,-21.8688754989365,
0.));
#190319=CARTESIAN_POINT('Ctrl Pts',(13.5560089839385,-21.8688754989365,
12.));
#190320=CARTESIAN_POINT('Ctrl Pts',(13.5574447178424,-21.8966821688824,
0.));
#190321=CARTESIAN_POINT('Ctrl Pts',(13.5574447178424,-21.8966821688824,
12.));
#190322=CARTESIAN_POINT('Ctrl Pts',(13.5588214586604,-21.9245617765769,
0.));
#190323=CARTESIAN_POINT('Ctrl Pts',(13.5588214586604,-21.9245617765769,
12.));
#190324=CARTESIAN_POINT('Ctrl Pts',(13.5601389185257,-21.9525138592813,
0.));
#190325=CARTESIAN_POINT('Ctrl Pts',(13.5601389185257,-21.9525138592813,
12.));
#190326=CARTESIAN_POINT('Ctrl Pts',(13.5613968357561,-21.9805379899168,
0.));
#190327=CARTESIAN_POINT('Ctrl Pts',(13.5613968357561,-21.9805379899168,
12.));
#190328=CARTESIAN_POINT('Ctrl Pts',(13.5625949868333,-22.0086337943449,
0.));
#190329=CARTESIAN_POINT('Ctrl Pts',(13.5625949868333,-22.0086337943449,
12.));
#190330=CARTESIAN_POINT('Ctrl Pts',(13.5637332022473,-22.0368009736295,
0.));
#190331=CARTESIAN_POINT('Ctrl Pts',(13.5637332022473,-22.0368009736295,
12.));
#190332=CARTESIAN_POINT('Ctrl Pts',(13.5648113689033,-22.065039308961,0.));
#190333=CARTESIAN_POINT('Ctrl Pts',(13.5648113689033,-22.065039308961,12.));
#190334=CARTESIAN_POINT('Ctrl Pts',(13.5658294169284,-22.0933486464593,
0.));
#190335=CARTESIAN_POINT('Ctrl Pts',(13.5658294169284,-22.0933486464593,
12.));
#190336=CARTESIAN_POINT('Ctrl Pts',(13.5667873105359,-22.1217288871975,
0.));
#190337=CARTESIAN_POINT('Ctrl Pts',(13.5667873105359,-22.1217288871975,
12.));
#190338=CARTESIAN_POINT('Ctrl Pts',(13.5675054919061,-22.1444897575194,
0.));
#190339=CARTESIAN_POINT('Ctrl Pts',(13.5675054919061,-22.1444897575194,
12.));
#190340=CARTESIAN_POINT('Ctrl Pts',(13.5680170531805,-22.1615922805008,
0.));
#190341=CARTESIAN_POINT('Ctrl Pts',(13.5680170531805,-22.1615922805008,
12.));
#190342=CARTESIAN_POINT('Ctrl Pts',(13.5683460612942,-22.1730081264608,
0.));
#190343=CARTESIAN_POINT('Ctrl Pts',(13.5683460612942,-22.1730081264608,
12.));
#190344=CARTESIAN_POINT('Ctrl Pts',(13.5685075571671,-22.178719590434,0.));
#190345=CARTESIAN_POINT('Ctrl Pts',(13.5685075571671,-22.178719590434,12.));
#190346=CARTESIAN_POINT('',(13.5685075571671,-22.178719590434,0.));
#190347=CARTESIAN_POINT('Ctrl Pts',(12.7689476255362,-18.5896416359912,
0.));
#190348=CARTESIAN_POINT('Ctrl Pts',(12.7689524524483,-18.5896460962964,
0.));
#190349=CARTESIAN_POINT('Ctrl Pts',(12.768986426692,-18.5896919669165,0.));
#190350=CARTESIAN_POINT('Ctrl Pts',(12.769110348199,-18.589871621843,0.));
#190351=CARTESIAN_POINT('Ctrl Pts',(12.7694215127918,-18.5903328777227,
0.));
#190352=CARTESIAN_POINT('Ctrl Pts',(12.7700520897173,-18.5912775137806,
0.));
#190353=CARTESIAN_POINT('Ctrl Pts',(12.7709195951156,-18.5925859134579,
0.));
#190354=CARTESIAN_POINT('Ctrl Pts',(12.7720142287172,-18.5942490615407,
0.));
#190355=CARTESIAN_POINT('Ctrl Pts',(12.7733231262108,-18.5962551167772,
0.));
#190356=CARTESIAN_POINT('Ctrl Pts',(12.7748328937638,-18.598591752595,0.));
#190357=CARTESIAN_POINT('Ctrl Pts',(12.7765325225081,-18.6012488486709,
0.));
#190358=CARTESIAN_POINT('Ctrl Pts',(12.7784139605066,-18.6042190183704,
0.));
#190359=CARTESIAN_POINT('Ctrl Pts',(12.7804705387658,-18.6074961535723,
0.));
#190360=CARTESIAN_POINT('Ctrl Pts',(12.7826959526924,-18.611074482622,0.));
#190361=CARTESIAN_POINT('Ctrl Pts',(12.7850831657901,-18.6149475565188,
0.));
#190362=CARTESIAN_POINT('Ctrl Pts',(12.7876249657834,-18.6191087624752,
0.));
#190363=CARTESIAN_POINT('Ctrl Pts',(12.7903142925234,-18.6235516265575,
0.));
#190364=CARTESIAN_POINT('Ctrl Pts',(12.7931447451555,-18.6282702819371,
0.));
#190365=CARTESIAN_POINT('Ctrl Pts',(12.796110622225,-18.6332595057006,0.));
#190366=CARTESIAN_POINT('Ctrl Pts',(12.7992066625264,-18.63851447924,0.));
#190367=CARTESIAN_POINT('Ctrl Pts',(12.8024278770152,-18.6440306327456,
0.));
#190368=CARTESIAN_POINT('Ctrl Pts',(12.805769331162,-18.6498034438987,0.));
#190369=CARTESIAN_POINT('Ctrl Pts',(12.8092261933858,-18.6558284825773,
0.));
#190370=CARTESIAN_POINT('Ctrl Pts',(12.8127937909631,-18.6621014624746,
0.));
#190371=CARTESIAN_POINT('Ctrl Pts',(12.8164676687362,-18.66861829528,0.));
#190372=CARTESIAN_POINT('Ctrl Pts',(12.8202436318474,-18.6753751301092,
0.));
#190373=CARTESIAN_POINT('Ctrl Pts',(12.8241176980017,-18.6823683094139,
0.));
#190374=CARTESIAN_POINT('Ctrl Pts',(12.8280860635231,-18.6895943376172,
0.));
#190375=CARTESIAN_POINT('Ctrl Pts',(12.8321450599789,-18.6970498410172,
0.));
#190376=CARTESIAN_POINT('Ctrl Pts',(12.8362911280361,-18.7047315436294,
0.));
#190377=CARTESIAN_POINT('Ctrl Pts',(12.8405208263431,-18.7126362754445,
0.));
#190378=CARTESIAN_POINT('Ctrl Pts',(12.8448308329494,-18.7207609737702,
0.));
#190379=CARTESIAN_POINT('Ctrl Pts',(12.8492179511591,-18.7291026886554,
0.));
#190380=CARTESIAN_POINT('Ctrl Pts',(12.8536791086316,-18.7376585820854,
0.));
#190381=CARTESIAN_POINT('Ctrl Pts',(12.8582113455646,-18.7464259171251,
0.));
#190382=CARTESIAN_POINT('Ctrl Pts',(12.8628118054171,-18.7554020493887,
0.));
#190383=CARTESIAN_POINT('Ctrl Pts',(12.8674777239653,-18.7645844169564,
0.));
#190384=CARTESIAN_POINT('Ctrl Pts',(12.872206421181,-18.7739705329022,0.));
#190385=CARTESIAN_POINT('Ctrl Pts',(12.8769952998095,-18.7835579840477,
0.));
#190386=CARTESIAN_POINT('Ctrl Pts',(12.8818418427475,-18.7933444285868,
0.));
#190387=CARTESIAN_POINT('Ctrl Pts',(12.8867436109546,-18.8033275941943,
0.));
#190388=CARTESIAN_POINT('Ctrl Pts',(12.8916982409935,-18.813505275782,0.));
#190389=CARTESIAN_POINT('Ctrl Pts',(12.8967034410754,-18.8238753319129,
0.));
#190390=CARTESIAN_POINT('Ctrl Pts',(12.9017569871738,-18.8344356812591,
0.));
#190391=CARTESIAN_POINT('Ctrl Pts',(12.9068567191854,-18.8451842990984,
0.));
#190392=CARTESIAN_POINT('Ctrl Pts',(12.9120005369063,-18.8561192136198,
0.));
#190393=CARTESIAN_POINT('Ctrl Pts',(12.9171863977045,-18.8672385038326,
0.));
#190394=CARTESIAN_POINT('Ctrl Pts',(12.9224123144981,-18.8785402977528,
0.));
#190395=CARTESIAN_POINT('Ctrl Pts',(12.9276763536373,-18.8900227704889,
0.));
#190396=CARTESIAN_POINT('Ctrl Pts',(12.9329766328184,-18.9016841423403,
0.));
#190397=CARTESIAN_POINT('Ctrl Pts',(12.9383113190374,-18.9135226769466,
0.));
#190398=CARTESIAN_POINT('Ctrl Pts',(12.9436786266105,-18.9255366795195,
0.));
#190399=CARTESIAN_POINT('Ctrl Pts',(12.9490768151821,-18.9377244950435,
0.));
#190400=CARTESIAN_POINT('Ctrl Pts',(12.9545041877377,-18.9500845064715,
0.));
#190401=CARTESIAN_POINT('Ctrl Pts',(12.9599590886319,-18.9626151329229,
0.));
#190402=CARTESIAN_POINT('Ctrl Pts',(12.9654399021869,-18.9753148284475,
0.));
#190403=CARTESIAN_POINT('Ctrl Pts',(12.9709450512747,-18.9881820807586,
0.));
#190404=CARTESIAN_POINT('Ctrl Pts',(12.9764729959205,-19.0012154099791,
0.));
#190405=CARTESIAN_POINT('Ctrl Pts',(12.9820222318715,-19.0144133673348,
0.));
#190406=CARTESIAN_POINT('Ctrl Pts',(12.9875912893003,-19.0277745339908,
0.));
#190407=CARTESIAN_POINT('Ctrl Pts',(12.9931787316514,-19.0412975200398,
0.));
#190408=CARTESIAN_POINT('Ctrl Pts',(12.9987831544502,-19.0549809634355,
0.));
#190409=CARTESIAN_POINT('Ctrl Pts',(13.0044031841381,-19.0688235289437,
0.));
#190410=CARTESIAN_POINT('Ctrl Pts',(13.0100374768785,-19.0828239070482,
0.));
#190411=CARTESIAN_POINT('Ctrl Pts',(13.0156847176093,-19.0969808131226,
0.));
#190412=CARTESIAN_POINT('Ctrl Pts',(13.0213436191326,-19.1112929866308,
0.));
#190413=CARTESIAN_POINT('Ctrl Pts',(13.0270129211976,-19.1257591903099,
0.));
#190414=CARTESIAN_POINT('Ctrl Pts',(13.0326913895841,-19.1403782093389,
0.));
#190415=CARTESIAN_POINT('Ctrl Pts',(13.0383778152072,-19.1551488505233,
0.));
#190416=CARTESIAN_POINT('Ctrl Pts',(13.0440710133775,-19.1700699416625,
0.));
#190417=CARTESIAN_POINT('Ctrl Pts',(13.0497698230442,-19.1851403308826,
0.));
#190418=CARTESIAN_POINT('Ctrl Pts',(13.0554731060537,-19.2003588859771,
0.));
#190419=CARTESIAN_POINT('Ctrl Pts',(13.0611797463912,-19.2157244937141,
0.));
#190420=CARTESIAN_POINT('Ctrl Pts',(13.0668886494791,-19.2312360592031,
0.));
#190421=CARTESIAN_POINT('Ctrl Pts',(13.0725987415856,-19.2468925053988,
0.));
#190422=CARTESIAN_POINT('Ctrl Pts',(13.0783089692117,-19.2626927725596,
0.));
#190423=CARTESIAN_POINT('Ctrl Pts',(13.0840182984949,-19.2786358177198,
0.));
#190424=CARTESIAN_POINT('Ctrl Pts',(13.0897257145969,-19.2947206141246,
0.));
#190425=CARTESIAN_POINT('Ctrl Pts',(13.095430221148,-19.3109461507358,0.));
#190426=CARTESIAN_POINT('Ctrl Pts',(13.1011308397591,-19.3273114318268,
0.));
#190427=CARTESIAN_POINT('Ctrl Pts',(13.1068266095186,-19.3438154765395,
0.));
#190428=CARTESIAN_POINT('Ctrl Pts',(13.1125165865021,-19.3604573184516,
0.));
#190429=CARTESIAN_POINT('Ctrl Pts',(13.118199843271,-19.3772360051093,0.));
#190430=CARTESIAN_POINT('Ctrl Pts',(13.1238754684177,-19.3941505976267,
0.));
#190431=CARTESIAN_POINT('Ctrl Pts',(13.1295425661635,-19.4112001703561,
0.));
#190432=CARTESIAN_POINT('Ctrl Pts',(13.1352002559439,-19.4283838105265,
0.));
#190433=CARTESIAN_POINT('Ctrl Pts',(13.140847672006,-19.4457006178875,0.));
#190434=CARTESIAN_POINT('Ctrl Pts',(13.1464839629966,-19.463149704325,0.));
#190435=CARTESIAN_POINT('Ctrl Pts',(13.1521082915846,-19.4807301935256,
0.));
#190436=CARTESIAN_POINT('Ctrl Pts',(13.1577198341238,-19.498441220707,0.));
#190437=CARTESIAN_POINT('Ctrl Pts',(13.1633177803097,-19.5162819323207,
0.));
#190438=CARTESIAN_POINT('Ctrl Pts',(13.1689013328432,-19.5342514857564,
0.));
#190439=CARTESIAN_POINT('Ctrl Pts',(13.1744697070918,-19.5523490490254,
0.));
#190440=CARTESIAN_POINT('Ctrl Pts',(13.1800221307682,-19.5705738004682,
0.));
#190441=CARTESIAN_POINT('Ctrl Pts',(13.1855578436479,-19.5889249285352,
0.));
#190442=CARTESIAN_POINT('Ctrl Pts',(13.1910760972818,-19.6074016315421,
0.));
#190443=CARTESIAN_POINT('Ctrl Pts',(13.196576154715,-19.6260031174244,0.));
#190444=CARTESIAN_POINT('Ctrl Pts',(13.202057290206,-19.6447286034764,0.));
#190445=CARTESIAN_POINT('Ctrl Pts',(13.2075187889522,-19.6635773160924,
0.));
#190446=CARTESIAN_POINT('Ctrl Pts',(13.2129599468478,-19.6825484905812,
0.));
#190447=CARTESIAN_POINT('Ctrl Pts',(13.2183800702431,-19.7016413709678,
0.));
#190448=CARTESIAN_POINT('Ctrl Pts',(13.2237784757065,-19.7208552097867,
0.));
#190449=CARTESIAN_POINT('Ctrl Pts',(13.2291544897902,-19.7401892678701,
0.));
#190450=CARTESIAN_POINT('Ctrl Pts',(13.2345074487968,-19.7596428141176,
0.));
#190451=CARTESIAN_POINT('Ctrl Pts',(13.239836698568,-19.7792151253297,0.));
#190452=CARTESIAN_POINT('Ctrl Pts',(13.2451415942809,-19.7989054860501,
0.));
#190453=CARTESIAN_POINT('Ctrl Pts',(13.2504215002458,-19.8187131883919,
0.));
#190454=CARTESIAN_POINT('Ctrl Pts',(13.2556757897085,-19.8386375318632,
0.));
#190455=CARTESIAN_POINT('Ctrl Pts',(13.2609038446525,-19.8586778231711,
0.));
#190456=CARTESIAN_POINT('Ctrl Pts',(13.2661050556128,-19.8788333760571,
0.));
#190457=CARTESIAN_POINT('Ctrl Pts',(13.2712788215015,-19.8991035111739,
0.));
#190458=CARTESIAN_POINT('Ctrl Pts',(13.2764245494354,-19.9194875559419,
0.));
#190459=CARTESIAN_POINT('Ctrl Pts',(13.2815416545662,-19.939984844402,0.));
#190460=CARTESIAN_POINT('Ctrl Pts',(13.2866295599152,-19.9605947170589,
0.));
#190461=CARTESIAN_POINT('Ctrl Pts',(13.2916876962098,-19.9813165207174,
0.));
#190462=CARTESIAN_POINT('Ctrl Pts',(13.296715501731,-20.0021496083742,0.));
#190463=CARTESIAN_POINT('Ctrl Pts',(13.3017124221639,-20.023093339104,0.));
#190464=CARTESIAN_POINT('Ctrl Pts',(13.3066779104515,-20.0441470779345,
0.));
#190465=CARTESIAN_POINT('Ctrl Pts',(13.3116114266514,-20.0653101957188,
0.));
#190466=CARTESIAN_POINT('Ctrl Pts',(13.3165124377962,-20.0865820689884,
0.));
#190467=CARTESIAN_POINT('Ctrl Pts',(13.3213804177588,-20.1079620798377,
0.));
#190468=CARTESIAN_POINT('Ctrl Pts',(13.3262148471228,-20.1294496158405,
0.));
#190469=CARTESIAN_POINT('Ctrl Pts',(13.3310152130565,-20.1510440699477,
0.));
#190470=CARTESIAN_POINT('Ctrl Pts',(13.3357810091903,-20.1727448403818,
0.));
#190471=CARTESIAN_POINT('Ctrl Pts',(13.3405117354969,-20.1945513305233,
0.));
#190472=CARTESIAN_POINT('Ctrl Pts',(13.3452068981762,-20.2164629487855,
0.));
#190473=CARTESIAN_POINT('Ctrl Pts',(13.3498660095381,-20.2384791085354,
0.));
#190474=CARTESIAN_POINT('Ctrl Pts',(13.3544885878886,-20.2605992280117,
0.));
#190475=CARTESIAN_POINT('Ctrl Pts',(13.3590741574194,-20.2828227302337,
0.));
#190476=CARTESIAN_POINT('Ctrl Pts',(13.3636222481016,-20.3051490429049,
0.));
#190477=CARTESIAN_POINT('Ctrl Pts',(13.3681323955828,-20.3275775983032,
0.));
#190478=CARTESIAN_POINT('Ctrl Pts',(13.3726041410869,-20.3501078331818,
0.));
#190479=CARTESIAN_POINT('Ctrl Pts',(13.377037031319,-20.3727391887187,0.));
#190480=CARTESIAN_POINT('Ctrl Pts',(13.3814306183721,-20.3954711104505,
0.));
#190481=CARTESIAN_POINT('Ctrl Pts',(13.3857844596387,-20.4183030482002,
0.));
#190482=CARTESIAN_POINT('Ctrl Pts',(13.3900981177254,-20.4412344560007,
0.));
#190483=CARTESIAN_POINT('Ctrl Pts',(13.3943711603739,-20.4642647920038,
0.));
#190484=CARTESIAN_POINT('Ctrl Pts',(13.3986031603716,-20.4873935184041,
0.));
#190485=CARTESIAN_POINT('Ctrl Pts',(13.4027936954529,-20.5106201013755,
0.));
#190486=CARTESIAN_POINT('Ctrl Pts',(13.4069423482076,-20.5339440109958,
0.));
#190487=CARTESIAN_POINT('Ctrl Pts',(13.4110487059912,-20.557364721164,0.));
#190488=CARTESIAN_POINT('Ctrl Pts',(13.415112360841,-20.5808817095155,0.));
#190489=CARTESIAN_POINT('Ctrl Pts',(13.4191329093931,-20.6044944573151,
0.));
#190490=CARTESIAN_POINT('Ctrl Pts',(13.4231099528178,-20.6282024494234,
0.));
#190491=CARTESIAN_POINT('Ctrl Pts',(13.427043096765,-20.6520051742868,0.));
#190492=CARTESIAN_POINT('Ctrl Pts',(13.4309319513119,-20.6759021239102,
0.));
#190493=CARTESIAN_POINT('Ctrl Pts',(13.4347761309154,-20.6998927938288,
0.));
#190494=CARTESIAN_POINT('Ctrl Pts',(13.4385752543663,-20.7239766830676,
0.));
#190495=CARTESIAN_POINT('Ctrl Pts',(13.4423289447561,-20.7481532941014,
0.));
#190496=CARTESIAN_POINT('Ctrl Pts',(13.4460368293689,-20.7724221327609,
0.));
#190497=CARTESIAN_POINT('Ctrl Pts',(13.4496985395637,-20.7967827081228,
0.));
#190498=CARTESIAN_POINT('Ctrl Pts',(13.4533137106667,-20.821234532398,0.));
#190499=CARTESIAN_POINT('Ctrl Pts',(13.4568819818631,-20.8457771208083,
0.));
#190500=CARTESIAN_POINT('Ctrl Pts',(13.4604029960983,-20.8704099914641,
0.));
#190501=CARTESIAN_POINT('Ctrl Pts',(13.4638763999725,-20.8951326652158,
0.));
#190502=CARTESIAN_POINT('Ctrl Pts',(13.4673018437717,-20.9199446657583,
0.));
#190503=CARTESIAN_POINT('Ctrl Pts',(13.4706789815166,-20.9448455197557,
0.));
#190504=CARTESIAN_POINT('Ctrl Pts',(13.4740074710086,-20.9698347569477,
0.));
#190505=CARTESIAN_POINT('Ctrl Pts',(13.4772869738878,-20.9949119102592,
0.));
#190506=CARTESIAN_POINT('Ctrl Pts',(13.4805171556822,-21.0200765158884,
0.));
#190507=CARTESIAN_POINT('Ctrl Pts',(13.4836976858912,-21.0453281134245,
0.));
#190508=CARTESIAN_POINT('Ctrl Pts',(13.4868282377191,-21.0706662455199,
0.));
#190509=CARTESIAN_POINT('Ctrl Pts',(13.4899084877717,-21.0960904575046,
0.));
#190510=CARTESIAN_POINT('Ctrl Pts',(13.4929381157778,-21.1216002970207,
0.));
#190511=CARTESIAN_POINT('Ctrl Pts',(13.4959168042934,-21.1471953136209,
0.));
#190512=CARTESIAN_POINT('Ctrl Pts',(13.4988442384491,-21.1728750584175,
0.));
#190513=CARTESIAN_POINT('Ctrl Pts',(13.5017201056088,-21.1986390835828,
0.));
#190514=CARTESIAN_POINT('Ctrl Pts',(13.5045440957404,-21.2244869429332,
0.));
#190515=CARTESIAN_POINT('Ctrl Pts',(13.5073159019452,-21.250418192743,0.));
#190516=CARTESIAN_POINT('Ctrl Pts',(13.5100352209205,-21.2764323924442,
0.));
#190517=CARTESIAN_POINT('Ctrl Pts',(13.5127017534971,-21.3025291054235,
0.));
#190518=CARTESIAN_POINT('Ctrl Pts',(13.5153152050555,-21.3287078996341,
0.));
#190519=CARTESIAN_POINT('Ctrl Pts',(13.5178752862466,-21.3549683486222,
0.));
#190520=CARTESIAN_POINT('Ctrl Pts',(13.5203817122503,-21.3813100304973,
0.));
#190521=CARTESIAN_POINT('Ctrl Pts',(13.5228342013516,-21.4077325259324,
0.));
#190522=CARTESIAN_POINT('Ctrl Pts',(13.5252324737801,-21.4342354165259,
0.));
#190523=CARTESIAN_POINT('Ctrl Pts',(13.5275762503555,-21.4608182828697,
0.));
#190524=CARTESIAN_POINT('Ctrl Pts',(13.5298652514355,-21.4874807030468,
0.));
#190525=CARTESIAN_POINT('Ctrl Pts',(13.5320991952138,-21.5142222501666,
0.));
#190526=CARTESIAN_POINT('Ctrl Pts',(13.5342777983214,-21.5410424932503,
0.));
#190527=CARTESIAN_POINT('Ctrl Pts',(13.536400779028,-21.5679410019002,0.));
#190528=CARTESIAN_POINT('Ctrl Pts',(13.5384678597195,-21.5949173499013,
0.));
#190529=CARTESIAN_POINT('Ctrl Pts',(13.5404787697791,-21.6219711193946,
0.));
#190530=CARTESIAN_POINT('Ctrl Pts',(13.5424332480699,-21.6491019044648,
0.));
#190531=CARTESIAN_POINT('Ctrl Pts',(13.5443310461526,-21.6763093157699,
0.));
#190532=CARTESIAN_POINT('Ctrl Pts',(13.5461719295048,-21.7035929822955,
0.));
#190533=CARTESIAN_POINT('Ctrl Pts',(13.5479556704481,-21.7309525412281,
0.));
#190534=CARTESIAN_POINT('Ctrl Pts',(13.5496820422211,-21.7583876294554,
0.));
#190535=CARTESIAN_POINT('Ctrl Pts',(13.551350812725,-21.7858978745865,0.));
#190536=CARTESIAN_POINT('Ctrl Pts',(13.5529617381573,-21.8134828857967,
0.));
#190537=CARTESIAN_POINT('Ctrl Pts',(13.5545145573031,-21.8411422456075,
0.));
#190538=CARTESIAN_POINT('Ctrl Pts',(13.5560089839385,-21.8688754989365,
0.));
#190539=CARTESIAN_POINT('Ctrl Pts',(13.5574447178424,-21.8966821688824,
0.));
#190540=CARTESIAN_POINT('Ctrl Pts',(13.5588214586604,-21.9245617765769,
0.));
#190541=CARTESIAN_POINT('Ctrl Pts',(13.5601389185257,-21.9525138592813,
0.));
#190542=CARTESIAN_POINT('Ctrl Pts',(13.5613968357561,-21.9805379899168,
0.));
#190543=CARTESIAN_POINT('Ctrl Pts',(13.5625949868333,-22.0086337943449,
0.));
#190544=CARTESIAN_POINT('Ctrl Pts',(13.5637332022473,-22.0368009736295,
0.));
#190545=CARTESIAN_POINT('Ctrl Pts',(13.5648113689033,-22.065039308961,0.));
#190546=CARTESIAN_POINT('Ctrl Pts',(13.5658294169284,-22.0933486464593,
0.));
#190547=CARTESIAN_POINT('Ctrl Pts',(13.5667873105359,-22.1217288871975,
0.));
#190548=CARTESIAN_POINT('Ctrl Pts',(13.5675054919061,-22.1444897575194,
0.));
#190549=CARTESIAN_POINT('Ctrl Pts',(13.5680170531805,-22.1615922805008,
0.));
#190550=CARTESIAN_POINT('Ctrl Pts',(13.5683460612942,-22.1730081264608,
0.));
#190551=CARTESIAN_POINT('Ctrl Pts',(13.5685075571671,-22.178719590434,0.));
#190552=CARTESIAN_POINT('',(13.5685075571671,-22.178719590434,0.));
#190553=CARTESIAN_POINT('Origin',(7.17139709155223,-20.2687213152502,0.));
#190554=CARTESIAN_POINT('',(7.52250298901263,-21.2610617890679,0.));
#190555=CARTESIAN_POINT('',(7.52250298901263,-21.2610617890679,0.));
#190556=CARTESIAN_POINT('',(3.58569854577611,-10.1343606576251,0.));
#190557=CARTESIAN_POINT('Ctrl Pts',(12.4230808101438,-22.8400320311649,
0.));
#190558=CARTESIAN_POINT('Ctrl Pts',(12.4230808101438,-22.8400320311649,
12.));
#190559=CARTESIAN_POINT('Ctrl Pts',(12.418215285186,-22.8370364396459,0.));
#190560=CARTESIAN_POINT('Ctrl Pts',(12.418215285186,-22.8370364396459,12.));
#190561=CARTESIAN_POINT('Ctrl Pts',(12.4084933766346,-22.8310435872748,
0.));
#190562=CARTESIAN_POINT('Ctrl Pts',(12.4084933766346,-22.8310435872748,
12.));
#190563=CARTESIAN_POINT('Ctrl Pts',(12.3939379378998,-22.8220493007173,
0.));
#190564=CARTESIAN_POINT('Ctrl Pts',(12.3939379378998,-22.8220493007173,
12.));
#190565=CARTESIAN_POINT('Ctrl Pts',(12.374585536673,-22.81004690224,0.));
#190566=CARTESIAN_POINT('Ctrl Pts',(12.374585536673,-22.81004690224,12.));
#190567=CARTESIAN_POINT('Ctrl Pts',(12.3504864740319,-22.795027221673,0.));
#190568=CARTESIAN_POINT('Ctrl Pts',(12.3504864740319,-22.795027221673,12.));
#190569=CARTESIAN_POINT('Ctrl Pts',(12.3264788926075,-22.7799908974768,
0.));
#190570=CARTESIAN_POINT('Ctrl Pts',(12.3264788926075,-22.7799908974768,
12.));
#190571=CARTESIAN_POINT('Ctrl Pts',(12.3025628601792,-22.764938010105,0.));
#190572=CARTESIAN_POINT('Ctrl Pts',(12.3025628601792,-22.764938010105,12.));
#190573=CARTESIAN_POINT('Ctrl Pts',(12.2787384750742,-22.7498686970069,
0.));
#190574=CARTESIAN_POINT('Ctrl Pts',(12.2787384750742,-22.7498686970069,
12.));
#190575=CARTESIAN_POINT('Ctrl Pts',(12.2550058702395,-22.7347831655287,
0.));
#190576=CARTESIAN_POINT('Ctrl Pts',(12.2550058702395,-22.7347831655287,
12.));
#190577=CARTESIAN_POINT('Ctrl Pts',(12.2313652198061,-22.7196817119374,
0.));
#190578=CARTESIAN_POINT('Ctrl Pts',(12.2313652198061,-22.7196817119374,
12.));
#190579=CARTESIAN_POINT('Ctrl Pts',(12.2078167360284,-22.7045647168747,
0.));
#190580=CARTESIAN_POINT('Ctrl Pts',(12.2078167360284,-22.7045647168747,
12.));
#190581=CARTESIAN_POINT('Ctrl Pts',(12.1843606579261,-22.6894326205037,
0.));
#190582=CARTESIAN_POINT('Ctrl Pts',(12.1843606579261,-22.6894326205037,
12.));
#190583=CARTESIAN_POINT('Ctrl Pts',(12.1609972423099,-22.6742859034944,
0.));
#190584=CARTESIAN_POINT('Ctrl Pts',(12.1609972423099,-22.6742859034944,
12.));
#190585=CARTESIAN_POINT('Ctrl Pts',(12.1377267537145,-22.6591250653965,
0.));
#190586=CARTESIAN_POINT('Ctrl Pts',(12.1377267537145,-22.6591250653965,
12.));
#190587=CARTESIAN_POINT('Ctrl Pts',(12.1145494550383,-22.6439506046605,
0.));
#190588=CARTESIAN_POINT('Ctrl Pts',(12.1145494550383,-22.6439506046605,
12.));
#190589=CARTESIAN_POINT('Ctrl Pts',(12.0914655972823,-22.6287629967056,
0.));
#190590=CARTESIAN_POINT('Ctrl Pts',(12.0914655972823,-22.6287629967056,
12.));
#190591=CARTESIAN_POINT('Ctrl Pts',(12.0684754113862,-22.6135626764898,
0.));
#190592=CARTESIAN_POINT('Ctrl Pts',(12.0684754113862,-22.6135626764898,
12.));
#190593=CARTESIAN_POINT('Ctrl Pts',(12.0455791139128,-22.5983500505644,
0.));
#190594=CARTESIAN_POINT('Ctrl Pts',(12.0455791139128,-22.5983500505644,
12.));
#190595=CARTESIAN_POINT('Ctrl Pts',(12.0227769113127,-22.5831255061282,
0.));
#190596=CARTESIAN_POINT('Ctrl Pts',(12.0227769113127,-22.5831255061282,
12.));
#190597=CARTESIAN_POINT('Ctrl Pts',(12.0000690046694,-22.5678894211181,
0.));
#190598=CARTESIAN_POINT('Ctrl Pts',(12.0000690046694,-22.5678894211181,
12.));
#190599=CARTESIAN_POINT('Ctrl Pts',(11.9774555943496,-22.5526421741158,
0.));
#190600=CARTESIAN_POINT('Ctrl Pts',(11.9774555943496,-22.5526421741158,
12.));
#190601=CARTESIAN_POINT('Ctrl Pts',(11.9549368843997,-22.5373841537307,
0.));
#190602=CARTESIAN_POINT('Ctrl Pts',(11.9549368843997,-22.5373841537307,
12.));
#190603=CARTESIAN_POINT('Ctrl Pts',(11.9325130877803,-22.5221157697883,
0.));
#190604=CARTESIAN_POINT('Ctrl Pts',(11.9325130877803,-22.5221157697883,
12.));
#190605=CARTESIAN_POINT('Ctrl Pts',(11.9101844254557,-22.5068374513973,
0.));
#190606=CARTESIAN_POINT('Ctrl Pts',(11.9101844254557,-22.5068374513973,
12.));
#190607=CARTESIAN_POINT('Ctrl Pts',(11.8879511239942,-22.4915496418485,
0.));
#190608=CARTESIAN_POINT('Ctrl Pts',(11.8879511239942,-22.4915496418485,
12.));
#190609=CARTESIAN_POINT('Ctrl Pts',(11.8658134137019,-22.4762527946702,
0.));
#190610=CARTESIAN_POINT('Ctrl Pts',(11.8658134137019,-22.4762527946702,
12.));
#190611=CARTESIAN_POINT('Ctrl Pts',(11.8437715264487,-22.4609473690472,
0.));
#190612=CARTESIAN_POINT('Ctrl Pts',(11.8437715264487,-22.4609473690472,
12.));
#190613=CARTESIAN_POINT('Ctrl Pts',(11.8218256937889,-22.4456338258735,
0.));
#190614=CARTESIAN_POINT('Ctrl Pts',(11.8218256937889,-22.4456338258735,
12.));
#190615=CARTESIAN_POINT('Ctrl Pts',(11.7999761445173,-22.430312622646,0.));
#190616=CARTESIAN_POINT('Ctrl Pts',(11.7999761445173,-22.430312622646,12.));
#190617=CARTESIAN_POINT('Ctrl Pts',(11.7782231042039,-22.4149842125008,
0.));
#190618=CARTESIAN_POINT('Ctrl Pts',(11.7782231042039,-22.4149842125008,
12.));
#190619=CARTESIAN_POINT('Ctrl Pts',(11.7565667964764,-22.3996490469191,
0.));
#190620=CARTESIAN_POINT('Ctrl Pts',(11.7565667964764,-22.3996490469191,
12.));
#190621=CARTESIAN_POINT('Ctrl Pts',(11.7350074437961,-22.3843075773899,
0.));
#190622=CARTESIAN_POINT('Ctrl Pts',(11.7350074437961,-22.3843075773899,
12.));
#190623=CARTESIAN_POINT('Ctrl Pts',(11.7135452684532,-22.3689602575491,
0.));
#190624=CARTESIAN_POINT('Ctrl Pts',(11.7135452684532,-22.3689602575491,
12.));
#190625=CARTESIAN_POINT('Ctrl Pts',(11.6921804934056,-22.3536075450029,
0.));
#190626=CARTESIAN_POINT('Ctrl Pts',(11.6921804934056,-22.3536075450029,
12.));
#190627=CARTESIAN_POINT('Ctrl Pts',(11.6709133432985,-22.3382499035619,
0.));
#190628=CARTESIAN_POINT('Ctrl Pts',(11.6709133432985,-22.3382499035619,
12.));
#190629=CARTESIAN_POINT('Ctrl Pts',(11.6497440449857,-22.3228878043976,
0.));
#190630=CARTESIAN_POINT('Ctrl Pts',(11.6497440449857,-22.3228878043976,
12.));
#190631=CARTESIAN_POINT('Ctrl Pts',(11.6286728270009,-22.3075217249049,
0.));
#190632=CARTESIAN_POINT('Ctrl Pts',(11.6286728270009,-22.3075217249049,
12.));
#190633=CARTESIAN_POINT('Ctrl Pts',(11.6076999192357,-22.2921521480356,
0.));
#190634=CARTESIAN_POINT('Ctrl Pts',(11.6076999192357,-22.2921521480356,
12.));
#190635=CARTESIAN_POINT('Ctrl Pts',(11.5868255525188,-22.2767795614348,
0.));
#190636=CARTESIAN_POINT('Ctrl Pts',(11.5868255525188,-22.2767795614348,
12.));
#190637=CARTESIAN_POINT('Ctrl Pts',(11.5660499582403,-22.2614044566898,
0.));
#190638=CARTESIAN_POINT('Ctrl Pts',(11.5660499582403,-22.2614044566898,
12.));
#190639=CARTESIAN_POINT('Ctrl Pts',(11.5453733679121,-22.2460273284654,
0.));
#190640=CARTESIAN_POINT('Ctrl Pts',(11.5453733679121,-22.2460273284654,
12.));
#190641=CARTESIAN_POINT('Ctrl Pts',(11.5247960128477,-22.2306486738901,
0.));
#190642=CARTESIAN_POINT('Ctrl Pts',(11.5247960128477,-22.2306486738901,
12.));
#190643=CARTESIAN_POINT('Ctrl Pts',(11.5043181244242,-22.2152689931022,
0.));
#190644=CARTESIAN_POINT('Ctrl Pts',(11.5043181244242,-22.2152689931022,
12.));
#190645=CARTESIAN_POINT('Ctrl Pts',(11.483939934259,-22.1998887896436,0.));
#190646=CARTESIAN_POINT('Ctrl Pts',(11.483939934259,-22.1998887896436,12.));
#190647=CARTESIAN_POINT('Ctrl Pts',(11.463661674411,-22.184508570917,0.));
#190648=CARTESIAN_POINT('Ctrl Pts',(11.463661674411,-22.184508570917,12.));
#190649=CARTESIAN_POINT('Ctrl Pts',(11.443483577557,-22.1691288486096,0.));
#190650=CARTESIAN_POINT('Ctrl Pts',(11.443483577557,-22.1691288486096,12.));
#190651=CARTESIAN_POINT('Ctrl Pts',(11.4234058771742,-22.1537501391487,
0.));
#190652=CARTESIAN_POINT('Ctrl Pts',(11.4234058771742,-22.1537501391487,
12.));
#190653=CARTESIAN_POINT('Ctrl Pts',(11.4034288076908,-22.1383729640964,
0.));
#190654=CARTESIAN_POINT('Ctrl Pts',(11.4034288076908,-22.1383729640964,
12.));
#190655=CARTESIAN_POINT('Ctrl Pts',(11.3835526044256,-22.1229978500186,
0.));
#190656=CARTESIAN_POINT('Ctrl Pts',(11.3835526044256,-22.1229978500186,
12.));
#190657=CARTESIAN_POINT('Ctrl Pts',(11.3637775035367,-22.1076253283979,
0.));
#190658=CARTESIAN_POINT('Ctrl Pts',(11.3637775035367,-22.1076253283979,
12.));
#190659=CARTESIAN_POINT('Ctrl Pts',(11.3441037419553,-22.0922559355294,
0.));
#190660=CARTESIAN_POINT('Ctrl Pts',(11.3441037419553,-22.0922559355294,
12.));
#190661=CARTESIAN_POINT('Ctrl Pts',(11.3245315573168,-22.0768902124267,
0.));
#190662=CARTESIAN_POINT('Ctrl Pts',(11.3245315573168,-22.0768902124267,
12.));
#190663=CARTESIAN_POINT('Ctrl Pts',(11.3050611878771,-22.0615287047179,
0.));
#190664=CARTESIAN_POINT('Ctrl Pts',(11.3050611878771,-22.0615287047179,
12.));
#190665=CARTESIAN_POINT('Ctrl Pts',(11.2856928724374,-22.046171962566,0.));
#190666=CARTESIAN_POINT('Ctrl Pts',(11.2856928724374,-22.046171962566,12.));
#190667=CARTESIAN_POINT('Ctrl Pts',(11.2664268504206,-22.030820540835,0.));
#190668=CARTESIAN_POINT('Ctrl Pts',(11.2664268504206,-22.030820540835,12.));
#190669=CARTESIAN_POINT('Ctrl Pts',(11.2472633619275,-22.0154749992363,
0.));
#190670=CARTESIAN_POINT('Ctrl Pts',(11.2472633619275,-22.0154749992363,
12.));
#190671=CARTESIAN_POINT('Ctrl Pts',(11.2282026477896,-22.0001359024839,
0.));
#190672=CARTESIAN_POINT('Ctrl Pts',(11.2282026477896,-22.0001359024839,
12.));
#190673=CARTESIAN_POINT('Ctrl Pts',(11.2092449496125,-21.9848038204439,
0.));
#190674=CARTESIAN_POINT('Ctrl Pts',(11.2092449496125,-21.9848038204439,
12.));
#190675=CARTESIAN_POINT('Ctrl Pts',(11.190390509811,-21.9694793282914,0.));
#190676=CARTESIAN_POINT('Ctrl Pts',(11.190390509811,-21.9694793282914,12.));
#190677=CARTESIAN_POINT('Ctrl Pts',(11.1716395716376,-21.9541630066506,
0.));
#190678=CARTESIAN_POINT('Ctrl Pts',(11.1716395716376,-21.9541630066506,
12.));
#190679=CARTESIAN_POINT('Ctrl Pts',(11.1529923792003,-21.9388554416439,
0.));
#190680=CARTESIAN_POINT('Ctrl Pts',(11.1529923792003,-21.9388554416439,
12.));
#190681=CARTESIAN_POINT('Ctrl Pts',(11.1344491774741,-21.923557224952,0.));
#190682=CARTESIAN_POINT('Ctrl Pts',(11.1344491774741,-21.923557224952,12.));
#190683=CARTESIAN_POINT('Ctrl Pts',(11.1160102123024,-21.9082689538688,
0.));
#190684=CARTESIAN_POINT('Ctrl Pts',(11.1160102123024,-21.9082689538688,
12.));
#190685=CARTESIAN_POINT('Ctrl Pts',(11.0976757303944,-21.8929912313608,
0.));
#190686=CARTESIAN_POINT('Ctrl Pts',(11.0976757303944,-21.8929912313608,
12.));
#190687=CARTESIAN_POINT('Ctrl Pts',(11.0794459793057,-21.877724666119,0.));
#190688=CARTESIAN_POINT('Ctrl Pts',(11.0794459793057,-21.877724666119,12.));
#190689=CARTESIAN_POINT('Ctrl Pts',(11.0613212074363,-21.8624698726318,
0.));
#190690=CARTESIAN_POINT('Ctrl Pts',(11.0613212074363,-21.8624698726318,
12.));
#190691=CARTESIAN_POINT('Ctrl Pts',(11.0433016640807,-21.8472274713103,
0.));
#190692=CARTESIAN_POINT('Ctrl Pts',(11.0433016640807,-21.8472274713103,
12.));
#190693=CARTESIAN_POINT('Ctrl Pts',(11.0253875994598,-21.8319980886033,
0.));
#190694=CARTESIAN_POINT('Ctrl Pts',(11.0253875994598,-21.8319980886033,
12.));
#190695=CARTESIAN_POINT('Ctrl Pts',(11.0075792647477,-21.8167823571168,
0.));
#190696=CARTESIAN_POINT('Ctrl Pts',(11.0075792647477,-21.8167823571168,
12.));
#190697=CARTESIAN_POINT('Ctrl Pts',(10.9898769120912,-21.8015809157301,
0.));
#190698=CARTESIAN_POINT('Ctrl Pts',(10.9898769120912,-21.8015809157301,
12.));
#190699=CARTESIAN_POINT('Ctrl Pts',(10.9722807946155,-21.7863944097141,
0.));
#190700=CARTESIAN_POINT('Ctrl Pts',(10.9722807946155,-21.7863944097141,
12.));
#190701=CARTESIAN_POINT('Ctrl Pts',(10.9547911664455,-21.7712234908464,
0.));
#190702=CARTESIAN_POINT('Ctrl Pts',(10.9547911664455,-21.7712234908464,
12.));
#190703=CARTESIAN_POINT('Ctrl Pts',(10.9374082827444,-21.7560688175247,
0.));
#190704=CARTESIAN_POINT('Ctrl Pts',(10.9374082827444,-21.7560688175247,
12.));
#190705=CARTESIAN_POINT('Ctrl Pts',(10.9201323997384,-21.7409310548797,
0.));
#190706=CARTESIAN_POINT('Ctrl Pts',(10.9201323997384,-21.7409310548797,
12.));
#190707=CARTESIAN_POINT('Ctrl Pts',(10.902963774734,-21.7258108748873,0.));
#190708=CARTESIAN_POINT('Ctrl Pts',(10.902963774734,-21.7258108748873,12.));
#190709=CARTESIAN_POINT('Ctrl Pts',(10.8859026661293,-21.7107089564825,
0.));
#190710=CARTESIAN_POINT('Ctrl Pts',(10.8859026661293,-21.7107089564825,
12.));
#190711=CARTESIAN_POINT('Ctrl Pts',(10.8689493334095,-21.6956259856672,
0.));
#190712=CARTESIAN_POINT('Ctrl Pts',(10.8689493334095,-21.6956259856672,
12.));
#190713=CARTESIAN_POINT('Ctrl Pts',(10.8521040371835,-21.6805626556467,
0.));
#190714=CARTESIAN_POINT('Ctrl Pts',(10.8521040371835,-21.6805626556467,
12.));
#190715=CARTESIAN_POINT('Ctrl Pts',(10.8353670392272,-21.6655196669732,
0.));
#190716=CARTESIAN_POINT('Ctrl Pts',(10.8353670392272,-21.6655196669732,
12.));
#190717=CARTESIAN_POINT('Ctrl Pts',(10.8187386025136,-21.6504977276866,
0.));
#190718=CARTESIAN_POINT('Ctrl Pts',(10.8187386025136,-21.6504977276866,
12.));
#190719=CARTESIAN_POINT('Ctrl Pts',(10.8022189912369,-21.6354975534557,
0.));
#190720=CARTESIAN_POINT('Ctrl Pts',(10.8022189912369,-21.6354975534557,
12.));
#190721=CARTESIAN_POINT('Ctrl Pts',(10.7858084708261,-21.6205198677173,
0.));
#190722=CARTESIAN_POINT('Ctrl Pts',(10.7858084708261,-21.6205198677173,
12.));
#190723=CARTESIAN_POINT('Ctrl Pts',(10.7695073079552,-21.6055654018176,
0.));
#190724=CARTESIAN_POINT('Ctrl Pts',(10.7695073079552,-21.6055654018176,
12.));
#190725=CARTESIAN_POINT('Ctrl Pts',(10.7533157705941,-21.5906348951743,
0.));
#190726=CARTESIAN_POINT('Ctrl Pts',(10.7533157705941,-21.5906348951743,
12.));
#190727=CARTESIAN_POINT('Ctrl Pts',(10.7372341280467,-21.5757290954371,
0.));
#190728=CARTESIAN_POINT('Ctrl Pts',(10.7372341280467,-21.5757290954371,
12.));
#190729=CARTESIAN_POINT('Ctrl Pts',(10.7212626509816,-21.5608487586468,
0.));
#190730=CARTESIAN_POINT('Ctrl Pts',(10.7212626509816,-21.5608487586468,
12.));
#190731=CARTESIAN_POINT('Ctrl Pts',(10.7054016114571,-21.5459946493955,
0.));
#190732=CARTESIAN_POINT('Ctrl Pts',(10.7054016114571,-21.5459946493955,
12.));
#190733=CARTESIAN_POINT('Ctrl Pts',(10.689651282929,-21.5311675409807,0.));
#190734=CARTESIAN_POINT('Ctrl Pts',(10.689651282929,-21.5311675409807,12.));
#190735=CARTESIAN_POINT('Ctrl Pts',(10.6740119402834,-21.51636821558,0.));
#190736=CARTESIAN_POINT('Ctrl Pts',(10.6740119402834,-21.51636821558,12.));
#190737=CARTESIAN_POINT('Ctrl Pts',(10.6584838598939,-21.5015974644449,
0.));
#190738=CARTESIAN_POINT('Ctrl Pts',(10.6584838598939,-21.5015974644449,
12.));
#190739=CARTESIAN_POINT('Ctrl Pts',(10.6430673196607,-21.4868560880889,
0.));
#190740=CARTESIAN_POINT('Ctrl Pts',(10.6430673196607,-21.4868560880889,
12.));
#190741=CARTESIAN_POINT('Ctrl Pts',(10.6277625990456,-21.4721448964766,
0.));
#190742=CARTESIAN_POINT('Ctrl Pts',(10.6277625990456,-21.4721448964766,
12.));
#190743=CARTESIAN_POINT('Ctrl Pts',(10.6125699790961,-21.4574647092097,
0.));
#190744=CARTESIAN_POINT('Ctrl Pts',(10.6125699790961,-21.4574647092097,
12.));
#190745=CARTESIAN_POINT('Ctrl Pts',(10.5974897424622,-21.4428163557144,
0.));
#190746=CARTESIAN_POINT('Ctrl Pts',(10.5974897424622,-21.4428163557144,
12.));
#190747=CARTESIAN_POINT('Ctrl Pts',(10.5825221734573,-21.4282006754631,
0.));
#190748=CARTESIAN_POINT('Ctrl Pts',(10.5825221734573,-21.4282006754631,
12.));
#190749=CARTESIAN_POINT('Ctrl Pts',(10.5676675581108,-21.4136185181979,
0.));
#190750=CARTESIAN_POINT('Ctrl Pts',(10.5676675581108,-21.4136185181979,
12.));
#190751=CARTESIAN_POINT('Ctrl Pts',(10.5529261842108,-21.3990707441497,
0.));
#190752=CARTESIAN_POINT('Ctrl Pts',(10.5529261842108,-21.3990707441497,
12.));
#190753=CARTESIAN_POINT('Ctrl Pts',(10.5382983413421,-21.3845582242602,
0.));
#190754=CARTESIAN_POINT('Ctrl Pts',(10.5382983413421,-21.3845582242602,
12.));
#190755=CARTESIAN_POINT('Ctrl Pts',(10.5237843209057,-21.3700818403936,
0.));
#190756=CARTESIAN_POINT('Ctrl Pts',(10.5237843209057,-21.3700818403936,
12.));
#190757=CARTESIAN_POINT('Ctrl Pts',(10.5093844161685,-21.3556424855814,
0.));
#190758=CARTESIAN_POINT('Ctrl Pts',(10.5093844161685,-21.3556424855814,
12.));
#190759=CARTESIAN_POINT('Ctrl Pts',(10.4950989223336,-21.3412410642904,
0.));
#190760=CARTESIAN_POINT('Ctrl Pts',(10.4950989223336,-21.3412410642904,
12.));
#190761=CARTESIAN_POINT('Ctrl Pts',(10.4809281365931,-21.3268784926819,
0.));
#190762=CARTESIAN_POINT('Ctrl Pts',(10.4809281365931,-21.3268784926819,
12.));
#190763=CARTESIAN_POINT('Ctrl Pts',(10.4668723581768,-21.3125556988731,
0.));
#190764=CARTESIAN_POINT('Ctrl Pts',(10.4668723581768,-21.3125556988731,
12.));
#190765=CARTESIAN_POINT('Ctrl Pts',(10.4529318883874,-21.2982736231931,
0.));
#190766=CARTESIAN_POINT('Ctrl Pts',(10.4529318883874,-21.2982736231931,
12.));
#190767=CARTESIAN_POINT('Ctrl Pts',(10.4391070306391,-21.2840332184483,
0.));
#190768=CARTESIAN_POINT('Ctrl Pts',(10.4391070306391,-21.2840332184483,
12.));
#190769=CARTESIAN_POINT('Ctrl Pts',(10.42539809054,-21.2698354502403,0.));
#190770=CARTESIAN_POINT('Ctrl Pts',(10.42539809054,-21.2698354502403,12.));
#190771=CARTESIAN_POINT('Ctrl Pts',(10.4118053759588,-21.255681297275,0.));
#190772=CARTESIAN_POINT('Ctrl Pts',(10.4118053759588,-21.255681297275,12.));
#190773=CARTESIAN_POINT('Ctrl Pts',(10.3983291970846,-21.2415717516714,
0.));
#190774=CARTESIAN_POINT('Ctrl Pts',(10.3983291970846,-21.2415717516714,
12.));
#190775=CARTESIAN_POINT('Ctrl Pts',(10.3849698664786,-21.22750781927,0.));
#190776=CARTESIAN_POINT('Ctrl Pts',(10.3849698664786,-21.22750781927,12.));
#190777=CARTESIAN_POINT('Ctrl Pts',(10.371727699113,-21.2134905199345,0.));
#190778=CARTESIAN_POINT('Ctrl Pts',(10.371727699113,-21.2134905199345,12.));
#190779=CARTESIAN_POINT('Ctrl Pts',(10.3586030124587,-21.199520887919,0.));
#190780=CARTESIAN_POINT('Ctrl Pts',(10.3586030124587,-21.199520887919,12.));
#190781=CARTESIAN_POINT('Ctrl Pts',(10.34559612657,-21.1855999722416,0.));
#190782=CARTESIAN_POINT('Ctrl Pts',(10.34559612657,-21.1855999722416,12.));
#190783=CARTESIAN_POINT('Ctrl Pts',(10.3327073641572,-21.1717288370509,
0.));
#190784=CARTESIAN_POINT('Ctrl Pts',(10.3327073641572,-21.1717288370509,
12.));
#190785=CARTESIAN_POINT('Ctrl Pts',(10.3199370506544,-21.1579085619965,
0.));
#190786=CARTESIAN_POINT('Ctrl Pts',(10.3199370506544,-21.1579085619965,
12.));
#190787=CARTESIAN_POINT('Ctrl Pts',(10.3072855142687,-21.1441402425843,
0.));
#190788=CARTESIAN_POINT('Ctrl Pts',(10.3072855142687,-21.1441402425843,
12.));
#190789=CARTESIAN_POINT('Ctrl Pts',(10.2947530860721,-21.1304249906002,
0.));
#190790=CARTESIAN_POINT('Ctrl Pts',(10.2947530860721,-21.1304249906002,
12.));
#190791=CARTESIAN_POINT('Ctrl Pts',(10.2823401001072,-21.1167639345631,
0.));
#190792=CARTESIAN_POINT('Ctrl Pts',(10.2823401001072,-21.1167639345631,
12.));
#190793=CARTESIAN_POINT('Ctrl Pts',(10.2700468934744,-21.1031582201627,
0.));
#190794=CARTESIAN_POINT('Ctrl Pts',(10.2700468934744,-21.1031582201627,
12.));
#190795=CARTESIAN_POINT('Ctrl Pts',(10.2578738064181,-21.0896090107063,
0.));
#190796=CARTESIAN_POINT('Ctrl Pts',(10.2578738064181,-21.0896090107063,
12.));
#190797=CARTESIAN_POINT('Ctrl Pts',(10.2458211823912,-21.0761174875445,
0.));
#190798=CARTESIAN_POINT('Ctrl Pts',(10.2458211823912,-21.0761174875445,
12.));
#190799=CARTESIAN_POINT('Ctrl Pts',(10.2338893681567,-21.0626848505663,
0.));
#190800=CARTESIAN_POINT('Ctrl Pts',(10.2338893681567,-21.0626848505663,
12.));
#190801=CARTESIAN_POINT('Ctrl Pts',(10.2220787139154,-21.0493123187483,
0.));
#190802=CARTESIAN_POINT('Ctrl Pts',(10.2220787139154,-21.0493123187483,
12.));
#190803=CARTESIAN_POINT('Ctrl Pts',(10.2103895734123,-21.0360011306815,
0.));
#190804=CARTESIAN_POINT('Ctrl Pts',(10.2103895734123,-21.0360011306815,
12.));
#190805=CARTESIAN_POINT('Ctrl Pts',(10.1988223040425,-21.0227525451107,
0.));
#190806=CARTESIAN_POINT('Ctrl Pts',(10.1988223040425,-21.0227525451107,
12.));
#190807=CARTESIAN_POINT('Ctrl Pts',(10.187377266936,-21.0095678414486,0.));
#190808=CARTESIAN_POINT('Ctrl Pts',(10.187377266936,-21.0095678414486,12.));
#190809=CARTESIAN_POINT('Ctrl Pts',(10.1760548270767,-20.9964483203686,
0.));
#190810=CARTESIAN_POINT('Ctrl Pts',(10.1760548270767,-20.9964483203686,
12.));
#190811=CARTESIAN_POINT('Ctrl Pts',(10.1648553534568,-20.9833953044736,
0.));
#190812=CARTESIAN_POINT('Ctrl Pts',(10.1648553534568,-20.9833953044736,
12.));
#190813=CARTESIAN_POINT('Ctrl Pts',(10.1537792192065,-20.9704101389369,
0.));
#190814=CARTESIAN_POINT('Ctrl Pts',(10.1537792192065,-20.9704101389369,
12.));
#190815=CARTESIAN_POINT('Ctrl Pts',(10.1428268017256,-20.9574941921591,
0.));
#190816=CARTESIAN_POINT('Ctrl Pts',(10.1428268017256,-20.9574941921591,
12.));
#190817=CARTESIAN_POINT('Ctrl Pts',(10.1319984827908,-20.9446488563933,
0.));
#190818=CARTESIAN_POINT('Ctrl Pts',(10.1319984827908,-20.9446488563933,
12.));
#190819=CARTESIAN_POINT('Ctrl Pts',(10.1212946487057,-20.9318755484734,
0.));
#190820=CARTESIAN_POINT('Ctrl Pts',(10.1212946487057,-20.9318755484734,
12.));
#190821=CARTESIAN_POINT('Ctrl Pts',(10.1107156904836,-20.919175710627,0.));
#190822=CARTESIAN_POINT('Ctrl Pts',(10.1107156904836,-20.919175710627,12.));
#190823=CARTESIAN_POINT('Ctrl Pts',(10.1002620040076,-20.9065508112557,
0.));
#190824=CARTESIAN_POINT('Ctrl Pts',(10.1002620040076,-20.9065508112557,
12.));
#190825=CARTESIAN_POINT('Ctrl Pts',(10.0899339901915,-20.894002345737,0.));
#190826=CARTESIAN_POINT('Ctrl Pts',(10.0899339901915,-20.894002345737,12.));
#190827=CARTESIAN_POINT('Ctrl Pts',(10.0797320551154,-20.881531837184,0.));
#190828=CARTESIAN_POINT('Ctrl Pts',(10.0797320551154,-20.881531837184,12.));
#190829=CARTESIAN_POINT('Ctrl Pts',(10.0696566102218,-20.86914083737,0.));
#190830=CARTESIAN_POINT('Ctrl Pts',(10.0696566102218,-20.86914083737,12.));
#190831=CARTESIAN_POINT('Ctrl Pts',(10.0597080725375,-20.8568309277316,
0.));
#190832=CARTESIAN_POINT('Ctrl Pts',(10.0597080725375,-20.8568309277316,
12.));
#190833=CARTESIAN_POINT('Ctrl Pts',(10.0498868648733,-20.8446037203402,
0.));
#190834=CARTESIAN_POINT('Ctrl Pts',(10.0498868648733,-20.8446037203402,
12.));
#190835=CARTESIAN_POINT('Ctrl Pts',(10.0401934160234,-20.8324608588909,
0.));
#190836=CARTESIAN_POINT('Ctrl Pts',(10.0401934160234,-20.8324608588909,
12.));
#190837=CARTESIAN_POINT('Ctrl Pts',(10.0306281609435,-20.8204040196602,
0.));
#190838=CARTESIAN_POINT('Ctrl Pts',(10.0306281609435,-20.8204040196602,
12.));
#190839=CARTESIAN_POINT('Ctrl Pts',(10.0211915410095,-20.8084349126888,
0.));
#190840=CARTESIAN_POINT('Ctrl Pts',(10.0211915410095,-20.8084349126888,
12.));
#190841=CARTESIAN_POINT('Ctrl Pts',(10.0118840042786,-20.7965552829908,
0.));
#190842=CARTESIAN_POINT('Ctrl Pts',(10.0118840042786,-20.7965552829908,
12.));
#190843=CARTESIAN_POINT('Ctrl Pts',(10.0027060057389,-20.7847669117568,
0.));
#190844=CARTESIAN_POINT('Ctrl Pts',(10.0027060057389,-20.7847669117568,
12.));
#190845=CARTESIAN_POINT('Ctrl Pts',(9.9936580075464,-20.7730716175417,0.));
#190846=CARTESIAN_POINT('Ctrl Pts',(9.9936580075464,-20.7730716175417,12.));
#190847=CARTESIAN_POINT('Ctrl Pts',(9.98474047926852,-20.761471257499,0.));
#190848=CARTESIAN_POINT('Ctrl Pts',(9.98474047926852,-20.761471257499,12.));
#190849=CARTESIAN_POINT('Ctrl Pts',(9.97595389823469,-20.7499677289627,
0.));
#190850=CARTESIAN_POINT('Ctrl Pts',(9.97595389823469,-20.7499677289627,
12.));
#190851=CARTESIAN_POINT('Ctrl Pts',(9.96729874986201,-20.7385629709795,
0.));
#190852=CARTESIAN_POINT('Ctrl Pts',(9.96729874986201,-20.7385629709795,
12.));
#190853=CARTESIAN_POINT('Ctrl Pts',(9.95877552798397,-20.7272589658751,
0.));
#190854=CARTESIAN_POINT('Ctrl Pts',(9.95877552798397,-20.7272589658751,
12.));
#190855=CARTESIAN_POINT('Ctrl Pts',(9.95038473514948,-20.7160577407579,
0.));
#190856=CARTESIAN_POINT('Ctrl Pts',(9.95038473514948,-20.7160577407579,
12.));
#190857=CARTESIAN_POINT('Ctrl Pts',(9.94212688298236,-20.7049613692234,
0.));
#190858=CARTESIAN_POINT('Ctrl Pts',(9.94212688298236,-20.7049613692234,
12.));
#190859=CARTESIAN_POINT('Ctrl Pts',(9.93400249259729,-20.6939719732484,
0.));
#190860=CARTESIAN_POINT('Ctrl Pts',(9.93400249259729,-20.6939719732484,
12.));
#190861=CARTESIAN_POINT('Ctrl Pts',(9.92601209498748,-20.6830917250255,
0.));
#190862=CARTESIAN_POINT('Ctrl Pts',(9.92601209498748,-20.6830917250255,
12.));
#190863=CARTESIAN_POINT('Ctrl Pts',(9.91815623141288,-20.6723228488263,
0.));
#190864=CARTESIAN_POINT('Ctrl Pts',(9.91815623141288,-20.6723228488263,
12.));
#190865=CARTESIAN_POINT('Ctrl Pts',(9.91043545377007,-20.6616676228315,
0.));
#190866=CARTESIAN_POINT('Ctrl Pts',(9.91043545377007,-20.6616676228315,
12.));
#190867=CARTESIAN_POINT('Ctrl Pts',(9.90285032516692,-20.6511283817414,
0.));
#190868=CARTESIAN_POINT('Ctrl Pts',(9.90285032516692,-20.6511283817414,
12.));
#190869=CARTESIAN_POINT('Ctrl Pts',(9.89540142049119,-20.6407075193976,
0.));
#190870=CARTESIAN_POINT('Ctrl Pts',(9.89540142049119,-20.6407075193976,
12.));
#190871=CARTESIAN_POINT('Ctrl Pts',(9.88808932697305,-20.6304074914087,
0.));
#190872=CARTESIAN_POINT('Ctrl Pts',(9.88808932697305,-20.6304074914087,
12.));
#190873=CARTESIAN_POINT('Ctrl Pts',(9.88091464472675,-20.6202308177475,
0.));
#190874=CARTESIAN_POINT('Ctrl Pts',(9.88091464472675,-20.6202308177475,
12.));
#190875=CARTESIAN_POINT('Ctrl Pts',(9.87387798732955,-20.6101800854494,
0.));
#190876=CARTESIAN_POINT('Ctrl Pts',(9.87387798732955,-20.6101800854494,
12.));
#190877=CARTESIAN_POINT('Ctrl Pts',(9.86697998242622,-20.6002579513699,
0.));
#190878=CARTESIAN_POINT('Ctrl Pts',(9.86697998242622,-20.6002579513699,
12.));
#190879=CARTESIAN_POINT('Ctrl Pts',(9.86022127232747,-20.5904671449754,
0.));
#190880=CARTESIAN_POINT('Ctrl Pts',(9.86022127232747,-20.5904671449754,
12.));
#190881=CARTESIAN_POINT('Ctrl Pts',(9.8536025145698,-20.5808104710015,0.));
#190882=CARTESIAN_POINT('Ctrl Pts',(9.8536025145698,-20.5808104710015,12.));
#190883=CARTESIAN_POINT('Ctrl Pts',(9.84712438256277,-20.5712908125139,
0.));
#190884=CARTESIAN_POINT('Ctrl Pts',(9.84712438256277,-20.5712908125139,
12.));
#190885=CARTESIAN_POINT('Ctrl Pts',(9.84078756677565,-20.5619111362402,
0.));
#190886=CARTESIAN_POINT('Ctrl Pts',(9.84078756677565,-20.5619111362402,
12.));
#190887=CARTESIAN_POINT('Ctrl Pts',(9.83459277585315,-20.552674497646,0.));
#190888=CARTESIAN_POINT('Ctrl Pts',(9.83459277585315,-20.552674497646,12.));
#190889=CARTESIAN_POINT('Ctrl Pts',(9.82854073773876,-20.5435840460721,
0.));
#190890=CARTESIAN_POINT('Ctrl Pts',(9.82854073773876,-20.5435840460721,
12.));
#190891=CARTESIAN_POINT('Ctrl Pts',(9.82263220080362,-20.5346430299517,
0.));
#190892=CARTESIAN_POINT('Ctrl Pts',(9.82263220080362,-20.5346430299517,
12.));
#190893=CARTESIAN_POINT('Ctrl Pts',(9.81686793455942,-20.5258548000629,
0.));
#190894=CARTESIAN_POINT('Ctrl Pts',(9.81686793455942,-20.5258548000629,
12.));
#190895=CARTESIAN_POINT('Ctrl Pts',(9.81124873025281,-20.517222812284,0.));
#190896=CARTESIAN_POINT('Ctrl Pts',(9.81124873025281,-20.517222812284,12.));
#190897=CARTESIAN_POINT('Ctrl Pts',(9.80577540161087,-20.5087506310505,
0.));
#190898=CARTESIAN_POINT('Ctrl Pts',(9.80577540161087,-20.5087506310505,
12.));
#190899=CARTESIAN_POINT('Ctrl Pts',(9.80044878520948,-20.5004419312107,
0.));
#190900=CARTESIAN_POINT('Ctrl Pts',(9.80044878520948,-20.5004419312107,
12.));
#190901=CARTESIAN_POINT('Ctrl Pts',(9.7952697428833,-20.4923005087943,0.));
#190902=CARTESIAN_POINT('Ctrl Pts',(9.7952697428833,-20.4923005087943,12.));
#190903=CARTESIAN_POINT('Ctrl Pts',(9.79023916498655,-20.4843302955329,
0.));
#190904=CARTESIAN_POINT('Ctrl Pts',(9.79023916498655,-20.4843302955329,
12.));
#190905=CARTESIAN_POINT('Ctrl Pts',(9.78535797314166,-20.4765353711586,
0.));
#190906=CARTESIAN_POINT('Ctrl Pts',(9.78535797314166,-20.4765353711586,
12.));
#190907=CARTESIAN_POINT('Ctrl Pts',(9.7806271237332,-20.4689199790669,0.));
#190908=CARTESIAN_POINT('Ctrl Pts',(9.7806271237332,-20.4689199790669,12.));
#190909=CARTESIAN_POINT('Ctrl Pts',(9.77604760815528,-20.4614885274975,
0.));
#190910=CARTESIAN_POINT('Ctrl Pts',(9.77604760815528,-20.4614885274975,
12.));
#190911=CARTESIAN_POINT('Ctrl Pts',(9.77162045104069,-20.4542455817527,
0.));
#190912=CARTESIAN_POINT('Ctrl Pts',(9.77162045104069,-20.4542455817527,
12.));
#190913=CARTESIAN_POINT('Ctrl Pts',(9.76734670980891,-20.447195862298,0.));
#190914=CARTESIAN_POINT('Ctrl Pts',(9.76734670980891,-20.447195862298,12.));
#190915=CARTESIAN_POINT('Ctrl Pts',(9.76322747195494,-20.44034423294,0.));
#190916=CARTESIAN_POINT('Ctrl Pts',(9.76322747195494,-20.44034423294,12.));
#190917=CARTESIAN_POINT('Ctrl Pts',(9.75926386289922,-20.4336957355473,
0.));
#190918=CARTESIAN_POINT('Ctrl Pts',(9.75926386289922,-20.4336957355473,
12.));
#190919=CARTESIAN_POINT('Ctrl Pts',(9.75545705902417,-20.4272556476629,
0.));
#190920=CARTESIAN_POINT('Ctrl Pts',(9.75545705902417,-20.4272556476629,
12.));
#190921=CARTESIAN_POINT('Ctrl Pts',(9.75180829786429,-20.4210295275817,
0.));
#190922=CARTESIAN_POINT('Ctrl Pts',(9.75180829786429,-20.4210295275817,
12.));
#190923=CARTESIAN_POINT('Ctrl Pts',(9.74831889242173,-20.4150232777393,
0.));
#190924=CARTESIAN_POINT('Ctrl Pts',(9.74831889242173,-20.4150232777393,
12.));
#190925=CARTESIAN_POINT('Ctrl Pts',(9.74499021838537,-20.4092430879861,
0.));
#190926=CARTESIAN_POINT('Ctrl Pts',(9.74499021838537,-20.4092430879861,
12.));
#190927=CARTESIAN_POINT('Ctrl Pts',(9.74182369656271,-20.4036953576549,
0.));
#190928=CARTESIAN_POINT('Ctrl Pts',(9.74182369656271,-20.4036953576549,
12.));
#190929=CARTESIAN_POINT('Ctrl Pts',(9.738820776132,-20.3983866213331,0.));
#190930=CARTESIAN_POINT('Ctrl Pts',(9.738820776132,-20.3983866213331,12.));
#190931=CARTESIAN_POINT('Ctrl Pts',(9.73598292014242,-20.3933234845647,
0.));
#190932=CARTESIAN_POINT('Ctrl Pts',(9.73598292014242,-20.3933234845647,
12.));
#190933=CARTESIAN_POINT('Ctrl Pts',(9.73331167102807,-20.3885129129912,
0.));
#190934=CARTESIAN_POINT('Ctrl Pts',(9.73331167102807,-20.3885129129912,
12.));
#190935=CARTESIAN_POINT('Ctrl Pts',(9.73080870123726,-20.3839624556742,
0.));
#190936=CARTESIAN_POINT('Ctrl Pts',(9.73080870123726,-20.3839624556742,
12.));
#190937=CARTESIAN_POINT('Ctrl Pts',(9.72847589116541,-20.3796805893304,
0.));
#190938=CARTESIAN_POINT('Ctrl Pts',(9.72847589116541,-20.3796805893304,
12.));
#190939=CARTESIAN_POINT('Ctrl Pts',(9.7263153173288,-20.3756766651951,0.));
#190940=CARTESIAN_POINT('Ctrl Pts',(9.7263153173288,-20.3756766651951,12.));
#190941=CARTESIAN_POINT('Ctrl Pts',(9.72432910043194,-20.371960235676,0.));
#190942=CARTESIAN_POINT('Ctrl Pts',(9.72432910043194,-20.371960235676,12.));
#190943=CARTESIAN_POINT('Ctrl Pts',(9.72251930722489,-20.3685406190576,
0.));
#190944=CARTESIAN_POINT('Ctrl Pts',(9.72251930722489,-20.3685406190576,
12.));
#190945=CARTESIAN_POINT('Ctrl Pts',(9.7208877838108,-20.3654261611056,0.));
#190946=CARTESIAN_POINT('Ctrl Pts',(9.7208877838108,-20.3654261611056,12.));
#190947=CARTESIAN_POINT('Ctrl Pts',(9.71943648548099,-20.3626256913981,
0.));
#190948=CARTESIAN_POINT('Ctrl Pts',(9.71943648548099,-20.3626256913981,
12.));
#190949=CARTESIAN_POINT('Ctrl Pts',(9.71816778328006,-20.3601498764344,
0.));
#190950=CARTESIAN_POINT('Ctrl Pts',(9.71816778328006,-20.3601498764344,
12.));
#190951=CARTESIAN_POINT('Ctrl Pts',(9.71708493723096,-20.3580133103356,
0.));
#190952=CARTESIAN_POINT('Ctrl Pts',(9.71708493723096,-20.3580133103356,
12.));
#190953=CARTESIAN_POINT('Ctrl Pts',(9.71619192554185,-20.3562337557875,
0.));
#190954=CARTESIAN_POINT('Ctrl Pts',(9.71619192554185,-20.3562337557875,
12.));
#190955=CARTESIAN_POINT('Ctrl Pts',(9.71549257088172,-20.3548282742361,
0.));
#190956=CARTESIAN_POINT('Ctrl Pts',(9.71549257088172,-20.3548282742361,
12.));
#190957=CARTESIAN_POINT('Ctrl Pts',(9.7149897805202,-20.3538098605706,0.));
#190958=CARTESIAN_POINT('Ctrl Pts',(9.7149897805202,-20.3538098605706,12.));
#190959=CARTESIAN_POINT('Ctrl Pts',(9.7147459035068,-20.3533097561886,0.));
#190960=CARTESIAN_POINT('Ctrl Pts',(9.7147459035068,-20.3533097561886,12.));
#190961=CARTESIAN_POINT('Ctrl Pts',(9.71465227853041,-20.3531126095522,
0.));
#190962=CARTESIAN_POINT('Ctrl Pts',(9.71465227853041,-20.3531126095522,
12.));
#190963=CARTESIAN_POINT('Ctrl Pts',(9.71462954053041,-20.353060251684,0.));
#190964=CARTESIAN_POINT('Ctrl Pts',(9.71462954053041,-20.353060251684,12.));
#190965=CARTESIAN_POINT('Ctrl Pts',(9.71462809124915,-20.353053841303,0.));
#190966=CARTESIAN_POINT('Ctrl Pts',(9.71462809124915,-20.353053841303,12.));
#190967=CARTESIAN_POINT('',(12.4230808101438,-22.8400320311649,0.));
#190968=CARTESIAN_POINT('Ctrl Pts',(12.4230808101438,-22.8400320311649,
0.));
#190969=CARTESIAN_POINT('Ctrl Pts',(12.418215285186,-22.8370364396459,0.));
#190970=CARTESIAN_POINT('Ctrl Pts',(12.4084933766346,-22.8310435872748,
0.));
#190971=CARTESIAN_POINT('Ctrl Pts',(12.3939379378998,-22.8220493007173,
0.));
#190972=CARTESIAN_POINT('Ctrl Pts',(12.374585536673,-22.81004690224,0.));
#190973=CARTESIAN_POINT('Ctrl Pts',(12.3504864740319,-22.795027221673,0.));
#190974=CARTESIAN_POINT('Ctrl Pts',(12.3264788926075,-22.7799908974768,
0.));
#190975=CARTESIAN_POINT('Ctrl Pts',(12.3025628601792,-22.764938010105,0.));
#190976=CARTESIAN_POINT('Ctrl Pts',(12.2787384750742,-22.7498686970069,
0.));
#190977=CARTESIAN_POINT('Ctrl Pts',(12.2550058702395,-22.7347831655287,
0.));
#190978=CARTESIAN_POINT('Ctrl Pts',(12.2313652198061,-22.7196817119374,
0.));
#190979=CARTESIAN_POINT('Ctrl Pts',(12.2078167360284,-22.7045647168747,
0.));
#190980=CARTESIAN_POINT('Ctrl Pts',(12.1843606579261,-22.6894326205037,
0.));
#190981=CARTESIAN_POINT('Ctrl Pts',(12.1609972423099,-22.6742859034944,
0.));
#190982=CARTESIAN_POINT('Ctrl Pts',(12.1377267537145,-22.6591250653965,
0.));
#190983=CARTESIAN_POINT('Ctrl Pts',(12.1145494550383,-22.6439506046605,
0.));
#190984=CARTESIAN_POINT('Ctrl Pts',(12.0914655972823,-22.6287629967056,
0.));
#190985=CARTESIAN_POINT('Ctrl Pts',(12.0684754113862,-22.6135626764898,
0.));
#190986=CARTESIAN_POINT('Ctrl Pts',(12.0455791139128,-22.5983500505644,
0.));
#190987=CARTESIAN_POINT('Ctrl Pts',(12.0227769113127,-22.5831255061282,
0.));
#190988=CARTESIAN_POINT('Ctrl Pts',(12.0000690046694,-22.5678894211181,
0.));
#190989=CARTESIAN_POINT('Ctrl Pts',(11.9774555943496,-22.5526421741158,
0.));
#190990=CARTESIAN_POINT('Ctrl Pts',(11.9549368843997,-22.5373841537307,
0.));
#190991=CARTESIAN_POINT('Ctrl Pts',(11.9325130877803,-22.5221157697883,
0.));
#190992=CARTESIAN_POINT('Ctrl Pts',(11.9101844254557,-22.5068374513973,
0.));
#190993=CARTESIAN_POINT('Ctrl Pts',(11.8879511239942,-22.4915496418485,
0.));
#190994=CARTESIAN_POINT('Ctrl Pts',(11.8658134137019,-22.4762527946702,
0.));
#190995=CARTESIAN_POINT('Ctrl Pts',(11.8437715264487,-22.4609473690472,
0.));
#190996=CARTESIAN_POINT('Ctrl Pts',(11.8218256937889,-22.4456338258735,
0.));
#190997=CARTESIAN_POINT('Ctrl Pts',(11.7999761445173,-22.430312622646,0.));
#190998=CARTESIAN_POINT('Ctrl Pts',(11.7782231042039,-22.4149842125008,
0.));
#190999=CARTESIAN_POINT('Ctrl Pts',(11.7565667964764,-22.3996490469191,
0.));
#191000=CARTESIAN_POINT('Ctrl Pts',(11.7350074437961,-22.3843075773899,
0.));
#191001=CARTESIAN_POINT('Ctrl Pts',(11.7135452684532,-22.3689602575491,
0.));
#191002=CARTESIAN_POINT('Ctrl Pts',(11.6921804934056,-22.3536075450029,
0.));
#191003=CARTESIAN_POINT('Ctrl Pts',(11.6709133432985,-22.3382499035619,
0.));
#191004=CARTESIAN_POINT('Ctrl Pts',(11.6497440449857,-22.3228878043976,
0.));
#191005=CARTESIAN_POINT('Ctrl Pts',(11.6286728270009,-22.3075217249049,
0.));
#191006=CARTESIAN_POINT('Ctrl Pts',(11.6076999192357,-22.2921521480356,
0.));
#191007=CARTESIAN_POINT('Ctrl Pts',(11.5868255525188,-22.2767795614348,
0.));
#191008=CARTESIAN_POINT('Ctrl Pts',(11.5660499582403,-22.2614044566898,
0.));
#191009=CARTESIAN_POINT('Ctrl Pts',(11.5453733679121,-22.2460273284654,
0.));
#191010=CARTESIAN_POINT('Ctrl Pts',(11.5247960128477,-22.2306486738901,
0.));
#191011=CARTESIAN_POINT('Ctrl Pts',(11.5043181244242,-22.2152689931022,
0.));
#191012=CARTESIAN_POINT('Ctrl Pts',(11.483939934259,-22.1998887896436,0.));
#191013=CARTESIAN_POINT('Ctrl Pts',(11.463661674411,-22.184508570917,0.));
#191014=CARTESIAN_POINT('Ctrl Pts',(11.443483577557,-22.1691288486096,0.));
#191015=CARTESIAN_POINT('Ctrl Pts',(11.4234058771742,-22.1537501391487,
0.));
#191016=CARTESIAN_POINT('Ctrl Pts',(11.4034288076908,-22.1383729640964,
0.));
#191017=CARTESIAN_POINT('Ctrl Pts',(11.3835526044256,-22.1229978500186,
0.));
#191018=CARTESIAN_POINT('Ctrl Pts',(11.3637775035367,-22.1076253283979,
0.));
#191019=CARTESIAN_POINT('Ctrl Pts',(11.3441037419553,-22.0922559355294,
0.));
#191020=CARTESIAN_POINT('Ctrl Pts',(11.3245315573168,-22.0768902124267,
0.));
#191021=CARTESIAN_POINT('Ctrl Pts',(11.3050611878771,-22.0615287047179,
0.));
#191022=CARTESIAN_POINT('Ctrl Pts',(11.2856928724374,-22.046171962566,0.));
#191023=CARTESIAN_POINT('Ctrl Pts',(11.2664268504206,-22.030820540835,0.));
#191024=CARTESIAN_POINT('Ctrl Pts',(11.2472633619275,-22.0154749992363,
0.));
#191025=CARTESIAN_POINT('Ctrl Pts',(11.2282026477896,-22.0001359024839,
0.));
#191026=CARTESIAN_POINT('Ctrl Pts',(11.2092449496125,-21.9848038204439,
0.));
#191027=CARTESIAN_POINT('Ctrl Pts',(11.190390509811,-21.9694793282914,0.));
#191028=CARTESIAN_POINT('Ctrl Pts',(11.1716395716376,-21.9541630066506,
0.));
#191029=CARTESIAN_POINT('Ctrl Pts',(11.1529923792003,-21.9388554416439,
0.));
#191030=CARTESIAN_POINT('Ctrl Pts',(11.1344491774741,-21.923557224952,0.));
#191031=CARTESIAN_POINT('Ctrl Pts',(11.1160102123024,-21.9082689538688,
0.));
#191032=CARTESIAN_POINT('Ctrl Pts',(11.0976757303944,-21.8929912313608,
0.));
#191033=CARTESIAN_POINT('Ctrl Pts',(11.0794459793057,-21.877724666119,0.));
#191034=CARTESIAN_POINT('Ctrl Pts',(11.0613212074363,-21.8624698726318,
0.));
#191035=CARTESIAN_POINT('Ctrl Pts',(11.0433016640807,-21.8472274713103,
0.));
#191036=CARTESIAN_POINT('Ctrl Pts',(11.0253875994598,-21.8319980886033,
0.));
#191037=CARTESIAN_POINT('Ctrl Pts',(11.0075792647477,-21.8167823571168,
0.));
#191038=CARTESIAN_POINT('Ctrl Pts',(10.9898769120912,-21.8015809157301,
0.));
#191039=CARTESIAN_POINT('Ctrl Pts',(10.9722807946155,-21.7863944097141,
0.));
#191040=CARTESIAN_POINT('Ctrl Pts',(10.9547911664455,-21.7712234908464,
0.));
#191041=CARTESIAN_POINT('Ctrl Pts',(10.9374082827444,-21.7560688175247,
0.));
#191042=CARTESIAN_POINT('Ctrl Pts',(10.9201323997384,-21.7409310548797,
0.));
#191043=CARTESIAN_POINT('Ctrl Pts',(10.902963774734,-21.7258108748873,0.));
#191044=CARTESIAN_POINT('Ctrl Pts',(10.8859026661293,-21.7107089564825,
0.));
#191045=CARTESIAN_POINT('Ctrl Pts',(10.8689493334095,-21.6956259856672,
0.));
#191046=CARTESIAN_POINT('Ctrl Pts',(10.8521040371835,-21.6805626556467,
0.));
#191047=CARTESIAN_POINT('Ctrl Pts',(10.8353670392272,-21.6655196669732,
0.));
#191048=CARTESIAN_POINT('Ctrl Pts',(10.8187386025136,-21.6504977276866,
0.));
#191049=CARTESIAN_POINT('Ctrl Pts',(10.8022189912369,-21.6354975534557,
0.));
#191050=CARTESIAN_POINT('Ctrl Pts',(10.7858084708261,-21.6205198677173,
0.));
#191051=CARTESIAN_POINT('Ctrl Pts',(10.7695073079552,-21.6055654018176,
0.));
#191052=CARTESIAN_POINT('Ctrl Pts',(10.7533157705941,-21.5906348951743,
0.));
#191053=CARTESIAN_POINT('Ctrl Pts',(10.7372341280467,-21.5757290954371,
0.));
#191054=CARTESIAN_POINT('Ctrl Pts',(10.7212626509816,-21.5608487586468,
0.));
#191055=CARTESIAN_POINT('Ctrl Pts',(10.7054016114571,-21.5459946493955,
0.));
#191056=CARTESIAN_POINT('Ctrl Pts',(10.689651282929,-21.5311675409807,0.));
#191057=CARTESIAN_POINT('Ctrl Pts',(10.6740119402834,-21.51636821558,0.));
#191058=CARTESIAN_POINT('Ctrl Pts',(10.6584838598939,-21.5015974644449,
0.));
#191059=CARTESIAN_POINT('Ctrl Pts',(10.6430673196607,-21.4868560880889,
0.));
#191060=CARTESIAN_POINT('Ctrl Pts',(10.6277625990456,-21.4721448964766,
0.));
#191061=CARTESIAN_POINT('Ctrl Pts',(10.6125699790961,-21.4574647092097,
0.));
#191062=CARTESIAN_POINT('Ctrl Pts',(10.5974897424622,-21.4428163557144,
0.));
#191063=CARTESIAN_POINT('Ctrl Pts',(10.5825221734573,-21.4282006754631,
0.));
#191064=CARTESIAN_POINT('Ctrl Pts',(10.5676675581108,-21.4136185181979,
0.));
#191065=CARTESIAN_POINT('Ctrl Pts',(10.5529261842108,-21.3990707441497,
0.));
#191066=CARTESIAN_POINT('Ctrl Pts',(10.5382983413421,-21.3845582242602,
0.));
#191067=CARTESIAN_POINT('Ctrl Pts',(10.5237843209057,-21.3700818403936,
0.));
#191068=CARTESIAN_POINT('Ctrl Pts',(10.5093844161685,-21.3556424855814,
0.));
#191069=CARTESIAN_POINT('Ctrl Pts',(10.4950989223336,-21.3412410642904,
0.));
#191070=CARTESIAN_POINT('Ctrl Pts',(10.4809281365931,-21.3268784926819,
0.));
#191071=CARTESIAN_POINT('Ctrl Pts',(10.4668723581768,-21.3125556988731,
0.));
#191072=CARTESIAN_POINT('Ctrl Pts',(10.4529318883874,-21.2982736231931,
0.));
#191073=CARTESIAN_POINT('Ctrl Pts',(10.4391070306391,-21.2840332184483,
0.));
#191074=CARTESIAN_POINT('Ctrl Pts',(10.42539809054,-21.2698354502403,0.));
#191075=CARTESIAN_POINT('Ctrl Pts',(10.4118053759588,-21.255681297275,0.));
#191076=CARTESIAN_POINT('Ctrl Pts',(10.3983291970846,-21.2415717516714,
0.));
#191077=CARTESIAN_POINT('Ctrl Pts',(10.3849698664786,-21.22750781927,0.));
#191078=CARTESIAN_POINT('Ctrl Pts',(10.371727699113,-21.2134905199345,0.));
#191079=CARTESIAN_POINT('Ctrl Pts',(10.3586030124587,-21.199520887919,0.));
#191080=CARTESIAN_POINT('Ctrl Pts',(10.34559612657,-21.1855999722416,0.));
#191081=CARTESIAN_POINT('Ctrl Pts',(10.3327073641572,-21.1717288370509,
0.));
#191082=CARTESIAN_POINT('Ctrl Pts',(10.3199370506544,-21.1579085619965,
0.));
#191083=CARTESIAN_POINT('Ctrl Pts',(10.3072855142687,-21.1441402425843,
0.));
#191084=CARTESIAN_POINT('Ctrl Pts',(10.2947530860721,-21.1304249906002,
0.));
#191085=CARTESIAN_POINT('Ctrl Pts',(10.2823401001072,-21.1167639345631,
0.));
#191086=CARTESIAN_POINT('Ctrl Pts',(10.2700468934744,-21.1031582201627,
0.));
#191087=CARTESIAN_POINT('Ctrl Pts',(10.2578738064181,-21.0896090107063,
0.));
#191088=CARTESIAN_POINT('Ctrl Pts',(10.2458211823912,-21.0761174875445,
0.));
#191089=CARTESIAN_POINT('Ctrl Pts',(10.2338893681567,-21.0626848505663,
0.));
#191090=CARTESIAN_POINT('Ctrl Pts',(10.2220787139154,-21.0493123187483,
0.));
#191091=CARTESIAN_POINT('Ctrl Pts',(10.2103895734123,-21.0360011306815,
0.));
#191092=CARTESIAN_POINT('Ctrl Pts',(10.1988223040425,-21.0227525451107,
0.));
#191093=CARTESIAN_POINT('Ctrl Pts',(10.187377266936,-21.0095678414486,0.));
#191094=CARTESIAN_POINT('Ctrl Pts',(10.1760548270767,-20.9964483203686,
0.));
#191095=CARTESIAN_POINT('Ctrl Pts',(10.1648553534568,-20.9833953044736,
0.));
#191096=CARTESIAN_POINT('Ctrl Pts',(10.1537792192065,-20.9704101389369,
0.));
#191097=CARTESIAN_POINT('Ctrl Pts',(10.1428268017256,-20.9574941921591,
0.));
#191098=CARTESIAN_POINT('Ctrl Pts',(10.1319984827908,-20.9446488563933,
0.));
#191099=CARTESIAN_POINT('Ctrl Pts',(10.1212946487057,-20.9318755484734,
0.));
#191100=CARTESIAN_POINT('Ctrl Pts',(10.1107156904836,-20.919175710627,0.));
#191101=CARTESIAN_POINT('Ctrl Pts',(10.1002620040076,-20.9065508112557,
0.));
#191102=CARTESIAN_POINT('Ctrl Pts',(10.0899339901915,-20.894002345737,0.));
#191103=CARTESIAN_POINT('Ctrl Pts',(10.0797320551154,-20.881531837184,0.));
#191104=CARTESIAN_POINT('Ctrl Pts',(10.0696566102218,-20.86914083737,0.));
#191105=CARTESIAN_POINT('Ctrl Pts',(10.0597080725375,-20.8568309277316,
0.));
#191106=CARTESIAN_POINT('Ctrl Pts',(10.0498868648733,-20.8446037203402,
0.));
#191107=CARTESIAN_POINT('Ctrl Pts',(10.0401934160234,-20.8324608588909,
0.));
#191108=CARTESIAN_POINT('Ctrl Pts',(10.0306281609435,-20.8204040196602,
0.));
#191109=CARTESIAN_POINT('Ctrl Pts',(10.0211915410095,-20.8084349126888,
0.));
#191110=CARTESIAN_POINT('Ctrl Pts',(10.0118840042786,-20.7965552829908,
0.));
#191111=CARTESIAN_POINT('Ctrl Pts',(10.0027060057389,-20.7847669117568,
0.));
#191112=CARTESIAN_POINT('Ctrl Pts',(9.9936580075464,-20.7730716175417,0.));
#191113=CARTESIAN_POINT('Ctrl Pts',(9.98474047926852,-20.761471257499,0.));
#191114=CARTESIAN_POINT('Ctrl Pts',(9.97595389823469,-20.7499677289627,
0.));
#191115=CARTESIAN_POINT('Ctrl Pts',(9.96729874986201,-20.7385629709795,
0.));
#191116=CARTESIAN_POINT('Ctrl Pts',(9.95877552798397,-20.7272589658751,
0.));
#191117=CARTESIAN_POINT('Ctrl Pts',(9.95038473514948,-20.7160577407579,
0.));
#191118=CARTESIAN_POINT('Ctrl Pts',(9.94212688298236,-20.7049613692234,
0.));
#191119=CARTESIAN_POINT('Ctrl Pts',(9.93400249259729,-20.6939719732484,
0.));
#191120=CARTESIAN_POINT('Ctrl Pts',(9.92601209498748,-20.6830917250255,
0.));
#191121=CARTESIAN_POINT('Ctrl Pts',(9.91815623141288,-20.6723228488263,
0.));
#191122=CARTESIAN_POINT('Ctrl Pts',(9.91043545377007,-20.6616676228315,
0.));
#191123=CARTESIAN_POINT('Ctrl Pts',(9.90285032516692,-20.6511283817414,
0.));
#191124=CARTESIAN_POINT('Ctrl Pts',(9.89540142049119,-20.6407075193976,
0.));
#191125=CARTESIAN_POINT('Ctrl Pts',(9.88808932697305,-20.6304074914087,
0.));
#191126=CARTESIAN_POINT('Ctrl Pts',(9.88091464472675,-20.6202308177475,
0.));
#191127=CARTESIAN_POINT('Ctrl Pts',(9.87387798732955,-20.6101800854494,
0.));
#191128=CARTESIAN_POINT('Ctrl Pts',(9.86697998242622,-20.6002579513699,
0.));
#191129=CARTESIAN_POINT('Ctrl Pts',(9.86022127232747,-20.5904671449754,
0.));
#191130=CARTESIAN_POINT('Ctrl Pts',(9.8536025145698,-20.5808104710015,0.));
#191131=CARTESIAN_POINT('Ctrl Pts',(9.84712438256277,-20.5712908125139,
0.));
#191132=CARTESIAN_POINT('Ctrl Pts',(9.84078756677565,-20.5619111362402,
0.));
#191133=CARTESIAN_POINT('Ctrl Pts',(9.83459277585315,-20.552674497646,0.));
#191134=CARTESIAN_POINT('Ctrl Pts',(9.82854073773876,-20.5435840460721,
0.));
#191135=CARTESIAN_POINT('Ctrl Pts',(9.82263220080362,-20.5346430299517,
0.));
#191136=CARTESIAN_POINT('Ctrl Pts',(9.81686793455942,-20.5258548000629,
0.));
#191137=CARTESIAN_POINT('Ctrl Pts',(9.81124873025281,-20.517222812284,0.));
#191138=CARTESIAN_POINT('Ctrl Pts',(9.80577540161087,-20.5087506310505,
0.));
#191139=CARTESIAN_POINT('Ctrl Pts',(9.80044878520948,-20.5004419312107,
0.));
#191140=CARTESIAN_POINT('Ctrl Pts',(9.7952697428833,-20.4923005087943,0.));
#191141=CARTESIAN_POINT('Ctrl Pts',(9.79023916498655,-20.4843302955329,
0.));
#191142=CARTESIAN_POINT('Ctrl Pts',(9.78535797314166,-20.4765353711586,
0.));
#191143=CARTESIAN_POINT('Ctrl Pts',(9.7806271237332,-20.4689199790669,0.));
#191144=CARTESIAN_POINT('Ctrl Pts',(9.77604760815528,-20.4614885274975,
0.));
#191145=CARTESIAN_POINT('Ctrl Pts',(9.77162045104069,-20.4542455817527,
0.));
#191146=CARTESIAN_POINT('Ctrl Pts',(9.76734670980891,-20.447195862298,0.));
#191147=CARTESIAN_POINT('Ctrl Pts',(9.76322747195494,-20.44034423294,0.));
#191148=CARTESIAN_POINT('Ctrl Pts',(9.75926386289922,-20.4336957355473,
0.));
#191149=CARTESIAN_POINT('Ctrl Pts',(9.75545705902417,-20.4272556476629,
0.));
#191150=CARTESIAN_POINT('Ctrl Pts',(9.75180829786429,-20.4210295275817,
0.));
#191151=CARTESIAN_POINT('Ctrl Pts',(9.74831889242173,-20.4150232777393,
0.));
#191152=CARTESIAN_POINT('Ctrl Pts',(9.74499021838537,-20.4092430879861,
0.));
#191153=CARTESIAN_POINT('Ctrl Pts',(9.74182369656271,-20.4036953576549,
0.));
#191154=CARTESIAN_POINT('Ctrl Pts',(9.738820776132,-20.3983866213331,0.));
#191155=CARTESIAN_POINT('Ctrl Pts',(9.73598292014242,-20.3933234845647,
0.));
#191156=CARTESIAN_POINT('Ctrl Pts',(9.73331167102807,-20.3885129129912,
0.));
#191157=CARTESIAN_POINT('Ctrl Pts',(9.73080870123726,-20.3839624556742,
0.));
#191158=CARTESIAN_POINT('Ctrl Pts',(9.72847589116541,-20.3796805893304,
0.));
#191159=CARTESIAN_POINT('Ctrl Pts',(9.7263153173288,-20.3756766651951,0.));
#191160=CARTESIAN_POINT('Ctrl Pts',(9.72432910043194,-20.371960235676,0.));
#191161=CARTESIAN_POINT('Ctrl Pts',(9.72251930722489,-20.3685406190576,
0.));
#191162=CARTESIAN_POINT('Ctrl Pts',(9.7208877838108,-20.3654261611056,0.));
#191163=CARTESIAN_POINT('Ctrl Pts',(9.71943648548099,-20.3626256913981,
0.));
#191164=CARTESIAN_POINT('Ctrl Pts',(9.71816778328006,-20.3601498764344,
0.));
#191165=CARTESIAN_POINT('Ctrl Pts',(9.71708493723096,-20.3580133103356,
0.));
#191166=CARTESIAN_POINT('Ctrl Pts',(9.71619192554185,-20.3562337557875,
0.));
#191167=CARTESIAN_POINT('Ctrl Pts',(9.71549257088172,-20.3548282742361,
0.));
#191168=CARTESIAN_POINT('Ctrl Pts',(9.7149897805202,-20.3538098605706,0.));
#191169=CARTESIAN_POINT('Ctrl Pts',(9.7147459035068,-20.3533097561886,0.));
#191170=CARTESIAN_POINT('Ctrl Pts',(9.71465227853041,-20.3531126095522,
0.));
#191171=CARTESIAN_POINT('Ctrl Pts',(9.71462954053041,-20.353060251684,0.));
#191172=CARTESIAN_POINT('Ctrl Pts',(9.71462809124915,-20.353053841303,0.));
#191173=CARTESIAN_POINT('',(12.4230808101438,-22.8400320311649,0.));
#191174=CARTESIAN_POINT('Ctrl Pts',(7.52250298901263,-21.2610617890679,
0.));
#191175=CARTESIAN_POINT('Ctrl Pts',(7.52250298901263,-21.2610617890679,
12.));
#191176=CARTESIAN_POINT('Ctrl Pts',(7.52250649703969,-21.2610673466886,
0.));
#191177=CARTESIAN_POINT('Ctrl Pts',(7.52250649703969,-21.2610673466886,
12.));
#191178=CARTESIAN_POINT('Ctrl Pts',(7.52252744144903,-21.2611204474866,
0.));
#191179=CARTESIAN_POINT('Ctrl Pts',(7.52252744144903,-21.2611204474866,
12.));
#191180=CARTESIAN_POINT('Ctrl Pts',(7.5226006423166,-21.261326054066,0.));
#191181=CARTESIAN_POINT('Ctrl Pts',(7.5226006423166,-21.261326054066,12.));
#191182=CARTESIAN_POINT('Ctrl Pts',(7.52278182242669,-21.2618521283555,
0.));
#191183=CARTESIAN_POINT('Ctrl Pts',(7.52278182242669,-21.2618521283555,
12.));
#191184=CARTESIAN_POINT('Ctrl Pts',(7.52314642316199,-21.262927782038,0.));
#191185=CARTESIAN_POINT('Ctrl Pts',(7.52314642316199,-21.262927782038,12.));
#191186=CARTESIAN_POINT('Ctrl Pts',(7.52364573027552,-21.2644161259962,
0.));
#191187=CARTESIAN_POINT('Ctrl Pts',(7.52364573027552,-21.2644161259962,
12.));
#191188=CARTESIAN_POINT('Ctrl Pts',(7.52427261074297,-21.2663059157058,
0.));
#191189=CARTESIAN_POINT('Ctrl Pts',(7.52427261074297,-21.2663059157058,
12.));
#191190=CARTESIAN_POINT('Ctrl Pts',(7.5250177033353,-21.2685823838671,0.));
#191191=CARTESIAN_POINT('Ctrl Pts',(7.5250177033353,-21.2685823838671,12.));
#191192=CARTESIAN_POINT('Ctrl Pts',(7.52587126095529,-21.2712301573466,
0.));
#191193=CARTESIAN_POINT('Ctrl Pts',(7.52587126095529,-21.2712301573466,
12.));
#191194=CARTESIAN_POINT('Ctrl Pts',(7.5268252691854,-21.2742366113579,0.));
#191195=CARTESIAN_POINT('Ctrl Pts',(7.5268252691854,-21.2742366113579,12.));
#191196=CARTESIAN_POINT('Ctrl Pts',(7.52787386225332,-21.2775925269652,
0.));
#191197=CARTESIAN_POINT('Ctrl Pts',(7.52787386225332,-21.2775925269652,
12.));
#191198=CARTESIAN_POINT('Ctrl Pts',(7.52901217930407,-21.2812902781143,
0.));
#191199=CARTESIAN_POINT('Ctrl Pts',(7.52901217930407,-21.2812902781143,
12.));
#191200=CARTESIAN_POINT('Ctrl Pts',(7.53023562438229,-21.2853226580657,
0.));
#191201=CARTESIAN_POINT('Ctrl Pts',(7.53023562438229,-21.2853226580657,
12.));
#191202=CARTESIAN_POINT('Ctrl Pts',(7.53153906987855,-21.2896816163842,
0.));
#191203=CARTESIAN_POINT('Ctrl Pts',(7.53153906987855,-21.2896816163842,
12.));
#191204=CARTESIAN_POINT('Ctrl Pts',(7.53291726078526,-21.2943588989331,
0.));
#191205=CARTESIAN_POINT('Ctrl Pts',(7.53291726078526,-21.2943588989331,
12.));
#191206=CARTESIAN_POINT('Ctrl Pts',(7.53436505309942,-21.2993464250717,
0.));
#191207=CARTESIAN_POINT('Ctrl Pts',(7.53436505309942,-21.2993464250717,
12.));
#191208=CARTESIAN_POINT('Ctrl Pts',(7.53587778251735,-21.3046368712157,
0.));
#191209=CARTESIAN_POINT('Ctrl Pts',(7.53587778251735,-21.3046368712157,
12.));
#191210=CARTESIAN_POINT('Ctrl Pts',(7.53745129364615,-21.310223716773,0.));
#191211=CARTESIAN_POINT('Ctrl Pts',(7.53745129364615,-21.310223716773,12.));
#191212=CARTESIAN_POINT('Ctrl Pts',(7.53908175169898,-21.3161009456256,
0.));
#191213=CARTESIAN_POINT('Ctrl Pts',(7.53908175169898,-21.3161009456256,
12.));
#191214=CARTESIAN_POINT('Ctrl Pts',(7.54076552038278,-21.3222628524165,
0.));
#191215=CARTESIAN_POINT('Ctrl Pts',(7.54076552038278,-21.3222628524165,
12.));
#191216=CARTESIAN_POINT('Ctrl Pts',(7.5424990037703,-21.328703791771,0.));
#191217=CARTESIAN_POINT('Ctrl Pts',(7.5424990037703,-21.328703791771,12.));
#191218=CARTESIAN_POINT('Ctrl Pts',(7.54427868151267,-21.3354182340149,
0.));
#191219=CARTESIAN_POINT('Ctrl Pts',(7.54427868151267,-21.3354182340149,
12.));
#191220=CARTESIAN_POINT('Ctrl Pts',(7.54610114948346,-21.3424008295038,
0.));
#191221=CARTESIAN_POINT('Ctrl Pts',(7.54610114948346,-21.3424008295038,
12.));
#191222=CARTESIAN_POINT('Ctrl Pts',(7.5479631624633,-21.3496464761531,0.));
#191223=CARTESIAN_POINT('Ctrl Pts',(7.5479631624633,-21.3496464761531,12.));
#191224=CARTESIAN_POINT('Ctrl Pts',(7.54986166521309,-21.3571503685855,
0.));
#191225=CARTESIAN_POINT('Ctrl Pts',(7.54986166521309,-21.3571503685855,
12.));
#191226=CARTESIAN_POINT('Ctrl Pts',(7.55179375777443,-21.3649079431865,
0.));
#191227=CARTESIAN_POINT('Ctrl Pts',(7.55179375777443,-21.3649079431865,
12.));
#191228=CARTESIAN_POINT('Ctrl Pts',(7.55375667080028,-21.3729148390243,
0.));
#191229=CARTESIAN_POINT('Ctrl Pts',(7.55375667080028,-21.3729148390243,
12.));
#191230=CARTESIAN_POINT('Ctrl Pts',(7.55574773403502,-21.3811668478932,
0.));
#191231=CARTESIAN_POINT('Ctrl Pts',(7.55574773403502,-21.3811668478932,
12.));
#191232=CARTESIAN_POINT('Ctrl Pts',(7.55776435731416,-21.3896598842117,
0.));
#191233=CARTESIAN_POINT('Ctrl Pts',(7.55776435731416,-21.3896598842117,
12.));
#191234=CARTESIAN_POINT('Ctrl Pts',(7.5598040370061,-21.3983899952987,0.));
#191235=CARTESIAN_POINT('Ctrl Pts',(7.5598040370061,-21.3983899952987,12.));
#191236=CARTESIAN_POINT('Ctrl Pts',(7.56186435703621,-21.4073533630365,
0.));
#191237=CARTESIAN_POINT('Ctrl Pts',(7.56186435703621,-21.4073533630365,
12.));
#191238=CARTESIAN_POINT('Ctrl Pts',(7.56394299313684,-21.4165463106254,
0.));
#191239=CARTESIAN_POINT('Ctrl Pts',(7.56394299313684,-21.4165463106254,
12.));
#191240=CARTESIAN_POINT('Ctrl Pts',(7.56603771218711,-21.4259653015736,
0.));
#191241=CARTESIAN_POINT('Ctrl Pts',(7.56603771218711,-21.4259653015736,
12.));
#191242=CARTESIAN_POINT('Ctrl Pts',(7.56814636360847,-21.4356069261513,
0.));
#191243=CARTESIAN_POINT('Ctrl Pts',(7.56814636360847,-21.4356069261513,
12.));
#191244=CARTESIAN_POINT('Ctrl Pts',(7.57026687261165,-21.4454678907509,
0.));
#191245=CARTESIAN_POINT('Ctrl Pts',(7.57026687261165,-21.4454678907509,
12.));
#191246=CARTESIAN_POINT('Ctrl Pts',(7.57239723223505,-21.4555450053142,
0.));
#191247=CARTESIAN_POINT('Ctrl Pts',(7.57239723223505,-21.4555450053142,
12.));
#191248=CARTESIAN_POINT('Ctrl Pts',(7.57453549743411,-21.4658351740128,
0.));
#191249=CARTESIAN_POINT('Ctrl Pts',(7.57453549743411,-21.4658351740128,
12.));
#191250=CARTESIAN_POINT('Ctrl Pts',(7.57667978402986,-21.4763353936762,
0.));
#191251=CARTESIAN_POINT('Ctrl Pts',(7.57667978402986,-21.4763353936762,
12.));
#191252=CARTESIAN_POINT('Ctrl Pts',(7.57882826679131,-21.4870427508194,
0.));
#191253=CARTESIAN_POINT('Ctrl Pts',(7.57882826679131,-21.4870427508194,
12.));
#191254=CARTESIAN_POINT('Ctrl Pts',(7.58097917790743,-21.4979544192744,
0.));
#191255=CARTESIAN_POINT('Ctrl Pts',(7.58097917790743,-21.4979544192744,
12.));
#191256=CARTESIAN_POINT('Ctrl Pts',(7.58313080519179,-21.5090676573873,
0.));
#191257=CARTESIAN_POINT('Ctrl Pts',(7.58313080519179,-21.5090676573873,
12.));
#191258=CARTESIAN_POINT('Ctrl Pts',(7.58528148919129,-21.5203798035299,
0.));
#191259=CARTESIAN_POINT('Ctrl Pts',(7.58528148919129,-21.5203798035299,
12.));
#191260=CARTESIAN_POINT('Ctrl Pts',(7.58742962034833,-21.5318882716736,
0.));
#191261=CARTESIAN_POINT('Ctrl Pts',(7.58742962034833,-21.5318882716736,
12.));
#191262=CARTESIAN_POINT('Ctrl Pts',(7.58957363620013,-21.543590547011,0.));
#191263=CARTESIAN_POINT('Ctrl Pts',(7.58957363620013,-21.543590547011,12.));
#191264=CARTESIAN_POINT('Ctrl Pts',(7.59171201844776,-21.5554841813462,
0.));
#191265=CARTESIAN_POINT('Ctrl Pts',(7.59171201844776,-21.5554841813462,
12.));
#191266=CARTESIAN_POINT('Ctrl Pts',(7.59384329124918,-21.5675667904726,
0.));
#191267=CARTESIAN_POINT('Ctrl Pts',(7.59384329124918,-21.5675667904726,
12.));
#191268=CARTESIAN_POINT('Ctrl Pts',(7.59596601973583,-21.5798360518978,
0.));
#191269=CARTESIAN_POINT('Ctrl Pts',(7.59596601973583,-21.5798360518978,
12.));
#191270=CARTESIAN_POINT('Ctrl Pts',(7.59807880846194,-21.5922897024466,
0.));
#191271=CARTESIAN_POINT('Ctrl Pts',(7.59807880846194,-21.5922897024466,
12.));
#191272=CARTESIAN_POINT('Ctrl Pts',(7.6001802998824,-21.6049255358843,0.));
#191273=CARTESIAN_POINT('Ctrl Pts',(7.6001802998824,-21.6049255358843,12.));
#191274=CARTESIAN_POINT('Ctrl Pts',(7.60226917285428,-21.617741400599,0.));
#191275=CARTESIAN_POINT('Ctrl Pts',(7.60226917285428,-21.617741400599,12.));
#191276=CARTESIAN_POINT('Ctrl Pts',(7.60434414118295,-21.6307351973822,
0.));
#191277=CARTESIAN_POINT('Ctrl Pts',(7.60434414118295,-21.6307351973822,
12.));
#191278=CARTESIAN_POINT('Ctrl Pts',(7.60640395216356,-21.6439048771743,
0.));
#191279=CARTESIAN_POINT('Ctrl Pts',(7.60640395216356,-21.6439048771743,
12.));
#191280=CARTESIAN_POINT('Ctrl Pts',(7.60844738512873,-21.6572484388081,
0.));
#191281=CARTESIAN_POINT('Ctrl Pts',(7.60844738512873,-21.6572484388081,
12.));
#191282=CARTESIAN_POINT('Ctrl Pts',(7.61047325000955,-21.6707639267576,
0.));
#191283=CARTESIAN_POINT('Ctrl Pts',(7.61047325000955,-21.6707639267576,
12.));
#191284=CARTESIAN_POINT('Ctrl Pts',(7.61248038630268,-21.6844494295815,
0.));
#191285=CARTESIAN_POINT('Ctrl Pts',(7.61248038630268,-21.6844494295815,
12.));
#191286=CARTESIAN_POINT('Ctrl Pts',(7.61446766202786,-21.6983030783322,
0.));
#191287=CARTESIAN_POINT('Ctrl Pts',(7.61446766202786,-21.6983030783322,
12.));
#191288=CARTESIAN_POINT('Ctrl Pts',(7.6164339727042,-21.7123230449834,0.));
#191289=CARTESIAN_POINT('Ctrl Pts',(7.6164339727042,-21.7123230449834,12.));
#191290=CARTESIAN_POINT('Ctrl Pts',(7.61837824030537,-21.7265075407975,
0.));
#191291=CARTESIAN_POINT('Ctrl Pts',(7.61837824030537,-21.7265075407975,
12.));
#191292=CARTESIAN_POINT('Ctrl Pts',(7.62029941230854,-21.7408548148656,
0.));
#191293=CARTESIAN_POINT('Ctrl Pts',(7.62029941230854,-21.7408548148656,
12.));
#191294=CARTESIAN_POINT('Ctrl Pts',(7.62219646084228,-21.7553631528328,
0.));
#191295=CARTESIAN_POINT('Ctrl Pts',(7.62219646084228,-21.7553631528328,
12.));
#191296=CARTESIAN_POINT('Ctrl Pts',(7.62406838181165,-21.7700308755584,
0.));
#191297=CARTESIAN_POINT('Ctrl Pts',(7.62406838181165,-21.7700308755584,
12.));
#191298=CARTESIAN_POINT('Ctrl Pts',(7.62591419404512,-21.7848563378021,
0.));
#191299=CARTESIAN_POINT('Ctrl Pts',(7.62591419404512,-21.7848563378021,
12.));
#191300=CARTESIAN_POINT('Ctrl Pts',(7.62773293842388,-21.799837926858,0.));
#191301=CARTESIAN_POINT('Ctrl Pts',(7.62773293842388,-21.799837926858,12.));
#191302=CARTESIAN_POINT('Ctrl Pts',(7.62952367718126,-21.814974061509,0.));
#191303=CARTESIAN_POINT('Ctrl Pts',(7.62952367718126,-21.814974061509,12.));
#191304=CARTESIAN_POINT('Ctrl Pts',(7.63128549323022,-21.8302631910195,
0.));
#191305=CARTESIAN_POINT('Ctrl Pts',(7.63128549323022,-21.8302631910195,
12.));
#191306=CARTESIAN_POINT('Ctrl Pts',(7.63301748948935,-21.8457037941084,
0.));
#191307=CARTESIAN_POINT('Ctrl Pts',(7.63301748948935,-21.8457037941084,
12.));
#191308=CARTESIAN_POINT('Ctrl Pts',(7.63471878821225,-21.8612943779089,
0.));
#191309=CARTESIAN_POINT('Ctrl Pts',(7.63471878821225,-21.8612943779089,
12.));
#191310=CARTESIAN_POINT('Ctrl Pts',(7.63638853033399,-21.8770334769496,
0.));
#191311=CARTESIAN_POINT('Ctrl Pts',(7.63638853033399,-21.8770334769496,
12.));
#191312=CARTESIAN_POINT('Ctrl Pts',(7.63802587492034,-21.8929196523514,
0.));
#191313=CARTESIAN_POINT('Ctrl Pts',(7.63802587492034,-21.8929196523514,
12.));
#191314=CARTESIAN_POINT('Ctrl Pts',(7.63962999860926,-21.9089514909874,
0.));
#191315=CARTESIAN_POINT('Ctrl Pts',(7.63962999860926,-21.9089514909874,
12.));
#191316=CARTESIAN_POINT('Ctrl Pts',(7.64120009506531,-21.9251276046546,
0.));
#191317=CARTESIAN_POINT('Ctrl Pts',(7.64120009506531,-21.9251276046546,
12.));
#191318=CARTESIAN_POINT('Ctrl Pts',(7.64273537442681,-21.9414466292072,
0.));
#191319=CARTESIAN_POINT('Ctrl Pts',(7.64273537442681,-21.9414466292072,
12.));
#191320=CARTESIAN_POINT('Ctrl Pts',(7.64423506279122,-21.9579072237651,
0.));
#191321=CARTESIAN_POINT('Ctrl Pts',(7.64423506279122,-21.9579072237651,
12.));
#191322=CARTESIAN_POINT('Ctrl Pts',(7.64569840177335,-21.9745080700798,
0.));
#191323=CARTESIAN_POINT('Ctrl Pts',(7.64569840177335,-21.9745080700798,
12.));
#191324=CARTESIAN_POINT('Ctrl Pts',(7.64712464805249,-21.9912478718542,
0.));
#191325=CARTESIAN_POINT('Ctrl Pts',(7.64712464805249,-21.9912478718542,
12.));
#191326=CARTESIAN_POINT('Ctrl Pts',(7.64851307293351,-22.0081253540774,
0.));
#191327=CARTESIAN_POINT('Ctrl Pts',(7.64851307293351,-22.0081253540774,
12.));
#191328=CARTESIAN_POINT('Ctrl Pts',(7.64986296190168,-22.0251392623209,
0.));
#191329=CARTESIAN_POINT('Ctrl Pts',(7.64986296190168,-22.0251392623209,
12.));
#191330=CARTESIAN_POINT('Ctrl Pts',(7.65117361421358,-22.0422883621174,
0.));
#191331=CARTESIAN_POINT('Ctrl Pts',(7.65117361421358,-22.0422883621174,
12.));
#191332=CARTESIAN_POINT('Ctrl Pts',(7.65244434253112,-22.0595714384431,
0.));
#191333=CARTESIAN_POINT('Ctrl Pts',(7.65244434253112,-22.0595714384431,
12.));
#191334=CARTESIAN_POINT('Ctrl Pts',(7.65367447254949,-22.0769872951596,
0.));
#191335=CARTESIAN_POINT('Ctrl Pts',(7.65367447254949,-22.0769872951596,
12.));
#191336=CARTESIAN_POINT('Ctrl Pts',(7.65486334263643,-22.094534754469,0.));
#191337=CARTESIAN_POINT('Ctrl Pts',(7.65486334263643,-22.094534754469,12.));
#191338=CARTESIAN_POINT('Ctrl Pts',(7.65601030346806,-22.1122126563329,
0.));
#191339=CARTESIAN_POINT('Ctrl Pts',(7.65601030346806,-22.1122126563329,
12.));
#191340=CARTESIAN_POINT('Ctrl Pts',(7.65711471769396,-22.1300198579675,
0.));
#191341=CARTESIAN_POINT('Ctrl Pts',(7.65711471769396,-22.1300198579675,
12.));
#191342=CARTESIAN_POINT('Ctrl Pts',(7.65817595963348,-22.1479552334211,
0.));
#191343=CARTESIAN_POINT('Ctrl Pts',(7.65817595963348,-22.1479552334211,
12.));
#191344=CARTESIAN_POINT('Ctrl Pts',(7.6591934149693,-22.1660176731178,0.));
#191345=CARTESIAN_POINT('Ctrl Pts',(7.6591934149693,-22.1660176731178,12.));
#191346=CARTESIAN_POINT('Ctrl Pts',(7.66016648045004,-22.1842060834091,
0.));
#191347=CARTESIAN_POINT('Ctrl Pts',(7.66016648045004,-22.1842060834091,
12.));
#191348=CARTESIAN_POINT('Ctrl Pts',(7.6610945635927,-22.2025193860964,0.));
#191349=CARTESIAN_POINT('Ctrl Pts',(7.6610945635927,-22.2025193860964,12.));
#191350=CARTESIAN_POINT('Ctrl Pts',(7.66197708240399,-22.2209565180085,
0.));
#191351=CARTESIAN_POINT('Ctrl Pts',(7.66197708240399,-22.2209565180085,
12.));
#191352=CARTESIAN_POINT('Ctrl Pts',(7.66281346512508,-22.2395164306547,
0.));
#191353=CARTESIAN_POINT('Ctrl Pts',(7.66281346512508,-22.2395164306547,
12.));
#191354=CARTESIAN_POINT('Ctrl Pts',(7.6636031499764,-22.258198089848,0.));
#191355=CARTESIAN_POINT('Ctrl Pts',(7.6636031499764,-22.258198089848,12.));
#191356=CARTESIAN_POINT('Ctrl Pts',(7.66434558490978,-22.2770004753335,
0.));
#191357=CARTESIAN_POINT('Ctrl Pts',(7.66434558490978,-22.2770004753335,
12.));
#191358=CARTESIAN_POINT('Ctrl Pts',(7.66504022736298,-22.2959225803937,
0.));
#191359=CARTESIAN_POINT('Ctrl Pts',(7.66504022736298,-22.2959225803937,
12.));
#191360=CARTESIAN_POINT('Ctrl Pts',(7.66568654402493,-22.314963411484,0.));
#191361=CARTESIAN_POINT('Ctrl Pts',(7.66568654402493,-22.314963411484,12.));
#191362=CARTESIAN_POINT('Ctrl Pts',(7.66628401061951,-22.3341219879469,
0.));
#191363=CARTESIAN_POINT('Ctrl Pts',(7.66628401061951,-22.3341219879469,
12.));
#191364=CARTESIAN_POINT('Ctrl Pts',(7.66683211169157,-22.3533973417021,
0.));
#191365=CARTESIAN_POINT('Ctrl Pts',(7.66683211169157,-22.3533973417021,
12.));
#191366=CARTESIAN_POINT('Ctrl Pts',(7.66733034039882,-22.372788516936,0.));
#191367=CARTESIAN_POINT('Ctrl Pts',(7.66733034039882,-22.372788516936,12.));
#191368=CARTESIAN_POINT('Ctrl Pts',(7.66777819830789,-22.3922945697773,
0.));
#191369=CARTESIAN_POINT('Ctrl Pts',(7.66777819830789,-22.3922945697773,
12.));
#191370=CARTESIAN_POINT('Ctrl Pts',(7.66817519519639,-22.4119145679758,
0.));
#191371=CARTESIAN_POINT('Ctrl Pts',(7.66817519519639,-22.4119145679758,
12.));
#191372=CARTESIAN_POINT('Ctrl Pts',(7.66852084886703,-22.4316475906603,
0.));
#191373=CARTESIAN_POINT('Ctrl Pts',(7.66852084886703,-22.4316475906603,
12.));
#191374=CARTESIAN_POINT('Ctrl Pts',(7.66881468496634,-22.4514927280855,
0.));
#191375=CARTESIAN_POINT('Ctrl Pts',(7.66881468496634,-22.4514927280855,
12.));
#191376=CARTESIAN_POINT('Ctrl Pts',(7.6690562368083,-22.47144908137,0.));
#191377=CARTESIAN_POINT('Ctrl Pts',(7.6690562368083,-22.47144908137,12.));
#191378=CARTESIAN_POINT('Ctrl Pts',(7.66924504520314,-22.4915157622312,
0.));
#191379=CARTESIAN_POINT('Ctrl Pts',(7.66924504520314,-22.4915157622312,
12.));
#191380=CARTESIAN_POINT('Ctrl Pts',(7.66938065829107,-22.5116918927032,
0.));
#191381=CARTESIAN_POINT('Ctrl Pts',(7.66938065829107,-22.5116918927032,
12.));
#191382=CARTESIAN_POINT('Ctrl Pts',(7.66946263138143,-22.53197660492,0.));
#191383=CARTESIAN_POINT('Ctrl Pts',(7.66946263138143,-22.53197660492,12.));
#191384=CARTESIAN_POINT('Ctrl Pts',(7.66949052679692,-22.5523690409116,
0.));
#191385=CARTESIAN_POINT('Ctrl Pts',(7.66949052679692,-22.5523690409116,
12.));
#191386=CARTESIAN_POINT('Ctrl Pts',(7.66946391372305,-22.5728683523831,
0.));
#191387=CARTESIAN_POINT('Ctrl Pts',(7.66946391372305,-22.5728683523831,
12.));
#191388=CARTESIAN_POINT('Ctrl Pts',(7.66938236806232,-22.5934737004953,
0.));
#191389=CARTESIAN_POINT('Ctrl Pts',(7.66938236806232,-22.5934737004953,
12.));
#191390=CARTESIAN_POINT('Ctrl Pts',(7.66924547229413,-22.6141842556243,
0.));
#191391=CARTESIAN_POINT('Ctrl Pts',(7.66924547229413,-22.6141842556243,
12.));
#191392=CARTESIAN_POINT('Ctrl Pts',(7.66905281533714,-22.6349991971541,
0.));
#191393=CARTESIAN_POINT('Ctrl Pts',(7.66905281533714,-22.6349991971541,
12.));
#191394=CARTESIAN_POINT('Ctrl Pts',(7.66880399241322,-22.6559177133127,
0.));
#191395=CARTESIAN_POINT('Ctrl Pts',(7.66880399241322,-22.6559177133127,
12.));
#191396=CARTESIAN_POINT('Ctrl Pts',(7.66849860491742,-22.6769390009885,
0.));
#191397=CARTESIAN_POINT('Ctrl Pts',(7.66849860491742,-22.6769390009885,
12.));
#191398=CARTESIAN_POINT('Ctrl Pts',(7.66813626029274,-22.6980622655446,
0.));
#191399=CARTESIAN_POINT('Ctrl Pts',(7.66813626029274,-22.6980622655446,
12.));
#191400=CARTESIAN_POINT('Ctrl Pts',(7.66771657191027,-22.7192867206245,
0.));
#191401=CARTESIAN_POINT('Ctrl Pts',(7.66771657191027,-22.7192867206245,
12.));
#191402=CARTESIAN_POINT('Ctrl Pts',(7.66723915895439,-22.7406115879513,
0.));
#191403=CARTESIAN_POINT('Ctrl Pts',(7.66723915895439,-22.7406115879513,
12.));
#191404=CARTESIAN_POINT('Ctrl Pts',(7.66670364630298,-22.7620360971843,
0.));
#191405=CARTESIAN_POINT('Ctrl Pts',(7.66670364630298,-22.7620360971843,
12.));
#191406=CARTESIAN_POINT('Ctrl Pts',(7.66610966441272,-22.7835594857699,
0.));
#191407=CARTESIAN_POINT('Ctrl Pts',(7.66610966441272,-22.7835594857699,
12.));
#191408=CARTESIAN_POINT('Ctrl Pts',(7.66545684920986,-22.8051809987833,
0.));
#191409=CARTESIAN_POINT('Ctrl Pts',(7.66545684920986,-22.8051809987833,
12.));
#191410=CARTESIAN_POINT('Ctrl Pts',(7.66474484198548,-22.8268998887678,
0.));
#191411=CARTESIAN_POINT('Ctrl Pts',(7.66474484198548,-22.8268998887678,
12.));
#191412=CARTESIAN_POINT('Ctrl Pts',(7.66397328929802,-22.848715415557,0.));
#191413=CARTESIAN_POINT('Ctrl Pts',(7.66397328929802,-22.848715415557,12.));
#191414=CARTESIAN_POINT('Ctrl Pts',(7.66314184287336,-22.8706268461283,
0.));
#191415=CARTESIAN_POINT('Ctrl Pts',(7.66314184287336,-22.8706268461283,
12.));
#191416=CARTESIAN_POINT('Ctrl Pts',(7.66225015950155,-22.8926334544883,
0.));
#191417=CARTESIAN_POINT('Ctrl Pts',(7.66225015950155,-22.8926334544883,
12.));
#191418=CARTESIAN_POINT('Ctrl Pts',(7.66129790094107,-22.9147345215421,
0.));
#191419=CARTESIAN_POINT('Ctrl Pts',(7.66129790094107,-22.9147345215421,
12.));
#191420=CARTESIAN_POINT('Ctrl Pts',(7.66028473382777,-22.9369293349593,
0.));
#191421=CARTESIAN_POINT('Ctrl Pts',(7.66028473382777,-22.9369293349593,
12.));
#191422=CARTESIAN_POINT('Ctrl Pts',(7.65921032958901,-22.959217189033,0.));
#191423=CARTESIAN_POINT('Ctrl Pts',(7.65921032958901,-22.959217189033,12.));
#191424=CARTESIAN_POINT('Ctrl Pts',(7.65807436436431,-22.9815973845296,
0.));
#191425=CARTESIAN_POINT('Ctrl Pts',(7.65807436436431,-22.9815973845296,
12.));
#191426=CARTESIAN_POINT('Ctrl Pts',(7.65687651891303,-23.0040692285814,
0.));
#191427=CARTESIAN_POINT('Ctrl Pts',(7.65687651891303,-23.0040692285814,
12.));
#191428=CARTESIAN_POINT('Ctrl Pts',(7.65561647852533,-23.0266320345787,
0.));
#191429=CARTESIAN_POINT('Ctrl Pts',(7.65561647852533,-23.0266320345787,
12.));
#191430=CARTESIAN_POINT('Ctrl Pts',(7.65429393293945,-23.0492851220528,
0.));
#191431=CARTESIAN_POINT('Ctrl Pts',(7.65429393293945,-23.0492851220528,
12.));
#191432=CARTESIAN_POINT('Ctrl Pts',(7.65290857626357,-23.072027816555,0.));
#191433=CARTESIAN_POINT('Ctrl Pts',(7.65290857626357,-23.072027816555,12.));
#191434=CARTESIAN_POINT('Ctrl Pts',(7.65146010690475,-23.094859449525,0.));
#191435=CARTESIAN_POINT('Ctrl Pts',(7.65146010690475,-23.094859449525,12.));
#191436=CARTESIAN_POINT('Ctrl Pts',(7.64994822749859,-23.1177793581679,
0.));
#191437=CARTESIAN_POINT('Ctrl Pts',(7.64994822749859,-23.1177793581679,
12.));
#191438=CARTESIAN_POINT('Ctrl Pts',(7.64837264482942,-23.1407868853819,
0.));
#191439=CARTESIAN_POINT('Ctrl Pts',(7.64837264482942,-23.1407868853819,
12.));
#191440=CARTESIAN_POINT('Ctrl Pts',(7.64673306975804,-23.1638813796694,
0.));
#191441=CARTESIAN_POINT('Ctrl Pts',(7.64673306975804,-23.1638813796694,
12.));
#191442=CARTESIAN_POINT('Ctrl Pts',(7.64502921715482,-23.1870621950452,
0.));
#191443=CARTESIAN_POINT('Ctrl Pts',(7.64502921715482,-23.1870621950452,
12.));
#191444=CARTESIAN_POINT('Ctrl Pts',(7.64326080583679,-23.2103286909398,
0.));
#191445=CARTESIAN_POINT('Ctrl Pts',(7.64326080583679,-23.2103286909398,
12.));
#191446=CARTESIAN_POINT('Ctrl Pts',(7.64142755851504,-23.2336802320912,
0.));
#191447=CARTESIAN_POINT('Ctrl Pts',(7.64142755851504,-23.2336802320912,
12.));
#191448=CARTESIAN_POINT('Ctrl Pts',(7.63952920172834,-23.2571161884488,
0.));
#191449=CARTESIAN_POINT('Ctrl Pts',(7.63952920172834,-23.2571161884488,
12.));
#191450=CARTESIAN_POINT('Ctrl Pts',(7.63756546576373,-23.2806359350855,
0.));
#191451=CARTESIAN_POINT('Ctrl Pts',(7.63756546576373,-23.2806359350855,
12.));
#191452=CARTESIAN_POINT('Ctrl Pts',(7.63553608458782,-23.3042388521022,
0.));
#191453=CARTESIAN_POINT('Ctrl Pts',(7.63553608458782,-23.3042388521022,
12.));
#191454=CARTESIAN_POINT('Ctrl Pts',(7.63344079578161,-23.3279243245241,
0.));
#191455=CARTESIAN_POINT('Ctrl Pts',(7.63344079578161,-23.3279243245241,
12.));
#191456=CARTESIAN_POINT('Ctrl Pts',(7.63127934048136,-23.3516917421972,
0.));
#191457=CARTESIAN_POINT('Ctrl Pts',(7.63127934048136,-23.3516917421972,
12.));
#191458=CARTESIAN_POINT('Ctrl Pts',(7.62905146332592,-23.3755404996636,
0.));
#191459=CARTESIAN_POINT('Ctrl Pts',(7.62905146332592,-23.3755404996636,
12.));
#191460=CARTESIAN_POINT('Ctrl Pts',(7.62675691240328,-23.399469996112,0.));
#191461=CARTESIAN_POINT('Ctrl Pts',(7.62675691240328,-23.399469996112,12.));
#191462=CARTESIAN_POINT('Ctrl Pts',(7.62439543920049,-23.4234796353542,
0.));
#191463=CARTESIAN_POINT('Ctrl Pts',(7.62439543920049,-23.4234796353542,
12.));
#191464=CARTESIAN_POINT('Ctrl Pts',(7.62196679855954,-23.4475688257854,
0.));
#191465=CARTESIAN_POINT('Ctrl Pts',(7.62196679855954,-23.4475688257854,
12.));
#191466=CARTESIAN_POINT('Ctrl Pts',(7.61947074863976,-23.4717369803438,
0.));
#191467=CARTESIAN_POINT('Ctrl Pts',(7.61947074863976,-23.4717369803438,
12.));
#191468=CARTESIAN_POINT('Ctrl Pts',(7.61690705088318,-23.4959835164609,
0.));
#191469=CARTESIAN_POINT('Ctrl Pts',(7.61690705088318,-23.4959835164609,
12.));
#191470=CARTESIAN_POINT('Ctrl Pts',(7.61427546999297,-23.5203078560129,
0.));
#191471=CARTESIAN_POINT('Ctrl Pts',(7.61427546999297,-23.5203078560129,
12.));
#191472=CARTESIAN_POINT('Ctrl Pts',(7.61157577385371,-23.544709425203,0.));
#191473=CARTESIAN_POINT('Ctrl Pts',(7.61157577385371,-23.544709425203,12.));
#191474=CARTESIAN_POINT('Ctrl Pts',(7.60880773344599,-23.5691876544244,
0.));
#191475=CARTESIAN_POINT('Ctrl Pts',(7.60880773344599,-23.5691876544244,
12.));
#191476=CARTESIAN_POINT('Ctrl Pts',(7.60597112277093,-23.5937419781245,
0.));
#191477=CARTESIAN_POINT('Ctrl Pts',(7.60597112277093,-23.5937419781245,
12.));
#191478=CARTESIAN_POINT('Ctrl Pts',(7.60306571877805,-23.6183718346576,
0.));
#191479=CARTESIAN_POINT('Ctrl Pts',(7.60306571877805,-23.6183718346576,
12.));
#191480=CARTESIAN_POINT('Ctrl Pts',(7.60009130130125,-23.6430766661418,
0.));
#191481=CARTESIAN_POINT('Ctrl Pts',(7.60009130130125,-23.6430766661418,
12.));
#191482=CARTESIAN_POINT('Ctrl Pts',(7.59704765299566,-23.6678559182875,
0.));
#191483=CARTESIAN_POINT('Ctrl Pts',(7.59704765299566,-23.6678559182875,
12.));
#191484=CARTESIAN_POINT('Ctrl Pts',(7.59393455934034,-23.6927090405066,
0.));
#191485=CARTESIAN_POINT('Ctrl Pts',(7.59393455934034,-23.6927090405066,
12.));
#191486=CARTESIAN_POINT('Ctrl Pts',(7.5907518086532,-23.7176354860457,0.));
#191487=CARTESIAN_POINT('Ctrl Pts',(7.5907518086532,-23.7176354860457,12.));
#191488=CARTESIAN_POINT('Ctrl Pts',(7.58749919210825,-23.7426347121006,
0.));
#191489=CARTESIAN_POINT('Ctrl Pts',(7.58749919210825,-23.7426347121006,
12.));
#191490=CARTESIAN_POINT('Ctrl Pts',(7.5841765037627,-23.7677061799376,0.));
#191491=CARTESIAN_POINT('Ctrl Pts',(7.5841765037627,-23.7677061799376,12.));
#191492=CARTESIAN_POINT('Ctrl Pts',(7.58078354058212,-23.7928493549908,
0.));
#191493=CARTESIAN_POINT('Ctrl Pts',(7.58078354058212,-23.7928493549908,
12.));
#191494=CARTESIAN_POINT('Ctrl Pts',(7.57732010249065,-23.8180637069976,
0.));
#191495=CARTESIAN_POINT('Ctrl Pts',(7.57732010249065,-23.8180637069976,
12.));
#191496=CARTESIAN_POINT('Ctrl Pts',(7.57378599219813,-23.8433487096132,
0.));
#191497=CARTESIAN_POINT('Ctrl Pts',(7.57378599219813,-23.8433487096132,
12.));
#191498=CARTESIAN_POINT('Ctrl Pts',(7.57018101500708,-23.8687038399595,
0.));
#191499=CARTESIAN_POINT('Ctrl Pts',(7.57018101500708,-23.8687038399595,
12.));
#191500=CARTESIAN_POINT('Ctrl Pts',(7.5665049786379,-23.8941285782002,0.));
#191501=CARTESIAN_POINT('Ctrl Pts',(7.5665049786379,-23.8941285782002,12.));
#191502=CARTESIAN_POINT('Ctrl Pts',(7.56275769304772,-23.9196224070759,
0.));
#191503=CARTESIAN_POINT('Ctrl Pts',(7.56275769304772,-23.9196224070759,
12.));
#191504=CARTESIAN_POINT('Ctrl Pts',(7.55893897027679,-23.9451848115002,
0.));
#191505=CARTESIAN_POINT('Ctrl Pts',(7.55893897027679,-23.9451848115002,
12.));
#191506=CARTESIAN_POINT('Ctrl Pts',(7.55504862424807,-23.9708152779886,
0.));
#191507=CARTESIAN_POINT('Ctrl Pts',(7.55504862424807,-23.9708152779886,
12.));
#191508=CARTESIAN_POINT('Ctrl Pts',(7.55108647097431,-23.9965132953187,
0.));
#191509=CARTESIAN_POINT('Ctrl Pts',(7.55108647097431,-23.9965132953187,
12.));
#191510=CARTESIAN_POINT('Ctrl Pts',(7.54705232885894,-24.0222783554531,
0.));
#191511=CARTESIAN_POINT('Ctrl Pts',(7.54705232885894,-24.0222783554531,
12.));
#191512=CARTESIAN_POINT('Ctrl Pts',(7.54294601896127,-24.0481099543353,
0.));
#191513=CARTESIAN_POINT('Ctrl Pts',(7.54294601896127,-24.0481099543353,
12.));
#191514=CARTESIAN_POINT('Ctrl Pts',(7.53876736531004,-24.0740075927984,
0.));
#191515=CARTESIAN_POINT('Ctrl Pts',(7.53876736531004,-24.0740075927984,
12.));
#191516=CARTESIAN_POINT('Ctrl Pts',(7.53451619514658,-24.0999707772643,
0.));
#191517=CARTESIAN_POINT('Ctrl Pts',(7.53451619514658,-24.0999707772643,
12.));
#191518=CARTESIAN_POINT('Ctrl Pts',(7.53019233935536,-24.1259990209211,
0.));
#191519=CARTESIAN_POINT('Ctrl Pts',(7.53019233935536,-24.1259990209211,
12.));
#191520=CARTESIAN_POINT('Ctrl Pts',(7.52579563201478,-24.152091842537,0.));
#191521=CARTESIAN_POINT('Ctrl Pts',(7.52579563201478,-24.152091842537,12.));
#191522=CARTESIAN_POINT('Ctrl Pts',(7.52132590953862,-24.1782487641602,
0.));
#191523=CARTESIAN_POINT('Ctrl Pts',(7.52132590953862,-24.1782487641602,
12.));
#191524=CARTESIAN_POINT('Ctrl Pts',(7.51678300997997,-24.2044693092356,
0.));
#191525=CARTESIAN_POINT('Ctrl Pts',(7.51678300997997,-24.2044693092356,
12.));
#191526=CARTESIAN_POINT('Ctrl Pts',(7.51216677222198,-24.230753000389,0.));
#191527=CARTESIAN_POINT('Ctrl Pts',(7.51216677222198,-24.230753000389,12.));
#191528=CARTESIAN_POINT('Ctrl Pts',(7.50747703535114,-24.2570993577032,
0.));
#191529=CARTESIAN_POINT('Ctrl Pts',(7.50747703535114,-24.2570993577032,
12.));
#191530=CARTESIAN_POINT('Ctrl Pts',(7.50271363765098,-24.2835078958966,
0.));
#191531=CARTESIAN_POINT('Ctrl Pts',(7.50271363765098,-24.2835078958966,
12.));
#191532=CARTESIAN_POINT('Ctrl Pts',(7.49787641695358,-24.3099781253345,
0.));
#191533=CARTESIAN_POINT('Ctrl Pts',(7.49787641695358,-24.3099781253345,
12.));
#191534=CARTESIAN_POINT('Ctrl Pts',(7.49296521252329,-24.3365095573673,
0.));
#191535=CARTESIAN_POINT('Ctrl Pts',(7.49296521252329,-24.3365095573673,
12.));
#191536=CARTESIAN_POINT('Ctrl Pts',(7.48797986651827,-24.3631017084513,
0.));
#191537=CARTESIAN_POINT('Ctrl Pts',(7.48797986651827,-24.3631017084513,
12.));
#191538=CARTESIAN_POINT('Ctrl Pts',(7.48292022569253,-24.3897541049248,
0.));
#191539=CARTESIAN_POINT('Ctrl Pts',(7.48292022569253,-24.3897541049248,
12.));
#191540=CARTESIAN_POINT('Ctrl Pts',(7.47778614286572,-24.4164662871165,
0.));
#191541=CARTESIAN_POINT('Ctrl Pts',(7.47778614286572,-24.4164662871165,
12.));
#191542=CARTESIAN_POINT('Ctrl Pts',(7.47257747883318,-24.4432378146501,
0.));
#191543=CARTESIAN_POINT('Ctrl Pts',(7.47257747883318,-24.4432378146501,
12.));
#191544=CARTESIAN_POINT('Ctrl Pts',(7.46729410308922,-24.4700682684544,
0.));
#191545=CARTESIAN_POINT('Ctrl Pts',(7.46729410308922,-24.4700682684544,
12.));
#191546=CARTESIAN_POINT('Ctrl Pts',(7.46193588961641,-24.4969572391509,
0.));
#191547=CARTESIAN_POINT('Ctrl Pts',(7.46193588961641,-24.4969572391509,
12.));
#191548=CARTESIAN_POINT('Ctrl Pts',(7.45650271336044,-24.52390431731,0.));
#191549=CARTESIAN_POINT('Ctrl Pts',(7.45650271336044,-24.52390431731,12.));
#191550=CARTESIAN_POINT('Ctrl Pts',(7.45099444651295,-24.550909083158,0.));
#191551=CARTESIAN_POINT('Ctrl Pts',(7.45099444651295,-24.550909083158,12.));
#191552=CARTESIAN_POINT('Ctrl Pts',(7.44541095473162,-24.5779710960865,
0.));
#191553=CARTESIAN_POINT('Ctrl Pts',(7.44541095473162,-24.5779710960865,
12.));
#191554=CARTESIAN_POINT('Ctrl Pts',(7.43975209375374,-24.6050898852349,
0.));
#191555=CARTESIAN_POINT('Ctrl Pts',(7.43975209375374,-24.6050898852349,
12.));
#191556=CARTESIAN_POINT('Ctrl Pts',(7.4340177048922,-24.6322649369472,0.));
#191557=CARTESIAN_POINT('Ctrl Pts',(7.4340177048922,-24.6322649369472,12.));
#191558=CARTESIAN_POINT('Ctrl Pts',(7.4282076215868,-24.659495712869,0.));
#191559=CARTESIAN_POINT('Ctrl Pts',(7.4282076215868,-24.659495712869,12.));
#191560=CARTESIAN_POINT('Ctrl Pts',(7.42232167765762,-24.6867816727118,
0.));
#191561=CARTESIAN_POINT('Ctrl Pts',(7.42232167765762,-24.6867816727118,
12.));
#191562=CARTESIAN_POINT('Ctrl Pts',(7.41635971481242,-24.7141222949988,
0.));
#191563=CARTESIAN_POINT('Ctrl Pts',(7.41635971481242,-24.7141222949988,
12.));
#191564=CARTESIAN_POINT('Ctrl Pts',(7.41032159082172,-24.7415170994754,
0.));
#191565=CARTESIAN_POINT('Ctrl Pts',(7.41032159082172,-24.7415170994754,
12.));
#191566=CARTESIAN_POINT('Ctrl Pts',(7.40420718661754,-24.7689656669005,
0.));
#191567=CARTESIAN_POINT('Ctrl Pts',(7.40420718661754,-24.7689656669005,
12.));
#191568=CARTESIAN_POINT('Ctrl Pts',(7.39801641583612,-24.7964676646518,
0.));
#191569=CARTESIAN_POINT('Ctrl Pts',(7.39801641583612,-24.7964676646518,
12.));
#191570=CARTESIAN_POINT('Ctrl Pts',(7.3917492258684,-24.8240228521042,0.));
#191571=CARTESIAN_POINT('Ctrl Pts',(7.3917492258684,-24.8240228521042,12.));
#191572=CARTESIAN_POINT('Ctrl Pts',(7.38540558904945,-24.8516310625367,
0.));
#191573=CARTESIAN_POINT('Ctrl Pts',(7.38540558904945,-24.8516310625367,
12.));
#191574=CARTESIAN_POINT('Ctrl Pts',(7.37898549641609,-24.8792921911309,
0.));
#191575=CARTESIAN_POINT('Ctrl Pts',(7.37898549641609,-24.8792921911309,
12.));
#191576=CARTESIAN_POINT('Ctrl Pts',(7.37378825962717,-24.9014633826201,
0.));
#191577=CARTESIAN_POINT('Ctrl Pts',(7.37378825962717,-24.9014633826201,
12.));
#191578=CARTESIAN_POINT('Ctrl Pts',(7.36985593120695,-24.9181155530631,
0.));
#191579=CARTESIAN_POINT('Ctrl Pts',(7.36985593120695,-24.9181155530631,
12.));
#191580=CARTESIAN_POINT('Ctrl Pts',(7.36721909029059,-24.9292275670705,
0.));
#191581=CARTESIAN_POINT('Ctrl Pts',(7.36721909029059,-24.9292275670705,
12.));
#191582=CARTESIAN_POINT('Ctrl Pts',(7.36589684767343,-24.9347862158358,
0.));
#191583=CARTESIAN_POINT('Ctrl Pts',(7.36589684767343,-24.9347862158358,
12.));
#191584=CARTESIAN_POINT('',(7.36589684767343,-24.9347862158358,0.));
#191585=CARTESIAN_POINT('Ctrl Pts',(7.52250298901263,-21.2610617890679,
0.));
#191586=CARTESIAN_POINT('Ctrl Pts',(7.52250649703969,-21.2610673466886,
0.));
#191587=CARTESIAN_POINT('Ctrl Pts',(7.52252744144903,-21.2611204474866,
0.));
#191588=CARTESIAN_POINT('Ctrl Pts',(7.5226006423166,-21.261326054066,0.));
#191589=CARTESIAN_POINT('Ctrl Pts',(7.52278182242669,-21.2618521283555,
0.));
#191590=CARTESIAN_POINT('Ctrl Pts',(7.52314642316199,-21.262927782038,0.));
#191591=CARTESIAN_POINT('Ctrl Pts',(7.52364573027552,-21.2644161259962,
0.));
#191592=CARTESIAN_POINT('Ctrl Pts',(7.52427261074297,-21.2663059157058,
0.));
#191593=CARTESIAN_POINT('Ctrl Pts',(7.5250177033353,-21.2685823838671,0.));
#191594=CARTESIAN_POINT('Ctrl Pts',(7.52587126095529,-21.2712301573466,
0.));
#191595=CARTESIAN_POINT('Ctrl Pts',(7.5268252691854,-21.2742366113579,0.));
#191596=CARTESIAN_POINT('Ctrl Pts',(7.52787386225332,-21.2775925269652,
0.));
#191597=CARTESIAN_POINT('Ctrl Pts',(7.52901217930407,-21.2812902781143,
0.));
#191598=CARTESIAN_POINT('Ctrl Pts',(7.53023562438229,-21.2853226580657,
0.));
#191599=CARTESIAN_POINT('Ctrl Pts',(7.53153906987855,-21.2896816163842,
0.));
#191600=CARTESIAN_POINT('Ctrl Pts',(7.53291726078526,-21.2943588989331,
0.));
#191601=CARTESIAN_POINT('Ctrl Pts',(7.53436505309942,-21.2993464250717,
0.));
#191602=CARTESIAN_POINT('Ctrl Pts',(7.53587778251735,-21.3046368712157,
0.));
#191603=CARTESIAN_POINT('Ctrl Pts',(7.53745129364615,-21.310223716773,0.));
#191604=CARTESIAN_POINT('Ctrl Pts',(7.53908175169898,-21.3161009456256,
0.));
#191605=CARTESIAN_POINT('Ctrl Pts',(7.54076552038278,-21.3222628524165,
0.));
#191606=CARTESIAN_POINT('Ctrl Pts',(7.5424990037703,-21.328703791771,0.));
#191607=CARTESIAN_POINT('Ctrl Pts',(7.54427868151267,-21.3354182340149,
0.));
#191608=CARTESIAN_POINT('Ctrl Pts',(7.54610114948346,-21.3424008295038,
0.));
#191609=CARTESIAN_POINT('Ctrl Pts',(7.5479631624633,-21.3496464761531,0.));
#191610=CARTESIAN_POINT('Ctrl Pts',(7.54986166521309,-21.3571503685855,
0.));
#191611=CARTESIAN_POINT('Ctrl Pts',(7.55179375777443,-21.3649079431865,
0.));
#191612=CARTESIAN_POINT('Ctrl Pts',(7.55375667080028,-21.3729148390243,
0.));
#191613=CARTESIAN_POINT('Ctrl Pts',(7.55574773403502,-21.3811668478932,
0.));
#191614=CARTESIAN_POINT('Ctrl Pts',(7.55776435731416,-21.3896598842117,
0.));
#191615=CARTESIAN_POINT('Ctrl Pts',(7.5598040370061,-21.3983899952987,0.));
#191616=CARTESIAN_POINT('Ctrl Pts',(7.56186435703621,-21.4073533630365,
0.));
#191617=CARTESIAN_POINT('Ctrl Pts',(7.56394299313684,-21.4165463106254,
0.));
#191618=CARTESIAN_POINT('Ctrl Pts',(7.56603771218711,-21.4259653015736,
0.));
#191619=CARTESIAN_POINT('Ctrl Pts',(7.56814636360847,-21.4356069261513,
0.));
#191620=CARTESIAN_POINT('Ctrl Pts',(7.57026687261165,-21.4454678907509,
0.));
#191621=CARTESIAN_POINT('Ctrl Pts',(7.57239723223505,-21.4555450053142,
0.));
#191622=CARTESIAN_POINT('Ctrl Pts',(7.57453549743411,-21.4658351740128,
0.));
#191623=CARTESIAN_POINT('Ctrl Pts',(7.57667978402986,-21.4763353936762,
0.));
#191624=CARTESIAN_POINT('Ctrl Pts',(7.57882826679131,-21.4870427508194,
0.));
#191625=CARTESIAN_POINT('Ctrl Pts',(7.58097917790743,-21.4979544192744,
0.));
#191626=CARTESIAN_POINT('Ctrl Pts',(7.58313080519179,-21.5090676573873,
0.));
#191627=CARTESIAN_POINT('Ctrl Pts',(7.58528148919129,-21.5203798035299,
0.));
#191628=CARTESIAN_POINT('Ctrl Pts',(7.58742962034833,-21.5318882716736,
0.));
#191629=CARTESIAN_POINT('Ctrl Pts',(7.58957363620013,-21.543590547011,0.));
#191630=CARTESIAN_POINT('Ctrl Pts',(7.59171201844776,-21.5554841813462,
0.));
#191631=CARTESIAN_POINT('Ctrl Pts',(7.59384329124918,-21.5675667904726,
0.));
#191632=CARTESIAN_POINT('Ctrl Pts',(7.59596601973583,-21.5798360518978,
0.));
#191633=CARTESIAN_POINT('Ctrl Pts',(7.59807880846194,-21.5922897024466,
0.));
#191634=CARTESIAN_POINT('Ctrl Pts',(7.6001802998824,-21.6049255358843,0.));
#191635=CARTESIAN_POINT('Ctrl Pts',(7.60226917285428,-21.617741400599,0.));
#191636=CARTESIAN_POINT('Ctrl Pts',(7.60434414118295,-21.6307351973822,
0.));
#191637=CARTESIAN_POINT('Ctrl Pts',(7.60640395216356,-21.6439048771743,
0.));
#191638=CARTESIAN_POINT('Ctrl Pts',(7.60844738512873,-21.6572484388081,
0.));
#191639=CARTESIAN_POINT('Ctrl Pts',(7.61047325000955,-21.6707639267576,
0.));
#191640=CARTESIAN_POINT('Ctrl Pts',(7.61248038630268,-21.6844494295815,
0.));
#191641=CARTESIAN_POINT('Ctrl Pts',(7.61446766202786,-21.6983030783322,
0.));
#191642=CARTESIAN_POINT('Ctrl Pts',(7.6164339727042,-21.7123230449834,0.));
#191643=CARTESIAN_POINT('Ctrl Pts',(7.61837824030537,-21.7265075407975,
0.));
#191644=CARTESIAN_POINT('Ctrl Pts',(7.62029941230854,-21.7408548148656,
0.));
#191645=CARTESIAN_POINT('Ctrl Pts',(7.62219646084228,-21.7553631528328,
0.));
#191646=CARTESIAN_POINT('Ctrl Pts',(7.62406838181165,-21.7700308755584,
0.));
#191647=CARTESIAN_POINT('Ctrl Pts',(7.62591419404512,-21.7848563378021,
0.));
#191648=CARTESIAN_POINT('Ctrl Pts',(7.62773293842388,-21.799837926858,0.));
#191649=CARTESIAN_POINT('Ctrl Pts',(7.62952367718126,-21.814974061509,0.));
#191650=CARTESIAN_POINT('Ctrl Pts',(7.63128549323022,-21.8302631910195,
0.));
#191651=CARTESIAN_POINT('Ctrl Pts',(7.63301748948935,-21.8457037941084,
0.));
#191652=CARTESIAN_POINT('Ctrl Pts',(7.63471878821225,-21.8612943779089,
0.));
#191653=CARTESIAN_POINT('Ctrl Pts',(7.63638853033399,-21.8770334769496,
0.));
#191654=CARTESIAN_POINT('Ctrl Pts',(7.63802587492034,-21.8929196523514,
0.));
#191655=CARTESIAN_POINT('Ctrl Pts',(7.63962999860926,-21.9089514909874,
0.));
#191656=CARTESIAN_POINT('Ctrl Pts',(7.64120009506531,-21.9251276046546,
0.));
#191657=CARTESIAN_POINT('Ctrl Pts',(7.64273537442681,-21.9414466292072,
0.));
#191658=CARTESIAN_POINT('Ctrl Pts',(7.64423506279122,-21.9579072237651,
0.));
#191659=CARTESIAN_POINT('Ctrl Pts',(7.64569840177335,-21.9745080700798,
0.));
#191660=CARTESIAN_POINT('Ctrl Pts',(7.64712464805249,-21.9912478718542,
0.));
#191661=CARTESIAN_POINT('Ctrl Pts',(7.64851307293351,-22.0081253540774,
0.));
#191662=CARTESIAN_POINT('Ctrl Pts',(7.64986296190168,-22.0251392623209,
0.));
#191663=CARTESIAN_POINT('Ctrl Pts',(7.65117361421358,-22.0422883621174,
0.));
#191664=CARTESIAN_POINT('Ctrl Pts',(7.65244434253112,-22.0595714384431,
0.));
#191665=CARTESIAN_POINT('Ctrl Pts',(7.65367447254949,-22.0769872951596,
0.));
#191666=CARTESIAN_POINT('Ctrl Pts',(7.65486334263643,-22.094534754469,0.));
#191667=CARTESIAN_POINT('Ctrl Pts',(7.65601030346806,-22.1122126563329,
0.));
#191668=CARTESIAN_POINT('Ctrl Pts',(7.65711471769396,-22.1300198579675,
0.));
#191669=CARTESIAN_POINT('Ctrl Pts',(7.65817595963348,-22.1479552334211,
0.));
#191670=CARTESIAN_POINT('Ctrl Pts',(7.6591934149693,-22.1660176731178,0.));
#191671=CARTESIAN_POINT('Ctrl Pts',(7.66016648045004,-22.1842060834091,
0.));
#191672=CARTESIAN_POINT('Ctrl Pts',(7.6610945635927,-22.2025193860964,0.));
#191673=CARTESIAN_POINT('Ctrl Pts',(7.66197708240399,-22.2209565180085,
0.));
#191674=CARTESIAN_POINT('Ctrl Pts',(7.66281346512508,-22.2395164306547,
0.));
#191675=CARTESIAN_POINT('Ctrl Pts',(7.6636031499764,-22.258198089848,0.));
#191676=CARTESIAN_POINT('Ctrl Pts',(7.66434558490978,-22.2770004753335,
0.));
#191677=CARTESIAN_POINT('Ctrl Pts',(7.66504022736298,-22.2959225803937,
0.));
#191678=CARTESIAN_POINT('Ctrl Pts',(7.66568654402493,-22.314963411484,0.));
#191679=CARTESIAN_POINT('Ctrl Pts',(7.66628401061951,-22.3341219879469,
0.));
#191680=CARTESIAN_POINT('Ctrl Pts',(7.66683211169157,-22.3533973417021,
0.));
#191681=CARTESIAN_POINT('Ctrl Pts',(7.66733034039882,-22.372788516936,0.));
#191682=CARTESIAN_POINT('Ctrl Pts',(7.66777819830789,-22.3922945697773,
0.));
#191683=CARTESIAN_POINT('Ctrl Pts',(7.66817519519639,-22.4119145679758,
0.));
#191684=CARTESIAN_POINT('Ctrl Pts',(7.66852084886703,-22.4316475906603,
0.));
#191685=CARTESIAN_POINT('Ctrl Pts',(7.66881468496634,-22.4514927280855,
0.));
#191686=CARTESIAN_POINT('Ctrl Pts',(7.6690562368083,-22.47144908137,0.));
#191687=CARTESIAN_POINT('Ctrl Pts',(7.66924504520314,-22.4915157622312,
0.));
#191688=CARTESIAN_POINT('Ctrl Pts',(7.66938065829107,-22.5116918927032,
0.));
#191689=CARTESIAN_POINT('Ctrl Pts',(7.66946263138143,-22.53197660492,0.));
#191690=CARTESIAN_POINT('Ctrl Pts',(7.66949052679692,-22.5523690409116,
0.));
#191691=CARTESIAN_POINT('Ctrl Pts',(7.66946391372305,-22.5728683523831,
0.));
#191692=CARTESIAN_POINT('Ctrl Pts',(7.66938236806232,-22.5934737004953,
0.));
#191693=CARTESIAN_POINT('Ctrl Pts',(7.66924547229413,-22.6141842556243,
0.));
#191694=CARTESIAN_POINT('Ctrl Pts',(7.66905281533714,-22.6349991971541,
0.));
#191695=CARTESIAN_POINT('Ctrl Pts',(7.66880399241322,-22.6559177133127,
0.));
#191696=CARTESIAN_POINT('Ctrl Pts',(7.66849860491742,-22.6769390009885,
0.));
#191697=CARTESIAN_POINT('Ctrl Pts',(7.66813626029274,-22.6980622655446,
0.));
#191698=CARTESIAN_POINT('Ctrl Pts',(7.66771657191027,-22.7192867206245,
0.));
#191699=CARTESIAN_POINT('Ctrl Pts',(7.66723915895439,-22.7406115879513,
0.));
#191700=CARTESIAN_POINT('Ctrl Pts',(7.66670364630298,-22.7620360971843,
0.));
#191701=CARTESIAN_POINT('Ctrl Pts',(7.66610966441272,-22.7835594857699,
0.));
#191702=CARTESIAN_POINT('Ctrl Pts',(7.66545684920986,-22.8051809987833,
0.));
#191703=CARTESIAN_POINT('Ctrl Pts',(7.66474484198548,-22.8268998887678,
0.));
#191704=CARTESIAN_POINT('Ctrl Pts',(7.66397328929802,-22.848715415557,0.));
#191705=CARTESIAN_POINT('Ctrl Pts',(7.66314184287336,-22.8706268461283,
0.));
#191706=CARTESIAN_POINT('Ctrl Pts',(7.66225015950155,-22.8926334544883,
0.));
#191707=CARTESIAN_POINT('Ctrl Pts',(7.66129790094107,-22.9147345215421,
0.));
#191708=CARTESIAN_POINT('Ctrl Pts',(7.66028473382777,-22.9369293349593,
0.));
#191709=CARTESIAN_POINT('Ctrl Pts',(7.65921032958901,-22.959217189033,0.));
#191710=CARTESIAN_POINT('Ctrl Pts',(7.65807436436431,-22.9815973845296,
0.));
#191711=CARTESIAN_POINT('Ctrl Pts',(7.65687651891303,-23.0040692285814,
0.));
#191712=CARTESIAN_POINT('Ctrl Pts',(7.65561647852533,-23.0266320345787,
0.));
#191713=CARTESIAN_POINT('Ctrl Pts',(7.65429393293945,-23.0492851220528,
0.));
#191714=CARTESIAN_POINT('Ctrl Pts',(7.65290857626357,-23.072027816555,0.));
#191715=CARTESIAN_POINT('Ctrl Pts',(7.65146010690475,-23.094859449525,0.));
#191716=CARTESIAN_POINT('Ctrl Pts',(7.64994822749859,-23.1177793581679,
0.));
#191717=CARTESIAN_POINT('Ctrl Pts',(7.64837264482942,-23.1407868853819,
0.));
#191718=CARTESIAN_POINT('Ctrl Pts',(7.64673306975804,-23.1638813796694,
0.));
#191719=CARTESIAN_POINT('Ctrl Pts',(7.64502921715482,-23.1870621950452,
0.));
#191720=CARTESIAN_POINT('Ctrl Pts',(7.64326080583679,-23.2103286909398,
0.));
#191721=CARTESIAN_POINT('Ctrl Pts',(7.64142755851504,-23.2336802320912,
0.));
#191722=CARTESIAN_POINT('Ctrl Pts',(7.63952920172834,-23.2571161884488,
0.));
#191723=CARTESIAN_POINT('Ctrl Pts',(7.63756546576373,-23.2806359350855,
0.));
#191724=CARTESIAN_POINT('Ctrl Pts',(7.63553608458782,-23.3042388521022,
0.));
#191725=CARTESIAN_POINT('Ctrl Pts',(7.63344079578161,-23.3279243245241,
0.));
#191726=CARTESIAN_POINT('Ctrl Pts',(7.63127934048136,-23.3516917421972,
0.));
#191727=CARTESIAN_POINT('Ctrl Pts',(7.62905146332592,-23.3755404996636,
0.));
#191728=CARTESIAN_POINT('Ctrl Pts',(7.62675691240328,-23.399469996112,0.));
#191729=CARTESIAN_POINT('Ctrl Pts',(7.62439543920049,-23.4234796353542,
0.));
#191730=CARTESIAN_POINT('Ctrl Pts',(7.62196679855954,-23.4475688257854,
0.));
#191731=CARTESIAN_POINT('Ctrl Pts',(7.61947074863976,-23.4717369803438,
0.));
#191732=CARTESIAN_POINT('Ctrl Pts',(7.61690705088318,-23.4959835164609,
0.));
#191733=CARTESIAN_POINT('Ctrl Pts',(7.61427546999297,-23.5203078560129,
0.));
#191734=CARTESIAN_POINT('Ctrl Pts',(7.61157577385371,-23.544709425203,0.));
#191735=CARTESIAN_POINT('Ctrl Pts',(7.60880773344599,-23.5691876544244,
0.));
#191736=CARTESIAN_POINT('Ctrl Pts',(7.60597112277093,-23.5937419781245,
0.));
#191737=CARTESIAN_POINT('Ctrl Pts',(7.60306571877805,-23.6183718346576,
0.));
#191738=CARTESIAN_POINT('Ctrl Pts',(7.60009130130125,-23.6430766661418,
0.));
#191739=CARTESIAN_POINT('Ctrl Pts',(7.59704765299566,-23.6678559182875,
0.));
#191740=CARTESIAN_POINT('Ctrl Pts',(7.59393455934034,-23.6927090405066,
0.));
#191741=CARTESIAN_POINT('Ctrl Pts',(7.5907518086532,-23.7176354860457,0.));
#191742=CARTESIAN_POINT('Ctrl Pts',(7.58749919210825,-23.7426347121006,
0.));
#191743=CARTESIAN_POINT('Ctrl Pts',(7.5841765037627,-23.7677061799376,0.));
#191744=CARTESIAN_POINT('Ctrl Pts',(7.58078354058212,-23.7928493549908,
0.));
#191745=CARTESIAN_POINT('Ctrl Pts',(7.57732010249065,-23.8180637069976,
0.));
#191746=CARTESIAN_POINT('Ctrl Pts',(7.57378599219813,-23.8433487096132,
0.));
#191747=CARTESIAN_POINT('Ctrl Pts',(7.57018101500708,-23.8687038399595,
0.));
#191748=CARTESIAN_POINT('Ctrl Pts',(7.5665049786379,-23.8941285782002,0.));
#191749=CARTESIAN_POINT('Ctrl Pts',(7.56275769304772,-23.9196224070759,
0.));
#191750=CARTESIAN_POINT('Ctrl Pts',(7.55893897027679,-23.9451848115002,
0.));
#191751=CARTESIAN_POINT('Ctrl Pts',(7.55504862424807,-23.9708152779886,
0.));
#191752=CARTESIAN_POINT('Ctrl Pts',(7.55108647097431,-23.9965132953187,
0.));
#191753=CARTESIAN_POINT('Ctrl Pts',(7.54705232885894,-24.0222783554531,
0.));
#191754=CARTESIAN_POINT('Ctrl Pts',(7.54294601896127,-24.0481099543353,
0.));
#191755=CARTESIAN_POINT('Ctrl Pts',(7.53876736531004,-24.0740075927984,
0.));
#191756=CARTESIAN_POINT('Ctrl Pts',(7.53451619514658,-24.0999707772643,
0.));
#191757=CARTESIAN_POINT('Ctrl Pts',(7.53019233935536,-24.1259990209211,
0.));
#191758=CARTESIAN_POINT('Ctrl Pts',(7.52579563201478,-24.152091842537,0.));
#191759=CARTESIAN_POINT('Ctrl Pts',(7.52132590953862,-24.1782487641602,
0.));
#191760=CARTESIAN_POINT('Ctrl Pts',(7.51678300997997,-24.2044693092356,
0.));
#191761=CARTESIAN_POINT('Ctrl Pts',(7.51216677222198,-24.230753000389,0.));
#191762=CARTESIAN_POINT('Ctrl Pts',(7.50747703535114,-24.2570993577032,
0.));
#191763=CARTESIAN_POINT('Ctrl Pts',(7.50271363765098,-24.2835078958966,
0.));
#191764=CARTESIAN_POINT('Ctrl Pts',(7.49787641695358,-24.3099781253345,
0.));
#191765=CARTESIAN_POINT('Ctrl Pts',(7.49296521252329,-24.3365095573673,
0.));
#191766=CARTESIAN_POINT('Ctrl Pts',(7.48797986651827,-24.3631017084513,
0.));
#191767=CARTESIAN_POINT('Ctrl Pts',(7.48292022569253,-24.3897541049248,
0.));
#191768=CARTESIAN_POINT('Ctrl Pts',(7.47778614286572,-24.4164662871165,
0.));
#191769=CARTESIAN_POINT('Ctrl Pts',(7.47257747883318,-24.4432378146501,
0.));
#191770=CARTESIAN_POINT('Ctrl Pts',(7.46729410308922,-24.4700682684544,
0.));
#191771=CARTESIAN_POINT('Ctrl Pts',(7.46193588961641,-24.4969572391509,
0.));
#191772=CARTESIAN_POINT('Ctrl Pts',(7.45650271336044,-24.52390431731,0.));
#191773=CARTESIAN_POINT('Ctrl Pts',(7.45099444651295,-24.550909083158,0.));
#191774=CARTESIAN_POINT('Ctrl Pts',(7.44541095473162,-24.5779710960865,
0.));
#191775=CARTESIAN_POINT('Ctrl Pts',(7.43975209375374,-24.6050898852349,
0.));
#191776=CARTESIAN_POINT('Ctrl Pts',(7.4340177048922,-24.6322649369472,0.));
#191777=CARTESIAN_POINT('Ctrl Pts',(7.4282076215868,-24.659495712869,0.));
#191778=CARTESIAN_POINT('Ctrl Pts',(7.42232167765762,-24.6867816727118,
0.));
#191779=CARTESIAN_POINT('Ctrl Pts',(7.41635971481242,-24.7141222949988,
0.));
#191780=CARTESIAN_POINT('Ctrl Pts',(7.41032159082172,-24.7415170994754,
0.));
#191781=CARTESIAN_POINT('Ctrl Pts',(7.40420718661754,-24.7689656669005,
0.));
#191782=CARTESIAN_POINT('Ctrl Pts',(7.39801641583612,-24.7964676646518,
0.));
#191783=CARTESIAN_POINT('Ctrl Pts',(7.3917492258684,-24.8240228521042,0.));
#191784=CARTESIAN_POINT('Ctrl Pts',(7.38540558904945,-24.8516310625367,
0.));
#191785=CARTESIAN_POINT('Ctrl Pts',(7.37898549641609,-24.8792921911309,
0.));
#191786=CARTESIAN_POINT('Ctrl Pts',(7.37378825962717,-24.9014633826201,
0.));
#191787=CARTESIAN_POINT('Ctrl Pts',(7.36985593120695,-24.9181155530631,
0.));
#191788=CARTESIAN_POINT('Ctrl Pts',(7.36721909029059,-24.9292275670705,
0.));
#191789=CARTESIAN_POINT('Ctrl Pts',(7.36589684767343,-24.9347862158358,
0.));
#191790=CARTESIAN_POINT('',(7.36589684767343,-24.9347862158358,0.));
#191791=CARTESIAN_POINT('Origin',(1.68110656504246,-21.4341755315424,0.));
#191792=CARTESIAN_POINT('',(1.76341220531179,-22.4835757167854,0.));
#191793=CARTESIAN_POINT('',(1.76341220531179,-22.4835757167854,0.));
#191794=CARTESIAN_POINT('',(0.840553282521226,-10.7170877657712,0.));
#191795=CARTESIAN_POINT('Ctrl Pts',(6.08833931617698,-25.2771067246846,
0.));
#191796=CARTESIAN_POINT('Ctrl Pts',(6.08833931617698,-25.2771067246846,
12.));
#191797=CARTESIAN_POINT('Ctrl Pts',(6.08441489609824,-25.2729539149479,
0.));
#191798=CARTESIAN_POINT('Ctrl Pts',(6.08441489609824,-25.2729539149479,
12.));
#191799=CARTESIAN_POINT('Ctrl Pts',(6.07657531787577,-25.2646490489816,
0.));
#191800=CARTESIAN_POINT('Ctrl Pts',(6.07657531787577,-25.2646490489816,
12.));
#191801=CARTESIAN_POINT('Ctrl Pts',(6.06484373634696,-25.2521940105523,
0.));
#191802=CARTESIAN_POINT('Ctrl Pts',(6.06484373634696,-25.2521940105523,
12.));
#191803=CARTESIAN_POINT('Ctrl Pts',(6.04925720151412,-25.2355918138798,
0.));
#191804=CARTESIAN_POINT('Ctrl Pts',(6.04925720151412,-25.2355918138798,
12.));
#191805=CARTESIAN_POINT('Ctrl Pts',(6.02986667390187,-25.2148466201368,
0.));
#191806=CARTESIAN_POINT('Ctrl Pts',(6.02986667390187,-25.2148466201368,
12.));
#191807=CARTESIAN_POINT('Ctrl Pts',(6.0105688180476,-25.1941090269638,0.));
#191808=CARTESIAN_POINT('Ctrl Pts',(6.0105688180476,-25.1941090269638,12.));
#191809=CARTESIAN_POINT('Ctrl Pts',(5.99136367859838,-25.1733791296154,
0.));
#191810=CARTESIAN_POINT('Ctrl Pts',(5.99136367859838,-25.1733791296154,
12.));
#191811=CARTESIAN_POINT('Ctrl Pts',(5.97225131495636,-25.1526570863065,
0.));
#191812=CARTESIAN_POINT('Ctrl Pts',(5.97225131495636,-25.1526570863065,
12.));
#191813=CARTESIAN_POINT('Ctrl Pts',(5.95323180187347,-25.1319431317273,
0.));
#191814=CARTESIAN_POINT('Ctrl Pts',(5.95323180187347,-25.1319431317273,
12.));
#191815=CARTESIAN_POINT('Ctrl Pts',(5.93430523086776,-25.1112375971182,
0.));
#191816=CARTESIAN_POINT('Ctrl Pts',(5.93430523086776,-25.1112375971182,
12.));
#191817=CARTESIAN_POINT('Ctrl Pts',(5.91547170844382,-25.0905409050863,
0.));
#191818=CARTESIAN_POINT('Ctrl Pts',(5.91547170844382,-25.0905409050863,
12.));
#191819=CARTESIAN_POINT('Ctrl Pts',(5.89673135155458,-25.0698535426593,
0.));
#191820=CARTESIAN_POINT('Ctrl Pts',(5.89673135155458,-25.0698535426593,
12.));
#191821=CARTESIAN_POINT('Ctrl Pts',(5.87808428385329,-25.0491760405965,
0.));
#191822=CARTESIAN_POINT('Ctrl Pts',(5.87808428385329,-25.0491760405965,
12.));
#191823=CARTESIAN_POINT('Ctrl Pts',(5.8595306315681,-25.0285089498922,0.));
#191824=CARTESIAN_POINT('Ctrl Pts',(5.8595306315681,-25.0285089498922,12.));
#191825=CARTESIAN_POINT('Ctrl Pts',(5.84107051963073,-25.0078528200558,
0.));
#191826=CARTESIAN_POINT('Ctrl Pts',(5.84107051963073,-25.0078528200558,
12.));
#191827=CARTESIAN_POINT('Ctrl Pts',(5.82270406744213,-24.9872081752709,
0.));
#191828=CARTESIAN_POINT('Ctrl Pts',(5.82270406744213,-24.9872081752709,
12.));
#191829=CARTESIAN_POINT('Ctrl Pts',(5.80443138549747,-24.9665754954463,
0.));
#191830=CARTESIAN_POINT('Ctrl Pts',(5.80443138549747,-24.9665754954463,
12.));
#191831=CARTESIAN_POINT('Ctrl Pts',(5.78625257775702,-24.9459552293308,
0.));
#191832=CARTESIAN_POINT('Ctrl Pts',(5.78625257775702,-24.9459552293308,
12.));
#191833=CARTESIAN_POINT('Ctrl Pts',(5.76816774342236,-24.9253478043632,
0.));
#191834=CARTESIAN_POINT('Ctrl Pts',(5.76816774342236,-24.9253478043632,
12.));
#191835=CARTESIAN_POINT('Ctrl Pts',(5.75017697890812,-24.9047536376467,
0.));
#191836=CARTESIAN_POINT('Ctrl Pts',(5.75017697890812,-24.9047536376467,
12.));
#191837=CARTESIAN_POINT('Ctrl Pts',(5.73228037976926,-24.8841731467219,
0.));
#191838=CARTESIAN_POINT('Ctrl Pts',(5.73228037976926,-24.8841731467219,
12.));
#191839=CARTESIAN_POINT('Ctrl Pts',(5.71447804252019,-24.8636067597677,
0.));
#191840=CARTESIAN_POINT('Ctrl Pts',(5.71447804252019,-24.8636067597677,
12.));
#191841=CARTESIAN_POINT('Ctrl Pts',(5.69677006679429,-24.8430549277634,
0.));
#191842=CARTESIAN_POINT('Ctrl Pts',(5.69677006679429,-24.8430549277634,
12.));
#191843=CARTESIAN_POINT('Ctrl Pts',(5.67915655496524,-24.822518122386,0.));
#191844=CARTESIAN_POINT('Ctrl Pts',(5.67915655496524,-24.822518122386,12.));
#191845=CARTESIAN_POINT('Ctrl Pts',(5.66163761114903,-24.8019968304618,
0.));
#191846=CARTESIAN_POINT('Ctrl Pts',(5.66163761114903,-24.8019968304618,
12.));
#191847=CARTESIAN_POINT('Ctrl Pts',(5.64421334042247,-24.7814915496728,
0.));
#191848=CARTESIAN_POINT('Ctrl Pts',(5.64421334042247,-24.7814915496728,
12.));
#191849=CARTESIAN_POINT('Ctrl Pts',(5.62688384790918,-24.76100278357,0.));
#191850=CARTESIAN_POINT('Ctrl Pts',(5.62688384790918,-24.76100278357,12.));
#191851=CARTESIAN_POINT('Ctrl Pts',(5.60964923798494,-24.7405310372736,
0.));
#191852=CARTESIAN_POINT('Ctrl Pts',(5.60964923798494,-24.7405310372736,
12.));
#191853=CARTESIAN_POINT('Ctrl Pts',(5.59250961323995,-24.7200768119079,
0.));
#191854=CARTESIAN_POINT('Ctrl Pts',(5.59250961323995,-24.7200768119079,
12.));
#191855=CARTESIAN_POINT('Ctrl Pts',(5.57546507427766,-24.6996406035507,
0.));
#191856=CARTESIAN_POINT('Ctrl Pts',(5.57546507427766,-24.6996406035507,
12.));
#191857=CARTESIAN_POINT('Ctrl Pts',(5.55851572025389,-24.6792229061785,
0.));
#191858=CARTESIAN_POINT('Ctrl Pts',(5.55851572025389,-24.6792229061785,
12.));
#191859=CARTESIAN_POINT('Ctrl Pts',(5.54166164919592,-24.6588242134733,
0.));
#191860=CARTESIAN_POINT('Ctrl Pts',(5.54166164919592,-24.6588242134733,
12.));
#191861=CARTESIAN_POINT('Ctrl Pts',(5.52490295840996,-24.6384450211466,
0.));
#191862=CARTESIAN_POINT('Ctrl Pts',(5.52490295840996,-24.6384450211466,
12.));
#191863=CARTESIAN_POINT('Ctrl Pts',(5.50823974481959,-24.618085828918,0.));
#191864=CARTESIAN_POINT('Ctrl Pts',(5.50823974481959,-24.618085828918,12.));
#191865=CARTESIAN_POINT('Ctrl Pts',(5.49167210537235,-24.5977471429365,
0.));
#191866=CARTESIAN_POINT('Ctrl Pts',(5.49167210537235,-24.5977471429365,
12.));
#191867=CARTESIAN_POINT('Ctrl Pts',(5.47520013724403,-24.5774294770329,
0.));
#191868=CARTESIAN_POINT('Ctrl Pts',(5.47520013724403,-24.5774294770329,
12.));
#191869=CARTESIAN_POINT('Ctrl Pts',(5.45882393762244,-24.5571333514841,
0.));
#191870=CARTESIAN_POINT('Ctrl Pts',(5.45882393762244,-24.5571333514841,
12.));
#191871=CARTESIAN_POINT('Ctrl Pts',(5.44254360356865,-24.5368592922861,
0.));
#191872=CARTESIAN_POINT('Ctrl Pts',(5.44254360356865,-24.5368592922861,
12.));
#191873=CARTESIAN_POINT('Ctrl Pts',(5.42635923183411,-24.5166078302107,
0.));
#191874=CARTESIAN_POINT('Ctrl Pts',(5.42635923183411,-24.5166078302107,
12.));
#191875=CARTESIAN_POINT('Ctrl Pts',(5.41027091869242,-24.4963794999831,
0.));
#191876=CARTESIAN_POINT('Ctrl Pts',(5.41027091869242,-24.4963794999831,
12.));
#191877=CARTESIAN_POINT('Ctrl Pts',(5.3942787597383,-24.4761748393322,0.));
#191878=CARTESIAN_POINT('Ctrl Pts',(5.3942787597383,-24.4761748393322,12.));
#191879=CARTESIAN_POINT('Ctrl Pts',(5.37838284973706,-24.4559943883159,
0.));
#191880=CARTESIAN_POINT('Ctrl Pts',(5.37838284973706,-24.4559943883159,
12.));
#191881=CARTESIAN_POINT('Ctrl Pts',(5.36258328273639,-24.4358386899152,
0.));
#191882=CARTESIAN_POINT('Ctrl Pts',(5.36258328273639,-24.4358386899152,
12.));
#191883=CARTESIAN_POINT('Ctrl Pts',(5.34688015213546,-24.4157082904615,
0.));
#191884=CARTESIAN_POINT('Ctrl Pts',(5.34688015213546,-24.4157082904615,
12.));
#191885=CARTESIAN_POINT('Ctrl Pts',(5.33127355076036,-24.3956037401293,
0.));
#191886=CARTESIAN_POINT('Ctrl Pts',(5.33127355076036,-24.3956037401293,
12.));
#191887=CARTESIAN_POINT('Ctrl Pts',(5.31576357092524,-24.3755255933917,
0.));
#191888=CARTESIAN_POINT('Ctrl Pts',(5.31576357092524,-24.3755255933917,
12.));
#191889=CARTESIAN_POINT('Ctrl Pts',(5.30035030449058,-24.3554744095075,
0.));
#191890=CARTESIAN_POINT('Ctrl Pts',(5.30035030449058,-24.3554744095075,
12.));
#191891=CARTESIAN_POINT('Ctrl Pts',(5.28503384290644,-24.3354507529415,
0.));
#191892=CARTESIAN_POINT('Ctrl Pts',(5.28503384290644,-24.3354507529415,
12.));
#191893=CARTESIAN_POINT('Ctrl Pts',(5.26981427718796,-24.3154551932222,
0.));
#191894=CARTESIAN_POINT('Ctrl Pts',(5.26981427718796,-24.3154551932222,
12.));
#191895=CARTESIAN_POINT('Ctrl Pts',(5.25469169788855,-24.2954883048448,
0.));
#191896=CARTESIAN_POINT('Ctrl Pts',(5.25469169788855,-24.2954883048448,
12.));
#191897=CARTESIAN_POINT('Ctrl Pts',(5.23966619506289,-24.2755506671526,
0.));
#191898=CARTESIAN_POINT('Ctrl Pts',(5.23966619506289,-24.2755506671526,
12.));
#191899=CARTESIAN_POINT('Ctrl Pts',(5.22473785822441,-24.2556428642294,
0.));
#191900=CARTESIAN_POINT('Ctrl Pts',(5.22473785822441,-24.2556428642294,
12.));
#191901=CARTESIAN_POINT('Ctrl Pts',(5.20990677629173,-24.2357654847765,
0.));
#191902=CARTESIAN_POINT('Ctrl Pts',(5.20990677629173,-24.2357654847765,
12.));
#191903=CARTESIAN_POINT('Ctrl Pts',(5.19517303753642,-24.215919122017,0.));
#191904=CARTESIAN_POINT('Ctrl Pts',(5.19517303753642,-24.215919122017,12.));
#191905=CARTESIAN_POINT('Ctrl Pts',(5.18053672961392,-24.1961043738754,
0.));
#191906=CARTESIAN_POINT('Ctrl Pts',(5.18053672961392,-24.1961043738754,
12.));
#191907=CARTESIAN_POINT('Ctrl Pts',(5.16599793957979,-24.1763218431343,
0.));
#191908=CARTESIAN_POINT('Ctrl Pts',(5.16599793957979,-24.1763218431343,
12.));
#191909=CARTESIAN_POINT('Ctrl Pts',(5.15155675390075,-24.1565721375971,
0.));
#191910=CARTESIAN_POINT('Ctrl Pts',(5.15155675390075,-24.1565721375971,
12.));
#191911=CARTESIAN_POINT('Ctrl Pts',(5.13721325845744,-24.1368558702443,
0.));
#191912=CARTESIAN_POINT('Ctrl Pts',(5.13721325845744,-24.1368558702443,
12.));
#191913=CARTESIAN_POINT('Ctrl Pts',(5.12296753853859,-24.117173659394,0.));
#191914=CARTESIAN_POINT('Ctrl Pts',(5.12296753853859,-24.117173659394,12.));
#191915=CARTESIAN_POINT('Ctrl Pts',(5.10881967883132,-24.0975261288446,
0.));
#191916=CARTESIAN_POINT('Ctrl Pts',(5.10881967883132,-24.0975261288446,
12.));
#191917=CARTESIAN_POINT('Ctrl Pts',(5.09476976342625,-24.0779139079266,
0.));
#191918=CARTESIAN_POINT('Ctrl Pts',(5.09476976342625,-24.0779139079266,
12.));
#191919=CARTESIAN_POINT('Ctrl Pts',(5.08081787581276,-24.0583376315638,
0.));
#191920=CARTESIAN_POINT('Ctrl Pts',(5.08081787581276,-24.0583376315638,
12.));
#191921=CARTESIAN_POINT('Ctrl Pts',(5.06696409886641,-24.0387979403268,
0.));
#191922=CARTESIAN_POINT('Ctrl Pts',(5.06696409886641,-24.0387979403268,
12.));
#191923=CARTESIAN_POINT('Ctrl Pts',(5.05320851483065,-24.0192954804896,
0.));
#191924=CARTESIAN_POINT('Ctrl Pts',(5.05320851483065,-24.0192954804896,
12.));
#191925=CARTESIAN_POINT('Ctrl Pts',(5.03955120528521,-23.9998309040746,
0.));
#191926=CARTESIAN_POINT('Ctrl Pts',(5.03955120528521,-23.9998309040746,
12.));
#191927=CARTESIAN_POINT('Ctrl Pts',(5.02599225112454,-23.9804048689227,
0.));
#191928=CARTESIAN_POINT('Ctrl Pts',(5.02599225112454,-23.9804048689227,
12.));
#191929=CARTESIAN_POINT('Ctrl Pts',(5.01253173257452,-23.9610180388271,
0.));
#191930=CARTESIAN_POINT('Ctrl Pts',(5.01253173257452,-23.9610180388271,
12.));
#191931=CARTESIAN_POINT('Ctrl Pts',(4.99916972919306,-23.9416710836529,
0.));
#191932=CARTESIAN_POINT('Ctrl Pts',(4.99916972919306,-23.9416710836529,
12.));
#191933=CARTESIAN_POINT('Ctrl Pts',(4.98590631986532,-23.9223646794592,
0.));
#191934=CARTESIAN_POINT('Ctrl Pts',(4.98590631986532,-23.9223646794592,
12.));
#191935=CARTESIAN_POINT('Ctrl Pts',(4.97274158279226,-23.9030995086163,
0.));
#191936=CARTESIAN_POINT('Ctrl Pts',(4.97274158279226,-23.9030995086163,
12.));
#191937=CARTESIAN_POINT('Ctrl Pts',(4.9596755954656,-23.8838762599218,0.));
#191938=CARTESIAN_POINT('Ctrl Pts',(4.9596755954656,-23.8838762599218,12.));
#191939=CARTESIAN_POINT('Ctrl Pts',(4.9467084346586,-23.8646956287168,0.));
#191940=CARTESIAN_POINT('Ctrl Pts',(4.9467084346586,-23.8646956287168,12.));
#191941=CARTESIAN_POINT('Ctrl Pts',(4.93384017643432,-23.8455583170057,
0.));
#191942=CARTESIAN_POINT('Ctrl Pts',(4.93384017643432,-23.8455583170057,
12.));
#191943=CARTESIAN_POINT('Ctrl Pts',(4.92107089613968,-23.8264650335717,
0.));
#191944=CARTESIAN_POINT('Ctrl Pts',(4.92107089613968,-23.8264650335717,
12.));
#191945=CARTESIAN_POINT('Ctrl Pts',(4.90840066839344,-23.8074164940896,
0.));
#191946=CARTESIAN_POINT('Ctrl Pts',(4.90840066839344,-23.8074164940896,
12.));
#191947=CARTESIAN_POINT('Ctrl Pts',(4.89582956706775,-23.7884134212384,
0.));
#191948=CARTESIAN_POINT('Ctrl Pts',(4.89582956706775,-23.7884134212384,
12.));
#191949=CARTESIAN_POINT('Ctrl Pts',(4.88335766525573,-23.7694565448049,
0.));
#191950=CARTESIAN_POINT('Ctrl Pts',(4.88335766525573,-23.7694565448049,
12.));
#191951=CARTESIAN_POINT('Ctrl Pts',(4.87098503527152,-23.7505466018245,
0.));
#191952=CARTESIAN_POINT('Ctrl Pts',(4.87098503527152,-23.7505466018245,
12.));
#191953=CARTESIAN_POINT('Ctrl Pts',(4.85871174865499,-23.7316843367313,
0.));
#191954=CARTESIAN_POINT('Ctrl Pts',(4.85871174865499,-23.7316843367313,
12.));
#191955=CARTESIAN_POINT('Ctrl Pts',(4.84653787616425,-23.7128705015017,
0.));
#191956=CARTESIAN_POINT('Ctrl Pts',(4.84653787616425,-23.7128705015017,
12.));
#191957=CARTESIAN_POINT('Ctrl Pts',(4.83446348776265,-23.6941058557971,
0.));
#191958=CARTESIAN_POINT('Ctrl Pts',(4.83446348776265,-23.6941058557971,
12.));
#191959=CARTESIAN_POINT('Ctrl Pts',(4.82248865259562,-23.675391167102,0.));
#191960=CARTESIAN_POINT('Ctrl Pts',(4.82248865259562,-23.675391167102,12.));
#191961=CARTESIAN_POINT('Ctrl Pts',(4.81061343896432,-23.6567272108628,
0.));
#191962=CARTESIAN_POINT('Ctrl Pts',(4.81061343896432,-23.6567272108628,
12.));
#191963=CARTESIAN_POINT('Ctrl Pts',(4.7988379143322,-23.6381147706579,0.));
#191964=CARTESIAN_POINT('Ctrl Pts',(4.7988379143322,-23.6381147706579,12.));
#191965=CARTESIAN_POINT('Ctrl Pts',(4.78716214532097,-23.6195546383624,
0.));
#191966=CARTESIAN_POINT('Ctrl Pts',(4.78716214532097,-23.6195546383624,
12.));
#191967=CARTESIAN_POINT('Ctrl Pts',(4.77558619769872,-23.6010476143099,
0.));
#191968=CARTESIAN_POINT('Ctrl Pts',(4.77558619769872,-23.6010476143099,
12.));
#191969=CARTESIAN_POINT('Ctrl Pts',(4.76411013636251,-23.5825945074535,
0.));
#191970=CARTESIAN_POINT('Ctrl Pts',(4.76411013636251,-23.5825945074535,
12.));
#191971=CARTESIAN_POINT('Ctrl Pts',(4.75273402530617,-23.5641961355168,
0.));
#191972=CARTESIAN_POINT('Ctrl Pts',(4.75273402530617,-23.5641961355168,
12.));
#191973=CARTESIAN_POINT('Ctrl Pts',(4.74145792760698,-23.545853325171,0.));
#191974=CARTESIAN_POINT('Ctrl Pts',(4.74145792760698,-23.545853325171,12.));
#191975=CARTESIAN_POINT('Ctrl Pts',(4.73028190543029,-23.5275669122372,
0.));
#191976=CARTESIAN_POINT('Ctrl Pts',(4.73028190543029,-23.5275669122372,
12.));
#191977=CARTESIAN_POINT('Ctrl Pts',(4.71920602001901,-23.509337741878,0.));
#191978=CARTESIAN_POINT('Ctrl Pts',(4.71920602001901,-23.509337741878,12.));
#191979=CARTESIAN_POINT('Ctrl Pts',(4.70823033167818,-23.491166668789,0.));
#191980=CARTESIAN_POINT('Ctrl Pts',(4.70823033167818,-23.491166668789,12.));
#191981=CARTESIAN_POINT('Ctrl Pts',(4.69735489975024,-23.4730545573853,
0.));
#191982=CARTESIAN_POINT('Ctrl Pts',(4.69735489975024,-23.4730545573853,
12.));
#191983=CARTESIAN_POINT('Ctrl Pts',(4.68657978258303,-23.455002281986,0.));
#191984=CARTESIAN_POINT('Ctrl Pts',(4.68657978258303,-23.455002281986,12.));
#191985=CARTESIAN_POINT('Ctrl Pts',(4.67590503753058,-23.4370107270451,
0.));
#191986=CARTESIAN_POINT('Ctrl Pts',(4.67590503753058,-23.4370107270451,
12.));
#191987=CARTESIAN_POINT('Ctrl Pts',(4.6653307209467,-23.4190807873803,0.));
#191988=CARTESIAN_POINT('Ctrl Pts',(4.6653307209467,-23.4190807873803,12.));
#191989=CARTESIAN_POINT('Ctrl Pts',(4.65485688816924,-23.4012133683959,
0.));
#191990=CARTESIAN_POINT('Ctrl Pts',(4.65485688816924,-23.4012133683959,
12.));
#191991=CARTESIAN_POINT('Ctrl Pts',(4.6444835934993,-23.3834093863068,0.));
#191992=CARTESIAN_POINT('Ctrl Pts',(4.6444835934993,-23.3834093863068,12.));
#191993=CARTESIAN_POINT('Ctrl Pts',(4.63421089016541,-23.3656697683489,
0.));
#191994=CARTESIAN_POINT('Ctrl Pts',(4.63421089016541,-23.3656697683489,
12.));
#191995=CARTESIAN_POINT('Ctrl Pts',(4.62403883030805,-23.3479954530272,
0.));
#191996=CARTESIAN_POINT('Ctrl Pts',(4.62403883030805,-23.3479954530272,
12.));
#191997=CARTESIAN_POINT('Ctrl Pts',(4.6139674649783,-23.3303873903938,0.));
#191998=CARTESIAN_POINT('Ctrl Pts',(4.6139674649783,-23.3303873903938,12.));
#191999=CARTESIAN_POINT('Ctrl Pts',(4.60399684412163,-23.3128465423115,
0.));
#192000=CARTESIAN_POINT('Ctrl Pts',(4.60399684412163,-23.3128465423115,
12.));
#192001=CARTESIAN_POINT('Ctrl Pts',(4.5941270165575,-23.2953738827191,0.));
#192002=CARTESIAN_POINT('Ctrl Pts',(4.5941270165575,-23.2953738827191,12.));
#192003=CARTESIAN_POINT('Ctrl Pts',(4.5843580299469,-23.2779703978876,0.));
#192004=CARTESIAN_POINT('Ctrl Pts',(4.5843580299469,-23.2779703978876,12.));
#192005=CARTESIAN_POINT('Ctrl Pts',(4.57468993076097,-23.2606370866866,
0.));
#192006=CARTESIAN_POINT('Ctrl Pts',(4.57468993076097,-23.2606370866866,
12.));
#192007=CARTESIAN_POINT('Ctrl Pts',(4.56512276427839,-23.2433749609131,
0.));
#192008=CARTESIAN_POINT('Ctrl Pts',(4.56512276427839,-23.2433749609131,
12.));
#192009=CARTESIAN_POINT('Ctrl Pts',(4.55565657456975,-23.2261850456064,
0.));
#192010=CARTESIAN_POINT('Ctrl Pts',(4.55565657456975,-23.2261850456064,
12.));
#192011=CARTESIAN_POINT('Ctrl Pts',(4.54629140447544,-23.2090683793629,
0.));
#192012=CARTESIAN_POINT('Ctrl Pts',(4.54629140447544,-23.2090683793629,
12.));
#192013=CARTESIAN_POINT('Ctrl Pts',(4.53702729557566,-23.1920260146465,
0.));
#192014=CARTESIAN_POINT('Ctrl Pts',(4.53702729557566,-23.1920260146465,
12.));
#192015=CARTESIAN_POINT('Ctrl Pts',(4.52786428815014,-23.1750590180908,
0.));
#192016=CARTESIAN_POINT('Ctrl Pts',(4.52786428815014,-23.1750590180908,
12.));
#192017=CARTESIAN_POINT('Ctrl Pts',(4.51880242116748,-23.1581684708761,
0.));
#192018=CARTESIAN_POINT('Ctrl Pts',(4.51880242116748,-23.1581684708761,
12.));
#192019=CARTESIAN_POINT('Ctrl Pts',(4.5098417322706,-23.1413554691123,0.));
#192020=CARTESIAN_POINT('Ctrl Pts',(4.5098417322706,-23.1413554691123,12.));
#192021=CARTESIAN_POINT('Ctrl Pts',(4.50098225775171,-23.1246211242115,
0.));
#192022=CARTESIAN_POINT('Ctrl Pts',(4.50098225775171,-23.1246211242115,
12.));
#192023=CARTESIAN_POINT('Ctrl Pts',(4.49222403252216,-23.1079665632636,
0.));
#192024=CARTESIAN_POINT('Ctrl Pts',(4.49222403252216,-23.1079665632636,
12.));
#192025=CARTESIAN_POINT('Ctrl Pts',(4.48356709006788,-23.0913929293922,
0.));
#192026=CARTESIAN_POINT('Ctrl Pts',(4.48356709006788,-23.0913929293922,
12.));
#192027=CARTESIAN_POINT('Ctrl Pts',(4.47501146242856,-23.0749013821881,
0.));
#192028=CARTESIAN_POINT('Ctrl Pts',(4.47501146242856,-23.0749013821881,
12.));
#192029=CARTESIAN_POINT('Ctrl Pts',(4.4665571801823,-23.0584930981732,0.));
#192030=CARTESIAN_POINT('Ctrl Pts',(4.4665571801823,-23.0584930981732,12.));
#192031=CARTESIAN_POINT('Ctrl Pts',(4.45820427241683,-23.0421692712467,
0.));
#192032=CARTESIAN_POINT('Ctrl Pts',(4.45820427241683,-23.0421692712467,
12.));
#192033=CARTESIAN_POINT('Ctrl Pts',(4.44995276669686,-23.0259311131392,
0.));
#192034=CARTESIAN_POINT('Ctrl Pts',(4.44995276669686,-23.0259311131392,
12.));
#192035=CARTESIAN_POINT('Ctrl Pts',(4.44180268901643,-23.0097798538395,
0.));
#192036=CARTESIAN_POINT('Ctrl Pts',(4.44180268901643,-23.0097798538395,
12.));
#192037=CARTESIAN_POINT('Ctrl Pts',(4.43375406376879,-22.9937167421006,
0.));
#192038=CARTESIAN_POINT('Ctrl Pts',(4.43375406376879,-22.9937167421006,
12.));
#192039=CARTESIAN_POINT('Ctrl Pts',(4.42580691372751,-22.977743046002,0.));
#192040=CARTESIAN_POINT('Ctrl Pts',(4.42580691372751,-22.977743046002,12.));
#192041=CARTESIAN_POINT('Ctrl Pts',(4.41796126001302,-22.9618600534866,
0.));
#192042=CARTESIAN_POINT('Ctrl Pts',(4.41796126001302,-22.9618600534866,
12.));
#192043=CARTESIAN_POINT('Ctrl Pts',(4.41021712205553,-22.9460690729093,
0.));
#192044=CARTESIAN_POINT('Ctrl Pts',(4.41021712205553,-22.9460690729093,
12.));
#192045=CARTESIAN_POINT('Ctrl Pts',(4.40257451754323,-22.930371433555,0.));
#192046=CARTESIAN_POINT('Ctrl Pts',(4.40257451754323,-22.930371433555,12.));
#192047=CARTESIAN_POINT('Ctrl Pts',(4.39503346238473,-22.9147684862426,
0.));
#192048=CARTESIAN_POINT('Ctrl Pts',(4.39503346238473,-22.9147684862426,
12.));
#192049=CARTESIAN_POINT('Ctrl Pts',(4.38759397068405,-22.8992616040108,
0.));
#192050=CARTESIAN_POINT('Ctrl Pts',(4.38759397068405,-22.8992616040108,
12.));
#192051=CARTESIAN_POINT('Ctrl Pts',(4.38025605470092,-22.8838521827701,
0.));
#192052=CARTESIAN_POINT('Ctrl Pts',(4.38025605470092,-22.8838521827701,
12.));
#192053=CARTESIAN_POINT('Ctrl Pts',(4.37301972480745,-22.8685416419725,
0.));
#192054=CARTESIAN_POINT('Ctrl Pts',(4.37301972480745,-22.8685416419725,
12.));
#192055=CARTESIAN_POINT('Ctrl Pts',(4.36588498942997,-22.8533314252422,
0.));
#192056=CARTESIAN_POINT('Ctrl Pts',(4.36588498942997,-22.8533314252422,
12.));
#192057=CARTESIAN_POINT('Ctrl Pts',(4.35885185500546,-22.8382230011184,
0.));
#192058=CARTESIAN_POINT('Ctrl Pts',(4.35885185500546,-22.8382230011184,
12.));
#192059=CARTESIAN_POINT('Ctrl Pts',(4.3519203259479,-22.8232178638876,0.));
#192060=CARTESIAN_POINT('Ctrl Pts',(4.3519203259479,-22.8232178638876,12.));
#192061=CARTESIAN_POINT('Ctrl Pts',(4.34509040460062,-22.8083175343791,
0.));
#192062=CARTESIAN_POINT('Ctrl Pts',(4.34509040460062,-22.8083175343791,
12.));
#192063=CARTESIAN_POINT('Ctrl Pts',(4.33836209118446,-22.7935235607806,
0.));
#192064=CARTESIAN_POINT('Ctrl Pts',(4.33836209118446,-22.7935235607806,
12.));
#192065=CARTESIAN_POINT('Ctrl Pts',(4.33173538373189,-22.7788375194076,
0.));
#192066=CARTESIAN_POINT('Ctrl Pts',(4.33173538373189,-22.7788375194076,
12.));
#192067=CARTESIAN_POINT('Ctrl Pts',(4.32521027803754,-22.7642610156475,
0.));
#192068=CARTESIAN_POINT('Ctrl Pts',(4.32521027803754,-22.7642610156475,
12.));
#192069=CARTESIAN_POINT('Ctrl Pts',(4.31878676761235,-22.7497956849848,
0.));
#192070=CARTESIAN_POINT('Ctrl Pts',(4.31878676761235,-22.7497956849848,
12.));
#192071=CARTESIAN_POINT('Ctrl Pts',(4.31246484362549,-22.7354431939926,
0.));
#192072=CARTESIAN_POINT('Ctrl Pts',(4.31246484362549,-22.7354431939926,
12.));
#192073=CARTESIAN_POINT('Ctrl Pts',(4.30624449484069,-22.7212052413386,
0.));
#192074=CARTESIAN_POINT('Ctrl Pts',(4.30624449484069,-22.7212052413386,
12.));
#192075=CARTESIAN_POINT('Ctrl Pts',(4.3001257075406,-22.7070835587564,0.));
#192076=CARTESIAN_POINT('Ctrl Pts',(4.3001257075406,-22.7070835587564,12.));
#192077=CARTESIAN_POINT('Ctrl Pts',(4.29410846547056,-22.6930799122548,
0.));
#192078=CARTESIAN_POINT('Ctrl Pts',(4.29410846547056,-22.6930799122548,
12.));
#192079=CARTESIAN_POINT('Ctrl Pts',(4.28819274977763,-22.6791961033538,
0.));
#192080=CARTESIAN_POINT('Ctrl Pts',(4.28819274977763,-22.6791961033538,
12.));
#192081=CARTESIAN_POINT('Ctrl Pts',(4.28237853894058,-22.6654339703109,
0.));
#192082=CARTESIAN_POINT('Ctrl Pts',(4.28237853894058,-22.6654339703109,
12.));
#192083=CARTESIAN_POINT('Ctrl Pts',(4.2766658086912,-22.6517953893303,0.));
#192084=CARTESIAN_POINT('Ctrl Pts',(4.2766658086912,-22.6517953893303,12.));
#192085=CARTESIAN_POINT('Ctrl Pts',(4.27105453193004,-22.6382822758172,
0.));
#192086=CARTESIAN_POINT('Ctrl Pts',(4.27105453193004,-22.6382822758172,
12.));
#192087=CARTESIAN_POINT('Ctrl Pts',(4.26554467865576,-22.6248965859977,
0.));
#192088=CARTESIAN_POINT('Ctrl Pts',(4.26554467865576,-22.6248965859977,
12.));
#192089=CARTESIAN_POINT('Ctrl Pts',(4.26013621588305,-22.6116403184821,
0.));
#192090=CARTESIAN_POINT('Ctrl Pts',(4.26013621588305,-22.6116403184821,
12.));
#192091=CARTESIAN_POINT('Ctrl Pts',(4.25482910755481,-22.5985155158636,
0.));
#192092=CARTESIAN_POINT('Ctrl Pts',(4.25482910755481,-22.5985155158636,
12.));
#192093=CARTESIAN_POINT('Ctrl Pts',(4.24962331444177,-22.5855242662477,
0.));
#192094=CARTESIAN_POINT('Ctrl Pts',(4.24962331444177,-22.5855242662477,
12.));
#192095=CARTESIAN_POINT('Ctrl Pts',(4.24451879404851,-22.572668704992,0.));
#192096=CARTESIAN_POINT('Ctrl Pts',(4.24451879404851,-22.572668704992,12.));
#192097=CARTESIAN_POINT('Ctrl Pts',(4.23951550052522,-22.5599510166429,
0.));
#192098=CARTESIAN_POINT('Ctrl Pts',(4.23951550052522,-22.5599510166429,
12.));
#192099=CARTESIAN_POINT('Ctrl Pts',(4.23461338456712,-22.5473734368086,
0.));
#192100=CARTESIAN_POINT('Ctrl Pts',(4.23461338456712,-22.5473734368086,
12.));
#192101=CARTESIAN_POINT('Ctrl Pts',(4.22981239330733,-22.5349382540588,
0.));
#192102=CARTESIAN_POINT('Ctrl Pts',(4.22981239330733,-22.5349382540588,
12.));
#192103=CARTESIAN_POINT('Ctrl Pts',(4.22511247020041,-22.5226478117886,
0.));
#192104=CARTESIAN_POINT('Ctrl Pts',(4.22511247020041,-22.5226478117886,
12.));
#192105=CARTESIAN_POINT('Ctrl Pts',(4.22051355490196,-22.5105045108881,
0.));
#192106=CARTESIAN_POINT('Ctrl Pts',(4.22051355490196,-22.5105045108881,
12.));
#192107=CARTESIAN_POINT('Ctrl Pts',(4.21601558313906,-22.4985108124228,
0.));
#192108=CARTESIAN_POINT('Ctrl Pts',(4.21601558313906,-22.4985108124228,
12.));
#192109=CARTESIAN_POINT('Ctrl Pts',(4.21161848657428,-22.4866692403147,
0.));
#192110=CARTESIAN_POINT('Ctrl Pts',(4.21161848657428,-22.4866692403147,
12.));
#192111=CARTESIAN_POINT('Ctrl Pts',(4.20732219265648,-22.4749823839917,
0.));
#192112=CARTESIAN_POINT('Ctrl Pts',(4.20732219265648,-22.4749823839917,
12.));
#192113=CARTESIAN_POINT('Ctrl Pts',(4.20312662448174,-22.4634529011437,
0.));
#192114=CARTESIAN_POINT('Ctrl Pts',(4.20312662448174,-22.4634529011437,
12.));
#192115=CARTESIAN_POINT('Ctrl Pts',(4.19903170066358,-22.4520835205422,
0.));
#192116=CARTESIAN_POINT('Ctrl Pts',(4.19903170066358,-22.4520835205422,
12.));
#192117=CARTESIAN_POINT('Ctrl Pts',(4.1950373351886,-22.4408770448917,0.));
#192118=CARTESIAN_POINT('Ctrl Pts',(4.1950373351886,-22.4408770448917,12.));
#192119=CARTESIAN_POINT('Ctrl Pts',(4.19114343726932,-22.4298363535416,
0.));
#192120=CARTESIAN_POINT('Ctrl Pts',(4.19114343726932,-22.4298363535416,
12.));
#192121=CARTESIAN_POINT('Ctrl Pts',(4.18734991117707,-22.4189644056109,
0.));
#192122=CARTESIAN_POINT('Ctrl Pts',(4.18734991117707,-22.4189644056109,
12.));
#192123=CARTESIAN_POINT('Ctrl Pts',(4.18365665600839,-22.4082642454448,
0.));
#192124=CARTESIAN_POINT('Ctrl Pts',(4.18365665600839,-22.4082642454448,
12.));
#192125=CARTESIAN_POINT('Ctrl Pts',(4.18006356544879,-22.3977390078074,
0.));
#192126=CARTESIAN_POINT('Ctrl Pts',(4.18006356544879,-22.3977390078074,
12.));
#192127=CARTESIAN_POINT('Ctrl Pts',(4.17657052752834,-22.3873919231339,
0.));
#192128=CARTESIAN_POINT('Ctrl Pts',(4.17657052752834,-22.3873919231339,
12.));
#192129=CARTESIAN_POINT('Ctrl Pts',(4.17317742436162,-22.3772263228624,
0.));
#192130=CARTESIAN_POINT('Ctrl Pts',(4.17317742436162,-22.3772263228624,
12.));
#192131=CARTESIAN_POINT('Ctrl Pts',(4.16988413199469,-22.3672456427605,
0.));
#192132=CARTESIAN_POINT('Ctrl Pts',(4.16988413199469,-22.3672456427605,
12.));
#192133=CARTESIAN_POINT('Ctrl Pts',(4.16669052026602,-22.3574534257397,
0.));
#192134=CARTESIAN_POINT('Ctrl Pts',(4.16669052026602,-22.3574534257397,
12.));
#192135=CARTESIAN_POINT('Ctrl Pts',(4.1635964526318,-22.3478533253886,0.));
#192136=CARTESIAN_POINT('Ctrl Pts',(4.1635964526318,-22.3478533253886,12.));
#192137=CARTESIAN_POINT('Ctrl Pts',(4.16060178604153,-22.3384491078599,
0.));
#192138=CARTESIAN_POINT('Ctrl Pts',(4.16060178604153,-22.3384491078599,
12.));
#192139=CARTESIAN_POINT('Ctrl Pts',(4.15770637047882,-22.3292446628957,
0.));
#192140=CARTESIAN_POINT('Ctrl Pts',(4.15770637047882,-22.3292446628957,
12.));
#192141=CARTESIAN_POINT('Ctrl Pts',(4.15491004835278,-22.3202440186979,
0.));
#192142=CARTESIAN_POINT('Ctrl Pts',(4.15491004835278,-22.3202440186979,
12.));
#192143=CARTESIAN_POINT('Ctrl Pts',(4.15221265396992,-22.3114513545186,
0.));
#192144=CARTESIAN_POINT('Ctrl Pts',(4.15221265396992,-22.3114513545186,
12.));
#192145=CARTESIAN_POINT('Ctrl Pts',(4.14961401285525,-22.3028710166935,
0.));
#192146=CARTESIAN_POINT('Ctrl Pts',(4.14961401285525,-22.3028710166935,
12.));
#192147=CARTESIAN_POINT('Ctrl Pts',(4.14711394168559,-22.2945075198468,
0.));
#192148=CARTESIAN_POINT('Ctrl Pts',(4.14711394168559,-22.2945075198468,
12.));
#192149=CARTESIAN_POINT('Ctrl Pts',(4.14471224859295,-22.2863655389167,
0.));
#192150=CARTESIAN_POINT('Ctrl Pts',(4.14471224859295,-22.2863655389167,
12.));
#192151=CARTESIAN_POINT('Ctrl Pts',(4.14240873321982,-22.2784499072026,
0.));
#192152=CARTESIAN_POINT('Ctrl Pts',(4.14240873321982,-22.2784499072026,
12.));
#192153=CARTESIAN_POINT('Ctrl Pts',(4.14020318715987,-22.2707656042456,
0.));
#192154=CARTESIAN_POINT('Ctrl Pts',(4.14020318715987,-22.2707656042456,
12.));
#192155=CARTESIAN_POINT('Ctrl Pts',(4.13809539255418,-22.263317791397,0.));
#192156=CARTESIAN_POINT('Ctrl Pts',(4.13809539255418,-22.263317791397,12.));
#192157=CARTESIAN_POINT('Ctrl Pts',(4.13608511977226,-22.2561118708422,
0.));
#192158=CARTESIAN_POINT('Ctrl Pts',(4.13608511977226,-22.2561118708422,
12.));
#192159=CARTESIAN_POINT('Ctrl Pts',(4.13417212558808,-22.2491535317789,
0.));
#192160=CARTESIAN_POINT('Ctrl Pts',(4.13417212558808,-22.2491535317789,
12.));
#192161=CARTESIAN_POINT('Ctrl Pts',(4.1323561506016,-22.2424488153523,0.));
#192162=CARTESIAN_POINT('Ctrl Pts',(4.1323561506016,-22.2424488153523,12.));
#192163=CARTESIAN_POINT('Ctrl Pts',(4.13063692157499,-22.2360040565534,
0.));
#192164=CARTESIAN_POINT('Ctrl Pts',(4.13063692157499,-22.2360040565534,
12.));
#192165=CARTESIAN_POINT('Ctrl Pts',(4.12901415463378,-22.2298258043947,
0.));
#192166=CARTESIAN_POINT('Ctrl Pts',(4.12901415463378,-22.2298258043947,
12.));
#192167=CARTESIAN_POINT('Ctrl Pts',(4.12748755830099,-22.2239207458781,
0.));
#192168=CARTESIAN_POINT('Ctrl Pts',(4.12748755830099,-22.2239207458781,
12.));
#192169=CARTESIAN_POINT('Ctrl Pts',(4.12605683613299,-22.2182956401341,
0.));
#192170=CARTESIAN_POINT('Ctrl Pts',(4.12605683613299,-22.2182956401341,
12.));
#192171=CARTESIAN_POINT('Ctrl Pts',(4.12472167516602,-22.2129576146671,
0.));
#192172=CARTESIAN_POINT('Ctrl Pts',(4.12472167516602,-22.2129576146671,
12.));
#192173=CARTESIAN_POINT('Ctrl Pts',(4.12348173702024,-22.2079143941719,
0.));
#192174=CARTESIAN_POINT('Ctrl Pts',(4.12348173702024,-22.2079143941719,
12.));
#192175=CARTESIAN_POINT('Ctrl Pts',(4.12233664408237,-22.2031746532106,
0.));
#192176=CARTESIAN_POINT('Ctrl Pts',(4.12233664408237,-22.2031746532106,
12.));
#192177=CARTESIAN_POINT('Ctrl Pts',(4.12128598183533,-22.1987479618246,
0.));
#192178=CARTESIAN_POINT('Ctrl Pts',(4.12128598183533,-22.1987479618246,
12.));
#192179=CARTESIAN_POINT('Ctrl Pts',(4.12032932637738,-22.1946440958098,
0.));
#192180=CARTESIAN_POINT('Ctrl Pts',(4.12032932637738,-22.1946440958098,
12.));
#192181=CARTESIAN_POINT('Ctrl Pts',(4.11946626228623,-22.1908725908525,
0.));
#192182=CARTESIAN_POINT('Ctrl Pts',(4.11946626228623,-22.1908725908525,
12.));
#192183=CARTESIAN_POINT('Ctrl Pts',(4.11869641271752,-22.1874419861496,
0.));
#192184=CARTESIAN_POINT('Ctrl Pts',(4.11869641271752,-22.1874419861496,
12.));
#192185=CARTESIAN_POINT('Ctrl Pts',(4.11801938107464,-22.1843613164855,
0.));
#192186=CARTESIAN_POINT('Ctrl Pts',(4.11801938107464,-22.1843613164855,
12.));
#192187=CARTESIAN_POINT('Ctrl Pts',(4.11743469691765,-22.1816414985788,
0.));
#192188=CARTESIAN_POINT('Ctrl Pts',(4.11743469691765,-22.1816414985788,
12.));
#192189=CARTESIAN_POINT('Ctrl Pts',(4.11694173195041,-22.179297473024,0.));
#192190=CARTESIAN_POINT('Ctrl Pts',(4.11694173195041,-22.179297473024,12.));
#192191=CARTESIAN_POINT('Ctrl Pts',(4.11653973150558,-22.177347426894,0.));
#192192=CARTESIAN_POINT('Ctrl Pts',(4.11653973150558,-22.177347426894,12.));
#192193=CARTESIAN_POINT('Ctrl Pts',(4.11622797217066,-22.1758088296598,
0.));
#192194=CARTESIAN_POINT('Ctrl Pts',(4.11622797217066,-22.1758088296598,
12.));
#192195=CARTESIAN_POINT('Ctrl Pts',(4.11600589882767,-22.1746949858773,
0.));
#192196=CARTESIAN_POINT('Ctrl Pts',(4.11600589882767,-22.1746949858773,
12.));
#192197=CARTESIAN_POINT('Ctrl Pts',(4.11589976826061,-22.174148802123,0.));
#192198=CARTESIAN_POINT('Ctrl Pts',(4.11589976826061,-22.174148802123,12.));
#192199=CARTESIAN_POINT('Ctrl Pts',(4.1158603587821,-22.1739341411684,0.));
#192200=CARTESIAN_POINT('Ctrl Pts',(4.1158603587821,-22.1739341411684,12.));
#192201=CARTESIAN_POINT('Ctrl Pts',(4.11585194677412,-22.1738776823239,
0.));
#192202=CARTESIAN_POINT('Ctrl Pts',(4.11585194677412,-22.1738776823239,
12.));
#192203=CARTESIAN_POINT('Ctrl Pts',(4.11585220600461,-22.1738711152697,
0.));
#192204=CARTESIAN_POINT('Ctrl Pts',(4.11585220600461,-22.1738711152697,
12.));
#192205=CARTESIAN_POINT('',(6.08833931617698,-25.2771067246846,0.));
#192206=CARTESIAN_POINT('Ctrl Pts',(6.08833931617698,-25.2771067246846,
0.));
#192207=CARTESIAN_POINT('Ctrl Pts',(6.08441489609824,-25.2729539149479,
0.));
#192208=CARTESIAN_POINT('Ctrl Pts',(6.07657531787577,-25.2646490489816,
0.));
#192209=CARTESIAN_POINT('Ctrl Pts',(6.06484373634696,-25.2521940105523,
0.));
#192210=CARTESIAN_POINT('Ctrl Pts',(6.04925720151412,-25.2355918138798,
0.));
#192211=CARTESIAN_POINT('Ctrl Pts',(6.02986667390187,-25.2148466201368,
0.));
#192212=CARTESIAN_POINT('Ctrl Pts',(6.0105688180476,-25.1941090269638,0.));
#192213=CARTESIAN_POINT('Ctrl Pts',(5.99136367859838,-25.1733791296154,
0.));
#192214=CARTESIAN_POINT('Ctrl Pts',(5.97225131495636,-25.1526570863065,
0.));
#192215=CARTESIAN_POINT('Ctrl Pts',(5.95323180187347,-25.1319431317273,
0.));
#192216=CARTESIAN_POINT('Ctrl Pts',(5.93430523086776,-25.1112375971182,
0.));
#192217=CARTESIAN_POINT('Ctrl Pts',(5.91547170844382,-25.0905409050863,
0.));
#192218=CARTESIAN_POINT('Ctrl Pts',(5.89673135155458,-25.0698535426593,
0.));
#192219=CARTESIAN_POINT('Ctrl Pts',(5.87808428385329,-25.0491760405965,
0.));
#192220=CARTESIAN_POINT('Ctrl Pts',(5.8595306315681,-25.0285089498922,0.));
#192221=CARTESIAN_POINT('Ctrl Pts',(5.84107051963073,-25.0078528200558,
0.));
#192222=CARTESIAN_POINT('Ctrl Pts',(5.82270406744213,-24.9872081752709,
0.));
#192223=CARTESIAN_POINT('Ctrl Pts',(5.80443138549747,-24.9665754954463,
0.));
#192224=CARTESIAN_POINT('Ctrl Pts',(5.78625257775702,-24.9459552293308,
0.));
#192225=CARTESIAN_POINT('Ctrl Pts',(5.76816774342236,-24.9253478043632,
0.));
#192226=CARTESIAN_POINT('Ctrl Pts',(5.75017697890812,-24.9047536376467,
0.));
#192227=CARTESIAN_POINT('Ctrl Pts',(5.73228037976926,-24.8841731467219,
0.));
#192228=CARTESIAN_POINT('Ctrl Pts',(5.71447804252019,-24.8636067597677,
0.));
#192229=CARTESIAN_POINT('Ctrl Pts',(5.69677006679429,-24.8430549277634,
0.));
#192230=CARTESIAN_POINT('Ctrl Pts',(5.67915655496524,-24.822518122386,0.));
#192231=CARTESIAN_POINT('Ctrl Pts',(5.66163761114903,-24.8019968304618,
0.));
#192232=CARTESIAN_POINT('Ctrl Pts',(5.64421334042247,-24.7814915496728,
0.));
#192233=CARTESIAN_POINT('Ctrl Pts',(5.62688384790918,-24.76100278357,0.));
#192234=CARTESIAN_POINT('Ctrl Pts',(5.60964923798494,-24.7405310372736,
0.));
#192235=CARTESIAN_POINT('Ctrl Pts',(5.59250961323995,-24.7200768119079,
0.));
#192236=CARTESIAN_POINT('Ctrl Pts',(5.57546507427766,-24.6996406035507,
0.));
#192237=CARTESIAN_POINT('Ctrl Pts',(5.55851572025389,-24.6792229061785,
0.));
#192238=CARTESIAN_POINT('Ctrl Pts',(5.54166164919592,-24.6588242134733,
0.));
#192239=CARTESIAN_POINT('Ctrl Pts',(5.52490295840996,-24.6384450211466,
0.));
#192240=CARTESIAN_POINT('Ctrl Pts',(5.50823974481959,-24.618085828918,0.));
#192241=CARTESIAN_POINT('Ctrl Pts',(5.49167210537235,-24.5977471429365,
0.));
#192242=CARTESIAN_POINT('Ctrl Pts',(5.47520013724403,-24.5774294770329,
0.));
#192243=CARTESIAN_POINT('Ctrl Pts',(5.45882393762244,-24.5571333514841,
0.));
#192244=CARTESIAN_POINT('Ctrl Pts',(5.44254360356865,-24.5368592922861,
0.));
#192245=CARTESIAN_POINT('Ctrl Pts',(5.42635923183411,-24.5166078302107,
0.));
#192246=CARTESIAN_POINT('Ctrl Pts',(5.41027091869242,-24.4963794999831,
0.));
#192247=CARTESIAN_POINT('Ctrl Pts',(5.3942787597383,-24.4761748393322,0.));
#192248=CARTESIAN_POINT('Ctrl Pts',(5.37838284973706,-24.4559943883159,
0.));
#192249=CARTESIAN_POINT('Ctrl Pts',(5.36258328273639,-24.4358386899152,
0.));
#192250=CARTESIAN_POINT('Ctrl Pts',(5.34688015213546,-24.4157082904615,
0.));
#192251=CARTESIAN_POINT('Ctrl Pts',(5.33127355076036,-24.3956037401293,
0.));
#192252=CARTESIAN_POINT('Ctrl Pts',(5.31576357092524,-24.3755255933917,
0.));
#192253=CARTESIAN_POINT('Ctrl Pts',(5.30035030449058,-24.3554744095075,
0.));
#192254=CARTESIAN_POINT('Ctrl Pts',(5.28503384290644,-24.3354507529415,
0.));
#192255=CARTESIAN_POINT('Ctrl Pts',(5.26981427718796,-24.3154551932222,
0.));
#192256=CARTESIAN_POINT('Ctrl Pts',(5.25469169788855,-24.2954883048448,
0.));
#192257=CARTESIAN_POINT('Ctrl Pts',(5.23966619506289,-24.2755506671526,
0.));
#192258=CARTESIAN_POINT('Ctrl Pts',(5.22473785822441,-24.2556428642294,
0.));
#192259=CARTESIAN_POINT('Ctrl Pts',(5.20990677629173,-24.2357654847765,
0.));
#192260=CARTESIAN_POINT('Ctrl Pts',(5.19517303753642,-24.215919122017,0.));
#192261=CARTESIAN_POINT('Ctrl Pts',(5.18053672961392,-24.1961043738754,
0.));
#192262=CARTESIAN_POINT('Ctrl Pts',(5.16599793957979,-24.1763218431343,
0.));
#192263=CARTESIAN_POINT('Ctrl Pts',(5.15155675390075,-24.1565721375971,
0.));
#192264=CARTESIAN_POINT('Ctrl Pts',(5.13721325845744,-24.1368558702443,
0.));
#192265=CARTESIAN_POINT('Ctrl Pts',(5.12296753853859,-24.117173659394,0.));
#192266=CARTESIAN_POINT('Ctrl Pts',(5.10881967883132,-24.0975261288446,
0.));
#192267=CARTESIAN_POINT('Ctrl Pts',(5.09476976342625,-24.0779139079266,
0.));
#192268=CARTESIAN_POINT('Ctrl Pts',(5.08081787581276,-24.0583376315638,
0.));
#192269=CARTESIAN_POINT('Ctrl Pts',(5.06696409886641,-24.0387979403268,
0.));
#192270=CARTESIAN_POINT('Ctrl Pts',(5.05320851483065,-24.0192954804896,
0.));
#192271=CARTESIAN_POINT('Ctrl Pts',(5.03955120528521,-23.9998309040746,
0.));
#192272=CARTESIAN_POINT('Ctrl Pts',(5.02599225112454,-23.9804048689227,
0.));
#192273=CARTESIAN_POINT('Ctrl Pts',(5.01253173257452,-23.9610180388271,
0.));
#192274=CARTESIAN_POINT('Ctrl Pts',(4.99916972919306,-23.9416710836529,
0.));
#192275=CARTESIAN_POINT('Ctrl Pts',(4.98590631986532,-23.9223646794592,
0.));
#192276=CARTESIAN_POINT('Ctrl Pts',(4.97274158279226,-23.9030995086163,
0.));
#192277=CARTESIAN_POINT('Ctrl Pts',(4.9596755954656,-23.8838762599218,0.));
#192278=CARTESIAN_POINT('Ctrl Pts',(4.9467084346586,-23.8646956287168,0.));
#192279=CARTESIAN_POINT('Ctrl Pts',(4.93384017643432,-23.8455583170057,
0.));
#192280=CARTESIAN_POINT('Ctrl Pts',(4.92107089613968,-23.8264650335717,
0.));
#192281=CARTESIAN_POINT('Ctrl Pts',(4.90840066839344,-23.8074164940896,
0.));
#192282=CARTESIAN_POINT('Ctrl Pts',(4.89582956706775,-23.7884134212384,
0.));
#192283=CARTESIAN_POINT('Ctrl Pts',(4.88335766525573,-23.7694565448049,
0.));
#192284=CARTESIAN_POINT('Ctrl Pts',(4.87098503527152,-23.7505466018245,
0.));
#192285=CARTESIAN_POINT('Ctrl Pts',(4.85871174865499,-23.7316843367313,
0.));
#192286=CARTESIAN_POINT('Ctrl Pts',(4.84653787616425,-23.7128705015017,
0.));
#192287=CARTESIAN_POINT('Ctrl Pts',(4.83446348776265,-23.6941058557971,
0.));
#192288=CARTESIAN_POINT('Ctrl Pts',(4.82248865259562,-23.675391167102,0.));
#192289=CARTESIAN_POINT('Ctrl Pts',(4.81061343896432,-23.6567272108628,
0.));
#192290=CARTESIAN_POINT('Ctrl Pts',(4.7988379143322,-23.6381147706579,0.));
#192291=CARTESIAN_POINT('Ctrl Pts',(4.78716214532097,-23.6195546383624,
0.));
#192292=CARTESIAN_POINT('Ctrl Pts',(4.77558619769872,-23.6010476143099,
0.));
#192293=CARTESIAN_POINT('Ctrl Pts',(4.76411013636251,-23.5825945074535,
0.));
#192294=CARTESIAN_POINT('Ctrl Pts',(4.75273402530617,-23.5641961355168,
0.));
#192295=CARTESIAN_POINT('Ctrl Pts',(4.74145792760698,-23.545853325171,0.));
#192296=CARTESIAN_POINT('Ctrl Pts',(4.73028190543029,-23.5275669122372,
0.));
#192297=CARTESIAN_POINT('Ctrl Pts',(4.71920602001901,-23.509337741878,0.));
#192298=CARTESIAN_POINT('Ctrl Pts',(4.70823033167818,-23.491166668789,0.));
#192299=CARTESIAN_POINT('Ctrl Pts',(4.69735489975024,-23.4730545573853,
0.));
#192300=CARTESIAN_POINT('Ctrl Pts',(4.68657978258303,-23.455002281986,0.));
#192301=CARTESIAN_POINT('Ctrl Pts',(4.67590503753058,-23.4370107270451,
0.));
#192302=CARTESIAN_POINT('Ctrl Pts',(4.6653307209467,-23.4190807873803,0.));
#192303=CARTESIAN_POINT('Ctrl Pts',(4.65485688816924,-23.4012133683959,
0.));
#192304=CARTESIAN_POINT('Ctrl Pts',(4.6444835934993,-23.3834093863068,0.));
#192305=CARTESIAN_POINT('Ctrl Pts',(4.63421089016541,-23.3656697683489,
0.));
#192306=CARTESIAN_POINT('Ctrl Pts',(4.62403883030805,-23.3479954530272,
0.));
#192307=CARTESIAN_POINT('Ctrl Pts',(4.6139674649783,-23.3303873903938,0.));
#192308=CARTESIAN_POINT('Ctrl Pts',(4.60399684412163,-23.3128465423115,
0.));
#192309=CARTESIAN_POINT('Ctrl Pts',(4.5941270165575,-23.2953738827191,0.));
#192310=CARTESIAN_POINT('Ctrl Pts',(4.5843580299469,-23.2779703978876,0.));
#192311=CARTESIAN_POINT('Ctrl Pts',(4.57468993076097,-23.2606370866866,
0.));
#192312=CARTESIAN_POINT('Ctrl Pts',(4.56512276427839,-23.2433749609131,
0.));
#192313=CARTESIAN_POINT('Ctrl Pts',(4.55565657456975,-23.2261850456064,
0.));
#192314=CARTESIAN_POINT('Ctrl Pts',(4.54629140447544,-23.2090683793629,
0.));
#192315=CARTESIAN_POINT('Ctrl Pts',(4.53702729557566,-23.1920260146465,
0.));
#192316=CARTESIAN_POINT('Ctrl Pts',(4.52786428815014,-23.1750590180908,
0.));
#192317=CARTESIAN_POINT('Ctrl Pts',(4.51880242116748,-23.1581684708761,
0.));
#192318=CARTESIAN_POINT('Ctrl Pts',(4.5098417322706,-23.1413554691123,0.));
#192319=CARTESIAN_POINT('Ctrl Pts',(4.50098225775171,-23.1246211242115,
0.));
#192320=CARTESIAN_POINT('Ctrl Pts',(4.49222403252216,-23.1079665632636,
0.));
#192321=CARTESIAN_POINT('Ctrl Pts',(4.48356709006788,-23.0913929293922,
0.));
#192322=CARTESIAN_POINT('Ctrl Pts',(4.47501146242856,-23.0749013821881,
0.));
#192323=CARTESIAN_POINT('Ctrl Pts',(4.4665571801823,-23.0584930981732,0.));
#192324=CARTESIAN_POINT('Ctrl Pts',(4.45820427241683,-23.0421692712467,
0.));
#192325=CARTESIAN_POINT('Ctrl Pts',(4.44995276669686,-23.0259311131392,
0.));
#192326=CARTESIAN_POINT('Ctrl Pts',(4.44180268901643,-23.0097798538395,
0.));
#192327=CARTESIAN_POINT('Ctrl Pts',(4.43375406376879,-22.9937167421006,
0.));
#192328=CARTESIAN_POINT('Ctrl Pts',(4.42580691372751,-22.977743046002,0.));
#192329=CARTESIAN_POINT('Ctrl Pts',(4.41796126001302,-22.9618600534866,
0.));
#192330=CARTESIAN_POINT('Ctrl Pts',(4.41021712205553,-22.9460690729093,
0.));
#192331=CARTESIAN_POINT('Ctrl Pts',(4.40257451754323,-22.930371433555,0.));
#192332=CARTESIAN_POINT('Ctrl Pts',(4.39503346238473,-22.9147684862426,
0.));
#192333=CARTESIAN_POINT('Ctrl Pts',(4.38759397068405,-22.8992616040108,
0.));
#192334=CARTESIAN_POINT('Ctrl Pts',(4.38025605470092,-22.8838521827701,
0.));
#192335=CARTESIAN_POINT('Ctrl Pts',(4.37301972480745,-22.8685416419725,
0.));
#192336=CARTESIAN_POINT('Ctrl Pts',(4.36588498942997,-22.8533314252422,
0.));
#192337=CARTESIAN_POINT('Ctrl Pts',(4.35885185500546,-22.8382230011184,
0.));
#192338=CARTESIAN_POINT('Ctrl Pts',(4.3519203259479,-22.8232178638876,0.));
#192339=CARTESIAN_POINT('Ctrl Pts',(4.34509040460062,-22.8083175343791,
0.));
#192340=CARTESIAN_POINT('Ctrl Pts',(4.33836209118446,-22.7935235607806,
0.));
#192341=CARTESIAN_POINT('Ctrl Pts',(4.33173538373189,-22.7788375194076,
0.));
#192342=CARTESIAN_POINT('Ctrl Pts',(4.32521027803754,-22.7642610156475,
0.));
#192343=CARTESIAN_POINT('Ctrl Pts',(4.31878676761235,-22.7497956849848,
0.));
#192344=CARTESIAN_POINT('Ctrl Pts',(4.31246484362549,-22.7354431939926,
0.));
#192345=CARTESIAN_POINT('Ctrl Pts',(4.30624449484069,-22.7212052413386,
0.));
#192346=CARTESIAN_POINT('Ctrl Pts',(4.3001257075406,-22.7070835587564,0.));
#192347=CARTESIAN_POINT('Ctrl Pts',(4.29410846547056,-22.6930799122548,
0.));
#192348=CARTESIAN_POINT('Ctrl Pts',(4.28819274977763,-22.6791961033538,
0.));
#192349=CARTESIAN_POINT('Ctrl Pts',(4.28237853894058,-22.6654339703109,
0.));
#192350=CARTESIAN_POINT('Ctrl Pts',(4.2766658086912,-22.6517953893303,0.));
#192351=CARTESIAN_POINT('Ctrl Pts',(4.27105453193004,-22.6382822758172,
0.));
#192352=CARTESIAN_POINT('Ctrl Pts',(4.26554467865576,-22.6248965859977,
0.));
#192353=CARTESIAN_POINT('Ctrl Pts',(4.26013621588305,-22.6116403184821,
0.));
#192354=CARTESIAN_POINT('Ctrl Pts',(4.25482910755481,-22.5985155158636,
0.));
#192355=CARTESIAN_POINT('Ctrl Pts',(4.24962331444177,-22.5855242662477,
0.));
#192356=CARTESIAN_POINT('Ctrl Pts',(4.24451879404851,-22.572668704992,0.));
#192357=CARTESIAN_POINT('Ctrl Pts',(4.23951550052522,-22.5599510166429,
0.));
#192358=CARTESIAN_POINT('Ctrl Pts',(4.23461338456712,-22.5473734368086,
0.));
#192359=CARTESIAN_POINT('Ctrl Pts',(4.22981239330733,-22.5349382540588,
0.));
#192360=CARTESIAN_POINT('Ctrl Pts',(4.22511247020041,-22.5226478117886,
0.));
#192361=CARTESIAN_POINT('Ctrl Pts',(4.22051355490196,-22.5105045108881,
0.));
#192362=CARTESIAN_POINT('Ctrl Pts',(4.21601558313906,-22.4985108124228,
0.));
#192363=CARTESIAN_POINT('Ctrl Pts',(4.21161848657428,-22.4866692403147,
0.));
#192364=CARTESIAN_POINT('Ctrl Pts',(4.20732219265648,-22.4749823839917,
0.));
#192365=CARTESIAN_POINT('Ctrl Pts',(4.20312662448174,-22.4634529011437,
0.));
#192366=CARTESIAN_POINT('Ctrl Pts',(4.19903170066358,-22.4520835205422,
0.));
#192367=CARTESIAN_POINT('Ctrl Pts',(4.1950373351886,-22.4408770448917,0.));
#192368=CARTESIAN_POINT('Ctrl Pts',(4.19114343726932,-22.4298363535416,
0.));
#192369=CARTESIAN_POINT('Ctrl Pts',(4.18734991117707,-22.4189644056109,
0.));
#192370=CARTESIAN_POINT('Ctrl Pts',(4.18365665600839,-22.4082642454448,
0.));
#192371=CARTESIAN_POINT('Ctrl Pts',(4.18006356544879,-22.3977390078074,
0.));
#192372=CARTESIAN_POINT('Ctrl Pts',(4.17657052752834,-22.3873919231339,
0.));
#192373=CARTESIAN_POINT('Ctrl Pts',(4.17317742436162,-22.3772263228624,
0.));
#192374=CARTESIAN_POINT('Ctrl Pts',(4.16988413199469,-22.3672456427605,
0.));
#192375=CARTESIAN_POINT('Ctrl Pts',(4.16669052026602,-22.3574534257397,
0.));
#192376=CARTESIAN_POINT('Ctrl Pts',(4.1635964526318,-22.3478533253886,0.));
#192377=CARTESIAN_POINT('Ctrl Pts',(4.16060178604153,-22.3384491078599,
0.));
#192378=CARTESIAN_POINT('Ctrl Pts',(4.15770637047882,-22.3292446628957,
0.));
#192379=CARTESIAN_POINT('Ctrl Pts',(4.15491004835278,-22.3202440186979,
0.));
#192380=CARTESIAN_POINT('Ctrl Pts',(4.15221265396992,-22.3114513545186,
0.));
#192381=CARTESIAN_POINT('Ctrl Pts',(4.14961401285525,-22.3028710166935,
0.));
#192382=CARTESIAN_POINT('Ctrl Pts',(4.14711394168559,-22.2945075198468,
0.));
#192383=CARTESIAN_POINT('Ctrl Pts',(4.14471224859295,-22.2863655389167,
0.));
#192384=CARTESIAN_POINT('Ctrl Pts',(4.14240873321982,-22.2784499072026,
0.));
#192385=CARTESIAN_POINT('Ctrl Pts',(4.14020318715987,-22.2707656042456,
0.));
#192386=CARTESIAN_POINT('Ctrl Pts',(4.13809539255418,-22.263317791397,0.));
#192387=CARTESIAN_POINT('Ctrl Pts',(4.13608511977226,-22.2561118708422,
0.));
#192388=CARTESIAN_POINT('Ctrl Pts',(4.13417212558808,-22.2491535317789,
0.));
#192389=CARTESIAN_POINT('Ctrl Pts',(4.1323561506016,-22.2424488153523,0.));
#192390=CARTESIAN_POINT('Ctrl Pts',(4.13063692157499,-22.2360040565534,
0.));
#192391=CARTESIAN_POINT('Ctrl Pts',(4.12901415463378,-22.2298258043947,
0.));
#192392=CARTESIAN_POINT('Ctrl Pts',(4.12748755830099,-22.2239207458781,
0.));
#192393=CARTESIAN_POINT('Ctrl Pts',(4.12605683613299,-22.2182956401341,
0.));
#192394=CARTESIAN_POINT('Ctrl Pts',(4.12472167516602,-22.2129576146671,
0.));
#192395=CARTESIAN_POINT('Ctrl Pts',(4.12348173702024,-22.2079143941719,
0.));
#192396=CARTESIAN_POINT('Ctrl Pts',(4.12233664408237,-22.2031746532106,
0.));
#192397=CARTESIAN_POINT('Ctrl Pts',(4.12128598183533,-22.1987479618246,
0.));
#192398=CARTESIAN_POINT('Ctrl Pts',(4.12032932637738,-22.1946440958098,
0.));
#192399=CARTESIAN_POINT('Ctrl Pts',(4.11946626228623,-22.1908725908525,
0.));
#192400=CARTESIAN_POINT('Ctrl Pts',(4.11869641271752,-22.1874419861496,
0.));
#192401=CARTESIAN_POINT('Ctrl Pts',(4.11801938107464,-22.1843613164855,
0.));
#192402=CARTESIAN_POINT('Ctrl Pts',(4.11743469691765,-22.1816414985788,
0.));
#192403=CARTESIAN_POINT('Ctrl Pts',(4.11694173195041,-22.179297473024,0.));
#192404=CARTESIAN_POINT('Ctrl Pts',(4.11653973150558,-22.177347426894,0.));
#192405=CARTESIAN_POINT('Ctrl Pts',(4.11622797217066,-22.1758088296598,
0.));
#192406=CARTESIAN_POINT('Ctrl Pts',(4.11600589882767,-22.1746949858773,
0.));
#192407=CARTESIAN_POINT('Ctrl Pts',(4.11589976826061,-22.174148802123,0.));
#192408=CARTESIAN_POINT('Ctrl Pts',(4.1158603587821,-22.1739341411684,0.));
#192409=CARTESIAN_POINT('Ctrl Pts',(4.11585194677412,-22.1738776823239,
0.));
#192410=CARTESIAN_POINT('Ctrl Pts',(4.11585220600461,-22.1738711152697,
0.));
#192411=CARTESIAN_POINT('',(6.08833931617698,-25.2771067246846,0.));
#192412=CARTESIAN_POINT('Ctrl Pts',(1.76341220531179,-22.4835757167854,
0.));
#192413=CARTESIAN_POINT('Ctrl Pts',(1.76341220531179,-22.4835757167854,
12.));
#192414=CARTESIAN_POINT('Ctrl Pts',(1.76341415538764,-22.483581992979,0.));
#192415=CARTESIAN_POINT('Ctrl Pts',(1.76341415538764,-22.483581992979,12.));
#192416=CARTESIAN_POINT('Ctrl Pts',(1.7634206426357,-22.4836387052232,0.));
#192417=CARTESIAN_POINT('Ctrl Pts',(1.7634206426357,-22.4836387052232,12.));
#192418=CARTESIAN_POINT('Ctrl Pts',(1.76343813434565,-22.483856251707,0.));
#192419=CARTESIAN_POINT('Ctrl Pts',(1.76343813434565,-22.483856251707,12.));
#192420=CARTESIAN_POINT('Ctrl Pts',(1.76347698284791,-22.4844112933129,
0.));
#192421=CARTESIAN_POINT('Ctrl Pts',(1.76347698284791,-22.4844112933129,
12.));
#192422=CARTESIAN_POINT('Ctrl Pts',(1.76355076045546,-22.4855446605991,
0.));
#192423=CARTESIAN_POINT('Ctrl Pts',(1.76355076045546,-22.4855446605991,
12.));
#192424=CARTESIAN_POINT('Ctrl Pts',(1.76364784232963,-22.4871115206571,
0.));
#192425=CARTESIAN_POINT('Ctrl Pts',(1.76364784232963,-22.4871115206571,
12.));
#192426=CARTESIAN_POINT('Ctrl Pts',(1.76376424879504,-22.4890991659478,
0.));
#192427=CARTESIAN_POINT('Ctrl Pts',(1.76376424879504,-22.4890991659478,
12.));
#192428=CARTESIAN_POINT('Ctrl Pts',(1.76389475965723,-22.4914909094908,
0.));
#192429=CARTESIAN_POINT('Ctrl Pts',(1.76389475965723,-22.4914909094908,
12.));
#192430=CARTESIAN_POINT('Ctrl Pts',(1.764033938803,-22.4942693792449,0.));
#192431=CARTESIAN_POINT('Ctrl Pts',(1.764033938803,-22.4942693792449,12.));
#192432=CARTESIAN_POINT('Ctrl Pts',(1.76417731243462,-22.4974203063191,
0.));
#192433=CARTESIAN_POINT('Ctrl Pts',(1.76417731243462,-22.4974203063191,
12.));
#192434=CARTESIAN_POINT('Ctrl Pts',(1.76432160068725,-22.5009332677316,
0.));
#192435=CARTESIAN_POINT('Ctrl Pts',(1.76432160068725,-22.5009332677316,
12.));
#192436=CARTESIAN_POINT('Ctrl Pts',(1.76446408210366,-22.5047996391978,
0.));
#192437=CARTESIAN_POINT('Ctrl Pts',(1.76446408210366,-22.5047996391978,
12.));
#192438=CARTESIAN_POINT('Ctrl Pts',(1.76460218257323,-22.5090112700212,
0.));
#192439=CARTESIAN_POINT('Ctrl Pts',(1.76460218257323,-22.5090112700212,
12.));
#192440=CARTESIAN_POINT('Ctrl Pts',(1.76473303281158,-22.5135590569554,
0.));
#192441=CARTESIAN_POINT('Ctrl Pts',(1.76473303281158,-22.5135590569554,
12.));
#192442=CARTESIAN_POINT('Ctrl Pts',(1.76485369319896,-22.5184336670207,
0.));
#192443=CARTESIAN_POINT('Ctrl Pts',(1.76485369319896,-22.5184336670207,
12.));
#192444=CARTESIAN_POINT('Ctrl Pts',(1.76496128643369,-22.5236259635515,
0.));
#192445=CARTESIAN_POINT('Ctrl Pts',(1.76496128643369,-22.5236259635515,
12.));
#192446=CARTESIAN_POINT('Ctrl Pts',(1.76505320262751,-22.529127665298,0.));
#192447=CARTESIAN_POINT('Ctrl Pts',(1.76505320262751,-22.529127665298,12.));
#192448=CARTESIAN_POINT('Ctrl Pts',(1.7651271156325,-22.5349313983571,0.));
#192449=CARTESIAN_POINT('Ctrl Pts',(1.7651271156325,-22.5349313983571,12.));
#192450=CARTESIAN_POINT('Ctrl Pts',(1.76518087841492,-22.5410303590891,
0.));
#192451=CARTESIAN_POINT('Ctrl Pts',(1.76518087841492,-22.5410303590891,
12.));
#192452=CARTESIAN_POINT('Ctrl Pts',(1.76521245524047,-22.5474180954006,
0.));
#192453=CARTESIAN_POINT('Ctrl Pts',(1.76521245524047,-22.5474180954006,
12.));
#192454=CARTESIAN_POINT('Ctrl Pts',(1.76521983384062,-22.5540882235837,
0.));
#192455=CARTESIAN_POINT('Ctrl Pts',(1.76521983384062,-22.5540882235837,
12.));
#192456=CARTESIAN_POINT('Ctrl Pts',(1.76520104500449,-22.5610344912501,
0.));
#192457=CARTESIAN_POINT('Ctrl Pts',(1.76520104500449,-22.5610344912501,
12.));
#192458=CARTESIAN_POINT('Ctrl Pts',(1.76515418518829,-22.5682508499873,
0.));
#192459=CARTESIAN_POINT('Ctrl Pts',(1.76515418518829,-22.5682508499873,
12.));
#192460=CARTESIAN_POINT('Ctrl Pts',(1.76507744026747,-22.5757315316355,
0.));
#192461=CARTESIAN_POINT('Ctrl Pts',(1.76507744026747,-22.5757315316355,
12.));
#192462=CARTESIAN_POINT('Ctrl Pts',(1.76496910283088,-22.5834711038024,
0.));
#192463=CARTESIAN_POINT('Ctrl Pts',(1.76496910283088,-22.5834711038024,
12.));
#192464=CARTESIAN_POINT('Ctrl Pts',(1.76482755288411,-22.5914644078106,
0.));
#192465=CARTESIAN_POINT('Ctrl Pts',(1.76482755288411,-22.5914644078106,
12.));
#192466=CARTESIAN_POINT('Ctrl Pts',(1.76465124413556,-22.5997065145638,
0.));
#192467=CARTESIAN_POINT('Ctrl Pts',(1.76465124413556,-22.5997065145638,
12.));
#192468=CARTESIAN_POINT('Ctrl Pts',(1.76443868648015,-22.6081926681342,
0.));
#192469=CARTESIAN_POINT('Ctrl Pts',(1.76443868648015,-22.6081926681342,
12.));
#192470=CARTESIAN_POINT('Ctrl Pts',(1.76418843543739,-22.6169182517693,
0.));
#192471=CARTESIAN_POINT('Ctrl Pts',(1.76418843543739,-22.6169182517693,
12.));
#192472=CARTESIAN_POINT('Ctrl Pts',(1.76389909571402,-22.6258787994847,
0.));
#192473=CARTESIAN_POINT('Ctrl Pts',(1.76389909571402,-22.6258787994847,
12.));
#192474=CARTESIAN_POINT('Ctrl Pts',(1.76356932176272,-22.635069997936,0.));
#192475=CARTESIAN_POINT('Ctrl Pts',(1.76356932176272,-22.635069997936,12.));
#192476=CARTESIAN_POINT('Ctrl Pts',(1.76319782013913,-22.6444876940425,
0.));
#192477=CARTESIAN_POINT('Ctrl Pts',(1.76319782013913,-22.6444876940425,
12.));
#192478=CARTESIAN_POINT('Ctrl Pts',(1.76278334912559,-22.6541278938413,
0.));
#192479=CARTESIAN_POINT('Ctrl Pts',(1.76278334912559,-22.6541278938413,
12.));
#192480=CARTESIAN_POINT('Ctrl Pts',(1.76232471392567,-22.6639867471756,
0.));
#192481=CARTESIAN_POINT('Ctrl Pts',(1.76232471392567,-22.6639867471756,
12.));
#192482=CARTESIAN_POINT('Ctrl Pts',(1.76182076289525,-22.6740605356699,
0.));
#192483=CARTESIAN_POINT('Ctrl Pts',(1.76182076289525,-22.6740605356699,
12.));
#192484=CARTESIAN_POINT('Ctrl Pts',(1.76127038310612,-22.6843456585245,
0.));
#192485=CARTESIAN_POINT('Ctrl Pts',(1.76127038310612,-22.6843456585245,
12.));
#192486=CARTESIAN_POINT('Ctrl Pts',(1.76067249704884,-22.6948386219843,
0.));
#192487=CARTESIAN_POINT('Ctrl Pts',(1.76067249704884,-22.6948386219843,
12.));
#192488=CARTESIAN_POINT('Ctrl Pts',(1.76002606202398,-22.7055360375481,
0.));
#192489=CARTESIAN_POINT('Ctrl Pts',(1.76002606202398,-22.7055360375481,
12.));
#192490=CARTESIAN_POINT('Ctrl Pts',(1.75933006905924,-22.7164346186007,
0.));
#192491=CARTESIAN_POINT('Ctrl Pts',(1.75933006905924,-22.7164346186007,
12.));
#192492=CARTESIAN_POINT('Ctrl Pts',(1.75858354204634,-22.7275311777305,
0.));
#192493=CARTESIAN_POINT('Ctrl Pts',(1.75858354204634,-22.7275311777305,
12.));
#192494=CARTESIAN_POINT('Ctrl Pts',(1.75778553673249,-22.7388226235565,
0.));
#192495=CARTESIAN_POINT('Ctrl Pts',(1.75778553673249,-22.7388226235565,
12.));
#192496=CARTESIAN_POINT('Ctrl Pts',(1.75693513908911,-22.7503059556455,
0.));
#192497=CARTESIAN_POINT('Ctrl Pts',(1.75693513908911,-22.7503059556455,
12.));
#192498=CARTESIAN_POINT('Ctrl Pts',(1.7560314637164,-22.7619782595013,0.));
#192499=CARTESIAN_POINT('Ctrl Pts',(1.7560314637164,-22.7619782595013,12.));
#192500=CARTESIAN_POINT('Ctrl Pts',(1.75507365227127,-22.7738367016115,
0.));
#192501=CARTESIAN_POINT('Ctrl Pts',(1.75507365227127,-22.7738367016115,
12.));
#192502=CARTESIAN_POINT('Ctrl Pts',(1.75406087182929,-22.7858785242358,
0.));
#192503=CARTESIAN_POINT('Ctrl Pts',(1.75406087182929,-22.7858785242358,
12.));
#192504=CARTESIAN_POINT('Ctrl Pts',(1.75299231391461,-22.7981010424312,
0.));
#192505=CARTESIAN_POINT('Ctrl Pts',(1.75299231391461,-22.7981010424312,
12.));
#192506=CARTESIAN_POINT('Ctrl Pts',(1.75186719365589,-22.8105016414712,
0.));
#192507=CARTESIAN_POINT('Ctrl Pts',(1.75186719365589,-22.8105016414712,
12.));
#192508=CARTESIAN_POINT('Ctrl Pts',(1.75068474890883,-22.8230777741285,
0.));
#192509=CARTESIAN_POINT('Ctrl Pts',(1.75068474890883,-22.8230777741285,
12.));
#192510=CARTESIAN_POINT('Ctrl Pts',(1.74944423940117,-22.8358269579854,
0.));
#192511=CARTESIAN_POINT('Ctrl Pts',(1.74944423940117,-22.8358269579854,
12.));
#192512=CARTESIAN_POINT('Ctrl Pts',(1.74814494588491,-22.8487467728075,
0.));
#192513=CARTESIAN_POINT('Ctrl Pts',(1.74814494588491,-22.8487467728075,
12.));
#192514=CARTESIAN_POINT('Ctrl Pts',(1.74678616930663,-22.8618348580234,
0.));
#192515=CARTESIAN_POINT('Ctrl Pts',(1.74678616930663,-22.8618348580234,
12.));
#192516=CARTESIAN_POINT('Ctrl Pts',(1.74536722998199,-22.8750889101696,
0.));
#192517=CARTESIAN_POINT('Ctrl Pts',(1.74536722998199,-22.8750889101696,
12.));
#192518=CARTESIAN_POINT('Ctrl Pts',(1.74388746677702,-22.8885066803351,
0.));
#192519=CARTESIAN_POINT('Ctrl Pts',(1.74388746677702,-22.8885066803351,
12.));
#192520=CARTESIAN_POINT('Ctrl Pts',(1.74234623630079,-22.9020859716144,
0.));
#192521=CARTESIAN_POINT('Ctrl Pts',(1.74234623630079,-22.9020859716144,
12.));
#192522=CARTESIAN_POINT('Ctrl Pts',(1.74074291231056,-22.9158246373365,
0.));
#192523=CARTESIAN_POINT('Ctrl Pts',(1.74074291231056,-22.9158246373365,
12.));
#192524=CARTESIAN_POINT('Ctrl Pts',(1.73907688511664,-22.9297205792587,
0.));
#192525=CARTESIAN_POINT('Ctrl Pts',(1.73907688511664,-22.9297205792587,
12.));
#192526=CARTESIAN_POINT('Ctrl Pts',(1.73734756100038,-22.9437717457825,
0.));
#192527=CARTESIAN_POINT('Ctrl Pts',(1.73734756100038,-22.9437717457825,
12.));
#192528=CARTESIAN_POINT('Ctrl Pts',(1.73555436162771,-22.9579761301062,
0.));
#192529=CARTESIAN_POINT('Ctrl Pts',(1.73555436162771,-22.9579761301062,
12.));
#192530=CARTESIAN_POINT('Ctrl Pts',(1.73369672350817,-22.9723317685688,
0.));
#192531=CARTESIAN_POINT('Ctrl Pts',(1.73369672350817,-22.9723317685688,
12.));
#192532=CARTESIAN_POINT('Ctrl Pts',(1.73177409750193,-22.9868367391978,
0.));
#192533=CARTESIAN_POINT('Ctrl Pts',(1.73177409750193,-22.9868367391978,
12.));
#192534=CARTESIAN_POINT('Ctrl Pts',(1.72978594832137,-23.0014891601891,
0.));
#192535=CARTESIAN_POINT('Ctrl Pts',(1.72978594832137,-23.0014891601891,
12.));
#192536=CARTESIAN_POINT('Ctrl Pts',(1.72773175404702,-23.0162871884167,
0.));
#192537=CARTESIAN_POINT('Ctrl Pts',(1.72773175404702,-23.0162871884167,
12.));
#192538=CARTESIAN_POINT('Ctrl Pts',(1.72561100564033,-23.031229017888,0.));
#192539=CARTESIAN_POINT('Ctrl Pts',(1.72561100564033,-23.031229017888,12.));
#192540=CARTESIAN_POINT('Ctrl Pts',(1.72342320653731,-23.0463128785528,
0.));
#192541=CARTESIAN_POINT('Ctrl Pts',(1.72342320653731,-23.0463128785528,
12.));
#192542=CARTESIAN_POINT('Ctrl Pts',(1.7211678722598,-23.061537035156,0.));
#192543=CARTESIAN_POINT('Ctrl Pts',(1.7211678722598,-23.061537035156,12.));
#192544=CARTESIAN_POINT('Ctrl Pts',(1.71884453003027,-23.0768997860709,
0.));
#192545=CARTESIAN_POINT('Ctrl Pts',(1.71884453003027,-23.0768997860709,
12.));
#192546=CARTESIAN_POINT('Ctrl Pts',(1.71645271839311,-23.0923994621216,
0.));
#192547=CARTESIAN_POINT('Ctrl Pts',(1.71645271839311,-23.0923994621216,
12.));
#192548=CARTESIAN_POINT('Ctrl Pts',(1.71399198684724,-23.1080344254291,
0.));
#192549=CARTESIAN_POINT('Ctrl Pts',(1.71399198684724,-23.1080344254291,
12.));
#192550=CARTESIAN_POINT('Ctrl Pts',(1.71146189552192,-23.1238030684929,
0.));
#192551=CARTESIAN_POINT('Ctrl Pts',(1.71146189552192,-23.1238030684929,
12.));
#192552=CARTESIAN_POINT('Ctrl Pts',(1.70886201485459,-23.1397038132358,
0.));
#192553=CARTESIAN_POINT('Ctrl Pts',(1.70886201485459,-23.1397038132358,
12.));
#192554=CARTESIAN_POINT('Ctrl Pts',(1.70619192527846,-23.1557351100613,
0.));
#192555=CARTESIAN_POINT('Ctrl Pts',(1.70619192527846,-23.1557351100613,
12.));
#192556=CARTESIAN_POINT('Ctrl Pts',(1.70345121691259,-23.1718954368749,
0.));
#192557=CARTESIAN_POINT('Ctrl Pts',(1.70345121691259,-23.1718954368749,
12.));
#192558=CARTESIAN_POINT('Ctrl Pts',(1.70063948926987,-23.1881832981848,
0.));
#192559=CARTESIAN_POINT('Ctrl Pts',(1.70063948926987,-23.1881832981848,
12.));
#192560=CARTESIAN_POINT('Ctrl Pts',(1.69775635099425,-23.2045972243765,
0.));
#192561=CARTESIAN_POINT('Ctrl Pts',(1.69775635099425,-23.2045972243765,
12.));
#192562=CARTESIAN_POINT('Ctrl Pts',(1.69480141959945,-23.2211357709374,
0.));
#192563=CARTESIAN_POINT('Ctrl Pts',(1.69480141959945,-23.2211357709374,
12.));
#192564=CARTESIAN_POINT('Ctrl Pts',(1.69177432121716,-23.2377975177014,
0.));
#192565=CARTESIAN_POINT('Ctrl Pts',(1.69177432121716,-23.2377975177014,
12.));
#192566=CARTESIAN_POINT('Ctrl Pts',(1.6886746903491,-23.2545810680536,0.));
#192567=CARTESIAN_POINT('Ctrl Pts',(1.6886746903491,-23.2545810680536,12.));
#192568=CARTESIAN_POINT('Ctrl Pts',(1.68550216963274,-23.2714850482245,
0.));
#192569=CARTESIAN_POINT('Ctrl Pts',(1.68550216963274,-23.2714850482245,
12.));
#192570=CARTESIAN_POINT('Ctrl Pts',(1.68225640962181,-23.2885081066949,
0.));
#192571=CARTESIAN_POINT('Ctrl Pts',(1.68225640962181,-23.2885081066949,
12.));
#192572=CARTESIAN_POINT('Ctrl Pts',(1.67893706857123,-23.3056489135611,
0.));
#192573=CARTESIAN_POINT('Ctrl Pts',(1.67893706857123,-23.3056489135611,
12.));
#192574=CARTESIAN_POINT('Ctrl Pts',(1.67554381222987,-23.3229061599145,
0.));
#192575=CARTESIAN_POINT('Ctrl Pts',(1.67554381222987,-23.3229061599145,
12.));
#192576=CARTESIAN_POINT('Ctrl Pts',(1.67207631363905,-23.3402785571866,
0.));
#192577=CARTESIAN_POINT('Ctrl Pts',(1.67207631363905,-23.3402785571866,
12.));
#192578=CARTESIAN_POINT('Ctrl Pts',(1.66853425293977,-23.3577648365747,
0.));
#192579=CARTESIAN_POINT('Ctrl Pts',(1.66853425293977,-23.3577648365747,
12.));
#192580=CARTESIAN_POINT('Ctrl Pts',(1.66491731718864,-23.375363748555,0.));
#192581=CARTESIAN_POINT('Ctrl Pts',(1.66491731718864,-23.375363748555,12.));
#192582=CARTESIAN_POINT('Ctrl Pts',(1.66122520018008,-23.3930740623622,
0.));
#192583=CARTESIAN_POINT('Ctrl Pts',(1.66122520018008,-23.3930740623622,
12.));
#192584=CARTESIAN_POINT('Ctrl Pts',(1.65745760227507,-23.4108945654803,
0.));
#192585=CARTESIAN_POINT('Ctrl Pts',(1.65745760227507,-23.4108945654803,
12.));
#192586=CARTESIAN_POINT('Ctrl Pts',(1.6536142302373,-23.4288240631034,0.));
#192587=CARTESIAN_POINT('Ctrl Pts',(1.6536142302373,-23.4288240631034,12.));
#192588=CARTESIAN_POINT('Ctrl Pts',(1.64969479707339,-23.446861377656,0.));
#192589=CARTESIAN_POINT('Ctrl Pts',(1.64969479707339,-23.446861377656,12.));
#192590=CARTESIAN_POINT('Ctrl Pts',(1.64569902187608,-23.4650053483919,
0.));
#192591=CARTESIAN_POINT('Ctrl Pts',(1.64569902187608,-23.4650053483919,
12.));
#192592=CARTESIAN_POINT('Ctrl Pts',(1.64162662967524,-23.4832548309638,
0.));
#192593=CARTESIAN_POINT('Ctrl Pts',(1.64162662967524,-23.4832548309638,
12.));
#192594=CARTESIAN_POINT('Ctrl Pts',(1.63747735129474,-23.5016086970006,
0.));
#192595=CARTESIAN_POINT('Ctrl Pts',(1.63747735129474,-23.5016086970006,
12.));
#192596=CARTESIAN_POINT('Ctrl Pts',(1.63325092321731,-23.5200658336624,
0.));
#192597=CARTESIAN_POINT('Ctrl Pts',(1.63325092321731,-23.5200658336624,
12.));
#192598=CARTESIAN_POINT('Ctrl Pts',(1.62894708745231,-23.5386251432278,
0.));
#192599=CARTESIAN_POINT('Ctrl Pts',(1.62894708745231,-23.5386251432278,
12.));
#192600=CARTESIAN_POINT('Ctrl Pts',(1.62456559140071,-23.5572855427617,
0.));
#192601=CARTESIAN_POINT('Ctrl Pts',(1.62456559140071,-23.5572855427617,
12.));
#192602=CARTESIAN_POINT('Ctrl Pts',(1.62010618772869,-23.5760459637608,
0.));
#192603=CARTESIAN_POINT('Ctrl Pts',(1.62010618772869,-23.5760459637608,
12.));
#192604=CARTESIAN_POINT('Ctrl Pts',(1.61556863424697,-23.5949053517996,
0.));
#192605=CARTESIAN_POINT('Ctrl Pts',(1.61556863424697,-23.5949053517996,
12.));
#192606=CARTESIAN_POINT('Ctrl Pts',(1.61095269379773,-23.6138626661644,
0.));
#192607=CARTESIAN_POINT('Ctrl Pts',(1.61095269379773,-23.6138626661644,
12.));
#192608=CARTESIAN_POINT('Ctrl Pts',(1.60625813414666,-23.6329168794916,
0.));
#192609=CARTESIAN_POINT('Ctrl Pts',(1.60625813414666,-23.6329168794916,
12.));
#192610=CARTESIAN_POINT('Ctrl Pts',(1.60148472786588,-23.6520669774863,
0.));
#192611=CARTESIAN_POINT('Ctrl Pts',(1.60148472786588,-23.6520669774863,
12.));
#192612=CARTESIAN_POINT('Ctrl Pts',(1.59663225222458,-23.6713119586302,
0.));
#192613=CARTESIAN_POINT('Ctrl Pts',(1.59663225222458,-23.6713119586302,
12.));
#192614=CARTESIAN_POINT('Ctrl Pts',(1.59170048908631,-23.6906508338833,
0.));
#192615=CARTESIAN_POINT('Ctrl Pts',(1.59170048908631,-23.6906508338833,
12.));
#192616=CARTESIAN_POINT('Ctrl Pts',(1.58668922481222,-23.7100826263835,
0.));
#192617=CARTESIAN_POINT('Ctrl Pts',(1.58668922481222,-23.7100826263835,
12.));
#192618=CARTESIAN_POINT('Ctrl Pts',(1.58159825017362,-23.7296063711308,
0.));
#192619=CARTESIAN_POINT('Ctrl Pts',(1.58159825017362,-23.7296063711308,
12.));
#192620=CARTESIAN_POINT('Ctrl Pts',(1.57642736025251,-23.7492211147369,
0.));
#192621=CARTESIAN_POINT('Ctrl Pts',(1.57642736025251,-23.7492211147369,
12.));
#192622=CARTESIAN_POINT('Ctrl Pts',(1.57117635434412,-23.7689259151869,
0.));
#192623=CARTESIAN_POINT('Ctrl Pts',(1.57117635434412,-23.7689259151869,
12.));
#192624=CARTESIAN_POINT('Ctrl Pts',(1.56584503586844,-23.788719841588,0.));
#192625=CARTESIAN_POINT('Ctrl Pts',(1.56584503586844,-23.788719841588,12.));
#192626=CARTESIAN_POINT('Ctrl Pts',(1.56043321228631,-23.8086019739192,
0.));
#192627=CARTESIAN_POINT('Ctrl Pts',(1.56043321228631,-23.8086019739192,
12.));
#192628=CARTESIAN_POINT('Ctrl Pts',(1.55494069502627,-23.8285714027631,
0.));
#192629=CARTESIAN_POINT('Ctrl Pts',(1.55494069502627,-23.8285714027631,
12.));
#192630=CARTESIAN_POINT('Ctrl Pts',(1.5493672994053,-23.8486272290698,0.));
#192631=CARTESIAN_POINT('Ctrl Pts',(1.5493672994053,-23.8486272290698,12.));
#192632=CARTESIAN_POINT('Ctrl Pts',(1.54371284453977,-23.8687685639635,
0.));
#192633=CARTESIAN_POINT('Ctrl Pts',(1.54371284453977,-23.8687685639635,
12.));
#192634=CARTESIAN_POINT('Ctrl Pts',(1.53797715326748,-23.8889945285313,
0.));
#192635=CARTESIAN_POINT('Ctrl Pts',(1.53797715326748,-23.8889945285313,
12.));
#192636=CARTESIAN_POINT('Ctrl Pts',(1.53216005207462,-23.9093042536119,
0.));
#192637=CARTESIAN_POINT('Ctrl Pts',(1.53216005207462,-23.9093042536119,
12.));
#192638=CARTESIAN_POINT('Ctrl Pts',(1.52626137103039,-23.9296968795761,
0.));
#192639=CARTESIAN_POINT('Ctrl Pts',(1.52626137103039,-23.9296968795761,
12.));
#192640=CARTESIAN_POINT('Ctrl Pts',(1.52028094372806,-23.9501715561038,
0.));
#192641=CARTESIAN_POINT('Ctrl Pts',(1.52028094372806,-23.9501715561038,
12.));
#192642=CARTESIAN_POINT('Ctrl Pts',(1.51421860720628,-23.9707274420145,
0.));
#192643=CARTESIAN_POINT('Ctrl Pts',(1.51421860720628,-23.9707274420145,
12.));
#192644=CARTESIAN_POINT('Ctrl Pts',(1.50807420187702,-23.991363705093,0.));
#192645=CARTESIAN_POINT('Ctrl Pts',(1.50807420187702,-23.991363705093,12.));
#192646=CARTESIAN_POINT('Ctrl Pts',(1.50184757146099,-24.0120795219086,
0.));
#192647=CARTESIAN_POINT('Ctrl Pts',(1.50184757146099,-24.0120795219086,
12.));
#192648=CARTESIAN_POINT('Ctrl Pts',(1.49553856292798,-24.0328740776331,
0.));
#192649=CARTESIAN_POINT('Ctrl Pts',(1.49553856292798,-24.0328740776331,
12.));
#192650=CARTESIAN_POINT('Ctrl Pts',(1.48914702644883,-24.053746565843,0.));
#192651=CARTESIAN_POINT('Ctrl Pts',(1.48914702644883,-24.053746565843,12.));
#192652=CARTESIAN_POINT('Ctrl Pts',(1.4826728153368,-24.074696188353,0.));
#192653=CARTESIAN_POINT('Ctrl Pts',(1.4826728153368,-24.074696188353,12.));
#192654=CARTESIAN_POINT('Ctrl Pts',(1.47611578597741,-24.0957221550782,
0.));
#192655=CARTESIAN_POINT('Ctrl Pts',(1.47611578597741,-24.0957221550782,
12.));
#192656=CARTESIAN_POINT('Ctrl Pts',(1.46947579776991,-24.1168236838827,
0.));
#192657=CARTESIAN_POINT('Ctrl Pts',(1.46947579776991,-24.1168236838827,
12.));
#192658=CARTESIAN_POINT('Ctrl Pts',(1.46275271307398,-24.1380000004272,
0.));
#192659=CARTESIAN_POINT('Ctrl Pts',(1.46275271307398,-24.1380000004272,
12.));
#192660=CARTESIAN_POINT('Ctrl Pts',(1.45594639716314,-24.1592503380105,
0.));
#192661=CARTESIAN_POINT('Ctrl Pts',(1.45594639716314,-24.1592503380105,
12.));
#192662=CARTESIAN_POINT('Ctrl Pts',(1.4490567181872,-24.1805739374033,0.));
#192663=CARTESIAN_POINT('Ctrl Pts',(1.4490567181872,-24.1805739374033,12.));
#192664=CARTESIAN_POINT('Ctrl Pts',(1.44208354711074,-24.2019700467214,
0.));
#192665=CARTESIAN_POINT('Ctrl Pts',(1.44208354711074,-24.2019700467214,
12.));
#192666=CARTESIAN_POINT('Ctrl Pts',(1.43502675765502,-24.2234379212978,
0.));
#192667=CARTESIAN_POINT('Ctrl Pts',(1.43502675765502,-24.2234379212978,
12.));
#192668=CARTESIAN_POINT('Ctrl Pts',(1.42788622624851,-24.2449768235485,
0.));
#192669=CARTESIAN_POINT('Ctrl Pts',(1.42788622624851,-24.2449768235485,
12.));
#192670=CARTESIAN_POINT('Ctrl Pts',(1.42066183198252,-24.2665860228357,
0.));
#192671=CARTESIAN_POINT('Ctrl Pts',(1.42066183198252,-24.2665860228357,
12.));
#192672=CARTESIAN_POINT('Ctrl Pts',(1.41335345657684,-24.2882647953214,
0.));
#192673=CARTESIAN_POINT('Ctrl Pts',(1.41335345657684,-24.2882647953214,
12.));
#192674=CARTESIAN_POINT('Ctrl Pts',(1.4059609843434,-24.3100124238316,0.));
#192675=CARTESIAN_POINT('Ctrl Pts',(1.4059609843434,-24.3100124238316,12.));
#192676=CARTESIAN_POINT('Ctrl Pts',(1.3984843021281,-24.3318281977647,0.));
#192677=CARTESIAN_POINT('Ctrl Pts',(1.3984843021281,-24.3318281977647,12.));
#192678=CARTESIAN_POINT('Ctrl Pts',(1.3909232992639,-24.3537114129877,0.));
#192679=CARTESIAN_POINT('Ctrl Pts',(1.3909232992639,-24.3537114129877,12.));
#192680=CARTESIAN_POINT('Ctrl Pts',(1.38327786752998,-24.37566137173,0.));
#192681=CARTESIAN_POINT('Ctrl Pts',(1.38327786752998,-24.37566137173,12.));
#192682=CARTESIAN_POINT('Ctrl Pts',(1.37554790111607,-24.3976773824731,
0.));
#192683=CARTESIAN_POINT('Ctrl Pts',(1.37554790111607,-24.3976773824731,
12.));
#192684=CARTESIAN_POINT('Ctrl Pts',(1.36773329659954,-24.4197587598337,
0.));
#192685=CARTESIAN_POINT('Ctrl Pts',(1.36773329659954,-24.4197587598337,
12.));
#192686=CARTESIAN_POINT('Ctrl Pts',(1.35983395290624,-24.4419048244524,
0.));
#192687=CARTESIAN_POINT('Ctrl Pts',(1.35983395290624,-24.4419048244524,
12.));
#192688=CARTESIAN_POINT('Ctrl Pts',(1.35184977125644,-24.4641149028894,
0.));
#192689=CARTESIAN_POINT('Ctrl Pts',(1.35184977125644,-24.4641149028894,
12.));
#192690=CARTESIAN_POINT('Ctrl Pts',(1.34378065512335,-24.4863883275135,
0.));
#192691=CARTESIAN_POINT('Ctrl Pts',(1.34378065512335,-24.4863883275135,
12.));
#192692=CARTESIAN_POINT('Ctrl Pts',(1.33562651019684,-24.5087244363856,
0.));
#192693=CARTESIAN_POINT('Ctrl Pts',(1.33562651019684,-24.5087244363856,
12.));
#192694=CARTESIAN_POINT('Ctrl Pts',(1.32738724435326,-24.5311225731434,
0.));
#192695=CARTESIAN_POINT('Ctrl Pts',(1.32738724435326,-24.5311225731434,
12.));
#192696=CARTESIAN_POINT('Ctrl Pts',(1.31906276763669,-24.5535820868671,
0.));
#192697=CARTESIAN_POINT('Ctrl Pts',(1.31906276763669,-24.5535820868671,
12.));
#192698=CARTESIAN_POINT('Ctrl Pts',(1.31065299222023,-24.576102332018,0.));
#192699=CARTESIAN_POINT('Ctrl Pts',(1.31065299222023,-24.576102332018,12.));
#192700=CARTESIAN_POINT('Ctrl Pts',(1.30215783236363,-24.5986826684025,
0.));
#192701=CARTESIAN_POINT('Ctrl Pts',(1.30215783236363,-24.5986826684025,
12.));
#192702=CARTESIAN_POINT('Ctrl Pts',(1.29357720438107,-24.6213224611228,
0.));
#192703=CARTESIAN_POINT('Ctrl Pts',(1.29357720438107,-24.6213224611228,
12.));
#192704=CARTESIAN_POINT('Ctrl Pts',(1.28491102661513,-24.6440210805278,
0.));
#192705=CARTESIAN_POINT('Ctrl Pts',(1.28491102661513,-24.6440210805278,
12.));
#192706=CARTESIAN_POINT('Ctrl Pts',(1.2761592194164,-24.666777902156,0.));
#192707=CARTESIAN_POINT('Ctrl Pts',(1.2761592194164,-24.666777902156,12.));
#192708=CARTESIAN_POINT('Ctrl Pts',(1.26732170513497,-24.6895923066837,
0.));
#192709=CARTESIAN_POINT('Ctrl Pts',(1.26732170513497,-24.6895923066837,
12.));
#192710=CARTESIAN_POINT('Ctrl Pts',(1.25839840807414,-24.7124636797895,
0.));
#192711=CARTESIAN_POINT('Ctrl Pts',(1.25839840807414,-24.7124636797895,
12.));
#192712=CARTESIAN_POINT('Ctrl Pts',(1.24938925444323,-24.7353914120012,
0.));
#192713=CARTESIAN_POINT('Ctrl Pts',(1.24938925444323,-24.7353914120012,
12.));
#192714=CARTESIAN_POINT('Ctrl Pts',(1.24029417231987,-24.7583748985439,
0.));
#192715=CARTESIAN_POINT('Ctrl Pts',(1.24029417231987,-24.7583748985439,
12.));
#192716=CARTESIAN_POINT('Ctrl Pts',(1.23111309161843,-24.78141353918,0.));
#192717=CARTESIAN_POINT('Ctrl Pts',(1.23111309161843,-24.78141353918,12.));
#192718=CARTESIAN_POINT('Ctrl Pts',(1.22184594406526,-24.8045067380536,
0.));
#192719=CARTESIAN_POINT('Ctrl Pts',(1.22184594406526,-24.8045067380536,
12.));
#192720=CARTESIAN_POINT('Ctrl Pts',(1.21249266318205,-24.8276539035092,
0.));
#192721=CARTESIAN_POINT('Ctrl Pts',(1.21249266318205,-24.8276539035092,
12.));
#192722=CARTESIAN_POINT('Ctrl Pts',(1.20305318426015,-24.8508544481973,
0.));
#192723=CARTESIAN_POINT('Ctrl Pts',(1.20305318426015,-24.8508544481973,
12.));
#192724=CARTESIAN_POINT('Ctrl Pts',(1.19352744434059,-24.8741077892074,
0.));
#192725=CARTESIAN_POINT('Ctrl Pts',(1.19352744434059,-24.8741077892074,
12.));
#192726=CARTESIAN_POINT('Ctrl Pts',(1.18391538220098,-24.8974133481829,
0.));
#192727=CARTESIAN_POINT('Ctrl Pts',(1.18391538220098,-24.8974133481829,
12.));
#192728=CARTESIAN_POINT('Ctrl Pts',(1.17421693835039,-24.9207705514449,
0.));
#192729=CARTESIAN_POINT('Ctrl Pts',(1.17421693835039,-24.9207705514449,
12.));
#192730=CARTESIAN_POINT('Ctrl Pts',(1.16443205502852,-24.9441788300932,
0.));
#192731=CARTESIAN_POINT('Ctrl Pts',(1.16443205502852,-24.9441788300932,
12.));
#192732=CARTESIAN_POINT('Ctrl Pts',(1.15456067621894,-24.9676376201501,
0.));
#192733=CARTESIAN_POINT('Ctrl Pts',(1.15456067621894,-24.9676376201501,
12.));
#192734=CARTESIAN_POINT('Ctrl Pts',(1.14460274758206,-24.9911463621431,
0.));
#192735=CARTESIAN_POINT('Ctrl Pts',(1.14460274758206,-24.9911463621431,
12.));
#192736=CARTESIAN_POINT('Ctrl Pts',(1.13455821638535,-25.0147045006193,
0.));
#192737=CARTESIAN_POINT('Ctrl Pts',(1.13455821638535,-25.0147045006193,
12.));
#192738=CARTESIAN_POINT('Ctrl Pts',(1.12442703144455,-25.0383114836898,
0.));
#192739=CARTESIAN_POINT('Ctrl Pts',(1.12442703144455,-25.0383114836898,
12.));
#192740=CARTESIAN_POINT('Ctrl Pts',(1.1142091430689,-25.0619667625336,0.));
#192741=CARTESIAN_POINT('Ctrl Pts',(1.1142091430689,-25.0619667625336,12.));
#192742=CARTESIAN_POINT('Ctrl Pts',(1.1039045030174,-25.085669790968,0.));
#192743=CARTESIAN_POINT('Ctrl Pts',(1.1039045030174,-25.085669790968,12.));
#192744=CARTESIAN_POINT('Ctrl Pts',(1.09351306445299,-25.1094200248448,
0.));
#192745=CARTESIAN_POINT('Ctrl Pts',(1.09351306445299,-25.1094200248448,
12.));
#192746=CARTESIAN_POINT('Ctrl Pts',(1.08303478197174,-25.1332169227415,
0.));
#192747=CARTESIAN_POINT('Ctrl Pts',(1.08303478197174,-25.1332169227415,
12.));
#192748=CARTESIAN_POINT('Ctrl Pts',(1.07246961165459,-25.1570599469311,
0.));
#192749=CARTESIAN_POINT('Ctrl Pts',(1.07246961165459,-25.1570599469311,
12.));
#192750=CARTESIAN_POINT('Ctrl Pts',(1.06181751111754,-25.1809485642191,
0.));
#192751=CARTESIAN_POINT('Ctrl Pts',(1.06181751111754,-25.1809485642191,
12.));
#192752=CARTESIAN_POINT('Ctrl Pts',(1.05107843957925,-25.2048822469027,
0.));
#192753=CARTESIAN_POINT('Ctrl Pts',(1.05107843957925,-25.2048822469027,
12.));
#192754=CARTESIAN_POINT('Ctrl Pts',(1.04025235791514,-25.2288604735087,
0.));
#192755=CARTESIAN_POINT('Ctrl Pts',(1.04025235791514,-25.2288604735087,
12.));
#192756=CARTESIAN_POINT('Ctrl Pts',(1.0293392287683,-25.2528827300427,0.));
#192757=CARTESIAN_POINT('Ctrl Pts',(1.0293392287683,-25.2528827300427,12.));
#192758=CARTESIAN_POINT('Ctrl Pts',(1.01833901642272,-25.2769485087268,
0.));
#192759=CARTESIAN_POINT('Ctrl Pts',(1.01833901642272,-25.2769485087268,
12.));
#192760=CARTESIAN_POINT('Ctrl Pts',(1.00725168656933,-25.3010573055557,
0.));
#192761=CARTESIAN_POINT('Ctrl Pts',(1.00725168656933,-25.3010573055557,
12.));
#192762=CARTESIAN_POINT('Ctrl Pts',(0.996077206120918,-25.3252086182976,
0.));
#192763=CARTESIAN_POINT('Ctrl Pts',(0.996077206120918,-25.3252086182976,
12.));
#192764=CARTESIAN_POINT('Ctrl Pts',(0.984815543004088,-25.3494019441444,
0.));
#192765=CARTESIAN_POINT('Ctrl Pts',(0.984815543004088,-25.3494019441444,
12.));
#192766=CARTESIAN_POINT('Ctrl Pts',(0.973466666000047,-25.3736367778842,
0.));
#192767=CARTESIAN_POINT('Ctrl Pts',(0.973466666000047,-25.3736367778842,
12.));
#192768=CARTESIAN_POINT('Ctrl Pts',(0.962030544502801,-25.3979126089155,
0.));
#192769=CARTESIAN_POINT('Ctrl Pts',(0.962030544502801,-25.3979126089155,
12.));
#192770=CARTESIAN_POINT('Ctrl Pts',(0.950507148596967,-25.4222289223155,
0.));
#192771=CARTESIAN_POINT('Ctrl Pts',(0.950507148596967,-25.4222289223155,
12.));
#192772=CARTESIAN_POINT('Ctrl Pts',(0.938896449495631,-25.4465852044835,
0.));
#192773=CARTESIAN_POINT('Ctrl Pts',(0.938896449495631,-25.4465852044835,
12.));
#192774=CARTESIAN_POINT('Ctrl Pts',(0.927198419885603,-25.4709809474996,
0.));
#192775=CARTESIAN_POINT('Ctrl Pts',(0.927198419885603,-25.4709809474996,
12.));
#192776=CARTESIAN_POINT('Ctrl Pts',(0.915413034335331,-25.4954156541787,
0.));
#192777=CARTESIAN_POINT('Ctrl Pts',(0.915413034335331,-25.4954156541787,
12.));
#192778=CARTESIAN_POINT('Ctrl Pts',(0.903540269651152,-25.5198888424195,
0.));
#192779=CARTESIAN_POINT('Ctrl Pts',(0.903540269651152,-25.5198888424195,
12.));
#192780=CARTESIAN_POINT('Ctrl Pts',(0.891580105349464,-25.5444000508223,
0.));
#192781=CARTESIAN_POINT('Ctrl Pts',(0.891580105349464,-25.5444000508223,
12.));
#192782=CARTESIAN_POINT('Ctrl Pts',(0.879532523835088,-25.568948840818,
0.));
#192783=CARTESIAN_POINT('Ctrl Pts',(0.879532523835088,-25.568948840818,
12.));
#192784=CARTESIAN_POINT('Ctrl Pts',(0.867397509339468,-25.5935347843616,
0.));
#192785=CARTESIAN_POINT('Ctrl Pts',(0.867397509339468,-25.5935347843616,
12.));
#192786=CARTESIAN_POINT('Ctrl Pts',(0.855175047037614,-25.618157453608,
0.));
#192787=CARTESIAN_POINT('Ctrl Pts',(0.855175047037614,-25.618157453608,
12.));
#192788=CARTESIAN_POINT('Ctrl Pts',(0.842865122121542,-25.6428164100078,
0.));
#192789=CARTESIAN_POINT('Ctrl Pts',(0.842865122121542,-25.6428164100078,
12.));
#192790=CARTESIAN_POINT('Ctrl Pts',(0.830467718864366,-25.6675111931957,
0.));
#192791=CARTESIAN_POINT('Ctrl Pts',(0.830467718864366,-25.6675111931957,
12.));
#192792=CARTESIAN_POINT('Ctrl Pts',(0.817982819786718,-25.6922413110172,
0.));
#192793=CARTESIAN_POINT('Ctrl Pts',(0.817982819786718,-25.6922413110172,
12.));
#192794=CARTESIAN_POINT('Ctrl Pts',(0.805410404552592,-25.7170062262474,
0.));
#192795=CARTESIAN_POINT('Ctrl Pts',(0.805410404552592,-25.7170062262474,
12.));
#192796=CARTESIAN_POINT('Ctrl Pts',(0.792750451613533,-25.7418053757671,
0.));
#192797=CARTESIAN_POINT('Ctrl Pts',(0.792750451613533,-25.7418053757671,
12.));
#192798=CARTESIAN_POINT('Ctrl Pts',(0.780002940289024,-25.7666381946871,
0.));
#192799=CARTESIAN_POINT('Ctrl Pts',(0.780002940289024,-25.7666381946871,
12.));
#192800=CARTESIAN_POINT('Ctrl Pts',(0.767167852648638,-25.7915041383304,
0.));
#192801=CARTESIAN_POINT('Ctrl Pts',(0.767167852648638,-25.7915041383304,
12.));
#192802=CARTESIAN_POINT('Ctrl Pts',(0.754245175608287,-25.816402705995,
0.));
#192803=CARTESIAN_POINT('Ctrl Pts',(0.754245175608287,-25.816402705995,
12.));
#192804=CARTESIAN_POINT('Ctrl Pts',(0.741234902664695,-25.841333461908,
0.));
#192805=CARTESIAN_POINT('Ctrl Pts',(0.741234902664695,-25.841333461908,
12.));
#192806=CARTESIAN_POINT('Ctrl Pts',(0.728137036485876,-25.8662960624285,
0.));
#192807=CARTESIAN_POINT('Ctrl Pts',(0.728137036485876,-25.8662960624285,
12.));
#192808=CARTESIAN_POINT('Ctrl Pts',(0.714951588533752,-25.8912902615141,
0.));
#192809=CARTESIAN_POINT('Ctrl Pts',(0.714951588533752,-25.8912902615141,
12.));
#192810=CARTESIAN_POINT('Ctrl Pts',(0.701678575236601,-25.9163158909645,
0.));
#192811=CARTESIAN_POINT('Ctrl Pts',(0.701678575236601,-25.9163158909645,
12.));
#192812=CARTESIAN_POINT('Ctrl Pts',(0.688318015065675,-25.941372847213,
0.));
#192813=CARTESIAN_POINT('Ctrl Pts',(0.688318015065675,-25.941372847213,
12.));
#192814=CARTESIAN_POINT('Ctrl Pts',(0.677559543215902,-25.9614434298092,
0.));
#192815=CARTESIAN_POINT('Ctrl Pts',(0.677559543215902,-25.9614434298092,
12.));
#192816=CARTESIAN_POINT('Ctrl Pts',(0.669451306784414,-25.9765104298171,
0.));
#192817=CARTESIAN_POINT('Ctrl Pts',(0.669451306784414,-25.9765104298171,
12.));
#192818=CARTESIAN_POINT('Ctrl Pts',(0.664028313188911,-25.9865613464809,
0.));
#192819=CARTESIAN_POINT('Ctrl Pts',(0.664028313188911,-25.9865613464809,
12.));
#192820=CARTESIAN_POINT('Ctrl Pts',(0.66131244073089,-25.991588367311,0.));
#192821=CARTESIAN_POINT('Ctrl Pts',(0.66131244073089,-25.991588367311,12.));
#192822=CARTESIAN_POINT('',(0.66131244073089,-25.991588367311,0.));
#192823=CARTESIAN_POINT('Ctrl Pts',(1.76341220531179,-22.4835757167854,
0.));
#192824=CARTESIAN_POINT('Ctrl Pts',(1.76341415538764,-22.483581992979,0.));
#192825=CARTESIAN_POINT('Ctrl Pts',(1.7634206426357,-22.4836387052232,0.));
#192826=CARTESIAN_POINT('Ctrl Pts',(1.76343813434565,-22.483856251707,0.));
#192827=CARTESIAN_POINT('Ctrl Pts',(1.76347698284791,-22.4844112933129,
0.));
#192828=CARTESIAN_POINT('Ctrl Pts',(1.76355076045546,-22.4855446605991,
0.));
#192829=CARTESIAN_POINT('Ctrl Pts',(1.76364784232963,-22.4871115206571,
0.));
#192830=CARTESIAN_POINT('Ctrl Pts',(1.76376424879504,-22.4890991659478,
0.));
#192831=CARTESIAN_POINT('Ctrl Pts',(1.76389475965723,-22.4914909094908,
0.));
#192832=CARTESIAN_POINT('Ctrl Pts',(1.764033938803,-22.4942693792449,0.));
#192833=CARTESIAN_POINT('Ctrl Pts',(1.76417731243462,-22.4974203063191,
0.));
#192834=CARTESIAN_POINT('Ctrl Pts',(1.76432160068725,-22.5009332677316,
0.));
#192835=CARTESIAN_POINT('Ctrl Pts',(1.76446408210366,-22.5047996391978,
0.));
#192836=CARTESIAN_POINT('Ctrl Pts',(1.76460218257323,-22.5090112700212,
0.));
#192837=CARTESIAN_POINT('Ctrl Pts',(1.76473303281158,-22.5135590569554,
0.));
#192838=CARTESIAN_POINT('Ctrl Pts',(1.76485369319896,-22.5184336670207,
0.));
#192839=CARTESIAN_POINT('Ctrl Pts',(1.76496128643369,-22.5236259635515,
0.));
#192840=CARTESIAN_POINT('Ctrl Pts',(1.76505320262751,-22.529127665298,0.));
#192841=CARTESIAN_POINT('Ctrl Pts',(1.7651271156325,-22.5349313983571,0.));
#192842=CARTESIAN_POINT('Ctrl Pts',(1.76518087841492,-22.5410303590891,
0.));
#192843=CARTESIAN_POINT('Ctrl Pts',(1.76521245524047,-22.5474180954006,
0.));
#192844=CARTESIAN_POINT('Ctrl Pts',(1.76521983384062,-22.5540882235837,
0.));
#192845=CARTESIAN_POINT('Ctrl Pts',(1.76520104500449,-22.5610344912501,
0.));
#192846=CARTESIAN_POINT('Ctrl Pts',(1.76515418518829,-22.5682508499873,
0.));
#192847=CARTESIAN_POINT('Ctrl Pts',(1.76507744026747,-22.5757315316355,
0.));
#192848=CARTESIAN_POINT('Ctrl Pts',(1.76496910283088,-22.5834711038024,
0.));
#192849=CARTESIAN_POINT('Ctrl Pts',(1.76482755288411,-22.5914644078106,
0.));
#192850=CARTESIAN_POINT('Ctrl Pts',(1.76465124413556,-22.5997065145638,
0.));
#192851=CARTESIAN_POINT('Ctrl Pts',(1.76443868648015,-22.6081926681342,
0.));
#192852=CARTESIAN_POINT('Ctrl Pts',(1.76418843543739,-22.6169182517693,
0.));
#192853=CARTESIAN_POINT('Ctrl Pts',(1.76389909571402,-22.6258787994847,
0.));
#192854=CARTESIAN_POINT('Ctrl Pts',(1.76356932176272,-22.635069997936,0.));
#192855=CARTESIAN_POINT('Ctrl Pts',(1.76319782013913,-22.6444876940425,
0.));
#192856=CARTESIAN_POINT('Ctrl Pts',(1.76278334912559,-22.6541278938413,
0.));
#192857=CARTESIAN_POINT('Ctrl Pts',(1.76232471392567,-22.6639867471756,
0.));
#192858=CARTESIAN_POINT('Ctrl Pts',(1.76182076289525,-22.6740605356699,
0.));
#192859=CARTESIAN_POINT('Ctrl Pts',(1.76127038310612,-22.6843456585245,
0.));
#192860=CARTESIAN_POINT('Ctrl Pts',(1.76067249704884,-22.6948386219843,
0.));
#192861=CARTESIAN_POINT('Ctrl Pts',(1.76002606202398,-22.7055360375481,
0.));
#192862=CARTESIAN_POINT('Ctrl Pts',(1.75933006905924,-22.7164346186007,
0.));
#192863=CARTESIAN_POINT('Ctrl Pts',(1.75858354204634,-22.7275311777305,
0.));
#192864=CARTESIAN_POINT('Ctrl Pts',(1.75778553673249,-22.7388226235565,
0.));
#192865=CARTESIAN_POINT('Ctrl Pts',(1.75693513908911,-22.7503059556455,
0.));
#192866=CARTESIAN_POINT('Ctrl Pts',(1.7560314637164,-22.7619782595013,0.));
#192867=CARTESIAN_POINT('Ctrl Pts',(1.75507365227127,-22.7738367016115,
0.));
#192868=CARTESIAN_POINT('Ctrl Pts',(1.75406087182929,-22.7858785242358,
0.));
#192869=CARTESIAN_POINT('Ctrl Pts',(1.75299231391461,-22.7981010424312,
0.));
#192870=CARTESIAN_POINT('Ctrl Pts',(1.75186719365589,-22.8105016414712,
0.));
#192871=CARTESIAN_POINT('Ctrl Pts',(1.75068474890883,-22.8230777741285,
0.));
#192872=CARTESIAN_POINT('Ctrl Pts',(1.74944423940117,-22.8358269579854,
0.));
#192873=CARTESIAN_POINT('Ctrl Pts',(1.74814494588491,-22.8487467728075,
0.));
#192874=CARTESIAN_POINT('Ctrl Pts',(1.74678616930663,-22.8618348580234,
0.));
#192875=CARTESIAN_POINT('Ctrl Pts',(1.74536722998199,-22.8750889101696,
0.));
#192876=CARTESIAN_POINT('Ctrl Pts',(1.74388746677702,-22.8885066803351,
0.));
#192877=CARTESIAN_POINT('Ctrl Pts',(1.74234623630079,-22.9020859716144,
0.));
#192878=CARTESIAN_POINT('Ctrl Pts',(1.74074291231056,-22.9158246373365,
0.));
#192879=CARTESIAN_POINT('Ctrl Pts',(1.73907688511664,-22.9297205792587,
0.));
#192880=CARTESIAN_POINT('Ctrl Pts',(1.73734756100038,-22.9437717457825,
0.));
#192881=CARTESIAN_POINT('Ctrl Pts',(1.73555436162771,-22.9579761301062,
0.));
#192882=CARTESIAN_POINT('Ctrl Pts',(1.73369672350817,-22.9723317685688,
0.));
#192883=CARTESIAN_POINT('Ctrl Pts',(1.73177409750193,-22.9868367391978,
0.));
#192884=CARTESIAN_POINT('Ctrl Pts',(1.72978594832137,-23.0014891601891,
0.));
#192885=CARTESIAN_POINT('Ctrl Pts',(1.72773175404702,-23.0162871884167,
0.));
#192886=CARTESIAN_POINT('Ctrl Pts',(1.72561100564033,-23.031229017888,0.));
#192887=CARTESIAN_POINT('Ctrl Pts',(1.72342320653731,-23.0463128785528,
0.));
#192888=CARTESIAN_POINT('Ctrl Pts',(1.7211678722598,-23.061537035156,0.));
#192889=CARTESIAN_POINT('Ctrl Pts',(1.71884453003027,-23.0768997860709,
0.));
#192890=CARTESIAN_POINT('Ctrl Pts',(1.71645271839311,-23.0923994621216,
0.));
#192891=CARTESIAN_POINT('Ctrl Pts',(1.71399198684724,-23.1080344254291,
0.));
#192892=CARTESIAN_POINT('Ctrl Pts',(1.71146189552192,-23.1238030684929,
0.));
#192893=CARTESIAN_POINT('Ctrl Pts',(1.70886201485459,-23.1397038132358,
0.));
#192894=CARTESIAN_POINT('Ctrl Pts',(1.70619192527846,-23.1557351100613,
0.));
#192895=CARTESIAN_POINT('Ctrl Pts',(1.70345121691259,-23.1718954368749,
0.));
#192896=CARTESIAN_POINT('Ctrl Pts',(1.70063948926987,-23.1881832981848,
0.));
#192897=CARTESIAN_POINT('Ctrl Pts',(1.69775635099425,-23.2045972243765,
0.));
#192898=CARTESIAN_POINT('Ctrl Pts',(1.69480141959945,-23.2211357709374,
0.));
#192899=CARTESIAN_POINT('Ctrl Pts',(1.69177432121716,-23.2377975177014,
0.));
#192900=CARTESIAN_POINT('Ctrl Pts',(1.6886746903491,-23.2545810680536,0.));
#192901=CARTESIAN_POINT('Ctrl Pts',(1.68550216963274,-23.2714850482245,
0.));
#192902=CARTESIAN_POINT('Ctrl Pts',(1.68225640962181,-23.2885081066949,
0.));
#192903=CARTESIAN_POINT('Ctrl Pts',(1.67893706857123,-23.3056489135611,
0.));
#192904=CARTESIAN_POINT('Ctrl Pts',(1.67554381222987,-23.3229061599145,
0.));
#192905=CARTESIAN_POINT('Ctrl Pts',(1.67207631363905,-23.3402785571866,
0.));
#192906=CARTESIAN_POINT('Ctrl Pts',(1.66853425293977,-23.3577648365747,
0.));
#192907=CARTESIAN_POINT('Ctrl Pts',(1.66491731718864,-23.375363748555,0.));
#192908=CARTESIAN_POINT('Ctrl Pts',(1.66122520018008,-23.3930740623622,
0.));
#192909=CARTESIAN_POINT('Ctrl Pts',(1.65745760227507,-23.4108945654803,
0.));
#192910=CARTESIAN_POINT('Ctrl Pts',(1.6536142302373,-23.4288240631034,0.));
#192911=CARTESIAN_POINT('Ctrl Pts',(1.64969479707339,-23.446861377656,0.));
#192912=CARTESIAN_POINT('Ctrl Pts',(1.64569902187608,-23.4650053483919,
0.));
#192913=CARTESIAN_POINT('Ctrl Pts',(1.64162662967524,-23.4832548309638,
0.));
#192914=CARTESIAN_POINT('Ctrl Pts',(1.63747735129474,-23.5016086970006,
0.));
#192915=CARTESIAN_POINT('Ctrl Pts',(1.63325092321731,-23.5200658336624,
0.));
#192916=CARTESIAN_POINT('Ctrl Pts',(1.62894708745231,-23.5386251432278,
0.));
#192917=CARTESIAN_POINT('Ctrl Pts',(1.62456559140071,-23.5572855427617,
0.));
#192918=CARTESIAN_POINT('Ctrl Pts',(1.62010618772869,-23.5760459637608,
0.));
#192919=CARTESIAN_POINT('Ctrl Pts',(1.61556863424697,-23.5949053517996,
0.));
#192920=CARTESIAN_POINT('Ctrl Pts',(1.61095269379773,-23.6138626661644,
0.));
#192921=CARTESIAN_POINT('Ctrl Pts',(1.60625813414666,-23.6329168794916,
0.));
#192922=CARTESIAN_POINT('Ctrl Pts',(1.60148472786588,-23.6520669774863,
0.));
#192923=CARTESIAN_POINT('Ctrl Pts',(1.59663225222458,-23.6713119586302,
0.));
#192924=CARTESIAN_POINT('Ctrl Pts',(1.59170048908631,-23.6906508338833,
0.));
#192925=CARTESIAN_POINT('Ctrl Pts',(1.58668922481222,-23.7100826263835,
0.));
#192926=CARTESIAN_POINT('Ctrl Pts',(1.58159825017362,-23.7296063711308,
0.));
#192927=CARTESIAN_POINT('Ctrl Pts',(1.57642736025251,-23.7492211147369,
0.));
#192928=CARTESIAN_POINT('Ctrl Pts',(1.57117635434412,-23.7689259151869,
0.));
#192929=CARTESIAN_POINT('Ctrl Pts',(1.56584503586844,-23.788719841588,0.));
#192930=CARTESIAN_POINT('Ctrl Pts',(1.56043321228631,-23.8086019739192,
0.));
#192931=CARTESIAN_POINT('Ctrl Pts',(1.55494069502627,-23.8285714027631,
0.));
#192932=CARTESIAN_POINT('Ctrl Pts',(1.5493672994053,-23.8486272290698,0.));
#192933=CARTESIAN_POINT('Ctrl Pts',(1.54371284453977,-23.8687685639635,
0.));
#192934=CARTESIAN_POINT('Ctrl Pts',(1.53797715326748,-23.8889945285313,
0.));
#192935=CARTESIAN_POINT('Ctrl Pts',(1.53216005207462,-23.9093042536119,
0.));
#192936=CARTESIAN_POINT('Ctrl Pts',(1.52626137103039,-23.9296968795761,
0.));
#192937=CARTESIAN_POINT('Ctrl Pts',(1.52028094372806,-23.9501715561038,
0.));
#192938=CARTESIAN_POINT('Ctrl Pts',(1.51421860720628,-23.9707274420145,
0.));
#192939=CARTESIAN_POINT('Ctrl Pts',(1.50807420187702,-23.991363705093,0.));
#192940=CARTESIAN_POINT('Ctrl Pts',(1.50184757146099,-24.0120795219086,
0.));
#192941=CARTESIAN_POINT('Ctrl Pts',(1.49553856292798,-24.0328740776331,
0.));
#192942=CARTESIAN_POINT('Ctrl Pts',(1.48914702644883,-24.053746565843,0.));
#192943=CARTESIAN_POINT('Ctrl Pts',(1.4826728153368,-24.074696188353,0.));
#192944=CARTESIAN_POINT('Ctrl Pts',(1.47611578597741,-24.0957221550782,
0.));
#192945=CARTESIAN_POINT('Ctrl Pts',(1.46947579776991,-24.1168236838827,
0.));
#192946=CARTESIAN_POINT('Ctrl Pts',(1.46275271307398,-24.1380000004272,
0.));
#192947=CARTESIAN_POINT('Ctrl Pts',(1.45594639716314,-24.1592503380105,
0.));
#192948=CARTESIAN_POINT('Ctrl Pts',(1.4490567181872,-24.1805739374033,0.));
#192949=CARTESIAN_POINT('Ctrl Pts',(1.44208354711074,-24.2019700467214,
0.));
#192950=CARTESIAN_POINT('Ctrl Pts',(1.43502675765502,-24.2234379212978,
0.));
#192951=CARTESIAN_POINT('Ctrl Pts',(1.42788622624851,-24.2449768235485,
0.));
#192952=CARTESIAN_POINT('Ctrl Pts',(1.42066183198252,-24.2665860228357,
0.));
#192953=CARTESIAN_POINT('Ctrl Pts',(1.41335345657684,-24.2882647953214,
0.));
#192954=CARTESIAN_POINT('Ctrl Pts',(1.4059609843434,-24.3100124238316,0.));
#192955=CARTESIAN_POINT('Ctrl Pts',(1.3984843021281,-24.3318281977647,0.));
#192956=CARTESIAN_POINT('Ctrl Pts',(1.3909232992639,-24.3537114129877,0.));
#192957=CARTESIAN_POINT('Ctrl Pts',(1.38327786752998,-24.37566137173,0.));
#192958=CARTESIAN_POINT('Ctrl Pts',(1.37554790111607,-24.3976773824731,
0.));
#192959=CARTESIAN_POINT('Ctrl Pts',(1.36773329659954,-24.4197587598337,
0.));
#192960=CARTESIAN_POINT('Ctrl Pts',(1.35983395290624,-24.4419048244524,
0.));
#192961=CARTESIAN_POINT('Ctrl Pts',(1.35184977125644,-24.4641149028894,
0.));
#192962=CARTESIAN_POINT('Ctrl Pts',(1.34378065512335,-24.4863883275135,
0.));
#192963=CARTESIAN_POINT('Ctrl Pts',(1.33562651019684,-24.5087244363856,
0.));
#192964=CARTESIAN_POINT('Ctrl Pts',(1.32738724435326,-24.5311225731434,
0.));
#192965=CARTESIAN_POINT('Ctrl Pts',(1.31906276763669,-24.5535820868671,
0.));
#192966=CARTESIAN_POINT('Ctrl Pts',(1.31065299222023,-24.576102332018,0.));
#192967=CARTESIAN_POINT('Ctrl Pts',(1.30215783236363,-24.5986826684025,
0.));
#192968=CARTESIAN_POINT('Ctrl Pts',(1.29357720438107,-24.6213224611228,
0.));
#192969=CARTESIAN_POINT('Ctrl Pts',(1.28491102661513,-24.6440210805278,
0.));
#192970=CARTESIAN_POINT('Ctrl Pts',(1.2761592194164,-24.666777902156,0.));
#192971=CARTESIAN_POINT('Ctrl Pts',(1.26732170513497,-24.6895923066837,
0.));
#192972=CARTESIAN_POINT('Ctrl Pts',(1.25839840807414,-24.7124636797895,
0.));
#192973=CARTESIAN_POINT('Ctrl Pts',(1.24938925444323,-24.7353914120012,
0.));
#192974=CARTESIAN_POINT('Ctrl Pts',(1.24029417231987,-24.7583748985439,
0.));
#192975=CARTESIAN_POINT('Ctrl Pts',(1.23111309161843,-24.78141353918,0.));
#192976=CARTESIAN_POINT('Ctrl Pts',(1.22184594406526,-24.8045067380536,
0.));
#192977=CARTESIAN_POINT('Ctrl Pts',(1.21249266318205,-24.8276539035092,
0.));
#192978=CARTESIAN_POINT('Ctrl Pts',(1.20305318426015,-24.8508544481973,
0.));
#192979=CARTESIAN_POINT('Ctrl Pts',(1.19352744434059,-24.8741077892074,
0.));
#192980=CARTESIAN_POINT('Ctrl Pts',(1.18391538220098,-24.8974133481829,
0.));
#192981=CARTESIAN_POINT('Ctrl Pts',(1.17421693835039,-24.9207705514449,
0.));
#192982=CARTESIAN_POINT('Ctrl Pts',(1.16443205502852,-24.9441788300932,
0.));
#192983=CARTESIAN_POINT('Ctrl Pts',(1.15456067621894,-24.9676376201501,
0.));
#192984=CARTESIAN_POINT('Ctrl Pts',(1.14460274758206,-24.9911463621431,
0.));
#192985=CARTESIAN_POINT('Ctrl Pts',(1.13455821638535,-25.0147045006193,
0.));
#192986=CARTESIAN_POINT('Ctrl Pts',(1.12442703144455,-25.0383114836898,
0.));
#192987=CARTESIAN_POINT('Ctrl Pts',(1.1142091430689,-25.0619667625336,0.));
#192988=CARTESIAN_POINT('Ctrl Pts',(1.1039045030174,-25.085669790968,0.));
#192989=CARTESIAN_POINT('Ctrl Pts',(1.09351306445299,-25.1094200248448,
0.));
#192990=CARTESIAN_POINT('Ctrl Pts',(1.08303478197174,-25.1332169227415,
0.));
#192991=CARTESIAN_POINT('Ctrl Pts',(1.07246961165459,-25.1570599469311,
0.));
#192992=CARTESIAN_POINT('Ctrl Pts',(1.06181751111754,-25.1809485642191,
0.));
#192993=CARTESIAN_POINT('Ctrl Pts',(1.05107843957925,-25.2048822469027,
0.));
#192994=CARTESIAN_POINT('Ctrl Pts',(1.04025235791514,-25.2288604735087,
0.));
#192995=CARTESIAN_POINT('Ctrl Pts',(1.0293392287683,-25.2528827300427,0.));
#192996=CARTESIAN_POINT('Ctrl Pts',(1.01833901642272,-25.2769485087268,
0.));
#192997=CARTESIAN_POINT('Ctrl Pts',(1.00725168656933,-25.3010573055557,
0.));
#192998=CARTESIAN_POINT('Ctrl Pts',(0.996077206120918,-25.3252086182976,
0.));
#192999=CARTESIAN_POINT('Ctrl Pts',(0.984815543004088,-25.3494019441444,
0.));
#193000=CARTESIAN_POINT('Ctrl Pts',(0.973466666000047,-25.3736367778842,
0.));
#193001=CARTESIAN_POINT('Ctrl Pts',(0.962030544502801,-25.3979126089155,
0.));
#193002=CARTESIAN_POINT('Ctrl Pts',(0.950507148596967,-25.4222289223155,
0.));
#193003=CARTESIAN_POINT('Ctrl Pts',(0.938896449495631,-25.4465852044835,
0.));
#193004=CARTESIAN_POINT('Ctrl Pts',(0.927198419885603,-25.4709809474996,
0.));
#193005=CARTESIAN_POINT('Ctrl Pts',(0.915413034335331,-25.4954156541787,
0.));
#193006=CARTESIAN_POINT('Ctrl Pts',(0.903540269651152,-25.5198888424195,
0.));
#193007=CARTESIAN_POINT('Ctrl Pts',(0.891580105349464,-25.5444000508223,
0.));
#193008=CARTESIAN_POINT('Ctrl Pts',(0.879532523835088,-25.568948840818,
0.));
#193009=CARTESIAN_POINT('Ctrl Pts',(0.867397509339468,-25.5935347843616,
0.));
#193010=CARTESIAN_POINT('Ctrl Pts',(0.855175047037614,-25.618157453608,
0.));
#193011=CARTESIAN_POINT('Ctrl Pts',(0.842865122121542,-25.6428164100078,
0.));
#193012=CARTESIAN_POINT('Ctrl Pts',(0.830467718864366,-25.6675111931957,
0.));
#193013=CARTESIAN_POINT('Ctrl Pts',(0.817982819786718,-25.6922413110172,
0.));
#193014=CARTESIAN_POINT('Ctrl Pts',(0.805410404552592,-25.7170062262474,
0.));
#193015=CARTESIAN_POINT('Ctrl Pts',(0.792750451613533,-25.7418053757671,
0.));
#193016=CARTESIAN_POINT('Ctrl Pts',(0.780002940289024,-25.7666381946871,
0.));
#193017=CARTESIAN_POINT('Ctrl Pts',(0.767167852648638,-25.7915041383304,
0.));
#193018=CARTESIAN_POINT('Ctrl Pts',(0.754245175608287,-25.816402705995,
0.));
#193019=CARTESIAN_POINT('Ctrl Pts',(0.741234902664695,-25.841333461908,
0.));
#193020=CARTESIAN_POINT('Ctrl Pts',(0.728137036485876,-25.8662960624285,
0.));
#193021=CARTESIAN_POINT('Ctrl Pts',(0.714951588533752,-25.8912902615141,
0.));
#193022=CARTESIAN_POINT('Ctrl Pts',(0.701678575236601,-25.9163158909645,
0.));
#193023=CARTESIAN_POINT('Ctrl Pts',(0.688318015065675,-25.941372847213,
0.));
#193024=CARTESIAN_POINT('Ctrl Pts',(0.677559543215902,-25.9614434298092,
0.));
#193025=CARTESIAN_POINT('Ctrl Pts',(0.669451306784414,-25.9765104298171,
0.));
#193026=CARTESIAN_POINT('Ctrl Pts',(0.664028313188911,-25.9865613464809,
0.));
#193027=CARTESIAN_POINT('Ctrl Pts',(0.66131244073089,-25.991588367311,0.));
#193028=CARTESIAN_POINT('',(0.66131244073089,-25.991588367311,0.));
#193029=CARTESIAN_POINT('Origin',(-3.92374859571502,-21.1389261070099,0.));
#193030=CARTESIAN_POINT('',(-4.11585220600463,-22.1738711152697,0.));
#193031=CARTESIAN_POINT('',(-4.11585220600463,-22.1738711152697,0.));
#193032=CARTESIAN_POINT('',(-1.96187429785751,-10.5694630535049,0.));
#193033=CARTESIAN_POINT('Ctrl Pts',(-0.661312440730913,-25.991588367311,
0.));
#193034=CARTESIAN_POINT('Ctrl Pts',(-0.661312440730913,-25.991588367311,
12.));
#193035=CARTESIAN_POINT('Ctrl Pts',(-0.664028313187638,-25.9865613464773,
0.));
#193036=CARTESIAN_POINT('Ctrl Pts',(-0.664028313187638,-25.9865613464773,
12.));
#193037=CARTESIAN_POINT('Ctrl Pts',(-0.669451306780837,-25.9765104298071,
0.));
#193038=CARTESIAN_POINT('Ctrl Pts',(-0.669451306780837,-25.9765104298071,
12.));
#193039=CARTESIAN_POINT('Ctrl Pts',(-0.677559543209739,-25.9614434297919,
0.));
#193040=CARTESIAN_POINT('Ctrl Pts',(-0.677559543209739,-25.9614434297919,
12.));
#193041=CARTESIAN_POINT('Ctrl Pts',(-0.688318015057743,-25.9413728471909,
0.));
#193042=CARTESIAN_POINT('Ctrl Pts',(-0.688318015057743,-25.9413728471909,
12.));
#193043=CARTESIAN_POINT('Ctrl Pts',(-0.701678575228768,-25.9163158909426,
0.));
#193044=CARTESIAN_POINT('Ctrl Pts',(-0.701678575228768,-25.9163158909426,
12.));
#193045=CARTESIAN_POINT('Ctrl Pts',(-0.714951588527651,-25.891290261497,
0.));
#193046=CARTESIAN_POINT('Ctrl Pts',(-0.714951588527651,-25.891290261497,
12.));
#193047=CARTESIAN_POINT('Ctrl Pts',(-0.728137036482348,-25.8662960624185,
0.));
#193048=CARTESIAN_POINT('Ctrl Pts',(-0.728137036482348,-25.8662960624185,
12.));
#193049=CARTESIAN_POINT('Ctrl Pts',(-0.741234902663818,-25.8413334619055,
0.));
#193050=CARTESIAN_POINT('Ctrl Pts',(-0.741234902663818,-25.8413334619055,
12.));
#193051=CARTESIAN_POINT('Ctrl Pts',(-0.754245175609535,-25.8164027059984,
0.));
#193052=CARTESIAN_POINT('Ctrl Pts',(-0.754245175609535,-25.8164027059984,
12.));
#193053=CARTESIAN_POINT('Ctrl Pts',(-0.76716785265118,-25.7915041383376,
0.));
#193054=CARTESIAN_POINT('Ctrl Pts',(-0.76716785265118,-25.7915041383376,
12.));
#193055=CARTESIAN_POINT('Ctrl Pts',(-0.780002940291976,-25.7666381946955,
0.));
#193056=CARTESIAN_POINT('Ctrl Pts',(-0.780002940291976,-25.7666381946955,
12.));
#193057=CARTESIAN_POINT('Ctrl Pts',(-0.792750451616139,-25.7418053757746,
0.));
#193058=CARTESIAN_POINT('Ctrl Pts',(-0.792750451616139,-25.7418053757746,
12.));
#193059=CARTESIAN_POINT('Ctrl Pts',(-0.805410404554365,-25.7170062262525,
0.));
#193060=CARTESIAN_POINT('Ctrl Pts',(-0.805410404554365,-25.7170062262525,
12.));
#193061=CARTESIAN_POINT('Ctrl Pts',(-0.817982819787476,-25.6922413110194,
0.));
#193062=CARTESIAN_POINT('Ctrl Pts',(-0.817982819787476,-25.6922413110194,
12.));
#193063=CARTESIAN_POINT('Ctrl Pts',(-0.830467718864218,-25.6675111931952,
0.));
#193064=CARTESIAN_POINT('Ctrl Pts',(-0.830467718864218,-25.6675111931952,
12.));
#193065=CARTESIAN_POINT('Ctrl Pts',(-0.842865122120771,-25.6428164100055,
0.));
#193066=CARTESIAN_POINT('Ctrl Pts',(-0.842865122120771,-25.6428164100055,
12.));
#193067=CARTESIAN_POINT('Ctrl Pts',(-0.85517504703656,-25.6181574536049,
0.));
#193068=CARTESIAN_POINT('Ctrl Pts',(-0.85517504703656,-25.6181574536049,
12.));
#193069=CARTESIAN_POINT('Ctrl Pts',(-0.867397509338443,-25.5935347843585,
0.));
#193070=CARTESIAN_POINT('Ctrl Pts',(-0.867397509338443,-25.5935347843585,
12.));
#193071=CARTESIAN_POINT('Ctrl Pts',(-0.879532523834307,-25.5689488408156,
0.));
#193072=CARTESIAN_POINT('Ctrl Pts',(-0.879532523834307,-25.5689488408156,
12.));
#193073=CARTESIAN_POINT('Ctrl Pts',(-0.891580105349052,-25.5444000508211,
0.));
#193074=CARTESIAN_POINT('Ctrl Pts',(-0.891580105349052,-25.5444000508211,
12.));
#193075=CARTESIAN_POINT('Ctrl Pts',(-0.903540269651119,-25.5198888424194,
0.));
#193076=CARTESIAN_POINT('Ctrl Pts',(-0.903540269651119,-25.5198888424194,
12.));
#193077=CARTESIAN_POINT('Ctrl Pts',(-0.915413034335626,-25.4954156541795,
0.));
#193078=CARTESIAN_POINT('Ctrl Pts',(-0.915413034335626,-25.4954156541795,
12.));
#193079=CARTESIAN_POINT('Ctrl Pts',(-0.927198419886107,-25.4709809475009,
0.));
#193080=CARTESIAN_POINT('Ctrl Pts',(-0.927198419886107,-25.4709809475009,
12.));
#193081=CARTESIAN_POINT('Ctrl Pts',(-0.938896449496205,-25.4465852044849,
0.));
#193082=CARTESIAN_POINT('Ctrl Pts',(-0.938896449496205,-25.4465852044849,
12.));
#193083=CARTESIAN_POINT('Ctrl Pts',(-0.950507148597481,-25.4222289223167,
0.));
#193084=CARTESIAN_POINT('Ctrl Pts',(-0.950507148597481,-25.4222289223167,
12.));
#193085=CARTESIAN_POINT('Ctrl Pts',(-0.962030544503155,-25.3979126089163,
0.));
#193086=CARTESIAN_POINT('Ctrl Pts',(-0.962030544503155,-25.3979126089163,
12.));
#193087=CARTESIAN_POINT('Ctrl Pts',(-0.973466666000176,-25.3736367778845,
0.));
#193088=CARTESIAN_POINT('Ctrl Pts',(-0.973466666000176,-25.3736367778845,
12.));
#193089=CARTESIAN_POINT('Ctrl Pts',(-0.984815543003984,-25.3494019441441,
0.));
#193090=CARTESIAN_POINT('Ctrl Pts',(-0.984815543003984,-25.3494019441441,
12.));
#193091=CARTESIAN_POINT('Ctrl Pts',(-0.996077206120636,-25.3252086182968,
0.));
#193092=CARTESIAN_POINT('Ctrl Pts',(-0.996077206120636,-25.3252086182968,
12.));
#193093=CARTESIAN_POINT('Ctrl Pts',(-1.00725168656897,-25.3010573055548,
0.));
#193094=CARTESIAN_POINT('Ctrl Pts',(-1.00725168656897,-25.3010573055548,
12.));
#193095=CARTESIAN_POINT('Ctrl Pts',(-1.01833901642238,-25.276948508726,
0.));
#193096=CARTESIAN_POINT('Ctrl Pts',(-1.01833901642238,-25.276948508726,
12.));
#193097=CARTESIAN_POINT('Ctrl Pts',(-1.02933922876807,-25.2528827300422,
0.));
#193098=CARTESIAN_POINT('Ctrl Pts',(-1.02933922876807,-25.2528827300422,
12.));
#193099=CARTESIAN_POINT('Ctrl Pts',(-1.04025235791508,-25.2288604735086,
0.));
#193100=CARTESIAN_POINT('Ctrl Pts',(-1.04025235791508,-25.2288604735086,
12.));
#193101=CARTESIAN_POINT('Ctrl Pts',(-1.05107843957933,-25.2048822469028,
0.));
#193102=CARTESIAN_POINT('Ctrl Pts',(-1.05107843957933,-25.2048822469028,
12.));
#193103=CARTESIAN_POINT('Ctrl Pts',(-1.06181751111769,-25.1809485642192,
0.));
#193104=CARTESIAN_POINT('Ctrl Pts',(-1.06181751111769,-25.1809485642192,
12.));
#193105=CARTESIAN_POINT('Ctrl Pts',(-1.07246961165477,-25.157059946931,
0.));
#193106=CARTESIAN_POINT('Ctrl Pts',(-1.07246961165477,-25.157059946931,
12.));
#193107=CARTESIAN_POINT('Ctrl Pts',(-1.08303478197189,-25.1332169227413,
0.));
#193108=CARTESIAN_POINT('Ctrl Pts',(-1.08303478197189,-25.1332169227413,
12.));
#193109=CARTESIAN_POINT('Ctrl Pts',(-1.09351306445309,-25.1094200248446,
0.));
#193110=CARTESIAN_POINT('Ctrl Pts',(-1.09351306445309,-25.1094200248446,
12.));
#193111=CARTESIAN_POINT('Ctrl Pts',(-1.10390450301746,-25.0856697909679,
0.));
#193112=CARTESIAN_POINT('Ctrl Pts',(-1.10390450301746,-25.0856697909679,
12.));
#193113=CARTESIAN_POINT('Ctrl Pts',(-1.1142091430689,-25.0619667625336,
0.));
#193114=CARTESIAN_POINT('Ctrl Pts',(-1.1142091430689,-25.0619667625336,
12.));
#193115=CARTESIAN_POINT('Ctrl Pts',(-1.12442703144453,-25.0383114836899,
0.));
#193116=CARTESIAN_POINT('Ctrl Pts',(-1.12442703144453,-25.0383114836899,
12.));
#193117=CARTESIAN_POINT('Ctrl Pts',(-1.13455821638531,-25.0147045006196,
0.));
#193118=CARTESIAN_POINT('Ctrl Pts',(-1.13455821638531,-25.0147045006196,
12.));
#193119=CARTESIAN_POINT('Ctrl Pts',(-1.14460274758202,-24.9911463621433,
0.));
#193120=CARTESIAN_POINT('Ctrl Pts',(-1.14460274758202,-24.9911463621433,
12.));
#193121=CARTESIAN_POINT('Ctrl Pts',(-1.1545606762189,-24.9676376201502,
0.));
#193122=CARTESIAN_POINT('Ctrl Pts',(-1.1545606762189,-24.9676376201502,
12.));
#193123=CARTESIAN_POINT('Ctrl Pts',(-1.16443205502851,-24.9441788300932,
0.));
#193124=CARTESIAN_POINT('Ctrl Pts',(-1.16443205502851,-24.9441788300932,
12.));
#193125=CARTESIAN_POINT('Ctrl Pts',(-1.17421693835042,-24.9207705514448,
0.));
#193126=CARTESIAN_POINT('Ctrl Pts',(-1.17421693835042,-24.9207705514448,
12.));
#193127=CARTESIAN_POINT('Ctrl Pts',(-1.18391538220104,-24.8974133481829,
0.));
#193128=CARTESIAN_POINT('Ctrl Pts',(-1.18391538220104,-24.8974133481829,
12.));
#193129=CARTESIAN_POINT('Ctrl Pts',(-1.19352744434065,-24.8741077892075,
0.));
#193130=CARTESIAN_POINT('Ctrl Pts',(-1.19352744434065,-24.8741077892075,
12.));
#193131=CARTESIAN_POINT('Ctrl Pts',(-1.20305318426021,-24.8508544481974,
0.));
#193132=CARTESIAN_POINT('Ctrl Pts',(-1.20305318426021,-24.8508544481974,
12.));
#193133=CARTESIAN_POINT('Ctrl Pts',(-1.21249266318209,-24.8276539035092,
0.));
#193134=CARTESIAN_POINT('Ctrl Pts',(-1.21249266318209,-24.8276539035092,
12.));
#193135=CARTESIAN_POINT('Ctrl Pts',(-1.22184594406529,-24.8045067380536,
0.));
#193136=CARTESIAN_POINT('Ctrl Pts',(-1.22184594406529,-24.8045067380536,
12.));
#193137=CARTESIAN_POINT('Ctrl Pts',(-1.23111309161845,-24.7814135391799,
0.));
#193138=CARTESIAN_POINT('Ctrl Pts',(-1.23111309161845,-24.7814135391799,
12.));
#193139=CARTESIAN_POINT('Ctrl Pts',(-1.2402941723199,-24.7583748985438,
0.));
#193140=CARTESIAN_POINT('Ctrl Pts',(-1.2402941723199,-24.7583748985438,
12.));
#193141=CARTESIAN_POINT('Ctrl Pts',(-1.24938925444327,-24.7353914120011,
0.));
#193142=CARTESIAN_POINT('Ctrl Pts',(-1.24938925444327,-24.7353914120011,
12.));
#193143=CARTESIAN_POINT('Ctrl Pts',(-1.25839840807419,-24.7124636797894,
0.));
#193144=CARTESIAN_POINT('Ctrl Pts',(-1.25839840807419,-24.7124636797894,
12.));
#193145=CARTESIAN_POINT('Ctrl Pts',(-1.26732170513501,-24.6895923066836,
0.));
#193146=CARTESIAN_POINT('Ctrl Pts',(-1.26732170513501,-24.6895923066836,
12.));
#193147=CARTESIAN_POINT('Ctrl Pts',(-1.27615921941643,-24.6667779021559,
0.));
#193148=CARTESIAN_POINT('Ctrl Pts',(-1.27615921941643,-24.6667779021559,
12.));
#193149=CARTESIAN_POINT('Ctrl Pts',(-1.28491102661515,-24.6440210805278,
0.));
#193150=CARTESIAN_POINT('Ctrl Pts',(-1.28491102661515,-24.6440210805278,
12.));
#193151=CARTESIAN_POINT('Ctrl Pts',(-1.29357720438108,-24.6213224611229,
0.));
#193152=CARTESIAN_POINT('Ctrl Pts',(-1.29357720438108,-24.6213224611229,
12.));
#193153=CARTESIAN_POINT('Ctrl Pts',(-1.30215783236363,-24.5986826684027,
0.));
#193154=CARTESIAN_POINT('Ctrl Pts',(-1.30215783236363,-24.5986826684027,
12.));
#193155=CARTESIAN_POINT('Ctrl Pts',(-1.31065299222023,-24.5761023320183,
0.));
#193156=CARTESIAN_POINT('Ctrl Pts',(-1.31065299222023,-24.5761023320183,
12.));
#193157=CARTESIAN_POINT('Ctrl Pts',(-1.31906276763669,-24.5535820868674,
0.));
#193158=CARTESIAN_POINT('Ctrl Pts',(-1.31906276763669,-24.5535820868674,
12.));
#193159=CARTESIAN_POINT('Ctrl Pts',(-1.32738724435327,-24.5311225731435,
0.));
#193160=CARTESIAN_POINT('Ctrl Pts',(-1.32738724435327,-24.5311225731435,
12.));
#193161=CARTESIAN_POINT('Ctrl Pts',(-1.33562651019687,-24.5087244363856,
0.));
#193162=CARTESIAN_POINT('Ctrl Pts',(-1.33562651019687,-24.5087244363856,
12.));
#193163=CARTESIAN_POINT('Ctrl Pts',(-1.34378065512339,-24.4863883275134,
0.));
#193164=CARTESIAN_POINT('Ctrl Pts',(-1.34378065512339,-24.4863883275134,
12.));
#193165=CARTESIAN_POINT('Ctrl Pts',(-1.35184977125649,-24.4641149028892,
0.));
#193166=CARTESIAN_POINT('Ctrl Pts',(-1.35184977125649,-24.4641149028892,
12.));
#193167=CARTESIAN_POINT('Ctrl Pts',(-1.35983395290628,-24.4419048244523,
0.));
#193168=CARTESIAN_POINT('Ctrl Pts',(-1.35983395290628,-24.4419048244523,
12.));
#193169=CARTESIAN_POINT('Ctrl Pts',(-1.36773329659957,-24.4197587598337,
0.));
#193170=CARTESIAN_POINT('Ctrl Pts',(-1.36773329659957,-24.4197587598337,
12.));
#193171=CARTESIAN_POINT('Ctrl Pts',(-1.3755479011161,-24.3976773824732,
0.));
#193172=CARTESIAN_POINT('Ctrl Pts',(-1.3755479011161,-24.3976773824732,
12.));
#193173=CARTESIAN_POINT('Ctrl Pts',(-1.38327786753,-24.3756613717299,0.));
#193174=CARTESIAN_POINT('Ctrl Pts',(-1.38327786753,-24.3756613717299,12.));
#193175=CARTESIAN_POINT('Ctrl Pts',(-1.39092329926389,-24.3537114129875,
0.));
#193176=CARTESIAN_POINT('Ctrl Pts',(-1.39092329926389,-24.3537114129875,
12.));
#193177=CARTESIAN_POINT('Ctrl Pts',(-1.39848430212808,-24.3318281977643,
0.));
#193178=CARTESIAN_POINT('Ctrl Pts',(-1.39848430212808,-24.3318281977643,
12.));
#193179=CARTESIAN_POINT('Ctrl Pts',(-1.40596098434338,-24.3100124238311,
0.));
#193180=CARTESIAN_POINT('Ctrl Pts',(-1.40596098434338,-24.3100124238311,
12.));
#193181=CARTESIAN_POINT('Ctrl Pts',(-1.41335345657684,-24.288264795321,
0.));
#193182=CARTESIAN_POINT('Ctrl Pts',(-1.41335345657684,-24.288264795321,
12.));
#193183=CARTESIAN_POINT('Ctrl Pts',(-1.42066183198254,-24.2665860228356,
0.));
#193184=CARTESIAN_POINT('Ctrl Pts',(-1.42066183198254,-24.2665860228356,
12.));
#193185=CARTESIAN_POINT('Ctrl Pts',(-1.42788622624855,-24.2449768235488,
0.));
#193186=CARTESIAN_POINT('Ctrl Pts',(-1.42788622624855,-24.2449768235488,
12.));
#193187=CARTESIAN_POINT('Ctrl Pts',(-1.43502675765509,-24.2234379212984,
0.));
#193188=CARTESIAN_POINT('Ctrl Pts',(-1.43502675765509,-24.2234379212984,
12.));
#193189=CARTESIAN_POINT('Ctrl Pts',(-1.44208354711083,-24.201970046722,
0.));
#193190=CARTESIAN_POINT('Ctrl Pts',(-1.44208354711083,-24.201970046722,
12.));
#193191=CARTESIAN_POINT('Ctrl Pts',(-1.44905671818729,-24.1805739374038,
0.));
#193192=CARTESIAN_POINT('Ctrl Pts',(-1.44905671818729,-24.1805739374038,
12.));
#193193=CARTESIAN_POINT('Ctrl Pts',(-1.45594639716319,-24.1592503380107,
0.));
#193194=CARTESIAN_POINT('Ctrl Pts',(-1.45594639716319,-24.1592503380107,
12.));
#193195=CARTESIAN_POINT('Ctrl Pts',(-1.46275271307399,-24.1380000004272,
0.));
#193196=CARTESIAN_POINT('Ctrl Pts',(-1.46275271307399,-24.1380000004272,
12.));
#193197=CARTESIAN_POINT('Ctrl Pts',(-1.46947579776992,-24.1168236838824,
0.));
#193198=CARTESIAN_POINT('Ctrl Pts',(-1.46947579776992,-24.1168236838824,
12.));
#193199=CARTESIAN_POINT('Ctrl Pts',(-1.47611578597743,-24.0957221550778,
0.));
#193200=CARTESIAN_POINT('Ctrl Pts',(-1.47611578597743,-24.0957221550778,
12.));
#193201=CARTESIAN_POINT('Ctrl Pts',(-1.48267281533684,-24.0746961883528,
0.));
#193202=CARTESIAN_POINT('Ctrl Pts',(-1.48267281533684,-24.0746961883528,
12.));
#193203=CARTESIAN_POINT('Ctrl Pts',(-1.48914702644888,-24.0537465658429,
0.));
#193204=CARTESIAN_POINT('Ctrl Pts',(-1.48914702644888,-24.0537465658429,
12.));
#193205=CARTESIAN_POINT('Ctrl Pts',(-1.49553856292802,-24.0328740776331,
0.));
#193206=CARTESIAN_POINT('Ctrl Pts',(-1.49553856292802,-24.0328740776331,
12.));
#193207=CARTESIAN_POINT('Ctrl Pts',(-1.501847571461,-24.0120795219086,0.));
#193208=CARTESIAN_POINT('Ctrl Pts',(-1.501847571461,-24.0120795219086,12.));
#193209=CARTESIAN_POINT('Ctrl Pts',(-1.50807420187695,-23.9913637050927,
0.));
#193210=CARTESIAN_POINT('Ctrl Pts',(-1.50807420187695,-23.9913637050927,
12.));
#193211=CARTESIAN_POINT('Ctrl Pts',(-1.51421860720615,-23.970727442014,
0.));
#193212=CARTESIAN_POINT('Ctrl Pts',(-1.51421860720615,-23.970727442014,
12.));
#193213=CARTESIAN_POINT('Ctrl Pts',(-1.52028094372793,-23.9501715561033,
0.));
#193214=CARTESIAN_POINT('Ctrl Pts',(-1.52028094372793,-23.9501715561033,
12.));
#193215=CARTESIAN_POINT('Ctrl Pts',(-1.52626137103033,-23.9296968795757,
0.));
#193216=CARTESIAN_POINT('Ctrl Pts',(-1.52626137103033,-23.9296968795757,
12.));
#193217=CARTESIAN_POINT('Ctrl Pts',(-1.53216005207464,-23.9093042536119,
0.));
#193218=CARTESIAN_POINT('Ctrl Pts',(-1.53216005207464,-23.9093042536119,
12.));
#193219=CARTESIAN_POINT('Ctrl Pts',(-1.53797715326759,-23.8889945285318,
0.));
#193220=CARTESIAN_POINT('Ctrl Pts',(-1.53797715326759,-23.8889945285318,
12.));
#193221=CARTESIAN_POINT('Ctrl Pts',(-1.54371284453991,-23.8687685639642,
0.));
#193222=CARTESIAN_POINT('Ctrl Pts',(-1.54371284453991,-23.8687685639642,
12.));
#193223=CARTESIAN_POINT('Ctrl Pts',(-1.54936729940542,-23.8486272290705,
0.));
#193224=CARTESIAN_POINT('Ctrl Pts',(-1.54936729940542,-23.8486272290705,
12.));
#193225=CARTESIAN_POINT('Ctrl Pts',(-1.55494069502636,-23.8285714027636,
0.));
#193226=CARTESIAN_POINT('Ctrl Pts',(-1.55494069502636,-23.8285714027636,
12.));
#193227=CARTESIAN_POINT('Ctrl Pts',(-1.56043321228635,-23.8086019739194,
0.));
#193228=CARTESIAN_POINT('Ctrl Pts',(-1.56043321228635,-23.8086019739194,
12.));
#193229=CARTESIAN_POINT('Ctrl Pts',(-1.56584503586844,-23.7887198415878,
0.));
#193230=CARTESIAN_POINT('Ctrl Pts',(-1.56584503586844,-23.7887198415878,
12.));
#193231=CARTESIAN_POINT('Ctrl Pts',(-1.57117635434409,-23.7689259151862,
0.));
#193232=CARTESIAN_POINT('Ctrl Pts',(-1.57117635434409,-23.7689259151862,
12.));
#193233=CARTESIAN_POINT('Ctrl Pts',(-1.57642736025247,-23.749221114736,
0.));
#193234=CARTESIAN_POINT('Ctrl Pts',(-1.57642736025247,-23.749221114736,
12.));
#193235=CARTESIAN_POINT('Ctrl Pts',(-1.58159825017359,-23.72960637113,0.));
#193236=CARTESIAN_POINT('Ctrl Pts',(-1.58159825017359,-23.72960637113,12.));
#193237=CARTESIAN_POINT('Ctrl Pts',(-1.58668922481222,-23.710082626383,
0.));
#193238=CARTESIAN_POINT('Ctrl Pts',(-1.58668922481222,-23.710082626383,
12.));
#193239=CARTESIAN_POINT('Ctrl Pts',(-1.59170048908634,-23.6906508338833,
0.));
#193240=CARTESIAN_POINT('Ctrl Pts',(-1.59170048908634,-23.6906508338833,
12.));
#193241=CARTESIAN_POINT('Ctrl Pts',(-1.59663225222464,-23.671311958631,
0.));
#193242=CARTESIAN_POINT('Ctrl Pts',(-1.59663225222464,-23.671311958631,
12.));
#193243=CARTESIAN_POINT('Ctrl Pts',(-1.60148472786596,-23.6520669774876,
0.));
#193244=CARTESIAN_POINT('Ctrl Pts',(-1.60148472786596,-23.6520669774876,
12.));
#193245=CARTESIAN_POINT('Ctrl Pts',(-1.60625813414674,-23.6329168794929,
0.));
#193246=CARTESIAN_POINT('Ctrl Pts',(-1.60625813414674,-23.6329168794929,
12.));
#193247=CARTESIAN_POINT('Ctrl Pts',(-1.61095269379779,-23.6138626661653,
0.));
#193248=CARTESIAN_POINT('Ctrl Pts',(-1.61095269379779,-23.6138626661653,
12.));
#193249=CARTESIAN_POINT('Ctrl Pts',(-1.61556863424699,-23.5949053517997,
0.));
#193250=CARTESIAN_POINT('Ctrl Pts',(-1.61556863424699,-23.5949053517997,
12.));
#193251=CARTESIAN_POINT('Ctrl Pts',(-1.62010618772867,-23.57604596376,0.));
#193252=CARTESIAN_POINT('Ctrl Pts',(-1.62010618772867,-23.57604596376,12.));
#193253=CARTESIAN_POINT('Ctrl Pts',(-1.62456559140065,-23.5572855427601,
0.));
#193254=CARTESIAN_POINT('Ctrl Pts',(-1.62456559140065,-23.5572855427601,
12.));
#193255=CARTESIAN_POINT('Ctrl Pts',(-1.62894708745224,-23.538625143226,
0.));
#193256=CARTESIAN_POINT('Ctrl Pts',(-1.62894708745224,-23.538625143226,
12.));
#193257=CARTESIAN_POINT('Ctrl Pts',(-1.63325092321727,-23.5200658336612,
0.));
#193258=CARTESIAN_POINT('Ctrl Pts',(-1.63325092321727,-23.5200658336612,
12.));
#193259=CARTESIAN_POINT('Ctrl Pts',(-1.63747735129475,-23.5016086970003,
0.));
#193260=CARTESIAN_POINT('Ctrl Pts',(-1.63747735129475,-23.5016086970003,
12.));
#193261=CARTESIAN_POINT('Ctrl Pts',(-1.64162662967529,-23.4832548309645,
0.));
#193262=CARTESIAN_POINT('Ctrl Pts',(-1.64162662967529,-23.4832548309645,
12.));
#193263=CARTESIAN_POINT('Ctrl Pts',(-1.64569902187612,-23.4650053483932,
0.));
#193264=CARTESIAN_POINT('Ctrl Pts',(-1.64569902187612,-23.4650053483932,
12.));
#193265=CARTESIAN_POINT('Ctrl Pts',(-1.64969479707341,-23.4468613776574,
0.));
#193266=CARTESIAN_POINT('Ctrl Pts',(-1.64969479707341,-23.4468613776574,
12.));
#193267=CARTESIAN_POINT('Ctrl Pts',(-1.65361423023729,-23.4288240631043,
0.));
#193268=CARTESIAN_POINT('Ctrl Pts',(-1.65361423023729,-23.4288240631043,
12.));
#193269=CARTESIAN_POINT('Ctrl Pts',(-1.65745760227506,-23.4108945654805,
0.));
#193270=CARTESIAN_POINT('Ctrl Pts',(-1.65745760227506,-23.4108945654805,
12.));
#193271=CARTESIAN_POINT('Ctrl Pts',(-1.66122520018012,-23.3930740623619,
0.));
#193272=CARTESIAN_POINT('Ctrl Pts',(-1.66122520018012,-23.3930740623619,
12.));
#193273=CARTESIAN_POINT('Ctrl Pts',(-1.66491731718878,-23.3753637485545,
0.));
#193274=CARTESIAN_POINT('Ctrl Pts',(-1.66491731718878,-23.3753637485545,
12.));
#193275=CARTESIAN_POINT('Ctrl Pts',(-1.66853425293997,-23.3577648365744,
0.));
#193276=CARTESIAN_POINT('Ctrl Pts',(-1.66853425293997,-23.3577648365744,
12.));
#193277=CARTESIAN_POINT('Ctrl Pts',(-1.67207631363923,-23.3402785571865,
0.));
#193278=CARTESIAN_POINT('Ctrl Pts',(-1.67207631363923,-23.3402785571865,
12.));
#193279=CARTESIAN_POINT('Ctrl Pts',(-1.67554381222995,-23.3229061599145,
0.));
#193280=CARTESIAN_POINT('Ctrl Pts',(-1.67554381222995,-23.3229061599145,
12.));
#193281=CARTESIAN_POINT('Ctrl Pts',(-1.67893706857118,-23.3056489135611,
0.));
#193282=CARTESIAN_POINT('Ctrl Pts',(-1.67893706857118,-23.3056489135611,
12.));
#193283=CARTESIAN_POINT('Ctrl Pts',(-1.68225640962169,-23.2885081066951,
0.));
#193284=CARTESIAN_POINT('Ctrl Pts',(-1.68225640962169,-23.2885081066951,
12.));
#193285=CARTESIAN_POINT('Ctrl Pts',(-1.68550216963259,-23.2714850482246,
0.));
#193286=CARTESIAN_POINT('Ctrl Pts',(-1.68550216963259,-23.2714850482246,
12.));
#193287=CARTESIAN_POINT('Ctrl Pts',(-1.68867469034897,-23.2545810680537,
0.));
#193288=CARTESIAN_POINT('Ctrl Pts',(-1.68867469034897,-23.2545810680537,
12.));
#193289=CARTESIAN_POINT('Ctrl Pts',(-1.69177432121712,-23.2377975177013,
0.));
#193290=CARTESIAN_POINT('Ctrl Pts',(-1.69177432121712,-23.2377975177013,
12.));
#193291=CARTESIAN_POINT('Ctrl Pts',(-1.69480141959954,-23.2211357709374,
0.));
#193292=CARTESIAN_POINT('Ctrl Pts',(-1.69480141959954,-23.2211357709374,
12.));
#193293=CARTESIAN_POINT('Ctrl Pts',(-1.69775635099444,-23.2045972243767,
0.));
#193294=CARTESIAN_POINT('Ctrl Pts',(-1.69775635099444,-23.2045972243767,
12.));
#193295=CARTESIAN_POINT('Ctrl Pts',(-1.70063948927011,-23.1881832981851,
0.));
#193296=CARTESIAN_POINT('Ctrl Pts',(-1.70063948927011,-23.1881832981851,
12.));
#193297=CARTESIAN_POINT('Ctrl Pts',(-1.70345121691277,-23.1718954368751,
0.));
#193298=CARTESIAN_POINT('Ctrl Pts',(-1.70345121691277,-23.1718954368751,
12.));
#193299=CARTESIAN_POINT('Ctrl Pts',(-1.70619192527853,-23.1557351100614,
0.));
#193300=CARTESIAN_POINT('Ctrl Pts',(-1.70619192527853,-23.1557351100614,
12.));
#193301=CARTESIAN_POINT('Ctrl Pts',(-1.70886201485453,-23.1397038132356,
0.));
#193302=CARTESIAN_POINT('Ctrl Pts',(-1.70886201485453,-23.1397038132356,
12.));
#193303=CARTESIAN_POINT('Ctrl Pts',(-1.71146189552175,-23.1238030684925,
0.));
#193304=CARTESIAN_POINT('Ctrl Pts',(-1.71146189552175,-23.1238030684925,
12.));
#193305=CARTESIAN_POINT('Ctrl Pts',(-1.71399198684705,-23.1080344254286,
0.));
#193306=CARTESIAN_POINT('Ctrl Pts',(-1.71399198684705,-23.1080344254286,
12.));
#193307=CARTESIAN_POINT('Ctrl Pts',(-1.71645271839298,-23.0923994621213,
0.));
#193308=CARTESIAN_POINT('Ctrl Pts',(-1.71645271839298,-23.0923994621213,
12.));
#193309=CARTESIAN_POINT('Ctrl Pts',(-1.71884453003028,-23.0768997860709,
0.));
#193310=CARTESIAN_POINT('Ctrl Pts',(-1.71884453003028,-23.0768997860709,
12.));
#193311=CARTESIAN_POINT('Ctrl Pts',(-1.72116787225993,-23.0615370351562,
0.));
#193312=CARTESIAN_POINT('Ctrl Pts',(-1.72116787225993,-23.0615370351562,
12.));
#193313=CARTESIAN_POINT('Ctrl Pts',(-1.72342320653748,-23.0463128785531,
0.));
#193314=CARTESIAN_POINT('Ctrl Pts',(-1.72342320653748,-23.0463128785531,
12.));
#193315=CARTESIAN_POINT('Ctrl Pts',(-1.72561100564047,-23.0312290178883,
0.));
#193316=CARTESIAN_POINT('Ctrl Pts',(-1.72561100564047,-23.0312290178883,
12.));
#193317=CARTESIAN_POINT('Ctrl Pts',(-1.7277317540471,-23.0162871884168,
0.));
#193318=CARTESIAN_POINT('Ctrl Pts',(-1.7277317540471,-23.0162871884168,
12.));
#193319=CARTESIAN_POINT('Ctrl Pts',(-1.72978594832137,-23.001489160189,
0.));
#193320=CARTESIAN_POINT('Ctrl Pts',(-1.72978594832137,-23.001489160189,
12.));
#193321=CARTESIAN_POINT('Ctrl Pts',(-1.73177409750192,-22.9868367391978,
0.));
#193322=CARTESIAN_POINT('Ctrl Pts',(-1.73177409750192,-22.9868367391978,
12.));
#193323=CARTESIAN_POINT('Ctrl Pts',(-1.73369672350816,-22.9723317685688,
0.));
#193324=CARTESIAN_POINT('Ctrl Pts',(-1.73369672350816,-22.9723317685688,
12.));
#193325=CARTESIAN_POINT('Ctrl Pts',(-1.7355543616277,-22.9579761301063,
0.));
#193326=CARTESIAN_POINT('Ctrl Pts',(-1.7355543616277,-22.9579761301063,
12.));
#193327=CARTESIAN_POINT('Ctrl Pts',(-1.7373475610004,-22.9437717457826,
0.));
#193328=CARTESIAN_POINT('Ctrl Pts',(-1.7373475610004,-22.9437717457826,
12.));
#193329=CARTESIAN_POINT('Ctrl Pts',(-1.73907688511667,-22.9297205792586,
0.));
#193330=CARTESIAN_POINT('Ctrl Pts',(-1.73907688511667,-22.9297205792586,
12.));
#193331=CARTESIAN_POINT('Ctrl Pts',(-1.74074291231059,-22.9158246373363,
0.));
#193332=CARTESIAN_POINT('Ctrl Pts',(-1.74074291231059,-22.9158246373363,
12.));
#193333=CARTESIAN_POINT('Ctrl Pts',(-1.74234623630081,-22.9020859716141,
0.));
#193334=CARTESIAN_POINT('Ctrl Pts',(-1.74234623630081,-22.9020859716141,
12.));
#193335=CARTESIAN_POINT('Ctrl Pts',(-1.74388746677703,-22.888506680335,
0.));
#193336=CARTESIAN_POINT('Ctrl Pts',(-1.74388746677703,-22.888506680335,
12.));
#193337=CARTESIAN_POINT('Ctrl Pts',(-1.74536722998202,-22.8750889101696,
0.));
#193338=CARTESIAN_POINT('Ctrl Pts',(-1.74536722998202,-22.8750889101696,
12.));
#193339=CARTESIAN_POINT('Ctrl Pts',(-1.74678616930666,-22.8618348580235,
0.));
#193340=CARTESIAN_POINT('Ctrl Pts',(-1.74678616930666,-22.8618348580235,
12.));
#193341=CARTESIAN_POINT('Ctrl Pts',(-1.74814494588494,-22.8487467728076,
0.));
#193342=CARTESIAN_POINT('Ctrl Pts',(-1.74814494588494,-22.8487467728076,
12.));
#193343=CARTESIAN_POINT('Ctrl Pts',(-1.74944423940117,-22.8358269579853,
0.));
#193344=CARTESIAN_POINT('Ctrl Pts',(-1.74944423940117,-22.8358269579853,
12.));
#193345=CARTESIAN_POINT('Ctrl Pts',(-1.75068474890884,-22.8230777741284,
0.));
#193346=CARTESIAN_POINT('Ctrl Pts',(-1.75068474890884,-22.8230777741284,
12.));
#193347=CARTESIAN_POINT('Ctrl Pts',(-1.75186719365593,-22.8105016414713,
0.));
#193348=CARTESIAN_POINT('Ctrl Pts',(-1.75186719365593,-22.8105016414713,
12.));
#193349=CARTESIAN_POINT('Ctrl Pts',(-1.75299231391467,-22.7981010424314,
0.));
#193350=CARTESIAN_POINT('Ctrl Pts',(-1.75299231391467,-22.7981010424314,
12.));
#193351=CARTESIAN_POINT('Ctrl Pts',(-1.75406087182937,-22.7858785242361,
0.));
#193352=CARTESIAN_POINT('Ctrl Pts',(-1.75406087182937,-22.7858785242361,
12.));
#193353=CARTESIAN_POINT('Ctrl Pts',(-1.75507365227133,-22.7738367016118,
0.));
#193354=CARTESIAN_POINT('Ctrl Pts',(-1.75507365227133,-22.7738367016118,
12.));
#193355=CARTESIAN_POINT('Ctrl Pts',(-1.75603146371642,-22.7619782595013,
0.));
#193356=CARTESIAN_POINT('Ctrl Pts',(-1.75603146371642,-22.7619782595013,
12.));
#193357=CARTESIAN_POINT('Ctrl Pts',(-1.75693513908908,-22.750305955645,
0.));
#193358=CARTESIAN_POINT('Ctrl Pts',(-1.75693513908908,-22.750305955645,
12.));
#193359=CARTESIAN_POINT('Ctrl Pts',(-1.75778553673245,-22.7388226235559,
0.));
#193360=CARTESIAN_POINT('Ctrl Pts',(-1.75778553673245,-22.7388226235559,
12.));
#193361=CARTESIAN_POINT('Ctrl Pts',(-1.75858354204634,-22.72753117773,0.));
#193362=CARTESIAN_POINT('Ctrl Pts',(-1.75858354204634,-22.72753117773,12.));
#193363=CARTESIAN_POINT('Ctrl Pts',(-1.75933006905926,-22.7164346186006,
0.));
#193364=CARTESIAN_POINT('Ctrl Pts',(-1.75933006905926,-22.7164346186006,
12.));
#193365=CARTESIAN_POINT('Ctrl Pts',(-1.76002606202402,-22.7055360375485,
0.));
#193366=CARTESIAN_POINT('Ctrl Pts',(-1.76002606202402,-22.7055360375485,
12.));
#193367=CARTESIAN_POINT('Ctrl Pts',(-1.76067249704888,-22.6948386219851,
0.));
#193368=CARTESIAN_POINT('Ctrl Pts',(-1.76067249704888,-22.6948386219851,
12.));
#193369=CARTESIAN_POINT('Ctrl Pts',(-1.76127038310615,-22.684345658525,
0.));
#193370=CARTESIAN_POINT('Ctrl Pts',(-1.76127038310615,-22.684345658525,
12.));
#193371=CARTESIAN_POINT('Ctrl Pts',(-1.76182076289527,-22.67406053567,0.));
#193372=CARTESIAN_POINT('Ctrl Pts',(-1.76182076289527,-22.67406053567,12.));
#193373=CARTESIAN_POINT('Ctrl Pts',(-1.7623247139257,-22.6639867471753,
0.));
#193374=CARTESIAN_POINT('Ctrl Pts',(-1.7623247139257,-22.6639867471753,
12.));
#193375=CARTESIAN_POINT('Ctrl Pts',(-1.76278334912562,-22.654127893841,
0.));
#193376=CARTESIAN_POINT('Ctrl Pts',(-1.76278334912562,-22.654127893841,
12.));
#193377=CARTESIAN_POINT('Ctrl Pts',(-1.76319782013917,-22.6444876940423,
0.));
#193378=CARTESIAN_POINT('Ctrl Pts',(-1.76319782013917,-22.6444876940423,
12.));
#193379=CARTESIAN_POINT('Ctrl Pts',(-1.76356932176274,-22.6350699979359,
0.));
#193380=CARTESIAN_POINT('Ctrl Pts',(-1.76356932176274,-22.6350699979359,
12.));
#193381=CARTESIAN_POINT('Ctrl Pts',(-1.76389909571404,-22.6258787994848,
0.));
#193382=CARTESIAN_POINT('Ctrl Pts',(-1.76389909571404,-22.6258787994848,
12.));
#193383=CARTESIAN_POINT('Ctrl Pts',(-1.7641884354374,-22.6169182517694,
0.));
#193384=CARTESIAN_POINT('Ctrl Pts',(-1.7641884354374,-22.6169182517694,
12.));
#193385=CARTESIAN_POINT('Ctrl Pts',(-1.76443868648017,-22.6081926681343,
0.));
#193386=CARTESIAN_POINT('Ctrl Pts',(-1.76443868648017,-22.6081926681343,
12.));
#193387=CARTESIAN_POINT('Ctrl Pts',(-1.76465124413558,-22.5997065145638,
0.));
#193388=CARTESIAN_POINT('Ctrl Pts',(-1.76465124413558,-22.5997065145638,
12.));
#193389=CARTESIAN_POINT('Ctrl Pts',(-1.76482755288412,-22.5914644078106,
0.));
#193390=CARTESIAN_POINT('Ctrl Pts',(-1.76482755288412,-22.5914644078106,
12.));
#193391=CARTESIAN_POINT('Ctrl Pts',(-1.76496910283089,-22.5834711038022,
0.));
#193392=CARTESIAN_POINT('Ctrl Pts',(-1.76496910283089,-22.5834711038022,
12.));
#193393=CARTESIAN_POINT('Ctrl Pts',(-1.76507744026747,-22.5757315316353,
0.));
#193394=CARTESIAN_POINT('Ctrl Pts',(-1.76507744026747,-22.5757315316353,
12.));
#193395=CARTESIAN_POINT('Ctrl Pts',(-1.76515418518832,-22.5682508499874,
0.));
#193396=CARTESIAN_POINT('Ctrl Pts',(-1.76515418518832,-22.5682508499874,
12.));
#193397=CARTESIAN_POINT('Ctrl Pts',(-1.76520104500451,-22.5610344912501,
0.));
#193398=CARTESIAN_POINT('Ctrl Pts',(-1.76520104500451,-22.5610344912501,
12.));
#193399=CARTESIAN_POINT('Ctrl Pts',(-1.76521983384063,-22.5540882235837,
0.));
#193400=CARTESIAN_POINT('Ctrl Pts',(-1.76521983384063,-22.5540882235837,
12.));
#193401=CARTESIAN_POINT('Ctrl Pts',(-1.76521245524048,-22.5474180954006,
0.));
#193402=CARTESIAN_POINT('Ctrl Pts',(-1.76521245524048,-22.5474180954006,
12.));
#193403=CARTESIAN_POINT('Ctrl Pts',(-1.76518087841494,-22.5410303590892,
0.));
#193404=CARTESIAN_POINT('Ctrl Pts',(-1.76518087841494,-22.5410303590892,
12.));
#193405=CARTESIAN_POINT('Ctrl Pts',(-1.76512711563255,-22.5349313983571,
0.));
#193406=CARTESIAN_POINT('Ctrl Pts',(-1.76512711563255,-22.5349313983571,
12.));
#193407=CARTESIAN_POINT('Ctrl Pts',(-1.7650532026276,-22.529127665298,0.));
#193408=CARTESIAN_POINT('Ctrl Pts',(-1.7650532026276,-22.529127665298,12.));
#193409=CARTESIAN_POINT('Ctrl Pts',(-1.76496128643376,-22.5236259635515,
0.));
#193410=CARTESIAN_POINT('Ctrl Pts',(-1.76496128643376,-22.5236259635515,
12.));
#193411=CARTESIAN_POINT('Ctrl Pts',(-1.76485369319896,-22.5184336670207,
0.));
#193412=CARTESIAN_POINT('Ctrl Pts',(-1.76485369319896,-22.5184336670207,
12.));
#193413=CARTESIAN_POINT('Ctrl Pts',(-1.7647330328115,-22.5135590569554,
0.));
#193414=CARTESIAN_POINT('Ctrl Pts',(-1.7647330328115,-22.5135590569554,
12.));
#193415=CARTESIAN_POINT('Ctrl Pts',(-1.76460218257314,-22.5090112700212,
0.));
#193416=CARTESIAN_POINT('Ctrl Pts',(-1.76460218257314,-22.5090112700212,
12.));
#193417=CARTESIAN_POINT('Ctrl Pts',(-1.76446408210366,-22.5047996391978,
0.));
#193418=CARTESIAN_POINT('Ctrl Pts',(-1.76446408210366,-22.5047996391978,
12.));
#193419=CARTESIAN_POINT('Ctrl Pts',(-1.76432160068739,-22.5009332677316,
0.));
#193420=CARTESIAN_POINT('Ctrl Pts',(-1.76432160068739,-22.5009332677316,
12.));
#193421=CARTESIAN_POINT('Ctrl Pts',(-1.76417731243484,-22.4974203063191,
0.));
#193422=CARTESIAN_POINT('Ctrl Pts',(-1.76417731243484,-22.4974203063191,
12.));
#193423=CARTESIAN_POINT('Ctrl Pts',(-1.76403393880317,-22.4942693792449,
0.));
#193424=CARTESIAN_POINT('Ctrl Pts',(-1.76403393880317,-22.4942693792449,
12.));
#193425=CARTESIAN_POINT('Ctrl Pts',(-1.76389475965715,-22.4914909094908,
0.));
#193426=CARTESIAN_POINT('Ctrl Pts',(-1.76389475965715,-22.4914909094908,
12.));
#193427=CARTESIAN_POINT('Ctrl Pts',(-1.76376424879469,-22.4890991659479,
0.));
#193428=CARTESIAN_POINT('Ctrl Pts',(-1.76376424879469,-22.4890991659479,
12.));
#193429=CARTESIAN_POINT('Ctrl Pts',(-1.76364784232926,-22.4871115206572,
0.));
#193430=CARTESIAN_POINT('Ctrl Pts',(-1.76364784232926,-22.4871115206572,
12.));
#193431=CARTESIAN_POINT('Ctrl Pts',(-1.7635507604555,-22.4855446605991,
0.));
#193432=CARTESIAN_POINT('Ctrl Pts',(-1.7635507604555,-22.4855446605991,
12.));
#193433=CARTESIAN_POINT('Ctrl Pts',(-1.76347698284863,-22.4844112933125,
0.));
#193434=CARTESIAN_POINT('Ctrl Pts',(-1.76347698284863,-22.4844112933125,
12.));
#193435=CARTESIAN_POINT('Ctrl Pts',(-1.7634381343466,-22.4838562517064,
0.));
#193436=CARTESIAN_POINT('Ctrl Pts',(-1.7634381343466,-22.4838562517064,
12.));
#193437=CARTESIAN_POINT('Ctrl Pts',(-1.76342064263638,-22.4836387052228,
0.));
#193438=CARTESIAN_POINT('Ctrl Pts',(-1.76342064263638,-22.4836387052228,
12.));
#193439=CARTESIAN_POINT('Ctrl Pts',(-1.76341415538792,-22.4835819929788,
0.));
#193440=CARTESIAN_POINT('Ctrl Pts',(-1.76341415538792,-22.4835819929788,
12.));
#193441=CARTESIAN_POINT('Ctrl Pts',(-1.76341220531181,-22.4835757167854,
0.));
#193442=CARTESIAN_POINT('Ctrl Pts',(-1.76341220531181,-22.4835757167854,
12.));
#193443=CARTESIAN_POINT('',(-0.661312440730913,-25.991588367311,0.));
#193444=CARTESIAN_POINT('Ctrl Pts',(-0.661312440730913,-25.991588367311,
0.));
#193445=CARTESIAN_POINT('Ctrl Pts',(-0.664028313187638,-25.9865613464773,
0.));
#193446=CARTESIAN_POINT('Ctrl Pts',(-0.669451306780837,-25.9765104298071,
0.));
#193447=CARTESIAN_POINT('Ctrl Pts',(-0.677559543209739,-25.9614434297919,
0.));
#193448=CARTESIAN_POINT('Ctrl Pts',(-0.688318015057743,-25.9413728471909,
0.));
#193449=CARTESIAN_POINT('Ctrl Pts',(-0.701678575228768,-25.9163158909426,
0.));
#193450=CARTESIAN_POINT('Ctrl Pts',(-0.714951588527651,-25.891290261497,
0.));
#193451=CARTESIAN_POINT('Ctrl Pts',(-0.728137036482348,-25.8662960624185,
0.));
#193452=CARTESIAN_POINT('Ctrl Pts',(-0.741234902663818,-25.8413334619055,
0.));
#193453=CARTESIAN_POINT('Ctrl Pts',(-0.754245175609535,-25.8164027059984,
0.));
#193454=CARTESIAN_POINT('Ctrl Pts',(-0.76716785265118,-25.7915041383376,
0.));
#193455=CARTESIAN_POINT('Ctrl Pts',(-0.780002940291976,-25.7666381946955,
0.));
#193456=CARTESIAN_POINT('Ctrl Pts',(-0.792750451616139,-25.7418053757746,
0.));
#193457=CARTESIAN_POINT('Ctrl Pts',(-0.805410404554365,-25.7170062262525,
0.));
#193458=CARTESIAN_POINT('Ctrl Pts',(-0.817982819787476,-25.6922413110194,
0.));
#193459=CARTESIAN_POINT('Ctrl Pts',(-0.830467718864218,-25.6675111931952,
0.));
#193460=CARTESIAN_POINT('Ctrl Pts',(-0.842865122120771,-25.6428164100055,
0.));
#193461=CARTESIAN_POINT('Ctrl Pts',(-0.85517504703656,-25.6181574536049,
0.));
#193462=CARTESIAN_POINT('Ctrl Pts',(-0.867397509338443,-25.5935347843585,
0.));
#193463=CARTESIAN_POINT('Ctrl Pts',(-0.879532523834307,-25.5689488408156,
0.));
#193464=CARTESIAN_POINT('Ctrl Pts',(-0.891580105349052,-25.5444000508211,
0.));
#193465=CARTESIAN_POINT('Ctrl Pts',(-0.903540269651119,-25.5198888424194,
0.));
#193466=CARTESIAN_POINT('Ctrl Pts',(-0.915413034335626,-25.4954156541795,
0.));
#193467=CARTESIAN_POINT('Ctrl Pts',(-0.927198419886107,-25.4709809475009,
0.));
#193468=CARTESIAN_POINT('Ctrl Pts',(-0.938896449496205,-25.4465852044849,
0.));
#193469=CARTESIAN_POINT('Ctrl Pts',(-0.950507148597481,-25.4222289223167,
0.));
#193470=CARTESIAN_POINT('Ctrl Pts',(-0.962030544503155,-25.3979126089163,
0.));
#193471=CARTESIAN_POINT('Ctrl Pts',(-0.973466666000176,-25.3736367778845,
0.));
#193472=CARTESIAN_POINT('Ctrl Pts',(-0.984815543003984,-25.3494019441441,
0.));
#193473=CARTESIAN_POINT('Ctrl Pts',(-0.996077206120636,-25.3252086182968,
0.));
#193474=CARTESIAN_POINT('Ctrl Pts',(-1.00725168656897,-25.3010573055548,
0.));
#193475=CARTESIAN_POINT('Ctrl Pts',(-1.01833901642238,-25.276948508726,
0.));
#193476=CARTESIAN_POINT('Ctrl Pts',(-1.02933922876807,-25.2528827300422,
0.));
#193477=CARTESIAN_POINT('Ctrl Pts',(-1.04025235791508,-25.2288604735086,
0.));
#193478=CARTESIAN_POINT('Ctrl Pts',(-1.05107843957933,-25.2048822469028,
0.));
#193479=CARTESIAN_POINT('Ctrl Pts',(-1.06181751111769,-25.1809485642192,
0.));
#193480=CARTESIAN_POINT('Ctrl Pts',(-1.07246961165477,-25.157059946931,
0.));
#193481=CARTESIAN_POINT('Ctrl Pts',(-1.08303478197189,-25.1332169227413,
0.));
#193482=CARTESIAN_POINT('Ctrl Pts',(-1.09351306445309,-25.1094200248446,
0.));
#193483=CARTESIAN_POINT('Ctrl Pts',(-1.10390450301746,-25.0856697909679,
0.));
#193484=CARTESIAN_POINT('Ctrl Pts',(-1.1142091430689,-25.0619667625336,
0.));
#193485=CARTESIAN_POINT('Ctrl Pts',(-1.12442703144453,-25.0383114836899,
0.));
#193486=CARTESIAN_POINT('Ctrl Pts',(-1.13455821638531,-25.0147045006196,
0.));
#193487=CARTESIAN_POINT('Ctrl Pts',(-1.14460274758202,-24.9911463621433,
0.));
#193488=CARTESIAN_POINT('Ctrl Pts',(-1.1545606762189,-24.9676376201502,
0.));
#193489=CARTESIAN_POINT('Ctrl Pts',(-1.16443205502851,-24.9441788300932,
0.));
#193490=CARTESIAN_POINT('Ctrl Pts',(-1.17421693835042,-24.9207705514448,
0.));
#193491=CARTESIAN_POINT('Ctrl Pts',(-1.18391538220104,-24.8974133481829,
0.));
#193492=CARTESIAN_POINT('Ctrl Pts',(-1.19352744434065,-24.8741077892075,
0.));
#193493=CARTESIAN_POINT('Ctrl Pts',(-1.20305318426021,-24.8508544481974,
0.));
#193494=CARTESIAN_POINT('Ctrl Pts',(-1.21249266318209,-24.8276539035092,
0.));
#193495=CARTESIAN_POINT('Ctrl Pts',(-1.22184594406529,-24.8045067380536,
0.));
#193496=CARTESIAN_POINT('Ctrl Pts',(-1.23111309161845,-24.7814135391799,
0.));
#193497=CARTESIAN_POINT('Ctrl Pts',(-1.2402941723199,-24.7583748985438,
0.));
#193498=CARTESIAN_POINT('Ctrl Pts',(-1.24938925444327,-24.7353914120011,
0.));
#193499=CARTESIAN_POINT('Ctrl Pts',(-1.25839840807419,-24.7124636797894,
0.));
#193500=CARTESIAN_POINT('Ctrl Pts',(-1.26732170513501,-24.6895923066836,
0.));
#193501=CARTESIAN_POINT('Ctrl Pts',(-1.27615921941643,-24.6667779021559,
0.));
#193502=CARTESIAN_POINT('Ctrl Pts',(-1.28491102661515,-24.6440210805278,
0.));
#193503=CARTESIAN_POINT('Ctrl Pts',(-1.29357720438108,-24.6213224611229,
0.));
#193504=CARTESIAN_POINT('Ctrl Pts',(-1.30215783236363,-24.5986826684027,
0.));
#193505=CARTESIAN_POINT('Ctrl Pts',(-1.31065299222023,-24.5761023320183,
0.));
#193506=CARTESIAN_POINT('Ctrl Pts',(-1.31906276763669,-24.5535820868674,
0.));
#193507=CARTESIAN_POINT('Ctrl Pts',(-1.32738724435327,-24.5311225731435,
0.));
#193508=CARTESIAN_POINT('Ctrl Pts',(-1.33562651019687,-24.5087244363856,
0.));
#193509=CARTESIAN_POINT('Ctrl Pts',(-1.34378065512339,-24.4863883275134,
0.));
#193510=CARTESIAN_POINT('Ctrl Pts',(-1.35184977125649,-24.4641149028892,
0.));
#193511=CARTESIAN_POINT('Ctrl Pts',(-1.35983395290628,-24.4419048244523,
0.));
#193512=CARTESIAN_POINT('Ctrl Pts',(-1.36773329659957,-24.4197587598337,
0.));
#193513=CARTESIAN_POINT('Ctrl Pts',(-1.3755479011161,-24.3976773824732,
0.));
#193514=CARTESIAN_POINT('Ctrl Pts',(-1.38327786753,-24.3756613717299,0.));
#193515=CARTESIAN_POINT('Ctrl Pts',(-1.39092329926389,-24.3537114129875,
0.));
#193516=CARTESIAN_POINT('Ctrl Pts',(-1.39848430212808,-24.3318281977643,
0.));
#193517=CARTESIAN_POINT('Ctrl Pts',(-1.40596098434338,-24.3100124238311,
0.));
#193518=CARTESIAN_POINT('Ctrl Pts',(-1.41335345657684,-24.288264795321,
0.));
#193519=CARTESIAN_POINT('Ctrl Pts',(-1.42066183198254,-24.2665860228356,
0.));
#193520=CARTESIAN_POINT('Ctrl Pts',(-1.42788622624855,-24.2449768235488,
0.));
#193521=CARTESIAN_POINT('Ctrl Pts',(-1.43502675765509,-24.2234379212984,
0.));
#193522=CARTESIAN_POINT('Ctrl Pts',(-1.44208354711083,-24.201970046722,
0.));
#193523=CARTESIAN_POINT('Ctrl Pts',(-1.44905671818729,-24.1805739374038,
0.));
#193524=CARTESIAN_POINT('Ctrl Pts',(-1.45594639716319,-24.1592503380107,
0.));
#193525=CARTESIAN_POINT('Ctrl Pts',(-1.46275271307399,-24.1380000004272,
0.));
#193526=CARTESIAN_POINT('Ctrl Pts',(-1.46947579776992,-24.1168236838824,
0.));
#193527=CARTESIAN_POINT('Ctrl Pts',(-1.47611578597743,-24.0957221550778,
0.));
#193528=CARTESIAN_POINT('Ctrl Pts',(-1.48267281533684,-24.0746961883528,
0.));
#193529=CARTESIAN_POINT('Ctrl Pts',(-1.48914702644888,-24.0537465658429,
0.));
#193530=CARTESIAN_POINT('Ctrl Pts',(-1.49553856292802,-24.0328740776331,
0.));
#193531=CARTESIAN_POINT('Ctrl Pts',(-1.501847571461,-24.0120795219086,0.));
#193532=CARTESIAN_POINT('Ctrl Pts',(-1.50807420187695,-23.9913637050927,
0.));
#193533=CARTESIAN_POINT('Ctrl Pts',(-1.51421860720615,-23.970727442014,
0.));
#193534=CARTESIAN_POINT('Ctrl Pts',(-1.52028094372793,-23.9501715561033,
0.));
#193535=CARTESIAN_POINT('Ctrl Pts',(-1.52626137103033,-23.9296968795757,
0.));
#193536=CARTESIAN_POINT('Ctrl Pts',(-1.53216005207464,-23.9093042536119,
0.));
#193537=CARTESIAN_POINT('Ctrl Pts',(-1.53797715326759,-23.8889945285318,
0.));
#193538=CARTESIAN_POINT('Ctrl Pts',(-1.54371284453991,-23.8687685639642,
0.));
#193539=CARTESIAN_POINT('Ctrl Pts',(-1.54936729940542,-23.8486272290705,
0.));
#193540=CARTESIAN_POINT('Ctrl Pts',(-1.55494069502636,-23.8285714027636,
0.));
#193541=CARTESIAN_POINT('Ctrl Pts',(-1.56043321228635,-23.8086019739194,
0.));
#193542=CARTESIAN_POINT('Ctrl Pts',(-1.56584503586844,-23.7887198415878,
0.));
#193543=CARTESIAN_POINT('Ctrl Pts',(-1.57117635434409,-23.7689259151862,
0.));
#193544=CARTESIAN_POINT('Ctrl Pts',(-1.57642736025247,-23.749221114736,
0.));
#193545=CARTESIAN_POINT('Ctrl Pts',(-1.58159825017359,-23.72960637113,0.));
#193546=CARTESIAN_POINT('Ctrl Pts',(-1.58668922481222,-23.710082626383,
0.));
#193547=CARTESIAN_POINT('Ctrl Pts',(-1.59170048908634,-23.6906508338833,
0.));
#193548=CARTESIAN_POINT('Ctrl Pts',(-1.59663225222464,-23.671311958631,
0.));
#193549=CARTESIAN_POINT('Ctrl Pts',(-1.60148472786596,-23.6520669774876,
0.));
#193550=CARTESIAN_POINT('Ctrl Pts',(-1.60625813414674,-23.6329168794929,
0.));
#193551=CARTESIAN_POINT('Ctrl Pts',(-1.61095269379779,-23.6138626661653,
0.));
#193552=CARTESIAN_POINT('Ctrl Pts',(-1.61556863424699,-23.5949053517997,
0.));
#193553=CARTESIAN_POINT('Ctrl Pts',(-1.62010618772867,-23.57604596376,0.));
#193554=CARTESIAN_POINT('Ctrl Pts',(-1.62456559140065,-23.5572855427601,
0.));
#193555=CARTESIAN_POINT('Ctrl Pts',(-1.62894708745224,-23.538625143226,
0.));
#193556=CARTESIAN_POINT('Ctrl Pts',(-1.63325092321727,-23.5200658336612,
0.));
#193557=CARTESIAN_POINT('Ctrl Pts',(-1.63747735129475,-23.5016086970003,
0.));
#193558=CARTESIAN_POINT('Ctrl Pts',(-1.64162662967529,-23.4832548309645,
0.));
#193559=CARTESIAN_POINT('Ctrl Pts',(-1.64569902187612,-23.4650053483932,
0.));
#193560=CARTESIAN_POINT('Ctrl Pts',(-1.64969479707341,-23.4468613776574,
0.));
#193561=CARTESIAN_POINT('Ctrl Pts',(-1.65361423023729,-23.4288240631043,
0.));
#193562=CARTESIAN_POINT('Ctrl Pts',(-1.65745760227506,-23.4108945654805,
0.));
#193563=CARTESIAN_POINT('Ctrl Pts',(-1.66122520018012,-23.3930740623619,
0.));
#193564=CARTESIAN_POINT('Ctrl Pts',(-1.66491731718878,-23.3753637485545,
0.));
#193565=CARTESIAN_POINT('Ctrl Pts',(-1.66853425293997,-23.3577648365744,
0.));
#193566=CARTESIAN_POINT('Ctrl Pts',(-1.67207631363923,-23.3402785571865,
0.));
#193567=CARTESIAN_POINT('Ctrl Pts',(-1.67554381222995,-23.3229061599145,
0.));
#193568=CARTESIAN_POINT('Ctrl Pts',(-1.67893706857118,-23.3056489135611,
0.));
#193569=CARTESIAN_POINT('Ctrl Pts',(-1.68225640962169,-23.2885081066951,
0.));
#193570=CARTESIAN_POINT('Ctrl Pts',(-1.68550216963259,-23.2714850482246,
0.));
#193571=CARTESIAN_POINT('Ctrl Pts',(-1.68867469034897,-23.2545810680537,
0.));
#193572=CARTESIAN_POINT('Ctrl Pts',(-1.69177432121712,-23.2377975177013,
0.));
#193573=CARTESIAN_POINT('Ctrl Pts',(-1.69480141959954,-23.2211357709374,
0.));
#193574=CARTESIAN_POINT('Ctrl Pts',(-1.69775635099444,-23.2045972243767,
0.));
#193575=CARTESIAN_POINT('Ctrl Pts',(-1.70063948927011,-23.1881832981851,
0.));
#193576=CARTESIAN_POINT('Ctrl Pts',(-1.70345121691277,-23.1718954368751,
0.));
#193577=CARTESIAN_POINT('Ctrl Pts',(-1.70619192527853,-23.1557351100614,
0.));
#193578=CARTESIAN_POINT('Ctrl Pts',(-1.70886201485453,-23.1397038132356,
0.));
#193579=CARTESIAN_POINT('Ctrl Pts',(-1.71146189552175,-23.1238030684925,
0.));
#193580=CARTESIAN_POINT('Ctrl Pts',(-1.71399198684705,-23.1080344254286,
0.));
#193581=CARTESIAN_POINT('Ctrl Pts',(-1.71645271839298,-23.0923994621213,
0.));
#193582=CARTESIAN_POINT('Ctrl Pts',(-1.71884453003028,-23.0768997860709,
0.));
#193583=CARTESIAN_POINT('Ctrl Pts',(-1.72116787225993,-23.0615370351562,
0.));
#193584=CARTESIAN_POINT('Ctrl Pts',(-1.72342320653748,-23.0463128785531,
0.));
#193585=CARTESIAN_POINT('Ctrl Pts',(-1.72561100564047,-23.0312290178883,
0.));
#193586=CARTESIAN_POINT('Ctrl Pts',(-1.7277317540471,-23.0162871884168,
0.));
#193587=CARTESIAN_POINT('Ctrl Pts',(-1.72978594832137,-23.001489160189,
0.));
#193588=CARTESIAN_POINT('Ctrl Pts',(-1.73177409750192,-22.9868367391978,
0.));
#193589=CARTESIAN_POINT('Ctrl Pts',(-1.73369672350816,-22.9723317685688,
0.));
#193590=CARTESIAN_POINT('Ctrl Pts',(-1.7355543616277,-22.9579761301063,
0.));
#193591=CARTESIAN_POINT('Ctrl Pts',(-1.7373475610004,-22.9437717457826,
0.));
#193592=CARTESIAN_POINT('Ctrl Pts',(-1.73907688511667,-22.9297205792586,
0.));
#193593=CARTESIAN_POINT('Ctrl Pts',(-1.74074291231059,-22.9158246373363,
0.));
#193594=CARTESIAN_POINT('Ctrl Pts',(-1.74234623630081,-22.9020859716141,
0.));
#193595=CARTESIAN_POINT('Ctrl Pts',(-1.74388746677703,-22.888506680335,
0.));
#193596=CARTESIAN_POINT('Ctrl Pts',(-1.74536722998202,-22.8750889101696,
0.));
#193597=CARTESIAN_POINT('Ctrl Pts',(-1.74678616930666,-22.8618348580235,
0.));
#193598=CARTESIAN_POINT('Ctrl Pts',(-1.74814494588494,-22.8487467728076,
0.));
#193599=CARTESIAN_POINT('Ctrl Pts',(-1.74944423940117,-22.8358269579853,
0.));
#193600=CARTESIAN_POINT('Ctrl Pts',(-1.75068474890884,-22.8230777741284,
0.));
#193601=CARTESIAN_POINT('Ctrl Pts',(-1.75186719365593,-22.8105016414713,
0.));
#193602=CARTESIAN_POINT('Ctrl Pts',(-1.75299231391467,-22.7981010424314,
0.));
#193603=CARTESIAN_POINT('Ctrl Pts',(-1.75406087182937,-22.7858785242361,
0.));
#193604=CARTESIAN_POINT('Ctrl Pts',(-1.75507365227133,-22.7738367016118,
0.));
#193605=CARTESIAN_POINT('Ctrl Pts',(-1.75603146371642,-22.7619782595013,
0.));
#193606=CARTESIAN_POINT('Ctrl Pts',(-1.75693513908908,-22.750305955645,
0.));
#193607=CARTESIAN_POINT('Ctrl Pts',(-1.75778553673245,-22.7388226235559,
0.));
#193608=CARTESIAN_POINT('Ctrl Pts',(-1.75858354204634,-22.72753117773,0.));
#193609=CARTESIAN_POINT('Ctrl Pts',(-1.75933006905926,-22.7164346186006,
0.));
#193610=CARTESIAN_POINT('Ctrl Pts',(-1.76002606202402,-22.7055360375485,
0.));
#193611=CARTESIAN_POINT('Ctrl Pts',(-1.76067249704888,-22.6948386219851,
0.));
#193612=CARTESIAN_POINT('Ctrl Pts',(-1.76127038310615,-22.684345658525,
0.));
#193613=CARTESIAN_POINT('Ctrl Pts',(-1.76182076289527,-22.67406053567,0.));
#193614=CARTESIAN_POINT('Ctrl Pts',(-1.7623247139257,-22.6639867471753,
0.));
#193615=CARTESIAN_POINT('Ctrl Pts',(-1.76278334912562,-22.654127893841,
0.));
#193616=CARTESIAN_POINT('Ctrl Pts',(-1.76319782013917,-22.6444876940423,
0.));
#193617=CARTESIAN_POINT('Ctrl Pts',(-1.76356932176274,-22.6350699979359,
0.));
#193618=CARTESIAN_POINT('Ctrl Pts',(-1.76389909571404,-22.6258787994848,
0.));
#193619=CARTESIAN_POINT('Ctrl Pts',(-1.7641884354374,-22.6169182517694,
0.));
#193620=CARTESIAN_POINT('Ctrl Pts',(-1.76443868648017,-22.6081926681343,
0.));
#193621=CARTESIAN_POINT('Ctrl Pts',(-1.76465124413558,-22.5997065145638,
0.));
#193622=CARTESIAN_POINT('Ctrl Pts',(-1.76482755288412,-22.5914644078106,
0.));
#193623=CARTESIAN_POINT('Ctrl Pts',(-1.76496910283089,-22.5834711038022,
0.));
#193624=CARTESIAN_POINT('Ctrl Pts',(-1.76507744026747,-22.5757315316353,
0.));
#193625=CARTESIAN_POINT('Ctrl Pts',(-1.76515418518832,-22.5682508499874,
0.));
#193626=CARTESIAN_POINT('Ctrl Pts',(-1.76520104500451,-22.5610344912501,
0.));
#193627=CARTESIAN_POINT('Ctrl Pts',(-1.76521983384063,-22.5540882235837,
0.));
#193628=CARTESIAN_POINT('Ctrl Pts',(-1.76521245524048,-22.5474180954006,
0.));
#193629=CARTESIAN_POINT('Ctrl Pts',(-1.76518087841494,-22.5410303590892,
0.));
#193630=CARTESIAN_POINT('Ctrl Pts',(-1.76512711563255,-22.5349313983571,
0.));
#193631=CARTESIAN_POINT('Ctrl Pts',(-1.7650532026276,-22.529127665298,0.));
#193632=CARTESIAN_POINT('Ctrl Pts',(-1.76496128643376,-22.5236259635515,
0.));
#193633=CARTESIAN_POINT('Ctrl Pts',(-1.76485369319896,-22.5184336670207,
0.));
#193634=CARTESIAN_POINT('Ctrl Pts',(-1.7647330328115,-22.5135590569554,
0.));
#193635=CARTESIAN_POINT('Ctrl Pts',(-1.76460218257314,-22.5090112700212,
0.));
#193636=CARTESIAN_POINT('Ctrl Pts',(-1.76446408210366,-22.5047996391978,
0.));
#193637=CARTESIAN_POINT('Ctrl Pts',(-1.76432160068739,-22.5009332677316,
0.));
#193638=CARTESIAN_POINT('Ctrl Pts',(-1.76417731243484,-22.4974203063191,
0.));
#193639=CARTESIAN_POINT('Ctrl Pts',(-1.76403393880317,-22.4942693792449,
0.));
#193640=CARTESIAN_POINT('Ctrl Pts',(-1.76389475965715,-22.4914909094908,
0.));
#193641=CARTESIAN_POINT('Ctrl Pts',(-1.76376424879469,-22.4890991659479,
0.));
#193642=CARTESIAN_POINT('Ctrl Pts',(-1.76364784232926,-22.4871115206572,
0.));
#193643=CARTESIAN_POINT('Ctrl Pts',(-1.7635507604555,-22.4855446605991,
0.));
#193644=CARTESIAN_POINT('Ctrl Pts',(-1.76347698284863,-22.4844112933125,
0.));
#193645=CARTESIAN_POINT('Ctrl Pts',(-1.7634381343466,-22.4838562517064,
0.));
#193646=CARTESIAN_POINT('Ctrl Pts',(-1.76342064263638,-22.4836387052228,
0.));
#193647=CARTESIAN_POINT('Ctrl Pts',(-1.76341415538792,-22.4835819929788,
0.));
#193648=CARTESIAN_POINT('Ctrl Pts',(-1.76341220531181,-22.4835757167854,
0.));
#193649=CARTESIAN_POINT('',(-0.661312440730913,-25.991588367311,0.));
#193650=CARTESIAN_POINT('Ctrl Pts',(-4.11585220600463,-22.1738711152697,
0.));
#193651=CARTESIAN_POINT('Ctrl Pts',(-4.11585220600463,-22.1738711152697,
12.));
#193652=CARTESIAN_POINT('Ctrl Pts',(-4.11585194677443,-22.173877682324,
0.));
#193653=CARTESIAN_POINT('Ctrl Pts',(-4.11585194677443,-22.173877682324,
12.));
#193654=CARTESIAN_POINT('Ctrl Pts',(-4.11586035878288,-22.1739341411687,
0.));
#193655=CARTESIAN_POINT('Ctrl Pts',(-4.11586035878288,-22.1739341411687,
12.));
#193656=CARTESIAN_POINT('Ctrl Pts',(-4.11589976826167,-22.1741488021234,
0.));
#193657=CARTESIAN_POINT('Ctrl Pts',(-4.11589976826167,-22.1741488021234,
12.));
#193658=CARTESIAN_POINT('Ctrl Pts',(-4.11600589882846,-22.1746949858775,
0.));
#193659=CARTESIAN_POINT('Ctrl Pts',(-4.11600589882846,-22.1746949858775,
12.));
#193660=CARTESIAN_POINT('Ctrl Pts',(-4.11622797217069,-22.1758088296598,
0.));
#193661=CARTESIAN_POINT('Ctrl Pts',(-4.11622797217069,-22.1758088296598,
12.));
#193662=CARTESIAN_POINT('Ctrl Pts',(-4.11653973150519,-22.177347426894,
0.));
#193663=CARTESIAN_POINT('Ctrl Pts',(-4.11653973150519,-22.177347426894,
12.));
#193664=CARTESIAN_POINT('Ctrl Pts',(-4.11694173195005,-22.179297473024,
0.));
#193665=CARTESIAN_POINT('Ctrl Pts',(-4.11694173195005,-22.179297473024,
12.));
#193666=CARTESIAN_POINT('Ctrl Pts',(-4.11743469691757,-22.1816414985788,
0.));
#193667=CARTESIAN_POINT('Ctrl Pts',(-4.11743469691757,-22.1816414985788,
12.));
#193668=CARTESIAN_POINT('Ctrl Pts',(-4.11801938107481,-22.1843613164855,
0.));
#193669=CARTESIAN_POINT('Ctrl Pts',(-4.11801938107481,-22.1843613164855,
12.));
#193670=CARTESIAN_POINT('Ctrl Pts',(-4.11869641271774,-22.1874419861496,
0.));
#193671=CARTESIAN_POINT('Ctrl Pts',(-4.11869641271774,-22.1874419861496,
12.));
#193672=CARTESIAN_POINT('Ctrl Pts',(-4.11946626228637,-22.1908725908525,
0.));
#193673=CARTESIAN_POINT('Ctrl Pts',(-4.11946626228637,-22.1908725908525,
12.));
#193674=CARTESIAN_POINT('Ctrl Pts',(-4.12032932637737,-22.1946440958098,
0.));
#193675=CARTESIAN_POINT('Ctrl Pts',(-4.12032932637737,-22.1946440958098,
12.));
#193676=CARTESIAN_POINT('Ctrl Pts',(-4.12128598183523,-22.1987479618246,
0.));
#193677=CARTESIAN_POINT('Ctrl Pts',(-4.12128598183523,-22.1987479618246,
12.));
#193678=CARTESIAN_POINT('Ctrl Pts',(-4.12233664408228,-22.2031746532106,
0.));
#193679=CARTESIAN_POINT('Ctrl Pts',(-4.12233664408228,-22.2031746532106,
12.));
#193680=CARTESIAN_POINT('Ctrl Pts',(-4.12348173702024,-22.2079143941719,
0.));
#193681=CARTESIAN_POINT('Ctrl Pts',(-4.12348173702024,-22.2079143941719,
12.));
#193682=CARTESIAN_POINT('Ctrl Pts',(-4.12472167516608,-22.2129576146671,
0.));
#193683=CARTESIAN_POINT('Ctrl Pts',(-4.12472167516608,-22.2129576146671,
12.));
#193684=CARTESIAN_POINT('Ctrl Pts',(-4.12605683613308,-22.2182956401341,
0.));
#193685=CARTESIAN_POINT('Ctrl Pts',(-4.12605683613308,-22.2182956401341,
12.));
#193686=CARTESIAN_POINT('Ctrl Pts',(-4.12748755830105,-22.2239207458781,
0.));
#193687=CARTESIAN_POINT('Ctrl Pts',(-4.12748755830105,-22.2239207458781,
12.));
#193688=CARTESIAN_POINT('Ctrl Pts',(-4.1290141546338,-22.2298258043947,
0.));
#193689=CARTESIAN_POINT('Ctrl Pts',(-4.1290141546338,-22.2298258043947,
12.));
#193690=CARTESIAN_POINT('Ctrl Pts',(-4.13063692157499,-22.2360040565533,
0.));
#193691=CARTESIAN_POINT('Ctrl Pts',(-4.13063692157499,-22.2360040565533,
12.));
#193692=CARTESIAN_POINT('Ctrl Pts',(-4.13235615060161,-22.2424488153523,
0.));
#193693=CARTESIAN_POINT('Ctrl Pts',(-4.13235615060161,-22.2424488153523,
12.));
#193694=CARTESIAN_POINT('Ctrl Pts',(-4.13417212558811,-22.249153531779,
0.));
#193695=CARTESIAN_POINT('Ctrl Pts',(-4.13417212558811,-22.249153531779,
12.));
#193696=CARTESIAN_POINT('Ctrl Pts',(-4.13608511977226,-22.2561118708421,
0.));
#193697=CARTESIAN_POINT('Ctrl Pts',(-4.13608511977226,-22.2561118708421,
12.));
#193698=CARTESIAN_POINT('Ctrl Pts',(-4.13809539255423,-22.2633177913972,
0.));
#193699=CARTESIAN_POINT('Ctrl Pts',(-4.13809539255423,-22.2633177913972,
12.));
#193700=CARTESIAN_POINT('Ctrl Pts',(-4.14020318715992,-22.2707656042457,
0.));
#193701=CARTESIAN_POINT('Ctrl Pts',(-4.14020318715992,-22.2707656042457,
12.));
#193702=CARTESIAN_POINT('Ctrl Pts',(-4.14240873321985,-22.2784499072027,
0.));
#193703=CARTESIAN_POINT('Ctrl Pts',(-4.14240873321985,-22.2784499072027,
12.));
#193704=CARTESIAN_POINT('Ctrl Pts',(-4.14471224859296,-22.2863655389166,
0.));
#193705=CARTESIAN_POINT('Ctrl Pts',(-4.14471224859296,-22.2863655389166,
12.));
#193706=CARTESIAN_POINT('Ctrl Pts',(-4.14711394168557,-22.2945075198467,
0.));
#193707=CARTESIAN_POINT('Ctrl Pts',(-4.14711394168557,-22.2945075198467,
12.));
#193708=CARTESIAN_POINT('Ctrl Pts',(-4.14961401285523,-22.3028710166933,
0.));
#193709=CARTESIAN_POINT('Ctrl Pts',(-4.14961401285523,-22.3028710166933,
12.));
#193710=CARTESIAN_POINT('Ctrl Pts',(-4.15221265396991,-22.3114513545185,
0.));
#193711=CARTESIAN_POINT('Ctrl Pts',(-4.15221265396991,-22.3114513545185,
12.));
#193712=CARTESIAN_POINT('Ctrl Pts',(-4.15491004835282,-22.320244018698,
0.));
#193713=CARTESIAN_POINT('Ctrl Pts',(-4.15491004835282,-22.320244018698,
12.));
#193714=CARTESIAN_POINT('Ctrl Pts',(-4.15770637047891,-22.3292446628959,
0.));
#193715=CARTESIAN_POINT('Ctrl Pts',(-4.15770637047891,-22.3292446628959,
12.));
#193716=CARTESIAN_POINT('Ctrl Pts',(-4.16060178604165,-22.3384491078602,
0.));
#193717=CARTESIAN_POINT('Ctrl Pts',(-4.16060178604165,-22.3384491078602,
12.));
#193718=CARTESIAN_POINT('Ctrl Pts',(-4.16359645263189,-22.3478533253889,
0.));
#193719=CARTESIAN_POINT('Ctrl Pts',(-4.16359645263189,-22.3478533253889,
12.));
#193720=CARTESIAN_POINT('Ctrl Pts',(-4.16669052026601,-22.3574534257396,
0.));
#193721=CARTESIAN_POINT('Ctrl Pts',(-4.16669052026601,-22.3574534257396,
12.));
#193722=CARTESIAN_POINT('Ctrl Pts',(-4.16988413199458,-22.36724564276,0.));
#193723=CARTESIAN_POINT('Ctrl Pts',(-4.16988413199458,-22.36724564276,12.));
#193724=CARTESIAN_POINT('Ctrl Pts',(-4.17317742436146,-22.3772263228617,
0.));
#193725=CARTESIAN_POINT('Ctrl Pts',(-4.17317742436146,-22.3772263228617,
12.));
#193726=CARTESIAN_POINT('Ctrl Pts',(-4.17657052752826,-22.3873919231334,
0.));
#193727=CARTESIAN_POINT('Ctrl Pts',(-4.17657052752826,-22.3873919231334,
12.));
#193728=CARTESIAN_POINT('Ctrl Pts',(-4.18006356544883,-22.3977390078075,
0.));
#193729=CARTESIAN_POINT('Ctrl Pts',(-4.18006356544883,-22.3977390078075,
12.));
#193730=CARTESIAN_POINT('Ctrl Pts',(-4.18365665600851,-22.4082642454453,
0.));
#193731=CARTESIAN_POINT('Ctrl Pts',(-4.18365665600851,-22.4082642454453,
12.));
#193732=CARTESIAN_POINT('Ctrl Pts',(-4.18734991117722,-22.4189644056115,
0.));
#193733=CARTESIAN_POINT('Ctrl Pts',(-4.18734991117722,-22.4189644056115,
12.));
#193734=CARTESIAN_POINT('Ctrl Pts',(-4.19114343726943,-22.4298363535421,
0.));
#193735=CARTESIAN_POINT('Ctrl Pts',(-4.19114343726943,-22.4298363535421,
12.));
#193736=CARTESIAN_POINT('Ctrl Pts',(-4.19503733518862,-22.4408770448917,
0.));
#193737=CARTESIAN_POINT('Ctrl Pts',(-4.19503733518862,-22.4408770448917,
12.));
#193738=CARTESIAN_POINT('Ctrl Pts',(-4.19903170066356,-22.4520835205419,
0.));
#193739=CARTESIAN_POINT('Ctrl Pts',(-4.19903170066356,-22.4520835205419,
12.));
#193740=CARTESIAN_POINT('Ctrl Pts',(-4.20312662448172,-22.4634529011433,
0.));
#193741=CARTESIAN_POINT('Ctrl Pts',(-4.20312662448172,-22.4634529011433,
12.));
#193742=CARTESIAN_POINT('Ctrl Pts',(-4.20732219265649,-22.4749823839915,
0.));
#193743=CARTESIAN_POINT('Ctrl Pts',(-4.20732219265649,-22.4749823839915,
12.));
#193744=CARTESIAN_POINT('Ctrl Pts',(-4.21161848657429,-22.4866692403147,
0.));
#193745=CARTESIAN_POINT('Ctrl Pts',(-4.21161848657429,-22.4866692403147,
12.));
#193746=CARTESIAN_POINT('Ctrl Pts',(-4.21601558313909,-22.4985108124229,
0.));
#193747=CARTESIAN_POINT('Ctrl Pts',(-4.21601558313909,-22.4985108124229,
12.));
#193748=CARTESIAN_POINT('Ctrl Pts',(-4.22051355490198,-22.5105045108882,
0.));
#193749=CARTESIAN_POINT('Ctrl Pts',(-4.22051355490198,-22.5105045108882,
12.));
#193750=CARTESIAN_POINT('Ctrl Pts',(-4.22511247020041,-22.5226478117885,
0.));
#193751=CARTESIAN_POINT('Ctrl Pts',(-4.22511247020041,-22.5226478117885,
12.));
#193752=CARTESIAN_POINT('Ctrl Pts',(-4.22981239330732,-22.5349382540587,
0.));
#193753=CARTESIAN_POINT('Ctrl Pts',(-4.22981239330732,-22.5349382540587,
12.));
#193754=CARTESIAN_POINT('Ctrl Pts',(-4.23461338456714,-22.5473734368086,
0.));
#193755=CARTESIAN_POINT('Ctrl Pts',(-4.23461338456714,-22.5473734368086,
12.));
#193756=CARTESIAN_POINT('Ctrl Pts',(-4.23951550052527,-22.559951016643,
0.));
#193757=CARTESIAN_POINT('Ctrl Pts',(-4.23951550052527,-22.559951016643,
12.));
#193758=CARTESIAN_POINT('Ctrl Pts',(-4.2445187940486,-22.5726687049922,
0.));
#193759=CARTESIAN_POINT('Ctrl Pts',(-4.2445187940486,-22.5726687049922,
12.));
#193760=CARTESIAN_POINT('Ctrl Pts',(-4.24962331444186,-22.5855242662479,
0.));
#193761=CARTESIAN_POINT('Ctrl Pts',(-4.24962331444186,-22.5855242662479,
12.));
#193762=CARTESIAN_POINT('Ctrl Pts',(-4.25482910755486,-22.5985155158637,
0.));
#193763=CARTESIAN_POINT('Ctrl Pts',(-4.25482910755486,-22.5985155158637,
12.));
#193764=CARTESIAN_POINT('Ctrl Pts',(-4.26013621588304,-22.611640318482,
0.));
#193765=CARTESIAN_POINT('Ctrl Pts',(-4.26013621588304,-22.611640318482,
12.));
#193766=CARTESIAN_POINT('Ctrl Pts',(-4.26554467865572,-22.6248965859975,
0.));
#193767=CARTESIAN_POINT('Ctrl Pts',(-4.26554467865572,-22.6248965859975,
12.));
#193768=CARTESIAN_POINT('Ctrl Pts',(-4.27105453193,-22.6382822758171,0.));
#193769=CARTESIAN_POINT('Ctrl Pts',(-4.27105453193,-22.6382822758171,12.));
#193770=CARTESIAN_POINT('Ctrl Pts',(-4.27666580869118,-22.6517953893303,
0.));
#193771=CARTESIAN_POINT('Ctrl Pts',(-4.27666580869118,-22.6517953893303,
12.));
#193772=CARTESIAN_POINT('Ctrl Pts',(-4.2823785389406,-22.665433970311,0.));
#193773=CARTESIAN_POINT('Ctrl Pts',(-4.2823785389406,-22.665433970311,12.));
#193774=CARTESIAN_POINT('Ctrl Pts',(-4.28819274977767,-22.6791961033536,
0.));
#193775=CARTESIAN_POINT('Ctrl Pts',(-4.28819274977767,-22.6791961033536,
12.));
#193776=CARTESIAN_POINT('Ctrl Pts',(-4.29410846547062,-22.6930799122545,
0.));
#193777=CARTESIAN_POINT('Ctrl Pts',(-4.29410846547062,-22.6930799122545,
12.));
#193778=CARTESIAN_POINT('Ctrl Pts',(-4.30012570754067,-22.707083558756,
0.));
#193779=CARTESIAN_POINT('Ctrl Pts',(-4.30012570754067,-22.707083558756,
12.));
#193780=CARTESIAN_POINT('Ctrl Pts',(-4.30624449484075,-22.7212052413384,
0.));
#193781=CARTESIAN_POINT('Ctrl Pts',(-4.30624449484075,-22.7212052413384,
12.));
#193782=CARTESIAN_POINT('Ctrl Pts',(-4.31246484362551,-22.7354431939926,
0.));
#193783=CARTESIAN_POINT('Ctrl Pts',(-4.31246484362551,-22.7354431939926,
12.));
#193784=CARTESIAN_POINT('Ctrl Pts',(-4.31878676761231,-22.7497956849852,
0.));
#193785=CARTESIAN_POINT('Ctrl Pts',(-4.31878676761231,-22.7497956849852,
12.));
#193786=CARTESIAN_POINT('Ctrl Pts',(-4.32521027803748,-22.764261015648,
0.));
#193787=CARTESIAN_POINT('Ctrl Pts',(-4.32521027803748,-22.764261015648,
12.));
#193788=CARTESIAN_POINT('Ctrl Pts',(-4.33173538373183,-22.7788375194081,
0.));
#193789=CARTESIAN_POINT('Ctrl Pts',(-4.33173538373183,-22.7788375194081,
12.));
#193790=CARTESIAN_POINT('Ctrl Pts',(-4.33836209118444,-22.7935235607807,
0.));
#193791=CARTESIAN_POINT('Ctrl Pts',(-4.33836209118444,-22.7935235607807,
12.));
#193792=CARTESIAN_POINT('Ctrl Pts',(-4.34509040460066,-22.808317534379,
0.));
#193793=CARTESIAN_POINT('Ctrl Pts',(-4.34509040460066,-22.808317534379,
12.));
#193794=CARTESIAN_POINT('Ctrl Pts',(-4.35192032594802,-22.8232178638873,
0.));
#193795=CARTESIAN_POINT('Ctrl Pts',(-4.35192032594802,-22.8232178638873,
12.));
#193796=CARTESIAN_POINT('Ctrl Pts',(-4.3588518550056,-22.838223001118,0.));
#193797=CARTESIAN_POINT('Ctrl Pts',(-4.3588518550056,-22.838223001118,12.));
#193798=CARTESIAN_POINT('Ctrl Pts',(-4.36588498943011,-22.8533314252419,
0.));
#193799=CARTESIAN_POINT('Ctrl Pts',(-4.36588498943011,-22.8533314252419,
12.));
#193800=CARTESIAN_POINT('Ctrl Pts',(-4.37301972480753,-22.8685416419725,
0.));
#193801=CARTESIAN_POINT('Ctrl Pts',(-4.37301972480753,-22.8685416419725,
12.));
#193802=CARTESIAN_POINT('Ctrl Pts',(-4.38025605470091,-22.8838521827702,
0.));
#193803=CARTESIAN_POINT('Ctrl Pts',(-4.38025605470091,-22.8838521827702,
12.));
#193804=CARTESIAN_POINT('Ctrl Pts',(-4.38759397068393,-22.8992616040108,
0.));
#193805=CARTESIAN_POINT('Ctrl Pts',(-4.38759397068393,-22.8992616040108,
12.));
#193806=CARTESIAN_POINT('Ctrl Pts',(-4.39503346238455,-22.9147684862425,
0.));
#193807=CARTESIAN_POINT('Ctrl Pts',(-4.39503346238455,-22.9147684862425,
12.));
#193808=CARTESIAN_POINT('Ctrl Pts',(-4.40257451754308,-22.9303714335549,
0.));
#193809=CARTESIAN_POINT('Ctrl Pts',(-4.40257451754308,-22.9303714335549,
12.));
#193810=CARTESIAN_POINT('Ctrl Pts',(-4.41021712205549,-22.9460690729093,
0.));
#193811=CARTESIAN_POINT('Ctrl Pts',(-4.41021712205549,-22.9460690729093,
12.));
#193812=CARTESIAN_POINT('Ctrl Pts',(-4.41796126001311,-22.9618600534866,
0.));
#193813=CARTESIAN_POINT('Ctrl Pts',(-4.41796126001311,-22.9618600534866,
12.));
#193814=CARTESIAN_POINT('Ctrl Pts',(-4.42580691372772,-22.9777430460021,
0.));
#193815=CARTESIAN_POINT('Ctrl Pts',(-4.42580691372772,-22.9777430460021,
12.));
#193816=CARTESIAN_POINT('Ctrl Pts',(-4.43375406376906,-22.9937167421009,
0.));
#193817=CARTESIAN_POINT('Ctrl Pts',(-4.43375406376906,-22.9937167421009,
12.));
#193818=CARTESIAN_POINT('Ctrl Pts',(-4.44180268901667,-23.0097798538399,
0.));
#193819=CARTESIAN_POINT('Ctrl Pts',(-4.44180268901667,-23.0097798538399,
12.));
#193820=CARTESIAN_POINT('Ctrl Pts',(-4.44995276669699,-23.0259311131395,
0.));
#193821=CARTESIAN_POINT('Ctrl Pts',(-4.44995276669699,-23.0259311131395,
12.));
#193822=CARTESIAN_POINT('Ctrl Pts',(-4.45820427241677,-23.0421692712466,
0.));
#193823=CARTESIAN_POINT('Ctrl Pts',(-4.45820427241677,-23.0421692712466,
12.));
#193824=CARTESIAN_POINT('Ctrl Pts',(-4.46655718018206,-23.0584930981723,
0.));
#193825=CARTESIAN_POINT('Ctrl Pts',(-4.46655718018206,-23.0584930981723,
12.));
#193826=CARTESIAN_POINT('Ctrl Pts',(-4.47501146242822,-23.0749013821867,
0.));
#193827=CARTESIAN_POINT('Ctrl Pts',(-4.47501146242822,-23.0749013821867,
12.));
#193828=CARTESIAN_POINT('Ctrl Pts',(-4.48356709006757,-23.0913929293909,
0.));
#193829=CARTESIAN_POINT('Ctrl Pts',(-4.48356709006757,-23.0913929293909,
12.));
#193830=CARTESIAN_POINT('Ctrl Pts',(-4.49222403252202,-23.1079665632629,
0.));
#193831=CARTESIAN_POINT('Ctrl Pts',(-4.49222403252202,-23.1079665632629,
12.));
#193832=CARTESIAN_POINT('Ctrl Pts',(-4.50098225775179,-23.1246211242117,
0.));
#193833=CARTESIAN_POINT('Ctrl Pts',(-4.50098225775179,-23.1246211242117,
12.));
#193834=CARTESIAN_POINT('Ctrl Pts',(-4.50984173227088,-23.1413554691136,
0.));
#193835=CARTESIAN_POINT('Ctrl Pts',(-4.50984173227088,-23.1413554691136,
12.));
#193836=CARTESIAN_POINT('Ctrl Pts',(-4.51880242116786,-23.1581684708778,
0.));
#193837=CARTESIAN_POINT('Ctrl Pts',(-4.51880242116786,-23.1581684708778,
12.));
#193838=CARTESIAN_POINT('Ctrl Pts',(-4.52786428815049,-23.1750590180923,
0.));
#193839=CARTESIAN_POINT('Ctrl Pts',(-4.52786428815049,-23.1750590180923,
12.));
#193840=CARTESIAN_POINT('Ctrl Pts',(-4.53702729557586,-23.1920260146474,
0.));
#193841=CARTESIAN_POINT('Ctrl Pts',(-4.53702729557586,-23.1920260146474,
12.));
#193842=CARTESIAN_POINT('Ctrl Pts',(-4.54629140447543,-23.2090683793627,
0.));
#193843=CARTESIAN_POINT('Ctrl Pts',(-4.54629140447543,-23.2090683793627,
12.));
#193844=CARTESIAN_POINT('Ctrl Pts',(-4.55565657456957,-23.2261850456055,
0.));
#193845=CARTESIAN_POINT('Ctrl Pts',(-4.55565657456957,-23.2261850456055,
12.));
#193846=CARTESIAN_POINT('Ctrl Pts',(-4.56512276427812,-23.2433749609117,
0.));
#193847=CARTESIAN_POINT('Ctrl Pts',(-4.56512276427812,-23.2433749609117,
12.));
#193848=CARTESIAN_POINT('Ctrl Pts',(-4.57468993076071,-23.2606370866854,
0.));
#193849=CARTESIAN_POINT('Ctrl Pts',(-4.57468993076071,-23.2606370866854,
12.));
#193850=CARTESIAN_POINT('Ctrl Pts',(-4.58435802994675,-23.2779703978868,
0.));
#193851=CARTESIAN_POINT('Ctrl Pts',(-4.58435802994675,-23.2779703978868,
12.));
#193852=CARTESIAN_POINT('Ctrl Pts',(-4.5941270165575,-23.295373882719,0.));
#193853=CARTESIAN_POINT('Ctrl Pts',(-4.5941270165575,-23.295373882719,12.));
#193854=CARTESIAN_POINT('Ctrl Pts',(-4.60399684412176,-23.3128465423119,
0.));
#193855=CARTESIAN_POINT('Ctrl Pts',(-4.60399684412176,-23.3128465423119,
12.));
#193856=CARTESIAN_POINT('Ctrl Pts',(-4.61396746497849,-23.3303873903947,
0.));
#193857=CARTESIAN_POINT('Ctrl Pts',(-4.61396746497849,-23.3303873903947,
12.));
#193858=CARTESIAN_POINT('Ctrl Pts',(-4.62403883030825,-23.3479954530281,
0.));
#193859=CARTESIAN_POINT('Ctrl Pts',(-4.62403883030825,-23.3479954530281,
12.));
#193860=CARTESIAN_POINT('Ctrl Pts',(-4.63421089016555,-23.3656697683496,
0.));
#193861=CARTESIAN_POINT('Ctrl Pts',(-4.63421089016555,-23.3656697683496,
12.));
#193862=CARTESIAN_POINT('Ctrl Pts',(-4.64448359349936,-23.383409386307,
0.));
#193863=CARTESIAN_POINT('Ctrl Pts',(-4.64448359349936,-23.383409386307,
12.));
#193864=CARTESIAN_POINT('Ctrl Pts',(-4.65485688816923,-23.4012133683957,
0.));
#193865=CARTESIAN_POINT('Ctrl Pts',(-4.65485688816923,-23.4012133683957,
12.));
#193866=CARTESIAN_POINT('Ctrl Pts',(-4.66533072094664,-23.4190807873798,
0.));
#193867=CARTESIAN_POINT('Ctrl Pts',(-4.66533072094664,-23.4190807873798,
12.));
#193868=CARTESIAN_POINT('Ctrl Pts',(-4.67590503753051,-23.4370107270444,
0.));
#193869=CARTESIAN_POINT('Ctrl Pts',(-4.67590503753051,-23.4370107270444,
12.));
#193870=CARTESIAN_POINT('Ctrl Pts',(-4.68657978258298,-23.4550022819852,
0.));
#193871=CARTESIAN_POINT('Ctrl Pts',(-4.68657978258298,-23.4550022819852,
12.));
#193872=CARTESIAN_POINT('Ctrl Pts',(-4.69735489975024,-23.4730545573849,
0.));
#193873=CARTESIAN_POINT('Ctrl Pts',(-4.69735489975024,-23.4730545573849,
12.));
#193874=CARTESIAN_POINT('Ctrl Pts',(-4.70823033167821,-23.491166668789,
0.));
#193875=CARTESIAN_POINT('Ctrl Pts',(-4.70823033167821,-23.491166668789,
12.));
#193876=CARTESIAN_POINT('Ctrl Pts',(-4.71920602001905,-23.5093377418784,
0.));
#193877=CARTESIAN_POINT('Ctrl Pts',(-4.71920602001905,-23.5093377418784,
12.));
#193878=CARTESIAN_POINT('Ctrl Pts',(-4.73028190543032,-23.5275669122378,
0.));
#193879=CARTESIAN_POINT('Ctrl Pts',(-4.73028190543032,-23.5275669122378,
12.));
#193880=CARTESIAN_POINT('Ctrl Pts',(-4.74145792760699,-23.5458533251715,
0.));
#193881=CARTESIAN_POINT('Ctrl Pts',(-4.74145792760699,-23.5458533251715,
12.));
#193882=CARTESIAN_POINT('Ctrl Pts',(-4.75273402530616,-23.564196135517,
0.));
#193883=CARTESIAN_POINT('Ctrl Pts',(-4.75273402530616,-23.564196135517,
12.));
#193884=CARTESIAN_POINT('Ctrl Pts',(-4.76411013636252,-23.5825945074535,
0.));
#193885=CARTESIAN_POINT('Ctrl Pts',(-4.76411013636252,-23.5825945074535,
12.));
#193886=CARTESIAN_POINT('Ctrl Pts',(-4.77558619769876,-23.6010476143099,
0.));
#193887=CARTESIAN_POINT('Ctrl Pts',(-4.77558619769876,-23.6010476143099,
12.));
#193888=CARTESIAN_POINT('Ctrl Pts',(-4.78716214532105,-23.6195546383625,
0.));
#193889=CARTESIAN_POINT('Ctrl Pts',(-4.78716214532105,-23.6195546383625,
12.));
#193890=CARTESIAN_POINT('Ctrl Pts',(-4.79883791433231,-23.6381147706581,
0.));
#193891=CARTESIAN_POINT('Ctrl Pts',(-4.79883791433231,-23.6381147706581,
12.));
#193892=CARTESIAN_POINT('Ctrl Pts',(-4.81061343896443,-23.6567272108631,
0.));
#193893=CARTESIAN_POINT('Ctrl Pts',(-4.81061343896443,-23.6567272108631,
12.));
#193894=CARTESIAN_POINT('Ctrl Pts',(-4.82248865259571,-23.6753911671023,
0.));
#193895=CARTESIAN_POINT('Ctrl Pts',(-4.82248865259571,-23.6753911671023,
12.));
#193896=CARTESIAN_POINT('Ctrl Pts',(-4.83446348776268,-23.6941058557971,
0.));
#193897=CARTESIAN_POINT('Ctrl Pts',(-4.83446348776268,-23.6941058557971,
12.));
#193898=CARTESIAN_POINT('Ctrl Pts',(-4.84653787616424,-23.7128705015014,
0.));
#193899=CARTESIAN_POINT('Ctrl Pts',(-4.84653787616424,-23.7128705015014,
12.));
#193900=CARTESIAN_POINT('Ctrl Pts',(-4.85871174865492,-23.7316843367308,
0.));
#193901=CARTESIAN_POINT('Ctrl Pts',(-4.85871174865492,-23.7316843367308,
12.));
#193902=CARTESIAN_POINT('Ctrl Pts',(-4.87098503527144,-23.7505466018239,
0.));
#193903=CARTESIAN_POINT('Ctrl Pts',(-4.87098503527144,-23.7505466018239,
12.));
#193904=CARTESIAN_POINT('Ctrl Pts',(-4.88335766525566,-23.7694565448044,
0.));
#193905=CARTESIAN_POINT('Ctrl Pts',(-4.88335766525566,-23.7694565448044,
12.));
#193906=CARTESIAN_POINT('Ctrl Pts',(-4.89582956706772,-23.7884134212381,
0.));
#193907=CARTESIAN_POINT('Ctrl Pts',(-4.89582956706772,-23.7884134212381,
12.));
#193908=CARTESIAN_POINT('Ctrl Pts',(-4.90840066839348,-23.8074164940897,
0.));
#193909=CARTESIAN_POINT('Ctrl Pts',(-4.90840066839348,-23.8074164940897,
12.));
#193910=CARTESIAN_POINT('Ctrl Pts',(-4.92107089613977,-23.8264650335721,
0.));
#193911=CARTESIAN_POINT('Ctrl Pts',(-4.92107089613977,-23.8264650335721,
12.));
#193912=CARTESIAN_POINT('Ctrl Pts',(-4.93384017643442,-23.8455583170062,
0.));
#193913=CARTESIAN_POINT('Ctrl Pts',(-4.93384017643442,-23.8455583170062,
12.));
#193914=CARTESIAN_POINT('Ctrl Pts',(-4.94670843465869,-23.8646956287172,
0.));
#193915=CARTESIAN_POINT('Ctrl Pts',(-4.94670843465869,-23.8646956287172,
12.));
#193916=CARTESIAN_POINT('Ctrl Pts',(-4.95967559546566,-23.883876259922,
0.));
#193917=CARTESIAN_POINT('Ctrl Pts',(-4.95967559546566,-23.883876259922,
12.));
#193918=CARTESIAN_POINT('Ctrl Pts',(-4.9727415827923,-23.9030995086164,
0.));
#193919=CARTESIAN_POINT('Ctrl Pts',(-4.9727415827923,-23.9030995086164,
12.));
#193920=CARTESIAN_POINT('Ctrl Pts',(-4.98590631986534,-23.9223646794591,
0.));
#193921=CARTESIAN_POINT('Ctrl Pts',(-4.98590631986534,-23.9223646794591,
12.));
#193922=CARTESIAN_POINT('Ctrl Pts',(-4.9991697291931,-23.9416710836529,
0.));
#193923=CARTESIAN_POINT('Ctrl Pts',(-4.9991697291931,-23.9416710836529,
12.));
#193924=CARTESIAN_POINT('Ctrl Pts',(-5.01253173257459,-23.9610180388271,
0.));
#193925=CARTESIAN_POINT('Ctrl Pts',(-5.01253173257459,-23.9610180388271,
12.));
#193926=CARTESIAN_POINT('Ctrl Pts',(-5.02599225112462,-23.9804048689228,
0.));
#193927=CARTESIAN_POINT('Ctrl Pts',(-5.02599225112462,-23.9804048689228,
12.));
#193928=CARTESIAN_POINT('Ctrl Pts',(-5.03955120528528,-23.9998309040747,
0.));
#193929=CARTESIAN_POINT('Ctrl Pts',(-5.03955120528528,-23.9998309040747,
12.));
#193930=CARTESIAN_POINT('Ctrl Pts',(-5.05320851483069,-24.0192954804896,
0.));
#193931=CARTESIAN_POINT('Ctrl Pts',(-5.05320851483069,-24.0192954804896,
12.));
#193932=CARTESIAN_POINT('Ctrl Pts',(-5.0669640988664,-24.0387979403268,
0.));
#193933=CARTESIAN_POINT('Ctrl Pts',(-5.0669640988664,-24.0387979403268,
12.));
#193934=CARTESIAN_POINT('Ctrl Pts',(-5.08081787581271,-24.0583376315636,
0.));
#193935=CARTESIAN_POINT('Ctrl Pts',(-5.08081787581271,-24.0583376315636,
12.));
#193936=CARTESIAN_POINT('Ctrl Pts',(-5.09476976342618,-24.0779139079264,
0.));
#193937=CARTESIAN_POINT('Ctrl Pts',(-5.09476976342618,-24.0779139079264,
12.));
#193938=CARTESIAN_POINT('Ctrl Pts',(-5.10881967883126,-24.0975261288444,
0.));
#193939=CARTESIAN_POINT('Ctrl Pts',(-5.10881967883126,-24.0975261288444,
12.));
#193940=CARTESIAN_POINT('Ctrl Pts',(-5.12296753853858,-24.117173659394,
0.));
#193941=CARTESIAN_POINT('Ctrl Pts',(-5.12296753853858,-24.117173659394,
12.));
#193942=CARTESIAN_POINT('Ctrl Pts',(-5.13721325845746,-24.1368558702443,
0.));
#193943=CARTESIAN_POINT('Ctrl Pts',(-5.13721325845746,-24.1368558702443,
12.));
#193944=CARTESIAN_POINT('Ctrl Pts',(-5.1515567539008,-24.1565721375971,
0.));
#193945=CARTESIAN_POINT('Ctrl Pts',(-5.1515567539008,-24.1565721375971,
12.));
#193946=CARTESIAN_POINT('Ctrl Pts',(-5.16599793957987,-24.1763218431344,
0.));
#193947=CARTESIAN_POINT('Ctrl Pts',(-5.16599793957987,-24.1763218431344,
12.));
#193948=CARTESIAN_POINT('Ctrl Pts',(-5.180536729614,-24.1961043738756,0.));
#193949=CARTESIAN_POINT('Ctrl Pts',(-5.180536729614,-24.1961043738756,12.));
#193950=CARTESIAN_POINT('Ctrl Pts',(-5.19517303753648,-24.2159191220171,
0.));
#193951=CARTESIAN_POINT('Ctrl Pts',(-5.19517303753648,-24.2159191220171,
12.));
#193952=CARTESIAN_POINT('Ctrl Pts',(-5.20990677629177,-24.2357654847766,
0.));
#193953=CARTESIAN_POINT('Ctrl Pts',(-5.20990677629177,-24.2357654847766,
12.));
#193954=CARTESIAN_POINT('Ctrl Pts',(-5.22473785822443,-24.2556428642294,
0.));
#193955=CARTESIAN_POINT('Ctrl Pts',(-5.22473785822443,-24.2556428642294,
12.));
#193956=CARTESIAN_POINT('Ctrl Pts',(-5.2396661950629,-24.2755506671525,
0.));
#193957=CARTESIAN_POINT('Ctrl Pts',(-5.2396661950629,-24.2755506671525,
12.));
#193958=CARTESIAN_POINT('Ctrl Pts',(-5.25469169788857,-24.2954883048447,
0.));
#193959=CARTESIAN_POINT('Ctrl Pts',(-5.25469169788857,-24.2954883048447,
12.));
#193960=CARTESIAN_POINT('Ctrl Pts',(-5.269814277188,-24.3154551932221,0.));
#193961=CARTESIAN_POINT('Ctrl Pts',(-5.269814277188,-24.3154551932221,12.));
#193962=CARTESIAN_POINT('Ctrl Pts',(-5.28503384290649,-24.3354507529414,
0.));
#193963=CARTESIAN_POINT('Ctrl Pts',(-5.28503384290649,-24.3354507529414,
12.));
#193964=CARTESIAN_POINT('Ctrl Pts',(-5.30035030449064,-24.3554744095075,
0.));
#193965=CARTESIAN_POINT('Ctrl Pts',(-5.30035030449064,-24.3554744095075,
12.));
#193966=CARTESIAN_POINT('Ctrl Pts',(-5.31576357092527,-24.3755255933917,
0.));
#193967=CARTESIAN_POINT('Ctrl Pts',(-5.31576357092527,-24.3755255933917,
12.));
#193968=CARTESIAN_POINT('Ctrl Pts',(-5.33127355076035,-24.3956037401293,
0.));
#193969=CARTESIAN_POINT('Ctrl Pts',(-5.33127355076035,-24.3956037401293,
12.));
#193970=CARTESIAN_POINT('Ctrl Pts',(-5.34688015213538,-24.4157082904614,
0.));
#193971=CARTESIAN_POINT('Ctrl Pts',(-5.34688015213538,-24.4157082904614,
12.));
#193972=CARTESIAN_POINT('Ctrl Pts',(-5.36258328273628,-24.435838689915,
0.));
#193973=CARTESIAN_POINT('Ctrl Pts',(-5.36258328273628,-24.435838689915,
12.));
#193974=CARTESIAN_POINT('Ctrl Pts',(-5.37838284973696,-24.4559943883157,
0.));
#193975=CARTESIAN_POINT('Ctrl Pts',(-5.37838284973696,-24.4559943883157,
12.));
#193976=CARTESIAN_POINT('Ctrl Pts',(-5.39427875973825,-24.4761748393321,
0.));
#193977=CARTESIAN_POINT('Ctrl Pts',(-5.39427875973825,-24.4761748393321,
12.));
#193978=CARTESIAN_POINT('Ctrl Pts',(-5.41027091869242,-24.496379499983,
0.));
#193979=CARTESIAN_POINT('Ctrl Pts',(-5.41027091869242,-24.496379499983,
12.));
#193980=CARTESIAN_POINT('Ctrl Pts',(-5.4263592318342,-24.5166078302108,
0.));
#193981=CARTESIAN_POINT('Ctrl Pts',(-5.4263592318342,-24.5166078302108,
12.));
#193982=CARTESIAN_POINT('Ctrl Pts',(-5.44254360356881,-24.5368592922863,
0.));
#193983=CARTESIAN_POINT('Ctrl Pts',(-5.44254360356881,-24.5368592922863,
12.));
#193984=CARTESIAN_POINT('Ctrl Pts',(-5.45882393762262,-24.5571333514842,
0.));
#193985=CARTESIAN_POINT('Ctrl Pts',(-5.45882393762262,-24.5571333514842,
12.));
#193986=CARTESIAN_POINT('Ctrl Pts',(-5.4752001372442,-24.5774294770329,
0.));
#193987=CARTESIAN_POINT('Ctrl Pts',(-5.4752001372442,-24.5774294770329,
12.));
#193988=CARTESIAN_POINT('Ctrl Pts',(-5.49167210537248,-24.5977471429364,
0.));
#193989=CARTESIAN_POINT('Ctrl Pts',(-5.49167210537248,-24.5977471429364,
12.));
#193990=CARTESIAN_POINT('Ctrl Pts',(-5.50823974481963,-24.6180858289179,
0.));
#193991=CARTESIAN_POINT('Ctrl Pts',(-5.50823974481963,-24.6180858289179,
12.));
#193992=CARTESIAN_POINT('Ctrl Pts',(-5.52490295840993,-24.6384450211467,
0.));
#193993=CARTESIAN_POINT('Ctrl Pts',(-5.52490295840993,-24.6384450211467,
12.));
#193994=CARTESIAN_POINT('Ctrl Pts',(-5.54166164919584,-24.6588242134738,
0.));
#193995=CARTESIAN_POINT('Ctrl Pts',(-5.54166164919584,-24.6588242134738,
12.));
#193996=CARTESIAN_POINT('Ctrl Pts',(-5.55851572025377,-24.6792229061794,
0.));
#193997=CARTESIAN_POINT('Ctrl Pts',(-5.55851572025377,-24.6792229061794,
12.));
#193998=CARTESIAN_POINT('Ctrl Pts',(-5.57546507427756,-24.6996406035517,
0.));
#193999=CARTESIAN_POINT('Ctrl Pts',(-5.57546507427756,-24.6996406035517,
12.));
#194000=CARTESIAN_POINT('Ctrl Pts',(-5.59250961323988,-24.7200768119088,
0.));
#194001=CARTESIAN_POINT('Ctrl Pts',(-5.59250961323988,-24.7200768119088,
12.));
#194002=CARTESIAN_POINT('Ctrl Pts',(-5.60964923798492,-24.7405310372739,
0.));
#194003=CARTESIAN_POINT('Ctrl Pts',(-5.60964923798492,-24.7405310372739,
12.));
#194004=CARTESIAN_POINT('Ctrl Pts',(-5.62688384790924,-24.7610027835697,
0.));
#194005=CARTESIAN_POINT('Ctrl Pts',(-5.62688384790924,-24.7610027835697,
12.));
#194006=CARTESIAN_POINT('Ctrl Pts',(-5.64421334042262,-24.781491549672,
0.));
#194007=CARTESIAN_POINT('Ctrl Pts',(-5.64421334042262,-24.781491549672,
12.));
#194008=CARTESIAN_POINT('Ctrl Pts',(-5.66163761114922,-24.8019968304605,
0.));
#194009=CARTESIAN_POINT('Ctrl Pts',(-5.66163761114922,-24.8019968304605,
12.));
#194010=CARTESIAN_POINT('Ctrl Pts',(-5.67915655496543,-24.8225181223845,
0.));
#194011=CARTESIAN_POINT('Ctrl Pts',(-5.67915655496543,-24.8225181223845,
12.));
#194012=CARTESIAN_POINT('Ctrl Pts',(-5.69677006679445,-24.8430549277621,
0.));
#194013=CARTESIAN_POINT('Ctrl Pts',(-5.69677006679445,-24.8430549277621,
12.));
#194014=CARTESIAN_POINT('Ctrl Pts',(-5.71447804252028,-24.8636067597669,
0.));
#194015=CARTESIAN_POINT('Ctrl Pts',(-5.71447804252028,-24.8636067597669,
12.));
#194016=CARTESIAN_POINT('Ctrl Pts',(-5.73228037976928,-24.884173146722,
0.));
#194017=CARTESIAN_POINT('Ctrl Pts',(-5.73228037976928,-24.884173146722,
12.));
#194018=CARTESIAN_POINT('Ctrl Pts',(-5.75017697890805,-24.904753637648,
0.));
#194019=CARTESIAN_POINT('Ctrl Pts',(-5.75017697890805,-24.904753637648,
12.));
#194020=CARTESIAN_POINT('Ctrl Pts',(-5.76816774342221,-24.9253478043656,
0.));
#194021=CARTESIAN_POINT('Ctrl Pts',(-5.76816774342221,-24.9253478043656,
12.));
#194022=CARTESIAN_POINT('Ctrl Pts',(-5.78625257775682,-24.945955229334,
0.));
#194023=CARTESIAN_POINT('Ctrl Pts',(-5.78625257775682,-24.945955229334,
12.));
#194024=CARTESIAN_POINT('Ctrl Pts',(-5.80443138549727,-24.9665754954496,
0.));
#194025=CARTESIAN_POINT('Ctrl Pts',(-5.80443138549727,-24.9665754954496,
12.));
#194026=CARTESIAN_POINT('Ctrl Pts',(-5.822704067442,-24.9872081752734,0.));
#194027=CARTESIAN_POINT('Ctrl Pts',(-5.822704067442,-24.9872081752734,12.));
#194028=CARTESIAN_POINT('Ctrl Pts',(-5.84107051963072,-25.0078528200564,
0.));
#194029=CARTESIAN_POINT('Ctrl Pts',(-5.84107051963072,-25.0078528200564,
12.));
#194030=CARTESIAN_POINT('Ctrl Pts',(-5.85953063156827,-25.0285089498899,
0.));
#194031=CARTESIAN_POINT('Ctrl Pts',(-5.85953063156827,-25.0285089498899,
12.));
#194032=CARTESIAN_POINT('Ctrl Pts',(-5.87808428385367,-25.049176040591,
0.));
#194033=CARTESIAN_POINT('Ctrl Pts',(-5.87808428385367,-25.049176040591,
12.));
#194034=CARTESIAN_POINT('Ctrl Pts',(-5.89673135155515,-25.0698535426514,
0.));
#194035=CARTESIAN_POINT('Ctrl Pts',(-5.89673135155515,-25.0698535426514,
12.));
#194036=CARTESIAN_POINT('Ctrl Pts',(-5.91547170844448,-25.0905409050773,
0.));
#194037=CARTESIAN_POINT('Ctrl Pts',(-5.91547170844448,-25.0905409050773,
12.));
#194038=CARTESIAN_POINT('Ctrl Pts',(-5.93430523086836,-25.1112375971106,
0.));
#194039=CARTESIAN_POINT('Ctrl Pts',(-5.93430523086836,-25.1112375971106,
12.));
#194040=CARTESIAN_POINT('Ctrl Pts',(-5.95323180187379,-25.1319431317237,
0.));
#194041=CARTESIAN_POINT('Ctrl Pts',(-5.95323180187379,-25.1319431317237,
12.));
#194042=CARTESIAN_POINT('Ctrl Pts',(-5.97225131495618,-25.1526570863092,
0.));
#194043=CARTESIAN_POINT('Ctrl Pts',(-5.97225131495618,-25.1526570863092,
12.));
#194044=CARTESIAN_POINT('Ctrl Pts',(-5.99136367859755,-25.1733791296259,
0.));
#194045=CARTESIAN_POINT('Ctrl Pts',(-5.99136367859755,-25.1733791296259,
12.));
#194046=CARTESIAN_POINT('Ctrl Pts',(-6.01056881804614,-25.1941090269819,
0.));
#194047=CARTESIAN_POINT('Ctrl Pts',(-6.01056881804614,-25.1941090269819,
12.));
#194048=CARTESIAN_POINT('Ctrl Pts',(-6.02986667389998,-25.21484662016,0.));
#194049=CARTESIAN_POINT('Ctrl Pts',(-6.02986667389998,-25.21484662016,12.));
#194050=CARTESIAN_POINT('Ctrl Pts',(-6.04925720151219,-25.2355918139032,
0.));
#194051=CARTESIAN_POINT('Ctrl Pts',(-6.04925720151219,-25.2355918139032,
12.));
#194052=CARTESIAN_POINT('Ctrl Pts',(-6.06484373634547,-25.2521940105705,
0.));
#194053=CARTESIAN_POINT('Ctrl Pts',(-6.06484373634547,-25.2521940105705,
12.));
#194054=CARTESIAN_POINT('Ctrl Pts',(-6.07657531787491,-25.2646490489922,
0.));
#194055=CARTESIAN_POINT('Ctrl Pts',(-6.07657531787491,-25.2646490489922,
12.));
#194056=CARTESIAN_POINT('Ctrl Pts',(-6.08441489609794,-25.2729539149517,
0.));
#194057=CARTESIAN_POINT('Ctrl Pts',(-6.08441489609794,-25.2729539149517,
12.));
#194058=CARTESIAN_POINT('Ctrl Pts',(-6.088339316177,-25.2771067246846,0.));
#194059=CARTESIAN_POINT('Ctrl Pts',(-6.088339316177,-25.2771067246846,12.));
#194060=CARTESIAN_POINT('',(-6.088339316177,-25.2771067246846,0.));
#194061=CARTESIAN_POINT('Ctrl Pts',(-4.11585220600463,-22.1738711152697,
0.));
#194062=CARTESIAN_POINT('Ctrl Pts',(-4.11585194677443,-22.173877682324,
0.));
#194063=CARTESIAN_POINT('Ctrl Pts',(-4.11586035878288,-22.1739341411687,
0.));
#194064=CARTESIAN_POINT('Ctrl Pts',(-4.11589976826167,-22.1741488021234,
0.));
#194065=CARTESIAN_POINT('Ctrl Pts',(-4.11600589882846,-22.1746949858775,
0.));
#194066=CARTESIAN_POINT('Ctrl Pts',(-4.11622797217069,-22.1758088296598,
0.));
#194067=CARTESIAN_POINT('Ctrl Pts',(-4.11653973150519,-22.177347426894,
0.));
#194068=CARTESIAN_POINT('Ctrl Pts',(-4.11694173195005,-22.179297473024,
0.));
#194069=CARTESIAN_POINT('Ctrl Pts',(-4.11743469691757,-22.1816414985788,
0.));
#194070=CARTESIAN_POINT('Ctrl Pts',(-4.11801938107481,-22.1843613164855,
0.));
#194071=CARTESIAN_POINT('Ctrl Pts',(-4.11869641271774,-22.1874419861496,
0.));
#194072=CARTESIAN_POINT('Ctrl Pts',(-4.11946626228637,-22.1908725908525,
0.));
#194073=CARTESIAN_POINT('Ctrl Pts',(-4.12032932637737,-22.1946440958098,
0.));
#194074=CARTESIAN_POINT('Ctrl Pts',(-4.12128598183523,-22.1987479618246,
0.));
#194075=CARTESIAN_POINT('Ctrl Pts',(-4.12233664408228,-22.2031746532106,
0.));
#194076=CARTESIAN_POINT('Ctrl Pts',(-4.12348173702024,-22.2079143941719,
0.));
#194077=CARTESIAN_POINT('Ctrl Pts',(-4.12472167516608,-22.2129576146671,
0.));
#194078=CARTESIAN_POINT('Ctrl Pts',(-4.12605683613308,-22.2182956401341,
0.));
#194079=CARTESIAN_POINT('Ctrl Pts',(-4.12748755830105,-22.2239207458781,
0.));
#194080=CARTESIAN_POINT('Ctrl Pts',(-4.1290141546338,-22.2298258043947,
0.));
#194081=CARTESIAN_POINT('Ctrl Pts',(-4.13063692157499,-22.2360040565533,
0.));
#194082=CARTESIAN_POINT('Ctrl Pts',(-4.13235615060161,-22.2424488153523,
0.));
#194083=CARTESIAN_POINT('Ctrl Pts',(-4.13417212558811,-22.249153531779,
0.));
#194084=CARTESIAN_POINT('Ctrl Pts',(-4.13608511977226,-22.2561118708421,
0.));
#194085=CARTESIAN_POINT('Ctrl Pts',(-4.13809539255423,-22.2633177913972,
0.));
#194086=CARTESIAN_POINT('Ctrl Pts',(-4.14020318715992,-22.2707656042457,
0.));
#194087=CARTESIAN_POINT('Ctrl Pts',(-4.14240873321985,-22.2784499072027,
0.));
#194088=CARTESIAN_POINT('Ctrl Pts',(-4.14471224859296,-22.2863655389166,
0.));
#194089=CARTESIAN_POINT('Ctrl Pts',(-4.14711394168557,-22.2945075198467,
0.));
#194090=CARTESIAN_POINT('Ctrl Pts',(-4.14961401285523,-22.3028710166933,
0.));
#194091=CARTESIAN_POINT('Ctrl Pts',(-4.15221265396991,-22.3114513545185,
0.));
#194092=CARTESIAN_POINT('Ctrl Pts',(-4.15491004835282,-22.320244018698,
0.));
#194093=CARTESIAN_POINT('Ctrl Pts',(-4.15770637047891,-22.3292446628959,
0.));
#194094=CARTESIAN_POINT('Ctrl Pts',(-4.16060178604165,-22.3384491078602,
0.));
#194095=CARTESIAN_POINT('Ctrl Pts',(-4.16359645263189,-22.3478533253889,
0.));
#194096=CARTESIAN_POINT('Ctrl Pts',(-4.16669052026601,-22.3574534257396,
0.));
#194097=CARTESIAN_POINT('Ctrl Pts',(-4.16988413199458,-22.36724564276,0.));
#194098=CARTESIAN_POINT('Ctrl Pts',(-4.17317742436146,-22.3772263228617,
0.));
#194099=CARTESIAN_POINT('Ctrl Pts',(-4.17657052752826,-22.3873919231334,
0.));
#194100=CARTESIAN_POINT('Ctrl Pts',(-4.18006356544883,-22.3977390078075,
0.));
#194101=CARTESIAN_POINT('Ctrl Pts',(-4.18365665600851,-22.4082642454453,
0.));
#194102=CARTESIAN_POINT('Ctrl Pts',(-4.18734991117722,-22.4189644056115,
0.));
#194103=CARTESIAN_POINT('Ctrl Pts',(-4.19114343726943,-22.4298363535421,
0.));
#194104=CARTESIAN_POINT('Ctrl Pts',(-4.19503733518862,-22.4408770448917,
0.));
#194105=CARTESIAN_POINT('Ctrl Pts',(-4.19903170066356,-22.4520835205419,
0.));
#194106=CARTESIAN_POINT('Ctrl Pts',(-4.20312662448172,-22.4634529011433,
0.));
#194107=CARTESIAN_POINT('Ctrl Pts',(-4.20732219265649,-22.4749823839915,
0.));
#194108=CARTESIAN_POINT('Ctrl Pts',(-4.21161848657429,-22.4866692403147,
0.));
#194109=CARTESIAN_POINT('Ctrl Pts',(-4.21601558313909,-22.4985108124229,
0.));
#194110=CARTESIAN_POINT('Ctrl Pts',(-4.22051355490198,-22.5105045108882,
0.));
#194111=CARTESIAN_POINT('Ctrl Pts',(-4.22511247020041,-22.5226478117885,
0.));
#194112=CARTESIAN_POINT('Ctrl Pts',(-4.22981239330732,-22.5349382540587,
0.));
#194113=CARTESIAN_POINT('Ctrl Pts',(-4.23461338456714,-22.5473734368086,
0.));
#194114=CARTESIAN_POINT('Ctrl Pts',(-4.23951550052527,-22.559951016643,
0.));
#194115=CARTESIAN_POINT('Ctrl Pts',(-4.2445187940486,-22.5726687049922,
0.));
#194116=CARTESIAN_POINT('Ctrl Pts',(-4.24962331444186,-22.5855242662479,
0.));
#194117=CARTESIAN_POINT('Ctrl Pts',(-4.25482910755486,-22.5985155158637,
0.));
#194118=CARTESIAN_POINT('Ctrl Pts',(-4.26013621588304,-22.611640318482,
0.));
#194119=CARTESIAN_POINT('Ctrl Pts',(-4.26554467865572,-22.6248965859975,
0.));
#194120=CARTESIAN_POINT('Ctrl Pts',(-4.27105453193,-22.6382822758171,0.));
#194121=CARTESIAN_POINT('Ctrl Pts',(-4.27666580869118,-22.6517953893303,
0.));
#194122=CARTESIAN_POINT('Ctrl Pts',(-4.2823785389406,-22.665433970311,0.));
#194123=CARTESIAN_POINT('Ctrl Pts',(-4.28819274977767,-22.6791961033536,
0.));
#194124=CARTESIAN_POINT('Ctrl Pts',(-4.29410846547062,-22.6930799122545,
0.));
#194125=CARTESIAN_POINT('Ctrl Pts',(-4.30012570754067,-22.707083558756,
0.));
#194126=CARTESIAN_POINT('Ctrl Pts',(-4.30624449484075,-22.7212052413384,
0.));
#194127=CARTESIAN_POINT('Ctrl Pts',(-4.31246484362551,-22.7354431939926,
0.));
#194128=CARTESIAN_POINT('Ctrl Pts',(-4.31878676761231,-22.7497956849852,
0.));
#194129=CARTESIAN_POINT('Ctrl Pts',(-4.32521027803748,-22.764261015648,
0.));
#194130=CARTESIAN_POINT('Ctrl Pts',(-4.33173538373183,-22.7788375194081,
0.));
#194131=CARTESIAN_POINT('Ctrl Pts',(-4.33836209118444,-22.7935235607807,
0.));
#194132=CARTESIAN_POINT('Ctrl Pts',(-4.34509040460066,-22.808317534379,
0.));
#194133=CARTESIAN_POINT('Ctrl Pts',(-4.35192032594802,-22.8232178638873,
0.));
#194134=CARTESIAN_POINT('Ctrl Pts',(-4.3588518550056,-22.838223001118,0.));
#194135=CARTESIAN_POINT('Ctrl Pts',(-4.36588498943011,-22.8533314252419,
0.));
#194136=CARTESIAN_POINT('Ctrl Pts',(-4.37301972480753,-22.8685416419725,
0.));
#194137=CARTESIAN_POINT('Ctrl Pts',(-4.38025605470091,-22.8838521827702,
0.));
#194138=CARTESIAN_POINT('Ctrl Pts',(-4.38759397068393,-22.8992616040108,
0.));
#194139=CARTESIAN_POINT('Ctrl Pts',(-4.39503346238455,-22.9147684862425,
0.));
#194140=CARTESIAN_POINT('Ctrl Pts',(-4.40257451754308,-22.9303714335549,
0.));
#194141=CARTESIAN_POINT('Ctrl Pts',(-4.41021712205549,-22.9460690729093,
0.));
#194142=CARTESIAN_POINT('Ctrl Pts',(-4.41796126001311,-22.9618600534866,
0.));
#194143=CARTESIAN_POINT('Ctrl Pts',(-4.42580691372772,-22.9777430460021,
0.));
#194144=CARTESIAN_POINT('Ctrl Pts',(-4.43375406376906,-22.9937167421009,
0.));
#194145=CARTESIAN_POINT('Ctrl Pts',(-4.44180268901667,-23.0097798538399,
0.));
#194146=CARTESIAN_POINT('Ctrl Pts',(-4.44995276669699,-23.0259311131395,
0.));
#194147=CARTESIAN_POINT('Ctrl Pts',(-4.45820427241677,-23.0421692712466,
0.));
#194148=CARTESIAN_POINT('Ctrl Pts',(-4.46655718018206,-23.0584930981723,
0.));
#194149=CARTESIAN_POINT('Ctrl Pts',(-4.47501146242822,-23.0749013821867,
0.));
#194150=CARTESIAN_POINT('Ctrl Pts',(-4.48356709006757,-23.0913929293909,
0.));
#194151=CARTESIAN_POINT('Ctrl Pts',(-4.49222403252202,-23.1079665632629,
0.));
#194152=CARTESIAN_POINT('Ctrl Pts',(-4.50098225775179,-23.1246211242117,
0.));
#194153=CARTESIAN_POINT('Ctrl Pts',(-4.50984173227088,-23.1413554691136,
0.));
#194154=CARTESIAN_POINT('Ctrl Pts',(-4.51880242116786,-23.1581684708778,
0.));
#194155=CARTESIAN_POINT('Ctrl Pts',(-4.52786428815049,-23.1750590180923,
0.));
#194156=CARTESIAN_POINT('Ctrl Pts',(-4.53702729557586,-23.1920260146474,
0.));
#194157=CARTESIAN_POINT('Ctrl Pts',(-4.54629140447543,-23.2090683793627,
0.));
#194158=CARTESIAN_POINT('Ctrl Pts',(-4.55565657456957,-23.2261850456055,
0.));
#194159=CARTESIAN_POINT('Ctrl Pts',(-4.56512276427812,-23.2433749609117,
0.));
#194160=CARTESIAN_POINT('Ctrl Pts',(-4.57468993076071,-23.2606370866854,
0.));
#194161=CARTESIAN_POINT('Ctrl Pts',(-4.58435802994675,-23.2779703978868,
0.));
#194162=CARTESIAN_POINT('Ctrl Pts',(-4.5941270165575,-23.295373882719,0.));
#194163=CARTESIAN_POINT('Ctrl Pts',(-4.60399684412176,-23.3128465423119,
0.));
#194164=CARTESIAN_POINT('Ctrl Pts',(-4.61396746497849,-23.3303873903947,
0.));
#194165=CARTESIAN_POINT('Ctrl Pts',(-4.62403883030825,-23.3479954530281,
0.));
#194166=CARTESIAN_POINT('Ctrl Pts',(-4.63421089016555,-23.3656697683496,
0.));
#194167=CARTESIAN_POINT('Ctrl Pts',(-4.64448359349936,-23.383409386307,
0.));
#194168=CARTESIAN_POINT('Ctrl Pts',(-4.65485688816923,-23.4012133683957,
0.));
#194169=CARTESIAN_POINT('Ctrl Pts',(-4.66533072094664,-23.4190807873798,
0.));
#194170=CARTESIAN_POINT('Ctrl Pts',(-4.67590503753051,-23.4370107270444,
0.));
#194171=CARTESIAN_POINT('Ctrl Pts',(-4.68657978258298,-23.4550022819852,
0.));
#194172=CARTESIAN_POINT('Ctrl Pts',(-4.69735489975024,-23.4730545573849,
0.));
#194173=CARTESIAN_POINT('Ctrl Pts',(-4.70823033167821,-23.491166668789,
0.));
#194174=CARTESIAN_POINT('Ctrl Pts',(-4.71920602001905,-23.5093377418784,
0.));
#194175=CARTESIAN_POINT('Ctrl Pts',(-4.73028190543032,-23.5275669122378,
0.));
#194176=CARTESIAN_POINT('Ctrl Pts',(-4.74145792760699,-23.5458533251715,
0.));
#194177=CARTESIAN_POINT('Ctrl Pts',(-4.75273402530616,-23.564196135517,
0.));
#194178=CARTESIAN_POINT('Ctrl Pts',(-4.76411013636252,-23.5825945074535,
0.));
#194179=CARTESIAN_POINT('Ctrl Pts',(-4.77558619769876,-23.6010476143099,
0.));
#194180=CARTESIAN_POINT('Ctrl Pts',(-4.78716214532105,-23.6195546383625,
0.));
#194181=CARTESIAN_POINT('Ctrl Pts',(-4.79883791433231,-23.6381147706581,
0.));
#194182=CARTESIAN_POINT('Ctrl Pts',(-4.81061343896443,-23.6567272108631,
0.));
#194183=CARTESIAN_POINT('Ctrl Pts',(-4.82248865259571,-23.6753911671023,
0.));
#194184=CARTESIAN_POINT('Ctrl Pts',(-4.83446348776268,-23.6941058557971,
0.));
#194185=CARTESIAN_POINT('Ctrl Pts',(-4.84653787616424,-23.7128705015014,
0.));
#194186=CARTESIAN_POINT('Ctrl Pts',(-4.85871174865492,-23.7316843367308,
0.));
#194187=CARTESIAN_POINT('Ctrl Pts',(-4.87098503527144,-23.7505466018239,
0.));
#194188=CARTESIAN_POINT('Ctrl Pts',(-4.88335766525566,-23.7694565448044,
0.));
#194189=CARTESIAN_POINT('Ctrl Pts',(-4.89582956706772,-23.7884134212381,
0.));
#194190=CARTESIAN_POINT('Ctrl Pts',(-4.90840066839348,-23.8074164940897,
0.));
#194191=CARTESIAN_POINT('Ctrl Pts',(-4.92107089613977,-23.8264650335721,
0.));
#194192=CARTESIAN_POINT('Ctrl Pts',(-4.93384017643442,-23.8455583170062,
0.));
#194193=CARTESIAN_POINT('Ctrl Pts',(-4.94670843465869,-23.8646956287172,
0.));
#194194=CARTESIAN_POINT('Ctrl Pts',(-4.95967559546566,-23.883876259922,
0.));
#194195=CARTESIAN_POINT('Ctrl Pts',(-4.9727415827923,-23.9030995086164,
0.));
#194196=CARTESIAN_POINT('Ctrl Pts',(-4.98590631986534,-23.9223646794591,
0.));
#194197=CARTESIAN_POINT('Ctrl Pts',(-4.9991697291931,-23.9416710836529,
0.));
#194198=CARTESIAN_POINT('Ctrl Pts',(-5.01253173257459,-23.9610180388271,
0.));
#194199=CARTESIAN_POINT('Ctrl Pts',(-5.02599225112462,-23.9804048689228,
0.));
#194200=CARTESIAN_POINT('Ctrl Pts',(-5.03955120528528,-23.9998309040747,
0.));
#194201=CARTESIAN_POINT('Ctrl Pts',(-5.05320851483069,-24.0192954804896,
0.));
#194202=CARTESIAN_POINT('Ctrl Pts',(-5.0669640988664,-24.0387979403268,
0.));
#194203=CARTESIAN_POINT('Ctrl Pts',(-5.08081787581271,-24.0583376315636,
0.));
#194204=CARTESIAN_POINT('Ctrl Pts',(-5.09476976342618,-24.0779139079264,
0.));
#194205=CARTESIAN_POINT('Ctrl Pts',(-5.10881967883126,-24.0975261288444,
0.));
#194206=CARTESIAN_POINT('Ctrl Pts',(-5.12296753853858,-24.117173659394,
0.));
#194207=CARTESIAN_POINT('Ctrl Pts',(-5.13721325845746,-24.1368558702443,
0.));
#194208=CARTESIAN_POINT('Ctrl Pts',(-5.1515567539008,-24.1565721375971,
0.));
#194209=CARTESIAN_POINT('Ctrl Pts',(-5.16599793957987,-24.1763218431344,
0.));
#194210=CARTESIAN_POINT('Ctrl Pts',(-5.180536729614,-24.1961043738756,0.));
#194211=CARTESIAN_POINT('Ctrl Pts',(-5.19517303753648,-24.2159191220171,
0.));
#194212=CARTESIAN_POINT('Ctrl Pts',(-5.20990677629177,-24.2357654847766,
0.));
#194213=CARTESIAN_POINT('Ctrl Pts',(-5.22473785822443,-24.2556428642294,
0.));
#194214=CARTESIAN_POINT('Ctrl Pts',(-5.2396661950629,-24.2755506671525,
0.));
#194215=CARTESIAN_POINT('Ctrl Pts',(-5.25469169788857,-24.2954883048447,
0.));
#194216=CARTESIAN_POINT('Ctrl Pts',(-5.269814277188,-24.3154551932221,0.));
#194217=CARTESIAN_POINT('Ctrl Pts',(-5.28503384290649,-24.3354507529414,
0.));
#194218=CARTESIAN_POINT('Ctrl Pts',(-5.30035030449064,-24.3554744095075,
0.));
#194219=CARTESIAN_POINT('Ctrl Pts',(-5.31576357092527,-24.3755255933917,
0.));
#194220=CARTESIAN_POINT('Ctrl Pts',(-5.33127355076035,-24.3956037401293,
0.));
#194221=CARTESIAN_POINT('Ctrl Pts',(-5.34688015213538,-24.4157082904614,
0.));
#194222=CARTESIAN_POINT('Ctrl Pts',(-5.36258328273628,-24.435838689915,
0.));
#194223=CARTESIAN_POINT('Ctrl Pts',(-5.37838284973696,-24.4559943883157,
0.));
#194224=CARTESIAN_POINT('Ctrl Pts',(-5.39427875973825,-24.4761748393321,
0.));
#194225=CARTESIAN_POINT('Ctrl Pts',(-5.41027091869242,-24.496379499983,
0.));
#194226=CARTESIAN_POINT('Ctrl Pts',(-5.4263592318342,-24.5166078302108,
0.));
#194227=CARTESIAN_POINT('Ctrl Pts',(-5.44254360356881,-24.5368592922863,
0.));
#194228=CARTESIAN_POINT('Ctrl Pts',(-5.45882393762262,-24.5571333514842,
0.));
#194229=CARTESIAN_POINT('Ctrl Pts',(-5.4752001372442,-24.5774294770329,
0.));
#194230=CARTESIAN_POINT('Ctrl Pts',(-5.49167210537248,-24.5977471429364,
0.));
#194231=CARTESIAN_POINT('Ctrl Pts',(-5.50823974481963,-24.6180858289179,
0.));
#194232=CARTESIAN_POINT('Ctrl Pts',(-5.52490295840993,-24.6384450211467,
0.));
#194233=CARTESIAN_POINT('Ctrl Pts',(-5.54166164919584,-24.6588242134738,
0.));
#194234=CARTESIAN_POINT('Ctrl Pts',(-5.55851572025377,-24.6792229061794,
0.));
#194235=CARTESIAN_POINT('Ctrl Pts',(-5.57546507427756,-24.6996406035517,
0.));
#194236=CARTESIAN_POINT('Ctrl Pts',(-5.59250961323988,-24.7200768119088,
0.));
#194237=CARTESIAN_POINT('Ctrl Pts',(-5.60964923798492,-24.7405310372739,
0.));
#194238=CARTESIAN_POINT('Ctrl Pts',(-5.62688384790924,-24.7610027835697,
0.));
#194239=CARTESIAN_POINT('Ctrl Pts',(-5.64421334042262,-24.781491549672,
0.));
#194240=CARTESIAN_POINT('Ctrl Pts',(-5.66163761114922,-24.8019968304605,
0.));
#194241=CARTESIAN_POINT('Ctrl Pts',(-5.67915655496543,-24.8225181223845,
0.));
#194242=CARTESIAN_POINT('Ctrl Pts',(-5.69677006679445,-24.8430549277621,
0.));
#194243=CARTESIAN_POINT('Ctrl Pts',(-5.71447804252028,-24.8636067597669,
0.));
#194244=CARTESIAN_POINT('Ctrl Pts',(-5.73228037976928,-24.884173146722,
0.));
#194245=CARTESIAN_POINT('Ctrl Pts',(-5.75017697890805,-24.904753637648,
0.));
#194246=CARTESIAN_POINT('Ctrl Pts',(-5.76816774342221,-24.9253478043656,
0.));
#194247=CARTESIAN_POINT('Ctrl Pts',(-5.78625257775682,-24.945955229334,
0.));
#194248=CARTESIAN_POINT('Ctrl Pts',(-5.80443138549727,-24.9665754954496,
0.));
#194249=CARTESIAN_POINT('Ctrl Pts',(-5.822704067442,-24.9872081752734,0.));
#194250=CARTESIAN_POINT('Ctrl Pts',(-5.84107051963072,-25.0078528200564,
0.));
#194251=CARTESIAN_POINT('Ctrl Pts',(-5.85953063156827,-25.0285089498899,
0.));
#194252=CARTESIAN_POINT('Ctrl Pts',(-5.87808428385367,-25.049176040591,
0.));
#194253=CARTESIAN_POINT('Ctrl Pts',(-5.89673135155515,-25.0698535426514,
0.));
#194254=CARTESIAN_POINT('Ctrl Pts',(-5.91547170844448,-25.0905409050773,
0.));
#194255=CARTESIAN_POINT('Ctrl Pts',(-5.93430523086836,-25.1112375971106,
0.));
#194256=CARTESIAN_POINT('Ctrl Pts',(-5.95323180187379,-25.1319431317237,
0.));
#194257=CARTESIAN_POINT('Ctrl Pts',(-5.97225131495618,-25.1526570863092,
0.));
#194258=CARTESIAN_POINT('Ctrl Pts',(-5.99136367859755,-25.1733791296259,
0.));
#194259=CARTESIAN_POINT('Ctrl Pts',(-6.01056881804614,-25.1941090269819,
0.));
#194260=CARTESIAN_POINT('Ctrl Pts',(-6.02986667389998,-25.21484662016,0.));
#194261=CARTESIAN_POINT('Ctrl Pts',(-6.04925720151219,-25.2355918139032,
0.));
#194262=CARTESIAN_POINT('Ctrl Pts',(-6.06484373634547,-25.2521940105705,
0.));
#194263=CARTESIAN_POINT('Ctrl Pts',(-6.07657531787491,-25.2646490489922,
0.));
#194264=CARTESIAN_POINT('Ctrl Pts',(-6.08441489609794,-25.2729539149517,
0.));
#194265=CARTESIAN_POINT('Ctrl Pts',(-6.088339316177,-25.2771067246846,0.));
#194266=CARTESIAN_POINT('',(-6.088339316177,-25.2771067246846,0.));
#194267=CARTESIAN_POINT('Origin',(-9.26120677397565,-19.4030938020118,0.));
#194268=CARTESIAN_POINT('',(-9.71462809124917,-20.353053841303,0.));
#194269=CARTESIAN_POINT('',(-9.71462809124917,-20.353053841303,0.));
#194270=CARTESIAN_POINT('',(-4.63060338698782,-9.70154690100589,0.));
#194271=CARTESIAN_POINT('Ctrl Pts',(-7.36589684767345,-24.9347862158358,
0.));
#194272=CARTESIAN_POINT('Ctrl Pts',(-7.36589684767345,-24.9347862158358,
12.));
#194273=CARTESIAN_POINT('Ctrl Pts',(-7.36721909028843,-24.9292275670674,
0.));
#194274=CARTESIAN_POINT('Ctrl Pts',(-7.36721909028843,-24.9292275670674,
12.));
#194275=CARTESIAN_POINT('Ctrl Pts',(-7.36985593120091,-24.9181155530543,
0.));
#194276=CARTESIAN_POINT('Ctrl Pts',(-7.36985593120091,-24.9181155530543,
12.));
#194277=CARTESIAN_POINT('Ctrl Pts',(-7.37378825961676,-24.901463382605,
0.));
#194278=CARTESIAN_POINT('Ctrl Pts',(-7.37378825961676,-24.901463382605,
12.));
#194279=CARTESIAN_POINT('Ctrl Pts',(-7.3789854964027,-24.8792921911115,
0.));
#194280=CARTESIAN_POINT('Ctrl Pts',(-7.3789854964027,-24.8792921911115,
12.));
#194281=CARTESIAN_POINT('Ctrl Pts',(-7.38540558903621,-24.8516310625176,
0.));
#194282=CARTESIAN_POINT('Ctrl Pts',(-7.38540558903621,-24.8516310625176,
12.));
#194283=CARTESIAN_POINT('Ctrl Pts',(-7.39174922585809,-24.8240228520893,
0.));
#194284=CARTESIAN_POINT('Ctrl Pts',(-7.39174922585809,-24.8240228520893,
12.));
#194285=CARTESIAN_POINT('Ctrl Pts',(-7.39801641583013,-24.7964676646431,
0.));
#194286=CARTESIAN_POINT('Ctrl Pts',(-7.39801641583013,-24.7964676646431,
12.));
#194287=CARTESIAN_POINT('Ctrl Pts',(-7.40420718661603,-24.7689656668983,
0.));
#194288=CARTESIAN_POINT('Ctrl Pts',(-7.40420718661603,-24.7689656668983,
12.));
#194289=CARTESIAN_POINT('Ctrl Pts',(-7.41032159082382,-24.7415170994784,
0.));
#194290=CARTESIAN_POINT('Ctrl Pts',(-7.41032159082382,-24.7415170994784,
12.));
#194291=CARTESIAN_POINT('Ctrl Pts',(-7.41635971481674,-24.7141222950051,
0.));
#194292=CARTESIAN_POINT('Ctrl Pts',(-7.41635971481674,-24.7141222950051,
12.));
#194293=CARTESIAN_POINT('Ctrl Pts',(-7.42232167766266,-24.6867816727192,
0.));
#194294=CARTESIAN_POINT('Ctrl Pts',(-7.42232167766266,-24.6867816727192,
12.));
#194295=CARTESIAN_POINT('Ctrl Pts',(-7.42820762159126,-24.6594957128756,
0.));
#194296=CARTESIAN_POINT('Ctrl Pts',(-7.42820762159126,-24.6594957128756,
12.));
#194297=CARTESIAN_POINT('Ctrl Pts',(-7.43401770489524,-24.6322649369517,
0.));
#194298=CARTESIAN_POINT('Ctrl Pts',(-7.43401770489524,-24.6322649369517,
12.));
#194299=CARTESIAN_POINT('Ctrl Pts',(-7.43975209375504,-24.6050898852368,
0.));
#194300=CARTESIAN_POINT('Ctrl Pts',(-7.43975209375504,-24.6050898852368,
12.));
#194301=CARTESIAN_POINT('Ctrl Pts',(-7.44541095473135,-24.577971096086,
0.));
#194302=CARTESIAN_POINT('Ctrl Pts',(-7.44541095473135,-24.577971096086,
12.));
#194303=CARTESIAN_POINT('Ctrl Pts',(-7.4509944465116,-24.5509090831559,
0.));
#194304=CARTESIAN_POINT('Ctrl Pts',(-7.4509944465116,-24.5509090831559,
12.));
#194305=CARTESIAN_POINT('Ctrl Pts',(-7.45650271335862,-24.5239043173072,
0.));
#194306=CARTESIAN_POINT('Ctrl Pts',(-7.45650271335862,-24.5239043173072,
12.));
#194307=CARTESIAN_POINT('Ctrl Pts',(-7.46193588961464,-24.4969572391483,
0.));
#194308=CARTESIAN_POINT('Ctrl Pts',(-7.46193588961464,-24.4969572391483,
12.));
#194309=CARTESIAN_POINT('Ctrl Pts',(-7.46729410308787,-24.4700682684524,
0.));
#194310=CARTESIAN_POINT('Ctrl Pts',(-7.46729410308787,-24.4700682684524,
12.));
#194311=CARTESIAN_POINT('Ctrl Pts',(-7.47257747883246,-24.443237814649,
0.));
#194312=CARTESIAN_POINT('Ctrl Pts',(-7.47257747883246,-24.443237814649,
12.));
#194313=CARTESIAN_POINT('Ctrl Pts',(-7.47778614286565,-24.4164662871163,
0.));
#194314=CARTESIAN_POINT('Ctrl Pts',(-7.47778614286565,-24.4164662871163,
12.));
#194315=CARTESIAN_POINT('Ctrl Pts',(-7.48292022569301,-24.3897541049254,
0.));
#194316=CARTESIAN_POINT('Ctrl Pts',(-7.48292022569301,-24.3897541049254,
12.));
#194317=CARTESIAN_POINT('Ctrl Pts',(-7.48797986651909,-24.3631017084524,
0.));
#194318=CARTESIAN_POINT('Ctrl Pts',(-7.48797986651909,-24.3631017084524,
12.));
#194319=CARTESIAN_POINT('Ctrl Pts',(-7.49296521252421,-24.3365095573685,
0.));
#194320=CARTESIAN_POINT('Ctrl Pts',(-7.49296521252421,-24.3365095573685,
12.));
#194321=CARTESIAN_POINT('Ctrl Pts',(-7.49787641695439,-24.3099781253355,
0.));
#194322=CARTESIAN_POINT('Ctrl Pts',(-7.49787641695439,-24.3099781253355,
12.));
#194323=CARTESIAN_POINT('Ctrl Pts',(-7.50271363765152,-24.2835078958973,
0.));
#194324=CARTESIAN_POINT('Ctrl Pts',(-7.50271363765152,-24.2835078958973,
12.));
#194325=CARTESIAN_POINT('Ctrl Pts',(-7.50747703535134,-24.2570993577034,
0.));
#194326=CARTESIAN_POINT('Ctrl Pts',(-7.50747703535134,-24.2570993577034,
12.));
#194327=CARTESIAN_POINT('Ctrl Pts',(-7.51216677222181,-24.2307530003887,
0.));
#194328=CARTESIAN_POINT('Ctrl Pts',(-7.51216677222181,-24.2307530003887,
12.));
#194329=CARTESIAN_POINT('Ctrl Pts',(-7.51678300997949,-24.2044693092349,
0.));
#194330=CARTESIAN_POINT('Ctrl Pts',(-7.51678300997949,-24.2044693092349,
12.));
#194331=CARTESIAN_POINT('Ctrl Pts',(-7.52132590953802,-24.1782487641594,
0.));
#194332=CARTESIAN_POINT('Ctrl Pts',(-7.52132590953802,-24.1782487641594,
12.));
#194333=CARTESIAN_POINT('Ctrl Pts',(-7.52579563201424,-24.1520918425364,
0.));
#194334=CARTESIAN_POINT('Ctrl Pts',(-7.52579563201424,-24.1520918425364,
12.));
#194335=CARTESIAN_POINT('Ctrl Pts',(-7.53019233935502,-24.1259990209207,
0.));
#194336=CARTESIAN_POINT('Ctrl Pts',(-7.53019233935502,-24.1259990209207,
12.));
#194337=CARTESIAN_POINT('Ctrl Pts',(-7.53451619514649,-24.0999707772642,
0.));
#194338=CARTESIAN_POINT('Ctrl Pts',(-7.53451619514649,-24.0999707772642,
12.));
#194339=CARTESIAN_POINT('Ctrl Pts',(-7.53876736531014,-24.0740075927985,
0.));
#194340=CARTESIAN_POINT('Ctrl Pts',(-7.53876736531014,-24.0740075927985,
12.));
#194341=CARTESIAN_POINT('Ctrl Pts',(-7.54294601896145,-24.0481099543353,
0.));
#194342=CARTESIAN_POINT('Ctrl Pts',(-7.54294601896145,-24.0481099543353,
12.));
#194343=CARTESIAN_POINT('Ctrl Pts',(-7.5470523288591,-24.022278355453,0.));
#194344=CARTESIAN_POINT('Ctrl Pts',(-7.5470523288591,-24.022278355453,12.));
#194345=CARTESIAN_POINT('Ctrl Pts',(-7.55108647097441,-23.9965132953185,
0.));
#194346=CARTESIAN_POINT('Ctrl Pts',(-7.55108647097441,-23.9965132953185,
12.));
#194347=CARTESIAN_POINT('Ctrl Pts',(-7.55504862424812,-23.9708152779884,
0.));
#194348=CARTESIAN_POINT('Ctrl Pts',(-7.55504862424812,-23.9708152779884,
12.));
#194349=CARTESIAN_POINT('Ctrl Pts',(-7.55893897027683,-23.9451848115,0.));
#194350=CARTESIAN_POINT('Ctrl Pts',(-7.55893897027683,-23.9451848115,12.));
#194351=CARTESIAN_POINT('Ctrl Pts',(-7.56275769304773,-23.9196224070759,
0.));
#194352=CARTESIAN_POINT('Ctrl Pts',(-7.56275769304773,-23.9196224070759,
12.));
#194353=CARTESIAN_POINT('Ctrl Pts',(-7.56650497863792,-23.8941285782003,
0.));
#194354=CARTESIAN_POINT('Ctrl Pts',(-7.56650497863792,-23.8941285782003,
12.));
#194355=CARTESIAN_POINT('Ctrl Pts',(-7.57018101500711,-23.8687038399597,
0.));
#194356=CARTESIAN_POINT('Ctrl Pts',(-7.57018101500711,-23.8687038399597,
12.));
#194357=CARTESIAN_POINT('Ctrl Pts',(-7.57378599219817,-23.8433487096134,
0.));
#194358=CARTESIAN_POINT('Ctrl Pts',(-7.57378599219817,-23.8433487096134,
12.));
#194359=CARTESIAN_POINT('Ctrl Pts',(-7.57732010249066,-23.8180637069977,
0.));
#194360=CARTESIAN_POINT('Ctrl Pts',(-7.57732010249066,-23.8180637069977,
12.));
#194361=CARTESIAN_POINT('Ctrl Pts',(-7.58078354058212,-23.7928493549908,
0.));
#194362=CARTESIAN_POINT('Ctrl Pts',(-7.58078354058212,-23.7928493549908,
12.));
#194363=CARTESIAN_POINT('Ctrl Pts',(-7.58417650376272,-23.7677061799376,
0.));
#194364=CARTESIAN_POINT('Ctrl Pts',(-7.58417650376272,-23.7677061799376,
12.));
#194365=CARTESIAN_POINT('Ctrl Pts',(-7.58749919210832,-23.7426347121006,
0.));
#194366=CARTESIAN_POINT('Ctrl Pts',(-7.58749919210832,-23.7426347121006,
12.));
#194367=CARTESIAN_POINT('Ctrl Pts',(-7.59075180865327,-23.7176354860457,
0.));
#194368=CARTESIAN_POINT('Ctrl Pts',(-7.59075180865327,-23.7176354860457,
12.));
#194369=CARTESIAN_POINT('Ctrl Pts',(-7.59393455934042,-23.6927090405067,
0.));
#194370=CARTESIAN_POINT('Ctrl Pts',(-7.59393455934042,-23.6927090405067,
12.));
#194371=CARTESIAN_POINT('Ctrl Pts',(-7.59704765299572,-23.6678559182876,
0.));
#194372=CARTESIAN_POINT('Ctrl Pts',(-7.59704765299572,-23.6678559182876,
12.));
#194373=CARTESIAN_POINT('Ctrl Pts',(-7.6000913013013,-23.6430766661419,
0.));
#194374=CARTESIAN_POINT('Ctrl Pts',(-7.6000913013013,-23.6430766661419,
12.));
#194375=CARTESIAN_POINT('Ctrl Pts',(-7.60306571877806,-23.6183718346576,
0.));
#194376=CARTESIAN_POINT('Ctrl Pts',(-7.60306571877806,-23.6183718346576,
12.));
#194377=CARTESIAN_POINT('Ctrl Pts',(-7.60597112277094,-23.5937419781244,
0.));
#194378=CARTESIAN_POINT('Ctrl Pts',(-7.60597112277094,-23.5937419781244,
12.));
#194379=CARTESIAN_POINT('Ctrl Pts',(-7.608807733446,-23.5691876544243,0.));
#194380=CARTESIAN_POINT('Ctrl Pts',(-7.608807733446,-23.5691876544243,12.));
#194381=CARTESIAN_POINT('Ctrl Pts',(-7.61157577385372,-23.5447094252028,
0.));
#194382=CARTESIAN_POINT('Ctrl Pts',(-7.61157577385372,-23.5447094252028,
12.));
#194383=CARTESIAN_POINT('Ctrl Pts',(-7.61427546999299,-23.5203078560128,
0.));
#194384=CARTESIAN_POINT('Ctrl Pts',(-7.61427546999299,-23.5203078560128,
12.));
#194385=CARTESIAN_POINT('Ctrl Pts',(-7.61690705088319,-23.4959835164608,
0.));
#194386=CARTESIAN_POINT('Ctrl Pts',(-7.61690705088319,-23.4959835164608,
12.));
#194387=CARTESIAN_POINT('Ctrl Pts',(-7.61947074863978,-23.4717369803438,
0.));
#194388=CARTESIAN_POINT('Ctrl Pts',(-7.61947074863978,-23.4717369803438,
12.));
#194389=CARTESIAN_POINT('Ctrl Pts',(-7.62196679855957,-23.4475688257854,
0.));
#194390=CARTESIAN_POINT('Ctrl Pts',(-7.62196679855957,-23.4475688257854,
12.));
#194391=CARTESIAN_POINT('Ctrl Pts',(-7.62439543920055,-23.4234796353544,
0.));
#194392=CARTESIAN_POINT('Ctrl Pts',(-7.62439543920055,-23.4234796353544,
12.));
#194393=CARTESIAN_POINT('Ctrl Pts',(-7.62675691240335,-23.3994699961122,
0.));
#194394=CARTESIAN_POINT('Ctrl Pts',(-7.62675691240335,-23.3994699961122,
12.));
#194395=CARTESIAN_POINT('Ctrl Pts',(-7.62905146332598,-23.3755404996638,
0.));
#194396=CARTESIAN_POINT('Ctrl Pts',(-7.62905146332598,-23.3755404996638,
12.));
#194397=CARTESIAN_POINT('Ctrl Pts',(-7.63127934048139,-23.3516917421973,
0.));
#194398=CARTESIAN_POINT('Ctrl Pts',(-7.63127934048139,-23.3516917421973,
12.));
#194399=CARTESIAN_POINT('Ctrl Pts',(-7.63344079578163,-23.3279243245241,
0.));
#194400=CARTESIAN_POINT('Ctrl Pts',(-7.63344079578163,-23.3279243245241,
12.));
#194401=CARTESIAN_POINT('Ctrl Pts',(-7.63553608458784,-23.3042388521021,
0.));
#194402=CARTESIAN_POINT('Ctrl Pts',(-7.63553608458784,-23.3042388521021,
12.));
#194403=CARTESIAN_POINT('Ctrl Pts',(-7.63756546576375,-23.2806359350853,
0.));
#194404=CARTESIAN_POINT('Ctrl Pts',(-7.63756546576375,-23.2806359350853,
12.));
#194405=CARTESIAN_POINT('Ctrl Pts',(-7.63952920172837,-23.2571161884487,
0.));
#194406=CARTESIAN_POINT('Ctrl Pts',(-7.63952920172837,-23.2571161884487,
12.));
#194407=CARTESIAN_POINT('Ctrl Pts',(-7.64142755851508,-23.2336802320912,
0.));
#194408=CARTESIAN_POINT('Ctrl Pts',(-7.64142755851508,-23.2336802320912,
12.));
#194409=CARTESIAN_POINT('Ctrl Pts',(-7.64326080583684,-23.2103286909399,
0.));
#194410=CARTESIAN_POINT('Ctrl Pts',(-7.64326080583684,-23.2103286909399,
12.));
#194411=CARTESIAN_POINT('Ctrl Pts',(-7.64502921715483,-23.1870621950452,
0.));
#194412=CARTESIAN_POINT('Ctrl Pts',(-7.64502921715483,-23.1870621950452,
12.));
#194413=CARTESIAN_POINT('Ctrl Pts',(-7.64673306975797,-23.1638813796691,
0.));
#194414=CARTESIAN_POINT('Ctrl Pts',(-7.64673306975797,-23.1638813796691,
12.));
#194415=CARTESIAN_POINT('Ctrl Pts',(-7.64837264482929,-23.1407868853815,
0.));
#194416=CARTESIAN_POINT('Ctrl Pts',(-7.64837264482929,-23.1407868853815,
12.));
#194417=CARTESIAN_POINT('Ctrl Pts',(-7.64994822749845,-23.1177793581674,
0.));
#194418=CARTESIAN_POINT('Ctrl Pts',(-7.64994822749845,-23.1177793581674,
12.));
#194419=CARTESIAN_POINT('Ctrl Pts',(-7.65146010690465,-23.0948594495246,
0.));
#194420=CARTESIAN_POINT('Ctrl Pts',(-7.65146010690465,-23.0948594495246,
12.));
#194421=CARTESIAN_POINT('Ctrl Pts',(-7.65290857626357,-23.072027816555,
0.));
#194422=CARTESIAN_POINT('Ctrl Pts',(-7.65290857626357,-23.072027816555,
12.));
#194423=CARTESIAN_POINT('Ctrl Pts',(-7.65429393293955,-23.049285122053,
0.));
#194424=CARTESIAN_POINT('Ctrl Pts',(-7.65429393293955,-23.049285122053,
12.));
#194425=CARTESIAN_POINT('Ctrl Pts',(-7.65561647852555,-23.0266320345792,
0.));
#194426=CARTESIAN_POINT('Ctrl Pts',(-7.65561647852555,-23.0266320345792,
12.));
#194427=CARTESIAN_POINT('Ctrl Pts',(-7.6568765189133,-23.004069228582,0.));
#194428=CARTESIAN_POINT('Ctrl Pts',(-7.6568765189133,-23.004069228582,12.));
#194429=CARTESIAN_POINT('Ctrl Pts',(-7.65807436436453,-22.9815973845301,
0.));
#194430=CARTESIAN_POINT('Ctrl Pts',(-7.65807436436453,-22.9815973845301,
12.));
#194431=CARTESIAN_POINT('Ctrl Pts',(-7.65921032958912,-22.9592171890332,
0.));
#194432=CARTESIAN_POINT('Ctrl Pts',(-7.65921032958912,-22.9592171890332,
12.));
#194433=CARTESIAN_POINT('Ctrl Pts',(-7.66028473382777,-22.9369293349592,
0.));
#194434=CARTESIAN_POINT('Ctrl Pts',(-7.66028473382777,-22.9369293349592,
12.));
#194435=CARTESIAN_POINT('Ctrl Pts',(-7.661297900941,-22.9147345215418,0.));
#194436=CARTESIAN_POINT('Ctrl Pts',(-7.661297900941,-22.9147345215418,12.));
#194437=CARTESIAN_POINT('Ctrl Pts',(-7.66225015950148,-22.8926334544879,
0.));
#194438=CARTESIAN_POINT('Ctrl Pts',(-7.66225015950148,-22.8926334544879,
12.));
#194439=CARTESIAN_POINT('Ctrl Pts',(-7.66314184287334,-22.870626846128,
0.));
#194440=CARTESIAN_POINT('Ctrl Pts',(-7.66314184287334,-22.870626846128,
12.));
#194441=CARTESIAN_POINT('Ctrl Pts',(-7.66397328929805,-22.8487154155569,
0.));
#194442=CARTESIAN_POINT('Ctrl Pts',(-7.66397328929805,-22.8487154155569,
12.));
#194443=CARTESIAN_POINT('Ctrl Pts',(-7.66474484198553,-22.8268998887678,
0.));
#194444=CARTESIAN_POINT('Ctrl Pts',(-7.66474484198553,-22.8268998887678,
12.));
#194445=CARTESIAN_POINT('Ctrl Pts',(-7.66545684920988,-22.8051809987833,
0.));
#194446=CARTESIAN_POINT('Ctrl Pts',(-7.66545684920988,-22.8051809987833,
12.));
#194447=CARTESIAN_POINT('Ctrl Pts',(-7.66610966441259,-22.7835594857697,
0.));
#194448=CARTESIAN_POINT('Ctrl Pts',(-7.66610966441259,-22.7835594857697,
12.));
#194449=CARTESIAN_POINT('Ctrl Pts',(-7.66670364630273,-22.7620360971839,
0.));
#194450=CARTESIAN_POINT('Ctrl Pts',(-7.66670364630273,-22.7620360971839,
12.));
#194451=CARTESIAN_POINT('Ctrl Pts',(-7.66723915895413,-22.7406115879508,
0.));
#194452=CARTESIAN_POINT('Ctrl Pts',(-7.66723915895413,-22.7406115879508,
12.));
#194453=CARTESIAN_POINT('Ctrl Pts',(-7.6677165719101,-22.7192867206242,
0.));
#194454=CARTESIAN_POINT('Ctrl Pts',(-7.6677165719101,-22.7192867206242,
12.));
#194455=CARTESIAN_POINT('Ctrl Pts',(-7.66813626029277,-22.6980622655446,
0.));
#194456=CARTESIAN_POINT('Ctrl Pts',(-7.66813626029277,-22.6980622655446,
12.));
#194457=CARTESIAN_POINT('Ctrl Pts',(-7.66849860491763,-22.6769390009889,
0.));
#194458=CARTESIAN_POINT('Ctrl Pts',(-7.66849860491763,-22.6769390009889,
12.));
#194459=CARTESIAN_POINT('Ctrl Pts',(-7.66880399241354,-22.6559177133133,
0.));
#194460=CARTESIAN_POINT('Ctrl Pts',(-7.66880399241354,-22.6559177133133,
12.));
#194461=CARTESIAN_POINT('Ctrl Pts',(-7.66905281533745,-22.6349991971547,
0.));
#194462=CARTESIAN_POINT('Ctrl Pts',(-7.66905281533745,-22.6349991971547,
12.));
#194463=CARTESIAN_POINT('Ctrl Pts',(-7.66924547229435,-22.6141842556248,
0.));
#194464=CARTESIAN_POINT('Ctrl Pts',(-7.66924547229435,-22.6141842556248,
12.));
#194465=CARTESIAN_POINT('Ctrl Pts',(-7.66938236806241,-22.5934737004955,
0.));
#194466=CARTESIAN_POINT('Ctrl Pts',(-7.66938236806241,-22.5934737004955,
12.));
#194467=CARTESIAN_POINT('Ctrl Pts',(-7.66946391372299,-22.5728683523828,
0.));
#194468=CARTESIAN_POINT('Ctrl Pts',(-7.66946391372299,-22.5728683523828,
12.));
#194469=CARTESIAN_POINT('Ctrl Pts',(-7.66949052679672,-22.5523690409109,
0.));
#194470=CARTESIAN_POINT('Ctrl Pts',(-7.66949052679672,-22.5523690409109,
12.));
#194471=CARTESIAN_POINT('Ctrl Pts',(-7.66946263138116,-22.5319766049191,
0.));
#194472=CARTESIAN_POINT('Ctrl Pts',(-7.66946263138116,-22.5319766049191,
12.));
#194473=CARTESIAN_POINT('Ctrl Pts',(-7.66938065829083,-22.5116918927023,
0.));
#194474=CARTESIAN_POINT('Ctrl Pts',(-7.66938065829083,-22.5116918927023,
12.));
#194475=CARTESIAN_POINT('Ctrl Pts',(-7.66924504520302,-22.4915157622308,
0.));
#194476=CARTESIAN_POINT('Ctrl Pts',(-7.66924504520302,-22.4915157622308,
12.));
#194477=CARTESIAN_POINT('Ctrl Pts',(-7.66905623680836,-22.47144908137,0.));
#194478=CARTESIAN_POINT('Ctrl Pts',(-7.66905623680836,-22.47144908137,12.));
#194479=CARTESIAN_POINT('Ctrl Pts',(-7.6688146849666,-22.4514927280862,
0.));
#194480=CARTESIAN_POINT('Ctrl Pts',(-7.6688146849666,-22.4514927280862,
12.));
#194481=CARTESIAN_POINT('Ctrl Pts',(-7.66852084886746,-22.4316475906616,
0.));
#194482=CARTESIAN_POINT('Ctrl Pts',(-7.66852084886746,-22.4316475906616,
12.));
#194483=CARTESIAN_POINT('Ctrl Pts',(-7.66817519519682,-22.411914567977,
0.));
#194484=CARTESIAN_POINT('Ctrl Pts',(-7.66817519519682,-22.411914567977,
12.));
#194485=CARTESIAN_POINT('Ctrl Pts',(-7.6677781983082,-22.3922945697782,
0.));
#194486=CARTESIAN_POINT('Ctrl Pts',(-7.6677781983082,-22.3922945697782,
12.));
#194487=CARTESIAN_POINT('Ctrl Pts',(-7.66733034039887,-22.3727885169361,
0.));
#194488=CARTESIAN_POINT('Ctrl Pts',(-7.66733034039887,-22.3727885169361,
12.));
#194489=CARTESIAN_POINT('Ctrl Pts',(-7.66683211169134,-22.3533973417013,
0.));
#194490=CARTESIAN_POINT('Ctrl Pts',(-7.66683211169134,-22.3533973417013,
12.));
#194491=CARTESIAN_POINT('Ctrl Pts',(-7.66628401061906,-22.3341219879454,
0.));
#194492=CARTESIAN_POINT('Ctrl Pts',(-7.66628401061906,-22.3341219879454,
12.));
#194493=CARTESIAN_POINT('Ctrl Pts',(-7.66568654402442,-22.3149634114823,
0.));
#194494=CARTESIAN_POINT('Ctrl Pts',(-7.66568654402442,-22.3149634114823,
12.));
#194495=CARTESIAN_POINT('Ctrl Pts',(-7.66504022736263,-22.2959225803925,
0.));
#194496=CARTESIAN_POINT('Ctrl Pts',(-7.66504022736263,-22.2959225803925,
12.));
#194497=CARTESIAN_POINT('Ctrl Pts',(-7.66434558490973,-22.2770004753332,
0.));
#194498=CARTESIAN_POINT('Ctrl Pts',(-7.66434558490973,-22.2770004753332,
12.));
#194499=CARTESIAN_POINT('Ctrl Pts',(-7.66360314997662,-22.2581980898487,
0.));
#194500=CARTESIAN_POINT('Ctrl Pts',(-7.66360314997662,-22.2581980898487,
12.));
#194501=CARTESIAN_POINT('Ctrl Pts',(-7.66281346512546,-22.239516430656,
0.));
#194502=CARTESIAN_POINT('Ctrl Pts',(-7.66281346512546,-22.239516430656,
12.));
#194503=CARTESIAN_POINT('Ctrl Pts',(-7.66197708240436,-22.2209565180098,
0.));
#194504=CARTESIAN_POINT('Ctrl Pts',(-7.66197708240436,-22.2209565180098,
12.));
#194505=CARTESIAN_POINT('Ctrl Pts',(-7.66109456359292,-22.2025193860972,
0.));
#194506=CARTESIAN_POINT('Ctrl Pts',(-7.66109456359292,-22.2025193860972,
12.));
#194507=CARTESIAN_POINT('Ctrl Pts',(-7.66016648045008,-22.1842060834092,
0.));
#194508=CARTESIAN_POINT('Ctrl Pts',(-7.66016648045008,-22.1842060834092,
12.));
#194509=CARTESIAN_POINT('Ctrl Pts',(-7.65919341496926,-22.1660176731174,
0.));
#194510=CARTESIAN_POINT('Ctrl Pts',(-7.65919341496926,-22.1660176731174,
12.));
#194511=CARTESIAN_POINT('Ctrl Pts',(-7.65817595963351,-22.1479552334206,
0.));
#194512=CARTESIAN_POINT('Ctrl Pts',(-7.65817595963351,-22.1479552334206,
12.));
#194513=CARTESIAN_POINT('Ctrl Pts',(-7.65711471769407,-22.1300198579671,
0.));
#194514=CARTESIAN_POINT('Ctrl Pts',(-7.65711471769407,-22.1300198579671,
12.));
#194515=CARTESIAN_POINT('Ctrl Pts',(-7.65601030346819,-22.1122126563327,
0.));
#194516=CARTESIAN_POINT('Ctrl Pts',(-7.65601030346819,-22.1122126563327,
12.));
#194517=CARTESIAN_POINT('Ctrl Pts',(-7.65486334263651,-22.094534754469,
0.));
#194518=CARTESIAN_POINT('Ctrl Pts',(-7.65486334263651,-22.094534754469,
12.));
#194519=CARTESIAN_POINT('Ctrl Pts',(-7.65367447254945,-22.0769872951596,
0.));
#194520=CARTESIAN_POINT('Ctrl Pts',(-7.65367447254945,-22.0769872951596,
12.));
#194521=CARTESIAN_POINT('Ctrl Pts',(-7.65244434253104,-22.0595714384432,
0.));
#194522=CARTESIAN_POINT('Ctrl Pts',(-7.65244434253104,-22.0595714384432,
12.));
#194523=CARTESIAN_POINT('Ctrl Pts',(-7.65117361421347,-22.0422883621176,
0.));
#194524=CARTESIAN_POINT('Ctrl Pts',(-7.65117361421347,-22.0422883621176,
12.));
#194525=CARTESIAN_POINT('Ctrl Pts',(-7.64986296190157,-22.0251392623209,
0.));
#194526=CARTESIAN_POINT('Ctrl Pts',(-7.64986296190157,-22.0251392623209,
12.));
#194527=CARTESIAN_POINT('Ctrl Pts',(-7.64851307293346,-22.0081253540773,
0.));
#194528=CARTESIAN_POINT('Ctrl Pts',(-7.64851307293346,-22.0081253540773,
12.));
#194529=CARTESIAN_POINT('Ctrl Pts',(-7.64712464805258,-21.9912478718542,
0.));
#194530=CARTESIAN_POINT('Ctrl Pts',(-7.64712464805258,-21.9912478718542,
12.));
#194531=CARTESIAN_POINT('Ctrl Pts',(-7.64569840177359,-21.97450807008,0.));
#194532=CARTESIAN_POINT('Ctrl Pts',(-7.64569840177359,-21.97450807008,12.));
#194533=CARTESIAN_POINT('Ctrl Pts',(-7.64423506279154,-21.9579072237653,
0.));
#194534=CARTESIAN_POINT('Ctrl Pts',(-7.64423506279154,-21.9579072237653,
12.));
#194535=CARTESIAN_POINT('Ctrl Pts',(-7.64273537442707,-21.9414466292074,
0.));
#194536=CARTESIAN_POINT('Ctrl Pts',(-7.64273537442707,-21.9414466292074,
12.));
#194537=CARTESIAN_POINT('Ctrl Pts',(-7.6412000950654,-21.9251276046546,
0.));
#194538=CARTESIAN_POINT('Ctrl Pts',(-7.6412000950654,-21.9251276046546,
12.));
#194539=CARTESIAN_POINT('Ctrl Pts',(-7.63962999860917,-21.9089514909873,
0.));
#194540=CARTESIAN_POINT('Ctrl Pts',(-7.63962999860917,-21.9089514909873,
12.));
#194541=CARTESIAN_POINT('Ctrl Pts',(-7.63802587492008,-21.8929196523511,
0.));
#194542=CARTESIAN_POINT('Ctrl Pts',(-7.63802587492008,-21.8929196523511,
12.));
#194543=CARTESIAN_POINT('Ctrl Pts',(-7.63638853033368,-21.8770334769492,
0.));
#194544=CARTESIAN_POINT('Ctrl Pts',(-7.63638853033368,-21.8770334769492,
12.));
#194545=CARTESIAN_POINT('Ctrl Pts',(-7.63471878821204,-21.8612943779086,
0.));
#194546=CARTESIAN_POINT('Ctrl Pts',(-7.63471878821204,-21.8612943779086,
12.));
#194547=CARTESIAN_POINT('Ctrl Pts',(-7.63301748948936,-21.8457037941084,
0.));
#194548=CARTESIAN_POINT('Ctrl Pts',(-7.63301748948936,-21.8457037941084,
12.));
#194549=CARTESIAN_POINT('Ctrl Pts',(-7.6312854932304,-21.8302631910197,
0.));
#194550=CARTESIAN_POINT('Ctrl Pts',(-7.6312854932304,-21.8302631910197,
12.));
#194551=CARTESIAN_POINT('Ctrl Pts',(-7.62952367718151,-21.8149740615093,
0.));
#194552=CARTESIAN_POINT('Ctrl Pts',(-7.62952367718151,-21.8149740615093,
12.));
#194553=CARTESIAN_POINT('Ctrl Pts',(-7.62773293842409,-21.7998379268583,
0.));
#194554=CARTESIAN_POINT('Ctrl Pts',(-7.62773293842409,-21.7998379268583,
12.));
#194555=CARTESIAN_POINT('Ctrl Pts',(-7.62591419404521,-21.7848563378022,
0.));
#194556=CARTESIAN_POINT('Ctrl Pts',(-7.62591419404521,-21.7848563378022,
12.));
#194557=CARTESIAN_POINT('Ctrl Pts',(-7.62406838181164,-21.7700308755583,
0.));
#194558=CARTESIAN_POINT('Ctrl Pts',(-7.62406838181164,-21.7700308755583,
12.));
#194559=CARTESIAN_POINT('Ctrl Pts',(-7.62219646084226,-21.7553631528329,
0.));
#194560=CARTESIAN_POINT('Ctrl Pts',(-7.62219646084226,-21.7553631528329,
12.));
#194561=CARTESIAN_POINT('Ctrl Pts',(-7.62029941230855,-21.7408548148657,
0.));
#194562=CARTESIAN_POINT('Ctrl Pts',(-7.62029941230855,-21.7408548148657,
12.));
#194563=CARTESIAN_POINT('Ctrl Pts',(-7.61837824030542,-21.7265075407977,
0.));
#194564=CARTESIAN_POINT('Ctrl Pts',(-7.61837824030542,-21.7265075407977,
12.));
#194565=CARTESIAN_POINT('Ctrl Pts',(-7.61643397270425,-21.7123230449835,
0.));
#194566=CARTESIAN_POINT('Ctrl Pts',(-7.61643397270425,-21.7123230449835,
12.));
#194567=CARTESIAN_POINT('Ctrl Pts',(-7.61446766202787,-21.6983030783321,
0.));
#194568=CARTESIAN_POINT('Ctrl Pts',(-7.61446766202787,-21.6983030783321,
12.));
#194569=CARTESIAN_POINT('Ctrl Pts',(-7.61248038630265,-21.6844494295813,
0.));
#194570=CARTESIAN_POINT('Ctrl Pts',(-7.61248038630265,-21.6844494295813,
12.));
#194571=CARTESIAN_POINT('Ctrl Pts',(-7.6104732500095,-21.6707639267573,
0.));
#194572=CARTESIAN_POINT('Ctrl Pts',(-7.6104732500095,-21.6707639267573,
12.));
#194573=CARTESIAN_POINT('Ctrl Pts',(-7.60844738512872,-21.6572484388079,
0.));
#194574=CARTESIAN_POINT('Ctrl Pts',(-7.60844738512872,-21.6572484388079,
12.));
#194575=CARTESIAN_POINT('Ctrl Pts',(-7.60640395216359,-21.6439048771743,
0.));
#194576=CARTESIAN_POINT('Ctrl Pts',(-7.60640395216359,-21.6439048771743,
12.));
#194577=CARTESIAN_POINT('Ctrl Pts',(-7.604344141183,-21.6307351973823,0.));
#194578=CARTESIAN_POINT('Ctrl Pts',(-7.604344141183,-21.6307351973823,12.));
#194579=CARTESIAN_POINT('Ctrl Pts',(-7.60226917285432,-21.6177414005991,
0.));
#194580=CARTESIAN_POINT('Ctrl Pts',(-7.60226917285432,-21.6177414005991,
12.));
#194581=CARTESIAN_POINT('Ctrl Pts',(-7.60018029988238,-21.6049255358842,
0.));
#194582=CARTESIAN_POINT('Ctrl Pts',(-7.60018029988238,-21.6049255358842,
12.));
#194583=CARTESIAN_POINT('Ctrl Pts',(-7.59807880846193,-21.5922897024466,
0.));
#194584=CARTESIAN_POINT('Ctrl Pts',(-7.59807880846193,-21.5922897024466,
12.));
#194585=CARTESIAN_POINT('Ctrl Pts',(-7.59596601973589,-21.5798360518978,
0.));
#194586=CARTESIAN_POINT('Ctrl Pts',(-7.59596601973589,-21.5798360518978,
12.));
#194587=CARTESIAN_POINT('Ctrl Pts',(-7.5938432912493,-21.5675667904728,
0.));
#194588=CARTESIAN_POINT('Ctrl Pts',(-7.5938432912493,-21.5675667904728,
12.));
#194589=CARTESIAN_POINT('Ctrl Pts',(-7.59171201844793,-21.5554841813465,
0.));
#194590=CARTESIAN_POINT('Ctrl Pts',(-7.59171201844793,-21.5554841813465,
12.));
#194591=CARTESIAN_POINT('Ctrl Pts',(-7.58957363620026,-21.5435905470113,
0.));
#194592=CARTESIAN_POINT('Ctrl Pts',(-7.58957363620026,-21.5435905470113,
12.));
#194593=CARTESIAN_POINT('Ctrl Pts',(-7.58742962034834,-21.5318882716735,
0.));
#194594=CARTESIAN_POINT('Ctrl Pts',(-7.58742962034834,-21.5318882716735,
12.));
#194595=CARTESIAN_POINT('Ctrl Pts',(-7.58528148919114,-21.5203798035294,
0.));
#194596=CARTESIAN_POINT('Ctrl Pts',(-7.58528148919114,-21.5203798035294,
12.));
#194597=CARTESIAN_POINT('Ctrl Pts',(-7.58313080519159,-21.5090676573866,
0.));
#194598=CARTESIAN_POINT('Ctrl Pts',(-7.58313080519159,-21.5090676573866,
12.));
#194599=CARTESIAN_POINT('Ctrl Pts',(-7.5809791779073,-21.4979544192739,
0.));
#194600=CARTESIAN_POINT('Ctrl Pts',(-7.5809791779073,-21.4979544192739,
12.));
#194601=CARTESIAN_POINT('Ctrl Pts',(-7.57882826679131,-21.4870427508193,
0.));
#194602=CARTESIAN_POINT('Ctrl Pts',(-7.57882826679131,-21.4870427508193,
12.));
#194603=CARTESIAN_POINT('Ctrl Pts',(-7.57667978403003,-21.4763353936766,
0.));
#194604=CARTESIAN_POINT('Ctrl Pts',(-7.57667978403003,-21.4763353936766,
12.));
#194605=CARTESIAN_POINT('Ctrl Pts',(-7.57453549743435,-21.4658351740135,
0.));
#194606=CARTESIAN_POINT('Ctrl Pts',(-7.57453549743435,-21.4658351740135,
12.));
#194607=CARTESIAN_POINT('Ctrl Pts',(-7.57239723223521,-21.4555450053147,
0.));
#194608=CARTESIAN_POINT('Ctrl Pts',(-7.57239723223521,-21.4555450053147,
12.));
#194609=CARTESIAN_POINT('Ctrl Pts',(-7.5702668726117,-21.445467890751,0.));
#194610=CARTESIAN_POINT('Ctrl Pts',(-7.5702668726117,-21.445467890751,12.));
#194611=CARTESIAN_POINT('Ctrl Pts',(-7.56814636360842,-21.435606926151,
0.));
#194612=CARTESIAN_POINT('Ctrl Pts',(-7.56814636360842,-21.435606926151,
12.));
#194613=CARTESIAN_POINT('Ctrl Pts',(-7.56603771218706,-21.4259653015732,
0.));
#194614=CARTESIAN_POINT('Ctrl Pts',(-7.56603771218706,-21.4259653015732,
12.));
#194615=CARTESIAN_POINT('Ctrl Pts',(-7.56394299313683,-21.4165463106252,
0.));
#194616=CARTESIAN_POINT('Ctrl Pts',(-7.56394299313683,-21.4165463106252,
12.));
#194617=CARTESIAN_POINT('Ctrl Pts',(-7.56186435703622,-21.4073533630364,
0.));
#194618=CARTESIAN_POINT('Ctrl Pts',(-7.56186435703622,-21.4073533630364,
12.));
#194619=CARTESIAN_POINT('Ctrl Pts',(-7.55980403700615,-21.3983899952988,
0.));
#194620=CARTESIAN_POINT('Ctrl Pts',(-7.55980403700615,-21.3983899952988,
12.));
#194621=CARTESIAN_POINT('Ctrl Pts',(-7.55776435731422,-21.3896598842119,
0.));
#194622=CARTESIAN_POINT('Ctrl Pts',(-7.55776435731422,-21.3896598842119,
12.));
#194623=CARTESIAN_POINT('Ctrl Pts',(-7.55574773403508,-21.3811668478933,
0.));
#194624=CARTESIAN_POINT('Ctrl Pts',(-7.55574773403508,-21.3811668478933,
12.));
#194625=CARTESIAN_POINT('Ctrl Pts',(-7.55375667080032,-21.3729148390244,
0.));
#194626=CARTESIAN_POINT('Ctrl Pts',(-7.55375667080032,-21.3729148390244,
12.));
#194627=CARTESIAN_POINT('Ctrl Pts',(-7.55179375777442,-21.3649079431864,
0.));
#194628=CARTESIAN_POINT('Ctrl Pts',(-7.55179375777442,-21.3649079431864,
12.));
#194629=CARTESIAN_POINT('Ctrl Pts',(-7.54986166521307,-21.3571503685853,
0.));
#194630=CARTESIAN_POINT('Ctrl Pts',(-7.54986166521307,-21.3571503685853,
12.));
#194631=CARTESIAN_POINT('Ctrl Pts',(-7.54796316246327,-21.349646476153,
0.));
#194632=CARTESIAN_POINT('Ctrl Pts',(-7.54796316246327,-21.349646476153,
12.));
#194633=CARTESIAN_POINT('Ctrl Pts',(-7.54610114948351,-21.3424008295038,
0.));
#194634=CARTESIAN_POINT('Ctrl Pts',(-7.54610114948351,-21.3424008295038,
12.));
#194635=CARTESIAN_POINT('Ctrl Pts',(-7.54427868151269,-21.3354182340149,
0.));
#194636=CARTESIAN_POINT('Ctrl Pts',(-7.54427868151269,-21.3354182340149,
12.));
#194637=CARTESIAN_POINT('Ctrl Pts',(-7.54249900377032,-21.328703791771,
0.));
#194638=CARTESIAN_POINT('Ctrl Pts',(-7.54249900377032,-21.328703791771,
12.));
#194639=CARTESIAN_POINT('Ctrl Pts',(-7.5407655203828,-21.3222628524165,
0.));
#194640=CARTESIAN_POINT('Ctrl Pts',(-7.5407655203828,-21.3222628524165,
12.));
#194641=CARTESIAN_POINT('Ctrl Pts',(-7.53908175169899,-21.3161009456256,
0.));
#194642=CARTESIAN_POINT('Ctrl Pts',(-7.53908175169899,-21.3161009456256,
12.));
#194643=CARTESIAN_POINT('Ctrl Pts',(-7.5374512936462,-21.3102237167729,
0.));
#194644=CARTESIAN_POINT('Ctrl Pts',(-7.5374512936462,-21.3102237167729,
12.));
#194645=CARTESIAN_POINT('Ctrl Pts',(-7.53587778251743,-21.3046368712156,
0.));
#194646=CARTESIAN_POINT('Ctrl Pts',(-7.53587778251743,-21.3046368712156,
12.));
#194647=CARTESIAN_POINT('Ctrl Pts',(-7.53436505309949,-21.2993464250717,
0.));
#194648=CARTESIAN_POINT('Ctrl Pts',(-7.53436505309949,-21.2993464250717,
12.));
#194649=CARTESIAN_POINT('Ctrl Pts',(-7.53291726078527,-21.2943588989331,
0.));
#194650=CARTESIAN_POINT('Ctrl Pts',(-7.53291726078527,-21.2943588989331,
12.));
#194651=CARTESIAN_POINT('Ctrl Pts',(-7.53153906987847,-21.2896816163843,
0.));
#194652=CARTESIAN_POINT('Ctrl Pts',(-7.53153906987847,-21.2896816163843,
12.));
#194653=CARTESIAN_POINT('Ctrl Pts',(-7.53023562438221,-21.2853226580658,
0.));
#194654=CARTESIAN_POINT('Ctrl Pts',(-7.53023562438221,-21.2853226580658,
12.));
#194655=CARTESIAN_POINT('Ctrl Pts',(-7.52901217930407,-21.2812902781143,
0.));
#194656=CARTESIAN_POINT('Ctrl Pts',(-7.52901217930407,-21.2812902781143,
12.));
#194657=CARTESIAN_POINT('Ctrl Pts',(-7.52787386225344,-21.2775925269651,
0.));
#194658=CARTESIAN_POINT('Ctrl Pts',(-7.52787386225344,-21.2775925269651,
12.));
#194659=CARTESIAN_POINT('Ctrl Pts',(-7.52682526918561,-21.2742366113578,
0.));
#194660=CARTESIAN_POINT('Ctrl Pts',(-7.52682526918561,-21.2742366113578,
12.));
#194661=CARTESIAN_POINT('Ctrl Pts',(-7.52587126095544,-21.2712301573465,
0.));
#194662=CARTESIAN_POINT('Ctrl Pts',(-7.52587126095544,-21.2712301573465,
12.));
#194663=CARTESIAN_POINT('Ctrl Pts',(-7.52501770333522,-21.2685823838672,
0.));
#194664=CARTESIAN_POINT('Ctrl Pts',(-7.52501770333522,-21.2685823838672,
12.));
#194665=CARTESIAN_POINT('Ctrl Pts',(-7.52427261074264,-21.266305915706,
0.));
#194666=CARTESIAN_POINT('Ctrl Pts',(-7.52427261074264,-21.266305915706,
12.));
#194667=CARTESIAN_POINT('Ctrl Pts',(-7.52364573027521,-21.2644161259965,
0.));
#194668=CARTESIAN_POINT('Ctrl Pts',(-7.52364573027521,-21.2644161259965,
12.));
#194669=CARTESIAN_POINT('Ctrl Pts',(-7.52314642316203,-21.262927782038,
0.));
#194670=CARTESIAN_POINT('Ctrl Pts',(-7.52314642316203,-21.262927782038,
12.));
#194671=CARTESIAN_POINT('Ctrl Pts',(-7.52278182242728,-21.261852128355,
0.));
#194672=CARTESIAN_POINT('Ctrl Pts',(-7.52278182242728,-21.261852128355,
12.));
#194673=CARTESIAN_POINT('Ctrl Pts',(-7.52260064231736,-21.2613260540651,
0.));
#194674=CARTESIAN_POINT('Ctrl Pts',(-7.52260064231736,-21.2613260540651,
12.));
#194675=CARTESIAN_POINT('Ctrl Pts',(-7.52252744144958,-21.261120447486,
0.));
#194676=CARTESIAN_POINT('Ctrl Pts',(-7.52252744144958,-21.261120447486,
12.));
#194677=CARTESIAN_POINT('Ctrl Pts',(-7.52250649703992,-21.2610673466883,
0.));
#194678=CARTESIAN_POINT('Ctrl Pts',(-7.52250649703992,-21.2610673466883,
12.));
#194679=CARTESIAN_POINT('Ctrl Pts',(-7.52250298901266,-21.2610617890679,
0.));
#194680=CARTESIAN_POINT('Ctrl Pts',(-7.52250298901266,-21.2610617890679,
12.));
#194681=CARTESIAN_POINT('',(-7.36589684767345,-24.9347862158358,0.));
#194682=CARTESIAN_POINT('Ctrl Pts',(-7.36589684767345,-24.9347862158358,
0.));
#194683=CARTESIAN_POINT('Ctrl Pts',(-7.36721909028843,-24.9292275670674,
0.));
#194684=CARTESIAN_POINT('Ctrl Pts',(-7.36985593120091,-24.9181155530543,
0.));
#194685=CARTESIAN_POINT('Ctrl Pts',(-7.37378825961676,-24.901463382605,
0.));
#194686=CARTESIAN_POINT('Ctrl Pts',(-7.3789854964027,-24.8792921911115,
0.));
#194687=CARTESIAN_POINT('Ctrl Pts',(-7.38540558903621,-24.8516310625176,
0.));
#194688=CARTESIAN_POINT('Ctrl Pts',(-7.39174922585809,-24.8240228520893,
0.));
#194689=CARTESIAN_POINT('Ctrl Pts',(-7.39801641583013,-24.7964676646431,
0.));
#194690=CARTESIAN_POINT('Ctrl Pts',(-7.40420718661603,-24.7689656668983,
0.));
#194691=CARTESIAN_POINT('Ctrl Pts',(-7.41032159082382,-24.7415170994784,
0.));
#194692=CARTESIAN_POINT('Ctrl Pts',(-7.41635971481674,-24.7141222950051,
0.));
#194693=CARTESIAN_POINT('Ctrl Pts',(-7.42232167766266,-24.6867816727192,
0.));
#194694=CARTESIAN_POINT('Ctrl Pts',(-7.42820762159126,-24.6594957128756,
0.));
#194695=CARTESIAN_POINT('Ctrl Pts',(-7.43401770489524,-24.6322649369517,
0.));
#194696=CARTESIAN_POINT('Ctrl Pts',(-7.43975209375504,-24.6050898852368,
0.));
#194697=CARTESIAN_POINT('Ctrl Pts',(-7.44541095473135,-24.577971096086,
0.));
#194698=CARTESIAN_POINT('Ctrl Pts',(-7.4509944465116,-24.5509090831559,
0.));
#194699=CARTESIAN_POINT('Ctrl Pts',(-7.45650271335862,-24.5239043173072,
0.));
#194700=CARTESIAN_POINT('Ctrl Pts',(-7.46193588961464,-24.4969572391483,
0.));
#194701=CARTESIAN_POINT('Ctrl Pts',(-7.46729410308787,-24.4700682684524,
0.));
#194702=CARTESIAN_POINT('Ctrl Pts',(-7.47257747883246,-24.443237814649,
0.));
#194703=CARTESIAN_POINT('Ctrl Pts',(-7.47778614286565,-24.4164662871163,
0.));
#194704=CARTESIAN_POINT('Ctrl Pts',(-7.48292022569301,-24.3897541049254,
0.));
#194705=CARTESIAN_POINT('Ctrl Pts',(-7.48797986651909,-24.3631017084524,
0.));
#194706=CARTESIAN_POINT('Ctrl Pts',(-7.49296521252421,-24.3365095573685,
0.));
#194707=CARTESIAN_POINT('Ctrl Pts',(-7.49787641695439,-24.3099781253355,
0.));
#194708=CARTESIAN_POINT('Ctrl Pts',(-7.50271363765152,-24.2835078958973,
0.));
#194709=CARTESIAN_POINT('Ctrl Pts',(-7.50747703535134,-24.2570993577034,
0.));
#194710=CARTESIAN_POINT('Ctrl Pts',(-7.51216677222181,-24.2307530003887,
0.));
#194711=CARTESIAN_POINT('Ctrl Pts',(-7.51678300997949,-24.2044693092349,
0.));
#194712=CARTESIAN_POINT('Ctrl Pts',(-7.52132590953802,-24.1782487641594,
0.));
#194713=CARTESIAN_POINT('Ctrl Pts',(-7.52579563201424,-24.1520918425364,
0.));
#194714=CARTESIAN_POINT('Ctrl Pts',(-7.53019233935502,-24.1259990209207,
0.));
#194715=CARTESIAN_POINT('Ctrl Pts',(-7.53451619514649,-24.0999707772642,
0.));
#194716=CARTESIAN_POINT('Ctrl Pts',(-7.53876736531014,-24.0740075927985,
0.));
#194717=CARTESIAN_POINT('Ctrl Pts',(-7.54294601896145,-24.0481099543353,
0.));
#194718=CARTESIAN_POINT('Ctrl Pts',(-7.5470523288591,-24.022278355453,0.));
#194719=CARTESIAN_POINT('Ctrl Pts',(-7.55108647097441,-23.9965132953185,
0.));
#194720=CARTESIAN_POINT('Ctrl Pts',(-7.55504862424812,-23.9708152779884,
0.));
#194721=CARTESIAN_POINT('Ctrl Pts',(-7.55893897027683,-23.9451848115,0.));
#194722=CARTESIAN_POINT('Ctrl Pts',(-7.56275769304773,-23.9196224070759,
0.));
#194723=CARTESIAN_POINT('Ctrl Pts',(-7.56650497863792,-23.8941285782003,
0.));
#194724=CARTESIAN_POINT('Ctrl Pts',(-7.57018101500711,-23.8687038399597,
0.));
#194725=CARTESIAN_POINT('Ctrl Pts',(-7.57378599219817,-23.8433487096134,
0.));
#194726=CARTESIAN_POINT('Ctrl Pts',(-7.57732010249066,-23.8180637069977,
0.));
#194727=CARTESIAN_POINT('Ctrl Pts',(-7.58078354058212,-23.7928493549908,
0.));
#194728=CARTESIAN_POINT('Ctrl Pts',(-7.58417650376272,-23.7677061799376,
0.));
#194729=CARTESIAN_POINT('Ctrl Pts',(-7.58749919210832,-23.7426347121006,
0.));
#194730=CARTESIAN_POINT('Ctrl Pts',(-7.59075180865327,-23.7176354860457,
0.));
#194731=CARTESIAN_POINT('Ctrl Pts',(-7.59393455934042,-23.6927090405067,
0.));
#194732=CARTESIAN_POINT('Ctrl Pts',(-7.59704765299572,-23.6678559182876,
0.));
#194733=CARTESIAN_POINT('Ctrl Pts',(-7.6000913013013,-23.6430766661419,
0.));
#194734=CARTESIAN_POINT('Ctrl Pts',(-7.60306571877806,-23.6183718346576,
0.));
#194735=CARTESIAN_POINT('Ctrl Pts',(-7.60597112277094,-23.5937419781244,
0.));
#194736=CARTESIAN_POINT('Ctrl Pts',(-7.608807733446,-23.5691876544243,0.));
#194737=CARTESIAN_POINT('Ctrl Pts',(-7.61157577385372,-23.5447094252028,
0.));
#194738=CARTESIAN_POINT('Ctrl Pts',(-7.61427546999299,-23.5203078560128,
0.));
#194739=CARTESIAN_POINT('Ctrl Pts',(-7.61690705088319,-23.4959835164608,
0.));
#194740=CARTESIAN_POINT('Ctrl Pts',(-7.61947074863978,-23.4717369803438,
0.));
#194741=CARTESIAN_POINT('Ctrl Pts',(-7.62196679855957,-23.4475688257854,
0.));
#194742=CARTESIAN_POINT('Ctrl Pts',(-7.62439543920055,-23.4234796353544,
0.));
#194743=CARTESIAN_POINT('Ctrl Pts',(-7.62675691240335,-23.3994699961122,
0.));
#194744=CARTESIAN_POINT('Ctrl Pts',(-7.62905146332598,-23.3755404996638,
0.));
#194745=CARTESIAN_POINT('Ctrl Pts',(-7.63127934048139,-23.3516917421973,
0.));
#194746=CARTESIAN_POINT('Ctrl Pts',(-7.63344079578163,-23.3279243245241,
0.));
#194747=CARTESIAN_POINT('Ctrl Pts',(-7.63553608458784,-23.3042388521021,
0.));
#194748=CARTESIAN_POINT('Ctrl Pts',(-7.63756546576375,-23.2806359350853,
0.));
#194749=CARTESIAN_POINT('Ctrl Pts',(-7.63952920172837,-23.2571161884487,
0.));
#194750=CARTESIAN_POINT('Ctrl Pts',(-7.64142755851508,-23.2336802320912,
0.));
#194751=CARTESIAN_POINT('Ctrl Pts',(-7.64326080583684,-23.2103286909399,
0.));
#194752=CARTESIAN_POINT('Ctrl Pts',(-7.64502921715483,-23.1870621950452,
0.));
#194753=CARTESIAN_POINT('Ctrl Pts',(-7.64673306975797,-23.1638813796691,
0.));
#194754=CARTESIAN_POINT('Ctrl Pts',(-7.64837264482929,-23.1407868853815,
0.));
#194755=CARTESIAN_POINT('Ctrl Pts',(-7.64994822749845,-23.1177793581674,
0.));
#194756=CARTESIAN_POINT('Ctrl Pts',(-7.65146010690465,-23.0948594495246,
0.));
#194757=CARTESIAN_POINT('Ctrl Pts',(-7.65290857626357,-23.072027816555,
0.));
#194758=CARTESIAN_POINT('Ctrl Pts',(-7.65429393293955,-23.049285122053,
0.));
#194759=CARTESIAN_POINT('Ctrl Pts',(-7.65561647852555,-23.0266320345792,
0.));
#194760=CARTESIAN_POINT('Ctrl Pts',(-7.6568765189133,-23.004069228582,0.));
#194761=CARTESIAN_POINT('Ctrl Pts',(-7.65807436436453,-22.9815973845301,
0.));
#194762=CARTESIAN_POINT('Ctrl Pts',(-7.65921032958912,-22.9592171890332,
0.));
#194763=CARTESIAN_POINT('Ctrl Pts',(-7.66028473382777,-22.9369293349592,
0.));
#194764=CARTESIAN_POINT('Ctrl Pts',(-7.661297900941,-22.9147345215418,0.));
#194765=CARTESIAN_POINT('Ctrl Pts',(-7.66225015950148,-22.8926334544879,
0.));
#194766=CARTESIAN_POINT('Ctrl Pts',(-7.66314184287334,-22.870626846128,
0.));
#194767=CARTESIAN_POINT('Ctrl Pts',(-7.66397328929805,-22.8487154155569,
0.));
#194768=CARTESIAN_POINT('Ctrl Pts',(-7.66474484198553,-22.8268998887678,
0.));
#194769=CARTESIAN_POINT('Ctrl Pts',(-7.66545684920988,-22.8051809987833,
0.));
#194770=CARTESIAN_POINT('Ctrl Pts',(-7.66610966441259,-22.7835594857697,
0.));
#194771=CARTESIAN_POINT('Ctrl Pts',(-7.66670364630273,-22.7620360971839,
0.));
#194772=CARTESIAN_POINT('Ctrl Pts',(-7.66723915895413,-22.7406115879508,
0.));
#194773=CARTESIAN_POINT('Ctrl Pts',(-7.6677165719101,-22.7192867206242,
0.));
#194774=CARTESIAN_POINT('Ctrl Pts',(-7.66813626029277,-22.6980622655446,
0.));
#194775=CARTESIAN_POINT('Ctrl Pts',(-7.66849860491763,-22.6769390009889,
0.));
#194776=CARTESIAN_POINT('Ctrl Pts',(-7.66880399241354,-22.6559177133133,
0.));
#194777=CARTESIAN_POINT('Ctrl Pts',(-7.66905281533745,-22.6349991971547,
0.));
#194778=CARTESIAN_POINT('Ctrl Pts',(-7.66924547229435,-22.6141842556248,
0.));
#194779=CARTESIAN_POINT('Ctrl Pts',(-7.66938236806241,-22.5934737004955,
0.));
#194780=CARTESIAN_POINT('Ctrl Pts',(-7.66946391372299,-22.5728683523828,
0.));
#194781=CARTESIAN_POINT('Ctrl Pts',(-7.66949052679672,-22.5523690409109,
0.));
#194782=CARTESIAN_POINT('Ctrl Pts',(-7.66946263138116,-22.5319766049191,
0.));
#194783=CARTESIAN_POINT('Ctrl Pts',(-7.66938065829083,-22.5116918927023,
0.));
#194784=CARTESIAN_POINT('Ctrl Pts',(-7.66924504520302,-22.4915157622308,
0.));
#194785=CARTESIAN_POINT('Ctrl Pts',(-7.66905623680836,-22.47144908137,0.));
#194786=CARTESIAN_POINT('Ctrl Pts',(-7.6688146849666,-22.4514927280862,
0.));
#194787=CARTESIAN_POINT('Ctrl Pts',(-7.66852084886746,-22.4316475906616,
0.));
#194788=CARTESIAN_POINT('Ctrl Pts',(-7.66817519519682,-22.411914567977,
0.));
#194789=CARTESIAN_POINT('Ctrl Pts',(-7.6677781983082,-22.3922945697782,
0.));
#194790=CARTESIAN_POINT('Ctrl Pts',(-7.66733034039887,-22.3727885169361,
0.));
#194791=CARTESIAN_POINT('Ctrl Pts',(-7.66683211169134,-22.3533973417013,
0.));
#194792=CARTESIAN_POINT('Ctrl Pts',(-7.66628401061906,-22.3341219879454,
0.));
#194793=CARTESIAN_POINT('Ctrl Pts',(-7.66568654402442,-22.3149634114823,
0.));
#194794=CARTESIAN_POINT('Ctrl Pts',(-7.66504022736263,-22.2959225803925,
0.));
#194795=CARTESIAN_POINT('Ctrl Pts',(-7.66434558490973,-22.2770004753332,
0.));
#194796=CARTESIAN_POINT('Ctrl Pts',(-7.66360314997662,-22.2581980898487,
0.));
#194797=CARTESIAN_POINT('Ctrl Pts',(-7.66281346512546,-22.239516430656,
0.));
#194798=CARTESIAN_POINT('Ctrl Pts',(-7.66197708240436,-22.2209565180098,
0.));
#194799=CARTESIAN_POINT('Ctrl Pts',(-7.66109456359292,-22.2025193860972,
0.));
#194800=CARTESIAN_POINT('Ctrl Pts',(-7.66016648045008,-22.1842060834092,
0.));
#194801=CARTESIAN_POINT('Ctrl Pts',(-7.65919341496926,-22.1660176731174,
0.));
#194802=CARTESIAN_POINT('Ctrl Pts',(-7.65817595963351,-22.1479552334206,
0.));
#194803=CARTESIAN_POINT('Ctrl Pts',(-7.65711471769407,-22.1300198579671,
0.));
#194804=CARTESIAN_POINT('Ctrl Pts',(-7.65601030346819,-22.1122126563327,
0.));
#194805=CARTESIAN_POINT('Ctrl Pts',(-7.65486334263651,-22.094534754469,
0.));
#194806=CARTESIAN_POINT('Ctrl Pts',(-7.65367447254945,-22.0769872951596,
0.));
#194807=CARTESIAN_POINT('Ctrl Pts',(-7.65244434253104,-22.0595714384432,
0.));
#194808=CARTESIAN_POINT('Ctrl Pts',(-7.65117361421347,-22.0422883621176,
0.));
#194809=CARTESIAN_POINT('Ctrl Pts',(-7.64986296190157,-22.0251392623209,
0.));
#194810=CARTESIAN_POINT('Ctrl Pts',(-7.64851307293346,-22.0081253540773,
0.));
#194811=CARTESIAN_POINT('Ctrl Pts',(-7.64712464805258,-21.9912478718542,
0.));
#194812=CARTESIAN_POINT('Ctrl Pts',(-7.64569840177359,-21.97450807008,0.));
#194813=CARTESIAN_POINT('Ctrl Pts',(-7.64423506279154,-21.9579072237653,
0.));
#194814=CARTESIAN_POINT('Ctrl Pts',(-7.64273537442707,-21.9414466292074,
0.));
#194815=CARTESIAN_POINT('Ctrl Pts',(-7.6412000950654,-21.9251276046546,
0.));
#194816=CARTESIAN_POINT('Ctrl Pts',(-7.63962999860917,-21.9089514909873,
0.));
#194817=CARTESIAN_POINT('Ctrl Pts',(-7.63802587492008,-21.8929196523511,
0.));
#194818=CARTESIAN_POINT('Ctrl Pts',(-7.63638853033368,-21.8770334769492,
0.));
#194819=CARTESIAN_POINT('Ctrl Pts',(-7.63471878821204,-21.8612943779086,
0.));
#194820=CARTESIAN_POINT('Ctrl Pts',(-7.63301748948936,-21.8457037941084,
0.));
#194821=CARTESIAN_POINT('Ctrl Pts',(-7.6312854932304,-21.8302631910197,
0.));
#194822=CARTESIAN_POINT('Ctrl Pts',(-7.62952367718151,-21.8149740615093,
0.));
#194823=CARTESIAN_POINT('Ctrl Pts',(-7.62773293842409,-21.7998379268583,
0.));
#194824=CARTESIAN_POINT('Ctrl Pts',(-7.62591419404521,-21.7848563378022,
0.));
#194825=CARTESIAN_POINT('Ctrl Pts',(-7.62406838181164,-21.7700308755583,
0.));
#194826=CARTESIAN_POINT('Ctrl Pts',(-7.62219646084226,-21.7553631528329,
0.));
#194827=CARTESIAN_POINT('Ctrl Pts',(-7.62029941230855,-21.7408548148657,
0.));
#194828=CARTESIAN_POINT('Ctrl Pts',(-7.61837824030542,-21.7265075407977,
0.));
#194829=CARTESIAN_POINT('Ctrl Pts',(-7.61643397270425,-21.7123230449835,
0.));
#194830=CARTESIAN_POINT('Ctrl Pts',(-7.61446766202787,-21.6983030783321,
0.));
#194831=CARTESIAN_POINT('Ctrl Pts',(-7.61248038630265,-21.6844494295813,
0.));
#194832=CARTESIAN_POINT('Ctrl Pts',(-7.6104732500095,-21.6707639267573,
0.));
#194833=CARTESIAN_POINT('Ctrl Pts',(-7.60844738512872,-21.6572484388079,
0.));
#194834=CARTESIAN_POINT('Ctrl Pts',(-7.60640395216359,-21.6439048771743,
0.));
#194835=CARTESIAN_POINT('Ctrl Pts',(-7.604344141183,-21.6307351973823,0.));
#194836=CARTESIAN_POINT('Ctrl Pts',(-7.60226917285432,-21.6177414005991,
0.));
#194837=CARTESIAN_POINT('Ctrl Pts',(-7.60018029988238,-21.6049255358842,
0.));
#194838=CARTESIAN_POINT('Ctrl Pts',(-7.59807880846193,-21.5922897024466,
0.));
#194839=CARTESIAN_POINT('Ctrl Pts',(-7.59596601973589,-21.5798360518978,
0.));
#194840=CARTESIAN_POINT('Ctrl Pts',(-7.5938432912493,-21.5675667904728,
0.));
#194841=CARTESIAN_POINT('Ctrl Pts',(-7.59171201844793,-21.5554841813465,
0.));
#194842=CARTESIAN_POINT('Ctrl Pts',(-7.58957363620026,-21.5435905470113,
0.));
#194843=CARTESIAN_POINT('Ctrl Pts',(-7.58742962034834,-21.5318882716735,
0.));
#194844=CARTESIAN_POINT('Ctrl Pts',(-7.58528148919114,-21.5203798035294,
0.));
#194845=CARTESIAN_POINT('Ctrl Pts',(-7.58313080519159,-21.5090676573866,
0.));
#194846=CARTESIAN_POINT('Ctrl Pts',(-7.5809791779073,-21.4979544192739,
0.));
#194847=CARTESIAN_POINT('Ctrl Pts',(-7.57882826679131,-21.4870427508193,
0.));
#194848=CARTESIAN_POINT('Ctrl Pts',(-7.57667978403003,-21.4763353936766,
0.));
#194849=CARTESIAN_POINT('Ctrl Pts',(-7.57453549743435,-21.4658351740135,
0.));
#194850=CARTESIAN_POINT('Ctrl Pts',(-7.57239723223521,-21.4555450053147,
0.));
#194851=CARTESIAN_POINT('Ctrl Pts',(-7.5702668726117,-21.445467890751,0.));
#194852=CARTESIAN_POINT('Ctrl Pts',(-7.56814636360842,-21.435606926151,
0.));
#194853=CARTESIAN_POINT('Ctrl Pts',(-7.56603771218706,-21.4259653015732,
0.));
#194854=CARTESIAN_POINT('Ctrl Pts',(-7.56394299313683,-21.4165463106252,
0.));
#194855=CARTESIAN_POINT('Ctrl Pts',(-7.56186435703622,-21.4073533630364,
0.));
#194856=CARTESIAN_POINT('Ctrl Pts',(-7.55980403700615,-21.3983899952988,
0.));
#194857=CARTESIAN_POINT('Ctrl Pts',(-7.55776435731422,-21.3896598842119,
0.));
#194858=CARTESIAN_POINT('Ctrl Pts',(-7.55574773403508,-21.3811668478933,
0.));
#194859=CARTESIAN_POINT('Ctrl Pts',(-7.55375667080032,-21.3729148390244,
0.));
#194860=CARTESIAN_POINT('Ctrl Pts',(-7.55179375777442,-21.3649079431864,
0.));
#194861=CARTESIAN_POINT('Ctrl Pts',(-7.54986166521307,-21.3571503685853,
0.));
#194862=CARTESIAN_POINT('Ctrl Pts',(-7.54796316246327,-21.349646476153,
0.));
#194863=CARTESIAN_POINT('Ctrl Pts',(-7.54610114948351,-21.3424008295038,
0.));
#194864=CARTESIAN_POINT('Ctrl Pts',(-7.54427868151269,-21.3354182340149,
0.));
#194865=CARTESIAN_POINT('Ctrl Pts',(-7.54249900377032,-21.328703791771,
0.));
#194866=CARTESIAN_POINT('Ctrl Pts',(-7.5407655203828,-21.3222628524165,
0.));
#194867=CARTESIAN_POINT('Ctrl Pts',(-7.53908175169899,-21.3161009456256,
0.));
#194868=CARTESIAN_POINT('Ctrl Pts',(-7.5374512936462,-21.3102237167729,
0.));
#194869=CARTESIAN_POINT('Ctrl Pts',(-7.53587778251743,-21.3046368712156,
0.));
#194870=CARTESIAN_POINT('Ctrl Pts',(-7.53436505309949,-21.2993464250717,
0.));
#194871=CARTESIAN_POINT('Ctrl Pts',(-7.53291726078527,-21.2943588989331,
0.));
#194872=CARTESIAN_POINT('Ctrl Pts',(-7.53153906987847,-21.2896816163843,
0.));
#194873=CARTESIAN_POINT('Ctrl Pts',(-7.53023562438221,-21.2853226580658,
0.));
#194874=CARTESIAN_POINT('Ctrl Pts',(-7.52901217930407,-21.2812902781143,
0.));
#194875=CARTESIAN_POINT('Ctrl Pts',(-7.52787386225344,-21.2775925269651,
0.));
#194876=CARTESIAN_POINT('Ctrl Pts',(-7.52682526918561,-21.2742366113578,
0.));
#194877=CARTESIAN_POINT('Ctrl Pts',(-7.52587126095544,-21.2712301573465,
0.));
#194878=CARTESIAN_POINT('Ctrl Pts',(-7.52501770333522,-21.2685823838672,
0.));
#194879=CARTESIAN_POINT('Ctrl Pts',(-7.52427261074264,-21.266305915706,
0.));
#194880=CARTESIAN_POINT('Ctrl Pts',(-7.52364573027521,-21.2644161259965,
0.));
#194881=CARTESIAN_POINT('Ctrl Pts',(-7.52314642316203,-21.262927782038,
0.));
#194882=CARTESIAN_POINT('Ctrl Pts',(-7.52278182242728,-21.261852128355,
0.));
#194883=CARTESIAN_POINT('Ctrl Pts',(-7.52260064231736,-21.2613260540651,
0.));
#194884=CARTESIAN_POINT('Ctrl Pts',(-7.52252744144958,-21.261120447486,
0.));
#194885=CARTESIAN_POINT('Ctrl Pts',(-7.52250649703992,-21.2610673466883,
0.));
#194886=CARTESIAN_POINT('Ctrl Pts',(-7.52250298901266,-21.2610617890679,
0.));
#194887=CARTESIAN_POINT('',(-7.36589684767345,-24.9347862158358,0.));
#194888=CARTESIAN_POINT('Ctrl Pts',(-9.71462809124917,-20.353053841303,
0.));
#194889=CARTESIAN_POINT('Ctrl Pts',(-9.71462809124917,-20.353053841303,
12.));
#194890=CARTESIAN_POINT('Ctrl Pts',(-9.71462954053074,-20.353060251684,
0.));
#194891=CARTESIAN_POINT('Ctrl Pts',(-9.71462954053074,-20.353060251684,
12.));
#194892=CARTESIAN_POINT('Ctrl Pts',(-9.71465227853122,-20.3531126095522,
0.));
#194893=CARTESIAN_POINT('Ctrl Pts',(-9.71465227853122,-20.3531126095522,
12.));
#194894=CARTESIAN_POINT('Ctrl Pts',(-9.71474590350792,-20.3533097561886,
0.));
#194895=CARTESIAN_POINT('Ctrl Pts',(-9.71474590350792,-20.3533097561886,
12.));
#194896=CARTESIAN_POINT('Ctrl Pts',(-9.71498978052101,-20.3538098605706,
0.));
#194897=CARTESIAN_POINT('Ctrl Pts',(-9.71498978052101,-20.3538098605706,
12.));
#194898=CARTESIAN_POINT('Ctrl Pts',(-9.71549257088175,-20.3548282742361,
0.));
#194899=CARTESIAN_POINT('Ctrl Pts',(-9.71549257088175,-20.3548282742361,
12.));
#194900=CARTESIAN_POINT('Ctrl Pts',(-9.71619192554147,-20.3562337557875,
0.));
#194901=CARTESIAN_POINT('Ctrl Pts',(-9.71619192554147,-20.3562337557875,
12.));
#194902=CARTESIAN_POINT('Ctrl Pts',(-9.71708493723062,-20.3580133103357,
0.));
#194903=CARTESIAN_POINT('Ctrl Pts',(-9.71708493723062,-20.3580133103357,
12.));
#194904=CARTESIAN_POINT('Ctrl Pts',(-9.71816778327999,-20.3601498764344,
0.));
#194905=CARTESIAN_POINT('Ctrl Pts',(-9.71816778327999,-20.3601498764344,
12.));
#194906=CARTESIAN_POINT('Ctrl Pts',(-9.71943648548115,-20.362625691398,
0.));
#194907=CARTESIAN_POINT('Ctrl Pts',(-9.71943648548115,-20.362625691398,
12.));
#194908=CARTESIAN_POINT('Ctrl Pts',(-9.72088778381102,-20.3654261611055,
0.));
#194909=CARTESIAN_POINT('Ctrl Pts',(-9.72088778381102,-20.3654261611055,
12.));
#194910=CARTESIAN_POINT('Ctrl Pts',(-9.72251930722504,-20.3685406190576,
0.));
#194911=CARTESIAN_POINT('Ctrl Pts',(-9.72251930722504,-20.3685406190576,
12.));
#194912=CARTESIAN_POINT('Ctrl Pts',(-9.72432910043193,-20.371960235676,
0.));
#194913=CARTESIAN_POINT('Ctrl Pts',(-9.72432910043193,-20.371960235676,
12.));
#194914=CARTESIAN_POINT('Ctrl Pts',(-9.72631531732871,-20.3756766651952,
0.));
#194915=CARTESIAN_POINT('Ctrl Pts',(-9.72631531732871,-20.3756766651952,
12.));
#194916=CARTESIAN_POINT('Ctrl Pts',(-9.72847589116533,-20.3796805893304,
0.));
#194917=CARTESIAN_POINT('Ctrl Pts',(-9.72847589116533,-20.3796805893304,
12.));
#194918=CARTESIAN_POINT('Ctrl Pts',(-9.73080870123726,-20.3839624556742,
0.));
#194919=CARTESIAN_POINT('Ctrl Pts',(-9.73080870123726,-20.3839624556742,
12.));
#194920=CARTESIAN_POINT('Ctrl Pts',(-9.73331167102812,-20.3885129129912,
0.));
#194921=CARTESIAN_POINT('Ctrl Pts',(-9.73331167102812,-20.3885129129912,
12.));
#194922=CARTESIAN_POINT('Ctrl Pts',(-9.7359829201425,-20.3933234845646,
0.));
#194923=CARTESIAN_POINT('Ctrl Pts',(-9.7359829201425,-20.3933234845646,
12.));
#194924=CARTESIAN_POINT('Ctrl Pts',(-9.73882077613206,-20.3983866213331,
0.));
#194925=CARTESIAN_POINT('Ctrl Pts',(-9.73882077613206,-20.3983866213331,
12.));
#194926=CARTESIAN_POINT('Ctrl Pts',(-9.74182369656273,-20.4036953576549,
0.));
#194927=CARTESIAN_POINT('Ctrl Pts',(-9.74182369656273,-20.4036953576549,
12.));
#194928=CARTESIAN_POINT('Ctrl Pts',(-9.74499021838537,-20.4092430879861,
0.));
#194929=CARTESIAN_POINT('Ctrl Pts',(-9.74499021838537,-20.4092430879861,
12.));
#194930=CARTESIAN_POINT('Ctrl Pts',(-9.74831889242175,-20.4150232777393,
0.));
#194931=CARTESIAN_POINT('Ctrl Pts',(-9.74831889242175,-20.4150232777393,
12.));
#194932=CARTESIAN_POINT('Ctrl Pts',(-9.75180829786433,-20.4210295275818,
0.));
#194933=CARTESIAN_POINT('Ctrl Pts',(-9.75180829786433,-20.4210295275818,
12.));
#194934=CARTESIAN_POINT('Ctrl Pts',(-9.75545705902416,-20.4272556476629,
0.));
#194935=CARTESIAN_POINT('Ctrl Pts',(-9.75545705902416,-20.4272556476629,
12.));
#194936=CARTESIAN_POINT('Ctrl Pts',(-9.7592638628993,-20.4336957355474,
0.));
#194937=CARTESIAN_POINT('Ctrl Pts',(-9.7592638628993,-20.4336957355474,
12.));
#194938=CARTESIAN_POINT('Ctrl Pts',(-9.76322747195502,-20.4403442329401,
0.));
#194939=CARTESIAN_POINT('Ctrl Pts',(-9.76322747195502,-20.4403442329401,
12.));
#194940=CARTESIAN_POINT('Ctrl Pts',(-9.76734670980897,-20.447195862298,
0.));
#194941=CARTESIAN_POINT('Ctrl Pts',(-9.76734670980897,-20.447195862298,
12.));
#194942=CARTESIAN_POINT('Ctrl Pts',(-9.7716204510407,-20.4542455817527,
0.));
#194943=CARTESIAN_POINT('Ctrl Pts',(-9.7716204510407,-20.4542455817527,
12.));
#194944=CARTESIAN_POINT('Ctrl Pts',(-9.77604760815523,-20.4614885274973,
0.));
#194945=CARTESIAN_POINT('Ctrl Pts',(-9.77604760815523,-20.4614885274973,
12.));
#194946=CARTESIAN_POINT('Ctrl Pts',(-9.78062712373313,-20.4689199790668,
0.));
#194947=CARTESIAN_POINT('Ctrl Pts',(-9.78062712373313,-20.4689199790668,
12.));
#194948=CARTESIAN_POINT('Ctrl Pts',(-9.78535797314162,-20.4765353711585,
0.));
#194949=CARTESIAN_POINT('Ctrl Pts',(-9.78535797314162,-20.4765353711585,
12.));
#194950=CARTESIAN_POINT('Ctrl Pts',(-9.7902391649866,-20.4843302955329,
0.));
#194951=CARTESIAN_POINT('Ctrl Pts',(-9.7902391649866,-20.4843302955329,
12.));
#194952=CARTESIAN_POINT('Ctrl Pts',(-9.79526974288344,-20.4923005087945,
0.));
#194953=CARTESIAN_POINT('Ctrl Pts',(-9.79526974288344,-20.4923005087945,
12.));
#194954=CARTESIAN_POINT('Ctrl Pts',(-9.80044878520968,-20.500441931211,
0.));
#194955=CARTESIAN_POINT('Ctrl Pts',(-9.80044878520968,-20.500441931211,
12.));
#194956=CARTESIAN_POINT('Ctrl Pts',(-9.80577540161103,-20.5087506310507,
0.));
#194957=CARTESIAN_POINT('Ctrl Pts',(-9.80577540161103,-20.5087506310507,
12.));
#194958=CARTESIAN_POINT('Ctrl Pts',(-9.81124873025278,-20.5172228122839,
0.));
#194959=CARTESIAN_POINT('Ctrl Pts',(-9.81124873025278,-20.5172228122839,
12.));
#194960=CARTESIAN_POINT('Ctrl Pts',(-9.81686793455918,-20.5258548000625,
0.));
#194961=CARTESIAN_POINT('Ctrl Pts',(-9.81686793455918,-20.5258548000625,
12.));
#194962=CARTESIAN_POINT('Ctrl Pts',(-9.82263220080328,-20.534643029951,
0.));
#194963=CARTESIAN_POINT('Ctrl Pts',(-9.82263220080328,-20.534643029951,
12.));
#194964=CARTESIAN_POINT('Ctrl Pts',(-9.82854073773858,-20.5435840460717,
0.));
#194965=CARTESIAN_POINT('Ctrl Pts',(-9.82854073773858,-20.5435840460717,
12.));
#194966=CARTESIAN_POINT('Ctrl Pts',(-9.83459277585321,-20.5526744976461,
0.));
#194967=CARTESIAN_POINT('Ctrl Pts',(-9.83459277585321,-20.5526744976461,
12.));
#194968=CARTESIAN_POINT('Ctrl Pts',(-9.84078756677589,-20.5619111362406,
0.));
#194969=CARTESIAN_POINT('Ctrl Pts',(-9.84078756677589,-20.5619111362406,
12.));
#194970=CARTESIAN_POINT('Ctrl Pts',(-9.84712438256308,-20.5712908125145,
0.));
#194971=CARTESIAN_POINT('Ctrl Pts',(-9.84712438256308,-20.5712908125145,
12.));
#194972=CARTESIAN_POINT('Ctrl Pts',(-9.85360251457004,-20.580810471002,
0.));
#194973=CARTESIAN_POINT('Ctrl Pts',(-9.85360251457004,-20.580810471002,
12.));
#194974=CARTESIAN_POINT('Ctrl Pts',(-9.8602212723275,-20.5904671449754,
0.));
#194975=CARTESIAN_POINT('Ctrl Pts',(-9.8602212723275,-20.5904671449754,
12.));
#194976=CARTESIAN_POINT('Ctrl Pts',(-9.86697998242612,-20.6002579513696,
0.));
#194977=CARTESIAN_POINT('Ctrl Pts',(-9.86697998242612,-20.6002579513696,
12.));
#194978=CARTESIAN_POINT('Ctrl Pts',(-9.87387798732944,-20.6101800854491,
0.));
#194979=CARTESIAN_POINT('Ctrl Pts',(-9.87387798732944,-20.6101800854491,
12.));
#194980=CARTESIAN_POINT('Ctrl Pts',(-9.88091464472669,-20.6202308177472,
0.));
#194981=CARTESIAN_POINT('Ctrl Pts',(-9.88091464472669,-20.6202308177472,
12.));
#194982=CARTESIAN_POINT('Ctrl Pts',(-9.88808932697305,-20.6304074914086,
0.));
#194983=CARTESIAN_POINT('Ctrl Pts',(-9.88808932697305,-20.6304074914086,
12.));
#194984=CARTESIAN_POINT('Ctrl Pts',(-9.89540142049124,-20.6407075193977,
0.));
#194985=CARTESIAN_POINT('Ctrl Pts',(-9.89540142049124,-20.6407075193977,
12.));
#194986=CARTESIAN_POINT('Ctrl Pts',(-9.90285032516696,-20.6511283817415,
0.));
#194987=CARTESIAN_POINT('Ctrl Pts',(-9.90285032516696,-20.6511283817415,
12.));
#194988=CARTESIAN_POINT('Ctrl Pts',(-9.91043545377005,-20.6616676228315,
0.));
#194989=CARTESIAN_POINT('Ctrl Pts',(-9.91043545377005,-20.6616676228315,
12.));
#194990=CARTESIAN_POINT('Ctrl Pts',(-9.91815623141285,-20.6723228488261,
0.));
#194991=CARTESIAN_POINT('Ctrl Pts',(-9.91815623141285,-20.6723228488261,
12.));
#194992=CARTESIAN_POINT('Ctrl Pts',(-9.92601209498751,-20.6830917250255,
0.));
#194993=CARTESIAN_POINT('Ctrl Pts',(-9.92601209498751,-20.6830917250255,
12.));
#194994=CARTESIAN_POINT('Ctrl Pts',(-9.93400249259737,-20.6939719732485,
0.));
#194995=CARTESIAN_POINT('Ctrl Pts',(-9.93400249259737,-20.6939719732485,
12.));
#194996=CARTESIAN_POINT('Ctrl Pts',(-9.94212688298251,-20.7049613692237,
0.));
#194997=CARTESIAN_POINT('Ctrl Pts',(-9.94212688298251,-20.7049613692237,
12.));
#194998=CARTESIAN_POINT('Ctrl Pts',(-9.95038473514962,-20.716057740758,
0.));
#194999=CARTESIAN_POINT('Ctrl Pts',(-9.95038473514962,-20.716057740758,
12.));
#195000=CARTESIAN_POINT('Ctrl Pts',(-9.95877552798403,-20.7272589658752,
0.));
#195001=CARTESIAN_POINT('Ctrl Pts',(-9.95877552798403,-20.7272589658752,
12.));
#195002=CARTESIAN_POINT('Ctrl Pts',(-9.96729874986199,-20.7385629709795,
0.));
#195003=CARTESIAN_POINT('Ctrl Pts',(-9.96729874986199,-20.7385629709795,
12.));
#195004=CARTESIAN_POINT('Ctrl Pts',(-9.97595389823461,-20.7499677289625,
0.));
#195005=CARTESIAN_POINT('Ctrl Pts',(-9.97595389823461,-20.7499677289625,
12.));
#195006=CARTESIAN_POINT('Ctrl Pts',(-9.98474047926846,-20.7614712574989,
0.));
#195007=CARTESIAN_POINT('Ctrl Pts',(-9.98474047926846,-20.7614712574989,
12.));
#195008=CARTESIAN_POINT('Ctrl Pts',(-9.99365800754638,-20.7730716175417,
0.));
#195009=CARTESIAN_POINT('Ctrl Pts',(-9.99365800754638,-20.7730716175417,
12.));
#195010=CARTESIAN_POINT('Ctrl Pts',(-10.0027060057389,-20.7847669117568,
0.));
#195011=CARTESIAN_POINT('Ctrl Pts',(-10.0027060057389,-20.7847669117568,
12.));
#195012=CARTESIAN_POINT('Ctrl Pts',(-10.0118840042786,-20.7965552829907,
0.));
#195013=CARTESIAN_POINT('Ctrl Pts',(-10.0118840042786,-20.7965552829907,
12.));
#195014=CARTESIAN_POINT('Ctrl Pts',(-10.0211915410095,-20.8084349126885,
0.));
#195015=CARTESIAN_POINT('Ctrl Pts',(-10.0211915410095,-20.8084349126885,
12.));
#195016=CARTESIAN_POINT('Ctrl Pts',(-10.0306281609435,-20.8204040196599,
0.));
#195017=CARTESIAN_POINT('Ctrl Pts',(-10.0306281609435,-20.8204040196599,
12.));
#195018=CARTESIAN_POINT('Ctrl Pts',(-10.0401934160234,-20.8324608588906,
0.));
#195019=CARTESIAN_POINT('Ctrl Pts',(-10.0401934160234,-20.8324608588906,
12.));
#195020=CARTESIAN_POINT('Ctrl Pts',(-10.0498868648733,-20.8446037203402,
0.));
#195021=CARTESIAN_POINT('Ctrl Pts',(-10.0498868648733,-20.8446037203402,
12.));
#195022=CARTESIAN_POINT('Ctrl Pts',(-10.0597080725375,-20.856830927732,
0.));
#195023=CARTESIAN_POINT('Ctrl Pts',(-10.0597080725375,-20.856830927732,
12.));
#195024=CARTESIAN_POINT('Ctrl Pts',(-10.0696566102219,-20.8691408373705,
0.));
#195025=CARTESIAN_POINT('Ctrl Pts',(-10.0696566102219,-20.8691408373705,
12.));
#195026=CARTESIAN_POINT('Ctrl Pts',(-10.0797320551154,-20.8815318371844,
0.));
#195027=CARTESIAN_POINT('Ctrl Pts',(-10.0797320551154,-20.8815318371844,
12.));
#195028=CARTESIAN_POINT('Ctrl Pts',(-10.0899339901916,-20.8940023457371,
0.));
#195029=CARTESIAN_POINT('Ctrl Pts',(-10.0899339901916,-20.8940023457371,
12.));
#195030=CARTESIAN_POINT('Ctrl Pts',(-10.1002620040076,-20.9065508112556,
0.));
#195031=CARTESIAN_POINT('Ctrl Pts',(-10.1002620040076,-20.9065508112556,
12.));
#195032=CARTESIAN_POINT('Ctrl Pts',(-10.1107156904836,-20.9191757106266,
0.));
#195033=CARTESIAN_POINT('Ctrl Pts',(-10.1107156904836,-20.9191757106266,
12.));
#195034=CARTESIAN_POINT('Ctrl Pts',(-10.1212946487057,-20.931875548473,
0.));
#195035=CARTESIAN_POINT('Ctrl Pts',(-10.1212946487057,-20.931875548473,
12.));
#195036=CARTESIAN_POINT('Ctrl Pts',(-10.1319984827909,-20.944648856393,
0.));
#195037=CARTESIAN_POINT('Ctrl Pts',(-10.1319984827909,-20.944648856393,
12.));
#195038=CARTESIAN_POINT('Ctrl Pts',(-10.1428268017257,-20.9574941921591,
0.));
#195039=CARTESIAN_POINT('Ctrl Pts',(-10.1428268017257,-20.9574941921591,
12.));
#195040=CARTESIAN_POINT('Ctrl Pts',(-10.1537792192065,-20.970410138937,
0.));
#195041=CARTESIAN_POINT('Ctrl Pts',(-10.1537792192065,-20.970410138937,
12.));
#195042=CARTESIAN_POINT('Ctrl Pts',(-10.1648553534567,-20.9833953044736,
0.));
#195043=CARTESIAN_POINT('Ctrl Pts',(-10.1648553534567,-20.9833953044736,
12.));
#195044=CARTESIAN_POINT('Ctrl Pts',(-10.1760548270765,-20.9964483203685,
0.));
#195045=CARTESIAN_POINT('Ctrl Pts',(-10.1760548270765,-20.9964483203685,
12.));
#195046=CARTESIAN_POINT('Ctrl Pts',(-10.1873772669358,-21.0095678414486,
0.));
#195047=CARTESIAN_POINT('Ctrl Pts',(-10.1873772669358,-21.0095678414486,
12.));
#195048=CARTESIAN_POINT('Ctrl Pts',(-10.1988223040425,-21.0227525451107,
0.));
#195049=CARTESIAN_POINT('Ctrl Pts',(-10.1988223040425,-21.0227525451107,
12.));
#195050=CARTESIAN_POINT('Ctrl Pts',(-10.2103895734124,-21.0360011306814,
0.));
#195051=CARTESIAN_POINT('Ctrl Pts',(-10.2103895734124,-21.0360011306814,
12.));
#195052=CARTESIAN_POINT('Ctrl Pts',(-10.2220787139157,-21.0493123187483,
0.));
#195053=CARTESIAN_POINT('Ctrl Pts',(-10.2220787139157,-21.0493123187483,
12.));
#195054=CARTESIAN_POINT('Ctrl Pts',(-10.233889368157,-21.0626848505665,
0.));
#195055=CARTESIAN_POINT('Ctrl Pts',(-10.233889368157,-21.0626848505665,
12.));
#195056=CARTESIAN_POINT('Ctrl Pts',(-10.2458211823915,-21.0761174875448,
0.));
#195057=CARTESIAN_POINT('Ctrl Pts',(-10.2458211823915,-21.0761174875448,
12.));
#195058=CARTESIAN_POINT('Ctrl Pts',(-10.2578738064183,-21.0896090107066,
0.));
#195059=CARTESIAN_POINT('Ctrl Pts',(-10.2578738064183,-21.0896090107066,
12.));
#195060=CARTESIAN_POINT('Ctrl Pts',(-10.2700468934743,-21.1031582201625,
0.));
#195061=CARTESIAN_POINT('Ctrl Pts',(-10.2700468934743,-21.1031582201625,
12.));
#195062=CARTESIAN_POINT('Ctrl Pts',(-10.2823401001067,-21.1167639345623,
0.));
#195063=CARTESIAN_POINT('Ctrl Pts',(-10.2823401001067,-21.1167639345623,
12.));
#195064=CARTESIAN_POINT('Ctrl Pts',(-10.2947530860714,-21.130424990599,
0.));
#195065=CARTESIAN_POINT('Ctrl Pts',(-10.2947530860714,-21.130424990599,
12.));
#195066=CARTESIAN_POINT('Ctrl Pts',(-10.307285514268,-21.1441402425831,
0.));
#195067=CARTESIAN_POINT('Ctrl Pts',(-10.307285514268,-21.1441402425831,
12.));
#195068=CARTESIAN_POINT('Ctrl Pts',(-10.3199370506541,-21.1579085619959,
0.));
#195069=CARTESIAN_POINT('Ctrl Pts',(-10.3199370506541,-21.1579085619959,
12.));
#195070=CARTESIAN_POINT('Ctrl Pts',(-10.3327073641574,-21.1717288370512,
0.));
#195071=CARTESIAN_POINT('Ctrl Pts',(-10.3327073641574,-21.1717288370512,
12.));
#195072=CARTESIAN_POINT('Ctrl Pts',(-10.3455961265706,-21.1855999722427,
0.));
#195073=CARTESIAN_POINT('Ctrl Pts',(-10.3455961265706,-21.1855999722427,
12.));
#195074=CARTESIAN_POINT('Ctrl Pts',(-10.3586030124595,-21.1995208879205,
0.));
#195075=CARTESIAN_POINT('Ctrl Pts',(-10.3586030124595,-21.1995208879205,
12.));
#195076=CARTESIAN_POINT('Ctrl Pts',(-10.3717276991137,-21.2134905199359,
0.));
#195077=CARTESIAN_POINT('Ctrl Pts',(-10.3717276991137,-21.2134905199359,
12.));
#195078=CARTESIAN_POINT('Ctrl Pts',(-10.384969866479,-21.2275078192708,
0.));
#195079=CARTESIAN_POINT('Ctrl Pts',(-10.384969866479,-21.2275078192708,
12.));
#195080=CARTESIAN_POINT('Ctrl Pts',(-10.3983291970846,-21.2415717516713,
0.));
#195081=CARTESIAN_POINT('Ctrl Pts',(-10.3983291970846,-21.2415717516713,
12.));
#195082=CARTESIAN_POINT('Ctrl Pts',(-10.4118053759584,-21.2556812972741,
0.));
#195083=CARTESIAN_POINT('Ctrl Pts',(-10.4118053759584,-21.2556812972741,
12.));
#195084=CARTESIAN_POINT('Ctrl Pts',(-10.4253980905394,-21.2698354502391,
0.));
#195085=CARTESIAN_POINT('Ctrl Pts',(-10.4253980905394,-21.2698354502391,
12.));
#195086=CARTESIAN_POINT('Ctrl Pts',(-10.4391070306385,-21.2840332184471,
0.));
#195087=CARTESIAN_POINT('Ctrl Pts',(-10.4391070306385,-21.2840332184471,
12.));
#195088=CARTESIAN_POINT('Ctrl Pts',(-10.452931888387,-21.2982736231924,
0.));
#195089=CARTESIAN_POINT('Ctrl Pts',(-10.452931888387,-21.2982736231924,
12.));
#195090=CARTESIAN_POINT('Ctrl Pts',(-10.4668723581768,-21.312555698873,
0.));
#195091=CARTESIAN_POINT('Ctrl Pts',(-10.4668723581768,-21.312555698873,
12.));
#195092=CARTESIAN_POINT('Ctrl Pts',(-10.4809281365933,-21.3268784926823,
0.));
#195093=CARTESIAN_POINT('Ctrl Pts',(-10.4809281365933,-21.3268784926823,
12.));
#195094=CARTESIAN_POINT('Ctrl Pts',(-10.4950989223341,-21.3412410642912,
0.));
#195095=CARTESIAN_POINT('Ctrl Pts',(-10.4950989223341,-21.3412410642912,
12.));
#195096=CARTESIAN_POINT('Ctrl Pts',(-10.509384416169,-21.3556424855822,
0.));
#195097=CARTESIAN_POINT('Ctrl Pts',(-10.509384416169,-21.3556424855822,
12.));
#195098=CARTESIAN_POINT('Ctrl Pts',(-10.523784320906,-21.3700818403942,
0.));
#195099=CARTESIAN_POINT('Ctrl Pts',(-10.523784320906,-21.3700818403942,
12.));
#195100=CARTESIAN_POINT('Ctrl Pts',(-10.5382983413422,-21.3845582242604,
0.));
#195101=CARTESIAN_POINT('Ctrl Pts',(-10.5382983413422,-21.3845582242604,
12.));
#195102=CARTESIAN_POINT('Ctrl Pts',(-10.5529261842107,-21.3990707441495,
0.));
#195103=CARTESIAN_POINT('Ctrl Pts',(-10.5529261842107,-21.3990707441495,
12.));
#195104=CARTESIAN_POINT('Ctrl Pts',(-10.5676675581106,-21.4136185181974,
0.));
#195105=CARTESIAN_POINT('Ctrl Pts',(-10.5676675581106,-21.4136185181974,
12.));
#195106=CARTESIAN_POINT('Ctrl Pts',(-10.582522173457,-21.4282006754624,
0.));
#195107=CARTESIAN_POINT('Ctrl Pts',(-10.582522173457,-21.4282006754624,
12.));
#195108=CARTESIAN_POINT('Ctrl Pts',(-10.597489742462,-21.4428163557137,
0.));
#195109=CARTESIAN_POINT('Ctrl Pts',(-10.597489742462,-21.4428163557137,
12.));
#195110=CARTESIAN_POINT('Ctrl Pts',(-10.612569979096,-21.4574647092093,
0.));
#195111=CARTESIAN_POINT('Ctrl Pts',(-10.612569979096,-21.4574647092093,
12.));
#195112=CARTESIAN_POINT('Ctrl Pts',(-10.6277625990457,-21.4721448964766,
0.));
#195113=CARTESIAN_POINT('Ctrl Pts',(-10.6277625990457,-21.4721448964766,
12.));
#195114=CARTESIAN_POINT('Ctrl Pts',(-10.6430673196609,-21.4868560880893,
0.));
#195115=CARTESIAN_POINT('Ctrl Pts',(-10.6430673196609,-21.4868560880893,
12.));
#195116=CARTESIAN_POINT('Ctrl Pts',(-10.6584838598941,-21.5015974644454,
0.));
#195117=CARTESIAN_POINT('Ctrl Pts',(-10.6584838598941,-21.5015974644454,
12.));
#195118=CARTESIAN_POINT('Ctrl Pts',(-10.6740119402835,-21.5163682155805,
0.));
#195119=CARTESIAN_POINT('Ctrl Pts',(-10.6740119402835,-21.5163682155805,
12.));
#195120=CARTESIAN_POINT('Ctrl Pts',(-10.689651282929,-21.531167540981,0.));
#195121=CARTESIAN_POINT('Ctrl Pts',(-10.689651282929,-21.531167540981,12.));
#195122=CARTESIAN_POINT('Ctrl Pts',(-10.7054016114571,-21.5459946493955,
0.));
#195123=CARTESIAN_POINT('Ctrl Pts',(-10.7054016114571,-21.5459946493955,
12.));
#195124=CARTESIAN_POINT('Ctrl Pts',(-10.7212626509816,-21.5608487586467,
0.));
#195125=CARTESIAN_POINT('Ctrl Pts',(-10.7212626509816,-21.5608487586467,
12.));
#195126=CARTESIAN_POINT('Ctrl Pts',(-10.7372341280468,-21.5757290954372,
0.));
#195127=CARTESIAN_POINT('Ctrl Pts',(-10.7372341280468,-21.5757290954372,
12.));
#195128=CARTESIAN_POINT('Ctrl Pts',(-10.7533157705943,-21.5906348951745,
0.));
#195129=CARTESIAN_POINT('Ctrl Pts',(-10.7533157705943,-21.5906348951745,
12.));
#195130=CARTESIAN_POINT('Ctrl Pts',(-10.7695073079554,-21.6055654018179,
0.));
#195131=CARTESIAN_POINT('Ctrl Pts',(-10.7695073079554,-21.6055654018179,
12.));
#195132=CARTESIAN_POINT('Ctrl Pts',(-10.7858084708262,-21.6205198677176,
0.));
#195133=CARTESIAN_POINT('Ctrl Pts',(-10.7858084708262,-21.6205198677176,
12.));
#195134=CARTESIAN_POINT('Ctrl Pts',(-10.802218991237,-21.6354975534557,
0.));
#195135=CARTESIAN_POINT('Ctrl Pts',(-10.802218991237,-21.6354975534557,
12.));
#195136=CARTESIAN_POINT('Ctrl Pts',(-10.8187386025135,-21.6504977276864,
0.));
#195137=CARTESIAN_POINT('Ctrl Pts',(-10.8187386025135,-21.6504977276864,
12.));
#195138=CARTESIAN_POINT('Ctrl Pts',(-10.835367039227,-21.6655196669727,
0.));
#195139=CARTESIAN_POINT('Ctrl Pts',(-10.835367039227,-21.6655196669727,
12.));
#195140=CARTESIAN_POINT('Ctrl Pts',(-10.8521040371832,-21.6805626556461,
0.));
#195141=CARTESIAN_POINT('Ctrl Pts',(-10.8521040371832,-21.6805626556461,
12.));
#195142=CARTESIAN_POINT('Ctrl Pts',(-10.8689493334093,-21.6956259856667,
0.));
#195143=CARTESIAN_POINT('Ctrl Pts',(-10.8689493334093,-21.6956259856667,
12.));
#195144=CARTESIAN_POINT('Ctrl Pts',(-10.8859026661292,-21.7107089564822,
0.));
#195145=CARTESIAN_POINT('Ctrl Pts',(-10.8859026661292,-21.7107089564822,
12.));
#195146=CARTESIAN_POINT('Ctrl Pts',(-10.9029637747341,-21.7258108748874,
0.));
#195147=CARTESIAN_POINT('Ctrl Pts',(-10.9029637747341,-21.7258108748874,
12.));
#195148=CARTESIAN_POINT('Ctrl Pts',(-10.9201323997386,-21.74093105488,0.));
#195149=CARTESIAN_POINT('Ctrl Pts',(-10.9201323997386,-21.74093105488,12.));
#195150=CARTESIAN_POINT('Ctrl Pts',(-10.9374082827446,-21.7560688175252,
0.));
#195151=CARTESIAN_POINT('Ctrl Pts',(-10.9374082827446,-21.7560688175252,
12.));
#195152=CARTESIAN_POINT('Ctrl Pts',(-10.9547911664457,-21.7712234908468,
0.));
#195153=CARTESIAN_POINT('Ctrl Pts',(-10.9547911664457,-21.7712234908468,
12.));
#195154=CARTESIAN_POINT('Ctrl Pts',(-10.9722807946157,-21.7863944097143,
0.));
#195155=CARTESIAN_POINT('Ctrl Pts',(-10.9722807946157,-21.7863944097143,
12.));
#195156=CARTESIAN_POINT('Ctrl Pts',(-10.9898769120913,-21.8015809157302,
0.));
#195157=CARTESIAN_POINT('Ctrl Pts',(-10.9898769120913,-21.8015809157302,
12.));
#195158=CARTESIAN_POINT('Ctrl Pts',(-11.0075792647477,-21.8167823571168,
0.));
#195159=CARTESIAN_POINT('Ctrl Pts',(-11.0075792647477,-21.8167823571168,
12.));
#195160=CARTESIAN_POINT('Ctrl Pts',(-11.0253875994598,-21.8319980886033,
0.));
#195161=CARTESIAN_POINT('Ctrl Pts',(-11.0253875994598,-21.8319980886033,
12.));
#195162=CARTESIAN_POINT('Ctrl Pts',(-11.0433016640808,-21.8472274713103,
0.));
#195163=CARTESIAN_POINT('Ctrl Pts',(-11.0433016640808,-21.8472274713103,
12.));
#195164=CARTESIAN_POINT('Ctrl Pts',(-11.0613212074364,-21.8624698726319,
0.));
#195165=CARTESIAN_POINT('Ctrl Pts',(-11.0613212074364,-21.8624698726319,
12.));
#195166=CARTESIAN_POINT('Ctrl Pts',(-11.0794459793058,-21.8777246661191,
0.));
#195167=CARTESIAN_POINT('Ctrl Pts',(-11.0794459793058,-21.8777246661191,
12.));
#195168=CARTESIAN_POINT('Ctrl Pts',(-11.0976757303944,-21.8929912313608,
0.));
#195169=CARTESIAN_POINT('Ctrl Pts',(-11.0976757303944,-21.8929912313608,
12.));
#195170=CARTESIAN_POINT('Ctrl Pts',(-11.1160102123024,-21.9082689538687,
0.));
#195171=CARTESIAN_POINT('Ctrl Pts',(-11.1160102123024,-21.9082689538687,
12.));
#195172=CARTESIAN_POINT('Ctrl Pts',(-11.134449177474,-21.9235572249518,
0.));
#195173=CARTESIAN_POINT('Ctrl Pts',(-11.134449177474,-21.9235572249518,
12.));
#195174=CARTESIAN_POINT('Ctrl Pts',(-11.1529923792002,-21.9388554416437,
0.));
#195175=CARTESIAN_POINT('Ctrl Pts',(-11.1529923792002,-21.9388554416437,
12.));
#195176=CARTESIAN_POINT('Ctrl Pts',(-11.1716395716375,-21.9541630066504,
0.));
#195177=CARTESIAN_POINT('Ctrl Pts',(-11.1716395716375,-21.9541630066504,
12.));
#195178=CARTESIAN_POINT('Ctrl Pts',(-11.190390509811,-21.9694793282913,
0.));
#195179=CARTESIAN_POINT('Ctrl Pts',(-11.190390509811,-21.9694793282913,
12.));
#195180=CARTESIAN_POINT('Ctrl Pts',(-11.2092449496125,-21.9848038204439,
0.));
#195181=CARTESIAN_POINT('Ctrl Pts',(-11.2092449496125,-21.9848038204439,
12.));
#195182=CARTESIAN_POINT('Ctrl Pts',(-11.2282026477897,-22.0001359024839,
0.));
#195183=CARTESIAN_POINT('Ctrl Pts',(-11.2282026477897,-22.0001359024839,
12.));
#195184=CARTESIAN_POINT('Ctrl Pts',(-11.2472633619276,-22.0154749992364,
0.));
#195185=CARTESIAN_POINT('Ctrl Pts',(-11.2472633619276,-22.0154749992364,
12.));
#195186=CARTESIAN_POINT('Ctrl Pts',(-11.2664268504207,-22.0308205408351,
0.));
#195187=CARTESIAN_POINT('Ctrl Pts',(-11.2664268504207,-22.0308205408351,
12.));
#195188=CARTESIAN_POINT('Ctrl Pts',(-11.2856928724374,-22.046171962566,
0.));
#195189=CARTESIAN_POINT('Ctrl Pts',(-11.2856928724374,-22.046171962566,
12.));
#195190=CARTESIAN_POINT('Ctrl Pts',(-11.3050611878771,-22.0615287047179,
0.));
#195191=CARTESIAN_POINT('Ctrl Pts',(-11.3050611878771,-22.0615287047179,
12.));
#195192=CARTESIAN_POINT('Ctrl Pts',(-11.3245315573168,-22.0768902124267,
0.));
#195193=CARTESIAN_POINT('Ctrl Pts',(-11.3245315573168,-22.0768902124267,
12.));
#195194=CARTESIAN_POINT('Ctrl Pts',(-11.3441037419553,-22.0922559355293,
0.));
#195195=CARTESIAN_POINT('Ctrl Pts',(-11.3441037419553,-22.0922559355293,
12.));
#195196=CARTESIAN_POINT('Ctrl Pts',(-11.3637775035367,-22.1076253283978,
0.));
#195197=CARTESIAN_POINT('Ctrl Pts',(-11.3637775035367,-22.1076253283978,
12.));
#195198=CARTESIAN_POINT('Ctrl Pts',(-11.3835526044256,-22.1229978500185,
0.));
#195199=CARTESIAN_POINT('Ctrl Pts',(-11.3835526044256,-22.1229978500185,
12.));
#195200=CARTESIAN_POINT('Ctrl Pts',(-11.4034288076909,-22.1383729640963,
0.));
#195201=CARTESIAN_POINT('Ctrl Pts',(-11.4034288076909,-22.1383729640963,
12.));
#195202=CARTESIAN_POINT('Ctrl Pts',(-11.4234058771742,-22.1537501391486,
0.));
#195203=CARTESIAN_POINT('Ctrl Pts',(-11.4234058771742,-22.1537501391486,
12.));
#195204=CARTESIAN_POINT('Ctrl Pts',(-11.443483577557,-22.1691288486096,
0.));
#195205=CARTESIAN_POINT('Ctrl Pts',(-11.443483577557,-22.1691288486096,
12.));
#195206=CARTESIAN_POINT('Ctrl Pts',(-11.463661674411,-22.1845085709169,
0.));
#195207=CARTESIAN_POINT('Ctrl Pts',(-11.463661674411,-22.1845085709169,
12.));
#195208=CARTESIAN_POINT('Ctrl Pts',(-11.4839399342589,-22.1998887896435,
0.));
#195209=CARTESIAN_POINT('Ctrl Pts',(-11.4839399342589,-22.1998887896435,
12.));
#195210=CARTESIAN_POINT('Ctrl Pts',(-11.504318124424,-22.215268993102,0.));
#195211=CARTESIAN_POINT('Ctrl Pts',(-11.504318124424,-22.215268993102,12.));
#195212=CARTESIAN_POINT('Ctrl Pts',(-11.5247960128476,-22.2306486738899,
0.));
#195213=CARTESIAN_POINT('Ctrl Pts',(-11.5247960128476,-22.2306486738899,
12.));
#195214=CARTESIAN_POINT('Ctrl Pts',(-11.545373367912,-22.2460273284653,
0.));
#195215=CARTESIAN_POINT('Ctrl Pts',(-11.545373367912,-22.2460273284653,
12.));
#195216=CARTESIAN_POINT('Ctrl Pts',(-11.5660499582403,-22.2614044566898,
0.));
#195217=CARTESIAN_POINT('Ctrl Pts',(-11.5660499582403,-22.2614044566898,
12.));
#195218=CARTESIAN_POINT('Ctrl Pts',(-11.5868255525189,-22.2767795614349,
0.));
#195219=CARTESIAN_POINT('Ctrl Pts',(-11.5868255525189,-22.2767795614349,
12.));
#195220=CARTESIAN_POINT('Ctrl Pts',(-11.6076999192359,-22.2921521480357,
0.));
#195221=CARTESIAN_POINT('Ctrl Pts',(-11.6076999192359,-22.2921521480357,
12.));
#195222=CARTESIAN_POINT('Ctrl Pts',(-11.6286728270011,-22.3075217249049,
0.));
#195223=CARTESIAN_POINT('Ctrl Pts',(-11.6286728270011,-22.3075217249049,
12.));
#195224=CARTESIAN_POINT('Ctrl Pts',(-11.6497440449858,-22.3228878043976,
0.));
#195225=CARTESIAN_POINT('Ctrl Pts',(-11.6497440449858,-22.3228878043976,
12.));
#195226=CARTESIAN_POINT('Ctrl Pts',(-11.6709133432986,-22.3382499035618,
0.));
#195227=CARTESIAN_POINT('Ctrl Pts',(-11.6709133432986,-22.3382499035618,
12.));
#195228=CARTESIAN_POINT('Ctrl Pts',(-11.6921804934056,-22.3536075450028,
0.));
#195229=CARTESIAN_POINT('Ctrl Pts',(-11.6921804934056,-22.3536075450028,
12.));
#195230=CARTESIAN_POINT('Ctrl Pts',(-11.7135452684532,-22.3689602575492,
0.));
#195231=CARTESIAN_POINT('Ctrl Pts',(-11.7135452684532,-22.3689602575492,
12.));
#195232=CARTESIAN_POINT('Ctrl Pts',(-11.7350074437961,-22.3843075773905,
0.));
#195233=CARTESIAN_POINT('Ctrl Pts',(-11.7350074437961,-22.3843075773905,
12.));
#195234=CARTESIAN_POINT('Ctrl Pts',(-11.7565667964765,-22.39964904692,0.));
#195235=CARTESIAN_POINT('Ctrl Pts',(-11.7565667964765,-22.39964904692,12.));
#195236=CARTESIAN_POINT('Ctrl Pts',(-11.7782231042041,-22.4149842125018,
0.));
#195237=CARTESIAN_POINT('Ctrl Pts',(-11.7782231042041,-22.4149842125018,
12.));
#195238=CARTESIAN_POINT('Ctrl Pts',(-11.7999761445175,-22.4303126226468,
0.));
#195239=CARTESIAN_POINT('Ctrl Pts',(-11.7999761445175,-22.4303126226468,
12.));
#195240=CARTESIAN_POINT('Ctrl Pts',(-11.8218256937889,-22.4456338258738,
0.));
#195241=CARTESIAN_POINT('Ctrl Pts',(-11.8218256937889,-22.4456338258738,
12.));
#195242=CARTESIAN_POINT('Ctrl Pts',(-11.8437715264487,-22.4609473690469,
0.));
#195243=CARTESIAN_POINT('Ctrl Pts',(-11.8437715264487,-22.4609473690469,
12.));
#195244=CARTESIAN_POINT('Ctrl Pts',(-11.8658134137018,-22.4762527946694,
0.));
#195245=CARTESIAN_POINT('Ctrl Pts',(-11.8658134137018,-22.4762527946694,
12.));
#195246=CARTESIAN_POINT('Ctrl Pts',(-11.8879511239941,-22.4915496418472,
0.));
#195247=CARTESIAN_POINT('Ctrl Pts',(-11.8879511239941,-22.4915496418472,
12.));
#195248=CARTESIAN_POINT('Ctrl Pts',(-11.9101844254555,-22.5068374513958,
0.));
#195249=CARTESIAN_POINT('Ctrl Pts',(-11.9101844254555,-22.5068374513958,
12.));
#195250=CARTESIAN_POINT('Ctrl Pts',(-11.9325130877801,-22.5221157697869,
0.));
#195251=CARTESIAN_POINT('Ctrl Pts',(-11.9325130877801,-22.5221157697869,
12.));
#195252=CARTESIAN_POINT('Ctrl Pts',(-11.9549368843996,-22.5373841537299,
0.));
#195253=CARTESIAN_POINT('Ctrl Pts',(-11.9549368843996,-22.5373841537299,
12.));
#195254=CARTESIAN_POINT('Ctrl Pts',(-11.9774555943496,-22.5526421741159,
0.));
#195255=CARTESIAN_POINT('Ctrl Pts',(-11.9774555943496,-22.5526421741159,
12.));
#195256=CARTESIAN_POINT('Ctrl Pts',(-12.0000690046697,-22.5678894211194,
0.));
#195257=CARTESIAN_POINT('Ctrl Pts',(-12.0000690046697,-22.5678894211194,
12.));
#195258=CARTESIAN_POINT('Ctrl Pts',(-12.0227769113132,-22.5831255061306,
0.));
#195259=CARTESIAN_POINT('Ctrl Pts',(-12.0227769113132,-22.5831255061306,
12.));
#195260=CARTESIAN_POINT('Ctrl Pts',(-12.0455791139135,-22.5983500505675,
0.));
#195261=CARTESIAN_POINT('Ctrl Pts',(-12.0455791139135,-22.5983500505675,
12.));
#195262=CARTESIAN_POINT('Ctrl Pts',(-12.0684754113869,-22.613562676493,
0.));
#195263=CARTESIAN_POINT('Ctrl Pts',(-12.0684754113869,-22.613562676493,
12.));
#195264=CARTESIAN_POINT('Ctrl Pts',(-12.0914655972828,-22.628762996708,
0.));
#195265=CARTESIAN_POINT('Ctrl Pts',(-12.0914655972828,-22.628762996708,
12.));
#195266=CARTESIAN_POINT('Ctrl Pts',(-12.1145494550384,-22.6439506046611,
0.));
#195267=CARTESIAN_POINT('Ctrl Pts',(-12.1145494550384,-22.6439506046611,
12.));
#195268=CARTESIAN_POINT('Ctrl Pts',(-12.1377267537141,-22.6591250653942,
0.));
#195269=CARTESIAN_POINT('Ctrl Pts',(-12.1377267537141,-22.6591250653942,
12.));
#195270=CARTESIAN_POINT('Ctrl Pts',(-12.1609972423089,-22.6742859034891,
0.));
#195271=CARTESIAN_POINT('Ctrl Pts',(-12.1609972423089,-22.6742859034891,
12.));
#195272=CARTESIAN_POINT('Ctrl Pts',(-12.1843606579246,-22.6894326204959,
0.));
#195273=CARTESIAN_POINT('Ctrl Pts',(-12.1843606579246,-22.6894326204959,
12.));
#195274=CARTESIAN_POINT('Ctrl Pts',(-12.2078167360267,-22.7045647168659,
0.));
#195275=CARTESIAN_POINT('Ctrl Pts',(-12.2078167360267,-22.7045647168659,
12.));
#195276=CARTESIAN_POINT('Ctrl Pts',(-12.2313652198047,-22.7196817119299,
0.));
#195277=CARTESIAN_POINT('Ctrl Pts',(-12.2313652198047,-22.7196817119299,
12.));
#195278=CARTESIAN_POINT('Ctrl Pts',(-12.2550058702389,-22.7347831655251,
0.));
#195279=CARTESIAN_POINT('Ctrl Pts',(-12.2550058702389,-22.7347831655251,
12.));
#195280=CARTESIAN_POINT('Ctrl Pts',(-12.2787384750747,-22.7498686970096,
0.));
#195281=CARTESIAN_POINT('Ctrl Pts',(-12.2787384750747,-22.7498686970096,
12.));
#195282=CARTESIAN_POINT('Ctrl Pts',(-12.3025628601812,-22.7649380101154,
0.));
#195283=CARTESIAN_POINT('Ctrl Pts',(-12.3025628601812,-22.7649380101154,
12.));
#195284=CARTESIAN_POINT('Ctrl Pts',(-12.3264788926108,-22.7799908974947,
0.));
#195285=CARTESIAN_POINT('Ctrl Pts',(-12.3264788926108,-22.7799908974947,
12.));
#195286=CARTESIAN_POINT('Ctrl Pts',(-12.3504864740361,-22.7950272216959,
0.));
#195287=CARTESIAN_POINT('Ctrl Pts',(-12.3504864740361,-22.7950272216959,
12.));
#195288=CARTESIAN_POINT('Ctrl Pts',(-12.3745855366772,-22.8100469022632,
0.));
#195289=CARTESIAN_POINT('Ctrl Pts',(-12.3745855366772,-22.8100469022632,
12.));
#195290=CARTESIAN_POINT('Ctrl Pts',(-12.393937937903,-22.8220493007353,
0.));
#195291=CARTESIAN_POINT('Ctrl Pts',(-12.393937937903,-22.8220493007353,
12.));
#195292=CARTESIAN_POINT('Ctrl Pts',(-12.4084933766366,-22.8310435872852,
0.));
#195293=CARTESIAN_POINT('Ctrl Pts',(-12.4084933766366,-22.8310435872852,
12.));
#195294=CARTESIAN_POINT('Ctrl Pts',(-12.4182152851867,-22.8370364396497,
0.));
#195295=CARTESIAN_POINT('Ctrl Pts',(-12.4182152851867,-22.8370364396497,
12.));
#195296=CARTESIAN_POINT('Ctrl Pts',(-12.4230808101438,-22.8400320311648,
0.));
#195297=CARTESIAN_POINT('Ctrl Pts',(-12.4230808101438,-22.8400320311648,
12.));
#195298=CARTESIAN_POINT('',(-12.4230808101438,-22.8400320311648,0.));
#195299=CARTESIAN_POINT('Ctrl Pts',(-9.71462809124917,-20.353053841303,
0.));
#195300=CARTESIAN_POINT('Ctrl Pts',(-9.71462954053074,-20.353060251684,
0.));
#195301=CARTESIAN_POINT('Ctrl Pts',(-9.71465227853122,-20.3531126095522,
0.));
#195302=CARTESIAN_POINT('Ctrl Pts',(-9.71474590350792,-20.3533097561886,
0.));
#195303=CARTESIAN_POINT('Ctrl Pts',(-9.71498978052101,-20.3538098605706,
0.));
#195304=CARTESIAN_POINT('Ctrl Pts',(-9.71549257088175,-20.3548282742361,
0.));
#195305=CARTESIAN_POINT('Ctrl Pts',(-9.71619192554147,-20.3562337557875,
0.));
#195306=CARTESIAN_POINT('Ctrl Pts',(-9.71708493723062,-20.3580133103357,
0.));
#195307=CARTESIAN_POINT('Ctrl Pts',(-9.71816778327999,-20.3601498764344,
0.));
#195308=CARTESIAN_POINT('Ctrl Pts',(-9.71943648548115,-20.362625691398,
0.));
#195309=CARTESIAN_POINT('Ctrl Pts',(-9.72088778381102,-20.3654261611055,
0.));
#195310=CARTESIAN_POINT('Ctrl Pts',(-9.72251930722504,-20.3685406190576,
0.));
#195311=CARTESIAN_POINT('Ctrl Pts',(-9.72432910043193,-20.371960235676,
0.));
#195312=CARTESIAN_POINT('Ctrl Pts',(-9.72631531732871,-20.3756766651952,
0.));
#195313=CARTESIAN_POINT('Ctrl Pts',(-9.72847589116533,-20.3796805893304,
0.));
#195314=CARTESIAN_POINT('Ctrl Pts',(-9.73080870123726,-20.3839624556742,
0.));
#195315=CARTESIAN_POINT('Ctrl Pts',(-9.73331167102812,-20.3885129129912,
0.));
#195316=CARTESIAN_POINT('Ctrl Pts',(-9.7359829201425,-20.3933234845646,
0.));
#195317=CARTESIAN_POINT('Ctrl Pts',(-9.73882077613206,-20.3983866213331,
0.));
#195318=CARTESIAN_POINT('Ctrl Pts',(-9.74182369656273,-20.4036953576549,
0.));
#195319=CARTESIAN_POINT('Ctrl Pts',(-9.74499021838537,-20.4092430879861,
0.));
#195320=CARTESIAN_POINT('Ctrl Pts',(-9.74831889242175,-20.4150232777393,
0.));
#195321=CARTESIAN_POINT('Ctrl Pts',(-9.75180829786433,-20.4210295275818,
0.));
#195322=CARTESIAN_POINT('Ctrl Pts',(-9.75545705902416,-20.4272556476629,
0.));
#195323=CARTESIAN_POINT('Ctrl Pts',(-9.7592638628993,-20.4336957355474,
0.));
#195324=CARTESIAN_POINT('Ctrl Pts',(-9.76322747195502,-20.4403442329401,
0.));
#195325=CARTESIAN_POINT('Ctrl Pts',(-9.76734670980897,-20.447195862298,
0.));
#195326=CARTESIAN_POINT('Ctrl Pts',(-9.7716204510407,-20.4542455817527,
0.));
#195327=CARTESIAN_POINT('Ctrl Pts',(-9.77604760815523,-20.4614885274973,
0.));
#195328=CARTESIAN_POINT('Ctrl Pts',(-9.78062712373313,-20.4689199790668,
0.));
#195329=CARTESIAN_POINT('Ctrl Pts',(-9.78535797314162,-20.4765353711585,
0.));
#195330=CARTESIAN_POINT('Ctrl Pts',(-9.7902391649866,-20.4843302955329,
0.));
#195331=CARTESIAN_POINT('Ctrl Pts',(-9.79526974288344,-20.4923005087945,
0.));
#195332=CARTESIAN_POINT('Ctrl Pts',(-9.80044878520968,-20.500441931211,
0.));
#195333=CARTESIAN_POINT('Ctrl Pts',(-9.80577540161103,-20.5087506310507,
0.));
#195334=CARTESIAN_POINT('Ctrl Pts',(-9.81124873025278,-20.5172228122839,
0.));
#195335=CARTESIAN_POINT('Ctrl Pts',(-9.81686793455918,-20.5258548000625,
0.));
#195336=CARTESIAN_POINT('Ctrl Pts',(-9.82263220080328,-20.534643029951,
0.));
#195337=CARTESIAN_POINT('Ctrl Pts',(-9.82854073773858,-20.5435840460717,
0.));
#195338=CARTESIAN_POINT('Ctrl Pts',(-9.83459277585321,-20.5526744976461,
0.));
#195339=CARTESIAN_POINT('Ctrl Pts',(-9.84078756677589,-20.5619111362406,
0.));
#195340=CARTESIAN_POINT('Ctrl Pts',(-9.84712438256308,-20.5712908125145,
0.));
#195341=CARTESIAN_POINT('Ctrl Pts',(-9.85360251457004,-20.580810471002,
0.));
#195342=CARTESIAN_POINT('Ctrl Pts',(-9.8602212723275,-20.5904671449754,
0.));
#195343=CARTESIAN_POINT('Ctrl Pts',(-9.86697998242612,-20.6002579513696,
0.));
#195344=CARTESIAN_POINT('Ctrl Pts',(-9.87387798732944,-20.6101800854491,
0.));
#195345=CARTESIAN_POINT('Ctrl Pts',(-9.88091464472669,-20.6202308177472,
0.));
#195346=CARTESIAN_POINT('Ctrl Pts',(-9.88808932697305,-20.6304074914086,
0.));
#195347=CARTESIAN_POINT('Ctrl Pts',(-9.89540142049124,-20.6407075193977,
0.));
#195348=CARTESIAN_POINT('Ctrl Pts',(-9.90285032516696,-20.6511283817415,
0.));
#195349=CARTESIAN_POINT('Ctrl Pts',(-9.91043545377005,-20.6616676228315,
0.));
#195350=CARTESIAN_POINT('Ctrl Pts',(-9.91815623141285,-20.6723228488261,
0.));
#195351=CARTESIAN_POINT('Ctrl Pts',(-9.92601209498751,-20.6830917250255,
0.));
#195352=CARTESIAN_POINT('Ctrl Pts',(-9.93400249259737,-20.6939719732485,
0.));
#195353=CARTESIAN_POINT('Ctrl Pts',(-9.94212688298251,-20.7049613692237,
0.));
#195354=CARTESIAN_POINT('Ctrl Pts',(-9.95038473514962,-20.716057740758,
0.));
#195355=CARTESIAN_POINT('Ctrl Pts',(-9.95877552798403,-20.7272589658752,
0.));
#195356=CARTESIAN_POINT('Ctrl Pts',(-9.96729874986199,-20.7385629709795,
0.));
#195357=CARTESIAN_POINT('Ctrl Pts',(-9.97595389823461,-20.7499677289625,
0.));
#195358=CARTESIAN_POINT('Ctrl Pts',(-9.98474047926846,-20.7614712574989,
0.));
#195359=CARTESIAN_POINT('Ctrl Pts',(-9.99365800754638,-20.7730716175417,
0.));
#195360=CARTESIAN_POINT('Ctrl Pts',(-10.0027060057389,-20.7847669117568,
0.));
#195361=CARTESIAN_POINT('Ctrl Pts',(-10.0118840042786,-20.7965552829907,
0.));
#195362=CARTESIAN_POINT('Ctrl Pts',(-10.0211915410095,-20.8084349126885,
0.));
#195363=CARTESIAN_POINT('Ctrl Pts',(-10.0306281609435,-20.8204040196599,
0.));
#195364=CARTESIAN_POINT('Ctrl Pts',(-10.0401934160234,-20.8324608588906,
0.));
#195365=CARTESIAN_POINT('Ctrl Pts',(-10.0498868648733,-20.8446037203402,
0.));
#195366=CARTESIAN_POINT('Ctrl Pts',(-10.0597080725375,-20.856830927732,
0.));
#195367=CARTESIAN_POINT('Ctrl Pts',(-10.0696566102219,-20.8691408373705,
0.));
#195368=CARTESIAN_POINT('Ctrl Pts',(-10.0797320551154,-20.8815318371844,
0.));
#195369=CARTESIAN_POINT('Ctrl Pts',(-10.0899339901916,-20.8940023457371,
0.));
#195370=CARTESIAN_POINT('Ctrl Pts',(-10.1002620040076,-20.9065508112556,
0.));
#195371=CARTESIAN_POINT('Ctrl Pts',(-10.1107156904836,-20.9191757106266,
0.));
#195372=CARTESIAN_POINT('Ctrl Pts',(-10.1212946487057,-20.931875548473,
0.));
#195373=CARTESIAN_POINT('Ctrl Pts',(-10.1319984827909,-20.944648856393,
0.));
#195374=CARTESIAN_POINT('Ctrl Pts',(-10.1428268017257,-20.9574941921591,
0.));
#195375=CARTESIAN_POINT('Ctrl Pts',(-10.1537792192065,-20.970410138937,
0.));
#195376=CARTESIAN_POINT('Ctrl Pts',(-10.1648553534567,-20.9833953044736,
0.));
#195377=CARTESIAN_POINT('Ctrl Pts',(-10.1760548270765,-20.9964483203685,
0.));
#195378=CARTESIAN_POINT('Ctrl Pts',(-10.1873772669358,-21.0095678414486,
0.));
#195379=CARTESIAN_POINT('Ctrl Pts',(-10.1988223040425,-21.0227525451107,
0.));
#195380=CARTESIAN_POINT('Ctrl Pts',(-10.2103895734124,-21.0360011306814,
0.));
#195381=CARTESIAN_POINT('Ctrl Pts',(-10.2220787139157,-21.0493123187483,
0.));
#195382=CARTESIAN_POINT('Ctrl Pts',(-10.233889368157,-21.0626848505665,
0.));
#195383=CARTESIAN_POINT('Ctrl Pts',(-10.2458211823915,-21.0761174875448,
0.));
#195384=CARTESIAN_POINT('Ctrl Pts',(-10.2578738064183,-21.0896090107066,
0.));
#195385=CARTESIAN_POINT('Ctrl Pts',(-10.2700468934743,-21.1031582201625,
0.));
#195386=CARTESIAN_POINT('Ctrl Pts',(-10.2823401001067,-21.1167639345623,
0.));
#195387=CARTESIAN_POINT('Ctrl Pts',(-10.2947530860714,-21.130424990599,
0.));
#195388=CARTESIAN_POINT('Ctrl Pts',(-10.307285514268,-21.1441402425831,
0.));
#195389=CARTESIAN_POINT('Ctrl Pts',(-10.3199370506541,-21.1579085619959,
0.));
#195390=CARTESIAN_POINT('Ctrl Pts',(-10.3327073641574,-21.1717288370512,
0.));
#195391=CARTESIAN_POINT('Ctrl Pts',(-10.3455961265706,-21.1855999722427,
0.));
#195392=CARTESIAN_POINT('Ctrl Pts',(-10.3586030124595,-21.1995208879205,
0.));
#195393=CARTESIAN_POINT('Ctrl Pts',(-10.3717276991137,-21.2134905199359,
0.));
#195394=CARTESIAN_POINT('Ctrl Pts',(-10.384969866479,-21.2275078192708,
0.));
#195395=CARTESIAN_POINT('Ctrl Pts',(-10.3983291970846,-21.2415717516713,
0.));
#195396=CARTESIAN_POINT('Ctrl Pts',(-10.4118053759584,-21.2556812972741,
0.));
#195397=CARTESIAN_POINT('Ctrl Pts',(-10.4253980905394,-21.2698354502391,
0.));
#195398=CARTESIAN_POINT('Ctrl Pts',(-10.4391070306385,-21.2840332184471,
0.));
#195399=CARTESIAN_POINT('Ctrl Pts',(-10.452931888387,-21.2982736231924,
0.));
#195400=CARTESIAN_POINT('Ctrl Pts',(-10.4668723581768,-21.312555698873,
0.));
#195401=CARTESIAN_POINT('Ctrl Pts',(-10.4809281365933,-21.3268784926823,
0.));
#195402=CARTESIAN_POINT('Ctrl Pts',(-10.4950989223341,-21.3412410642912,
0.));
#195403=CARTESIAN_POINT('Ctrl Pts',(-10.509384416169,-21.3556424855822,
0.));
#195404=CARTESIAN_POINT('Ctrl Pts',(-10.523784320906,-21.3700818403942,
0.));
#195405=CARTESIAN_POINT('Ctrl Pts',(-10.5382983413422,-21.3845582242604,
0.));
#195406=CARTESIAN_POINT('Ctrl Pts',(-10.5529261842107,-21.3990707441495,
0.));
#195407=CARTESIAN_POINT('Ctrl Pts',(-10.5676675581106,-21.4136185181974,
0.));
#195408=CARTESIAN_POINT('Ctrl Pts',(-10.582522173457,-21.4282006754624,
0.));
#195409=CARTESIAN_POINT('Ctrl Pts',(-10.597489742462,-21.4428163557137,
0.));
#195410=CARTESIAN_POINT('Ctrl Pts',(-10.612569979096,-21.4574647092093,
0.));
#195411=CARTESIAN_POINT('Ctrl Pts',(-10.6277625990457,-21.4721448964766,
0.));
#195412=CARTESIAN_POINT('Ctrl Pts',(-10.6430673196609,-21.4868560880893,
0.));
#195413=CARTESIAN_POINT('Ctrl Pts',(-10.6584838598941,-21.5015974644454,
0.));
#195414=CARTESIAN_POINT('Ctrl Pts',(-10.6740119402835,-21.5163682155805,
0.));
#195415=CARTESIAN_POINT('Ctrl Pts',(-10.689651282929,-21.531167540981,0.));
#195416=CARTESIAN_POINT('Ctrl Pts',(-10.7054016114571,-21.5459946493955,
0.));
#195417=CARTESIAN_POINT('Ctrl Pts',(-10.7212626509816,-21.5608487586467,
0.));
#195418=CARTESIAN_POINT('Ctrl Pts',(-10.7372341280468,-21.5757290954372,
0.));
#195419=CARTESIAN_POINT('Ctrl Pts',(-10.7533157705943,-21.5906348951745,
0.));
#195420=CARTESIAN_POINT('Ctrl Pts',(-10.7695073079554,-21.6055654018179,
0.));
#195421=CARTESIAN_POINT('Ctrl Pts',(-10.7858084708262,-21.6205198677176,
0.));
#195422=CARTESIAN_POINT('Ctrl Pts',(-10.802218991237,-21.6354975534557,
0.));
#195423=CARTESIAN_POINT('Ctrl Pts',(-10.8187386025135,-21.6504977276864,
0.));
#195424=CARTESIAN_POINT('Ctrl Pts',(-10.835367039227,-21.6655196669727,
0.));
#195425=CARTESIAN_POINT('Ctrl Pts',(-10.8521040371832,-21.6805626556461,
0.));
#195426=CARTESIAN_POINT('Ctrl Pts',(-10.8689493334093,-21.6956259856667,
0.));
#195427=CARTESIAN_POINT('Ctrl Pts',(-10.8859026661292,-21.7107089564822,
0.));
#195428=CARTESIAN_POINT('Ctrl Pts',(-10.9029637747341,-21.7258108748874,
0.));
#195429=CARTESIAN_POINT('Ctrl Pts',(-10.9201323997386,-21.74093105488,0.));
#195430=CARTESIAN_POINT('Ctrl Pts',(-10.9374082827446,-21.7560688175252,
0.));
#195431=CARTESIAN_POINT('Ctrl Pts',(-10.9547911664457,-21.7712234908468,
0.));
#195432=CARTESIAN_POINT('Ctrl Pts',(-10.9722807946157,-21.7863944097143,
0.));
#195433=CARTESIAN_POINT('Ctrl Pts',(-10.9898769120913,-21.8015809157302,
0.));
#195434=CARTESIAN_POINT('Ctrl Pts',(-11.0075792647477,-21.8167823571168,
0.));
#195435=CARTESIAN_POINT('Ctrl Pts',(-11.0253875994598,-21.8319980886033,
0.));
#195436=CARTESIAN_POINT('Ctrl Pts',(-11.0433016640808,-21.8472274713103,
0.));
#195437=CARTESIAN_POINT('Ctrl Pts',(-11.0613212074364,-21.8624698726319,
0.));
#195438=CARTESIAN_POINT('Ctrl Pts',(-11.0794459793058,-21.8777246661191,
0.));
#195439=CARTESIAN_POINT('Ctrl Pts',(-11.0976757303944,-21.8929912313608,
0.));
#195440=CARTESIAN_POINT('Ctrl Pts',(-11.1160102123024,-21.9082689538687,
0.));
#195441=CARTESIAN_POINT('Ctrl Pts',(-11.134449177474,-21.9235572249518,
0.));
#195442=CARTESIAN_POINT('Ctrl Pts',(-11.1529923792002,-21.9388554416437,
0.));
#195443=CARTESIAN_POINT('Ctrl Pts',(-11.1716395716375,-21.9541630066504,
0.));
#195444=CARTESIAN_POINT('Ctrl Pts',(-11.190390509811,-21.9694793282913,
0.));
#195445=CARTESIAN_POINT('Ctrl Pts',(-11.2092449496125,-21.9848038204439,
0.));
#195446=CARTESIAN_POINT('Ctrl Pts',(-11.2282026477897,-22.0001359024839,
0.));
#195447=CARTESIAN_POINT('Ctrl Pts',(-11.2472633619276,-22.0154749992364,
0.));
#195448=CARTESIAN_POINT('Ctrl Pts',(-11.2664268504207,-22.0308205408351,
0.));
#195449=CARTESIAN_POINT('Ctrl Pts',(-11.2856928724374,-22.046171962566,
0.));
#195450=CARTESIAN_POINT('Ctrl Pts',(-11.3050611878771,-22.0615287047179,
0.));
#195451=CARTESIAN_POINT('Ctrl Pts',(-11.3245315573168,-22.0768902124267,
0.));
#195452=CARTESIAN_POINT('Ctrl Pts',(-11.3441037419553,-22.0922559355293,
0.));
#195453=CARTESIAN_POINT('Ctrl Pts',(-11.3637775035367,-22.1076253283978,
0.));
#195454=CARTESIAN_POINT('Ctrl Pts',(-11.3835526044256,-22.1229978500185,
0.));
#195455=CARTESIAN_POINT('Ctrl Pts',(-11.4034288076909,-22.1383729640963,
0.));
#195456=CARTESIAN_POINT('Ctrl Pts',(-11.4234058771742,-22.1537501391486,
0.));
#195457=CARTESIAN_POINT('Ctrl Pts',(-11.443483577557,-22.1691288486096,
0.));
#195458=CARTESIAN_POINT('Ctrl Pts',(-11.463661674411,-22.1845085709169,
0.));
#195459=CARTESIAN_POINT('Ctrl Pts',(-11.4839399342589,-22.1998887896435,
0.));
#195460=CARTESIAN_POINT('Ctrl Pts',(-11.504318124424,-22.215268993102,0.));
#195461=CARTESIAN_POINT('Ctrl Pts',(-11.5247960128476,-22.2306486738899,
0.));
#195462=CARTESIAN_POINT('Ctrl Pts',(-11.545373367912,-22.2460273284653,
0.));
#195463=CARTESIAN_POINT('Ctrl Pts',(-11.5660499582403,-22.2614044566898,
0.));
#195464=CARTESIAN_POINT('Ctrl Pts',(-11.5868255525189,-22.2767795614349,
0.));
#195465=CARTESIAN_POINT('Ctrl Pts',(-11.6076999192359,-22.2921521480357,
0.));
#195466=CARTESIAN_POINT('Ctrl Pts',(-11.6286728270011,-22.3075217249049,
0.));
#195467=CARTESIAN_POINT('Ctrl Pts',(-11.6497440449858,-22.3228878043976,
0.));
#195468=CARTESIAN_POINT('Ctrl Pts',(-11.6709133432986,-22.3382499035618,
0.));
#195469=CARTESIAN_POINT('Ctrl Pts',(-11.6921804934056,-22.3536075450028,
0.));
#195470=CARTESIAN_POINT('Ctrl Pts',(-11.7135452684532,-22.3689602575492,
0.));
#195471=CARTESIAN_POINT('Ctrl Pts',(-11.7350074437961,-22.3843075773905,
0.));
#195472=CARTESIAN_POINT('Ctrl Pts',(-11.7565667964765,-22.39964904692,0.));
#195473=CARTESIAN_POINT('Ctrl Pts',(-11.7782231042041,-22.4149842125018,
0.));
#195474=CARTESIAN_POINT('Ctrl Pts',(-11.7999761445175,-22.4303126226468,
0.));
#195475=CARTESIAN_POINT('Ctrl Pts',(-11.8218256937889,-22.4456338258738,
0.));
#195476=CARTESIAN_POINT('Ctrl Pts',(-11.8437715264487,-22.4609473690469,
0.));
#195477=CARTESIAN_POINT('Ctrl Pts',(-11.8658134137018,-22.4762527946694,
0.));
#195478=CARTESIAN_POINT('Ctrl Pts',(-11.8879511239941,-22.4915496418472,
0.));
#195479=CARTESIAN_POINT('Ctrl Pts',(-11.9101844254555,-22.5068374513958,
0.));
#195480=CARTESIAN_POINT('Ctrl Pts',(-11.9325130877801,-22.5221157697869,
0.));
#195481=CARTESIAN_POINT('Ctrl Pts',(-11.9549368843996,-22.5373841537299,
0.));
#195482=CARTESIAN_POINT('Ctrl Pts',(-11.9774555943496,-22.5526421741159,
0.));
#195483=CARTESIAN_POINT('Ctrl Pts',(-12.0000690046697,-22.5678894211194,
0.));
#195484=CARTESIAN_POINT('Ctrl Pts',(-12.0227769113132,-22.5831255061306,
0.));
#195485=CARTESIAN_POINT('Ctrl Pts',(-12.0455791139135,-22.5983500505675,
0.));
#195486=CARTESIAN_POINT('Ctrl Pts',(-12.0684754113869,-22.613562676493,
0.));
#195487=CARTESIAN_POINT('Ctrl Pts',(-12.0914655972828,-22.628762996708,
0.));
#195488=CARTESIAN_POINT('Ctrl Pts',(-12.1145494550384,-22.6439506046611,
0.));
#195489=CARTESIAN_POINT('Ctrl Pts',(-12.1377267537141,-22.6591250653942,
0.));
#195490=CARTESIAN_POINT('Ctrl Pts',(-12.1609972423089,-22.6742859034891,
0.));
#195491=CARTESIAN_POINT('Ctrl Pts',(-12.1843606579246,-22.6894326204959,
0.));
#195492=CARTESIAN_POINT('Ctrl Pts',(-12.2078167360267,-22.7045647168659,
0.));
#195493=CARTESIAN_POINT('Ctrl Pts',(-12.2313652198047,-22.7196817119299,
0.));
#195494=CARTESIAN_POINT('Ctrl Pts',(-12.2550058702389,-22.7347831655251,
0.));
#195495=CARTESIAN_POINT('Ctrl Pts',(-12.2787384750747,-22.7498686970096,
0.));
#195496=CARTESIAN_POINT('Ctrl Pts',(-12.3025628601812,-22.7649380101154,
0.));
#195497=CARTESIAN_POINT('Ctrl Pts',(-12.3264788926108,-22.7799908974947,
0.));
#195498=CARTESIAN_POINT('Ctrl Pts',(-12.3504864740361,-22.7950272216959,
0.));
#195499=CARTESIAN_POINT('Ctrl Pts',(-12.3745855366772,-22.8100469022632,
0.));
#195500=CARTESIAN_POINT('Ctrl Pts',(-12.393937937903,-22.8220493007353,
0.));
#195501=CARTESIAN_POINT('Ctrl Pts',(-12.4084933766366,-22.8310435872852,
0.));
#195502=CARTESIAN_POINT('Ctrl Pts',(-12.4182152851867,-22.8370364396497,
0.));
#195503=CARTESIAN_POINT('Ctrl Pts',(-12.4230808101438,-22.8400320311648,
0.));
#195504=CARTESIAN_POINT('',(-12.4230808101438,-22.8400320311648,0.));
#195505=CARTESIAN_POINT('Origin',(-13.9675290154577,-16.3449727195351,0.));
#195506=CARTESIAN_POINT('',(-14.6513681262571,-17.1452095830632,0.));
#195507=CARTESIAN_POINT('',(-14.6513681262571,-17.1452095830632,0.));
#195508=CARTESIAN_POINT('',(-6.98376450772884,-8.17248635976757,0.));
#195509=CARTESIAN_POINT('Ctrl Pts',(-13.5685075571671,-22.1787195904339,
0.));
#195510=CARTESIAN_POINT('Ctrl Pts',(-13.5685075571671,-22.1787195904339,
12.));
#195511=CARTESIAN_POINT('Ctrl Pts',(-13.5683460612913,-22.1730081264583,
0.));
#195512=CARTESIAN_POINT('Ctrl Pts',(-13.5683460612913,-22.1730081264583,
12.));
#195513=CARTESIAN_POINT('Ctrl Pts',(-13.5680170531724,-22.1615922804939,
0.));
#195514=CARTESIAN_POINT('Ctrl Pts',(-13.5680170531724,-22.1615922804939,
12.));
#195515=CARTESIAN_POINT('Ctrl Pts',(-13.5675054918922,-22.1444897575076,
0.));
#195516=CARTESIAN_POINT('Ctrl Pts',(-13.5675054918922,-22.1444897575076,
12.));
#195517=CARTESIAN_POINT('Ctrl Pts',(-13.5667873105179,-22.1217288871823,
0.));
#195518=CARTESIAN_POINT('Ctrl Pts',(-13.5667873105179,-22.1217288871823,
12.));
#195519=CARTESIAN_POINT('Ctrl Pts',(-13.5658294169107,-22.0933486464442,
0.));
#195520=CARTESIAN_POINT('Ctrl Pts',(-13.5658294169107,-22.0933486464442,
12.));
#195521=CARTESIAN_POINT('Ctrl Pts',(-13.5648113688895,-22.0650393089492,
0.));
#195522=CARTESIAN_POINT('Ctrl Pts',(-13.5648113688895,-22.0650393089492,
12.));
#195523=CARTESIAN_POINT('Ctrl Pts',(-13.5637332022393,-22.0368009736227,
0.));
#195524=CARTESIAN_POINT('Ctrl Pts',(-13.5637332022393,-22.0368009736227,
12.));
#195525=CARTESIAN_POINT('Ctrl Pts',(-13.5625949868313,-22.0086337943431,
0.));
#195526=CARTESIAN_POINT('Ctrl Pts',(-13.5625949868313,-22.0086337943431,
12.));
#195527=CARTESIAN_POINT('Ctrl Pts',(-13.5613968357589,-21.9805379899192,
0.));
#195528=CARTESIAN_POINT('Ctrl Pts',(-13.5613968357589,-21.9805379899192,
12.));
#195529=CARTESIAN_POINT('Ctrl Pts',(-13.5601389185315,-21.9525138592862,
0.));
#195530=CARTESIAN_POINT('Ctrl Pts',(-13.5601389185315,-21.9525138592862,
12.));
#195531=CARTESIAN_POINT('Ctrl Pts',(-13.5588214586672,-21.9245617765827,
0.));
#195532=CARTESIAN_POINT('Ctrl Pts',(-13.5588214586672,-21.9245617765827,
12.));
#195533=CARTESIAN_POINT('Ctrl Pts',(-13.5574447178485,-21.8966821688876,
0.));
#195534=CARTESIAN_POINT('Ctrl Pts',(-13.5574447178485,-21.8966821688876,
12.));
#195535=CARTESIAN_POINT('Ctrl Pts',(-13.5560089839426,-21.8688754989401,
0.));
#195536=CARTESIAN_POINT('Ctrl Pts',(-13.5560089839426,-21.8688754989401,
12.));
#195537=CARTESIAN_POINT('Ctrl Pts',(-13.5545145573049,-21.841142245609,
0.));
#195538=CARTESIAN_POINT('Ctrl Pts',(-13.5545145573049,-21.841142245609,
12.));
#195539=CARTESIAN_POINT('Ctrl Pts',(-13.5529617381569,-21.8134828857963,
0.));
#195540=CARTESIAN_POINT('Ctrl Pts',(-13.5529617381569,-21.8134828857963,
12.));
#195541=CARTESIAN_POINT('Ctrl Pts',(-13.5513508127232,-21.7858978745848,
0.));
#195542=CARTESIAN_POINT('Ctrl Pts',(-13.5513508127232,-21.7858978745848,
12.));
#195543=CARTESIAN_POINT('Ctrl Pts',(-13.5496820422187,-21.7583876294532,
0.));
#195544=CARTESIAN_POINT('Ctrl Pts',(-13.5496820422187,-21.7583876294532,
12.));
#195545=CARTESIAN_POINT('Ctrl Pts',(-13.5479556704457,-21.730952541226,
0.));
#195546=CARTESIAN_POINT('Ctrl Pts',(-13.5479556704457,-21.730952541226,
12.));
#195547=CARTESIAN_POINT('Ctrl Pts',(-13.546171929503,-21.7035929822939,
0.));
#195548=CARTESIAN_POINT('Ctrl Pts',(-13.546171929503,-21.7035929822939,
12.));
#195549=CARTESIAN_POINT('Ctrl Pts',(-13.5443310461516,-21.676309315769,
0.));
#195550=CARTESIAN_POINT('Ctrl Pts',(-13.5443310461516,-21.676309315769,
12.));
#195551=CARTESIAN_POINT('Ctrl Pts',(-13.5424332480698,-21.6491019044647,
0.));
#195552=CARTESIAN_POINT('Ctrl Pts',(-13.5424332480698,-21.6491019044647,
12.));
#195553=CARTESIAN_POINT('Ctrl Pts',(-13.5404787697798,-21.6219711193951,
0.));
#195554=CARTESIAN_POINT('Ctrl Pts',(-13.5404787697798,-21.6219711193951,
12.));
#195555=CARTESIAN_POINT('Ctrl Pts',(-13.5384678597206,-21.5949173499022,
0.));
#195556=CARTESIAN_POINT('Ctrl Pts',(-13.5384678597206,-21.5949173499022,
12.));
#195557=CARTESIAN_POINT('Ctrl Pts',(-13.5364007790292,-21.5679410019011,
0.));
#195558=CARTESIAN_POINT('Ctrl Pts',(-13.5364007790292,-21.5679410019011,
12.));
#195559=CARTESIAN_POINT('Ctrl Pts',(-13.5342777983225,-21.5410424932511,
0.));
#195560=CARTESIAN_POINT('Ctrl Pts',(-13.5342777983225,-21.5410424932511,
12.));
#195561=CARTESIAN_POINT('Ctrl Pts',(-13.5320991952145,-21.5142222501671,
0.));
#195562=CARTESIAN_POINT('Ctrl Pts',(-13.5320991952145,-21.5142222501671,
12.));
#195563=CARTESIAN_POINT('Ctrl Pts',(-13.5298652514357,-21.487480703047,
0.));
#195564=CARTESIAN_POINT('Ctrl Pts',(-13.5298652514357,-21.487480703047,
12.));
#195565=CARTESIAN_POINT('Ctrl Pts',(-13.5275762503553,-21.4608182828695,
0.));
#195566=CARTESIAN_POINT('Ctrl Pts',(-13.5275762503553,-21.4608182828695,
12.));
#195567=CARTESIAN_POINT('Ctrl Pts',(-13.5252324737795,-21.4342354165253,
0.));
#195568=CARTESIAN_POINT('Ctrl Pts',(-13.5252324737795,-21.4342354165253,
12.));
#195569=CARTESIAN_POINT('Ctrl Pts',(-13.5228342013508,-21.4077325259318,
0.));
#195570=CARTESIAN_POINT('Ctrl Pts',(-13.5228342013508,-21.4077325259318,
12.));
#195571=CARTESIAN_POINT('Ctrl Pts',(-13.5203817122497,-21.3813100304967,
0.));
#195572=CARTESIAN_POINT('Ctrl Pts',(-13.5203817122497,-21.3813100304967,
12.));
#195573=CARTESIAN_POINT('Ctrl Pts',(-13.5178752862461,-21.3549683486219,
0.));
#195574=CARTESIAN_POINT('Ctrl Pts',(-13.5178752862461,-21.3549683486219,
12.));
#195575=CARTESIAN_POINT('Ctrl Pts',(-13.5153152050554,-21.328707899634,
0.));
#195576=CARTESIAN_POINT('Ctrl Pts',(-13.5153152050554,-21.328707899634,
12.));
#195577=CARTESIAN_POINT('Ctrl Pts',(-13.5127017534972,-21.3025291054236,
0.));
#195578=CARTESIAN_POINT('Ctrl Pts',(-13.5127017534972,-21.3025291054236,
12.));
#195579=CARTESIAN_POINT('Ctrl Pts',(-13.5100352209207,-21.2764323924442,
0.));
#195580=CARTESIAN_POINT('Ctrl Pts',(-13.5100352209207,-21.2764323924442,
12.));
#195581=CARTESIAN_POINT('Ctrl Pts',(-13.5073159019454,-21.2504181927429,
0.));
#195582=CARTESIAN_POINT('Ctrl Pts',(-13.5073159019454,-21.2504181927429,
12.));
#195583=CARTESIAN_POINT('Ctrl Pts',(-13.5045440957404,-21.224486942933,
0.));
#195584=CARTESIAN_POINT('Ctrl Pts',(-13.5045440957404,-21.224486942933,
12.));
#195585=CARTESIAN_POINT('Ctrl Pts',(-13.5017201056088,-21.1986390835825,
0.));
#195586=CARTESIAN_POINT('Ctrl Pts',(-13.5017201056088,-21.1986390835825,
12.));
#195587=CARTESIAN_POINT('Ctrl Pts',(-13.4988442384491,-21.1728750584173,
0.));
#195588=CARTESIAN_POINT('Ctrl Pts',(-13.4988442384491,-21.1728750584173,
12.));
#195589=CARTESIAN_POINT('Ctrl Pts',(-13.4959168042934,-21.1471953136209,
0.));
#195590=CARTESIAN_POINT('Ctrl Pts',(-13.4959168042934,-21.1471953136209,
12.));
#195591=CARTESIAN_POINT('Ctrl Pts',(-13.4929381157778,-21.1216002970209,
0.));
#195592=CARTESIAN_POINT('Ctrl Pts',(-13.4929381157778,-21.1216002970209,
12.));
#195593=CARTESIAN_POINT('Ctrl Pts',(-13.4899084877718,-21.0960904575048,
0.));
#195594=CARTESIAN_POINT('Ctrl Pts',(-13.4899084877718,-21.0960904575048,
12.));
#195595=CARTESIAN_POINT('Ctrl Pts',(-13.4868282377192,-21.0706662455202,
0.));
#195596=CARTESIAN_POINT('Ctrl Pts',(-13.4868282377192,-21.0706662455202,
12.));
#195597=CARTESIAN_POINT('Ctrl Pts',(-13.4836976858912,-21.0453281134247,
0.));
#195598=CARTESIAN_POINT('Ctrl Pts',(-13.4836976858912,-21.0453281134247,
12.));
#195599=CARTESIAN_POINT('Ctrl Pts',(-13.4805171556822,-21.0200765158885,
0.));
#195600=CARTESIAN_POINT('Ctrl Pts',(-13.4805171556822,-21.0200765158885,
12.));
#195601=CARTESIAN_POINT('Ctrl Pts',(-13.4772869738879,-20.9949119102592,
0.));
#195602=CARTESIAN_POINT('Ctrl Pts',(-13.4772869738879,-20.9949119102592,
12.));
#195603=CARTESIAN_POINT('Ctrl Pts',(-13.4740074710087,-20.9698347569476,
0.));
#195604=CARTESIAN_POINT('Ctrl Pts',(-13.4740074710087,-20.9698347569476,
12.));
#195605=CARTESIAN_POINT('Ctrl Pts',(-13.4706789815167,-20.9448455197557,
0.));
#195606=CARTESIAN_POINT('Ctrl Pts',(-13.4706789815167,-20.9448455197557,
12.));
#195607=CARTESIAN_POINT('Ctrl Pts',(-13.4673018437718,-20.9199446657584,
0.));
#195608=CARTESIAN_POINT('Ctrl Pts',(-13.4673018437718,-20.9199446657584,
12.));
#195609=CARTESIAN_POINT('Ctrl Pts',(-13.4638763999726,-20.8951326652158,
0.));
#195610=CARTESIAN_POINT('Ctrl Pts',(-13.4638763999726,-20.8951326652158,
12.));
#195611=CARTESIAN_POINT('Ctrl Pts',(-13.4604029960983,-20.8704099914641,
0.));
#195612=CARTESIAN_POINT('Ctrl Pts',(-13.4604029960983,-20.8704099914641,
12.));
#195613=CARTESIAN_POINT('Ctrl Pts',(-13.4568819818631,-20.8457771208082,
0.));
#195614=CARTESIAN_POINT('Ctrl Pts',(-13.4568819818631,-20.8457771208082,
12.));
#195615=CARTESIAN_POINT('Ctrl Pts',(-13.4533137106667,-20.821234532398,
0.));
#195616=CARTESIAN_POINT('Ctrl Pts',(-13.4533137106667,-20.821234532398,
12.));
#195617=CARTESIAN_POINT('Ctrl Pts',(-13.4496985395637,-20.7967827081227,
0.));
#195618=CARTESIAN_POINT('Ctrl Pts',(-13.4496985395637,-20.7967827081227,
12.));
#195619=CARTESIAN_POINT('Ctrl Pts',(-13.4460368293688,-20.7724221327608,
0.));
#195620=CARTESIAN_POINT('Ctrl Pts',(-13.4460368293688,-20.7724221327608,
12.));
#195621=CARTESIAN_POINT('Ctrl Pts',(-13.4423289447561,-20.7481532941013,
0.));
#195622=CARTESIAN_POINT('Ctrl Pts',(-13.4423289447561,-20.7481532941013,
12.));
#195623=CARTESIAN_POINT('Ctrl Pts',(-13.4385752543663,-20.7239766830675,
0.));
#195624=CARTESIAN_POINT('Ctrl Pts',(-13.4385752543663,-20.7239766830675,
12.));
#195625=CARTESIAN_POINT('Ctrl Pts',(-13.4347761309154,-20.6998927938288,
0.));
#195626=CARTESIAN_POINT('Ctrl Pts',(-13.4347761309154,-20.6998927938288,
12.));
#195627=CARTESIAN_POINT('Ctrl Pts',(-13.4309319513119,-20.6759021239103,
0.));
#195628=CARTESIAN_POINT('Ctrl Pts',(-13.4309319513119,-20.6759021239103,
12.));
#195629=CARTESIAN_POINT('Ctrl Pts',(-13.4270430967652,-20.6520051742869,
0.));
#195630=CARTESIAN_POINT('Ctrl Pts',(-13.4270430967652,-20.6520051742869,
12.));
#195631=CARTESIAN_POINT('Ctrl Pts',(-13.4231099528179,-20.6282024494237,
0.));
#195632=CARTESIAN_POINT('Ctrl Pts',(-13.4231099528179,-20.6282024494237,
12.));
#195633=CARTESIAN_POINT('Ctrl Pts',(-13.4191329093933,-20.6044944573153,
0.));
#195634=CARTESIAN_POINT('Ctrl Pts',(-13.4191329093933,-20.6044944573153,
12.));
#195635=CARTESIAN_POINT('Ctrl Pts',(-13.4151123608411,-20.5808817095155,
0.));
#195636=CARTESIAN_POINT('Ctrl Pts',(-13.4151123608411,-20.5808817095155,
12.));
#195637=CARTESIAN_POINT('Ctrl Pts',(-13.4110487059912,-20.5573647211639,
0.));
#195638=CARTESIAN_POINT('Ctrl Pts',(-13.4110487059912,-20.5573647211639,
12.));
#195639=CARTESIAN_POINT('Ctrl Pts',(-13.4069423482076,-20.5339440109956,
0.));
#195640=CARTESIAN_POINT('Ctrl Pts',(-13.4069423482076,-20.5339440109956,
12.));
#195641=CARTESIAN_POINT('Ctrl Pts',(-13.4027936954529,-20.5106201013753,
0.));
#195642=CARTESIAN_POINT('Ctrl Pts',(-13.4027936954529,-20.5106201013753,
12.));
#195643=CARTESIAN_POINT('Ctrl Pts',(-13.3986031603716,-20.487393518404,
0.));
#195644=CARTESIAN_POINT('Ctrl Pts',(-13.3986031603716,-20.487393518404,
12.));
#195645=CARTESIAN_POINT('Ctrl Pts',(-13.3943711603739,-20.4642647920037,
0.));
#195646=CARTESIAN_POINT('Ctrl Pts',(-13.3943711603739,-20.4642647920037,
12.));
#195647=CARTESIAN_POINT('Ctrl Pts',(-13.3900981177255,-20.4412344560007,
0.));
#195648=CARTESIAN_POINT('Ctrl Pts',(-13.3900981177255,-20.4412344560007,
12.));
#195649=CARTESIAN_POINT('Ctrl Pts',(-13.3857844596387,-20.4183030482002,
0.));
#195650=CARTESIAN_POINT('Ctrl Pts',(-13.3857844596387,-20.4183030482002,
12.));
#195651=CARTESIAN_POINT('Ctrl Pts',(-13.3814306183719,-20.3954711104502,
0.));
#195652=CARTESIAN_POINT('Ctrl Pts',(-13.3814306183719,-20.3954711104502,
12.));
#195653=CARTESIAN_POINT('Ctrl Pts',(-13.3770370313188,-20.3727391887184,
0.));
#195654=CARTESIAN_POINT('Ctrl Pts',(-13.3770370313188,-20.3727391887184,
12.));
#195655=CARTESIAN_POINT('Ctrl Pts',(-13.3726041410867,-20.3501078331814,
0.));
#195656=CARTESIAN_POINT('Ctrl Pts',(-13.3726041410867,-20.3501078331814,
12.));
#195657=CARTESIAN_POINT('Ctrl Pts',(-13.3681323955826,-20.3275775983029,
0.));
#195658=CARTESIAN_POINT('Ctrl Pts',(-13.3681323955826,-20.3275775983029,
12.));
#195659=CARTESIAN_POINT('Ctrl Pts',(-13.3636222481016,-20.3051490429048,
0.));
#195660=CARTESIAN_POINT('Ctrl Pts',(-13.3636222481016,-20.3051490429048,
12.));
#195661=CARTESIAN_POINT('Ctrl Pts',(-13.3590741574195,-20.2828227302339,
0.));
#195662=CARTESIAN_POINT('Ctrl Pts',(-13.3590741574195,-20.2828227302339,
12.));
#195663=CARTESIAN_POINT('Ctrl Pts',(-13.3544885878889,-20.2605992280122,
0.));
#195664=CARTESIAN_POINT('Ctrl Pts',(-13.3544885878889,-20.2605992280122,
12.));
#195665=CARTESIAN_POINT('Ctrl Pts',(-13.3498660095386,-20.2384791085359,
0.));
#195666=CARTESIAN_POINT('Ctrl Pts',(-13.3498660095386,-20.2384791085359,
12.));
#195667=CARTESIAN_POINT('Ctrl Pts',(-13.3452068981766,-20.216462948786,
0.));
#195668=CARTESIAN_POINT('Ctrl Pts',(-13.3452068981766,-20.216462948786,
12.));
#195669=CARTESIAN_POINT('Ctrl Pts',(-13.3405117354971,-20.1945513305235,
0.));
#195670=CARTESIAN_POINT('Ctrl Pts',(-13.3405117354971,-20.1945513305235,
12.));
#195671=CARTESIAN_POINT('Ctrl Pts',(-13.3357810091903,-20.1727448403817,
0.));
#195672=CARTESIAN_POINT('Ctrl Pts',(-13.3357810091903,-20.1727448403817,
12.));
#195673=CARTESIAN_POINT('Ctrl Pts',(-13.3310152130564,-20.1510440699474,
0.));
#195674=CARTESIAN_POINT('Ctrl Pts',(-13.3310152130564,-20.1510440699474,
12.));
#195675=CARTESIAN_POINT('Ctrl Pts',(-13.3262148471226,-20.1294496158402,
0.));
#195676=CARTESIAN_POINT('Ctrl Pts',(-13.3262148471226,-20.1294496158402,
12.));
#195677=CARTESIAN_POINT('Ctrl Pts',(-13.3213804177587,-20.1079620798375,
0.));
#195678=CARTESIAN_POINT('Ctrl Pts',(-13.3213804177587,-20.1079620798375,
12.));
#195679=CARTESIAN_POINT('Ctrl Pts',(-13.3165124377963,-20.0865820689882,
0.));
#195680=CARTESIAN_POINT('Ctrl Pts',(-13.3165124377963,-20.0865820689882,
12.));
#195681=CARTESIAN_POINT('Ctrl Pts',(-13.3116114266515,-20.0653101957188,
0.));
#195682=CARTESIAN_POINT('Ctrl Pts',(-13.3116114266515,-20.0653101957188,
12.));
#195683=CARTESIAN_POINT('Ctrl Pts',(-13.3066779104515,-20.0441470779345,
0.));
#195684=CARTESIAN_POINT('Ctrl Pts',(-13.3066779104515,-20.0441470779345,
12.));
#195685=CARTESIAN_POINT('Ctrl Pts',(-13.3017124221637,-20.0230933391038,
0.));
#195686=CARTESIAN_POINT('Ctrl Pts',(-13.3017124221637,-20.0230933391038,
12.));
#195687=CARTESIAN_POINT('Ctrl Pts',(-13.2967155017306,-20.0021496083738,
0.));
#195688=CARTESIAN_POINT('Ctrl Pts',(-13.2967155017306,-20.0021496083738,
12.));
#195689=CARTESIAN_POINT('Ctrl Pts',(-13.2916876962094,-19.981316520717,
0.));
#195690=CARTESIAN_POINT('Ctrl Pts',(-13.2916876962094,-19.981316520717,
12.));
#195691=CARTESIAN_POINT('Ctrl Pts',(-13.286629559915,-19.9605947170586,
0.));
#195692=CARTESIAN_POINT('Ctrl Pts',(-13.286629559915,-19.9605947170586,
12.));
#195693=CARTESIAN_POINT('Ctrl Pts',(-13.2815416545663,-19.9399848444019,
0.));
#195694=CARTESIAN_POINT('Ctrl Pts',(-13.2815416545663,-19.9399848444019,
12.));
#195695=CARTESIAN_POINT('Ctrl Pts',(-13.2764245494357,-19.9194875559422,
0.));
#195696=CARTESIAN_POINT('Ctrl Pts',(-13.2764245494357,-19.9194875559422,
12.));
#195697=CARTESIAN_POINT('Ctrl Pts',(-13.271278821502,-19.8991035111745,
0.));
#195698=CARTESIAN_POINT('Ctrl Pts',(-13.271278821502,-19.8991035111745,
12.));
#195699=CARTESIAN_POINT('Ctrl Pts',(-13.2661050556132,-19.8788333760577,
0.));
#195700=CARTESIAN_POINT('Ctrl Pts',(-13.2661050556132,-19.8788333760577,
12.));
#195701=CARTESIAN_POINT('Ctrl Pts',(-13.2609038446529,-19.8586778231715,
0.));
#195702=CARTESIAN_POINT('Ctrl Pts',(-13.2609038446529,-19.8586778231715,
12.));
#195703=CARTESIAN_POINT('Ctrl Pts',(-13.2556757897086,-19.8386375318634,
0.));
#195704=CARTESIAN_POINT('Ctrl Pts',(-13.2556757897086,-19.8386375318634,
12.));
#195705=CARTESIAN_POINT('Ctrl Pts',(-13.2504215002457,-19.8187131883917,
0.));
#195706=CARTESIAN_POINT('Ctrl Pts',(-13.2504215002457,-19.8187131883917,
12.));
#195707=CARTESIAN_POINT('Ctrl Pts',(-13.2451415942805,-19.7989054860495,
0.));
#195708=CARTESIAN_POINT('Ctrl Pts',(-13.2451415942805,-19.7989054860495,
12.));
#195709=CARTESIAN_POINT('Ctrl Pts',(-13.2398366985675,-19.7792151253289,
0.));
#195710=CARTESIAN_POINT('Ctrl Pts',(-13.2398366985675,-19.7792151253289,
12.));
#195711=CARTESIAN_POINT('Ctrl Pts',(-13.2345074487963,-19.7596428141168,
0.));
#195712=CARTESIAN_POINT('Ctrl Pts',(-13.2345074487963,-19.7596428141168,
12.));
#195713=CARTESIAN_POINT('Ctrl Pts',(-13.2291544897899,-19.7401892678697,
0.));
#195714=CARTESIAN_POINT('Ctrl Pts',(-13.2291544897899,-19.7401892678697,
12.));
#195715=CARTESIAN_POINT('Ctrl Pts',(-13.2237784757066,-19.7208552097868,
0.));
#195716=CARTESIAN_POINT('Ctrl Pts',(-13.2237784757066,-19.7208552097868,
12.));
#195717=CARTESIAN_POINT('Ctrl Pts',(-13.2183800702436,-19.7016413709685,
0.));
#195718=CARTESIAN_POINT('Ctrl Pts',(-13.2183800702436,-19.7016413709685,
12.));
#195719=CARTESIAN_POINT('Ctrl Pts',(-13.2129599468485,-19.6825484905823,
0.));
#195720=CARTESIAN_POINT('Ctrl Pts',(-13.2129599468485,-19.6825484905823,
12.));
#195721=CARTESIAN_POINT('Ctrl Pts',(-13.2075187889529,-19.6635773160936,
0.));
#195722=CARTESIAN_POINT('Ctrl Pts',(-13.2075187889529,-19.6635773160936,
12.));
#195723=CARTESIAN_POINT('Ctrl Pts',(-13.2020572902065,-19.6447286034772,
0.));
#195724=CARTESIAN_POINT('Ctrl Pts',(-13.2020572902065,-19.6447286034772,
12.));
#195725=CARTESIAN_POINT('Ctrl Pts',(-13.1965761547151,-19.6260031174244,
0.));
#195726=CARTESIAN_POINT('Ctrl Pts',(-13.1965761547151,-19.6260031174244,
12.));
#195727=CARTESIAN_POINT('Ctrl Pts',(-13.1910760972814,-19.6074016315414,
0.));
#195728=CARTESIAN_POINT('Ctrl Pts',(-13.1910760972814,-19.6074016315414,
12.));
#195729=CARTESIAN_POINT('Ctrl Pts',(-13.1855578436471,-19.5889249285338,
0.));
#195730=CARTESIAN_POINT('Ctrl Pts',(-13.1855578436471,-19.5889249285338,
12.));
#195731=CARTESIAN_POINT('Ctrl Pts',(-13.1800221307673,-19.5705738004667,
0.));
#195732=CARTESIAN_POINT('Ctrl Pts',(-13.1800221307673,-19.5705738004667,
12.));
#195733=CARTESIAN_POINT('Ctrl Pts',(-13.1744697070911,-19.5523490490244,
0.));
#195734=CARTESIAN_POINT('Ctrl Pts',(-13.1744697070911,-19.5523490490244,
12.));
#195735=CARTESIAN_POINT('Ctrl Pts',(-13.1689013328431,-19.5342514857562,
0.));
#195736=CARTESIAN_POINT('Ctrl Pts',(-13.1689013328431,-19.5342514857562,
12.));
#195737=CARTESIAN_POINT('Ctrl Pts',(-13.1633177803101,-19.5162819323213,
0.));
#195738=CARTESIAN_POINT('Ctrl Pts',(-13.1633177803101,-19.5162819323213,
12.));
#195739=CARTESIAN_POINT('Ctrl Pts',(-13.1577198341245,-19.4984412207081,
0.));
#195740=CARTESIAN_POINT('Ctrl Pts',(-13.1577198341245,-19.4984412207081,
12.));
#195741=CARTESIAN_POINT('Ctrl Pts',(-13.1521082915853,-19.4807301935268,
0.));
#195742=CARTESIAN_POINT('Ctrl Pts',(-13.1521082915853,-19.4807301935268,
12.));
#195743=CARTESIAN_POINT('Ctrl Pts',(-13.1464839629971,-19.4631497043258,
0.));
#195744=CARTESIAN_POINT('Ctrl Pts',(-13.1464839629971,-19.4631497043258,
12.));
#195745=CARTESIAN_POINT('Ctrl Pts',(-13.1408476720061,-19.4457006178876,
0.));
#195746=CARTESIAN_POINT('Ctrl Pts',(-13.1408476720061,-19.4457006178876,
12.));
#195747=CARTESIAN_POINT('Ctrl Pts',(-13.1352002559438,-19.4283838105262,
0.));
#195748=CARTESIAN_POINT('Ctrl Pts',(-13.1352002559438,-19.4283838105262,
12.));
#195749=CARTESIAN_POINT('Ctrl Pts',(-13.1295425661634,-19.4112001703557,
0.));
#195750=CARTESIAN_POINT('Ctrl Pts',(-13.1295425661634,-19.4112001703557,
12.));
#195751=CARTESIAN_POINT('Ctrl Pts',(-13.1238754684177,-19.3941505976263,
0.));
#195752=CARTESIAN_POINT('Ctrl Pts',(-13.1238754684177,-19.3941505976263,
12.));
#195753=CARTESIAN_POINT('Ctrl Pts',(-13.118199843271,-19.3772360051091,
0.));
#195754=CARTESIAN_POINT('Ctrl Pts',(-13.118199843271,-19.3772360051091,
12.));
#195755=CARTESIAN_POINT('Ctrl Pts',(-13.1125165865022,-19.3604573184515,
0.));
#195756=CARTESIAN_POINT('Ctrl Pts',(-13.1125165865022,-19.3604573184515,
12.));
#195757=CARTESIAN_POINT('Ctrl Pts',(-13.1068266095186,-19.3438154765395,
0.));
#195758=CARTESIAN_POINT('Ctrl Pts',(-13.1068266095186,-19.3438154765395,
12.));
#195759=CARTESIAN_POINT('Ctrl Pts',(-13.1011308397591,-19.3273114318269,
0.));
#195760=CARTESIAN_POINT('Ctrl Pts',(-13.1011308397591,-19.3273114318269,
12.));
#195761=CARTESIAN_POINT('Ctrl Pts',(-13.0954302211479,-19.310946150736,
0.));
#195762=CARTESIAN_POINT('Ctrl Pts',(-13.0954302211479,-19.310946150736,
12.));
#195763=CARTESIAN_POINT('Ctrl Pts',(-13.0897257145969,-19.2947206141247,
0.));
#195764=CARTESIAN_POINT('Ctrl Pts',(-13.0897257145969,-19.2947206141247,
12.));
#195765=CARTESIAN_POINT('Ctrl Pts',(-13.0840182984949,-19.2786358177198,
0.));
#195766=CARTESIAN_POINT('Ctrl Pts',(-13.0840182984949,-19.2786358177198,
12.));
#195767=CARTESIAN_POINT('Ctrl Pts',(-13.0783089692118,-19.2626927725596,
0.));
#195768=CARTESIAN_POINT('Ctrl Pts',(-13.0783089692118,-19.2626927725596,
12.));
#195769=CARTESIAN_POINT('Ctrl Pts',(-13.0725987415859,-19.2468925053989,
0.));
#195770=CARTESIAN_POINT('Ctrl Pts',(-13.0725987415859,-19.2468925053989,
12.));
#195771=CARTESIAN_POINT('Ctrl Pts',(-13.0668886494795,-19.2312360592033,
0.));
#195772=CARTESIAN_POINT('Ctrl Pts',(-13.0668886494795,-19.2312360592033,
12.));
#195773=CARTESIAN_POINT('Ctrl Pts',(-13.0611797463915,-19.2157244937142,
0.));
#195774=CARTESIAN_POINT('Ctrl Pts',(-13.0611797463915,-19.2157244937142,
12.));
#195775=CARTESIAN_POINT('Ctrl Pts',(-13.0554731060538,-19.2003588859772,
0.));
#195776=CARTESIAN_POINT('Ctrl Pts',(-13.0554731060538,-19.2003588859772,
12.));
#195777=CARTESIAN_POINT('Ctrl Pts',(-13.0497698230441,-19.1851403308825,
0.));
#195778=CARTESIAN_POINT('Ctrl Pts',(-13.0497698230441,-19.1851403308825,
12.));
#195779=CARTESIAN_POINT('Ctrl Pts',(-13.0440710133772,-19.1700699416622,
0.));
#195780=CARTESIAN_POINT('Ctrl Pts',(-13.0440710133772,-19.1700699416622,
12.));
#195781=CARTESIAN_POINT('Ctrl Pts',(-13.0383778152068,-19.155148850523,
0.));
#195782=CARTESIAN_POINT('Ctrl Pts',(-13.0383778152068,-19.155148850523,
12.));
#195783=CARTESIAN_POINT('Ctrl Pts',(-13.0326913895838,-19.1403782093386,
0.));
#195784=CARTESIAN_POINT('Ctrl Pts',(-13.0326913895838,-19.1403782093386,
12.));
#195785=CARTESIAN_POINT('Ctrl Pts',(-13.0270129211976,-19.1257591903099,
0.));
#195786=CARTESIAN_POINT('Ctrl Pts',(-13.0270129211976,-19.1257591903099,
12.));
#195787=CARTESIAN_POINT('Ctrl Pts',(-13.0213436191328,-19.111292986631,
0.));
#195788=CARTESIAN_POINT('Ctrl Pts',(-13.0213436191328,-19.111292986631,
12.));
#195789=CARTESIAN_POINT('Ctrl Pts',(-13.0156847176097,-19.0969808131228,
0.));
#195790=CARTESIAN_POINT('Ctrl Pts',(-13.0156847176097,-19.0969808131228,
12.));
#195791=CARTESIAN_POINT('Ctrl Pts',(-13.0100374768788,-19.0828239070484,
0.));
#195792=CARTESIAN_POINT('Ctrl Pts',(-13.0100374768788,-19.0828239070484,
12.));
#195793=CARTESIAN_POINT('Ctrl Pts',(-13.0044031841382,-19.0688235289437,
0.));
#195794=CARTESIAN_POINT('Ctrl Pts',(-13.0044031841382,-19.0688235289437,
12.));
#195795=CARTESIAN_POINT('Ctrl Pts',(-12.9987831544502,-19.0549809634354,
0.));
#195796=CARTESIAN_POINT('Ctrl Pts',(-12.9987831544502,-19.0549809634354,
12.));
#195797=CARTESIAN_POINT('Ctrl Pts',(-12.9931787316514,-19.0412975200398,
0.));
#195798=CARTESIAN_POINT('Ctrl Pts',(-12.9931787316514,-19.0412975200398,
12.));
#195799=CARTESIAN_POINT('Ctrl Pts',(-12.9875912893003,-19.0277745339908,
0.));
#195800=CARTESIAN_POINT('Ctrl Pts',(-12.9875912893003,-19.0277745339908,
12.));
#195801=CARTESIAN_POINT('Ctrl Pts',(-12.9820222318716,-19.014413367335,
0.));
#195802=CARTESIAN_POINT('Ctrl Pts',(-12.9820222318716,-19.014413367335,
12.));
#195803=CARTESIAN_POINT('Ctrl Pts',(-12.9764729959206,-19.0012154099792,
0.));
#195804=CARTESIAN_POINT('Ctrl Pts',(-12.9764729959206,-19.0012154099792,
12.));
#195805=CARTESIAN_POINT('Ctrl Pts',(-12.9709450512747,-18.9881820807585,
0.));
#195806=CARTESIAN_POINT('Ctrl Pts',(-12.9709450512747,-18.9881820807585,
12.));
#195807=CARTESIAN_POINT('Ctrl Pts',(-12.9654399021868,-18.9753148284473,
0.));
#195808=CARTESIAN_POINT('Ctrl Pts',(-12.9654399021868,-18.9753148284473,
12.));
#195809=CARTESIAN_POINT('Ctrl Pts',(-12.9599590886318,-18.9626151329226,
0.));
#195810=CARTESIAN_POINT('Ctrl Pts',(-12.9599590886318,-18.9626151329226,
12.));
#195811=CARTESIAN_POINT('Ctrl Pts',(-12.9545041877377,-18.9500845064714,
0.));
#195812=CARTESIAN_POINT('Ctrl Pts',(-12.9545041877377,-18.9500845064714,
12.));
#195813=CARTESIAN_POINT('Ctrl Pts',(-12.9490768151821,-18.9377244950435,
0.));
#195814=CARTESIAN_POINT('Ctrl Pts',(-12.9490768151821,-18.9377244950435,
12.));
#195815=CARTESIAN_POINT('Ctrl Pts',(-12.9436786266106,-18.9255366795196,
0.));
#195816=CARTESIAN_POINT('Ctrl Pts',(-12.9436786266106,-18.9255366795196,
12.));
#195817=CARTESIAN_POINT('Ctrl Pts',(-12.9383113190375,-18.9135226769466,
0.));
#195818=CARTESIAN_POINT('Ctrl Pts',(-12.9383113190375,-18.9135226769466,
12.));
#195819=CARTESIAN_POINT('Ctrl Pts',(-12.9329766328184,-18.9016841423402,
0.));
#195820=CARTESIAN_POINT('Ctrl Pts',(-12.9329766328184,-18.9016841423402,
12.));
#195821=CARTESIAN_POINT('Ctrl Pts',(-12.9276763536373,-18.8900227704888,
0.));
#195822=CARTESIAN_POINT('Ctrl Pts',(-12.9276763536373,-18.8900227704888,
12.));
#195823=CARTESIAN_POINT('Ctrl Pts',(-12.9224123144982,-18.8785402977528,
0.));
#195824=CARTESIAN_POINT('Ctrl Pts',(-12.9224123144982,-18.8785402977528,
12.));
#195825=CARTESIAN_POINT('Ctrl Pts',(-12.9171863977047,-18.8672385038328,
0.));
#195826=CARTESIAN_POINT('Ctrl Pts',(-12.9171863977047,-18.8672385038328,
12.));
#195827=CARTESIAN_POINT('Ctrl Pts',(-12.9120005369066,-18.8561192136201,
0.));
#195828=CARTESIAN_POINT('Ctrl Pts',(-12.9120005369066,-18.8561192136201,
12.));
#195829=CARTESIAN_POINT('Ctrl Pts',(-12.9068567191856,-18.8451842990986,
0.));
#195830=CARTESIAN_POINT('Ctrl Pts',(-12.9068567191856,-18.8451842990986,
12.));
#195831=CARTESIAN_POINT('Ctrl Pts',(-12.9017569871738,-18.834435681259,
0.));
#195832=CARTESIAN_POINT('Ctrl Pts',(-12.9017569871738,-18.834435681259,
12.));
#195833=CARTESIAN_POINT('Ctrl Pts',(-12.8967034410752,-18.8238753319124,
0.));
#195834=CARTESIAN_POINT('Ctrl Pts',(-12.8967034410752,-18.8238753319124,
12.));
#195835=CARTESIAN_POINT('Ctrl Pts',(-12.8916982409931,-18.8135052757815,
0.));
#195836=CARTESIAN_POINT('Ctrl Pts',(-12.8916982409931,-18.8135052757815,
12.));
#195837=CARTESIAN_POINT('Ctrl Pts',(-12.8867436109543,-18.8033275941939,
0.));
#195838=CARTESIAN_POINT('Ctrl Pts',(-12.8867436109543,-18.8033275941939,
12.));
#195839=CARTESIAN_POINT('Ctrl Pts',(-12.8818418427474,-18.7933444285867,
0.));
#195840=CARTESIAN_POINT('Ctrl Pts',(-12.8818418427474,-18.7933444285867,
12.));
#195841=CARTESIAN_POINT('Ctrl Pts',(-12.8769952998097,-18.7835579840481,
0.));
#195842=CARTESIAN_POINT('Ctrl Pts',(-12.8769952998097,-18.7835579840481,
12.));
#195843=CARTESIAN_POINT('Ctrl Pts',(-12.8722064211814,-18.7739705329028,
0.));
#195844=CARTESIAN_POINT('Ctrl Pts',(-12.8722064211814,-18.7739705329028,
12.));
#195845=CARTESIAN_POINT('Ctrl Pts',(-12.8674777239656,-18.7645844169568,
0.));
#195846=CARTESIAN_POINT('Ctrl Pts',(-12.8674777239656,-18.7645844169568,
12.));
#195847=CARTESIAN_POINT('Ctrl Pts',(-12.8628118054172,-18.7554020493888,
0.));
#195848=CARTESIAN_POINT('Ctrl Pts',(-12.8628118054172,-18.7554020493888,
12.));
#195849=CARTESIAN_POINT('Ctrl Pts',(-12.8582113455645,-18.7464259171248,
0.));
#195850=CARTESIAN_POINT('Ctrl Pts',(-12.8582113455645,-18.7464259171248,
12.));
#195851=CARTESIAN_POINT('Ctrl Pts',(-12.8536791086315,-18.7376585820851,
0.));
#195852=CARTESIAN_POINT('Ctrl Pts',(-12.8536791086315,-18.7376585820851,
12.));
#195853=CARTESIAN_POINT('Ctrl Pts',(-12.849217951159,-18.7291026886552,
0.));
#195854=CARTESIAN_POINT('Ctrl Pts',(-12.849217951159,-18.7291026886552,
12.));
#195855=CARTESIAN_POINT('Ctrl Pts',(-12.8448308329494,-18.7207609737701,
0.));
#195856=CARTESIAN_POINT('Ctrl Pts',(-12.8448308329494,-18.7207609737701,
12.));
#195857=CARTESIAN_POINT('Ctrl Pts',(-12.8405208263432,-18.7126362754446,
0.));
#195858=CARTESIAN_POINT('Ctrl Pts',(-12.8405208263432,-18.7126362754446,
12.));
#195859=CARTESIAN_POINT('Ctrl Pts',(-12.8362911280362,-18.7047315436296,
0.));
#195860=CARTESIAN_POINT('Ctrl Pts',(-12.8362911280362,-18.7047315436296,
12.));
#195861=CARTESIAN_POINT('Ctrl Pts',(-12.832145059979,-18.6970498410173,
0.));
#195862=CARTESIAN_POINT('Ctrl Pts',(-12.832145059979,-18.6970498410173,
12.));
#195863=CARTESIAN_POINT('Ctrl Pts',(-12.8280860635231,-18.6895943376172,
0.));
#195864=CARTESIAN_POINT('Ctrl Pts',(-12.8280860635231,-18.6895943376172,
12.));
#195865=CARTESIAN_POINT('Ctrl Pts',(-12.8241176980016,-18.6823683094138,
0.));
#195866=CARTESIAN_POINT('Ctrl Pts',(-12.8241176980016,-18.6823683094138,
12.));
#195867=CARTESIAN_POINT('Ctrl Pts',(-12.8202436318473,-18.6753751301091,
0.));
#195868=CARTESIAN_POINT('Ctrl Pts',(-12.8202436318473,-18.6753751301091,
12.));
#195869=CARTESIAN_POINT('Ctrl Pts',(-12.8164676687361,-18.6686182952798,
0.));
#195870=CARTESIAN_POINT('Ctrl Pts',(-12.8164676687361,-18.6686182952798,
12.));
#195871=CARTESIAN_POINT('Ctrl Pts',(-12.8127937909632,-18.6621014624746,
0.));
#195872=CARTESIAN_POINT('Ctrl Pts',(-12.8127937909632,-18.6621014624746,
12.));
#195873=CARTESIAN_POINT('Ctrl Pts',(-12.8092261933858,-18.6558284825772,
0.));
#195874=CARTESIAN_POINT('Ctrl Pts',(-12.8092261933858,-18.6558284825772,
12.));
#195875=CARTESIAN_POINT('Ctrl Pts',(-12.805769331162,-18.6498034438986,
0.));
#195876=CARTESIAN_POINT('Ctrl Pts',(-12.805769331162,-18.6498034438986,
12.));
#195877=CARTESIAN_POINT('Ctrl Pts',(-12.8024278770153,-18.6440306327457,
0.));
#195878=CARTESIAN_POINT('Ctrl Pts',(-12.8024278770153,-18.6440306327457,
12.));
#195879=CARTESIAN_POINT('Ctrl Pts',(-12.7992066625264,-18.63851447924,0.));
#195880=CARTESIAN_POINT('Ctrl Pts',(-12.7992066625264,-18.63851447924,12.));
#195881=CARTESIAN_POINT('Ctrl Pts',(-12.7961106222251,-18.6332595057005,
0.));
#195882=CARTESIAN_POINT('Ctrl Pts',(-12.7961106222251,-18.6332595057005,
12.));
#195883=CARTESIAN_POINT('Ctrl Pts',(-12.7931447451556,-18.6282702819371,
0.));
#195884=CARTESIAN_POINT('Ctrl Pts',(-12.7931447451556,-18.6282702819371,
12.));
#195885=CARTESIAN_POINT('Ctrl Pts',(-12.7903142925235,-18.6235516265575,
0.));
#195886=CARTESIAN_POINT('Ctrl Pts',(-12.7903142925235,-18.6235516265575,
12.));
#195887=CARTESIAN_POINT('Ctrl Pts',(-12.7876249657834,-18.6191087624752,
0.));
#195888=CARTESIAN_POINT('Ctrl Pts',(-12.7876249657834,-18.6191087624752,
12.));
#195889=CARTESIAN_POINT('Ctrl Pts',(-12.78508316579,-18.6149475565189,0.));
#195890=CARTESIAN_POINT('Ctrl Pts',(-12.78508316579,-18.6149475565189,12.));
#195891=CARTESIAN_POINT('Ctrl Pts',(-12.7826959526924,-18.611074482622,
0.));
#195892=CARTESIAN_POINT('Ctrl Pts',(-12.7826959526924,-18.611074482622,
12.));
#195893=CARTESIAN_POINT('Ctrl Pts',(-12.7804705387658,-18.6074961535723,
0.));
#195894=CARTESIAN_POINT('Ctrl Pts',(-12.7804705387658,-18.6074961535723,
12.));
#195895=CARTESIAN_POINT('Ctrl Pts',(-12.7784139605067,-18.6042190183703,
0.));
#195896=CARTESIAN_POINT('Ctrl Pts',(-12.7784139605067,-18.6042190183703,
12.));
#195897=CARTESIAN_POINT('Ctrl Pts',(-12.7765325225083,-18.6012488486708,
0.));
#195898=CARTESIAN_POINT('Ctrl Pts',(-12.7765325225083,-18.6012488486708,
12.));
#195899=CARTESIAN_POINT('Ctrl Pts',(-12.7748328937639,-18.5985917525949,
0.));
#195900=CARTESIAN_POINT('Ctrl Pts',(-12.7748328937639,-18.5985917525949,
12.));
#195901=CARTESIAN_POINT('Ctrl Pts',(-12.7733231262107,-18.5962551167772,
0.));
#195902=CARTESIAN_POINT('Ctrl Pts',(-12.7733231262107,-18.5962551167772,
12.));
#195903=CARTESIAN_POINT('Ctrl Pts',(-12.7720142287169,-18.5942490615409,
0.));
#195904=CARTESIAN_POINT('Ctrl Pts',(-12.7720142287169,-18.5942490615409,
12.));
#195905=CARTESIAN_POINT('Ctrl Pts',(-12.7709195951154,-18.5925859134582,
0.));
#195906=CARTESIAN_POINT('Ctrl Pts',(-12.7709195951154,-18.5925859134582,
12.));
#195907=CARTESIAN_POINT('Ctrl Pts',(-12.7700520897174,-18.5912775137806,
0.));
#195908=CARTESIAN_POINT('Ctrl Pts',(-12.7700520897174,-18.5912775137806,
12.));
#195909=CARTESIAN_POINT('Ctrl Pts',(-12.7694215127923,-18.590332877722,
0.));
#195910=CARTESIAN_POINT('Ctrl Pts',(-12.7694215127923,-18.590332877722,
12.));
#195911=CARTESIAN_POINT('Ctrl Pts',(-12.7691103481996,-18.589871621842,
0.));
#195912=CARTESIAN_POINT('Ctrl Pts',(-12.7691103481996,-18.589871621842,
12.));
#195913=CARTESIAN_POINT('Ctrl Pts',(-12.7689864266924,-18.5896919669158,
0.));
#195914=CARTESIAN_POINT('Ctrl Pts',(-12.7689864266924,-18.5896919669158,
12.));
#195915=CARTESIAN_POINT('Ctrl Pts',(-12.7689524524484,-18.5896460962961,
0.));
#195916=CARTESIAN_POINT('Ctrl Pts',(-12.7689524524484,-18.5896460962961,
12.));
#195917=CARTESIAN_POINT('Ctrl Pts',(-12.7689476255363,-18.5896416359912,
0.));
#195918=CARTESIAN_POINT('Ctrl Pts',(-12.7689476255363,-18.5896416359912,
12.));
#195919=CARTESIAN_POINT('',(-13.5685075571671,-22.1787195904339,0.));
#195920=CARTESIAN_POINT('Ctrl Pts',(-13.5685075571671,-22.1787195904339,
0.));
#195921=CARTESIAN_POINT('Ctrl Pts',(-13.5683460612913,-22.1730081264583,
0.));
#195922=CARTESIAN_POINT('Ctrl Pts',(-13.5680170531724,-22.1615922804939,
0.));
#195923=CARTESIAN_POINT('Ctrl Pts',(-13.5675054918922,-22.1444897575076,
0.));
#195924=CARTESIAN_POINT('Ctrl Pts',(-13.5667873105179,-22.1217288871823,
0.));
#195925=CARTESIAN_POINT('Ctrl Pts',(-13.5658294169107,-22.0933486464442,
0.));
#195926=CARTESIAN_POINT('Ctrl Pts',(-13.5648113688895,-22.0650393089492,
0.));
#195927=CARTESIAN_POINT('Ctrl Pts',(-13.5637332022393,-22.0368009736227,
0.));
#195928=CARTESIAN_POINT('Ctrl Pts',(-13.5625949868313,-22.0086337943431,
0.));
#195929=CARTESIAN_POINT('Ctrl Pts',(-13.5613968357589,-21.9805379899192,
0.));
#195930=CARTESIAN_POINT('Ctrl Pts',(-13.5601389185315,-21.9525138592862,
0.));
#195931=CARTESIAN_POINT('Ctrl Pts',(-13.5588214586672,-21.9245617765827,
0.));
#195932=CARTESIAN_POINT('Ctrl Pts',(-13.5574447178485,-21.8966821688876,
0.));
#195933=CARTESIAN_POINT('Ctrl Pts',(-13.5560089839426,-21.8688754989401,
0.));
#195934=CARTESIAN_POINT('Ctrl Pts',(-13.5545145573049,-21.841142245609,
0.));
#195935=CARTESIAN_POINT('Ctrl Pts',(-13.5529617381569,-21.8134828857963,
0.));
#195936=CARTESIAN_POINT('Ctrl Pts',(-13.5513508127232,-21.7858978745848,
0.));
#195937=CARTESIAN_POINT('Ctrl Pts',(-13.5496820422187,-21.7583876294532,
0.));
#195938=CARTESIAN_POINT('Ctrl Pts',(-13.5479556704457,-21.730952541226,
0.));
#195939=CARTESIAN_POINT('Ctrl Pts',(-13.546171929503,-21.7035929822939,
0.));
#195940=CARTESIAN_POINT('Ctrl Pts',(-13.5443310461516,-21.676309315769,
0.));
#195941=CARTESIAN_POINT('Ctrl Pts',(-13.5424332480698,-21.6491019044647,
0.));
#195942=CARTESIAN_POINT('Ctrl Pts',(-13.5404787697798,-21.6219711193951,
0.));
#195943=CARTESIAN_POINT('Ctrl Pts',(-13.5384678597206,-21.5949173499022,
0.));
#195944=CARTESIAN_POINT('Ctrl Pts',(-13.5364007790292,-21.5679410019011,
0.));
#195945=CARTESIAN_POINT('Ctrl Pts',(-13.5342777983225,-21.5410424932511,
0.));
#195946=CARTESIAN_POINT('Ctrl Pts',(-13.5320991952145,-21.5142222501671,
0.));
#195947=CARTESIAN_POINT('Ctrl Pts',(-13.5298652514357,-21.487480703047,
0.));
#195948=CARTESIAN_POINT('Ctrl Pts',(-13.5275762503553,-21.4608182828695,
0.));
#195949=CARTESIAN_POINT('Ctrl Pts',(-13.5252324737795,-21.4342354165253,
0.));
#195950=CARTESIAN_POINT('Ctrl Pts',(-13.5228342013508,-21.4077325259318,
0.));
#195951=CARTESIAN_POINT('Ctrl Pts',(-13.5203817122497,-21.3813100304967,
0.));
#195952=CARTESIAN_POINT('Ctrl Pts',(-13.5178752862461,-21.3549683486219,
0.));
#195953=CARTESIAN_POINT('Ctrl Pts',(-13.5153152050554,-21.328707899634,
0.));
#195954=CARTESIAN_POINT('Ctrl Pts',(-13.5127017534972,-21.3025291054236,
0.));
#195955=CARTESIAN_POINT('Ctrl Pts',(-13.5100352209207,-21.2764323924442,
0.));
#195956=CARTESIAN_POINT('Ctrl Pts',(-13.5073159019454,-21.2504181927429,
0.));
#195957=CARTESIAN_POINT('Ctrl Pts',(-13.5045440957404,-21.224486942933,
0.));
#195958=CARTESIAN_POINT('Ctrl Pts',(-13.5017201056088,-21.1986390835825,
0.));
#195959=CARTESIAN_POINT('Ctrl Pts',(-13.4988442384491,-21.1728750584173,
0.));
#195960=CARTESIAN_POINT('Ctrl Pts',(-13.4959168042934,-21.1471953136209,
0.));
#195961=CARTESIAN_POINT('Ctrl Pts',(-13.4929381157778,-21.1216002970209,
0.));
#195962=CARTESIAN_POINT('Ctrl Pts',(-13.4899084877718,-21.0960904575048,
0.));
#195963=CARTESIAN_POINT('Ctrl Pts',(-13.4868282377192,-21.0706662455202,
0.));
#195964=CARTESIAN_POINT('Ctrl Pts',(-13.4836976858912,-21.0453281134247,
0.));
#195965=CARTESIAN_POINT('Ctrl Pts',(-13.4805171556822,-21.0200765158885,
0.));
#195966=CARTESIAN_POINT('Ctrl Pts',(-13.4772869738879,-20.9949119102592,
0.));
#195967=CARTESIAN_POINT('Ctrl Pts',(-13.4740074710087,-20.9698347569476,
0.));
#195968=CARTESIAN_POINT('Ctrl Pts',(-13.4706789815167,-20.9448455197557,
0.));
#195969=CARTESIAN_POINT('Ctrl Pts',(-13.4673018437718,-20.9199446657584,
0.));
#195970=CARTESIAN_POINT('Ctrl Pts',(-13.4638763999726,-20.8951326652158,
0.));
#195971=CARTESIAN_POINT('Ctrl Pts',(-13.4604029960983,-20.8704099914641,
0.));
#195972=CARTESIAN_POINT('Ctrl Pts',(-13.4568819818631,-20.8457771208082,
0.));
#195973=CARTESIAN_POINT('Ctrl Pts',(-13.4533137106667,-20.821234532398,
0.));
#195974=CARTESIAN_POINT('Ctrl Pts',(-13.4496985395637,-20.7967827081227,
0.));
#195975=CARTESIAN_POINT('Ctrl Pts',(-13.4460368293688,-20.7724221327608,
0.));
#195976=CARTESIAN_POINT('Ctrl Pts',(-13.4423289447561,-20.7481532941013,
0.));
#195977=CARTESIAN_POINT('Ctrl Pts',(-13.4385752543663,-20.7239766830675,
0.));
#195978=CARTESIAN_POINT('Ctrl Pts',(-13.4347761309154,-20.6998927938288,
0.));
#195979=CARTESIAN_POINT('Ctrl Pts',(-13.4309319513119,-20.6759021239103,
0.));
#195980=CARTESIAN_POINT('Ctrl Pts',(-13.4270430967652,-20.6520051742869,
0.));
#195981=CARTESIAN_POINT('Ctrl Pts',(-13.4231099528179,-20.6282024494237,
0.));
#195982=CARTESIAN_POINT('Ctrl Pts',(-13.4191329093933,-20.6044944573153,
0.));
#195983=CARTESIAN_POINT('Ctrl Pts',(-13.4151123608411,-20.5808817095155,
0.));
#195984=CARTESIAN_POINT('Ctrl Pts',(-13.4110487059912,-20.5573647211639,
0.));
#195985=CARTESIAN_POINT('Ctrl Pts',(-13.4069423482076,-20.5339440109956,
0.));
#195986=CARTESIAN_POINT('Ctrl Pts',(-13.4027936954529,-20.5106201013753,
0.));
#195987=CARTESIAN_POINT('Ctrl Pts',(-13.3986031603716,-20.487393518404,
0.));
#195988=CARTESIAN_POINT('Ctrl Pts',(-13.3943711603739,-20.4642647920037,
0.));
#195989=CARTESIAN_POINT('Ctrl Pts',(-13.3900981177255,-20.4412344560007,
0.));
#195990=CARTESIAN_POINT('Ctrl Pts',(-13.3857844596387,-20.4183030482002,
0.));
#195991=CARTESIAN_POINT('Ctrl Pts',(-13.3814306183719,-20.3954711104502,
0.));
#195992=CARTESIAN_POINT('Ctrl Pts',(-13.3770370313188,-20.3727391887184,
0.));
#195993=CARTESIAN_POINT('Ctrl Pts',(-13.3726041410867,-20.3501078331814,
0.));
#195994=CARTESIAN_POINT('Ctrl Pts',(-13.3681323955826,-20.3275775983029,
0.));
#195995=CARTESIAN_POINT('Ctrl Pts',(-13.3636222481016,-20.3051490429048,
0.));
#195996=CARTESIAN_POINT('Ctrl Pts',(-13.3590741574195,-20.2828227302339,
0.));
#195997=CARTESIAN_POINT('Ctrl Pts',(-13.3544885878889,-20.2605992280122,
0.));
#195998=CARTESIAN_POINT('Ctrl Pts',(-13.3498660095386,-20.2384791085359,
0.));
#195999=CARTESIAN_POINT('Ctrl Pts',(-13.3452068981766,-20.216462948786,
0.));
#196000=CARTESIAN_POINT('Ctrl Pts',(-13.3405117354971,-20.1945513305235,
0.));
#196001=CARTESIAN_POINT('Ctrl Pts',(-13.3357810091903,-20.1727448403817,
0.));
#196002=CARTESIAN_POINT('Ctrl Pts',(-13.3310152130564,-20.1510440699474,
0.));
#196003=CARTESIAN_POINT('Ctrl Pts',(-13.3262148471226,-20.1294496158402,
0.));
#196004=CARTESIAN_POINT('Ctrl Pts',(-13.3213804177587,-20.1079620798375,
0.));
#196005=CARTESIAN_POINT('Ctrl Pts',(-13.3165124377963,-20.0865820689882,
0.));
#196006=CARTESIAN_POINT('Ctrl Pts',(-13.3116114266515,-20.0653101957188,
0.));
#196007=CARTESIAN_POINT('Ctrl Pts',(-13.3066779104515,-20.0441470779345,
0.));
#196008=CARTESIAN_POINT('Ctrl Pts',(-13.3017124221637,-20.0230933391038,
0.));
#196009=CARTESIAN_POINT('Ctrl Pts',(-13.2967155017306,-20.0021496083738,
0.));
#196010=CARTESIAN_POINT('Ctrl Pts',(-13.2916876962094,-19.981316520717,
0.));
#196011=CARTESIAN_POINT('Ctrl Pts',(-13.286629559915,-19.9605947170586,
0.));
#196012=CARTESIAN_POINT('Ctrl Pts',(-13.2815416545663,-19.9399848444019,
0.));
#196013=CARTESIAN_POINT('Ctrl Pts',(-13.2764245494357,-19.9194875559422,
0.));
#196014=CARTESIAN_POINT('Ctrl Pts',(-13.271278821502,-19.8991035111745,
0.));
#196015=CARTESIAN_POINT('Ctrl Pts',(-13.2661050556132,-19.8788333760577,
0.));
#196016=CARTESIAN_POINT('Ctrl Pts',(-13.2609038446529,-19.8586778231715,
0.));
#196017=CARTESIAN_POINT('Ctrl Pts',(-13.2556757897086,-19.8386375318634,
0.));
#196018=CARTESIAN_POINT('Ctrl Pts',(-13.2504215002457,-19.8187131883917,
0.));
#196019=CARTESIAN_POINT('Ctrl Pts',(-13.2451415942805,-19.7989054860495,
0.));
#196020=CARTESIAN_POINT('Ctrl Pts',(-13.2398366985675,-19.7792151253289,
0.));
#196021=CARTESIAN_POINT('Ctrl Pts',(-13.2345074487963,-19.7596428141168,
0.));
#196022=CARTESIAN_POINT('Ctrl Pts',(-13.2291544897899,-19.7401892678697,
0.));
#196023=CARTESIAN_POINT('Ctrl Pts',(-13.2237784757066,-19.7208552097868,
0.));
#196024=CARTESIAN_POINT('Ctrl Pts',(-13.2183800702436,-19.7016413709685,
0.));
#196025=CARTESIAN_POINT('Ctrl Pts',(-13.2129599468485,-19.6825484905823,
0.));
#196026=CARTESIAN_POINT('Ctrl Pts',(-13.2075187889529,-19.6635773160936,
0.));
#196027=CARTESIAN_POINT('Ctrl Pts',(-13.2020572902065,-19.6447286034772,
0.));
#196028=CARTESIAN_POINT('Ctrl Pts',(-13.1965761547151,-19.6260031174244,
0.));
#196029=CARTESIAN_POINT('Ctrl Pts',(-13.1910760972814,-19.6074016315414,
0.));
#196030=CARTESIAN_POINT('Ctrl Pts',(-13.1855578436471,-19.5889249285338,
0.));
#196031=CARTESIAN_POINT('Ctrl Pts',(-13.1800221307673,-19.5705738004667,
0.));
#196032=CARTESIAN_POINT('Ctrl Pts',(-13.1744697070911,-19.5523490490244,
0.));
#196033=CARTESIAN_POINT('Ctrl Pts',(-13.1689013328431,-19.5342514857562,
0.));
#196034=CARTESIAN_POINT('Ctrl Pts',(-13.1633177803101,-19.5162819323213,
0.));
#196035=CARTESIAN_POINT('Ctrl Pts',(-13.1577198341245,-19.4984412207081,
0.));
#196036=CARTESIAN_POINT('Ctrl Pts',(-13.1521082915853,-19.4807301935268,
0.));
#196037=CARTESIAN_POINT('Ctrl Pts',(-13.1464839629971,-19.4631497043258,
0.));
#196038=CARTESIAN_POINT('Ctrl Pts',(-13.1408476720061,-19.4457006178876,
0.));
#196039=CARTESIAN_POINT('Ctrl Pts',(-13.1352002559438,-19.4283838105262,
0.));
#196040=CARTESIAN_POINT('Ctrl Pts',(-13.1295425661634,-19.4112001703557,
0.));
#196041=CARTESIAN_POINT('Ctrl Pts',(-13.1238754684177,-19.3941505976263,
0.));
#196042=CARTESIAN_POINT('Ctrl Pts',(-13.118199843271,-19.3772360051091,
0.));
#196043=CARTESIAN_POINT('Ctrl Pts',(-13.1125165865022,-19.3604573184515,
0.));
#196044=CARTESIAN_POINT('Ctrl Pts',(-13.1068266095186,-19.3438154765395,
0.));
#196045=CARTESIAN_POINT('Ctrl Pts',(-13.1011308397591,-19.3273114318269,
0.));
#196046=CARTESIAN_POINT('Ctrl Pts',(-13.0954302211479,-19.310946150736,
0.));
#196047=CARTESIAN_POINT('Ctrl Pts',(-13.0897257145969,-19.2947206141247,
0.));
#196048=CARTESIAN_POINT('Ctrl Pts',(-13.0840182984949,-19.2786358177198,
0.));
#196049=CARTESIAN_POINT('Ctrl Pts',(-13.0783089692118,-19.2626927725596,
0.));
#196050=CARTESIAN_POINT('Ctrl Pts',(-13.0725987415859,-19.2468925053989,
0.));
#196051=CARTESIAN_POINT('Ctrl Pts',(-13.0668886494795,-19.2312360592033,
0.));
#196052=CARTESIAN_POINT('Ctrl Pts',(-13.0611797463915,-19.2157244937142,
0.));
#196053=CARTESIAN_POINT('Ctrl Pts',(-13.0554731060538,-19.2003588859772,
0.));
#196054=CARTESIAN_POINT('Ctrl Pts',(-13.0497698230441,-19.1851403308825,
0.));
#196055=CARTESIAN_POINT('Ctrl Pts',(-13.0440710133772,-19.1700699416622,
0.));
#196056=CARTESIAN_POINT('Ctrl Pts',(-13.0383778152068,-19.155148850523,
0.));
#196057=CARTESIAN_POINT('Ctrl Pts',(-13.0326913895838,-19.1403782093386,
0.));
#196058=CARTESIAN_POINT('Ctrl Pts',(-13.0270129211976,-19.1257591903099,
0.));
#196059=CARTESIAN_POINT('Ctrl Pts',(-13.0213436191328,-19.111292986631,
0.));
#196060=CARTESIAN_POINT('Ctrl Pts',(-13.0156847176097,-19.0969808131228,
0.));
#196061=CARTESIAN_POINT('Ctrl Pts',(-13.0100374768788,-19.0828239070484,
0.));
#196062=CARTESIAN_POINT('Ctrl Pts',(-13.0044031841382,-19.0688235289437,
0.));
#196063=CARTESIAN_POINT('Ctrl Pts',(-12.9987831544502,-19.0549809634354,
0.));
#196064=CARTESIAN_POINT('Ctrl Pts',(-12.9931787316514,-19.0412975200398,
0.));
#196065=CARTESIAN_POINT('Ctrl Pts',(-12.9875912893003,-19.0277745339908,
0.));
#196066=CARTESIAN_POINT('Ctrl Pts',(-12.9820222318716,-19.014413367335,
0.));
#196067=CARTESIAN_POINT('Ctrl Pts',(-12.9764729959206,-19.0012154099792,
0.));
#196068=CARTESIAN_POINT('Ctrl Pts',(-12.9709450512747,-18.9881820807585,
0.));
#196069=CARTESIAN_POINT('Ctrl Pts',(-12.9654399021868,-18.9753148284473,
0.));
#196070=CARTESIAN_POINT('Ctrl Pts',(-12.9599590886318,-18.9626151329226,
0.));
#196071=CARTESIAN_POINT('Ctrl Pts',(-12.9545041877377,-18.9500845064714,
0.));
#196072=CARTESIAN_POINT('Ctrl Pts',(-12.9490768151821,-18.9377244950435,
0.));
#196073=CARTESIAN_POINT('Ctrl Pts',(-12.9436786266106,-18.9255366795196,
0.));
#196074=CARTESIAN_POINT('Ctrl Pts',(-12.9383113190375,-18.9135226769466,
0.));
#196075=CARTESIAN_POINT('Ctrl Pts',(-12.9329766328184,-18.9016841423402,
0.));
#196076=CARTESIAN_POINT('Ctrl Pts',(-12.9276763536373,-18.8900227704888,
0.));
#196077=CARTESIAN_POINT('Ctrl Pts',(-12.9224123144982,-18.8785402977528,
0.));
#196078=CARTESIAN_POINT('Ctrl Pts',(-12.9171863977047,-18.8672385038328,
0.));
#196079=CARTESIAN_POINT('Ctrl Pts',(-12.9120005369066,-18.8561192136201,
0.));
#196080=CARTESIAN_POINT('Ctrl Pts',(-12.9068567191856,-18.8451842990986,
0.));
#196081=CARTESIAN_POINT('Ctrl Pts',(-12.9017569871738,-18.834435681259,
0.));
#196082=CARTESIAN_POINT('Ctrl Pts',(-12.8967034410752,-18.8238753319124,
0.));
#196083=CARTESIAN_POINT('Ctrl Pts',(-12.8916982409931,-18.8135052757815,
0.));
#196084=CARTESIAN_POINT('Ctrl Pts',(-12.8867436109543,-18.8033275941939,
0.));
#196085=CARTESIAN_POINT('Ctrl Pts',(-12.8818418427474,-18.7933444285867,
0.));
#196086=CARTESIAN_POINT('Ctrl Pts',(-12.8769952998097,-18.7835579840481,
0.));
#196087=CARTESIAN_POINT('Ctrl Pts',(-12.8722064211814,-18.7739705329028,
0.));
#196088=CARTESIAN_POINT('Ctrl Pts',(-12.8674777239656,-18.7645844169568,
0.));
#196089=CARTESIAN_POINT('Ctrl Pts',(-12.8628118054172,-18.7554020493888,
0.));
#196090=CARTESIAN_POINT('Ctrl Pts',(-12.8582113455645,-18.7464259171248,
0.));
#196091=CARTESIAN_POINT('Ctrl Pts',(-12.8536791086315,-18.7376585820851,
0.));
#196092=CARTESIAN_POINT('Ctrl Pts',(-12.849217951159,-18.7291026886552,
0.));
#196093=CARTESIAN_POINT('Ctrl Pts',(-12.8448308329494,-18.7207609737701,
0.));
#196094=CARTESIAN_POINT('Ctrl Pts',(-12.8405208263432,-18.7126362754446,
0.));
#196095=CARTESIAN_POINT('Ctrl Pts',(-12.8362911280362,-18.7047315436296,
0.));
#196096=CARTESIAN_POINT('Ctrl Pts',(-12.832145059979,-18.6970498410173,
0.));
#196097=CARTESIAN_POINT('Ctrl Pts',(-12.8280860635231,-18.6895943376172,
0.));
#196098=CARTESIAN_POINT('Ctrl Pts',(-12.8241176980016,-18.6823683094138,
0.));
#196099=CARTESIAN_POINT('Ctrl Pts',(-12.8202436318473,-18.6753751301091,
0.));
#196100=CARTESIAN_POINT('Ctrl Pts',(-12.8164676687361,-18.6686182952798,
0.));
#196101=CARTESIAN_POINT('Ctrl Pts',(-12.8127937909632,-18.6621014624746,
0.));
#196102=CARTESIAN_POINT('Ctrl Pts',(-12.8092261933858,-18.6558284825772,
0.));
#196103=CARTESIAN_POINT('Ctrl Pts',(-12.805769331162,-18.6498034438986,
0.));
#196104=CARTESIAN_POINT('Ctrl Pts',(-12.8024278770153,-18.6440306327457,
0.));
#196105=CARTESIAN_POINT('Ctrl Pts',(-12.7992066625264,-18.63851447924,0.));
#196106=CARTESIAN_POINT('Ctrl Pts',(-12.7961106222251,-18.6332595057005,
0.));
#196107=CARTESIAN_POINT('Ctrl Pts',(-12.7931447451556,-18.6282702819371,
0.));
#196108=CARTESIAN_POINT('Ctrl Pts',(-12.7903142925235,-18.6235516265575,
0.));
#196109=CARTESIAN_POINT('Ctrl Pts',(-12.7876249657834,-18.6191087624752,
0.));
#196110=CARTESIAN_POINT('Ctrl Pts',(-12.78508316579,-18.6149475565189,0.));
#196111=CARTESIAN_POINT('Ctrl Pts',(-12.7826959526924,-18.611074482622,
0.));
#196112=CARTESIAN_POINT('Ctrl Pts',(-12.7804705387658,-18.6074961535723,
0.));
#196113=CARTESIAN_POINT('Ctrl Pts',(-12.7784139605067,-18.6042190183703,
0.));
#196114=CARTESIAN_POINT('Ctrl Pts',(-12.7765325225083,-18.6012488486708,
0.));
#196115=CARTESIAN_POINT('Ctrl Pts',(-12.7748328937639,-18.5985917525949,
0.));
#196116=CARTESIAN_POINT('Ctrl Pts',(-12.7733231262107,-18.5962551167772,
0.));
#196117=CARTESIAN_POINT('Ctrl Pts',(-12.7720142287169,-18.5942490615409,
0.));
#196118=CARTESIAN_POINT('Ctrl Pts',(-12.7709195951154,-18.5925859134582,
0.));
#196119=CARTESIAN_POINT('Ctrl Pts',(-12.7700520897174,-18.5912775137806,
0.));
#196120=CARTESIAN_POINT('Ctrl Pts',(-12.7694215127923,-18.590332877722,
0.));
#196121=CARTESIAN_POINT('Ctrl Pts',(-12.7691103481996,-18.589871621842,
0.));
#196122=CARTESIAN_POINT('Ctrl Pts',(-12.7689864266924,-18.5896919669158,
0.));
#196123=CARTESIAN_POINT('Ctrl Pts',(-12.7689524524484,-18.5896460962961,
0.));
#196124=CARTESIAN_POINT('Ctrl Pts',(-12.7689476255363,-18.5896416359912,
0.));
#196125=CARTESIAN_POINT('',(-13.5685075571671,-22.1787195904339,0.));
#196126=CARTESIAN_POINT('Ctrl Pts',(-14.6513681262571,-17.1452095830632,
0.));
#196127=CARTESIAN_POINT('Ctrl Pts',(-14.6513681262571,-17.1452095830632,
12.));
#196128=CARTESIAN_POINT('Ctrl Pts',(-14.6513711852843,-17.1452153999142,
0.));
#196129=CARTESIAN_POINT('Ctrl Pts',(-14.6513711852843,-17.1452153999142,
12.));
#196130=CARTESIAN_POINT('Ctrl Pts',(-14.6514066997196,-17.1452600887037,
0.));
#196131=CARTESIAN_POINT('Ctrl Pts',(-14.6514066997196,-17.1452600887037,
12.));
#196132=CARTESIAN_POINT('Ctrl Pts',(-14.6515481598068,-17.1454262858043,
0.));
#196133=CARTESIAN_POINT('Ctrl Pts',(-14.6515481598068,-17.1454262858043,
12.));
#196134=CARTESIAN_POINT('Ctrl Pts',(-14.6519131634508,-17.1458462295271,
0.));
#196135=CARTESIAN_POINT('Ctrl Pts',(-14.6519131634508,-17.1458462295271,
12.));
#196136=CARTESIAN_POINT('Ctrl Pts',(-14.6526624064978,-17.1466998098673,
0.));
#196137=CARTESIAN_POINT('Ctrl Pts',(-14.6526624064978,-17.1466998098673,
12.));
#196138=CARTESIAN_POINT('Ctrl Pts',(-14.6537016966184,-17.147876394491,
0.));
#196139=CARTESIAN_POINT('Ctrl Pts',(-14.6537016966184,-17.147876394491,
12.));
#196140=CARTESIAN_POINT('Ctrl Pts',(-14.655024862281,-17.1493641837558,
0.));
#196141=CARTESIAN_POINT('Ctrl Pts',(-14.655024862281,-17.1493641837558,
12.));
#196142=CARTESIAN_POINT('Ctrl Pts',(-14.6566237952435,-17.1511476869496,
0.));
#196143=CARTESIAN_POINT('Ctrl Pts',(-14.6566237952435,-17.1511476869496,
12.));
#196144=CARTESIAN_POINT('Ctrl Pts',(-14.6584900555302,-17.1532107762718,
0.));
#196145=CARTESIAN_POINT('Ctrl Pts',(-14.6584900555302,-17.1532107762718,
12.));
#196146=CARTESIAN_POINT('Ctrl Pts',(-14.6606167169642,-17.1555401986401,
0.));
#196147=CARTESIAN_POINT('Ctrl Pts',(-14.6606167169642,-17.1555401986401,
12.));
#196148=CARTESIAN_POINT('Ctrl Pts',(-14.6629987285992,-17.1581262646789,
0.));
#196149=CARTESIAN_POINT('Ctrl Pts',(-14.6629987285992,-17.1581262646789,
12.));
#196150=CARTESIAN_POINT('Ctrl Pts',(-14.6656319165057,-17.1609609517369,
0.));
#196151=CARTESIAN_POINT('Ctrl Pts',(-14.6656319165057,-17.1609609517369,
12.));
#196152=CARTESIAN_POINT('Ctrl Pts',(-14.6685123374423,-17.1640366762305,
0.));
#196153=CARTESIAN_POINT('Ctrl Pts',(-14.6685123374423,-17.1640366762305,
12.));
#196154=CARTESIAN_POINT('Ctrl Pts',(-14.671635583332,-17.167344972302,0.));
#196155=CARTESIAN_POINT('Ctrl Pts',(-14.671635583332,-17.167344972302,12.));
#196156=CARTESIAN_POINT('Ctrl Pts',(-14.6749971333867,-17.1708771619129,
0.));
#196157=CARTESIAN_POINT('Ctrl Pts',(-14.6749971333867,-17.1708771619129,
12.));
#196158=CARTESIAN_POINT('Ctrl Pts',(-14.6785925615677,-17.1746247499056,
0.));
#196159=CARTESIAN_POINT('Ctrl Pts',(-14.6785925615677,-17.1746247499056,
12.));
#196160=CARTESIAN_POINT('Ctrl Pts',(-14.6824178576167,-17.1785800350826,
0.));
#196161=CARTESIAN_POINT('Ctrl Pts',(-14.6824178576167,-17.1785800350826,
12.));
#196162=CARTESIAN_POINT('Ctrl Pts',(-14.686469452232,-17.1827361584719,
0.));
#196163=CARTESIAN_POINT('Ctrl Pts',(-14.686469452232,-17.1827361584719,
12.));
#196164=CARTESIAN_POINT('Ctrl Pts',(-14.6907440526958,-17.1870867909918,
0.));
#196165=CARTESIAN_POINT('Ctrl Pts',(-14.6907440526958,-17.1870867909918,
12.));
#196166=CARTESIAN_POINT('Ctrl Pts',(-14.6952385361706,-17.1916259308415,
0.));
#196167=CARTESIAN_POINT('Ctrl Pts',(-14.6952385361706,-17.1916259308415,
12.));
#196168=CARTESIAN_POINT('Ctrl Pts',(-14.699949811582,-17.1963476411694,
0.));
#196169=CARTESIAN_POINT('Ctrl Pts',(-14.699949811582,-17.1963476411694,
12.));
#196170=CARTESIAN_POINT('Ctrl Pts',(-14.7048748502663,-17.2012461084268,
0.));
#196171=CARTESIAN_POINT('Ctrl Pts',(-14.7048748502663,-17.2012461084268,
12.));
#196172=CARTESIAN_POINT('Ctrl Pts',(-14.7100107213586,-17.2063157097315,
0.));
#196173=CARTESIAN_POINT('Ctrl Pts',(-14.7100107213586,-17.2063157097315,
12.));
#196174=CARTESIAN_POINT('Ctrl Pts',(-14.7153546289339,-17.2115510835989,
0.));
#196175=CARTESIAN_POINT('Ctrl Pts',(-14.7153546289339,-17.2115510835989,
12.));
#196176=CARTESIAN_POINT('Ctrl Pts',(-14.7209039390327,-17.2169471814256,
0.));
#196177=CARTESIAN_POINT('Ctrl Pts',(-14.7209039390327,-17.2169471814256,
12.));
#196178=CARTESIAN_POINT('Ctrl Pts',(-14.7266561494282,-17.2224992099666,
0.));
#196179=CARTESIAN_POINT('Ctrl Pts',(-14.7266561494282,-17.2224992099666,
12.));
#196180=CARTESIAN_POINT('Ctrl Pts',(-14.7326088681163,-17.2282025904314,
0.));
#196181=CARTESIAN_POINT('Ctrl Pts',(-14.7326088681163,-17.2282025904314,
12.));
#196182=CARTESIAN_POINT('Ctrl Pts',(-14.7387597858117,-17.2340529062076,
0.));
#196183=CARTESIAN_POINT('Ctrl Pts',(-14.7387597858117,-17.2340529062076,
12.));
#196184=CARTESIAN_POINT('Ctrl Pts',(-14.7451066593792,-17.2400458713565,
0.));
#196185=CARTESIAN_POINT('Ctrl Pts',(-14.7451066593792,-17.2400458713565,
12.));
#196186=CARTESIAN_POINT('Ctrl Pts',(-14.7516473175124,-17.2461773413288,
0.));
#196187=CARTESIAN_POINT('Ctrl Pts',(-14.7516473175124,-17.2461773413288,
12.));
#196188=CARTESIAN_POINT('Ctrl Pts',(-14.7583796616617,-17.2524433146837,
0.));
#196189=CARTESIAN_POINT('Ctrl Pts',(-14.7583796616617,-17.2524433146837,
12.));
#196190=CARTESIAN_POINT('Ctrl Pts',(-14.7653016697591,-17.2588399401465,
0.));
#196191=CARTESIAN_POINT('Ctrl Pts',(-14.7653016697591,-17.2588399401465,
12.));
#196192=CARTESIAN_POINT('Ctrl Pts',(-14.7724113956731,-17.2653635155319,
0.));
#196193=CARTESIAN_POINT('Ctrl Pts',(-14.7724113956731,-17.2653635155319,
12.));
#196194=CARTESIAN_POINT('Ctrl Pts',(-14.7797069617804,-17.2720104735194,
0.));
#196195=CARTESIAN_POINT('Ctrl Pts',(-14.7797069617804,-17.2720104735194,
12.));
#196196=CARTESIAN_POINT('Ctrl Pts',(-14.787186553128,-17.2787773704849,
0.));
#196197=CARTESIAN_POINT('Ctrl Pts',(-14.787186553128,-17.2787773704849,
12.));
#196198=CARTESIAN_POINT('Ctrl Pts',(-14.7948484105249,-17.2856608733196,
0.));
#196199=CARTESIAN_POINT('Ctrl Pts',(-14.7948484105249,-17.2856608733196,
12.));
#196200=CARTESIAN_POINT('Ctrl Pts',(-14.8026908254276,-17.2926577496513,
0.));
#196201=CARTESIAN_POINT('Ctrl Pts',(-14.8026908254276,-17.2926577496513,
12.));
#196202=CARTESIAN_POINT('Ctrl Pts',(-14.8107121391036,-17.299764866148,
0.));
#196203=CARTESIAN_POINT('Ctrl Pts',(-14.8107121391036,-17.299764866148,
12.));
#196204=CARTESIAN_POINT('Ctrl Pts',(-14.8189107410162,-17.3069791853706,
0.));
#196205=CARTESIAN_POINT('Ctrl Pts',(-14.8189107410162,-17.3069791853706,
12.));
#196206=CARTESIAN_POINT('Ctrl Pts',(-14.8272850675379,-17.3142977632659,
0.));
#196207=CARTESIAN_POINT('Ctrl Pts',(-14.8272850675379,-17.3142977632659,
12.));
#196208=CARTESIAN_POINT('Ctrl Pts',(-14.8358336004197,-17.3217177462101,
0.));
#196209=CARTESIAN_POINT('Ctrl Pts',(-14.8358336004197,-17.3217177462101,
12.));
#196210=CARTESIAN_POINT('Ctrl Pts',(-14.8445548643508,-17.3292363662605,
0.));
#196211=CARTESIAN_POINT('Ctrl Pts',(-14.8445548643508,-17.3292363662605,
12.));
#196212=CARTESIAN_POINT('Ctrl Pts',(-14.8534474245434,-17.336850936485,
0.));
#196213=CARTESIAN_POINT('Ctrl Pts',(-14.8534474245434,-17.336850936485,
12.));
#196214=CARTESIAN_POINT('Ctrl Pts',(-14.8625098843417,-17.3445588463474,
0.));
#196215=CARTESIAN_POINT('Ctrl Pts',(-14.8625098843417,-17.3445588463474,
12.));
#196216=CARTESIAN_POINT('Ctrl Pts',(-14.8717408826956,-17.3523575568645,
0.));
#196217=CARTESIAN_POINT('Ctrl Pts',(-14.8717408826956,-17.3523575568645,
12.));
#196218=CARTESIAN_POINT('Ctrl Pts',(-14.8811390927423,-17.3602445978161,
0.));
#196219=CARTESIAN_POINT('Ctrl Pts',(-14.8811390927423,-17.3602445978161,
12.));
#196220=CARTESIAN_POINT('Ctrl Pts',(-14.8907032205788,-17.3682175653235,
0.));
#196221=CARTESIAN_POINT('Ctrl Pts',(-14.8907032205788,-17.3682175653235,
12.));
#196222=CARTESIAN_POINT('Ctrl Pts',(-14.900432003961,-17.3762741193076,
0.));
#196223=CARTESIAN_POINT('Ctrl Pts',(-14.900432003961,-17.3762741193076,
12.));
#196224=CARTESIAN_POINT('Ctrl Pts',(-14.9103242110058,-17.3844119809824,
0.));
#196225=CARTESIAN_POINT('Ctrl Pts',(-14.9103242110058,-17.3844119809824,
12.));
#196226=CARTESIAN_POINT('Ctrl Pts',(-14.9203786389342,-17.3926289303986,
0.));
#196227=CARTESIAN_POINT('Ctrl Pts',(-14.9203786389342,-17.3926289303986,
12.));
#196228=CARTESIAN_POINT('Ctrl Pts',(-14.9305941128757,-17.4009228040749,
0.));
#196229=CARTESIAN_POINT('Ctrl Pts',(-14.9305941128757,-17.4009228040749,
12.));
#196230=CARTESIAN_POINT('Ctrl Pts',(-14.940969484645,-17.4092914926071,
0.));
#196231=CARTESIAN_POINT('Ctrl Pts',(-14.940969484645,-17.4092914926071,
12.));
#196232=CARTESIAN_POINT('Ctrl Pts',(-14.9515036315143,-17.4177329382828,
0.));
#196233=CARTESIAN_POINT('Ctrl Pts',(-14.9515036315143,-17.4177329382828,
12.));
#196234=CARTESIAN_POINT('Ctrl Pts',(-14.9621954549827,-17.426245132709,
0.));
#196235=CARTESIAN_POINT('Ctrl Pts',(-14.9621954549827,-17.426245132709,
12.));
#196236=CARTESIAN_POINT('Ctrl Pts',(-14.9730438799452,-17.4348261151396,
0.));
#196237=CARTESIAN_POINT('Ctrl Pts',(-14.9730438799452,-17.4348261151396,
12.));
#196238=CARTESIAN_POINT('Ctrl Pts',(-14.9840478538358,-17.4434739707773,
0.));
#196239=CARTESIAN_POINT('Ctrl Pts',(-14.9840478538358,-17.4434739707773,
12.));
#196240=CARTESIAN_POINT('Ctrl Pts',(-14.9952063457778,-17.4521868291004,
0.));
#196241=CARTESIAN_POINT('Ctrl Pts',(-14.9952063457778,-17.4521868291004,
12.));
#196242=CARTESIAN_POINT('Ctrl Pts',(-15.0065183456921,-17.4609628621418,
0.));
#196243=CARTESIAN_POINT('Ctrl Pts',(-15.0065183456921,-17.4609628621418,
12.));
#196244=CARTESIAN_POINT('Ctrl Pts',(-15.0179828635086,-17.4698002829356,
0.));
#196245=CARTESIAN_POINT('Ctrl Pts',(-15.0179828635086,-17.4698002829356,
12.));
#196246=CARTESIAN_POINT('Ctrl Pts',(-15.029598928488,-17.4786973441417,
0.));
#196247=CARTESIAN_POINT('Ctrl Pts',(-15.029598928488,-17.4786973441417,
12.));
#196248=CARTESIAN_POINT('Ctrl Pts',(-15.0413655884993,-17.4876523366178,
0.));
#196249=CARTESIAN_POINT('Ctrl Pts',(-15.0413655884993,-17.4876523366178,
12.));
#196250=CARTESIAN_POINT('Ctrl Pts',(-15.0532819093085,-17.4966635880245,
0.));
#196251=CARTESIAN_POINT('Ctrl Pts',(-15.0532819093085,-17.4966635880245,
12.));
#196252=CARTESIAN_POINT('Ctrl Pts',(-15.0653469738306,-17.5057294613874,
0.));
#196253=CARTESIAN_POINT('Ctrl Pts',(-15.0653469738306,-17.5057294613874,
12.));
#196254=CARTESIAN_POINT('Ctrl Pts',(-15.0775598815748,-17.5148483539683,
0.));
#196255=CARTESIAN_POINT('Ctrl Pts',(-15.0775598815748,-17.5148483539683,
12.));
#196256=CARTESIAN_POINT('Ctrl Pts',(-15.0899197481082,-17.5240186961788,
0.));
#196257=CARTESIAN_POINT('Ctrl Pts',(-15.0899197481082,-17.5240186961788,
12.));
#196258=CARTESIAN_POINT('Ctrl Pts',(-15.1024257045033,-17.5332389504829,
0.));
#196259=CARTESIAN_POINT('Ctrl Pts',(-15.1024257045033,-17.5332389504829,
12.));
#196260=CARTESIAN_POINT('Ctrl Pts',(-15.1150768967729,-17.5425076102966,
0.));
#196261=CARTESIAN_POINT('Ctrl Pts',(-15.1150768967729,-17.5425076102966,
12.));
#196262=CARTESIAN_POINT('Ctrl Pts',(-15.127872485314,-17.5518231989122,
0.));
#196263=CARTESIAN_POINT('Ctrl Pts',(-15.127872485314,-17.5518231989122,
12.));
#196264=CARTESIAN_POINT('Ctrl Pts',(-15.1408116444877,-17.5611842686196,
0.));
#196265=CARTESIAN_POINT('Ctrl Pts',(-15.1408116444877,-17.5611842686196,
12.));
#196266=CARTESIAN_POINT('Ctrl Pts',(-15.1538935621715,-17.570589399803,
0.));
#196267=CARTESIAN_POINT('Ctrl Pts',(-15.1538935621715,-17.570589399803,
12.));
#196268=CARTESIAN_POINT('Ctrl Pts',(-15.1671174393137,-17.5800372000539,
0.));
#196269=CARTESIAN_POINT('Ctrl Pts',(-15.1671174393137,-17.5800372000539,
12.));
#196270=CARTESIAN_POINT('Ctrl Pts',(-15.1804824894605,-17.5895263032592,
0.));
#196271=CARTESIAN_POINT('Ctrl Pts',(-15.1804824894605,-17.5895263032592,
12.));
#196272=CARTESIAN_POINT('Ctrl Pts',(-15.1939879383268,-17.5990553687595,
0.));
#196273=CARTESIAN_POINT('Ctrl Pts',(-15.1939879383268,-17.5990553687595,
12.));
#196274=CARTESIAN_POINT('Ctrl Pts',(-15.2076330234686,-17.6086230806497,
0.));
#196275=CARTESIAN_POINT('Ctrl Pts',(-15.2076330234686,-17.6086230806497,
12.));
#196276=CARTESIAN_POINT('Ctrl Pts',(-15.22141699392,-17.6182281470467,0.));
#196277=CARTESIAN_POINT('Ctrl Pts',(-15.22141699392,-17.6182281470467,12.));
#196278=CARTESIAN_POINT('Ctrl Pts',(-15.2353391098367,-17.6278692993765,
0.));
#196279=CARTESIAN_POINT('Ctrl Pts',(-15.2353391098367,-17.6278692993765,
12.));
#196280=CARTESIAN_POINT('Ctrl Pts',(-15.2493986421091,-17.637545291637,
0.));
#196281=CARTESIAN_POINT('Ctrl Pts',(-15.2493986421091,-17.637545291637,
12.));
#196282=CARTESIAN_POINT('Ctrl Pts',(-15.263594872029,-17.6472548997329,
0.));
#196283=CARTESIAN_POINT('Ctrl Pts',(-15.263594872029,-17.6472548997329,
12.));
#196284=CARTESIAN_POINT('Ctrl Pts',(-15.2779270910238,-17.6569969209,0.));
#196285=CARTESIAN_POINT('Ctrl Pts',(-15.2779270910238,-17.6569969209,12.));
#196286=CARTESIAN_POINT('Ctrl Pts',(-15.2923946003598,-17.6667701731041,
0.));
#196287=CARTESIAN_POINT('Ctrl Pts',(-15.2923946003598,-17.6667701731041,
12.));
#196288=CARTESIAN_POINT('Ctrl Pts',(-15.3069967108501,-17.6765734944559,
0.));
#196289=CARTESIAN_POINT('Ctrl Pts',(-15.3069967108501,-17.6765734944559,
12.));
#196290=CARTESIAN_POINT('Ctrl Pts',(-15.3217327425341,-17.6864057426052,
0.));
#196291=CARTESIAN_POINT('Ctrl Pts',(-15.3217327425341,-17.6864057426052,
12.));
#196292=CARTESIAN_POINT('Ctrl Pts',(-15.3366020244069,-17.6962657941984,
0.));
#196293=CARTESIAN_POINT('Ctrl Pts',(-15.3366020244069,-17.6962657941984,
12.));
#196294=CARTESIAN_POINT('Ctrl Pts',(-15.3516038942064,-17.7061525444044,
0.));
#196295=CARTESIAN_POINT('Ctrl Pts',(-15.3516038942064,-17.7061525444044,
12.));
#196296=CARTESIAN_POINT('Ctrl Pts',(-15.3667376981702,-17.7160649064208,
0.));
#196297=CARTESIAN_POINT('Ctrl Pts',(-15.3667376981702,-17.7160649064208,
12.));
#196298=CARTESIAN_POINT('Ctrl Pts',(-15.3820027907965,-17.7260018109923,
0.));
#196299=CARTESIAN_POINT('Ctrl Pts',(-15.3820027907965,-17.7260018109923,
12.));
#196300=CARTESIAN_POINT('Ctrl Pts',(-15.3973985345796,-17.7359622059143,
0.));
#196301=CARTESIAN_POINT('Ctrl Pts',(-15.3973985345796,-17.7359622059143,
12.));
#196302=CARTESIAN_POINT('Ctrl Pts',(-15.4129242997828,-17.7459450555803,
0.));
#196303=CARTESIAN_POINT('Ctrl Pts',(-15.4129242997828,-17.7459450555803,
12.));
#196304=CARTESIAN_POINT('Ctrl Pts',(-15.4285794642658,-17.7559493405871,
0.));
#196305=CARTESIAN_POINT('Ctrl Pts',(-15.4285794642658,-17.7559493405871,
12.));
#196306=CARTESIAN_POINT('Ctrl Pts',(-15.4443634132865,-17.765974057326,
0.));
#196307=CARTESIAN_POINT('Ctrl Pts',(-15.4443634132865,-17.765974057326,
12.));
#196308=CARTESIAN_POINT('Ctrl Pts',(-15.460275539302,-17.7760182175817,
0.));
#196309=CARTESIAN_POINT('Ctrl Pts',(-15.460275539302,-17.7760182175817,
12.));
#196310=CARTESIAN_POINT('Ctrl Pts',(-15.4763152417506,-17.7860808481229,
0.));
#196311=CARTESIAN_POINT('Ctrl Pts',(-15.4763152417506,-17.7860808481229,
12.));
#196312=CARTESIAN_POINT('Ctrl Pts',(-15.4924819268529,-17.7961609903161,
0.));
#196313=CARTESIAN_POINT('Ctrl Pts',(-15.4924819268529,-17.7961609903161,
12.));
#196314=CARTESIAN_POINT('Ctrl Pts',(-15.5087750074728,-17.8062576997964,
0.));
#196315=CARTESIAN_POINT('Ctrl Pts',(-15.5087750074728,-17.8062576997964,
12.));
#196316=CARTESIAN_POINT('Ctrl Pts',(-15.5251939029558,-17.8163700461262,
0.));
#196317=CARTESIAN_POINT('Ctrl Pts',(-15.5251939029558,-17.8163700461262,
12.));
#196318=CARTESIAN_POINT('Ctrl Pts',(-15.5417380389639,-17.8264971124606,
0.));
#196319=CARTESIAN_POINT('Ctrl Pts',(-15.5417380389639,-17.8264971124606,
12.));
#196320=CARTESIAN_POINT('Ctrl Pts',(-15.5584068472976,-17.8366379952078,
0.));
#196321=CARTESIAN_POINT('Ctrl Pts',(-15.5584068472976,-17.8366379952078,
12.));
#196322=CARTESIAN_POINT('Ctrl Pts',(-15.5751997657154,-17.8467918036976,
0.));
#196323=CARTESIAN_POINT('Ctrl Pts',(-15.5751997657154,-17.8467918036976,
12.));
#196324=CARTESIAN_POINT('Ctrl Pts',(-15.5921162378183,-17.8569576598996,
0.));
#196325=CARTESIAN_POINT('Ctrl Pts',(-15.5921162378183,-17.8569576598996,
12.));
#196326=CARTESIAN_POINT('Ctrl Pts',(-15.6091557129205,-17.8671346981388,
0.));
#196327=CARTESIAN_POINT('Ctrl Pts',(-15.6091557129205,-17.8671346981388,
12.));
#196328=CARTESIAN_POINT('Ctrl Pts',(-15.6263176459107,-17.8773220648125,
0.));
#196329=CARTESIAN_POINT('Ctrl Pts',(-15.6263176459107,-17.8773220648125,
12.));
#196330=CARTESIAN_POINT('Ctrl Pts',(-15.6436014971088,-17.8875189181095,
0.));
#196331=CARTESIAN_POINT('Ctrl Pts',(-15.6436014971088,-17.8875189181095,
12.));
#196332=CARTESIAN_POINT('Ctrl Pts',(-15.6610067321036,-17.8977244277247,
0.));
#196333=CARTESIAN_POINT('Ctrl Pts',(-15.6610067321036,-17.8977244277247,
12.));
#196334=CARTESIAN_POINT('Ctrl Pts',(-15.6785328216467,-17.9079377746118,
0.));
#196335=CARTESIAN_POINT('Ctrl Pts',(-15.6785328216467,-17.9079377746118,
12.));
#196336=CARTESIAN_POINT('Ctrl Pts',(-15.6961792415526,-17.918158150746,
0.));
#196337=CARTESIAN_POINT('Ctrl Pts',(-15.6961792415526,-17.918158150746,
12.));
#196338=CARTESIAN_POINT('Ctrl Pts',(-15.713945472584,-17.9283847588837,
0.));
#196339=CARTESIAN_POINT('Ctrl Pts',(-15.713945472584,-17.9283847588837,
12.));
#196340=CARTESIAN_POINT('Ctrl Pts',(-15.7318310003334,-17.9386168123261,
0.));
#196341=CARTESIAN_POINT('Ctrl Pts',(-15.7318310003334,-17.9386168123261,
12.));
#196342=CARTESIAN_POINT('Ctrl Pts',(-15.7498353150856,-17.9488535346776,
0.));
#196343=CARTESIAN_POINT('Ctrl Pts',(-15.7498353150856,-17.9488535346776,
12.));
#196344=CARTESIAN_POINT('Ctrl Pts',(-15.7679579117072,-17.9590941596236,
0.));
#196345=CARTESIAN_POINT('Ctrl Pts',(-15.7679579117072,-17.9590941596236,
12.));
#196346=CARTESIAN_POINT('Ctrl Pts',(-15.786198289572,-17.9693379307297,
0.));
#196347=CARTESIAN_POINT('Ctrl Pts',(-15.786198289572,-17.9693379307297,
12.));
#196348=CARTESIAN_POINT('Ctrl Pts',(-15.8045559524674,-17.9795841012383,
0.));
#196349=CARTESIAN_POINT('Ctrl Pts',(-15.8045559524674,-17.9795841012383,
12.));
#196350=CARTESIAN_POINT('Ctrl Pts',(-15.8230304084963,-17.9898319338664,
0.));
#196351=CARTESIAN_POINT('Ctrl Pts',(-15.8230304084963,-17.9898319338664,
12.));
#196352=CARTESIAN_POINT('Ctrl Pts',(-15.8416211699682,-18.0000807006055,
0.));
#196353=CARTESIAN_POINT('Ctrl Pts',(-15.8416211699682,-18.0000807006055,
12.));
#196354=CARTESIAN_POINT('Ctrl Pts',(-15.8603277532834,-18.010329682521,
0.));
#196355=CARTESIAN_POINT('Ctrl Pts',(-15.8603277532834,-18.010329682521,
12.));
#196356=CARTESIAN_POINT('Ctrl Pts',(-15.8791496788685,-18.0205781695773,
0.));
#196357=CARTESIAN_POINT('Ctrl Pts',(-15.8791496788685,-18.0205781695773,
12.));
#196358=CARTESIAN_POINT('Ctrl Pts',(-15.8980864711043,-18.0308254604638,
0.));
#196359=CARTESIAN_POINT('Ctrl Pts',(-15.8980864711043,-18.0308254604638,
12.));
#196360=CARTESIAN_POINT('Ctrl Pts',(-15.9171376582436,-18.0410708624208,
0.));
#196361=CARTESIAN_POINT('Ctrl Pts',(-15.9171376582436,-18.0410708624208,
12.));
#196362=CARTESIAN_POINT('Ctrl Pts',(-15.9363027723244,-18.0513136910691,
0.));
#196363=CARTESIAN_POINT('Ctrl Pts',(-15.9363027723244,-18.0513136910691,
12.));
#196364=CARTESIAN_POINT('Ctrl Pts',(-15.9555813490645,-18.061553270236,
0.));
#196365=CARTESIAN_POINT('Ctrl Pts',(-15.9555813490645,-18.061553270236,
12.));
#196366=CARTESIAN_POINT('Ctrl Pts',(-15.9749729277848,-18.071788931796,
0.));
#196367=CARTESIAN_POINT('Ctrl Pts',(-15.9749729277848,-18.071788931796,
12.));
#196368=CARTESIAN_POINT('Ctrl Pts',(-15.9944770513616,-18.0820200155238,
0.));
#196369=CARTESIAN_POINT('Ctrl Pts',(-15.9944770513616,-18.0820200155238,
12.));
#196370=CARTESIAN_POINT('Ctrl Pts',(-16.0140932661612,-18.0922458689464,
0.));
#196371=CARTESIAN_POINT('Ctrl Pts',(-16.0140932661612,-18.0922458689464,
12.));
#196372=CARTESIAN_POINT('Ctrl Pts',(-16.0338211219694,-18.1024658471966,
0.));
#196373=CARTESIAN_POINT('Ctrl Pts',(-16.0338211219694,-18.1024658471966,
12.));
#196374=CARTESIAN_POINT('Ctrl Pts',(-16.0536601719124,-18.1126793128688,
0.));
#196375=CARTESIAN_POINT('Ctrl Pts',(-16.0536601719124,-18.1126793128688,
12.));
#196376=CARTESIAN_POINT('Ctrl Pts',(-16.0736099723665,-18.1228856358746,
0.));
#196377=CARTESIAN_POINT('Ctrl Pts',(-16.0736099723665,-18.1228856358746,
12.));
#196378=CARTESIAN_POINT('Ctrl Pts',(-16.0936700829108,-18.1330841933099,
0.));
#196379=CARTESIAN_POINT('Ctrl Pts',(-16.0936700829108,-18.1330841933099,
12.));
#196380=CARTESIAN_POINT('Ctrl Pts',(-16.1138400662791,-18.1432743693231,
0.));
#196381=CARTESIAN_POINT('Ctrl Pts',(-16.1138400662791,-18.1432743693231,
12.));
#196382=CARTESIAN_POINT('Ctrl Pts',(-16.1341194882987,-18.153455554985,
0.));
#196383=CARTESIAN_POINT('Ctrl Pts',(-16.1341194882987,-18.153455554985,
12.));
#196384=CARTESIAN_POINT('Ctrl Pts',(-16.1545079178261,-18.1636271481616,
0.));
#196385=CARTESIAN_POINT('Ctrl Pts',(-16.1545079178261,-18.1636271481616,
12.));
#196386=CARTESIAN_POINT('Ctrl Pts',(-16.1750049266673,-18.1737885533852,
0.));
#196387=CARTESIAN_POINT('Ctrl Pts',(-16.1750049266673,-18.1737885533852,
12.));
#196388=CARTESIAN_POINT('Ctrl Pts',(-16.1956100895076,-18.1839391817335,
0.));
#196389=CARTESIAN_POINT('Ctrl Pts',(-16.1956100895076,-18.1839391817335,
12.));
#196390=CARTESIAN_POINT('Ctrl Pts',(-16.2163229838878,-18.1940784507232,
0.));
#196391=CARTESIAN_POINT('Ctrl Pts',(-16.2163229838878,-18.1940784507232,
12.));
#196392=CARTESIAN_POINT('Ctrl Pts',(-16.237143190164,-18.2042057842037,
0.));
#196393=CARTESIAN_POINT('Ctrl Pts',(-16.237143190164,-18.2042057842037,
12.));
#196394=CARTESIAN_POINT('Ctrl Pts',(-16.2580702914615,-18.214320612253,
0.));
#196395=CARTESIAN_POINT('Ctrl Pts',(-16.2580702914615,-18.214320612253,
12.));
#196396=CARTESIAN_POINT('Ctrl Pts',(-16.2791038736223,-18.2244223710745,
0.));
#196397=CARTESIAN_POINT('Ctrl Pts',(-16.2791038736223,-18.2244223710745,
12.));
#196398=CARTESIAN_POINT('Ctrl Pts',(-16.3002435251378,-18.2345105028981,
0.));
#196399=CARTESIAN_POINT('Ctrl Pts',(-16.3002435251378,-18.2345105028981,
12.));
#196400=CARTESIAN_POINT('Ctrl Pts',(-16.3214888370988,-18.2445844558742,
0.));
#196401=CARTESIAN_POINT('Ctrl Pts',(-16.3214888370988,-18.2445844558742,
12.));
#196402=CARTESIAN_POINT('Ctrl Pts',(-16.342839403159,-18.2546436839609,
0.));
#196403=CARTESIAN_POINT('Ctrl Pts',(-16.342839403159,-18.2546436839609,
12.));
#196404=CARTESIAN_POINT('Ctrl Pts',(-16.3642948194869,-18.2646876468169,
0.));
#196405=CARTESIAN_POINT('Ctrl Pts',(-16.3642948194869,-18.2646876468169,
12.));
#196406=CARTESIAN_POINT('Ctrl Pts',(-16.385854684708,-18.2747158096934,
0.));
#196407=CARTESIAN_POINT('Ctrl Pts',(-16.385854684708,-18.2747158096934,
12.));
#196408=CARTESIAN_POINT('Ctrl Pts',(-16.4075185998454,-18.2847276433308,
0.));
#196409=CARTESIAN_POINT('Ctrl Pts',(-16.4075185998454,-18.2847276433308,
12.));
#196410=CARTESIAN_POINT('Ctrl Pts',(-16.4292861682377,-18.2947226238509,
0.));
#196411=CARTESIAN_POINT('Ctrl Pts',(-16.4292861682377,-18.2947226238509,
12.));
#196412=CARTESIAN_POINT('Ctrl Pts',(-16.4511569955231,-18.3047002326858,
0.));
#196413=CARTESIAN_POINT('Ctrl Pts',(-16.4511569955231,-18.3047002326858,
12.));
#196414=CARTESIAN_POINT('Ctrl Pts',(-16.4731306896439,-18.3146599565229,
0.));
#196415=CARTESIAN_POINT('Ctrl Pts',(-16.4731306896439,-18.3146599565229,
12.));
#196416=CARTESIAN_POINT('Ctrl Pts',(-16.4952068608344,-18.3246012872468,
0.));
#196417=CARTESIAN_POINT('Ctrl Pts',(-16.4952068608344,-18.3246012872468,
12.));
#196418=CARTESIAN_POINT('Ctrl Pts',(-16.5173851216045,-18.3345237218864,
0.));
#196419=CARTESIAN_POINT('Ctrl Pts',(-16.5173851216045,-18.3345237218864,
12.));
#196420=CARTESIAN_POINT('Ctrl Pts',(-16.539665086714,-18.3444267625601,
0.));
#196421=CARTESIAN_POINT('Ctrl Pts',(-16.539665086714,-18.3444267625601,
12.));
#196422=CARTESIAN_POINT('Ctrl Pts',(-16.5620463731414,-18.3543099164331,
0.));
#196423=CARTESIAN_POINT('Ctrl Pts',(-16.5620463731414,-18.3543099164331,
12.));
#196424=CARTESIAN_POINT('Ctrl Pts',(-16.5845286000219,-18.364172695589,
0.));
#196425=CARTESIAN_POINT('Ctrl Pts',(-16.5845286000219,-18.364172695589,
12.));
#196426=CARTESIAN_POINT('Ctrl Pts',(-16.6071113885711,-18.3740146168879,
0.));
#196427=CARTESIAN_POINT('Ctrl Pts',(-16.6071113885711,-18.3740146168879,
12.));
#196428=CARTESIAN_POINT('Ctrl Pts',(-16.6297943620056,-18.3838352018327,
0.));
#196429=CARTESIAN_POINT('Ctrl Pts',(-16.6297943620056,-18.3838352018327,
12.));
#196430=CARTESIAN_POINT('Ctrl Pts',(-16.6525771454513,-18.3936339764332,
0.));
#196431=CARTESIAN_POINT('Ctrl Pts',(-16.6525771454513,-18.3936339764332,
12.));
#196432=CARTESIAN_POINT('Ctrl Pts',(-16.6754593658513,-18.4034104710789,
0.));
#196433=CARTESIAN_POINT('Ctrl Pts',(-16.6754593658513,-18.4034104710789,
12.));
#196434=CARTESIAN_POINT('Ctrl Pts',(-16.698440651849,-18.4131642203989,
0.));
#196435=CARTESIAN_POINT('Ctrl Pts',(-16.698440651849,-18.4131642203989,
12.));
#196436=CARTESIAN_POINT('Ctrl Pts',(-16.7215206338818,-18.4228947633186,
0.));
#196437=CARTESIAN_POINT('Ctrl Pts',(-16.7215206338818,-18.4228947633186,
12.));
#196438=CARTESIAN_POINT('Ctrl Pts',(-16.7446989442882,-18.4326016431392,
0.));
#196439=CARTESIAN_POINT('Ctrl Pts',(-16.7446989442882,-18.4326016431392,
12.));
#196440=CARTESIAN_POINT('Ctrl Pts',(-16.7679752173992,-18.4422844076099,
0.));
#196441=CARTESIAN_POINT('Ctrl Pts',(-16.7679752173992,-18.4422844076099,
12.));
#196442=CARTESIAN_POINT('Ctrl Pts',(-16.791349089629,-18.4519426090124,
0.));
#196443=CARTESIAN_POINT('Ctrl Pts',(-16.791349089629,-18.4519426090124,
12.));
#196444=CARTESIAN_POINT('Ctrl Pts',(-16.8148201995472,-18.4615758042305,
0.));
#196445=CARTESIAN_POINT('Ctrl Pts',(-16.8148201995472,-18.4615758042305,
12.));
#196446=CARTESIAN_POINT('Ctrl Pts',(-16.8383881879707,-18.4711835548622,
0.));
#196447=CARTESIAN_POINT('Ctrl Pts',(-16.8383881879707,-18.4711835548622,
12.));
#196448=CARTESIAN_POINT('Ctrl Pts',(-16.8620526977169,-18.4807654268769,
0.));
#196449=CARTESIAN_POINT('Ctrl Pts',(-16.8620526977169,-18.4807654268769,
12.));
#196450=CARTESIAN_POINT('Ctrl Pts',(-16.8858133733086,-18.4903209902226,
0.));
#196451=CARTESIAN_POINT('Ctrl Pts',(-16.8858133733086,-18.4903209902226,
12.));
#196452=CARTESIAN_POINT('Ctrl Pts',(-16.9096698606942,-18.4998498184619,
0.));
#196453=CARTESIAN_POINT('Ctrl Pts',(-16.9096698606942,-18.4998498184619,
12.));
#196454=CARTESIAN_POINT('Ctrl Pts',(-16.9336218069353,-18.5093514883835,
0.));
#196455=CARTESIAN_POINT('Ctrl Pts',(-16.9336218069353,-18.5093514883835,
12.));
#196456=CARTESIAN_POINT('Ctrl Pts',(-16.957668859934,-18.518825579666,0.));
#196457=CARTESIAN_POINT('Ctrl Pts',(-16.957668859934,-18.518825579666,12.));
#196458=CARTESIAN_POINT('Ctrl Pts',(-16.9818106680382,-18.5282716744198,
0.));
#196459=CARTESIAN_POINT('Ctrl Pts',(-16.9818106680382,-18.5282716744198,
12.));
#196460=CARTESIAN_POINT('Ctrl Pts',(-17.0060468805099,-18.5376893576961,
0.));
#196461=CARTESIAN_POINT('Ctrl Pts',(-17.0060468805099,-18.5376893576961,
12.));
#196462=CARTESIAN_POINT('Ctrl Pts',(-17.030377148174,-18.5470782182089,
0.));
#196463=CARTESIAN_POINT('Ctrl Pts',(-17.030377148174,-18.5470782182089,
12.));
#196464=CARTESIAN_POINT('Ctrl Pts',(-17.0548011239751,-18.5564378489628,
0.));
#196465=CARTESIAN_POINT('Ctrl Pts',(-17.0548011239751,-18.5564378489628,
12.));
#196466=CARTESIAN_POINT('Ctrl Pts',(-17.0793184636079,-18.5657678479788,
0.));
#196467=CARTESIAN_POINT('Ctrl Pts',(-17.0793184636079,-18.5657678479788,
12.));
#196468=CARTESIAN_POINT('Ctrl Pts',(-17.1039288260002,-18.5750678188543,
0.));
#196469=CARTESIAN_POINT('Ctrl Pts',(-17.1039288260002,-18.5750678188543,
12.));
#196470=CARTESIAN_POINT('Ctrl Pts',(-17.1286318741185,-18.5843373717253,
0.));
#196471=CARTESIAN_POINT('Ctrl Pts',(-17.1286318741185,-18.5843373717253,
12.));
#196472=CARTESIAN_POINT('Ctrl Pts',(-17.1534272741646,-18.5935761222833,
0.));
#196473=CARTESIAN_POINT('Ctrl Pts',(-17.1534272741646,-18.5935761222833,
12.));
#196474=CARTESIAN_POINT('Ctrl Pts',(-17.1783146940131,-18.6027836898826,
0.));
#196475=CARTESIAN_POINT('Ctrl Pts',(-17.1783146940131,-18.6027836898826,
12.));
#196476=CARTESIAN_POINT('Ctrl Pts',(-17.2032938019288,-18.6119596959957,
0.));
#196477=CARTESIAN_POINT('Ctrl Pts',(-17.2032938019288,-18.6119596959957,
12.));
#196478=CARTESIAN_POINT('Ctrl Pts',(-17.2283642650519,-18.6211037624041,
0.));
#196479=CARTESIAN_POINT('Ctrl Pts',(-17.2283642650519,-18.6211037624041,
12.));
#196480=CARTESIAN_POINT('Ctrl Pts',(-17.2535257482186,-18.630215509794,
0.));
#196481=CARTESIAN_POINT('Ctrl Pts',(-17.2535257482186,-18.630215509794,
12.));
#196482=CARTESIAN_POINT('Ctrl Pts',(-17.278777912021,-18.639294555474,0.));
#196483=CARTESIAN_POINT('Ctrl Pts',(-17.278777912021,-18.639294555474,12.));
#196484=CARTESIAN_POINT('Ctrl Pts',(-17.3041204135069,-18.6483405141853,
0.));
#196485=CARTESIAN_POINT('Ctrl Pts',(-17.3041204135069,-18.6483405141853,
12.));
#196486=CARTESIAN_POINT('Ctrl Pts',(-17.3295529098612,-18.6573530024019,
0.));
#196487=CARTESIAN_POINT('Ctrl Pts',(-17.3295529098612,-18.6573530024019,
12.));
#196488=CARTESIAN_POINT('Ctrl Pts',(-17.3550750612438,-18.6663316416569,
0.));
#196489=CARTESIAN_POINT('Ctrl Pts',(-17.3550750612438,-18.6663316416569,
12.));
#196490=CARTESIAN_POINT('Ctrl Pts',(-17.3806865340744,-18.6752760624045,
0.));
#196491=CARTESIAN_POINT('Ctrl Pts',(-17.3806865340744,-18.6752760624045,
12.));
#196492=CARTESIAN_POINT('Ctrl Pts',(-17.4063870038563,-18.6841859073472,
0.));
#196493=CARTESIAN_POINT('Ctrl Pts',(-17.4063870038563,-18.6841859073472,
12.));
#196494=CARTESIAN_POINT('Ctrl Pts',(-17.4321761588148,-18.6930608357421,
0.));
#196495=CARTESIAN_POINT('Ctrl Pts',(-17.4321761588148,-18.6930608357421,
12.));
#196496=CARTESIAN_POINT('Ctrl Pts',(-17.4580537012764,-18.7019005250322,
0.));
#196497=CARTESIAN_POINT('Ctrl Pts',(-17.4580537012764,-18.7019005250322,
12.));
#196498=CARTESIAN_POINT('Ctrl Pts',(-17.4840193397176,-18.7107046613941,
0.));
#196499=CARTESIAN_POINT('Ctrl Pts',(-17.4840193397176,-18.7107046613941,
12.));
#196500=CARTESIAN_POINT('Ctrl Pts',(-17.5100727820891,-18.7194729318127,
0.));
#196501=CARTESIAN_POINT('Ctrl Pts',(-17.5100727820891,-18.7194729318127,
12.));
#196502=CARTESIAN_POINT('Ctrl Pts',(-17.5362137287604,-18.728205015716,
0.));
#196503=CARTESIAN_POINT('Ctrl Pts',(-17.5362137287604,-18.728205015716,
12.));
#196504=CARTESIAN_POINT('Ctrl Pts',(-17.5624418653248,-18.7369005764558,
0.));
#196505=CARTESIAN_POINT('Ctrl Pts',(-17.5624418653248,-18.7369005764558,
12.));
#196506=CARTESIAN_POINT('Ctrl Pts',(-17.5887568561361,-18.7455592536667,
0.));
#196507=CARTESIAN_POINT('Ctrl Pts',(-17.5887568561361,-18.7455592536667,
12.));
#196508=CARTESIAN_POINT('Ctrl Pts',(-17.6151583356989,-18.7541806530935,
0.));
#196509=CARTESIAN_POINT('Ctrl Pts',(-17.6151583356989,-18.7541806530935,
12.));
#196510=CARTESIAN_POINT('Ctrl Pts',(-17.6416459210646,-18.7627643613138,
0.));
#196511=CARTESIAN_POINT('Ctrl Pts',(-17.6416459210646,-18.7627643613138,
12.));
#196512=CARTESIAN_POINT('Ctrl Pts',(-17.6682192274197,-18.7713099642673,
0.));
#196513=CARTESIAN_POINT('Ctrl Pts',(-17.6682192274197,-18.7713099642673,
12.));
#196514=CARTESIAN_POINT('Ctrl Pts',(-17.6948778822982,-18.7798170641305,
0.));
#196515=CARTESIAN_POINT('Ctrl Pts',(-17.6948778822982,-18.7798170641305,
12.));
#196516=CARTESIAN_POINT('Ctrl Pts',(-17.7216215409019,-18.7882852976016,
0.));
#196517=CARTESIAN_POINT('Ctrl Pts',(-17.7216215409019,-18.7882852976016,
12.));
#196518=CARTESIAN_POINT('Ctrl Pts',(-17.7484498996917,-18.7967143519444,
0.));
#196519=CARTESIAN_POINT('Ctrl Pts',(-17.7484498996917,-18.7967143519444,
12.));
#196520=CARTESIAN_POINT('Ctrl Pts',(-17.7753627137898,-18.8051039860543,
0.));
#196521=CARTESIAN_POINT('Ctrl Pts',(-17.7753627137898,-18.8051039860543,
12.));
#196522=CARTESIAN_POINT('Ctrl Pts',(-17.8023598011135,-18.8134540340581,
0.));
#196523=CARTESIAN_POINT('Ctrl Pts',(-17.8023598011135,-18.8134540340581,
12.));
#196524=CARTESIAN_POINT('Ctrl Pts',(-17.8294410311105,-18.8217643886368,
0.));
#196525=CARTESIAN_POINT('Ctrl Pts',(-17.8294410311105,-18.8217643886368,
12.));
#196526=CARTESIAN_POINT('Ctrl Pts',(-17.8566063174871,-18.8300349896187,
0.));
#196527=CARTESIAN_POINT('Ctrl Pts',(-17.8566063174871,-18.8300349896187,
12.));
#196528=CARTESIAN_POINT('Ctrl Pts',(-17.8784057509434,-18.8366196462746,
0.));
#196529=CARTESIAN_POINT('Ctrl Pts',(-17.8784057509434,-18.8366196462746,
12.));
#196530=CARTESIAN_POINT('Ctrl Pts',(-17.8947931177853,-18.8415402351882,
0.));
#196531=CARTESIAN_POINT('Ctrl Pts',(-17.8947931177853,-18.8415402351882,
12.));
#196532=CARTESIAN_POINT('Ctrl Pts',(-17.9057348246611,-18.8448126709726,
0.));
#196533=CARTESIAN_POINT('Ctrl Pts',(-17.9057348246611,-18.8448126709726,
12.));
#196534=CARTESIAN_POINT('Ctrl Pts',(-17.9112098770111,-18.8464468996588,
0.));
#196535=CARTESIAN_POINT('Ctrl Pts',(-17.9112098770111,-18.8464468996588,
12.));
#196536=CARTESIAN_POINT('',(-17.9112098770111,-18.8464468996588,0.));
#196537=CARTESIAN_POINT('Ctrl Pts',(-14.6513681262571,-17.1452095830632,
0.));
#196538=CARTESIAN_POINT('Ctrl Pts',(-14.6513711852843,-17.1452153999142,
0.));
#196539=CARTESIAN_POINT('Ctrl Pts',(-14.6514066997196,-17.1452600887037,
0.));
#196540=CARTESIAN_POINT('Ctrl Pts',(-14.6515481598068,-17.1454262858043,
0.));
#196541=CARTESIAN_POINT('Ctrl Pts',(-14.6519131634508,-17.1458462295271,
0.));
#196542=CARTESIAN_POINT('Ctrl Pts',(-14.6526624064978,-17.1466998098673,
0.));
#196543=CARTESIAN_POINT('Ctrl Pts',(-14.6537016966184,-17.147876394491,
0.));
#196544=CARTESIAN_POINT('Ctrl Pts',(-14.655024862281,-17.1493641837558,
0.));
#196545=CARTESIAN_POINT('Ctrl Pts',(-14.6566237952435,-17.1511476869496,
0.));
#196546=CARTESIAN_POINT('Ctrl Pts',(-14.6584900555302,-17.1532107762718,
0.));
#196547=CARTESIAN_POINT('Ctrl Pts',(-14.6606167169642,-17.1555401986401,
0.));
#196548=CARTESIAN_POINT('Ctrl Pts',(-14.6629987285992,-17.1581262646789,
0.));
#196549=CARTESIAN_POINT('Ctrl Pts',(-14.6656319165057,-17.1609609517369,
0.));
#196550=CARTESIAN_POINT('Ctrl Pts',(-14.6685123374423,-17.1640366762305,
0.));
#196551=CARTESIAN_POINT('Ctrl Pts',(-14.671635583332,-17.167344972302,0.));
#196552=CARTESIAN_POINT('Ctrl Pts',(-14.6749971333867,-17.1708771619129,
0.));
#196553=CARTESIAN_POINT('Ctrl Pts',(-14.6785925615677,-17.1746247499056,
0.));
#196554=CARTESIAN_POINT('Ctrl Pts',(-14.6824178576167,-17.1785800350826,
0.));
#196555=CARTESIAN_POINT('Ctrl Pts',(-14.686469452232,-17.1827361584719,
0.));
#196556=CARTESIAN_POINT('Ctrl Pts',(-14.6907440526958,-17.1870867909918,
0.));
#196557=CARTESIAN_POINT('Ctrl Pts',(-14.6952385361706,-17.1916259308415,
0.));
#196558=CARTESIAN_POINT('Ctrl Pts',(-14.699949811582,-17.1963476411694,
0.));
#196559=CARTESIAN_POINT('Ctrl Pts',(-14.7048748502663,-17.2012461084268,
0.));
#196560=CARTESIAN_POINT('Ctrl Pts',(-14.7100107213586,-17.2063157097315,
0.));
#196561=CARTESIAN_POINT('Ctrl Pts',(-14.7153546289339,-17.2115510835989,
0.));
#196562=CARTESIAN_POINT('Ctrl Pts',(-14.7209039390327,-17.2169471814256,
0.));
#196563=CARTESIAN_POINT('Ctrl Pts',(-14.7266561494282,-17.2224992099666,
0.));
#196564=CARTESIAN_POINT('Ctrl Pts',(-14.7326088681163,-17.2282025904314,
0.));
#196565=CARTESIAN_POINT('Ctrl Pts',(-14.7387597858117,-17.2340529062076,
0.));
#196566=CARTESIAN_POINT('Ctrl Pts',(-14.7451066593792,-17.2400458713565,
0.));
#196567=CARTESIAN_POINT('Ctrl Pts',(-14.7516473175124,-17.2461773413288,
0.));
#196568=CARTESIAN_POINT('Ctrl Pts',(-14.7583796616617,-17.2524433146837,
0.));
#196569=CARTESIAN_POINT('Ctrl Pts',(-14.7653016697591,-17.2588399401465,
0.));
#196570=CARTESIAN_POINT('Ctrl Pts',(-14.7724113956731,-17.2653635155319,
0.));
#196571=CARTESIAN_POINT('Ctrl Pts',(-14.7797069617804,-17.2720104735194,
0.));
#196572=CARTESIAN_POINT('Ctrl Pts',(-14.787186553128,-17.2787773704849,
0.));
#196573=CARTESIAN_POINT('Ctrl Pts',(-14.7948484105249,-17.2856608733196,
0.));
#196574=CARTESIAN_POINT('Ctrl Pts',(-14.8026908254276,-17.2926577496513,
0.));
#196575=CARTESIAN_POINT('Ctrl Pts',(-14.8107121391036,-17.299764866148,
0.));
#196576=CARTESIAN_POINT('Ctrl Pts',(-14.8189107410162,-17.3069791853706,
0.));
#196577=CARTESIAN_POINT('Ctrl Pts',(-14.8272850675379,-17.3142977632659,
0.));
#196578=CARTESIAN_POINT('Ctrl Pts',(-14.8358336004197,-17.3217177462101,
0.));
#196579=CARTESIAN_POINT('Ctrl Pts',(-14.8445548643508,-17.3292363662605,
0.));
#196580=CARTESIAN_POINT('Ctrl Pts',(-14.8534474245434,-17.336850936485,
0.));
#196581=CARTESIAN_POINT('Ctrl Pts',(-14.8625098843417,-17.3445588463474,
0.));
#196582=CARTESIAN_POINT('Ctrl Pts',(-14.8717408826956,-17.3523575568645,
0.));
#196583=CARTESIAN_POINT('Ctrl Pts',(-14.8811390927423,-17.3602445978161,
0.));
#196584=CARTESIAN_POINT('Ctrl Pts',(-14.8907032205788,-17.3682175653235,
0.));
#196585=CARTESIAN_POINT('Ctrl Pts',(-14.900432003961,-17.3762741193076,
0.));
#196586=CARTESIAN_POINT('Ctrl Pts',(-14.9103242110058,-17.3844119809824,
0.));
#196587=CARTESIAN_POINT('Ctrl Pts',(-14.9203786389342,-17.3926289303986,
0.));
#196588=CARTESIAN_POINT('Ctrl Pts',(-14.9305941128757,-17.4009228040749,
0.));
#196589=CARTESIAN_POINT('Ctrl Pts',(-14.940969484645,-17.4092914926071,
0.));
#196590=CARTESIAN_POINT('Ctrl Pts',(-14.9515036315143,-17.4177329382828,
0.));
#196591=CARTESIAN_POINT('Ctrl Pts',(-14.9621954549827,-17.426245132709,
0.));
#196592=CARTESIAN_POINT('Ctrl Pts',(-14.9730438799452,-17.4348261151396,
0.));
#196593=CARTESIAN_POINT('Ctrl Pts',(-14.9840478538358,-17.4434739707773,
0.));
#196594=CARTESIAN_POINT('Ctrl Pts',(-14.9952063457778,-17.4521868291004,
0.));
#196595=CARTESIAN_POINT('Ctrl Pts',(-15.0065183456921,-17.4609628621418,
0.));
#196596=CARTESIAN_POINT('Ctrl Pts',(-15.0179828635086,-17.4698002829356,
0.));
#196597=CARTESIAN_POINT('Ctrl Pts',(-15.029598928488,-17.4786973441417,
0.));
#196598=CARTESIAN_POINT('Ctrl Pts',(-15.0413655884993,-17.4876523366178,
0.));
#196599=CARTESIAN_POINT('Ctrl Pts',(-15.0532819093085,-17.4966635880245,
0.));
#196600=CARTESIAN_POINT('Ctrl Pts',(-15.0653469738306,-17.5057294613874,
0.));
#196601=CARTESIAN_POINT('Ctrl Pts',(-15.0775598815748,-17.5148483539683,
0.));
#196602=CARTESIAN_POINT('Ctrl Pts',(-15.0899197481082,-17.5240186961788,
0.));
#196603=CARTESIAN_POINT('Ctrl Pts',(-15.1024257045033,-17.5332389504829,
0.));
#196604=CARTESIAN_POINT('Ctrl Pts',(-15.1150768967729,-17.5425076102966,
0.));
#196605=CARTESIAN_POINT('Ctrl Pts',(-15.127872485314,-17.5518231989122,
0.));
#196606=CARTESIAN_POINT('Ctrl Pts',(-15.1408116444877,-17.5611842686196,
0.));
#196607=CARTESIAN_POINT('Ctrl Pts',(-15.1538935621715,-17.570589399803,
0.));
#196608=CARTESIAN_POINT('Ctrl Pts',(-15.1671174393137,-17.5800372000539,
0.));
#196609=CARTESIAN_POINT('Ctrl Pts',(-15.1804824894605,-17.5895263032592,
0.));
#196610=CARTESIAN_POINT('Ctrl Pts',(-15.1939879383268,-17.5990553687595,
0.));
#196611=CARTESIAN_POINT('Ctrl Pts',(-15.2076330234686,-17.6086230806497,
0.));
#196612=CARTESIAN_POINT('Ctrl Pts',(-15.22141699392,-17.6182281470467,0.));
#196613=CARTESIAN_POINT('Ctrl Pts',(-15.2353391098367,-17.6278692993765,
0.));
#196614=CARTESIAN_POINT('Ctrl Pts',(-15.2493986421091,-17.637545291637,
0.));
#196615=CARTESIAN_POINT('Ctrl Pts',(-15.263594872029,-17.6472548997329,
0.));
#196616=CARTESIAN_POINT('Ctrl Pts',(-15.2779270910238,-17.6569969209,0.));
#196617=CARTESIAN_POINT('Ctrl Pts',(-15.2923946003598,-17.6667701731041,
0.));
#196618=CARTESIAN_POINT('Ctrl Pts',(-15.3069967108501,-17.6765734944559,
0.));
#196619=CARTESIAN_POINT('Ctrl Pts',(-15.3217327425341,-17.6864057426052,
0.));
#196620=CARTESIAN_POINT('Ctrl Pts',(-15.3366020244069,-17.6962657941984,
0.));
#196621=CARTESIAN_POINT('Ctrl Pts',(-15.3516038942064,-17.7061525444044,
0.));
#196622=CARTESIAN_POINT('Ctrl Pts',(-15.3667376981702,-17.7160649064208,
0.));
#196623=CARTESIAN_POINT('Ctrl Pts',(-15.3820027907965,-17.7260018109923,
0.));
#196624=CARTESIAN_POINT('Ctrl Pts',(-15.3973985345796,-17.7359622059143,
0.));
#196625=CARTESIAN_POINT('Ctrl Pts',(-15.4129242997828,-17.7459450555803,
0.));
#196626=CARTESIAN_POINT('Ctrl Pts',(-15.4285794642658,-17.7559493405871,
0.));
#196627=CARTESIAN_POINT('Ctrl Pts',(-15.4443634132865,-17.765974057326,
0.));
#196628=CARTESIAN_POINT('Ctrl Pts',(-15.460275539302,-17.7760182175817,
0.));
#196629=CARTESIAN_POINT('Ctrl Pts',(-15.4763152417506,-17.7860808481229,
0.));
#196630=CARTESIAN_POINT('Ctrl Pts',(-15.4924819268529,-17.7961609903161,
0.));
#196631=CARTESIAN_POINT('Ctrl Pts',(-15.5087750074728,-17.8062576997964,
0.));
#196632=CARTESIAN_POINT('Ctrl Pts',(-15.5251939029558,-17.8163700461262,
0.));
#196633=CARTESIAN_POINT('Ctrl Pts',(-15.5417380389639,-17.8264971124606,
0.));
#196634=CARTESIAN_POINT('Ctrl Pts',(-15.5584068472976,-17.8366379952078,
0.));
#196635=CARTESIAN_POINT('Ctrl Pts',(-15.5751997657154,-17.8467918036976,
0.));
#196636=CARTESIAN_POINT('Ctrl Pts',(-15.5921162378183,-17.8569576598996,
0.));
#196637=CARTESIAN_POINT('Ctrl Pts',(-15.6091557129205,-17.8671346981388,
0.));
#196638=CARTESIAN_POINT('Ctrl Pts',(-15.6263176459107,-17.8773220648125,
0.));
#196639=CARTESIAN_POINT('Ctrl Pts',(-15.6436014971088,-17.8875189181095,
0.));
#196640=CARTESIAN_POINT('Ctrl Pts',(-15.6610067321036,-17.8977244277247,
0.));
#196641=CARTESIAN_POINT('Ctrl Pts',(-15.6785328216467,-17.9079377746118,
0.));
#196642=CARTESIAN_POINT('Ctrl Pts',(-15.6961792415526,-17.918158150746,
0.));
#196643=CARTESIAN_POINT('Ctrl Pts',(-15.713945472584,-17.9283847588837,
0.));
#196644=CARTESIAN_POINT('Ctrl Pts',(-15.7318310003334,-17.9386168123261,
0.));
#196645=CARTESIAN_POINT('Ctrl Pts',(-15.7498353150856,-17.9488535346776,
0.));
#196646=CARTESIAN_POINT('Ctrl Pts',(-15.7679579117072,-17.9590941596236,
0.));
#196647=CARTESIAN_POINT('Ctrl Pts',(-15.786198289572,-17.9693379307297,
0.));
#196648=CARTESIAN_POINT('Ctrl Pts',(-15.8045559524674,-17.9795841012383,
0.));
#196649=CARTESIAN_POINT('Ctrl Pts',(-15.8230304084963,-17.9898319338664,
0.));
#196650=CARTESIAN_POINT('Ctrl Pts',(-15.8416211699682,-18.0000807006055,
0.));
#196651=CARTESIAN_POINT('Ctrl Pts',(-15.8603277532834,-18.010329682521,
0.));
#196652=CARTESIAN_POINT('Ctrl Pts',(-15.8791496788685,-18.0205781695773,
0.));
#196653=CARTESIAN_POINT('Ctrl Pts',(-15.8980864711043,-18.0308254604638,
0.));
#196654=CARTESIAN_POINT('Ctrl Pts',(-15.9171376582436,-18.0410708624208,
0.));
#196655=CARTESIAN_POINT('Ctrl Pts',(-15.9363027723244,-18.0513136910691,
0.));
#196656=CARTESIAN_POINT('Ctrl Pts',(-15.9555813490645,-18.061553270236,
0.));
#196657=CARTESIAN_POINT('Ctrl Pts',(-15.9749729277848,-18.071788931796,
0.));
#196658=CARTESIAN_POINT('Ctrl Pts',(-15.9944770513616,-18.0820200155238,
0.));
#196659=CARTESIAN_POINT('Ctrl Pts',(-16.0140932661612,-18.0922458689464,
0.));
#196660=CARTESIAN_POINT('Ctrl Pts',(-16.0338211219694,-18.1024658471966,
0.));
#196661=CARTESIAN_POINT('Ctrl Pts',(-16.0536601719124,-18.1126793128688,
0.));
#196662=CARTESIAN_POINT('Ctrl Pts',(-16.0736099723665,-18.1228856358746,
0.));
#196663=CARTESIAN_POINT('Ctrl Pts',(-16.0936700829108,-18.1330841933099,
0.));
#196664=CARTESIAN_POINT('Ctrl Pts',(-16.1138400662791,-18.1432743693231,
0.));
#196665=CARTESIAN_POINT('Ctrl Pts',(-16.1341194882987,-18.153455554985,
0.));
#196666=CARTESIAN_POINT('Ctrl Pts',(-16.1545079178261,-18.1636271481616,
0.));
#196667=CARTESIAN_POINT('Ctrl Pts',(-16.1750049266673,-18.1737885533852,
0.));
#196668=CARTESIAN_POINT('Ctrl Pts',(-16.1956100895076,-18.1839391817335,
0.));
#196669=CARTESIAN_POINT('Ctrl Pts',(-16.2163229838878,-18.1940784507232,
0.));
#196670=CARTESIAN_POINT('Ctrl Pts',(-16.237143190164,-18.2042057842037,
0.));
#196671=CARTESIAN_POINT('Ctrl Pts',(-16.2580702914615,-18.214320612253,
0.));
#196672=CARTESIAN_POINT('Ctrl Pts',(-16.2791038736223,-18.2244223710745,
0.));
#196673=CARTESIAN_POINT('Ctrl Pts',(-16.3002435251378,-18.2345105028981,
0.));
#196674=CARTESIAN_POINT('Ctrl Pts',(-16.3214888370988,-18.2445844558742,
0.));
#196675=CARTESIAN_POINT('Ctrl Pts',(-16.342839403159,-18.2546436839609,
0.));
#196676=CARTESIAN_POINT('Ctrl Pts',(-16.3642948194869,-18.2646876468169,
0.));
#196677=CARTESIAN_POINT('Ctrl Pts',(-16.385854684708,-18.2747158096934,
0.));
#196678=CARTESIAN_POINT('Ctrl Pts',(-16.4075185998454,-18.2847276433308,
0.));
#196679=CARTESIAN_POINT('Ctrl Pts',(-16.4292861682377,-18.2947226238509,
0.));
#196680=CARTESIAN_POINT('Ctrl Pts',(-16.4511569955231,-18.3047002326858,
0.));
#196681=CARTESIAN_POINT('Ctrl Pts',(-16.4731306896439,-18.3146599565229,
0.));
#196682=CARTESIAN_POINT('Ctrl Pts',(-16.4952068608344,-18.3246012872468,
0.));
#196683=CARTESIAN_POINT('Ctrl Pts',(-16.5173851216045,-18.3345237218864,
0.));
#196684=CARTESIAN_POINT('Ctrl Pts',(-16.539665086714,-18.3444267625601,
0.));
#196685=CARTESIAN_POINT('Ctrl Pts',(-16.5620463731414,-18.3543099164331,
0.));
#196686=CARTESIAN_POINT('Ctrl Pts',(-16.5845286000219,-18.364172695589,
0.));
#196687=CARTESIAN_POINT('Ctrl Pts',(-16.6071113885711,-18.3740146168879,
0.));
#196688=CARTESIAN_POINT('Ctrl Pts',(-16.6297943620056,-18.3838352018327,
0.));
#196689=CARTESIAN_POINT('Ctrl Pts',(-16.6525771454513,-18.3936339764332,
0.));
#196690=CARTESIAN_POINT('Ctrl Pts',(-16.6754593658513,-18.4034104710789,
0.));
#196691=CARTESIAN_POINT('Ctrl Pts',(-16.698440651849,-18.4131642203989,
0.));
#196692=CARTESIAN_POINT('Ctrl Pts',(-16.7215206338818,-18.4228947633186,
0.));
#196693=CARTESIAN_POINT('Ctrl Pts',(-16.7446989442882,-18.4326016431392,
0.));
#196694=CARTESIAN_POINT('Ctrl Pts',(-16.7679752173992,-18.4422844076099,
0.));
#196695=CARTESIAN_POINT('Ctrl Pts',(-16.791349089629,-18.4519426090124,
0.));
#196696=CARTESIAN_POINT('Ctrl Pts',(-16.8148201995472,-18.4615758042305,
0.));
#196697=CARTESIAN_POINT('Ctrl Pts',(-16.8383881879707,-18.4711835548622,
0.));
#196698=CARTESIAN_POINT('Ctrl Pts',(-16.8620526977169,-18.4807654268769,
0.));
#196699=CARTESIAN_POINT('Ctrl Pts',(-16.8858133733086,-18.4903209902226,
0.));
#196700=CARTESIAN_POINT('Ctrl Pts',(-16.9096698606942,-18.4998498184619,
0.));
#196701=CARTESIAN_POINT('Ctrl Pts',(-16.9336218069353,-18.5093514883835,
0.));
#196702=CARTESIAN_POINT('Ctrl Pts',(-16.957668859934,-18.518825579666,0.));
#196703=CARTESIAN_POINT('Ctrl Pts',(-16.9818106680382,-18.5282716744198,
0.));
#196704=CARTESIAN_POINT('Ctrl Pts',(-17.0060468805099,-18.5376893576961,
0.));
#196705=CARTESIAN_POINT('Ctrl Pts',(-17.030377148174,-18.5470782182089,
0.));
#196706=CARTESIAN_POINT('Ctrl Pts',(-17.0548011239751,-18.5564378489628,
0.));
#196707=CARTESIAN_POINT('Ctrl Pts',(-17.0793184636079,-18.5657678479788,
0.));
#196708=CARTESIAN_POINT('Ctrl Pts',(-17.1039288260002,-18.5750678188543,
0.));
#196709=CARTESIAN_POINT('Ctrl Pts',(-17.1286318741185,-18.5843373717253,
0.));
#196710=CARTESIAN_POINT('Ctrl Pts',(-17.1534272741646,-18.5935761222833,
0.));
#196711=CARTESIAN_POINT('Ctrl Pts',(-17.1783146940131,-18.6027836898826,
0.));
#196712=CARTESIAN_POINT('Ctrl Pts',(-17.2032938019288,-18.6119596959957,
0.));
#196713=CARTESIAN_POINT('Ctrl Pts',(-17.2283642650519,-18.6211037624041,
0.));
#196714=CARTESIAN_POINT('Ctrl Pts',(-17.2535257482186,-18.630215509794,
0.));
#196715=CARTESIAN_POINT('Ctrl Pts',(-17.278777912021,-18.639294555474,0.));
#196716=CARTESIAN_POINT('Ctrl Pts',(-17.3041204135069,-18.6483405141853,
0.));
#196717=CARTESIAN_POINT('Ctrl Pts',(-17.3295529098612,-18.6573530024019,
0.));
#196718=CARTESIAN_POINT('Ctrl Pts',(-17.3550750612438,-18.6663316416569,
0.));
#196719=CARTESIAN_POINT('Ctrl Pts',(-17.3806865340744,-18.6752760624045,
0.));
#196720=CARTESIAN_POINT('Ctrl Pts',(-17.4063870038563,-18.6841859073472,
0.));
#196721=CARTESIAN_POINT('Ctrl Pts',(-17.4321761588148,-18.6930608357421,
0.));
#196722=CARTESIAN_POINT('Ctrl Pts',(-17.4580537012764,-18.7019005250322,
0.));
#196723=CARTESIAN_POINT('Ctrl Pts',(-17.4840193397176,-18.7107046613941,
0.));
#196724=CARTESIAN_POINT('Ctrl Pts',(-17.5100727820891,-18.7194729318127,
0.));
#196725=CARTESIAN_POINT('Ctrl Pts',(-17.5362137287604,-18.728205015716,
0.));
#196726=CARTESIAN_POINT('Ctrl Pts',(-17.5624418653248,-18.7369005764558,
0.));
#196727=CARTESIAN_POINT('Ctrl Pts',(-17.5887568561361,-18.7455592536667,
0.));
#196728=CARTESIAN_POINT('Ctrl Pts',(-17.6151583356989,-18.7541806530935,
0.));
#196729=CARTESIAN_POINT('Ctrl Pts',(-17.6416459210646,-18.7627643613138,
0.));
#196730=CARTESIAN_POINT('Ctrl Pts',(-17.6682192274197,-18.7713099642673,
0.));
#196731=CARTESIAN_POINT('Ctrl Pts',(-17.6948778822982,-18.7798170641305,
0.));
#196732=CARTESIAN_POINT('Ctrl Pts',(-17.7216215409019,-18.7882852976016,
0.));
#196733=CARTESIAN_POINT('Ctrl Pts',(-17.7484498996917,-18.7967143519444,
0.));
#196734=CARTESIAN_POINT('Ctrl Pts',(-17.7753627137898,-18.8051039860543,
0.));
#196735=CARTESIAN_POINT('Ctrl Pts',(-17.8023598011135,-18.8134540340581,
0.));
#196736=CARTESIAN_POINT('Ctrl Pts',(-17.8294410311105,-18.8217643886368,
0.));
#196737=CARTESIAN_POINT('Ctrl Pts',(-17.8566063174871,-18.8300349896187,
0.));
#196738=CARTESIAN_POINT('Ctrl Pts',(-17.8784057509434,-18.8366196462746,
0.));
#196739=CARTESIAN_POINT('Ctrl Pts',(-17.8947931177853,-18.8415402351882,
0.));
#196740=CARTESIAN_POINT('Ctrl Pts',(-17.9057348246611,-18.8448126709726,
0.));
#196741=CARTESIAN_POINT('Ctrl Pts',(-17.9112098770111,-18.8464468996588,
0.));
#196742=CARTESIAN_POINT('',(-17.9112098770111,-18.8464468996588,0.));
#196743=CARTESIAN_POINT('Origin',(-17.7219872369693,-12.1729687575668,0.));
#196744=CARTESIAN_POINT('',(-18.5896416359912,-12.7689476255363,0.));
#196745=CARTESIAN_POINT('',(-18.5896416359912,-12.7689476255363,0.));
#196746=CARTESIAN_POINT('',(-8.86099361848466,-6.08648437878338,0.));
#196747=CARTESIAN_POINT('Ctrl Pts',(-18.8464468996588,-17.9112098770111,
0.));
#196748=CARTESIAN_POINT('Ctrl Pts',(-18.8464468996588,-17.9112098770111,
12.));
#196749=CARTESIAN_POINT('Ctrl Pts',(-18.8448126709692,-17.9057348246595,
0.));
#196750=CARTESIAN_POINT('Ctrl Pts',(-18.8448126709692,-17.9057348246595,
12.));
#196751=CARTESIAN_POINT('Ctrl Pts',(-18.8415402351786,-17.8947931177807,
0.));
#196752=CARTESIAN_POINT('Ctrl Pts',(-18.8415402351786,-17.8947931177807,
12.));
#196753=CARTESIAN_POINT('Ctrl Pts',(-18.8366196462581,-17.8784057509356,
0.));
#196754=CARTESIAN_POINT('Ctrl Pts',(-18.8366196462581,-17.8784057509356,
12.));
#196755=CARTESIAN_POINT('Ctrl Pts',(-18.8300349895974,-17.8566063174771,
0.));
#196756=CARTESIAN_POINT('Ctrl Pts',(-18.8300349895974,-17.8566063174771,
12.));
#196757=CARTESIAN_POINT('Ctrl Pts',(-18.8217643886157,-17.8294410311006,
0.));
#196758=CARTESIAN_POINT('Ctrl Pts',(-18.8217643886157,-17.8294410311006,
12.));
#196759=CARTESIAN_POINT('Ctrl Pts',(-18.8134540340417,-17.8023598011057,
0.));
#196760=CARTESIAN_POINT('Ctrl Pts',(-18.8134540340417,-17.8023598011057,
12.));
#196761=CARTESIAN_POINT('Ctrl Pts',(-18.8051039860448,-17.7753627137853,
0.));
#196762=CARTESIAN_POINT('Ctrl Pts',(-18.8051039860448,-17.7753627137853,
12.));
#196763=CARTESIAN_POINT('Ctrl Pts',(-18.7967143519419,-17.7484498996905,
0.));
#196764=CARTESIAN_POINT('Ctrl Pts',(-18.7967143519419,-17.7484498996905,
12.));
#196765=CARTESIAN_POINT('Ctrl Pts',(-18.788285297605,-17.7216215409035,
0.));
#196766=CARTESIAN_POINT('Ctrl Pts',(-18.788285297605,-17.7216215409035,
12.));
#196767=CARTESIAN_POINT('Ctrl Pts',(-18.7798170641374,-17.6948778823014,
0.));
#196768=CARTESIAN_POINT('Ctrl Pts',(-18.7798170641374,-17.6948778823014,
12.));
#196769=CARTESIAN_POINT('Ctrl Pts',(-18.7713099642754,-17.6682192274236,
0.));
#196770=CARTESIAN_POINT('Ctrl Pts',(-18.7713099642754,-17.6682192274236,
12.));
#196771=CARTESIAN_POINT('Ctrl Pts',(-18.762764361321,-17.6416459210681,
0.));
#196772=CARTESIAN_POINT('Ctrl Pts',(-18.762764361321,-17.6416459210681,
12.));
#196773=CARTESIAN_POINT('Ctrl Pts',(-18.7541806530984,-17.6151583357012,
0.));
#196774=CARTESIAN_POINT('Ctrl Pts',(-18.7541806530984,-17.6151583357012,
12.));
#196775=CARTESIAN_POINT('Ctrl Pts',(-18.7455592536687,-17.5887568561371,
0.));
#196776=CARTESIAN_POINT('Ctrl Pts',(-18.7455592536687,-17.5887568561371,
12.));
#196777=CARTESIAN_POINT('Ctrl Pts',(-18.7369005764553,-17.5624418653245,
0.));
#196778=CARTESIAN_POINT('Ctrl Pts',(-18.7369005764553,-17.5624418653245,
12.));
#196779=CARTESIAN_POINT('Ctrl Pts',(-18.7282050157138,-17.5362137287593,
0.));
#196780=CARTESIAN_POINT('Ctrl Pts',(-18.7282050157138,-17.5362137287593,
12.));
#196781=CARTESIAN_POINT('Ctrl Pts',(-18.7194729318098,-17.5100727820876,
0.));
#196782=CARTESIAN_POINT('Ctrl Pts',(-18.7194729318098,-17.5100727820876,
12.));
#196783=CARTESIAN_POINT('Ctrl Pts',(-18.7107046613912,-17.4840193397162,
0.));
#196784=CARTESIAN_POINT('Ctrl Pts',(-18.7107046613912,-17.4840193397162,
12.));
#196785=CARTESIAN_POINT('Ctrl Pts',(-18.70190052503,-17.4580537012753,0.));
#196786=CARTESIAN_POINT('Ctrl Pts',(-18.70190052503,-17.4580537012753,12.));
#196787=CARTESIAN_POINT('Ctrl Pts',(-18.6930608357409,-17.4321761588142,
0.));
#196788=CARTESIAN_POINT('Ctrl Pts',(-18.6930608357409,-17.4321761588142,
12.));
#196789=CARTESIAN_POINT('Ctrl Pts',(-18.6841859073471,-17.4063870038562,
0.));
#196790=CARTESIAN_POINT('Ctrl Pts',(-18.6841859073471,-17.4063870038562,
12.));
#196791=CARTESIAN_POINT('Ctrl Pts',(-18.6752760624052,-17.3806865340747,
0.));
#196792=CARTESIAN_POINT('Ctrl Pts',(-18.6752760624052,-17.3806865340747,
12.));
#196793=CARTESIAN_POINT('Ctrl Pts',(-18.6663316416582,-17.3550750612443,
0.));
#196794=CARTESIAN_POINT('Ctrl Pts',(-18.6663316416582,-17.3550750612443,
12.));
#196795=CARTESIAN_POINT('Ctrl Pts',(-18.6573530024033,-17.3295529098618,
0.));
#196796=CARTESIAN_POINT('Ctrl Pts',(-18.6573530024033,-17.3295529098618,
12.));
#196797=CARTESIAN_POINT('Ctrl Pts',(-18.6483405141865,-17.3041204135074,
0.));
#196798=CARTESIAN_POINT('Ctrl Pts',(-18.6483405141865,-17.3041204135074,
12.));
#196799=CARTESIAN_POINT('Ctrl Pts',(-18.6392945554748,-17.2787779120213,
0.));
#196800=CARTESIAN_POINT('Ctrl Pts',(-18.6392945554748,-17.2787779120213,
12.));
#196801=CARTESIAN_POINT('Ctrl Pts',(-18.6302155097943,-17.2535257482187,
0.));
#196802=CARTESIAN_POINT('Ctrl Pts',(-18.6302155097943,-17.2535257482187,
12.));
#196803=CARTESIAN_POINT('Ctrl Pts',(-18.6211037624038,-17.2283642650518,
0.));
#196804=CARTESIAN_POINT('Ctrl Pts',(-18.6211037624038,-17.2283642650518,
12.));
#196805=CARTESIAN_POINT('Ctrl Pts',(-18.6119596959949,-17.2032938019284,
0.));
#196806=CARTESIAN_POINT('Ctrl Pts',(-18.6119596959949,-17.2032938019284,
12.));
#196807=CARTESIAN_POINT('Ctrl Pts',(-18.6027836898817,-17.1783146940127,
0.));
#196808=CARTESIAN_POINT('Ctrl Pts',(-18.6027836898817,-17.1783146940127,
12.));
#196809=CARTESIAN_POINT('Ctrl Pts',(-18.5935761222825,-17.1534272741643,
0.));
#196810=CARTESIAN_POINT('Ctrl Pts',(-18.5935761222825,-17.1534272741643,
12.));
#196811=CARTESIAN_POINT('Ctrl Pts',(-18.5843373717247,-17.1286318741183,
0.));
#196812=CARTESIAN_POINT('Ctrl Pts',(-18.5843373717247,-17.1286318741183,
12.));
#196813=CARTESIAN_POINT('Ctrl Pts',(-18.5750678188542,-17.1039288260001,
0.));
#196814=CARTESIAN_POINT('Ctrl Pts',(-18.5750678188542,-17.1039288260001,
12.));
#196815=CARTESIAN_POINT('Ctrl Pts',(-18.5657678479789,-17.0793184636079,
0.));
#196816=CARTESIAN_POINT('Ctrl Pts',(-18.5657678479789,-17.0793184636079,
12.));
#196817=CARTESIAN_POINT('Ctrl Pts',(-18.556437848963,-17.0548011239751,
0.));
#196818=CARTESIAN_POINT('Ctrl Pts',(-18.556437848963,-17.0548011239751,
12.));
#196819=CARTESIAN_POINT('Ctrl Pts',(-18.547078218209,-17.0303771481738,
0.));
#196820=CARTESIAN_POINT('Ctrl Pts',(-18.547078218209,-17.0303771481738,
12.));
#196821=CARTESIAN_POINT('Ctrl Pts',(-18.5376893576961,-17.0060468805097,
0.));
#196822=CARTESIAN_POINT('Ctrl Pts',(-18.5376893576961,-17.0060468805097,
12.));
#196823=CARTESIAN_POINT('Ctrl Pts',(-18.5282716744197,-16.981810668038,
0.));
#196824=CARTESIAN_POINT('Ctrl Pts',(-18.5282716744197,-16.981810668038,
12.));
#196825=CARTESIAN_POINT('Ctrl Pts',(-18.5188255796659,-16.9576688599339,
0.));
#196826=CARTESIAN_POINT('Ctrl Pts',(-18.5188255796659,-16.9576688599339,
12.));
#196827=CARTESIAN_POINT('Ctrl Pts',(-18.5093514883835,-16.9336218069353,
0.));
#196828=CARTESIAN_POINT('Ctrl Pts',(-18.5093514883835,-16.9336218069353,
12.));
#196829=CARTESIAN_POINT('Ctrl Pts',(-18.499849818462,-16.9096698606943,
0.));
#196830=CARTESIAN_POINT('Ctrl Pts',(-18.499849818462,-16.9096698606943,
12.));
#196831=CARTESIAN_POINT('Ctrl Pts',(-18.4903209902227,-16.8858133733088,
0.));
#196832=CARTESIAN_POINT('Ctrl Pts',(-18.4903209902227,-16.8858133733088,
12.));
#196833=CARTESIAN_POINT('Ctrl Pts',(-18.4807654268771,-16.8620526977171,
0.));
#196834=CARTESIAN_POINT('Ctrl Pts',(-18.4807654268771,-16.8620526977171,
12.));
#196835=CARTESIAN_POINT('Ctrl Pts',(-18.4711835548623,-16.8383881879709,
0.));
#196836=CARTESIAN_POINT('Ctrl Pts',(-18.4711835548623,-16.8383881879709,
12.));
#196837=CARTESIAN_POINT('Ctrl Pts',(-18.4615758042305,-16.8148201995472,
0.));
#196838=CARTESIAN_POINT('Ctrl Pts',(-18.4615758042305,-16.8148201995472,
12.));
#196839=CARTESIAN_POINT('Ctrl Pts',(-18.4519426090124,-16.791349089629,
0.));
#196840=CARTESIAN_POINT('Ctrl Pts',(-18.4519426090124,-16.791349089629,
12.));
#196841=CARTESIAN_POINT('Ctrl Pts',(-18.44228440761,-16.7679752173992,0.));
#196842=CARTESIAN_POINT('Ctrl Pts',(-18.44228440761,-16.7679752173992,12.));
#196843=CARTESIAN_POINT('Ctrl Pts',(-18.4326016431392,-16.7446989442882,
0.));
#196844=CARTESIAN_POINT('Ctrl Pts',(-18.4326016431392,-16.7446989442882,
12.));
#196845=CARTESIAN_POINT('Ctrl Pts',(-18.4228947633187,-16.7215206338818,
0.));
#196846=CARTESIAN_POINT('Ctrl Pts',(-18.4228947633187,-16.7215206338818,
12.));
#196847=CARTESIAN_POINT('Ctrl Pts',(-18.413164220399,-16.6984406518491,
0.));
#196848=CARTESIAN_POINT('Ctrl Pts',(-18.413164220399,-16.6984406518491,
12.));
#196849=CARTESIAN_POINT('Ctrl Pts',(-18.403410471079,-16.6754593658513,
0.));
#196850=CARTESIAN_POINT('Ctrl Pts',(-18.403410471079,-16.6754593658513,
12.));
#196851=CARTESIAN_POINT('Ctrl Pts',(-18.3936339764332,-16.6525771454513,
0.));
#196852=CARTESIAN_POINT('Ctrl Pts',(-18.3936339764332,-16.6525771454513,
12.));
#196853=CARTESIAN_POINT('Ctrl Pts',(-18.3838352018327,-16.6297943620056,
0.));
#196854=CARTESIAN_POINT('Ctrl Pts',(-18.3838352018327,-16.6297943620056,
12.));
#196855=CARTESIAN_POINT('Ctrl Pts',(-18.3740146168879,-16.607111388571,
0.));
#196856=CARTESIAN_POINT('Ctrl Pts',(-18.3740146168879,-16.607111388571,
12.));
#196857=CARTESIAN_POINT('Ctrl Pts',(-18.3641726955889,-16.5845286000217,
0.));
#196858=CARTESIAN_POINT('Ctrl Pts',(-18.3641726955889,-16.5845286000217,
12.));
#196859=CARTESIAN_POINT('Ctrl Pts',(-18.354309916433,-16.5620463731413,
0.));
#196860=CARTESIAN_POINT('Ctrl Pts',(-18.354309916433,-16.5620463731413,
12.));
#196861=CARTESIAN_POINT('Ctrl Pts',(-18.34442676256,-16.5396650867139,0.));
#196862=CARTESIAN_POINT('Ctrl Pts',(-18.34442676256,-16.5396650867139,12.));
#196863=CARTESIAN_POINT('Ctrl Pts',(-18.3345237218864,-16.5173851216045,
0.));
#196864=CARTESIAN_POINT('Ctrl Pts',(-18.3345237218864,-16.5173851216045,
12.));
#196865=CARTESIAN_POINT('Ctrl Pts',(-18.3246012872469,-16.4952068608345,
0.));
#196866=CARTESIAN_POINT('Ctrl Pts',(-18.3246012872469,-16.4952068608345,
12.));
#196867=CARTESIAN_POINT('Ctrl Pts',(-18.3146599565231,-16.4731306896441,
0.));
#196868=CARTESIAN_POINT('Ctrl Pts',(-18.3146599565231,-16.4731306896441,
12.));
#196869=CARTESIAN_POINT('Ctrl Pts',(-18.304700232686,-16.4511569955233,
0.));
#196870=CARTESIAN_POINT('Ctrl Pts',(-18.304700232686,-16.4511569955233,
12.));
#196871=CARTESIAN_POINT('Ctrl Pts',(-18.294722623851,-16.4292861682379,
0.));
#196872=CARTESIAN_POINT('Ctrl Pts',(-18.294722623851,-16.4292861682379,
12.));
#196873=CARTESIAN_POINT('Ctrl Pts',(-18.2847276433309,-16.4075185998455,
0.));
#196874=CARTESIAN_POINT('Ctrl Pts',(-18.2847276433309,-16.4075185998455,
12.));
#196875=CARTESIAN_POINT('Ctrl Pts',(-18.2747158096934,-16.385854684708,
0.));
#196876=CARTESIAN_POINT('Ctrl Pts',(-18.2747158096934,-16.385854684708,
12.));
#196877=CARTESIAN_POINT('Ctrl Pts',(-18.2646876468169,-16.3642948194868,
0.));
#196878=CARTESIAN_POINT('Ctrl Pts',(-18.2646876468169,-16.3642948194868,
12.));
#196879=CARTESIAN_POINT('Ctrl Pts',(-18.2546436839608,-16.3428394031589,
0.));
#196880=CARTESIAN_POINT('Ctrl Pts',(-18.2546436839608,-16.3428394031589,
12.));
#196881=CARTESIAN_POINT('Ctrl Pts',(-18.2445844558742,-16.3214888370987,
0.));
#196882=CARTESIAN_POINT('Ctrl Pts',(-18.2445844558742,-16.3214888370987,
12.));
#196883=CARTESIAN_POINT('Ctrl Pts',(-18.2345105028982,-16.3002435251378,
0.));
#196884=CARTESIAN_POINT('Ctrl Pts',(-18.2345105028982,-16.3002435251378,
12.));
#196885=CARTESIAN_POINT('Ctrl Pts',(-18.2244223710746,-16.2791038736223,
0.));
#196886=CARTESIAN_POINT('Ctrl Pts',(-18.2244223710746,-16.2791038736223,
12.));
#196887=CARTESIAN_POINT('Ctrl Pts',(-18.2143206122529,-16.2580702914615,
0.));
#196888=CARTESIAN_POINT('Ctrl Pts',(-18.2143206122529,-16.2580702914615,
12.));
#196889=CARTESIAN_POINT('Ctrl Pts',(-18.2042057842035,-16.2371431901638,
0.));
#196890=CARTESIAN_POINT('Ctrl Pts',(-18.2042057842035,-16.2371431901638,
12.));
#196891=CARTESIAN_POINT('Ctrl Pts',(-18.1940784507229,-16.2163229838875,
0.));
#196892=CARTESIAN_POINT('Ctrl Pts',(-18.1940784507229,-16.2163229838875,
12.));
#196893=CARTESIAN_POINT('Ctrl Pts',(-18.1839391817331,-16.1956100895073,
0.));
#196894=CARTESIAN_POINT('Ctrl Pts',(-18.1839391817331,-16.1956100895073,
12.));
#196895=CARTESIAN_POINT('Ctrl Pts',(-18.1737885533849,-16.1750049266671,
0.));
#196896=CARTESIAN_POINT('Ctrl Pts',(-18.1737885533849,-16.1750049266671,
12.));
#196897=CARTESIAN_POINT('Ctrl Pts',(-18.1636271481615,-16.154507917826,
0.));
#196898=CARTESIAN_POINT('Ctrl Pts',(-18.1636271481615,-16.154507917826,
12.));
#196899=CARTESIAN_POINT('Ctrl Pts',(-18.1534555549852,-16.1341194882988,
0.));
#196900=CARTESIAN_POINT('Ctrl Pts',(-18.1534555549852,-16.1341194882988,
12.));
#196901=CARTESIAN_POINT('Ctrl Pts',(-18.1432743693235,-16.1138400662794,
0.));
#196902=CARTESIAN_POINT('Ctrl Pts',(-18.1432743693235,-16.1138400662794,
12.));
#196903=CARTESIAN_POINT('Ctrl Pts',(-18.1330841933105,-16.0936700829112,
0.));
#196904=CARTESIAN_POINT('Ctrl Pts',(-18.1330841933105,-16.0936700829112,
12.));
#196905=CARTESIAN_POINT('Ctrl Pts',(-18.1228856358751,-16.0736099723668,
0.));
#196906=CARTESIAN_POINT('Ctrl Pts',(-18.1228856358751,-16.0736099723668,
12.));
#196907=CARTESIAN_POINT('Ctrl Pts',(-18.112679312869,-16.0536601719126,
0.));
#196908=CARTESIAN_POINT('Ctrl Pts',(-18.112679312869,-16.0536601719126,
12.));
#196909=CARTESIAN_POINT('Ctrl Pts',(-18.1024658471966,-16.0338211219693,
0.));
#196910=CARTESIAN_POINT('Ctrl Pts',(-18.1024658471966,-16.0338211219693,
12.));
#196911=CARTESIAN_POINT('Ctrl Pts',(-18.0922458689462,-16.014093266161,
0.));
#196912=CARTESIAN_POINT('Ctrl Pts',(-18.0922458689462,-16.014093266161,
12.));
#196913=CARTESIAN_POINT('Ctrl Pts',(-18.0820200155236,-15.9944770513613,
0.));
#196914=CARTESIAN_POINT('Ctrl Pts',(-18.0820200155236,-15.9944770513613,
12.));
#196915=CARTESIAN_POINT('Ctrl Pts',(-18.0717889317958,-15.9749729277846,
0.));
#196916=CARTESIAN_POINT('Ctrl Pts',(-18.0717889317958,-15.9749729277846,
12.));
#196917=CARTESIAN_POINT('Ctrl Pts',(-18.061553270236,-15.9555813490644,
0.));
#196918=CARTESIAN_POINT('Ctrl Pts',(-18.061553270236,-15.9555813490644,
12.));
#196919=CARTESIAN_POINT('Ctrl Pts',(-18.0513136910691,-15.9363027723244,
0.));
#196920=CARTESIAN_POINT('Ctrl Pts',(-18.0513136910691,-15.9363027723244,
12.));
#196921=CARTESIAN_POINT('Ctrl Pts',(-18.0410708624208,-15.9171376582436,
0.));
#196922=CARTESIAN_POINT('Ctrl Pts',(-18.0410708624208,-15.9171376582436,
12.));
#196923=CARTESIAN_POINT('Ctrl Pts',(-18.0308254604636,-15.8980864711042,
0.));
#196924=CARTESIAN_POINT('Ctrl Pts',(-18.0308254604636,-15.8980864711042,
12.));
#196925=CARTESIAN_POINT('Ctrl Pts',(-18.0205781695769,-15.8791496788682,
0.));
#196926=CARTESIAN_POINT('Ctrl Pts',(-18.0205781695769,-15.8791496788682,
12.));
#196927=CARTESIAN_POINT('Ctrl Pts',(-18.0103296825205,-15.8603277532831,
0.));
#196928=CARTESIAN_POINT('Ctrl Pts',(-18.0103296825205,-15.8603277532831,
12.));
#196929=CARTESIAN_POINT('Ctrl Pts',(-18.0000807006052,-15.8416211699679,
0.));
#196930=CARTESIAN_POINT('Ctrl Pts',(-18.0000807006052,-15.8416211699679,
12.));
#196931=CARTESIAN_POINT('Ctrl Pts',(-17.9898319338664,-15.8230304084962,
0.));
#196932=CARTESIAN_POINT('Ctrl Pts',(-17.9898319338664,-15.8230304084962,
12.));
#196933=CARTESIAN_POINT('Ctrl Pts',(-17.9795841012386,-15.8045559524676,
0.));
#196934=CARTESIAN_POINT('Ctrl Pts',(-17.9795841012386,-15.8045559524676,
12.));
#196935=CARTESIAN_POINT('Ctrl Pts',(-17.9693379307303,-15.7861982895724,
0.));
#196936=CARTESIAN_POINT('Ctrl Pts',(-17.9693379307303,-15.7861982895724,
12.));
#196937=CARTESIAN_POINT('Ctrl Pts',(-17.9590941596242,-15.7679579117077,
0.));
#196938=CARTESIAN_POINT('Ctrl Pts',(-17.9590941596242,-15.7679579117077,
12.));
#196939=CARTESIAN_POINT('Ctrl Pts',(-17.9488535346781,-15.749835315086,
0.));
#196940=CARTESIAN_POINT('Ctrl Pts',(-17.9488535346781,-15.749835315086,
12.));
#196941=CARTESIAN_POINT('Ctrl Pts',(-17.9386168123262,-15.7318310003335,
0.));
#196942=CARTESIAN_POINT('Ctrl Pts',(-17.9386168123262,-15.7318310003335,
12.));
#196943=CARTESIAN_POINT('Ctrl Pts',(-17.9283847588836,-15.7139454725838,
0.));
#196944=CARTESIAN_POINT('Ctrl Pts',(-17.9283847588836,-15.7139454725838,
12.));
#196945=CARTESIAN_POINT('Ctrl Pts',(-17.9181581507455,-15.6961792415522,
0.));
#196946=CARTESIAN_POINT('Ctrl Pts',(-17.9181581507455,-15.6961792415522,
12.));
#196947=CARTESIAN_POINT('Ctrl Pts',(-17.9079377746111,-15.678532821646,
0.));
#196948=CARTESIAN_POINT('Ctrl Pts',(-17.9079377746111,-15.678532821646,
12.));
#196949=CARTESIAN_POINT('Ctrl Pts',(-17.897724427724,-15.661006732103,0.));
#196950=CARTESIAN_POINT('Ctrl Pts',(-17.897724427724,-15.661006732103,12.));
#196951=CARTESIAN_POINT('Ctrl Pts',(-17.8875189181091,-15.6436014971084,
0.));
#196952=CARTESIAN_POINT('Ctrl Pts',(-17.8875189181091,-15.6436014971084,
12.));
#196953=CARTESIAN_POINT('Ctrl Pts',(-17.8773220648125,-15.6263176459108,
0.));
#196954=CARTESIAN_POINT('Ctrl Pts',(-17.8773220648125,-15.6263176459108,
12.));
#196955=CARTESIAN_POINT('Ctrl Pts',(-17.8671346981394,-15.609155712921,
0.));
#196956=CARTESIAN_POINT('Ctrl Pts',(-17.8671346981394,-15.609155712921,
12.));
#196957=CARTESIAN_POINT('Ctrl Pts',(-17.8569576599006,-15.5921162378192,
0.));
#196958=CARTESIAN_POINT('Ctrl Pts',(-17.8569576599006,-15.5921162378192,
12.));
#196959=CARTESIAN_POINT('Ctrl Pts',(-17.8467918036987,-15.5751997657163,
0.));
#196960=CARTESIAN_POINT('Ctrl Pts',(-17.8467918036987,-15.5751997657163,
12.));
#196961=CARTESIAN_POINT('Ctrl Pts',(-17.8366379952085,-15.5584068472982,
0.));
#196962=CARTESIAN_POINT('Ctrl Pts',(-17.8366379952085,-15.5584068472982,
12.));
#196963=CARTESIAN_POINT('Ctrl Pts',(-17.8264971124607,-15.541738038964,
0.));
#196964=CARTESIAN_POINT('Ctrl Pts',(-17.8264971124607,-15.541738038964,
12.));
#196965=CARTESIAN_POINT('Ctrl Pts',(-17.8163700461256,-15.5251939029552,
0.));
#196966=CARTESIAN_POINT('Ctrl Pts',(-17.8163700461256,-15.5251939029552,
12.));
#196967=CARTESIAN_POINT('Ctrl Pts',(-17.8062576997952,-15.5087750074718,
0.));
#196968=CARTESIAN_POINT('Ctrl Pts',(-17.8062576997952,-15.5087750074718,
12.));
#196969=CARTESIAN_POINT('Ctrl Pts',(-17.7961609903148,-15.4924819268517,
0.));
#196970=CARTESIAN_POINT('Ctrl Pts',(-17.7961609903148,-15.4924819268517,
12.));
#196971=CARTESIAN_POINT('Ctrl Pts',(-17.786080848122,-15.4763152417497,
0.));
#196972=CARTESIAN_POINT('Ctrl Pts',(-17.786080848122,-15.4763152417497,
12.));
#196973=CARTESIAN_POINT('Ctrl Pts',(-17.7760182175815,-15.4602755393017,
0.));
#196974=CARTESIAN_POINT('Ctrl Pts',(-17.7760182175815,-15.4602755393017,
12.));
#196975=CARTESIAN_POINT('Ctrl Pts',(-17.7659740573265,-15.4443634132869,
0.));
#196976=CARTESIAN_POINT('Ctrl Pts',(-17.7659740573265,-15.4443634132869,
12.));
#196977=CARTESIAN_POINT('Ctrl Pts',(-17.7559493405881,-15.4285794642668,
0.));
#196978=CARTESIAN_POINT('Ctrl Pts',(-17.7559493405881,-15.4285794642668,
12.));
#196979=CARTESIAN_POINT('Ctrl Pts',(-17.7459450555812,-15.4129242997837,
0.));
#196980=CARTESIAN_POINT('Ctrl Pts',(-17.7459450555812,-15.4129242997837,
12.));
#196981=CARTESIAN_POINT('Ctrl Pts',(-17.735962205915,-15.3973985345802,
0.));
#196982=CARTESIAN_POINT('Ctrl Pts',(-17.735962205915,-15.3973985345802,
12.));
#196983=CARTESIAN_POINT('Ctrl Pts',(-17.7260018109924,-15.3820027907967,
0.));
#196984=CARTESIAN_POINT('Ctrl Pts',(-17.7260018109924,-15.3820027907967,
12.));
#196985=CARTESIAN_POINT('Ctrl Pts',(-17.7160649064206,-15.3667376981699,
0.));
#196986=CARTESIAN_POINT('Ctrl Pts',(-17.7160649064206,-15.3667376981699,
12.));
#196987=CARTESIAN_POINT('Ctrl Pts',(-17.7061525444042,-15.351603894206,
0.));
#196988=CARTESIAN_POINT('Ctrl Pts',(-17.7061525444042,-15.351603894206,
12.));
#196989=CARTESIAN_POINT('Ctrl Pts',(-17.6962657941983,-15.3366020244066,
0.));
#196990=CARTESIAN_POINT('Ctrl Pts',(-17.6962657941983,-15.3366020244066,
12.));
#196991=CARTESIAN_POINT('Ctrl Pts',(-17.6864057426052,-15.3217327425338,
0.));
#196992=CARTESIAN_POINT('Ctrl Pts',(-17.6864057426052,-15.3217327425338,
12.));
#196993=CARTESIAN_POINT('Ctrl Pts',(-17.676573494456,-15.3069967108501,
0.));
#196994=CARTESIAN_POINT('Ctrl Pts',(-17.676573494456,-15.3069967108501,
12.));
#196995=CARTESIAN_POINT('Ctrl Pts',(-17.6667701731041,-15.2923946003598,
0.));
#196996=CARTESIAN_POINT('Ctrl Pts',(-17.6667701731041,-15.2923946003598,
12.));
#196997=CARTESIAN_POINT('Ctrl Pts',(-17.6569969209,-15.2779270910239,0.));
#196998=CARTESIAN_POINT('Ctrl Pts',(-17.6569969209,-15.2779270910239,12.));
#196999=CARTESIAN_POINT('Ctrl Pts',(-17.6472548997328,-15.2635948720292,
0.));
#197000=CARTESIAN_POINT('Ctrl Pts',(-17.6472548997328,-15.2635948720292,
12.));
#197001=CARTESIAN_POINT('Ctrl Pts',(-17.6375452916369,-15.2493986421092,
0.));
#197002=CARTESIAN_POINT('Ctrl Pts',(-17.6375452916369,-15.2493986421092,
12.));
#197003=CARTESIAN_POINT('Ctrl Pts',(-17.6278692993764,-15.2353391098366,
0.));
#197004=CARTESIAN_POINT('Ctrl Pts',(-17.6278692993764,-15.2353391098366,
12.));
#197005=CARTESIAN_POINT('Ctrl Pts',(-17.6182281470468,-15.2214169939199,
0.));
#197006=CARTESIAN_POINT('Ctrl Pts',(-17.6182281470468,-15.2214169939199,
12.));
#197007=CARTESIAN_POINT('Ctrl Pts',(-17.60862308065,-15.2076330234686,0.));
#197008=CARTESIAN_POINT('Ctrl Pts',(-17.60862308065,-15.2076330234686,12.));
#197009=CARTESIAN_POINT('Ctrl Pts',(-17.5990553687599,-15.1939879383268,
0.));
#197010=CARTESIAN_POINT('Ctrl Pts',(-17.5990553687599,-15.1939879383268,
12.));
#197011=CARTESIAN_POINT('Ctrl Pts',(-17.5895263032595,-15.1804824894605,
0.));
#197012=CARTESIAN_POINT('Ctrl Pts',(-17.5895263032595,-15.1804824894605,
12.));
#197013=CARTESIAN_POINT('Ctrl Pts',(-17.580037200054,-15.1671174393137,
0.));
#197014=CARTESIAN_POINT('Ctrl Pts',(-17.580037200054,-15.1671174393137,
12.));
#197015=CARTESIAN_POINT('Ctrl Pts',(-17.5705893998029,-15.1538935621714,
0.));
#197016=CARTESIAN_POINT('Ctrl Pts',(-17.5705893998029,-15.1538935621714,
12.));
#197017=CARTESIAN_POINT('Ctrl Pts',(-17.5611842686192,-15.1408116444876,
0.));
#197018=CARTESIAN_POINT('Ctrl Pts',(-17.5611842686192,-15.1408116444876,
12.));
#197019=CARTESIAN_POINT('Ctrl Pts',(-17.5518231989117,-15.1278724853138,
0.));
#197020=CARTESIAN_POINT('Ctrl Pts',(-17.5518231989117,-15.1278724853138,
12.));
#197021=CARTESIAN_POINT('Ctrl Pts',(-17.5425076102963,-15.1150768967728,
0.));
#197022=CARTESIAN_POINT('Ctrl Pts',(-17.5425076102963,-15.1150768967728,
12.));
#197023=CARTESIAN_POINT('Ctrl Pts',(-17.5332389504829,-15.1024257045033,
0.));
#197024=CARTESIAN_POINT('Ctrl Pts',(-17.5332389504829,-15.1024257045033,
12.));
#197025=CARTESIAN_POINT('Ctrl Pts',(-17.5240186961791,-15.0899197481082,
0.));
#197026=CARTESIAN_POINT('Ctrl Pts',(-17.5240186961791,-15.0899197481082,
12.));
#197027=CARTESIAN_POINT('Ctrl Pts',(-17.5148483539687,-15.0775598815749,
0.));
#197028=CARTESIAN_POINT('Ctrl Pts',(-17.5148483539687,-15.0775598815749,
12.));
#197029=CARTESIAN_POINT('Ctrl Pts',(-17.5057294613877,-15.0653469738307,
0.));
#197030=CARTESIAN_POINT('Ctrl Pts',(-17.5057294613877,-15.0653469738307,
12.));
#197031=CARTESIAN_POINT('Ctrl Pts',(-17.4966635880246,-15.0532819093085,
0.));
#197032=CARTESIAN_POINT('Ctrl Pts',(-17.4966635880246,-15.0532819093085,
12.));
#197033=CARTESIAN_POINT('Ctrl Pts',(-17.4876523366178,-15.0413655884993,
0.));
#197034=CARTESIAN_POINT('Ctrl Pts',(-17.4876523366178,-15.0413655884993,
12.));
#197035=CARTESIAN_POINT('Ctrl Pts',(-17.4786973441417,-15.029598928488,
0.));
#197036=CARTESIAN_POINT('Ctrl Pts',(-17.4786973441417,-15.029598928488,
12.));
#197037=CARTESIAN_POINT('Ctrl Pts',(-17.4698002829357,-15.0179828635087,
0.));
#197038=CARTESIAN_POINT('Ctrl Pts',(-17.4698002829357,-15.0179828635087,
12.));
#197039=CARTESIAN_POINT('Ctrl Pts',(-17.4609628621419,-15.0065183456922,
0.));
#197040=CARTESIAN_POINT('Ctrl Pts',(-17.4609628621419,-15.0065183456922,
12.));
#197041=CARTESIAN_POINT('Ctrl Pts',(-17.4521868291005,-14.9952063457779,
0.));
#197042=CARTESIAN_POINT('Ctrl Pts',(-17.4521868291005,-14.9952063457779,
12.));
#197043=CARTESIAN_POINT('Ctrl Pts',(-17.4434739707773,-14.9840478538357,
0.));
#197044=CARTESIAN_POINT('Ctrl Pts',(-17.4434739707773,-14.9840478538357,
12.));
#197045=CARTESIAN_POINT('Ctrl Pts',(-17.4348261151395,-14.973043879945,
0.));
#197046=CARTESIAN_POINT('Ctrl Pts',(-17.4348261151395,-14.973043879945,
12.));
#197047=CARTESIAN_POINT('Ctrl Pts',(-17.4262451327088,-14.9621954549825,
0.));
#197048=CARTESIAN_POINT('Ctrl Pts',(-17.4262451327088,-14.9621954549825,
12.));
#197049=CARTESIAN_POINT('Ctrl Pts',(-17.4177329382827,-14.9515036315142,
0.));
#197050=CARTESIAN_POINT('Ctrl Pts',(-17.4177329382827,-14.9515036315142,
12.));
#197051=CARTESIAN_POINT('Ctrl Pts',(-17.4092914926071,-14.940969484645,
0.));
#197052=CARTESIAN_POINT('Ctrl Pts',(-17.4092914926071,-14.940969484645,
12.));
#197053=CARTESIAN_POINT('Ctrl Pts',(-17.400922804075,-14.9305941128758,
0.));
#197054=CARTESIAN_POINT('Ctrl Pts',(-17.400922804075,-14.9305941128758,
12.));
#197055=CARTESIAN_POINT('Ctrl Pts',(-17.3926289303987,-14.9203786389343,
0.));
#197056=CARTESIAN_POINT('Ctrl Pts',(-17.3926289303987,-14.9203786389343,
12.));
#197057=CARTESIAN_POINT('Ctrl Pts',(-17.3844119809823,-14.9103242110057,
0.));
#197058=CARTESIAN_POINT('Ctrl Pts',(-17.3844119809823,-14.9103242110057,
12.));
#197059=CARTESIAN_POINT('Ctrl Pts',(-17.3762741193075,-14.9004320039609,
0.));
#197060=CARTESIAN_POINT('Ctrl Pts',(-17.3762741193075,-14.9004320039609,
12.));
#197061=CARTESIAN_POINT('Ctrl Pts',(-17.3682175653236,-14.8907032205789,
0.));
#197062=CARTESIAN_POINT('Ctrl Pts',(-17.3682175653236,-14.8907032205789,
12.));
#197063=CARTESIAN_POINT('Ctrl Pts',(-17.3602445978163,-14.8811390927424,
0.));
#197064=CARTESIAN_POINT('Ctrl Pts',(-17.3602445978163,-14.8811390927424,
12.));
#197065=CARTESIAN_POINT('Ctrl Pts',(-17.3523575568648,-14.8717408826958,
0.));
#197066=CARTESIAN_POINT('Ctrl Pts',(-17.3523575568648,-14.8717408826958,
12.));
#197067=CARTESIAN_POINT('Ctrl Pts',(-17.3445588463477,-14.8625098843419,
0.));
#197068=CARTESIAN_POINT('Ctrl Pts',(-17.3445588463477,-14.8625098843419,
12.));
#197069=CARTESIAN_POINT('Ctrl Pts',(-17.336850936485,-14.8534474245433,
0.));
#197070=CARTESIAN_POINT('Ctrl Pts',(-17.336850936485,-14.8534474245433,
12.));
#197071=CARTESIAN_POINT('Ctrl Pts',(-17.3292363662601,-14.8445548643505,
0.));
#197072=CARTESIAN_POINT('Ctrl Pts',(-17.3292363662601,-14.8445548643505,
12.));
#197073=CARTESIAN_POINT('Ctrl Pts',(-17.3217177462096,-14.8358336004193,
0.));
#197074=CARTESIAN_POINT('Ctrl Pts',(-17.3217177462096,-14.8358336004193,
12.));
#197075=CARTESIAN_POINT('Ctrl Pts',(-17.3142977632656,-14.8272850675375,
0.));
#197076=CARTESIAN_POINT('Ctrl Pts',(-17.3142977632656,-14.8272850675375,
12.));
#197077=CARTESIAN_POINT('Ctrl Pts',(-17.3069791853705,-14.8189107410161,
0.));
#197078=CARTESIAN_POINT('Ctrl Pts',(-17.3069791853705,-14.8189107410161,
12.));
#197079=CARTESIAN_POINT('Ctrl Pts',(-17.2997648661483,-14.8107121391038,
0.));
#197080=CARTESIAN_POINT('Ctrl Pts',(-17.2997648661483,-14.8107121391038,
12.));
#197081=CARTESIAN_POINT('Ctrl Pts',(-17.2926577496519,-14.8026908254281,
0.));
#197082=CARTESIAN_POINT('Ctrl Pts',(-17.2926577496519,-14.8026908254281,
12.));
#197083=CARTESIAN_POINT('Ctrl Pts',(-17.28566087332,-14.7948484105253,0.));
#197084=CARTESIAN_POINT('Ctrl Pts',(-17.28566087332,-14.7948484105253,12.));
#197085=CARTESIAN_POINT('Ctrl Pts',(-17.278777370485,-14.787186553128,0.));
#197086=CARTESIAN_POINT('Ctrl Pts',(-17.278777370485,-14.787186553128,12.));
#197087=CARTESIAN_POINT('Ctrl Pts',(-17.2720104735192,-14.7797069617802,
0.));
#197088=CARTESIAN_POINT('Ctrl Pts',(-17.2720104735192,-14.7797069617802,
12.));
#197089=CARTESIAN_POINT('Ctrl Pts',(-17.2653635155317,-14.7724113956728,
0.));
#197090=CARTESIAN_POINT('Ctrl Pts',(-17.2653635155317,-14.7724113956728,
12.));
#197091=CARTESIAN_POINT('Ctrl Pts',(-17.2588399401464,-14.7653016697589,
0.));
#197092=CARTESIAN_POINT('Ctrl Pts',(-17.2588399401464,-14.7653016697589,
12.));
#197093=CARTESIAN_POINT('Ctrl Pts',(-17.2524433146837,-14.7583796616617,
0.));
#197094=CARTESIAN_POINT('Ctrl Pts',(-17.2524433146837,-14.7583796616617,
12.));
#197095=CARTESIAN_POINT('Ctrl Pts',(-17.2461773413289,-14.7516473175125,
0.));
#197096=CARTESIAN_POINT('Ctrl Pts',(-17.2461773413289,-14.7516473175125,
12.));
#197097=CARTESIAN_POINT('Ctrl Pts',(-17.2400458713566,-14.7451066593793,
0.));
#197098=CARTESIAN_POINT('Ctrl Pts',(-17.2400458713566,-14.7451066593793,
12.));
#197099=CARTESIAN_POINT('Ctrl Pts',(-17.2340529062077,-14.7387597858117,
0.));
#197100=CARTESIAN_POINT('Ctrl Pts',(-17.2340529062077,-14.7387597858117,
12.));
#197101=CARTESIAN_POINT('Ctrl Pts',(-17.2282025904314,-14.7326088681163,
0.));
#197102=CARTESIAN_POINT('Ctrl Pts',(-17.2282025904314,-14.7326088681163,
12.));
#197103=CARTESIAN_POINT('Ctrl Pts',(-17.2224992099666,-14.7266561494282,
0.));
#197104=CARTESIAN_POINT('Ctrl Pts',(-17.2224992099666,-14.7266561494282,
12.));
#197105=CARTESIAN_POINT('Ctrl Pts',(-17.2169471814255,-14.7209039390326,
0.));
#197106=CARTESIAN_POINT('Ctrl Pts',(-17.2169471814255,-14.7209039390326,
12.));
#197107=CARTESIAN_POINT('Ctrl Pts',(-17.2115510835988,-14.7153546289338,
0.));
#197108=CARTESIAN_POINT('Ctrl Pts',(-17.2115510835988,-14.7153546289338,
12.));
#197109=CARTESIAN_POINT('Ctrl Pts',(-17.2063157097316,-14.7100107213586,
0.));
#197110=CARTESIAN_POINT('Ctrl Pts',(-17.2063157097316,-14.7100107213586,
12.));
#197111=CARTESIAN_POINT('Ctrl Pts',(-17.2012461084268,-14.7048748502663,
0.));
#197112=CARTESIAN_POINT('Ctrl Pts',(-17.2012461084268,-14.7048748502663,
12.));
#197113=CARTESIAN_POINT('Ctrl Pts',(-17.1963476411694,-14.699949811582,
0.));
#197114=CARTESIAN_POINT('Ctrl Pts',(-17.1963476411694,-14.699949811582,
12.));
#197115=CARTESIAN_POINT('Ctrl Pts',(-17.1916259308416,-14.6952385361706,
0.));
#197116=CARTESIAN_POINT('Ctrl Pts',(-17.1916259308416,-14.6952385361706,
12.));
#197117=CARTESIAN_POINT('Ctrl Pts',(-17.1870867909918,-14.6907440526958,
0.));
#197118=CARTESIAN_POINT('Ctrl Pts',(-17.1870867909918,-14.6907440526958,
12.));
#197119=CARTESIAN_POINT('Ctrl Pts',(-17.182736158472,-14.6864694522319,
0.));
#197120=CARTESIAN_POINT('Ctrl Pts',(-17.182736158472,-14.6864694522319,
12.));
#197121=CARTESIAN_POINT('Ctrl Pts',(-17.1785800350827,-14.6824178576167,
0.));
#197122=CARTESIAN_POINT('Ctrl Pts',(-17.1785800350827,-14.6824178576167,
12.));
#197123=CARTESIAN_POINT('Ctrl Pts',(-17.1746247499057,-14.6785925615676,
0.));
#197124=CARTESIAN_POINT('Ctrl Pts',(-17.1746247499057,-14.6785925615676,
12.));
#197125=CARTESIAN_POINT('Ctrl Pts',(-17.1708771619129,-14.6749971333867,
0.));
#197126=CARTESIAN_POINT('Ctrl Pts',(-17.1708771619129,-14.6749971333867,
12.));
#197127=CARTESIAN_POINT('Ctrl Pts',(-17.1673449723019,-14.6716355833321,
0.));
#197128=CARTESIAN_POINT('Ctrl Pts',(-17.1673449723019,-14.6716355833321,
12.));
#197129=CARTESIAN_POINT('Ctrl Pts',(-17.1640366762304,-14.6685123374424,
0.));
#197130=CARTESIAN_POINT('Ctrl Pts',(-17.1640366762304,-14.6685123374424,
12.));
#197131=CARTESIAN_POINT('Ctrl Pts',(-17.1609609517369,-14.6656319165057,
0.));
#197132=CARTESIAN_POINT('Ctrl Pts',(-17.1609609517369,-14.6656319165057,
12.));
#197133=CARTESIAN_POINT('Ctrl Pts',(-17.1581262646789,-14.662998728599,
0.));
#197134=CARTESIAN_POINT('Ctrl Pts',(-17.1581262646789,-14.662998728599,
12.));
#197135=CARTESIAN_POINT('Ctrl Pts',(-17.1555401986403,-14.660616716964,
0.));
#197136=CARTESIAN_POINT('Ctrl Pts',(-17.1555401986403,-14.660616716964,
12.));
#197137=CARTESIAN_POINT('Ctrl Pts',(-17.1532107762719,-14.6584900555301,
0.));
#197138=CARTESIAN_POINT('Ctrl Pts',(-17.1532107762719,-14.6584900555301,
12.));
#197139=CARTESIAN_POINT('Ctrl Pts',(-17.1511476869495,-14.6566237952435,
0.));
#197140=CARTESIAN_POINT('Ctrl Pts',(-17.1511476869495,-14.6566237952435,
12.));
#197141=CARTESIAN_POINT('Ctrl Pts',(-17.1493641837556,-14.6550248622813,
0.));
#197142=CARTESIAN_POINT('Ctrl Pts',(-17.1493641837556,-14.6550248622813,
12.));
#197143=CARTESIAN_POINT('Ctrl Pts',(-17.1478763944909,-14.6537016966188,
0.));
#197144=CARTESIAN_POINT('Ctrl Pts',(-17.1478763944909,-14.6537016966188,
12.));
#197145=CARTESIAN_POINT('Ctrl Pts',(-17.1466998098673,-14.6526624064978,
0.));
#197146=CARTESIAN_POINT('Ctrl Pts',(-17.1466998098673,-14.6526624064978,
12.));
#197147=CARTESIAN_POINT('Ctrl Pts',(-17.1458462295273,-14.65191316345,0.));
#197148=CARTESIAN_POINT('Ctrl Pts',(-17.1458462295273,-14.65191316345,12.));
#197149=CARTESIAN_POINT('Ctrl Pts',(-17.1454262858045,-14.6515481598057,
0.));
#197150=CARTESIAN_POINT('Ctrl Pts',(-17.1454262858045,-14.6515481598057,
12.));
#197151=CARTESIAN_POINT('Ctrl Pts',(-17.1452600887039,-14.6514066997188,
0.));
#197152=CARTESIAN_POINT('Ctrl Pts',(-17.1452600887039,-14.6514066997188,
12.));
#197153=CARTESIAN_POINT('Ctrl Pts',(-17.1452153999142,-14.651371185284,
0.));
#197154=CARTESIAN_POINT('Ctrl Pts',(-17.1452153999142,-14.651371185284,
12.));
#197155=CARTESIAN_POINT('Ctrl Pts',(-17.1452095830633,-14.6513681262571,
0.));
#197156=CARTESIAN_POINT('Ctrl Pts',(-17.1452095830633,-14.6513681262571,
12.));
#197157=CARTESIAN_POINT('',(-18.8464468996588,-17.9112098770111,0.));
#197158=CARTESIAN_POINT('Ctrl Pts',(-18.8464468996588,-17.9112098770111,
0.));
#197159=CARTESIAN_POINT('Ctrl Pts',(-18.8448126709692,-17.9057348246595,
0.));
#197160=CARTESIAN_POINT('Ctrl Pts',(-18.8415402351786,-17.8947931177807,
0.));
#197161=CARTESIAN_POINT('Ctrl Pts',(-18.8366196462581,-17.8784057509356,
0.));
#197162=CARTESIAN_POINT('Ctrl Pts',(-18.8300349895974,-17.8566063174771,
0.));
#197163=CARTESIAN_POINT('Ctrl Pts',(-18.8217643886157,-17.8294410311006,
0.));
#197164=CARTESIAN_POINT('Ctrl Pts',(-18.8134540340417,-17.8023598011057,
0.));
#197165=CARTESIAN_POINT('Ctrl Pts',(-18.8051039860448,-17.7753627137853,
0.));
#197166=CARTESIAN_POINT('Ctrl Pts',(-18.7967143519419,-17.7484498996905,
0.));
#197167=CARTESIAN_POINT('Ctrl Pts',(-18.788285297605,-17.7216215409035,
0.));
#197168=CARTESIAN_POINT('Ctrl Pts',(-18.7798170641374,-17.6948778823014,
0.));
#197169=CARTESIAN_POINT('Ctrl Pts',(-18.7713099642754,-17.6682192274236,
0.));
#197170=CARTESIAN_POINT('Ctrl Pts',(-18.762764361321,-17.6416459210681,
0.));
#197171=CARTESIAN_POINT('Ctrl Pts',(-18.7541806530984,-17.6151583357012,
0.));
#197172=CARTESIAN_POINT('Ctrl Pts',(-18.7455592536687,-17.5887568561371,
0.));
#197173=CARTESIAN_POINT('Ctrl Pts',(-18.7369005764553,-17.5624418653245,
0.));
#197174=CARTESIAN_POINT('Ctrl Pts',(-18.7282050157138,-17.5362137287593,
0.));
#197175=CARTESIAN_POINT('Ctrl Pts',(-18.7194729318098,-17.5100727820876,
0.));
#197176=CARTESIAN_POINT('Ctrl Pts',(-18.7107046613912,-17.4840193397162,
0.));
#197177=CARTESIAN_POINT('Ctrl Pts',(-18.70190052503,-17.4580537012753,0.));
#197178=CARTESIAN_POINT('Ctrl Pts',(-18.6930608357409,-17.4321761588142,
0.));
#197179=CARTESIAN_POINT('Ctrl Pts',(-18.6841859073471,-17.4063870038562,
0.));
#197180=CARTESIAN_POINT('Ctrl Pts',(-18.6752760624052,-17.3806865340747,
0.));
#197181=CARTESIAN_POINT('Ctrl Pts',(-18.6663316416582,-17.3550750612443,
0.));
#197182=CARTESIAN_POINT('Ctrl Pts',(-18.6573530024033,-17.3295529098618,
0.));
#197183=CARTESIAN_POINT('Ctrl Pts',(-18.6483405141865,-17.3041204135074,
0.));
#197184=CARTESIAN_POINT('Ctrl Pts',(-18.6392945554748,-17.2787779120213,
0.));
#197185=CARTESIAN_POINT('Ctrl Pts',(-18.6302155097943,-17.2535257482187,
0.));
#197186=CARTESIAN_POINT('Ctrl Pts',(-18.6211037624038,-17.2283642650518,
0.));
#197187=CARTESIAN_POINT('Ctrl Pts',(-18.6119596959949,-17.2032938019284,
0.));
#197188=CARTESIAN_POINT('Ctrl Pts',(-18.6027836898817,-17.1783146940127,
0.));
#197189=CARTESIAN_POINT('Ctrl Pts',(-18.5935761222825,-17.1534272741643,
0.));
#197190=CARTESIAN_POINT('Ctrl Pts',(-18.5843373717247,-17.1286318741183,
0.));
#197191=CARTESIAN_POINT('Ctrl Pts',(-18.5750678188542,-17.1039288260001,
0.));
#197192=CARTESIAN_POINT('Ctrl Pts',(-18.5657678479789,-17.0793184636079,
0.));
#197193=CARTESIAN_POINT('Ctrl Pts',(-18.556437848963,-17.0548011239751,
0.));
#197194=CARTESIAN_POINT('Ctrl Pts',(-18.547078218209,-17.0303771481738,
0.));
#197195=CARTESIAN_POINT('Ctrl Pts',(-18.5376893576961,-17.0060468805097,
0.));
#197196=CARTESIAN_POINT('Ctrl Pts',(-18.5282716744197,-16.981810668038,
0.));
#197197=CARTESIAN_POINT('Ctrl Pts',(-18.5188255796659,-16.9576688599339,
0.));
#197198=CARTESIAN_POINT('Ctrl Pts',(-18.5093514883835,-16.9336218069353,
0.));
#197199=CARTESIAN_POINT('Ctrl Pts',(-18.499849818462,-16.9096698606943,
0.));
#197200=CARTESIAN_POINT('Ctrl Pts',(-18.4903209902227,-16.8858133733088,
0.));
#197201=CARTESIAN_POINT('Ctrl Pts',(-18.4807654268771,-16.8620526977171,
0.));
#197202=CARTESIAN_POINT('Ctrl Pts',(-18.4711835548623,-16.8383881879709,
0.));
#197203=CARTESIAN_POINT('Ctrl Pts',(-18.4615758042305,-16.8148201995472,
0.));
#197204=CARTESIAN_POINT('Ctrl Pts',(-18.4519426090124,-16.791349089629,
0.));
#197205=CARTESIAN_POINT('Ctrl Pts',(-18.44228440761,-16.7679752173992,0.));
#197206=CARTESIAN_POINT('Ctrl Pts',(-18.4326016431392,-16.7446989442882,
0.));
#197207=CARTESIAN_POINT('Ctrl Pts',(-18.4228947633187,-16.7215206338818,
0.));
#197208=CARTESIAN_POINT('Ctrl Pts',(-18.413164220399,-16.6984406518491,
0.));
#197209=CARTESIAN_POINT('Ctrl Pts',(-18.403410471079,-16.6754593658513,
0.));
#197210=CARTESIAN_POINT('Ctrl Pts',(-18.3936339764332,-16.6525771454513,
0.));
#197211=CARTESIAN_POINT('Ctrl Pts',(-18.3838352018327,-16.6297943620056,
0.));
#197212=CARTESIAN_POINT('Ctrl Pts',(-18.3740146168879,-16.607111388571,
0.));
#197213=CARTESIAN_POINT('Ctrl Pts',(-18.3641726955889,-16.5845286000217,
0.));
#197214=CARTESIAN_POINT('Ctrl Pts',(-18.354309916433,-16.5620463731413,
0.));
#197215=CARTESIAN_POINT('Ctrl Pts',(-18.34442676256,-16.5396650867139,0.));
#197216=CARTESIAN_POINT('Ctrl Pts',(-18.3345237218864,-16.5173851216045,
0.));
#197217=CARTESIAN_POINT('Ctrl Pts',(-18.3246012872469,-16.4952068608345,
0.));
#197218=CARTESIAN_POINT('Ctrl Pts',(-18.3146599565231,-16.4731306896441,
0.));
#197219=CARTESIAN_POINT('Ctrl Pts',(-18.304700232686,-16.4511569955233,
0.));
#197220=CARTESIAN_POINT('Ctrl Pts',(-18.294722623851,-16.4292861682379,
0.));
#197221=CARTESIAN_POINT('Ctrl Pts',(-18.2847276433309,-16.4075185998455,
0.));
#197222=CARTESIAN_POINT('Ctrl Pts',(-18.2747158096934,-16.385854684708,
0.));
#197223=CARTESIAN_POINT('Ctrl Pts',(-18.2646876468169,-16.3642948194868,
0.));
#197224=CARTESIAN_POINT('Ctrl Pts',(-18.2546436839608,-16.3428394031589,
0.));
#197225=CARTESIAN_POINT('Ctrl Pts',(-18.2445844558742,-16.3214888370987,
0.));
#197226=CARTESIAN_POINT('Ctrl Pts',(-18.2345105028982,-16.3002435251378,
0.));
#197227=CARTESIAN_POINT('Ctrl Pts',(-18.2244223710746,-16.2791038736223,
0.));
#197228=CARTESIAN_POINT('Ctrl Pts',(-18.2143206122529,-16.2580702914615,
0.));
#197229=CARTESIAN_POINT('Ctrl Pts',(-18.2042057842035,-16.2371431901638,
0.));
#197230=CARTESIAN_POINT('Ctrl Pts',(-18.1940784507229,-16.2163229838875,
0.));
#197231=CARTESIAN_POINT('Ctrl Pts',(-18.1839391817331,-16.1956100895073,
0.));
#197232=CARTESIAN_POINT('Ctrl Pts',(-18.1737885533849,-16.1750049266671,
0.));
#197233=CARTESIAN_POINT('Ctrl Pts',(-18.1636271481615,-16.154507917826,
0.));
#197234=CARTESIAN_POINT('Ctrl Pts',(-18.1534555549852,-16.1341194882988,
0.));
#197235=CARTESIAN_POINT('Ctrl Pts',(-18.1432743693235,-16.1138400662794,
0.));
#197236=CARTESIAN_POINT('Ctrl Pts',(-18.1330841933105,-16.0936700829112,
0.));
#197237=CARTESIAN_POINT('Ctrl Pts',(-18.1228856358751,-16.0736099723668,
0.));
#197238=CARTESIAN_POINT('Ctrl Pts',(-18.112679312869,-16.0536601719126,
0.));
#197239=CARTESIAN_POINT('Ctrl Pts',(-18.1024658471966,-16.0338211219693,
0.));
#197240=CARTESIAN_POINT('Ctrl Pts',(-18.0922458689462,-16.014093266161,
0.));
#197241=CARTESIAN_POINT('Ctrl Pts',(-18.0820200155236,-15.9944770513613,
0.));
#197242=CARTESIAN_POINT('Ctrl Pts',(-18.0717889317958,-15.9749729277846,
0.));
#197243=CARTESIAN_POINT('Ctrl Pts',(-18.061553270236,-15.9555813490644,
0.));
#197244=CARTESIAN_POINT('Ctrl Pts',(-18.0513136910691,-15.9363027723244,
0.));
#197245=CARTESIAN_POINT('Ctrl Pts',(-18.0410708624208,-15.9171376582436,
0.));
#197246=CARTESIAN_POINT('Ctrl Pts',(-18.0308254604636,-15.8980864711042,
0.));
#197247=CARTESIAN_POINT('Ctrl Pts',(-18.0205781695769,-15.8791496788682,
0.));
#197248=CARTESIAN_POINT('Ctrl Pts',(-18.0103296825205,-15.8603277532831,
0.));
#197249=CARTESIAN_POINT('Ctrl Pts',(-18.0000807006052,-15.8416211699679,
0.));
#197250=CARTESIAN_POINT('Ctrl Pts',(-17.9898319338664,-15.8230304084962,
0.));
#197251=CARTESIAN_POINT('Ctrl Pts',(-17.9795841012386,-15.8045559524676,
0.));
#197252=CARTESIAN_POINT('Ctrl Pts',(-17.9693379307303,-15.7861982895724,
0.));
#197253=CARTESIAN_POINT('Ctrl Pts',(-17.9590941596242,-15.7679579117077,
0.));
#197254=CARTESIAN_POINT('Ctrl Pts',(-17.9488535346781,-15.749835315086,
0.));
#197255=CARTESIAN_POINT('Ctrl Pts',(-17.9386168123262,-15.7318310003335,
0.));
#197256=CARTESIAN_POINT('Ctrl Pts',(-17.9283847588836,-15.7139454725838,
0.));
#197257=CARTESIAN_POINT('Ctrl Pts',(-17.9181581507455,-15.6961792415522,
0.));
#197258=CARTESIAN_POINT('Ctrl Pts',(-17.9079377746111,-15.678532821646,
0.));
#197259=CARTESIAN_POINT('Ctrl Pts',(-17.897724427724,-15.661006732103,0.));
#197260=CARTESIAN_POINT('Ctrl Pts',(-17.8875189181091,-15.6436014971084,
0.));
#197261=CARTESIAN_POINT('Ctrl Pts',(-17.8773220648125,-15.6263176459108,
0.));
#197262=CARTESIAN_POINT('Ctrl Pts',(-17.8671346981394,-15.609155712921,
0.));
#197263=CARTESIAN_POINT('Ctrl Pts',(-17.8569576599006,-15.5921162378192,
0.));
#197264=CARTESIAN_POINT('Ctrl Pts',(-17.8467918036987,-15.5751997657163,
0.));
#197265=CARTESIAN_POINT('Ctrl Pts',(-17.8366379952085,-15.5584068472982,
0.));
#197266=CARTESIAN_POINT('Ctrl Pts',(-17.8264971124607,-15.541738038964,
0.));
#197267=CARTESIAN_POINT('Ctrl Pts',(-17.8163700461256,-15.5251939029552,
0.));
#197268=CARTESIAN_POINT('Ctrl Pts',(-17.8062576997952,-15.5087750074718,
0.));
#197269=CARTESIAN_POINT('Ctrl Pts',(-17.7961609903148,-15.4924819268517,
0.));
#197270=CARTESIAN_POINT('Ctrl Pts',(-17.786080848122,-15.4763152417497,
0.));
#197271=CARTESIAN_POINT('Ctrl Pts',(-17.7760182175815,-15.4602755393017,
0.));
#197272=CARTESIAN_POINT('Ctrl Pts',(-17.7659740573265,-15.4443634132869,
0.));
#197273=CARTESIAN_POINT('Ctrl Pts',(-17.7559493405881,-15.4285794642668,
0.));
#197274=CARTESIAN_POINT('Ctrl Pts',(-17.7459450555812,-15.4129242997837,
0.));
#197275=CARTESIAN_POINT('Ctrl Pts',(-17.735962205915,-15.3973985345802,
0.));
#197276=CARTESIAN_POINT('Ctrl Pts',(-17.7260018109924,-15.3820027907967,
0.));
#197277=CARTESIAN_POINT('Ctrl Pts',(-17.7160649064206,-15.3667376981699,
0.));
#197278=CARTESIAN_POINT('Ctrl Pts',(-17.7061525444042,-15.351603894206,
0.));
#197279=CARTESIAN_POINT('Ctrl Pts',(-17.6962657941983,-15.3366020244066,
0.));
#197280=CARTESIAN_POINT('Ctrl Pts',(-17.6864057426052,-15.3217327425338,
0.));
#197281=CARTESIAN_POINT('Ctrl Pts',(-17.676573494456,-15.3069967108501,
0.));
#197282=CARTESIAN_POINT('Ctrl Pts',(-17.6667701731041,-15.2923946003598,
0.));
#197283=CARTESIAN_POINT('Ctrl Pts',(-17.6569969209,-15.2779270910239,0.));
#197284=CARTESIAN_POINT('Ctrl Pts',(-17.6472548997328,-15.2635948720292,
0.));
#197285=CARTESIAN_POINT('Ctrl Pts',(-17.6375452916369,-15.2493986421092,
0.));
#197286=CARTESIAN_POINT('Ctrl Pts',(-17.6278692993764,-15.2353391098366,
0.));
#197287=CARTESIAN_POINT('Ctrl Pts',(-17.6182281470468,-15.2214169939199,
0.));
#197288=CARTESIAN_POINT('Ctrl Pts',(-17.60862308065,-15.2076330234686,0.));
#197289=CARTESIAN_POINT('Ctrl Pts',(-17.5990553687599,-15.1939879383268,
0.));
#197290=CARTESIAN_POINT('Ctrl Pts',(-17.5895263032595,-15.1804824894605,
0.));
#197291=CARTESIAN_POINT('Ctrl Pts',(-17.580037200054,-15.1671174393137,
0.));
#197292=CARTESIAN_POINT('Ctrl Pts',(-17.5705893998029,-15.1538935621714,
0.));
#197293=CARTESIAN_POINT('Ctrl Pts',(-17.5611842686192,-15.1408116444876,
0.));
#197294=CARTESIAN_POINT('Ctrl Pts',(-17.5518231989117,-15.1278724853138,
0.));
#197295=CARTESIAN_POINT('Ctrl Pts',(-17.5425076102963,-15.1150768967728,
0.));
#197296=CARTESIAN_POINT('Ctrl Pts',(-17.5332389504829,-15.1024257045033,
0.));
#197297=CARTESIAN_POINT('Ctrl Pts',(-17.5240186961791,-15.0899197481082,
0.));
#197298=CARTESIAN_POINT('Ctrl Pts',(-17.5148483539687,-15.0775598815749,
0.));
#197299=CARTESIAN_POINT('Ctrl Pts',(-17.5057294613877,-15.0653469738307,
0.));
#197300=CARTESIAN_POINT('Ctrl Pts',(-17.4966635880246,-15.0532819093085,
0.));
#197301=CARTESIAN_POINT('Ctrl Pts',(-17.4876523366178,-15.0413655884993,
0.));
#197302=CARTESIAN_POINT('Ctrl Pts',(-17.4786973441417,-15.029598928488,
0.));
#197303=CARTESIAN_POINT('Ctrl Pts',(-17.4698002829357,-15.0179828635087,
0.));
#197304=CARTESIAN_POINT('Ctrl Pts',(-17.4609628621419,-15.0065183456922,
0.));
#197305=CARTESIAN_POINT('Ctrl Pts',(-17.4521868291005,-14.9952063457779,
0.));
#197306=CARTESIAN_POINT('Ctrl Pts',(-17.4434739707773,-14.9840478538357,
0.));
#197307=CARTESIAN_POINT('Ctrl Pts',(-17.4348261151395,-14.973043879945,
0.));
#197308=CARTESIAN_POINT('Ctrl Pts',(-17.4262451327088,-14.9621954549825,
0.));
#197309=CARTESIAN_POINT('Ctrl Pts',(-17.4177329382827,-14.9515036315142,
0.));
#197310=CARTESIAN_POINT('Ctrl Pts',(-17.4092914926071,-14.940969484645,
0.));
#197311=CARTESIAN_POINT('Ctrl Pts',(-17.400922804075,-14.9305941128758,
0.));
#197312=CARTESIAN_POINT('Ctrl Pts',(-17.3926289303987,-14.9203786389343,
0.));
#197313=CARTESIAN_POINT('Ctrl Pts',(-17.3844119809823,-14.9103242110057,
0.));
#197314=CARTESIAN_POINT('Ctrl Pts',(-17.3762741193075,-14.9004320039609,
0.));
#197315=CARTESIAN_POINT('Ctrl Pts',(-17.3682175653236,-14.8907032205789,
0.));
#197316=CARTESIAN_POINT('Ctrl Pts',(-17.3602445978163,-14.8811390927424,
0.));
#197317=CARTESIAN_POINT('Ctrl Pts',(-17.3523575568648,-14.8717408826958,
0.));
#197318=CARTESIAN_POINT('Ctrl Pts',(-17.3445588463477,-14.8625098843419,
0.));
#197319=CARTESIAN_POINT('Ctrl Pts',(-17.336850936485,-14.8534474245433,
0.));
#197320=CARTESIAN_POINT('Ctrl Pts',(-17.3292363662601,-14.8445548643505,
0.));
#197321=CARTESIAN_POINT('Ctrl Pts',(-17.3217177462096,-14.8358336004193,
0.));
#197322=CARTESIAN_POINT('Ctrl Pts',(-17.3142977632656,-14.8272850675375,
0.));
#197323=CARTESIAN_POINT('Ctrl Pts',(-17.3069791853705,-14.8189107410161,
0.));
#197324=CARTESIAN_POINT('Ctrl Pts',(-17.2997648661483,-14.8107121391038,
0.));
#197325=CARTESIAN_POINT('Ctrl Pts',(-17.2926577496519,-14.8026908254281,
0.));
#197326=CARTESIAN_POINT('Ctrl Pts',(-17.28566087332,-14.7948484105253,0.));
#197327=CARTESIAN_POINT('Ctrl Pts',(-17.278777370485,-14.787186553128,0.));
#197328=CARTESIAN_POINT('Ctrl Pts',(-17.2720104735192,-14.7797069617802,
0.));
#197329=CARTESIAN_POINT('Ctrl Pts',(-17.2653635155317,-14.7724113956728,
0.));
#197330=CARTESIAN_POINT('Ctrl Pts',(-17.2588399401464,-14.7653016697589,
0.));
#197331=CARTESIAN_POINT('Ctrl Pts',(-17.2524433146837,-14.7583796616617,
0.));
#197332=CARTESIAN_POINT('Ctrl Pts',(-17.2461773413289,-14.7516473175125,
0.));
#197333=CARTESIAN_POINT('Ctrl Pts',(-17.2400458713566,-14.7451066593793,
0.));
#197334=CARTESIAN_POINT('Ctrl Pts',(-17.2340529062077,-14.7387597858117,
0.));
#197335=CARTESIAN_POINT('Ctrl Pts',(-17.2282025904314,-14.7326088681163,
0.));
#197336=CARTESIAN_POINT('Ctrl Pts',(-17.2224992099666,-14.7266561494282,
0.));
#197337=CARTESIAN_POINT('Ctrl Pts',(-17.2169471814255,-14.7209039390326,
0.));
#197338=CARTESIAN_POINT('Ctrl Pts',(-17.2115510835988,-14.7153546289338,
0.));
#197339=CARTESIAN_POINT('Ctrl Pts',(-17.2063157097316,-14.7100107213586,
0.));
#197340=CARTESIAN_POINT('Ctrl Pts',(-17.2012461084268,-14.7048748502663,
0.));
#197341=CARTESIAN_POINT('Ctrl Pts',(-17.1963476411694,-14.699949811582,
0.));
#197342=CARTESIAN_POINT('Ctrl Pts',(-17.1916259308416,-14.6952385361706,
0.));
#197343=CARTESIAN_POINT('Ctrl Pts',(-17.1870867909918,-14.6907440526958,
0.));
#197344=CARTESIAN_POINT('Ctrl Pts',(-17.182736158472,-14.6864694522319,
0.));
#197345=CARTESIAN_POINT('Ctrl Pts',(-17.1785800350827,-14.6824178576167,
0.));
#197346=CARTESIAN_POINT('Ctrl Pts',(-17.1746247499057,-14.6785925615676,
0.));
#197347=CARTESIAN_POINT('Ctrl Pts',(-17.1708771619129,-14.6749971333867,
0.));
#197348=CARTESIAN_POINT('Ctrl Pts',(-17.1673449723019,-14.6716355833321,
0.));
#197349=CARTESIAN_POINT('Ctrl Pts',(-17.1640366762304,-14.6685123374424,
0.));
#197350=CARTESIAN_POINT('Ctrl Pts',(-17.1609609517369,-14.6656319165057,
0.));
#197351=CARTESIAN_POINT('Ctrl Pts',(-17.1581262646789,-14.662998728599,
0.));
#197352=CARTESIAN_POINT('Ctrl Pts',(-17.1555401986403,-14.660616716964,
0.));
#197353=CARTESIAN_POINT('Ctrl Pts',(-17.1532107762719,-14.6584900555301,
0.));
#197354=CARTESIAN_POINT('Ctrl Pts',(-17.1511476869495,-14.6566237952435,
0.));
#197355=CARTESIAN_POINT('Ctrl Pts',(-17.1493641837556,-14.6550248622813,
0.));
#197356=CARTESIAN_POINT('Ctrl Pts',(-17.1478763944909,-14.6537016966188,
0.));
#197357=CARTESIAN_POINT('Ctrl Pts',(-17.1466998098673,-14.6526624064978,
0.));
#197358=CARTESIAN_POINT('Ctrl Pts',(-17.1458462295273,-14.65191316345,0.));
#197359=CARTESIAN_POINT('Ctrl Pts',(-17.1454262858045,-14.6515481598057,
0.));
#197360=CARTESIAN_POINT('Ctrl Pts',(-17.1452600887039,-14.6514066997188,
0.));
#197361=CARTESIAN_POINT('Ctrl Pts',(-17.1452153999142,-14.651371185284,
0.));
#197362=CARTESIAN_POINT('Ctrl Pts',(-17.1452095830633,-14.6513681262571,
0.));
#197363=CARTESIAN_POINT('',(-18.8464468996588,-17.9112098770111,0.));
#197364=CARTESIAN_POINT('Ctrl Pts',(-18.5896416359912,-12.7689476255363,
0.));
#197365=CARTESIAN_POINT('Ctrl Pts',(-18.5896416359912,-12.7689476255363,
12.));
#197366=CARTESIAN_POINT('Ctrl Pts',(-18.5896460962964,-12.7689524524483,
0.));
#197367=CARTESIAN_POINT('Ctrl Pts',(-18.5896460962964,-12.7689524524483,
12.));
#197368=CARTESIAN_POINT('Ctrl Pts',(-18.5896919669165,-12.768986426692,
0.));
#197369=CARTESIAN_POINT('Ctrl Pts',(-18.5896919669165,-12.768986426692,
12.));
#197370=CARTESIAN_POINT('Ctrl Pts',(-18.589871621843,-12.769110348199,0.));
#197371=CARTESIAN_POINT('Ctrl Pts',(-18.589871621843,-12.769110348199,12.));
#197372=CARTESIAN_POINT('Ctrl Pts',(-18.5903328777227,-12.7694215127919,
0.));
#197373=CARTESIAN_POINT('Ctrl Pts',(-18.5903328777227,-12.7694215127919,
12.));
#197374=CARTESIAN_POINT('Ctrl Pts',(-18.5912775137806,-12.7700520897173,
0.));
#197375=CARTESIAN_POINT('Ctrl Pts',(-18.5912775137806,-12.7700520897173,
12.));
#197376=CARTESIAN_POINT('Ctrl Pts',(-18.5925859134579,-12.7709195951156,
0.));
#197377=CARTESIAN_POINT('Ctrl Pts',(-18.5925859134579,-12.7709195951156,
12.));
#197378=CARTESIAN_POINT('Ctrl Pts',(-18.5942490615407,-12.7720142287172,
0.));
#197379=CARTESIAN_POINT('Ctrl Pts',(-18.5942490615407,-12.7720142287172,
12.));
#197380=CARTESIAN_POINT('Ctrl Pts',(-18.5962551167772,-12.7733231262108,
0.));
#197381=CARTESIAN_POINT('Ctrl Pts',(-18.5962551167772,-12.7733231262108,
12.));
#197382=CARTESIAN_POINT('Ctrl Pts',(-18.598591752595,-12.7748328937638,
0.));
#197383=CARTESIAN_POINT('Ctrl Pts',(-18.598591752595,-12.7748328937638,
12.));
#197384=CARTESIAN_POINT('Ctrl Pts',(-18.6012488486709,-12.7765325225081,
0.));
#197385=CARTESIAN_POINT('Ctrl Pts',(-18.6012488486709,-12.7765325225081,
12.));
#197386=CARTESIAN_POINT('Ctrl Pts',(-18.6042190183704,-12.7784139605066,
0.));
#197387=CARTESIAN_POINT('Ctrl Pts',(-18.6042190183704,-12.7784139605066,
12.));
#197388=CARTESIAN_POINT('Ctrl Pts',(-18.6074961535723,-12.7804705387658,
0.));
#197389=CARTESIAN_POINT('Ctrl Pts',(-18.6074961535723,-12.7804705387658,
12.));
#197390=CARTESIAN_POINT('Ctrl Pts',(-18.6110744826219,-12.7826959526925,
0.));
#197391=CARTESIAN_POINT('Ctrl Pts',(-18.6110744826219,-12.7826959526925,
12.));
#197392=CARTESIAN_POINT('Ctrl Pts',(-18.6149475565188,-12.7850831657901,
0.));
#197393=CARTESIAN_POINT('Ctrl Pts',(-18.6149475565188,-12.7850831657901,
12.));
#197394=CARTESIAN_POINT('Ctrl Pts',(-18.6191087624752,-12.7876249657834,
0.));
#197395=CARTESIAN_POINT('Ctrl Pts',(-18.6191087624752,-12.7876249657834,
12.));
#197396=CARTESIAN_POINT('Ctrl Pts',(-18.6235516265575,-12.7903142925234,
0.));
#197397=CARTESIAN_POINT('Ctrl Pts',(-18.6235516265575,-12.7903142925234,
12.));
#197398=CARTESIAN_POINT('Ctrl Pts',(-18.6282702819371,-12.7931447451555,
0.));
#197399=CARTESIAN_POINT('Ctrl Pts',(-18.6282702819371,-12.7931447451555,
12.));
#197400=CARTESIAN_POINT('Ctrl Pts',(-18.6332595057006,-12.7961106222251,
0.));
#197401=CARTESIAN_POINT('Ctrl Pts',(-18.6332595057006,-12.7961106222251,
12.));
#197402=CARTESIAN_POINT('Ctrl Pts',(-18.63851447924,-12.7992066625264,0.));
#197403=CARTESIAN_POINT('Ctrl Pts',(-18.63851447924,-12.7992066625264,12.));
#197404=CARTESIAN_POINT('Ctrl Pts',(-18.6440306327456,-12.8024278770152,
0.));
#197405=CARTESIAN_POINT('Ctrl Pts',(-18.6440306327456,-12.8024278770152,
12.));
#197406=CARTESIAN_POINT('Ctrl Pts',(-18.6498034438987,-12.805769331162,
0.));
#197407=CARTESIAN_POINT('Ctrl Pts',(-18.6498034438987,-12.805769331162,
12.));
#197408=CARTESIAN_POINT('Ctrl Pts',(-18.6558284825773,-12.8092261933858,
0.));
#197409=CARTESIAN_POINT('Ctrl Pts',(-18.6558284825773,-12.8092261933858,
12.));
#197410=CARTESIAN_POINT('Ctrl Pts',(-18.6621014624746,-12.8127937909631,
0.));
#197411=CARTESIAN_POINT('Ctrl Pts',(-18.6621014624746,-12.8127937909631,
12.));
#197412=CARTESIAN_POINT('Ctrl Pts',(-18.6686182952799,-12.8164676687362,
0.));
#197413=CARTESIAN_POINT('Ctrl Pts',(-18.6686182952799,-12.8164676687362,
12.));
#197414=CARTESIAN_POINT('Ctrl Pts',(-18.6753751301092,-12.8202436318474,
0.));
#197415=CARTESIAN_POINT('Ctrl Pts',(-18.6753751301092,-12.8202436318474,
12.));
#197416=CARTESIAN_POINT('Ctrl Pts',(-18.6823683094139,-12.8241176980017,
0.));
#197417=CARTESIAN_POINT('Ctrl Pts',(-18.6823683094139,-12.8241176980017,
12.));
#197418=CARTESIAN_POINT('Ctrl Pts',(-18.6895943376171,-12.8280860635231,
0.));
#197419=CARTESIAN_POINT('Ctrl Pts',(-18.6895943376171,-12.8280860635231,
12.));
#197420=CARTESIAN_POINT('Ctrl Pts',(-18.6970498410172,-12.8321450599789,
0.));
#197421=CARTESIAN_POINT('Ctrl Pts',(-18.6970498410172,-12.8321450599789,
12.));
#197422=CARTESIAN_POINT('Ctrl Pts',(-18.7047315436294,-12.8362911280361,
0.));
#197423=CARTESIAN_POINT('Ctrl Pts',(-18.7047315436294,-12.8362911280361,
12.));
#197424=CARTESIAN_POINT('Ctrl Pts',(-18.7126362754445,-12.8405208263431,
0.));
#197425=CARTESIAN_POINT('Ctrl Pts',(-18.7126362754445,-12.8405208263431,
12.));
#197426=CARTESIAN_POINT('Ctrl Pts',(-18.7207609737702,-12.8448308329494,
0.));
#197427=CARTESIAN_POINT('Ctrl Pts',(-18.7207609737702,-12.8448308329494,
12.));
#197428=CARTESIAN_POINT('Ctrl Pts',(-18.7291026886554,-12.8492179511591,
0.));
#197429=CARTESIAN_POINT('Ctrl Pts',(-18.7291026886554,-12.8492179511591,
12.));
#197430=CARTESIAN_POINT('Ctrl Pts',(-18.7376585820854,-12.8536791086316,
0.));
#197431=CARTESIAN_POINT('Ctrl Pts',(-18.7376585820854,-12.8536791086316,
12.));
#197432=CARTESIAN_POINT('Ctrl Pts',(-18.7464259171251,-12.8582113455646,
0.));
#197433=CARTESIAN_POINT('Ctrl Pts',(-18.7464259171251,-12.8582113455646,
12.));
#197434=CARTESIAN_POINT('Ctrl Pts',(-18.7554020493887,-12.8628118054171,
0.));
#197435=CARTESIAN_POINT('Ctrl Pts',(-18.7554020493887,-12.8628118054171,
12.));
#197436=CARTESIAN_POINT('Ctrl Pts',(-18.7645844169564,-12.8674777239653,
0.));
#197437=CARTESIAN_POINT('Ctrl Pts',(-18.7645844169564,-12.8674777239653,
12.));
#197438=CARTESIAN_POINT('Ctrl Pts',(-18.7739705329022,-12.872206421181,
0.));
#197439=CARTESIAN_POINT('Ctrl Pts',(-18.7739705329022,-12.872206421181,
12.));
#197440=CARTESIAN_POINT('Ctrl Pts',(-18.7835579840477,-12.8769952998095,
0.));
#197441=CARTESIAN_POINT('Ctrl Pts',(-18.7835579840477,-12.8769952998095,
12.));
#197442=CARTESIAN_POINT('Ctrl Pts',(-18.7933444285868,-12.8818418427475,
0.));
#197443=CARTESIAN_POINT('Ctrl Pts',(-18.7933444285868,-12.8818418427475,
12.));
#197444=CARTESIAN_POINT('Ctrl Pts',(-18.8033275941943,-12.8867436109546,
0.));
#197445=CARTESIAN_POINT('Ctrl Pts',(-18.8033275941943,-12.8867436109546,
12.));
#197446=CARTESIAN_POINT('Ctrl Pts',(-18.813505275782,-12.8916982409935,
0.));
#197447=CARTESIAN_POINT('Ctrl Pts',(-18.813505275782,-12.8916982409935,
12.));
#197448=CARTESIAN_POINT('Ctrl Pts',(-18.8238753319129,-12.8967034410755,
0.));
#197449=CARTESIAN_POINT('Ctrl Pts',(-18.8238753319129,-12.8967034410755,
12.));
#197450=CARTESIAN_POINT('Ctrl Pts',(-18.834435681259,-12.9017569871738,
0.));
#197451=CARTESIAN_POINT('Ctrl Pts',(-18.834435681259,-12.9017569871738,
12.));
#197452=CARTESIAN_POINT('Ctrl Pts',(-18.8451842990984,-12.9068567191854,
0.));
#197453=CARTESIAN_POINT('Ctrl Pts',(-18.8451842990984,-12.9068567191854,
12.));
#197454=CARTESIAN_POINT('Ctrl Pts',(-18.8561192136198,-12.9120005369063,
0.));
#197455=CARTESIAN_POINT('Ctrl Pts',(-18.8561192136198,-12.9120005369063,
12.));
#197456=CARTESIAN_POINT('Ctrl Pts',(-18.8672385038326,-12.9171863977045,
0.));
#197457=CARTESIAN_POINT('Ctrl Pts',(-18.8672385038326,-12.9171863977045,
12.));
#197458=CARTESIAN_POINT('Ctrl Pts',(-18.8785402977527,-12.9224123144982,
0.));
#197459=CARTESIAN_POINT('Ctrl Pts',(-18.8785402977527,-12.9224123144982,
12.));
#197460=CARTESIAN_POINT('Ctrl Pts',(-18.8900227704889,-12.9276763536373,
0.));
#197461=CARTESIAN_POINT('Ctrl Pts',(-18.8900227704889,-12.9276763536373,
12.));
#197462=CARTESIAN_POINT('Ctrl Pts',(-18.9016841423403,-12.9329766328185,
0.));
#197463=CARTESIAN_POINT('Ctrl Pts',(-18.9016841423403,-12.9329766328185,
12.));
#197464=CARTESIAN_POINT('Ctrl Pts',(-18.9135226769465,-12.9383113190375,
0.));
#197465=CARTESIAN_POINT('Ctrl Pts',(-18.9135226769465,-12.9383113190375,
12.));
#197466=CARTESIAN_POINT('Ctrl Pts',(-18.9255366795195,-12.9436786266105,
0.));
#197467=CARTESIAN_POINT('Ctrl Pts',(-18.9255366795195,-12.9436786266105,
12.));
#197468=CARTESIAN_POINT('Ctrl Pts',(-18.9377244950435,-12.9490768151821,
0.));
#197469=CARTESIAN_POINT('Ctrl Pts',(-18.9377244950435,-12.9490768151821,
12.));
#197470=CARTESIAN_POINT('Ctrl Pts',(-18.9500845064715,-12.9545041877377,
0.));
#197471=CARTESIAN_POINT('Ctrl Pts',(-18.9500845064715,-12.9545041877377,
12.));
#197472=CARTESIAN_POINT('Ctrl Pts',(-18.9626151329229,-12.9599590886319,
0.));
#197473=CARTESIAN_POINT('Ctrl Pts',(-18.9626151329229,-12.9599590886319,
12.));
#197474=CARTESIAN_POINT('Ctrl Pts',(-18.9753148284475,-12.9654399021869,
0.));
#197475=CARTESIAN_POINT('Ctrl Pts',(-18.9753148284475,-12.9654399021869,
12.));
#197476=CARTESIAN_POINT('Ctrl Pts',(-18.9881820807586,-12.9709450512747,
0.));
#197477=CARTESIAN_POINT('Ctrl Pts',(-18.9881820807586,-12.9709450512747,
12.));
#197478=CARTESIAN_POINT('Ctrl Pts',(-19.0012154099791,-12.9764729959205,
0.));
#197479=CARTESIAN_POINT('Ctrl Pts',(-19.0012154099791,-12.9764729959205,
12.));
#197480=CARTESIAN_POINT('Ctrl Pts',(-19.0144133673348,-12.9820222318716,
0.));
#197481=CARTESIAN_POINT('Ctrl Pts',(-19.0144133673348,-12.9820222318716,
12.));
#197482=CARTESIAN_POINT('Ctrl Pts',(-19.0277745339908,-12.9875912893003,
0.));
#197483=CARTESIAN_POINT('Ctrl Pts',(-19.0277745339908,-12.9875912893003,
12.));
#197484=CARTESIAN_POINT('Ctrl Pts',(-19.0412975200398,-12.9931787316515,
0.));
#197485=CARTESIAN_POINT('Ctrl Pts',(-19.0412975200398,-12.9931787316515,
12.));
#197486=CARTESIAN_POINT('Ctrl Pts',(-19.0549809634355,-12.9987831544502,
0.));
#197487=CARTESIAN_POINT('Ctrl Pts',(-19.0549809634355,-12.9987831544502,
12.));
#197488=CARTESIAN_POINT('Ctrl Pts',(-19.0688235289437,-13.0044031841381,
0.));
#197489=CARTESIAN_POINT('Ctrl Pts',(-19.0688235289437,-13.0044031841381,
12.));
#197490=CARTESIAN_POINT('Ctrl Pts',(-19.0828239070482,-13.0100374768785,
0.));
#197491=CARTESIAN_POINT('Ctrl Pts',(-19.0828239070482,-13.0100374768785,
12.));
#197492=CARTESIAN_POINT('Ctrl Pts',(-19.0969808131226,-13.0156847176093,
0.));
#197493=CARTESIAN_POINT('Ctrl Pts',(-19.0969808131226,-13.0156847176093,
12.));
#197494=CARTESIAN_POINT('Ctrl Pts',(-19.1112929866308,-13.0213436191326,
0.));
#197495=CARTESIAN_POINT('Ctrl Pts',(-19.1112929866308,-13.0213436191326,
12.));
#197496=CARTESIAN_POINT('Ctrl Pts',(-19.1257591903099,-13.0270129211976,
0.));
#197497=CARTESIAN_POINT('Ctrl Pts',(-19.1257591903099,-13.0270129211976,
12.));
#197498=CARTESIAN_POINT('Ctrl Pts',(-19.1403782093389,-13.0326913895841,
0.));
#197499=CARTESIAN_POINT('Ctrl Pts',(-19.1403782093389,-13.0326913895841,
12.));
#197500=CARTESIAN_POINT('Ctrl Pts',(-19.1551488505233,-13.0383778152072,
0.));
#197501=CARTESIAN_POINT('Ctrl Pts',(-19.1551488505233,-13.0383778152072,
12.));
#197502=CARTESIAN_POINT('Ctrl Pts',(-19.1700699416625,-13.0440710133775,
0.));
#197503=CARTESIAN_POINT('Ctrl Pts',(-19.1700699416625,-13.0440710133775,
12.));
#197504=CARTESIAN_POINT('Ctrl Pts',(-19.1851403308825,-13.0497698230442,
0.));
#197505=CARTESIAN_POINT('Ctrl Pts',(-19.1851403308825,-13.0497698230442,
12.));
#197506=CARTESIAN_POINT('Ctrl Pts',(-19.2003588859771,-13.0554731060537,
0.));
#197507=CARTESIAN_POINT('Ctrl Pts',(-19.2003588859771,-13.0554731060537,
12.));
#197508=CARTESIAN_POINT('Ctrl Pts',(-19.2157244937141,-13.0611797463913,
0.));
#197509=CARTESIAN_POINT('Ctrl Pts',(-19.2157244937141,-13.0611797463913,
12.));
#197510=CARTESIAN_POINT('Ctrl Pts',(-19.2312360592031,-13.0668886494791,
0.));
#197511=CARTESIAN_POINT('Ctrl Pts',(-19.2312360592031,-13.0668886494791,
12.));
#197512=CARTESIAN_POINT('Ctrl Pts',(-19.2468925053988,-13.0725987415856,
0.));
#197513=CARTESIAN_POINT('Ctrl Pts',(-19.2468925053988,-13.0725987415856,
12.));
#197514=CARTESIAN_POINT('Ctrl Pts',(-19.2626927725596,-13.0783089692118,
0.));
#197515=CARTESIAN_POINT('Ctrl Pts',(-19.2626927725596,-13.0783089692118,
12.));
#197516=CARTESIAN_POINT('Ctrl Pts',(-19.2786358177198,-13.0840182984949,
0.));
#197517=CARTESIAN_POINT('Ctrl Pts',(-19.2786358177198,-13.0840182984949,
12.));
#197518=CARTESIAN_POINT('Ctrl Pts',(-19.2947206141246,-13.0897257145969,
0.));
#197519=CARTESIAN_POINT('Ctrl Pts',(-19.2947206141246,-13.0897257145969,
12.));
#197520=CARTESIAN_POINT('Ctrl Pts',(-19.3109461507358,-13.095430221148,
0.));
#197521=CARTESIAN_POINT('Ctrl Pts',(-19.3109461507358,-13.095430221148,
12.));
#197522=CARTESIAN_POINT('Ctrl Pts',(-19.3273114318268,-13.1011308397592,
0.));
#197523=CARTESIAN_POINT('Ctrl Pts',(-19.3273114318268,-13.1011308397592,
12.));
#197524=CARTESIAN_POINT('Ctrl Pts',(-19.3438154765395,-13.1068266095186,
0.));
#197525=CARTESIAN_POINT('Ctrl Pts',(-19.3438154765395,-13.1068266095186,
12.));
#197526=CARTESIAN_POINT('Ctrl Pts',(-19.3604573184516,-13.1125165865021,
0.));
#197527=CARTESIAN_POINT('Ctrl Pts',(-19.3604573184516,-13.1125165865021,
12.));
#197528=CARTESIAN_POINT('Ctrl Pts',(-19.3772360051093,-13.118199843271,
0.));
#197529=CARTESIAN_POINT('Ctrl Pts',(-19.3772360051093,-13.118199843271,
12.));
#197530=CARTESIAN_POINT('Ctrl Pts',(-19.3941505976267,-13.1238754684177,
0.));
#197531=CARTESIAN_POINT('Ctrl Pts',(-19.3941505976267,-13.1238754684177,
12.));
#197532=CARTESIAN_POINT('Ctrl Pts',(-19.4112001703561,-13.1295425661635,
0.));
#197533=CARTESIAN_POINT('Ctrl Pts',(-19.4112001703561,-13.1295425661635,
12.));
#197534=CARTESIAN_POINT('Ctrl Pts',(-19.4283838105265,-13.1352002559439,
0.));
#197535=CARTESIAN_POINT('Ctrl Pts',(-19.4283838105265,-13.1352002559439,
12.));
#197536=CARTESIAN_POINT('Ctrl Pts',(-19.4457006178875,-13.140847672006,
0.));
#197537=CARTESIAN_POINT('Ctrl Pts',(-19.4457006178875,-13.140847672006,
12.));
#197538=CARTESIAN_POINT('Ctrl Pts',(-19.463149704325,-13.1464839629966,
0.));
#197539=CARTESIAN_POINT('Ctrl Pts',(-19.463149704325,-13.1464839629966,
12.));
#197540=CARTESIAN_POINT('Ctrl Pts',(-19.4807301935256,-13.1521082915846,
0.));
#197541=CARTESIAN_POINT('Ctrl Pts',(-19.4807301935256,-13.1521082915846,
12.));
#197542=CARTESIAN_POINT('Ctrl Pts',(-19.498441220707,-13.1577198341238,
0.));
#197543=CARTESIAN_POINT('Ctrl Pts',(-19.498441220707,-13.1577198341238,
12.));
#197544=CARTESIAN_POINT('Ctrl Pts',(-19.5162819323207,-13.1633177803097,
0.));
#197545=CARTESIAN_POINT('Ctrl Pts',(-19.5162819323207,-13.1633177803097,
12.));
#197546=CARTESIAN_POINT('Ctrl Pts',(-19.5342514857564,-13.1689013328432,
0.));
#197547=CARTESIAN_POINT('Ctrl Pts',(-19.5342514857564,-13.1689013328432,
12.));
#197548=CARTESIAN_POINT('Ctrl Pts',(-19.5523490490254,-13.1744697070918,
0.));
#197549=CARTESIAN_POINT('Ctrl Pts',(-19.5523490490254,-13.1744697070918,
12.));
#197550=CARTESIAN_POINT('Ctrl Pts',(-19.5705738004682,-13.1800221307682,
0.));
#197551=CARTESIAN_POINT('Ctrl Pts',(-19.5705738004682,-13.1800221307682,
12.));
#197552=CARTESIAN_POINT('Ctrl Pts',(-19.5889249285352,-13.1855578436479,
0.));
#197553=CARTESIAN_POINT('Ctrl Pts',(-19.5889249285352,-13.1855578436479,
12.));
#197554=CARTESIAN_POINT('Ctrl Pts',(-19.6074016315421,-13.1910760972818,
0.));
#197555=CARTESIAN_POINT('Ctrl Pts',(-19.6074016315421,-13.1910760972818,
12.));
#197556=CARTESIAN_POINT('Ctrl Pts',(-19.6260031174244,-13.196576154715,
0.));
#197557=CARTESIAN_POINT('Ctrl Pts',(-19.6260031174244,-13.196576154715,
12.));
#197558=CARTESIAN_POINT('Ctrl Pts',(-19.6447286034764,-13.202057290206,
0.));
#197559=CARTESIAN_POINT('Ctrl Pts',(-19.6447286034764,-13.202057290206,
12.));
#197560=CARTESIAN_POINT('Ctrl Pts',(-19.6635773160924,-13.2075187889522,
0.));
#197561=CARTESIAN_POINT('Ctrl Pts',(-19.6635773160924,-13.2075187889522,
12.));
#197562=CARTESIAN_POINT('Ctrl Pts',(-19.6825484905812,-13.2129599468478,
0.));
#197563=CARTESIAN_POINT('Ctrl Pts',(-19.6825484905812,-13.2129599468478,
12.));
#197564=CARTESIAN_POINT('Ctrl Pts',(-19.7016413709678,-13.2183800702431,
0.));
#197565=CARTESIAN_POINT('Ctrl Pts',(-19.7016413709678,-13.2183800702431,
12.));
#197566=CARTESIAN_POINT('Ctrl Pts',(-19.7208552097867,-13.2237784757065,
0.));
#197567=CARTESIAN_POINT('Ctrl Pts',(-19.7208552097867,-13.2237784757065,
12.));
#197568=CARTESIAN_POINT('Ctrl Pts',(-19.7401892678701,-13.2291544897902,
0.));
#197569=CARTESIAN_POINT('Ctrl Pts',(-19.7401892678701,-13.2291544897902,
12.));
#197570=CARTESIAN_POINT('Ctrl Pts',(-19.7596428141176,-13.2345074487968,
0.));
#197571=CARTESIAN_POINT('Ctrl Pts',(-19.7596428141176,-13.2345074487968,
12.));
#197572=CARTESIAN_POINT('Ctrl Pts',(-19.7792151253297,-13.239836698568,
0.));
#197573=CARTESIAN_POINT('Ctrl Pts',(-19.7792151253297,-13.239836698568,
12.));
#197574=CARTESIAN_POINT('Ctrl Pts',(-19.7989054860501,-13.2451415942809,
0.));
#197575=CARTESIAN_POINT('Ctrl Pts',(-19.7989054860501,-13.2451415942809,
12.));
#197576=CARTESIAN_POINT('Ctrl Pts',(-19.8187131883919,-13.2504215002458,
0.));
#197577=CARTESIAN_POINT('Ctrl Pts',(-19.8187131883919,-13.2504215002458,
12.));
#197578=CARTESIAN_POINT('Ctrl Pts',(-19.8386375318632,-13.2556757897085,
0.));
#197579=CARTESIAN_POINT('Ctrl Pts',(-19.8386375318632,-13.2556757897085,
12.));
#197580=CARTESIAN_POINT('Ctrl Pts',(-19.8586778231711,-13.2609038446525,
0.));
#197581=CARTESIAN_POINT('Ctrl Pts',(-19.8586778231711,-13.2609038446525,
12.));
#197582=CARTESIAN_POINT('Ctrl Pts',(-19.8788333760571,-13.2661050556128,
0.));
#197583=CARTESIAN_POINT('Ctrl Pts',(-19.8788333760571,-13.2661050556128,
12.));
#197584=CARTESIAN_POINT('Ctrl Pts',(-19.8991035111739,-13.2712788215015,
0.));
#197585=CARTESIAN_POINT('Ctrl Pts',(-19.8991035111739,-13.2712788215015,
12.));
#197586=CARTESIAN_POINT('Ctrl Pts',(-19.9194875559419,-13.2764245494354,
0.));
#197587=CARTESIAN_POINT('Ctrl Pts',(-19.9194875559419,-13.2764245494354,
12.));
#197588=CARTESIAN_POINT('Ctrl Pts',(-19.9399848444019,-13.2815416545663,
0.));
#197589=CARTESIAN_POINT('Ctrl Pts',(-19.9399848444019,-13.2815416545663,
12.));
#197590=CARTESIAN_POINT('Ctrl Pts',(-19.9605947170589,-13.2866295599152,
0.));
#197591=CARTESIAN_POINT('Ctrl Pts',(-19.9605947170589,-13.2866295599152,
12.));
#197592=CARTESIAN_POINT('Ctrl Pts',(-19.9813165207174,-13.2916876962098,
0.));
#197593=CARTESIAN_POINT('Ctrl Pts',(-19.9813165207174,-13.2916876962098,
12.));
#197594=CARTESIAN_POINT('Ctrl Pts',(-20.0021496083742,-13.296715501731,
0.));
#197595=CARTESIAN_POINT('Ctrl Pts',(-20.0021496083742,-13.296715501731,
12.));
#197596=CARTESIAN_POINT('Ctrl Pts',(-20.023093339104,-13.3017124221639,
0.));
#197597=CARTESIAN_POINT('Ctrl Pts',(-20.023093339104,-13.3017124221639,
12.));
#197598=CARTESIAN_POINT('Ctrl Pts',(-20.0441470779345,-13.3066779104515,
0.));
#197599=CARTESIAN_POINT('Ctrl Pts',(-20.0441470779345,-13.3066779104515,
12.));
#197600=CARTESIAN_POINT('Ctrl Pts',(-20.0653101957188,-13.3116114266514,
0.));
#197601=CARTESIAN_POINT('Ctrl Pts',(-20.0653101957188,-13.3116114266514,
12.));
#197602=CARTESIAN_POINT('Ctrl Pts',(-20.0865820689883,-13.3165124377963,
0.));
#197603=CARTESIAN_POINT('Ctrl Pts',(-20.0865820689883,-13.3165124377963,
12.));
#197604=CARTESIAN_POINT('Ctrl Pts',(-20.1079620798377,-13.3213804177588,
0.));
#197605=CARTESIAN_POINT('Ctrl Pts',(-20.1079620798377,-13.3213804177588,
12.));
#197606=CARTESIAN_POINT('Ctrl Pts',(-20.1294496158405,-13.3262148471228,
0.));
#197607=CARTESIAN_POINT('Ctrl Pts',(-20.1294496158405,-13.3262148471228,
12.));
#197608=CARTESIAN_POINT('Ctrl Pts',(-20.1510440699477,-13.3310152130565,
0.));
#197609=CARTESIAN_POINT('Ctrl Pts',(-20.1510440699477,-13.3310152130565,
12.));
#197610=CARTESIAN_POINT('Ctrl Pts',(-20.1727448403818,-13.3357810091903,
0.));
#197611=CARTESIAN_POINT('Ctrl Pts',(-20.1727448403818,-13.3357810091903,
12.));
#197612=CARTESIAN_POINT('Ctrl Pts',(-20.1945513305233,-13.3405117354969,
0.));
#197613=CARTESIAN_POINT('Ctrl Pts',(-20.1945513305233,-13.3405117354969,
12.));
#197614=CARTESIAN_POINT('Ctrl Pts',(-20.2164629487855,-13.3452068981763,
0.));
#197615=CARTESIAN_POINT('Ctrl Pts',(-20.2164629487855,-13.3452068981763,
12.));
#197616=CARTESIAN_POINT('Ctrl Pts',(-20.2384791085354,-13.3498660095382,
0.));
#197617=CARTESIAN_POINT('Ctrl Pts',(-20.2384791085354,-13.3498660095382,
12.));
#197618=CARTESIAN_POINT('Ctrl Pts',(-20.2605992280117,-13.3544885878886,
0.));
#197619=CARTESIAN_POINT('Ctrl Pts',(-20.2605992280117,-13.3544885878886,
12.));
#197620=CARTESIAN_POINT('Ctrl Pts',(-20.2828227302337,-13.3590741574194,
0.));
#197621=CARTESIAN_POINT('Ctrl Pts',(-20.2828227302337,-13.3590741574194,
12.));
#197622=CARTESIAN_POINT('Ctrl Pts',(-20.3051490429049,-13.3636222481017,
0.));
#197623=CARTESIAN_POINT('Ctrl Pts',(-20.3051490429049,-13.3636222481017,
12.));
#197624=CARTESIAN_POINT('Ctrl Pts',(-20.3275775983032,-13.3681323955828,
0.));
#197625=CARTESIAN_POINT('Ctrl Pts',(-20.3275775983032,-13.3681323955828,
12.));
#197626=CARTESIAN_POINT('Ctrl Pts',(-20.3501078331818,-13.3726041410869,
0.));
#197627=CARTESIAN_POINT('Ctrl Pts',(-20.3501078331818,-13.3726041410869,
12.));
#197628=CARTESIAN_POINT('Ctrl Pts',(-20.3727391887187,-13.377037031319,
0.));
#197629=CARTESIAN_POINT('Ctrl Pts',(-20.3727391887187,-13.377037031319,
12.));
#197630=CARTESIAN_POINT('Ctrl Pts',(-20.3954711104505,-13.3814306183721,
0.));
#197631=CARTESIAN_POINT('Ctrl Pts',(-20.3954711104505,-13.3814306183721,
12.));
#197632=CARTESIAN_POINT('Ctrl Pts',(-20.4183030482002,-13.3857844596387,
0.));
#197633=CARTESIAN_POINT('Ctrl Pts',(-20.4183030482002,-13.3857844596387,
12.));
#197634=CARTESIAN_POINT('Ctrl Pts',(-20.4412344560007,-13.3900981177254,
0.));
#197635=CARTESIAN_POINT('Ctrl Pts',(-20.4412344560007,-13.3900981177254,
12.));
#197636=CARTESIAN_POINT('Ctrl Pts',(-20.4642647920038,-13.3943711603739,
0.));
#197637=CARTESIAN_POINT('Ctrl Pts',(-20.4642647920038,-13.3943711603739,
12.));
#197638=CARTESIAN_POINT('Ctrl Pts',(-20.4873935184041,-13.3986031603716,
0.));
#197639=CARTESIAN_POINT('Ctrl Pts',(-20.4873935184041,-13.3986031603716,
12.));
#197640=CARTESIAN_POINT('Ctrl Pts',(-20.5106201013755,-13.4027936954529,
0.));
#197641=CARTESIAN_POINT('Ctrl Pts',(-20.5106201013755,-13.4027936954529,
12.));
#197642=CARTESIAN_POINT('Ctrl Pts',(-20.5339440109958,-13.4069423482076,
0.));
#197643=CARTESIAN_POINT('Ctrl Pts',(-20.5339440109958,-13.4069423482076,
12.));
#197644=CARTESIAN_POINT('Ctrl Pts',(-20.557364721164,-13.4110487059912,
0.));
#197645=CARTESIAN_POINT('Ctrl Pts',(-20.557364721164,-13.4110487059912,
12.));
#197646=CARTESIAN_POINT('Ctrl Pts',(-20.5808817095155,-13.4151123608411,
0.));
#197647=CARTESIAN_POINT('Ctrl Pts',(-20.5808817095155,-13.4151123608411,
12.));
#197648=CARTESIAN_POINT('Ctrl Pts',(-20.6044944573151,-13.4191329093932,
0.));
#197649=CARTESIAN_POINT('Ctrl Pts',(-20.6044944573151,-13.4191329093932,
12.));
#197650=CARTESIAN_POINT('Ctrl Pts',(-20.6282024494234,-13.4231099528178,
0.));
#197651=CARTESIAN_POINT('Ctrl Pts',(-20.6282024494234,-13.4231099528178,
12.));
#197652=CARTESIAN_POINT('Ctrl Pts',(-20.6520051742868,-13.427043096765,
0.));
#197653=CARTESIAN_POINT('Ctrl Pts',(-20.6520051742868,-13.427043096765,
12.));
#197654=CARTESIAN_POINT('Ctrl Pts',(-20.6759021239102,-13.4309319513119,
0.));
#197655=CARTESIAN_POINT('Ctrl Pts',(-20.6759021239102,-13.4309319513119,
12.));
#197656=CARTESIAN_POINT('Ctrl Pts',(-20.6998927938288,-13.4347761309154,
0.));
#197657=CARTESIAN_POINT('Ctrl Pts',(-20.6998927938288,-13.4347761309154,
12.));
#197658=CARTESIAN_POINT('Ctrl Pts',(-20.7239766830675,-13.4385752543663,
0.));
#197659=CARTESIAN_POINT('Ctrl Pts',(-20.7239766830675,-13.4385752543663,
12.));
#197660=CARTESIAN_POINT('Ctrl Pts',(-20.7481532941014,-13.4423289447561,
0.));
#197661=CARTESIAN_POINT('Ctrl Pts',(-20.7481532941014,-13.4423289447561,
12.));
#197662=CARTESIAN_POINT('Ctrl Pts',(-20.7724221327609,-13.4460368293689,
0.));
#197663=CARTESIAN_POINT('Ctrl Pts',(-20.7724221327609,-13.4460368293689,
12.));
#197664=CARTESIAN_POINT('Ctrl Pts',(-20.7967827081228,-13.4496985395637,
0.));
#197665=CARTESIAN_POINT('Ctrl Pts',(-20.7967827081228,-13.4496985395637,
12.));
#197666=CARTESIAN_POINT('Ctrl Pts',(-20.821234532398,-13.4533137106667,
0.));
#197667=CARTESIAN_POINT('Ctrl Pts',(-20.821234532398,-13.4533137106667,
12.));
#197668=CARTESIAN_POINT('Ctrl Pts',(-20.8457771208083,-13.4568819818631,
0.));
#197669=CARTESIAN_POINT('Ctrl Pts',(-20.8457771208083,-13.4568819818631,
12.));
#197670=CARTESIAN_POINT('Ctrl Pts',(-20.8704099914641,-13.4604029960983,
0.));
#197671=CARTESIAN_POINT('Ctrl Pts',(-20.8704099914641,-13.4604029960983,
12.));
#197672=CARTESIAN_POINT('Ctrl Pts',(-20.8951326652158,-13.4638763999725,
0.));
#197673=CARTESIAN_POINT('Ctrl Pts',(-20.8951326652158,-13.4638763999725,
12.));
#197674=CARTESIAN_POINT('Ctrl Pts',(-20.9199446657583,-13.4673018437717,
0.));
#197675=CARTESIAN_POINT('Ctrl Pts',(-20.9199446657583,-13.4673018437717,
12.));
#197676=CARTESIAN_POINT('Ctrl Pts',(-20.9448455197557,-13.4706789815166,
0.));
#197677=CARTESIAN_POINT('Ctrl Pts',(-20.9448455197557,-13.4706789815166,
12.));
#197678=CARTESIAN_POINT('Ctrl Pts',(-20.9698347569477,-13.4740074710086,
0.));
#197679=CARTESIAN_POINT('Ctrl Pts',(-20.9698347569477,-13.4740074710086,
12.));
#197680=CARTESIAN_POINT('Ctrl Pts',(-20.9949119102592,-13.4772869738879,
0.));
#197681=CARTESIAN_POINT('Ctrl Pts',(-20.9949119102592,-13.4772869738879,
12.));
#197682=CARTESIAN_POINT('Ctrl Pts',(-21.0200765158884,-13.4805171556822,
0.));
#197683=CARTESIAN_POINT('Ctrl Pts',(-21.0200765158884,-13.4805171556822,
12.));
#197684=CARTESIAN_POINT('Ctrl Pts',(-21.0453281134245,-13.4836976858912,
0.));
#197685=CARTESIAN_POINT('Ctrl Pts',(-21.0453281134245,-13.4836976858912,
12.));
#197686=CARTESIAN_POINT('Ctrl Pts',(-21.0706662455199,-13.4868282377191,
0.));
#197687=CARTESIAN_POINT('Ctrl Pts',(-21.0706662455199,-13.4868282377191,
12.));
#197688=CARTESIAN_POINT('Ctrl Pts',(-21.0960904575046,-13.4899084877717,
0.));
#197689=CARTESIAN_POINT('Ctrl Pts',(-21.0960904575046,-13.4899084877717,
12.));
#197690=CARTESIAN_POINT('Ctrl Pts',(-21.1216002970207,-13.4929381157778,
0.));
#197691=CARTESIAN_POINT('Ctrl Pts',(-21.1216002970207,-13.4929381157778,
12.));
#197692=CARTESIAN_POINT('Ctrl Pts',(-21.1471953136209,-13.4959168042934,
0.));
#197693=CARTESIAN_POINT('Ctrl Pts',(-21.1471953136209,-13.4959168042934,
12.));
#197694=CARTESIAN_POINT('Ctrl Pts',(-21.1728750584175,-13.4988442384491,
0.));
#197695=CARTESIAN_POINT('Ctrl Pts',(-21.1728750584175,-13.4988442384491,
12.));
#197696=CARTESIAN_POINT('Ctrl Pts',(-21.1986390835828,-13.5017201056088,
0.));
#197697=CARTESIAN_POINT('Ctrl Pts',(-21.1986390835828,-13.5017201056088,
12.));
#197698=CARTESIAN_POINT('Ctrl Pts',(-21.2244869429332,-13.5045440957404,
0.));
#197699=CARTESIAN_POINT('Ctrl Pts',(-21.2244869429332,-13.5045440957404,
12.));
#197700=CARTESIAN_POINT('Ctrl Pts',(-21.250418192743,-13.5073159019452,
0.));
#197701=CARTESIAN_POINT('Ctrl Pts',(-21.250418192743,-13.5073159019452,
12.));
#197702=CARTESIAN_POINT('Ctrl Pts',(-21.2764323924442,-13.5100352209205,
0.));
#197703=CARTESIAN_POINT('Ctrl Pts',(-21.2764323924442,-13.5100352209205,
12.));
#197704=CARTESIAN_POINT('Ctrl Pts',(-21.3025291054235,-13.5127017534971,
0.));
#197705=CARTESIAN_POINT('Ctrl Pts',(-21.3025291054235,-13.5127017534971,
12.));
#197706=CARTESIAN_POINT('Ctrl Pts',(-21.3287078996341,-13.5153152050555,
0.));
#197707=CARTESIAN_POINT('Ctrl Pts',(-21.3287078996341,-13.5153152050555,
12.));
#197708=CARTESIAN_POINT('Ctrl Pts',(-21.3549683486222,-13.5178752862466,
0.));
#197709=CARTESIAN_POINT('Ctrl Pts',(-21.3549683486222,-13.5178752862466,
12.));
#197710=CARTESIAN_POINT('Ctrl Pts',(-21.3813100304973,-13.5203817122504,
0.));
#197711=CARTESIAN_POINT('Ctrl Pts',(-21.3813100304973,-13.5203817122504,
12.));
#197712=CARTESIAN_POINT('Ctrl Pts',(-21.4077325259324,-13.5228342013516,
0.));
#197713=CARTESIAN_POINT('Ctrl Pts',(-21.4077325259324,-13.5228342013516,
12.));
#197714=CARTESIAN_POINT('Ctrl Pts',(-21.4342354165259,-13.5252324737802,
0.));
#197715=CARTESIAN_POINT('Ctrl Pts',(-21.4342354165259,-13.5252324737802,
12.));
#197716=CARTESIAN_POINT('Ctrl Pts',(-21.4608182828697,-13.5275762503555,
0.));
#197717=CARTESIAN_POINT('Ctrl Pts',(-21.4608182828697,-13.5275762503555,
12.));
#197718=CARTESIAN_POINT('Ctrl Pts',(-21.4874807030468,-13.5298652514355,
0.));
#197719=CARTESIAN_POINT('Ctrl Pts',(-21.4874807030468,-13.5298652514355,
12.));
#197720=CARTESIAN_POINT('Ctrl Pts',(-21.5142222501666,-13.5320991952138,
0.));
#197721=CARTESIAN_POINT('Ctrl Pts',(-21.5142222501666,-13.5320991952138,
12.));
#197722=CARTESIAN_POINT('Ctrl Pts',(-21.5410424932503,-13.5342777983215,
0.));
#197723=CARTESIAN_POINT('Ctrl Pts',(-21.5410424932503,-13.5342777983215,
12.));
#197724=CARTESIAN_POINT('Ctrl Pts',(-21.5679410019001,-13.536400779028,
0.));
#197725=CARTESIAN_POINT('Ctrl Pts',(-21.5679410019001,-13.536400779028,
12.));
#197726=CARTESIAN_POINT('Ctrl Pts',(-21.5949173499013,-13.5384678597195,
0.));
#197727=CARTESIAN_POINT('Ctrl Pts',(-21.5949173499013,-13.5384678597195,
12.));
#197728=CARTESIAN_POINT('Ctrl Pts',(-21.6219711193946,-13.5404787697792,
0.));
#197729=CARTESIAN_POINT('Ctrl Pts',(-21.6219711193946,-13.5404787697792,
12.));
#197730=CARTESIAN_POINT('Ctrl Pts',(-21.6491019044648,-13.5424332480699,
0.));
#197731=CARTESIAN_POINT('Ctrl Pts',(-21.6491019044648,-13.5424332480699,
12.));
#197732=CARTESIAN_POINT('Ctrl Pts',(-21.6763093157699,-13.5443310461526,
0.));
#197733=CARTESIAN_POINT('Ctrl Pts',(-21.6763093157699,-13.5443310461526,
12.));
#197734=CARTESIAN_POINT('Ctrl Pts',(-21.7035929822955,-13.5461719295048,
0.));
#197735=CARTESIAN_POINT('Ctrl Pts',(-21.7035929822955,-13.5461719295048,
12.));
#197736=CARTESIAN_POINT('Ctrl Pts',(-21.7309525412281,-13.5479556704481,
0.));
#197737=CARTESIAN_POINT('Ctrl Pts',(-21.7309525412281,-13.5479556704481,
12.));
#197738=CARTESIAN_POINT('Ctrl Pts',(-21.7583876294554,-13.5496820422211,
0.));
#197739=CARTESIAN_POINT('Ctrl Pts',(-21.7583876294554,-13.5496820422211,
12.));
#197740=CARTESIAN_POINT('Ctrl Pts',(-21.7858978745865,-13.551350812725,
0.));
#197741=CARTESIAN_POINT('Ctrl Pts',(-21.7858978745865,-13.551350812725,
12.));
#197742=CARTESIAN_POINT('Ctrl Pts',(-21.8134828857967,-13.5529617381573,
0.));
#197743=CARTESIAN_POINT('Ctrl Pts',(-21.8134828857967,-13.5529617381573,
12.));
#197744=CARTESIAN_POINT('Ctrl Pts',(-21.8411422456075,-13.5545145573031,
0.));
#197745=CARTESIAN_POINT('Ctrl Pts',(-21.8411422456075,-13.5545145573031,
12.));
#197746=CARTESIAN_POINT('Ctrl Pts',(-21.8688754989365,-13.5560089839385,
0.));
#197747=CARTESIAN_POINT('Ctrl Pts',(-21.8688754989365,-13.5560089839385,
12.));
#197748=CARTESIAN_POINT('Ctrl Pts',(-21.8966821688824,-13.5574447178424,
0.));
#197749=CARTESIAN_POINT('Ctrl Pts',(-21.8966821688824,-13.5574447178424,
12.));
#197750=CARTESIAN_POINT('Ctrl Pts',(-21.9245617765769,-13.5588214586604,
0.));
#197751=CARTESIAN_POINT('Ctrl Pts',(-21.9245617765769,-13.5588214586604,
12.));
#197752=CARTESIAN_POINT('Ctrl Pts',(-21.9525138592813,-13.5601389185257,
0.));
#197753=CARTESIAN_POINT('Ctrl Pts',(-21.9525138592813,-13.5601389185257,
12.));
#197754=CARTESIAN_POINT('Ctrl Pts',(-21.9805379899168,-13.5613968357561,
0.));
#197755=CARTESIAN_POINT('Ctrl Pts',(-21.9805379899168,-13.5613968357561,
12.));
#197756=CARTESIAN_POINT('Ctrl Pts',(-22.0086337943449,-13.5625949868333,
0.));
#197757=CARTESIAN_POINT('Ctrl Pts',(-22.0086337943449,-13.5625949868333,
12.));
#197758=CARTESIAN_POINT('Ctrl Pts',(-22.0368009736295,-13.5637332022473,
0.));
#197759=CARTESIAN_POINT('Ctrl Pts',(-22.0368009736295,-13.5637332022473,
12.));
#197760=CARTESIAN_POINT('Ctrl Pts',(-22.0650393089609,-13.5648113689033,
0.));
#197761=CARTESIAN_POINT('Ctrl Pts',(-22.0650393089609,-13.5648113689033,
12.));
#197762=CARTESIAN_POINT('Ctrl Pts',(-22.0933486464593,-13.5658294169284,
0.));
#197763=CARTESIAN_POINT('Ctrl Pts',(-22.0933486464593,-13.5658294169284,
12.));
#197764=CARTESIAN_POINT('Ctrl Pts',(-22.1217288871975,-13.5667873105359,
0.));
#197765=CARTESIAN_POINT('Ctrl Pts',(-22.1217288871975,-13.5667873105359,
12.));
#197766=CARTESIAN_POINT('Ctrl Pts',(-22.1444897575194,-13.5675054919061,
0.));
#197767=CARTESIAN_POINT('Ctrl Pts',(-22.1444897575194,-13.5675054919061,
12.));
#197768=CARTESIAN_POINT('Ctrl Pts',(-22.1615922805008,-13.5680170531805,
0.));
#197769=CARTESIAN_POINT('Ctrl Pts',(-22.1615922805008,-13.5680170531805,
12.));
#197770=CARTESIAN_POINT('Ctrl Pts',(-22.1730081264608,-13.5683460612942,
0.));
#197771=CARTESIAN_POINT('Ctrl Pts',(-22.1730081264608,-13.5683460612942,
12.));
#197772=CARTESIAN_POINT('Ctrl Pts',(-22.1787195904339,-13.5685075571671,
0.));
#197773=CARTESIAN_POINT('Ctrl Pts',(-22.1787195904339,-13.5685075571671,
12.));
#197774=CARTESIAN_POINT('',(-22.1787195904339,-13.5685075571671,0.));
#197775=CARTESIAN_POINT('Ctrl Pts',(-18.5896416359912,-12.7689476255363,
0.));
#197776=CARTESIAN_POINT('Ctrl Pts',(-18.5896460962964,-12.7689524524483,
0.));
#197777=CARTESIAN_POINT('Ctrl Pts',(-18.5896919669165,-12.768986426692,
0.));
#197778=CARTESIAN_POINT('Ctrl Pts',(-18.589871621843,-12.769110348199,0.));
#197779=CARTESIAN_POINT('Ctrl Pts',(-18.5903328777227,-12.7694215127919,
0.));
#197780=CARTESIAN_POINT('Ctrl Pts',(-18.5912775137806,-12.7700520897173,
0.));
#197781=CARTESIAN_POINT('Ctrl Pts',(-18.5925859134579,-12.7709195951156,
0.));
#197782=CARTESIAN_POINT('Ctrl Pts',(-18.5942490615407,-12.7720142287172,
0.));
#197783=CARTESIAN_POINT('Ctrl Pts',(-18.5962551167772,-12.7733231262108,
0.));
#197784=CARTESIAN_POINT('Ctrl Pts',(-18.598591752595,-12.7748328937638,
0.));
#197785=CARTESIAN_POINT('Ctrl Pts',(-18.6012488486709,-12.7765325225081,
0.));
#197786=CARTESIAN_POINT('Ctrl Pts',(-18.6042190183704,-12.7784139605066,
0.));
#197787=CARTESIAN_POINT('Ctrl Pts',(-18.6074961535723,-12.7804705387658,
0.));
#197788=CARTESIAN_POINT('Ctrl Pts',(-18.6110744826219,-12.7826959526925,
0.));
#197789=CARTESIAN_POINT('Ctrl Pts',(-18.6149475565188,-12.7850831657901,
0.));
#197790=CARTESIAN_POINT('Ctrl Pts',(-18.6191087624752,-12.7876249657834,
0.));
#197791=CARTESIAN_POINT('Ctrl Pts',(-18.6235516265575,-12.7903142925234,
0.));
#197792=CARTESIAN_POINT('Ctrl Pts',(-18.6282702819371,-12.7931447451555,
0.));
#197793=CARTESIAN_POINT('Ctrl Pts',(-18.6332595057006,-12.7961106222251,
0.));
#197794=CARTESIAN_POINT('Ctrl Pts',(-18.63851447924,-12.7992066625264,0.));
#197795=CARTESIAN_POINT('Ctrl Pts',(-18.6440306327456,-12.8024278770152,
0.));
#197796=CARTESIAN_POINT('Ctrl Pts',(-18.6498034438987,-12.805769331162,
0.));
#197797=CARTESIAN_POINT('Ctrl Pts',(-18.6558284825773,-12.8092261933858,
0.));
#197798=CARTESIAN_POINT('Ctrl Pts',(-18.6621014624746,-12.8127937909631,
0.));
#197799=CARTESIAN_POINT('Ctrl Pts',(-18.6686182952799,-12.8164676687362,
0.));
#197800=CARTESIAN_POINT('Ctrl Pts',(-18.6753751301092,-12.8202436318474,
0.));
#197801=CARTESIAN_POINT('Ctrl Pts',(-18.6823683094139,-12.8241176980017,
0.));
#197802=CARTESIAN_POINT('Ctrl Pts',(-18.6895943376171,-12.8280860635231,
0.));
#197803=CARTESIAN_POINT('Ctrl Pts',(-18.6970498410172,-12.8321450599789,
0.));
#197804=CARTESIAN_POINT('Ctrl Pts',(-18.7047315436294,-12.8362911280361,
0.));
#197805=CARTESIAN_POINT('Ctrl Pts',(-18.7126362754445,-12.8405208263431,
0.));
#197806=CARTESIAN_POINT('Ctrl Pts',(-18.7207609737702,-12.8448308329494,
0.));
#197807=CARTESIAN_POINT('Ctrl Pts',(-18.7291026886554,-12.8492179511591,
0.));
#197808=CARTESIAN_POINT('Ctrl Pts',(-18.7376585820854,-12.8536791086316,
0.));
#197809=CARTESIAN_POINT('Ctrl Pts',(-18.7464259171251,-12.8582113455646,
0.));
#197810=CARTESIAN_POINT('Ctrl Pts',(-18.7554020493887,-12.8628118054171,
0.));
#197811=CARTESIAN_POINT('Ctrl Pts',(-18.7645844169564,-12.8674777239653,
0.));
#197812=CARTESIAN_POINT('Ctrl Pts',(-18.7739705329022,-12.872206421181,
0.));
#197813=CARTESIAN_POINT('Ctrl Pts',(-18.7835579840477,-12.8769952998095,
0.));
#197814=CARTESIAN_POINT('Ctrl Pts',(-18.7933444285868,-12.8818418427475,
0.));
#197815=CARTESIAN_POINT('Ctrl Pts',(-18.8033275941943,-12.8867436109546,
0.));
#197816=CARTESIAN_POINT('Ctrl Pts',(-18.813505275782,-12.8916982409935,
0.));
#197817=CARTESIAN_POINT('Ctrl Pts',(-18.8238753319129,-12.8967034410755,
0.));
#197818=CARTESIAN_POINT('Ctrl Pts',(-18.834435681259,-12.9017569871738,
0.));
#197819=CARTESIAN_POINT('Ctrl Pts',(-18.8451842990984,-12.9068567191854,
0.));
#197820=CARTESIAN_POINT('Ctrl Pts',(-18.8561192136198,-12.9120005369063,
0.));
#197821=CARTESIAN_POINT('Ctrl Pts',(-18.8672385038326,-12.9171863977045,
0.));
#197822=CARTESIAN_POINT('Ctrl Pts',(-18.8785402977527,-12.9224123144982,
0.));
#197823=CARTESIAN_POINT('Ctrl Pts',(-18.8900227704889,-12.9276763536373,
0.));
#197824=CARTESIAN_POINT('Ctrl Pts',(-18.9016841423403,-12.9329766328185,
0.));
#197825=CARTESIAN_POINT('Ctrl Pts',(-18.9135226769465,-12.9383113190375,
0.));
#197826=CARTESIAN_POINT('Ctrl Pts',(-18.9255366795195,-12.9436786266105,
0.));
#197827=CARTESIAN_POINT('Ctrl Pts',(-18.9377244950435,-12.9490768151821,
0.));
#197828=CARTESIAN_POINT('Ctrl Pts',(-18.9500845064715,-12.9545041877377,
0.));
#197829=CARTESIAN_POINT('Ctrl Pts',(-18.9626151329229,-12.9599590886319,
0.));
#197830=CARTESIAN_POINT('Ctrl Pts',(-18.9753148284475,-12.9654399021869,
0.));
#197831=CARTESIAN_POINT('Ctrl Pts',(-18.9881820807586,-12.9709450512747,
0.));
#197832=CARTESIAN_POINT('Ctrl Pts',(-19.0012154099791,-12.9764729959205,
0.));
#197833=CARTESIAN_POINT('Ctrl Pts',(-19.0144133673348,-12.9820222318716,
0.));
#197834=CARTESIAN_POINT('Ctrl Pts',(-19.0277745339908,-12.9875912893003,
0.));
#197835=CARTESIAN_POINT('Ctrl Pts',(-19.0412975200398,-12.9931787316515,
0.));
#197836=CARTESIAN_POINT('Ctrl Pts',(-19.0549809634355,-12.9987831544502,
0.));
#197837=CARTESIAN_POINT('Ctrl Pts',(-19.0688235289437,-13.0044031841381,
0.));
#197838=CARTESIAN_POINT('Ctrl Pts',(-19.0828239070482,-13.0100374768785,
0.));
#197839=CARTESIAN_POINT('Ctrl Pts',(-19.0969808131226,-13.0156847176093,
0.));
#197840=CARTESIAN_POINT('Ctrl Pts',(-19.1112929866308,-13.0213436191326,
0.));
#197841=CARTESIAN_POINT('Ctrl Pts',(-19.1257591903099,-13.0270129211976,
0.));
#197842=CARTESIAN_POINT('Ctrl Pts',(-19.1403782093389,-13.0326913895841,
0.));
#197843=CARTESIAN_POINT('Ctrl Pts',(-19.1551488505233,-13.0383778152072,
0.));
#197844=CARTESIAN_POINT('Ctrl Pts',(-19.1700699416625,-13.0440710133775,
0.));
#197845=CARTESIAN_POINT('Ctrl Pts',(-19.1851403308825,-13.0497698230442,
0.));
#197846=CARTESIAN_POINT('Ctrl Pts',(-19.2003588859771,-13.0554731060537,
0.));
#197847=CARTESIAN_POINT('Ctrl Pts',(-19.2157244937141,-13.0611797463913,
0.));
#197848=CARTESIAN_POINT('Ctrl Pts',(-19.2312360592031,-13.0668886494791,
0.));
#197849=CARTESIAN_POINT('Ctrl Pts',(-19.2468925053988,-13.0725987415856,
0.));
#197850=CARTESIAN_POINT('Ctrl Pts',(-19.2626927725596,-13.0783089692118,
0.));
#197851=CARTESIAN_POINT('Ctrl Pts',(-19.2786358177198,-13.0840182984949,
0.));
#197852=CARTESIAN_POINT('Ctrl Pts',(-19.2947206141246,-13.0897257145969,
0.));
#197853=CARTESIAN_POINT('Ctrl Pts',(-19.3109461507358,-13.095430221148,
0.));
#197854=CARTESIAN_POINT('Ctrl Pts',(-19.3273114318268,-13.1011308397592,
0.));
#197855=CARTESIAN_POINT('Ctrl Pts',(-19.3438154765395,-13.1068266095186,
0.));
#197856=CARTESIAN_POINT('Ctrl Pts',(-19.3604573184516,-13.1125165865021,
0.));
#197857=CARTESIAN_POINT('Ctrl Pts',(-19.3772360051093,-13.118199843271,
0.));
#197858=CARTESIAN_POINT('Ctrl Pts',(-19.3941505976267,-13.1238754684177,
0.));
#197859=CARTESIAN_POINT('Ctrl Pts',(-19.4112001703561,-13.1295425661635,
0.));
#197860=CARTESIAN_POINT('Ctrl Pts',(-19.4283838105265,-13.1352002559439,
0.));
#197861=CARTESIAN_POINT('Ctrl Pts',(-19.4457006178875,-13.140847672006,
0.));
#197862=CARTESIAN_POINT('Ctrl Pts',(-19.463149704325,-13.1464839629966,
0.));
#197863=CARTESIAN_POINT('Ctrl Pts',(-19.4807301935256,-13.1521082915846,
0.));
#197864=CARTESIAN_POINT('Ctrl Pts',(-19.498441220707,-13.1577198341238,
0.));
#197865=CARTESIAN_POINT('Ctrl Pts',(-19.5162819323207,-13.1633177803097,
0.));
#197866=CARTESIAN_POINT('Ctrl Pts',(-19.5342514857564,-13.1689013328432,
0.));
#197867=CARTESIAN_POINT('Ctrl Pts',(-19.5523490490254,-13.1744697070918,
0.));
#197868=CARTESIAN_POINT('Ctrl Pts',(-19.5705738004682,-13.1800221307682,
0.));
#197869=CARTESIAN_POINT('Ctrl Pts',(-19.5889249285352,-13.1855578436479,
0.));
#197870=CARTESIAN_POINT('Ctrl Pts',(-19.6074016315421,-13.1910760972818,
0.));
#197871=CARTESIAN_POINT('Ctrl Pts',(-19.6260031174244,-13.196576154715,
0.));
#197872=CARTESIAN_POINT('Ctrl Pts',(-19.6447286034764,-13.202057290206,
0.));
#197873=CARTESIAN_POINT('Ctrl Pts',(-19.6635773160924,-13.2075187889522,
0.));
#197874=CARTESIAN_POINT('Ctrl Pts',(-19.6825484905812,-13.2129599468478,
0.));
#197875=CARTESIAN_POINT('Ctrl Pts',(-19.7016413709678,-13.2183800702431,
0.));
#197876=CARTESIAN_POINT('Ctrl Pts',(-19.7208552097867,-13.2237784757065,
0.));
#197877=CARTESIAN_POINT('Ctrl Pts',(-19.7401892678701,-13.2291544897902,
0.));
#197878=CARTESIAN_POINT('Ctrl Pts',(-19.7596428141176,-13.2345074487968,
0.));
#197879=CARTESIAN_POINT('Ctrl Pts',(-19.7792151253297,-13.239836698568,
0.));
#197880=CARTESIAN_POINT('Ctrl Pts',(-19.7989054860501,-13.2451415942809,
0.));
#197881=CARTESIAN_POINT('Ctrl Pts',(-19.8187131883919,-13.2504215002458,
0.));
#197882=CARTESIAN_POINT('Ctrl Pts',(-19.8386375318632,-13.2556757897085,
0.));
#197883=CARTESIAN_POINT('Ctrl Pts',(-19.8586778231711,-13.2609038446525,
0.));
#197884=CARTESIAN_POINT('Ctrl Pts',(-19.8788333760571,-13.2661050556128,
0.));
#197885=CARTESIAN_POINT('Ctrl Pts',(-19.8991035111739,-13.2712788215015,
0.));
#197886=CARTESIAN_POINT('Ctrl Pts',(-19.9194875559419,-13.2764245494354,
0.));
#197887=CARTESIAN_POINT('Ctrl Pts',(-19.9399848444019,-13.2815416545663,
0.));
#197888=CARTESIAN_POINT('Ctrl Pts',(-19.9605947170589,-13.2866295599152,
0.));
#197889=CARTESIAN_POINT('Ctrl Pts',(-19.9813165207174,-13.2916876962098,
0.));
#197890=CARTESIAN_POINT('Ctrl Pts',(-20.0021496083742,-13.296715501731,
0.));
#197891=CARTESIAN_POINT('Ctrl Pts',(-20.023093339104,-13.3017124221639,
0.));
#197892=CARTESIAN_POINT('Ctrl Pts',(-20.0441470779345,-13.3066779104515,
0.));
#197893=CARTESIAN_POINT('Ctrl Pts',(-20.0653101957188,-13.3116114266514,
0.));
#197894=CARTESIAN_POINT('Ctrl Pts',(-20.0865820689883,-13.3165124377963,
0.));
#197895=CARTESIAN_POINT('Ctrl Pts',(-20.1079620798377,-13.3213804177588,
0.));
#197896=CARTESIAN_POINT('Ctrl Pts',(-20.1294496158405,-13.3262148471228,
0.));
#197897=CARTESIAN_POINT('Ctrl Pts',(-20.1510440699477,-13.3310152130565,
0.));
#197898=CARTESIAN_POINT('Ctrl Pts',(-20.1727448403818,-13.3357810091903,
0.));
#197899=CARTESIAN_POINT('Ctrl Pts',(-20.1945513305233,-13.3405117354969,
0.));
#197900=CARTESIAN_POINT('Ctrl Pts',(-20.2164629487855,-13.3452068981763,
0.));
#197901=CARTESIAN_POINT('Ctrl Pts',(-20.2384791085354,-13.3498660095382,
0.));
#197902=CARTESIAN_POINT('Ctrl Pts',(-20.2605992280117,-13.3544885878886,
0.));
#197903=CARTESIAN_POINT('Ctrl Pts',(-20.2828227302337,-13.3590741574194,
0.));
#197904=CARTESIAN_POINT('Ctrl Pts',(-20.3051490429049,-13.3636222481017,
0.));
#197905=CARTESIAN_POINT('Ctrl Pts',(-20.3275775983032,-13.3681323955828,
0.));
#197906=CARTESIAN_POINT('Ctrl Pts',(-20.3501078331818,-13.3726041410869,
0.));
#197907=CARTESIAN_POINT('Ctrl Pts',(-20.3727391887187,-13.377037031319,
0.));
#197908=CARTESIAN_POINT('Ctrl Pts',(-20.3954711104505,-13.3814306183721,
0.));
#197909=CARTESIAN_POINT('Ctrl Pts',(-20.4183030482002,-13.3857844596387,
0.));
#197910=CARTESIAN_POINT('Ctrl Pts',(-20.4412344560007,-13.3900981177254,
0.));
#197911=CARTESIAN_POINT('Ctrl Pts',(-20.4642647920038,-13.3943711603739,
0.));
#197912=CARTESIAN_POINT('Ctrl Pts',(-20.4873935184041,-13.3986031603716,
0.));
#197913=CARTESIAN_POINT('Ctrl Pts',(-20.5106201013755,-13.4027936954529,
0.));
#197914=CARTESIAN_POINT('Ctrl Pts',(-20.5339440109958,-13.4069423482076,
0.));
#197915=CARTESIAN_POINT('Ctrl Pts',(-20.557364721164,-13.4110487059912,
0.));
#197916=CARTESIAN_POINT('Ctrl Pts',(-20.5808817095155,-13.4151123608411,
0.));
#197917=CARTESIAN_POINT('Ctrl Pts',(-20.6044944573151,-13.4191329093932,
0.));
#197918=CARTESIAN_POINT('Ctrl Pts',(-20.6282024494234,-13.4231099528178,
0.));
#197919=CARTESIAN_POINT('Ctrl Pts',(-20.6520051742868,-13.427043096765,
0.));
#197920=CARTESIAN_POINT('Ctrl Pts',(-20.6759021239102,-13.4309319513119,
0.));
#197921=CARTESIAN_POINT('Ctrl Pts',(-20.6998927938288,-13.4347761309154,
0.));
#197922=CARTESIAN_POINT('Ctrl Pts',(-20.7239766830675,-13.4385752543663,
0.));
#197923=CARTESIAN_POINT('Ctrl Pts',(-20.7481532941014,-13.4423289447561,
0.));
#197924=CARTESIAN_POINT('Ctrl Pts',(-20.7724221327609,-13.4460368293689,
0.));
#197925=CARTESIAN_POINT('Ctrl Pts',(-20.7967827081228,-13.4496985395637,
0.));
#197926=CARTESIAN_POINT('Ctrl Pts',(-20.821234532398,-13.4533137106667,
0.));
#197927=CARTESIAN_POINT('Ctrl Pts',(-20.8457771208083,-13.4568819818631,
0.));
#197928=CARTESIAN_POINT('Ctrl Pts',(-20.8704099914641,-13.4604029960983,
0.));
#197929=CARTESIAN_POINT('Ctrl Pts',(-20.8951326652158,-13.4638763999725,
0.));
#197930=CARTESIAN_POINT('Ctrl Pts',(-20.9199446657583,-13.4673018437717,
0.));
#197931=CARTESIAN_POINT('Ctrl Pts',(-20.9448455197557,-13.4706789815166,
0.));
#197932=CARTESIAN_POINT('Ctrl Pts',(-20.9698347569477,-13.4740074710086,
0.));
#197933=CARTESIAN_POINT('Ctrl Pts',(-20.9949119102592,-13.4772869738879,
0.));
#197934=CARTESIAN_POINT('Ctrl Pts',(-21.0200765158884,-13.4805171556822,
0.));
#197935=CARTESIAN_POINT('Ctrl Pts',(-21.0453281134245,-13.4836976858912,
0.));
#197936=CARTESIAN_POINT('Ctrl Pts',(-21.0706662455199,-13.4868282377191,
0.));
#197937=CARTESIAN_POINT('Ctrl Pts',(-21.0960904575046,-13.4899084877717,
0.));
#197938=CARTESIAN_POINT('Ctrl Pts',(-21.1216002970207,-13.4929381157778,
0.));
#197939=CARTESIAN_POINT('Ctrl Pts',(-21.1471953136209,-13.4959168042934,
0.));
#197940=CARTESIAN_POINT('Ctrl Pts',(-21.1728750584175,-13.4988442384491,
0.));
#197941=CARTESIAN_POINT('Ctrl Pts',(-21.1986390835828,-13.5017201056088,
0.));
#197942=CARTESIAN_POINT('Ctrl Pts',(-21.2244869429332,-13.5045440957404,
0.));
#197943=CARTESIAN_POINT('Ctrl Pts',(-21.250418192743,-13.5073159019452,
0.));
#197944=CARTESIAN_POINT('Ctrl Pts',(-21.2764323924442,-13.5100352209205,
0.));
#197945=CARTESIAN_POINT('Ctrl Pts',(-21.3025291054235,-13.5127017534971,
0.));
#197946=CARTESIAN_POINT('Ctrl Pts',(-21.3287078996341,-13.5153152050555,
0.));
#197947=CARTESIAN_POINT('Ctrl Pts',(-21.3549683486222,-13.5178752862466,
0.));
#197948=CARTESIAN_POINT('Ctrl Pts',(-21.3813100304973,-13.5203817122504,
0.));
#197949=CARTESIAN_POINT('Ctrl Pts',(-21.4077325259324,-13.5228342013516,
0.));
#197950=CARTESIAN_POINT('Ctrl Pts',(-21.4342354165259,-13.5252324737802,
0.));
#197951=CARTESIAN_POINT('Ctrl Pts',(-21.4608182828697,-13.5275762503555,
0.));
#197952=CARTESIAN_POINT('Ctrl Pts',(-21.4874807030468,-13.5298652514355,
0.));
#197953=CARTESIAN_POINT('Ctrl Pts',(-21.5142222501666,-13.5320991952138,
0.));
#197954=CARTESIAN_POINT('Ctrl Pts',(-21.5410424932503,-13.5342777983215,
0.));
#197955=CARTESIAN_POINT('Ctrl Pts',(-21.5679410019001,-13.536400779028,
0.));
#197956=CARTESIAN_POINT('Ctrl Pts',(-21.5949173499013,-13.5384678597195,
0.));
#197957=CARTESIAN_POINT('Ctrl Pts',(-21.6219711193946,-13.5404787697792,
0.));
#197958=CARTESIAN_POINT('Ctrl Pts',(-21.6491019044648,-13.5424332480699,
0.));
#197959=CARTESIAN_POINT('Ctrl Pts',(-21.6763093157699,-13.5443310461526,
0.));
#197960=CARTESIAN_POINT('Ctrl Pts',(-21.7035929822955,-13.5461719295048,
0.));
#197961=CARTESIAN_POINT('Ctrl Pts',(-21.7309525412281,-13.5479556704481,
0.));
#197962=CARTESIAN_POINT('Ctrl Pts',(-21.7583876294554,-13.5496820422211,
0.));
#197963=CARTESIAN_POINT('Ctrl Pts',(-21.7858978745865,-13.551350812725,
0.));
#197964=CARTESIAN_POINT('Ctrl Pts',(-21.8134828857967,-13.5529617381573,
0.));
#197965=CARTESIAN_POINT('Ctrl Pts',(-21.8411422456075,-13.5545145573031,
0.));
#197966=CARTESIAN_POINT('Ctrl Pts',(-21.8688754989365,-13.5560089839385,
0.));
#197967=CARTESIAN_POINT('Ctrl Pts',(-21.8966821688824,-13.5574447178424,
0.));
#197968=CARTESIAN_POINT('Ctrl Pts',(-21.9245617765769,-13.5588214586604,
0.));
#197969=CARTESIAN_POINT('Ctrl Pts',(-21.9525138592813,-13.5601389185257,
0.));
#197970=CARTESIAN_POINT('Ctrl Pts',(-21.9805379899168,-13.5613968357561,
0.));
#197971=CARTESIAN_POINT('Ctrl Pts',(-22.0086337943449,-13.5625949868333,
0.));
#197972=CARTESIAN_POINT('Ctrl Pts',(-22.0368009736295,-13.5637332022473,
0.));
#197973=CARTESIAN_POINT('Ctrl Pts',(-22.0650393089609,-13.5648113689033,
0.));
#197974=CARTESIAN_POINT('Ctrl Pts',(-22.0933486464593,-13.5658294169284,
0.));
#197975=CARTESIAN_POINT('Ctrl Pts',(-22.1217288871975,-13.5667873105359,
0.));
#197976=CARTESIAN_POINT('Ctrl Pts',(-22.1444897575194,-13.5675054919061,
0.));
#197977=CARTESIAN_POINT('Ctrl Pts',(-22.1615922805008,-13.5680170531805,
0.));
#197978=CARTESIAN_POINT('Ctrl Pts',(-22.1730081264608,-13.5683460612942,
0.));
#197979=CARTESIAN_POINT('Ctrl Pts',(-22.1787195904339,-13.5685075571671,
0.));
#197980=CARTESIAN_POINT('',(-22.178719590434,-13.5685075571671,0.));
#197981=CARTESIAN_POINT('Origin',(-20.2687213152502,-7.17139709155223,0.));
#197982=CARTESIAN_POINT('',(-21.2610617890679,-7.52250298901264,0.));
#197983=CARTESIAN_POINT('',(-21.2610617890679,-7.52250298901264,0.));
#197984=CARTESIAN_POINT('',(-10.1343606576251,-3.58569854577611,0.));
#197985=CARTESIAN_POINT('Ctrl Pts',(-22.8400320311649,-12.4230808101438,
0.));
#197986=CARTESIAN_POINT('Ctrl Pts',(-22.8400320311649,-12.4230808101438,
12.));
#197987=CARTESIAN_POINT('Ctrl Pts',(-22.8370364396459,-12.418215285186,
0.));
#197988=CARTESIAN_POINT('Ctrl Pts',(-22.8370364396459,-12.418215285186,
12.));
#197989=CARTESIAN_POINT('Ctrl Pts',(-22.8310435872748,-12.4084933766346,
0.));
#197990=CARTESIAN_POINT('Ctrl Pts',(-22.8310435872748,-12.4084933766346,
12.));
#197991=CARTESIAN_POINT('Ctrl Pts',(-22.8220493007173,-12.3939379378998,
0.));
#197992=CARTESIAN_POINT('Ctrl Pts',(-22.8220493007173,-12.3939379378998,
12.));
#197993=CARTESIAN_POINT('Ctrl Pts',(-22.81004690224,-12.374585536673,0.));
#197994=CARTESIAN_POINT('Ctrl Pts',(-22.81004690224,-12.374585536673,12.));
#197995=CARTESIAN_POINT('Ctrl Pts',(-22.795027221673,-12.3504864740319,
0.));
#197996=CARTESIAN_POINT('Ctrl Pts',(-22.795027221673,-12.3504864740319,
12.));
#197997=CARTESIAN_POINT('Ctrl Pts',(-22.7799908974768,-12.3264788926075,
0.));
#197998=CARTESIAN_POINT('Ctrl Pts',(-22.7799908974768,-12.3264788926075,
12.));
#197999=CARTESIAN_POINT('Ctrl Pts',(-22.764938010105,-12.3025628601792,
0.));
#198000=CARTESIAN_POINT('Ctrl Pts',(-22.764938010105,-12.3025628601792,
12.));
#198001=CARTESIAN_POINT('Ctrl Pts',(-22.7498686970069,-12.2787384750742,
0.));
#198002=CARTESIAN_POINT('Ctrl Pts',(-22.7498686970069,-12.2787384750742,
12.));
#198003=CARTESIAN_POINT('Ctrl Pts',(-22.7347831655287,-12.2550058702395,
0.));
#198004=CARTESIAN_POINT('Ctrl Pts',(-22.7347831655287,-12.2550058702395,
12.));
#198005=CARTESIAN_POINT('Ctrl Pts',(-22.7196817119374,-12.2313652198061,
0.));
#198006=CARTESIAN_POINT('Ctrl Pts',(-22.7196817119374,-12.2313652198061,
12.));
#198007=CARTESIAN_POINT('Ctrl Pts',(-22.7045647168747,-12.2078167360284,
0.));
#198008=CARTESIAN_POINT('Ctrl Pts',(-22.7045647168747,-12.2078167360284,
12.));
#198009=CARTESIAN_POINT('Ctrl Pts',(-22.6894326205037,-12.1843606579261,
0.));
#198010=CARTESIAN_POINT('Ctrl Pts',(-22.6894326205037,-12.1843606579261,
12.));
#198011=CARTESIAN_POINT('Ctrl Pts',(-22.6742859034944,-12.1609972423099,
0.));
#198012=CARTESIAN_POINT('Ctrl Pts',(-22.6742859034944,-12.1609972423099,
12.));
#198013=CARTESIAN_POINT('Ctrl Pts',(-22.6591250653965,-12.1377267537145,
0.));
#198014=CARTESIAN_POINT('Ctrl Pts',(-22.6591250653965,-12.1377267537145,
12.));
#198015=CARTESIAN_POINT('Ctrl Pts',(-22.6439506046605,-12.1145494550383,
0.));
#198016=CARTESIAN_POINT('Ctrl Pts',(-22.6439506046605,-12.1145494550383,
12.));
#198017=CARTESIAN_POINT('Ctrl Pts',(-22.6287629967056,-12.0914655972823,
0.));
#198018=CARTESIAN_POINT('Ctrl Pts',(-22.6287629967056,-12.0914655972823,
12.));
#198019=CARTESIAN_POINT('Ctrl Pts',(-22.6135626764898,-12.0684754113862,
0.));
#198020=CARTESIAN_POINT('Ctrl Pts',(-22.6135626764898,-12.0684754113862,
12.));
#198021=CARTESIAN_POINT('Ctrl Pts',(-22.5983500505644,-12.0455791139128,
0.));
#198022=CARTESIAN_POINT('Ctrl Pts',(-22.5983500505644,-12.0455791139128,
12.));
#198023=CARTESIAN_POINT('Ctrl Pts',(-22.5831255061282,-12.0227769113127,
0.));
#198024=CARTESIAN_POINT('Ctrl Pts',(-22.5831255061282,-12.0227769113127,
12.));
#198025=CARTESIAN_POINT('Ctrl Pts',(-22.5678894211181,-12.0000690046695,
0.));
#198026=CARTESIAN_POINT('Ctrl Pts',(-22.5678894211181,-12.0000690046695,
12.));
#198027=CARTESIAN_POINT('Ctrl Pts',(-22.5526421741158,-11.9774555943496,
0.));
#198028=CARTESIAN_POINT('Ctrl Pts',(-22.5526421741158,-11.9774555943496,
12.));
#198029=CARTESIAN_POINT('Ctrl Pts',(-22.5373841537307,-11.9549368843997,
0.));
#198030=CARTESIAN_POINT('Ctrl Pts',(-22.5373841537307,-11.9549368843997,
12.));
#198031=CARTESIAN_POINT('Ctrl Pts',(-22.5221157697883,-11.9325130877803,
0.));
#198032=CARTESIAN_POINT('Ctrl Pts',(-22.5221157697883,-11.9325130877803,
12.));
#198033=CARTESIAN_POINT('Ctrl Pts',(-22.5068374513973,-11.9101844254557,
0.));
#198034=CARTESIAN_POINT('Ctrl Pts',(-22.5068374513973,-11.9101844254557,
12.));
#198035=CARTESIAN_POINT('Ctrl Pts',(-22.4915496418485,-11.8879511239942,
0.));
#198036=CARTESIAN_POINT('Ctrl Pts',(-22.4915496418485,-11.8879511239942,
12.));
#198037=CARTESIAN_POINT('Ctrl Pts',(-22.4762527946702,-11.8658134137019,
0.));
#198038=CARTESIAN_POINT('Ctrl Pts',(-22.4762527946702,-11.8658134137019,
12.));
#198039=CARTESIAN_POINT('Ctrl Pts',(-22.4609473690471,-11.8437715264487,
0.));
#198040=CARTESIAN_POINT('Ctrl Pts',(-22.4609473690471,-11.8437715264487,
12.));
#198041=CARTESIAN_POINT('Ctrl Pts',(-22.4456338258735,-11.8218256937889,
0.));
#198042=CARTESIAN_POINT('Ctrl Pts',(-22.4456338258735,-11.8218256937889,
12.));
#198043=CARTESIAN_POINT('Ctrl Pts',(-22.430312622646,-11.7999761445173,
0.));
#198044=CARTESIAN_POINT('Ctrl Pts',(-22.430312622646,-11.7999761445173,
12.));
#198045=CARTESIAN_POINT('Ctrl Pts',(-22.4149842125008,-11.7782231042039,
0.));
#198046=CARTESIAN_POINT('Ctrl Pts',(-22.4149842125008,-11.7782231042039,
12.));
#198047=CARTESIAN_POINT('Ctrl Pts',(-22.3996490469191,-11.7565667964764,
0.));
#198048=CARTESIAN_POINT('Ctrl Pts',(-22.3996490469191,-11.7565667964764,
12.));
#198049=CARTESIAN_POINT('Ctrl Pts',(-22.3843075773899,-11.7350074437961,
0.));
#198050=CARTESIAN_POINT('Ctrl Pts',(-22.3843075773899,-11.7350074437961,
12.));
#198051=CARTESIAN_POINT('Ctrl Pts',(-22.3689602575491,-11.7135452684532,
0.));
#198052=CARTESIAN_POINT('Ctrl Pts',(-22.3689602575491,-11.7135452684532,
12.));
#198053=CARTESIAN_POINT('Ctrl Pts',(-22.3536075450029,-11.6921804934056,
0.));
#198054=CARTESIAN_POINT('Ctrl Pts',(-22.3536075450029,-11.6921804934056,
12.));
#198055=CARTESIAN_POINT('Ctrl Pts',(-22.3382499035619,-11.6709133432985,
0.));
#198056=CARTESIAN_POINT('Ctrl Pts',(-22.3382499035619,-11.6709133432985,
12.));
#198057=CARTESIAN_POINT('Ctrl Pts',(-22.3228878043976,-11.6497440449857,
0.));
#198058=CARTESIAN_POINT('Ctrl Pts',(-22.3228878043976,-11.6497440449857,
12.));
#198059=CARTESIAN_POINT('Ctrl Pts',(-22.3075217249049,-11.6286728270009,
0.));
#198060=CARTESIAN_POINT('Ctrl Pts',(-22.3075217249049,-11.6286728270009,
12.));
#198061=CARTESIAN_POINT('Ctrl Pts',(-22.2921521480356,-11.6076999192357,
0.));
#198062=CARTESIAN_POINT('Ctrl Pts',(-22.2921521480356,-11.6076999192357,
12.));
#198063=CARTESIAN_POINT('Ctrl Pts',(-22.2767795614348,-11.5868255525188,
0.));
#198064=CARTESIAN_POINT('Ctrl Pts',(-22.2767795614348,-11.5868255525188,
12.));
#198065=CARTESIAN_POINT('Ctrl Pts',(-22.2614044566898,-11.5660499582403,
0.));
#198066=CARTESIAN_POINT('Ctrl Pts',(-22.2614044566898,-11.5660499582403,
12.));
#198067=CARTESIAN_POINT('Ctrl Pts',(-22.2460273284654,-11.5453733679121,
0.));
#198068=CARTESIAN_POINT('Ctrl Pts',(-22.2460273284654,-11.5453733679121,
12.));
#198069=CARTESIAN_POINT('Ctrl Pts',(-22.2306486738901,-11.5247960128477,
0.));
#198070=CARTESIAN_POINT('Ctrl Pts',(-22.2306486738901,-11.5247960128477,
12.));
#198071=CARTESIAN_POINT('Ctrl Pts',(-22.2152689931022,-11.5043181244242,
0.));
#198072=CARTESIAN_POINT('Ctrl Pts',(-22.2152689931022,-11.5043181244242,
12.));
#198073=CARTESIAN_POINT('Ctrl Pts',(-22.1998887896436,-11.483939934259,
0.));
#198074=CARTESIAN_POINT('Ctrl Pts',(-22.1998887896436,-11.483939934259,
12.));
#198075=CARTESIAN_POINT('Ctrl Pts',(-22.184508570917,-11.463661674411,0.));
#198076=CARTESIAN_POINT('Ctrl Pts',(-22.184508570917,-11.463661674411,12.));
#198077=CARTESIAN_POINT('Ctrl Pts',(-22.1691288486096,-11.443483577557,
0.));
#198078=CARTESIAN_POINT('Ctrl Pts',(-22.1691288486096,-11.443483577557,
12.));
#198079=CARTESIAN_POINT('Ctrl Pts',(-22.1537501391487,-11.4234058771742,
0.));
#198080=CARTESIAN_POINT('Ctrl Pts',(-22.1537501391487,-11.4234058771742,
12.));
#198081=CARTESIAN_POINT('Ctrl Pts',(-22.1383729640964,-11.4034288076908,
0.));
#198082=CARTESIAN_POINT('Ctrl Pts',(-22.1383729640964,-11.4034288076908,
12.));
#198083=CARTESIAN_POINT('Ctrl Pts',(-22.1229978500186,-11.3835526044256,
0.));
#198084=CARTESIAN_POINT('Ctrl Pts',(-22.1229978500186,-11.3835526044256,
12.));
#198085=CARTESIAN_POINT('Ctrl Pts',(-22.1076253283979,-11.3637775035367,
0.));
#198086=CARTESIAN_POINT('Ctrl Pts',(-22.1076253283979,-11.3637775035367,
12.));
#198087=CARTESIAN_POINT('Ctrl Pts',(-22.0922559355294,-11.3441037419553,
0.));
#198088=CARTESIAN_POINT('Ctrl Pts',(-22.0922559355294,-11.3441037419553,
12.));
#198089=CARTESIAN_POINT('Ctrl Pts',(-22.0768902124267,-11.3245315573168,
0.));
#198090=CARTESIAN_POINT('Ctrl Pts',(-22.0768902124267,-11.3245315573168,
12.));
#198091=CARTESIAN_POINT('Ctrl Pts',(-22.0615287047179,-11.3050611878771,
0.));
#198092=CARTESIAN_POINT('Ctrl Pts',(-22.0615287047179,-11.3050611878771,
12.));
#198093=CARTESIAN_POINT('Ctrl Pts',(-22.046171962566,-11.2856928724374,
0.));
#198094=CARTESIAN_POINT('Ctrl Pts',(-22.046171962566,-11.2856928724374,
12.));
#198095=CARTESIAN_POINT('Ctrl Pts',(-22.030820540835,-11.2664268504206,
0.));
#198096=CARTESIAN_POINT('Ctrl Pts',(-22.030820540835,-11.2664268504206,
12.));
#198097=CARTESIAN_POINT('Ctrl Pts',(-22.0154749992363,-11.2472633619275,
0.));
#198098=CARTESIAN_POINT('Ctrl Pts',(-22.0154749992363,-11.2472633619275,
12.));
#198099=CARTESIAN_POINT('Ctrl Pts',(-22.0001359024839,-11.2282026477896,
0.));
#198100=CARTESIAN_POINT('Ctrl Pts',(-22.0001359024839,-11.2282026477896,
12.));
#198101=CARTESIAN_POINT('Ctrl Pts',(-21.9848038204439,-11.2092449496125,
0.));
#198102=CARTESIAN_POINT('Ctrl Pts',(-21.9848038204439,-11.2092449496125,
12.));
#198103=CARTESIAN_POINT('Ctrl Pts',(-21.9694793282914,-11.190390509811,
0.));
#198104=CARTESIAN_POINT('Ctrl Pts',(-21.9694793282914,-11.190390509811,
12.));
#198105=CARTESIAN_POINT('Ctrl Pts',(-21.9541630066506,-11.1716395716376,
0.));
#198106=CARTESIAN_POINT('Ctrl Pts',(-21.9541630066506,-11.1716395716376,
12.));
#198107=CARTESIAN_POINT('Ctrl Pts',(-21.9388554416439,-11.1529923792003,
0.));
#198108=CARTESIAN_POINT('Ctrl Pts',(-21.9388554416439,-11.1529923792003,
12.));
#198109=CARTESIAN_POINT('Ctrl Pts',(-21.923557224952,-11.1344491774741,
0.));
#198110=CARTESIAN_POINT('Ctrl Pts',(-21.923557224952,-11.1344491774741,
12.));
#198111=CARTESIAN_POINT('Ctrl Pts',(-21.9082689538688,-11.1160102123024,
0.));
#198112=CARTESIAN_POINT('Ctrl Pts',(-21.9082689538688,-11.1160102123024,
12.));
#198113=CARTESIAN_POINT('Ctrl Pts',(-21.8929912313608,-11.0976757303944,
0.));
#198114=CARTESIAN_POINT('Ctrl Pts',(-21.8929912313608,-11.0976757303944,
12.));
#198115=CARTESIAN_POINT('Ctrl Pts',(-21.877724666119,-11.0794459793057,
0.));
#198116=CARTESIAN_POINT('Ctrl Pts',(-21.877724666119,-11.0794459793057,
12.));
#198117=CARTESIAN_POINT('Ctrl Pts',(-21.8624698726318,-11.0613212074363,
0.));
#198118=CARTESIAN_POINT('Ctrl Pts',(-21.8624698726318,-11.0613212074363,
12.));
#198119=CARTESIAN_POINT('Ctrl Pts',(-21.8472274713103,-11.0433016640807,
0.));
#198120=CARTESIAN_POINT('Ctrl Pts',(-21.8472274713103,-11.0433016640807,
12.));
#198121=CARTESIAN_POINT('Ctrl Pts',(-21.8319980886033,-11.0253875994598,
0.));
#198122=CARTESIAN_POINT('Ctrl Pts',(-21.8319980886033,-11.0253875994598,
12.));
#198123=CARTESIAN_POINT('Ctrl Pts',(-21.8167823571168,-11.0075792647477,
0.));
#198124=CARTESIAN_POINT('Ctrl Pts',(-21.8167823571168,-11.0075792647477,
12.));
#198125=CARTESIAN_POINT('Ctrl Pts',(-21.8015809157301,-10.9898769120912,
0.));
#198126=CARTESIAN_POINT('Ctrl Pts',(-21.8015809157301,-10.9898769120912,
12.));
#198127=CARTESIAN_POINT('Ctrl Pts',(-21.7863944097141,-10.9722807946155,
0.));
#198128=CARTESIAN_POINT('Ctrl Pts',(-21.7863944097141,-10.9722807946155,
12.));
#198129=CARTESIAN_POINT('Ctrl Pts',(-21.7712234908464,-10.9547911664455,
0.));
#198130=CARTESIAN_POINT('Ctrl Pts',(-21.7712234908464,-10.9547911664455,
12.));
#198131=CARTESIAN_POINT('Ctrl Pts',(-21.7560688175247,-10.9374082827444,
0.));
#198132=CARTESIAN_POINT('Ctrl Pts',(-21.7560688175247,-10.9374082827444,
12.));
#198133=CARTESIAN_POINT('Ctrl Pts',(-21.7409310548797,-10.9201323997384,
0.));
#198134=CARTESIAN_POINT('Ctrl Pts',(-21.7409310548797,-10.9201323997384,
12.));
#198135=CARTESIAN_POINT('Ctrl Pts',(-21.7258108748873,-10.902963774734,
0.));
#198136=CARTESIAN_POINT('Ctrl Pts',(-21.7258108748873,-10.902963774734,
12.));
#198137=CARTESIAN_POINT('Ctrl Pts',(-21.7107089564825,-10.8859026661293,
0.));
#198138=CARTESIAN_POINT('Ctrl Pts',(-21.7107089564825,-10.8859026661293,
12.));
#198139=CARTESIAN_POINT('Ctrl Pts',(-21.6956259856672,-10.8689493334095,
0.));
#198140=CARTESIAN_POINT('Ctrl Pts',(-21.6956259856672,-10.8689493334095,
12.));
#198141=CARTESIAN_POINT('Ctrl Pts',(-21.6805626556467,-10.8521040371835,
0.));
#198142=CARTESIAN_POINT('Ctrl Pts',(-21.6805626556467,-10.8521040371835,
12.));
#198143=CARTESIAN_POINT('Ctrl Pts',(-21.6655196669732,-10.8353670392272,
0.));
#198144=CARTESIAN_POINT('Ctrl Pts',(-21.6655196669732,-10.8353670392272,
12.));
#198145=CARTESIAN_POINT('Ctrl Pts',(-21.6504977276866,-10.8187386025136,
0.));
#198146=CARTESIAN_POINT('Ctrl Pts',(-21.6504977276866,-10.8187386025136,
12.));
#198147=CARTESIAN_POINT('Ctrl Pts',(-21.6354975534557,-10.8022189912369,
0.));
#198148=CARTESIAN_POINT('Ctrl Pts',(-21.6354975534557,-10.8022189912369,
12.));
#198149=CARTESIAN_POINT('Ctrl Pts',(-21.6205198677173,-10.7858084708261,
0.));
#198150=CARTESIAN_POINT('Ctrl Pts',(-21.6205198677173,-10.7858084708261,
12.));
#198151=CARTESIAN_POINT('Ctrl Pts',(-21.6055654018176,-10.7695073079552,
0.));
#198152=CARTESIAN_POINT('Ctrl Pts',(-21.6055654018176,-10.7695073079552,
12.));
#198153=CARTESIAN_POINT('Ctrl Pts',(-21.5906348951743,-10.7533157705941,
0.));
#198154=CARTESIAN_POINT('Ctrl Pts',(-21.5906348951743,-10.7533157705941,
12.));
#198155=CARTESIAN_POINT('Ctrl Pts',(-21.5757290954371,-10.7372341280467,
0.));
#198156=CARTESIAN_POINT('Ctrl Pts',(-21.5757290954371,-10.7372341280467,
12.));
#198157=CARTESIAN_POINT('Ctrl Pts',(-21.5608487586468,-10.7212626509816,
0.));
#198158=CARTESIAN_POINT('Ctrl Pts',(-21.5608487586468,-10.7212626509816,
12.));
#198159=CARTESIAN_POINT('Ctrl Pts',(-21.5459946493955,-10.7054016114571,
0.));
#198160=CARTESIAN_POINT('Ctrl Pts',(-21.5459946493955,-10.7054016114571,
12.));
#198161=CARTESIAN_POINT('Ctrl Pts',(-21.5311675409807,-10.689651282929,
0.));
#198162=CARTESIAN_POINT('Ctrl Pts',(-21.5311675409807,-10.689651282929,
12.));
#198163=CARTESIAN_POINT('Ctrl Pts',(-21.51636821558,-10.6740119402834,0.));
#198164=CARTESIAN_POINT('Ctrl Pts',(-21.51636821558,-10.6740119402834,12.));
#198165=CARTESIAN_POINT('Ctrl Pts',(-21.5015974644449,-10.6584838598939,
0.));
#198166=CARTESIAN_POINT('Ctrl Pts',(-21.5015974644449,-10.6584838598939,
12.));
#198167=CARTESIAN_POINT('Ctrl Pts',(-21.4868560880889,-10.6430673196607,
0.));
#198168=CARTESIAN_POINT('Ctrl Pts',(-21.4868560880889,-10.6430673196607,
12.));
#198169=CARTESIAN_POINT('Ctrl Pts',(-21.4721448964766,-10.6277625990456,
0.));
#198170=CARTESIAN_POINT('Ctrl Pts',(-21.4721448964766,-10.6277625990456,
12.));
#198171=CARTESIAN_POINT('Ctrl Pts',(-21.4574647092097,-10.6125699790961,
0.));
#198172=CARTESIAN_POINT('Ctrl Pts',(-21.4574647092097,-10.6125699790961,
12.));
#198173=CARTESIAN_POINT('Ctrl Pts',(-21.4428163557144,-10.5974897424622,
0.));
#198174=CARTESIAN_POINT('Ctrl Pts',(-21.4428163557144,-10.5974897424622,
12.));
#198175=CARTESIAN_POINT('Ctrl Pts',(-21.4282006754631,-10.5825221734573,
0.));
#198176=CARTESIAN_POINT('Ctrl Pts',(-21.4282006754631,-10.5825221734573,
12.));
#198177=CARTESIAN_POINT('Ctrl Pts',(-21.4136185181979,-10.5676675581108,
0.));
#198178=CARTESIAN_POINT('Ctrl Pts',(-21.4136185181979,-10.5676675581108,
12.));
#198179=CARTESIAN_POINT('Ctrl Pts',(-21.3990707441497,-10.5529261842108,
0.));
#198180=CARTESIAN_POINT('Ctrl Pts',(-21.3990707441497,-10.5529261842108,
12.));
#198181=CARTESIAN_POINT('Ctrl Pts',(-21.3845582242602,-10.5382983413421,
0.));
#198182=CARTESIAN_POINT('Ctrl Pts',(-21.3845582242602,-10.5382983413421,
12.));
#198183=CARTESIAN_POINT('Ctrl Pts',(-21.3700818403936,-10.5237843209057,
0.));
#198184=CARTESIAN_POINT('Ctrl Pts',(-21.3700818403936,-10.5237843209057,
12.));
#198185=CARTESIAN_POINT('Ctrl Pts',(-21.3556424855814,-10.5093844161685,
0.));
#198186=CARTESIAN_POINT('Ctrl Pts',(-21.3556424855814,-10.5093844161685,
12.));
#198187=CARTESIAN_POINT('Ctrl Pts',(-21.3412410642904,-10.4950989223337,
0.));
#198188=CARTESIAN_POINT('Ctrl Pts',(-21.3412410642904,-10.4950989223337,
12.));
#198189=CARTESIAN_POINT('Ctrl Pts',(-21.3268784926819,-10.4809281365931,
0.));
#198190=CARTESIAN_POINT('Ctrl Pts',(-21.3268784926819,-10.4809281365931,
12.));
#198191=CARTESIAN_POINT('Ctrl Pts',(-21.3125556988731,-10.4668723581768,
0.));
#198192=CARTESIAN_POINT('Ctrl Pts',(-21.3125556988731,-10.4668723581768,
12.));
#198193=CARTESIAN_POINT('Ctrl Pts',(-21.2982736231931,-10.4529318883874,
0.));
#198194=CARTESIAN_POINT('Ctrl Pts',(-21.2982736231931,-10.4529318883874,
12.));
#198195=CARTESIAN_POINT('Ctrl Pts',(-21.2840332184483,-10.4391070306391,
0.));
#198196=CARTESIAN_POINT('Ctrl Pts',(-21.2840332184483,-10.4391070306391,
12.));
#198197=CARTESIAN_POINT('Ctrl Pts',(-21.2698354502403,-10.42539809054,0.));
#198198=CARTESIAN_POINT('Ctrl Pts',(-21.2698354502403,-10.42539809054,12.));
#198199=CARTESIAN_POINT('Ctrl Pts',(-21.255681297275,-10.4118053759588,
0.));
#198200=CARTESIAN_POINT('Ctrl Pts',(-21.255681297275,-10.4118053759588,
12.));
#198201=CARTESIAN_POINT('Ctrl Pts',(-21.2415717516714,-10.3983291970846,
0.));
#198202=CARTESIAN_POINT('Ctrl Pts',(-21.2415717516714,-10.3983291970846,
12.));
#198203=CARTESIAN_POINT('Ctrl Pts',(-21.22750781927,-10.3849698664786,0.));
#198204=CARTESIAN_POINT('Ctrl Pts',(-21.22750781927,-10.3849698664786,12.));
#198205=CARTESIAN_POINT('Ctrl Pts',(-21.2134905199345,-10.371727699113,
0.));
#198206=CARTESIAN_POINT('Ctrl Pts',(-21.2134905199345,-10.371727699113,
12.));
#198207=CARTESIAN_POINT('Ctrl Pts',(-21.199520887919,-10.3586030124587,
0.));
#198208=CARTESIAN_POINT('Ctrl Pts',(-21.199520887919,-10.3586030124587,
12.));
#198209=CARTESIAN_POINT('Ctrl Pts',(-21.1855999722416,-10.34559612657,0.));
#198210=CARTESIAN_POINT('Ctrl Pts',(-21.1855999722416,-10.34559612657,12.));
#198211=CARTESIAN_POINT('Ctrl Pts',(-21.1717288370509,-10.3327073641572,
0.));
#198212=CARTESIAN_POINT('Ctrl Pts',(-21.1717288370509,-10.3327073641572,
12.));
#198213=CARTESIAN_POINT('Ctrl Pts',(-21.1579085619965,-10.3199370506544,
0.));
#198214=CARTESIAN_POINT('Ctrl Pts',(-21.1579085619965,-10.3199370506544,
12.));
#198215=CARTESIAN_POINT('Ctrl Pts',(-21.1441402425843,-10.3072855142687,
0.));
#198216=CARTESIAN_POINT('Ctrl Pts',(-21.1441402425843,-10.3072855142687,
12.));
#198217=CARTESIAN_POINT('Ctrl Pts',(-21.1304249906002,-10.2947530860721,
0.));
#198218=CARTESIAN_POINT('Ctrl Pts',(-21.1304249906002,-10.2947530860721,
12.));
#198219=CARTESIAN_POINT('Ctrl Pts',(-21.1167639345631,-10.2823401001072,
0.));
#198220=CARTESIAN_POINT('Ctrl Pts',(-21.1167639345631,-10.2823401001072,
12.));
#198221=CARTESIAN_POINT('Ctrl Pts',(-21.1031582201627,-10.2700468934744,
0.));
#198222=CARTESIAN_POINT('Ctrl Pts',(-21.1031582201627,-10.2700468934744,
12.));
#198223=CARTESIAN_POINT('Ctrl Pts',(-21.0896090107063,-10.2578738064181,
0.));
#198224=CARTESIAN_POINT('Ctrl Pts',(-21.0896090107063,-10.2578738064181,
12.));
#198225=CARTESIAN_POINT('Ctrl Pts',(-21.0761174875445,-10.2458211823912,
0.));
#198226=CARTESIAN_POINT('Ctrl Pts',(-21.0761174875445,-10.2458211823912,
12.));
#198227=CARTESIAN_POINT('Ctrl Pts',(-21.0626848505663,-10.2338893681567,
0.));
#198228=CARTESIAN_POINT('Ctrl Pts',(-21.0626848505663,-10.2338893681567,
12.));
#198229=CARTESIAN_POINT('Ctrl Pts',(-21.0493123187483,-10.2220787139154,
0.));
#198230=CARTESIAN_POINT('Ctrl Pts',(-21.0493123187483,-10.2220787139154,
12.));
#198231=CARTESIAN_POINT('Ctrl Pts',(-21.0360011306815,-10.2103895734123,
0.));
#198232=CARTESIAN_POINT('Ctrl Pts',(-21.0360011306815,-10.2103895734123,
12.));
#198233=CARTESIAN_POINT('Ctrl Pts',(-21.0227525451107,-10.1988223040425,
0.));
#198234=CARTESIAN_POINT('Ctrl Pts',(-21.0227525451107,-10.1988223040425,
12.));
#198235=CARTESIAN_POINT('Ctrl Pts',(-21.0095678414486,-10.187377266936,
0.));
#198236=CARTESIAN_POINT('Ctrl Pts',(-21.0095678414486,-10.187377266936,
12.));
#198237=CARTESIAN_POINT('Ctrl Pts',(-20.9964483203686,-10.1760548270767,
0.));
#198238=CARTESIAN_POINT('Ctrl Pts',(-20.9964483203686,-10.1760548270767,
12.));
#198239=CARTESIAN_POINT('Ctrl Pts',(-20.9833953044736,-10.1648553534568,
0.));
#198240=CARTESIAN_POINT('Ctrl Pts',(-20.9833953044736,-10.1648553534568,
12.));
#198241=CARTESIAN_POINT('Ctrl Pts',(-20.9704101389369,-10.1537792192065,
0.));
#198242=CARTESIAN_POINT('Ctrl Pts',(-20.9704101389369,-10.1537792192065,
12.));
#198243=CARTESIAN_POINT('Ctrl Pts',(-20.9574941921591,-10.1428268017256,
0.));
#198244=CARTESIAN_POINT('Ctrl Pts',(-20.9574941921591,-10.1428268017256,
12.));
#198245=CARTESIAN_POINT('Ctrl Pts',(-20.9446488563933,-10.1319984827908,
0.));
#198246=CARTESIAN_POINT('Ctrl Pts',(-20.9446488563933,-10.1319984827908,
12.));
#198247=CARTESIAN_POINT('Ctrl Pts',(-20.9318755484734,-10.1212946487057,
0.));
#198248=CARTESIAN_POINT('Ctrl Pts',(-20.9318755484734,-10.1212946487057,
12.));
#198249=CARTESIAN_POINT('Ctrl Pts',(-20.919175710627,-10.1107156904836,
0.));
#198250=CARTESIAN_POINT('Ctrl Pts',(-20.919175710627,-10.1107156904836,
12.));
#198251=CARTESIAN_POINT('Ctrl Pts',(-20.9065508112557,-10.1002620040076,
0.));
#198252=CARTESIAN_POINT('Ctrl Pts',(-20.9065508112557,-10.1002620040076,
12.));
#198253=CARTESIAN_POINT('Ctrl Pts',(-20.894002345737,-10.0899339901915,
0.));
#198254=CARTESIAN_POINT('Ctrl Pts',(-20.894002345737,-10.0899339901915,
12.));
#198255=CARTESIAN_POINT('Ctrl Pts',(-20.881531837184,-10.0797320551154,
0.));
#198256=CARTESIAN_POINT('Ctrl Pts',(-20.881531837184,-10.0797320551154,
12.));
#198257=CARTESIAN_POINT('Ctrl Pts',(-20.86914083737,-10.0696566102218,0.));
#198258=CARTESIAN_POINT('Ctrl Pts',(-20.86914083737,-10.0696566102218,12.));
#198259=CARTESIAN_POINT('Ctrl Pts',(-20.8568309277316,-10.0597080725375,
0.));
#198260=CARTESIAN_POINT('Ctrl Pts',(-20.8568309277316,-10.0597080725375,
12.));
#198261=CARTESIAN_POINT('Ctrl Pts',(-20.8446037203402,-10.0498868648733,
0.));
#198262=CARTESIAN_POINT('Ctrl Pts',(-20.8446037203402,-10.0498868648733,
12.));
#198263=CARTESIAN_POINT('Ctrl Pts',(-20.8324608588909,-10.0401934160234,
0.));
#198264=CARTESIAN_POINT('Ctrl Pts',(-20.8324608588909,-10.0401934160234,
12.));
#198265=CARTESIAN_POINT('Ctrl Pts',(-20.8204040196602,-10.0306281609435,
0.));
#198266=CARTESIAN_POINT('Ctrl Pts',(-20.8204040196602,-10.0306281609435,
12.));
#198267=CARTESIAN_POINT('Ctrl Pts',(-20.8084349126888,-10.0211915410095,
0.));
#198268=CARTESIAN_POINT('Ctrl Pts',(-20.8084349126888,-10.0211915410095,
12.));
#198269=CARTESIAN_POINT('Ctrl Pts',(-20.7965552829908,-10.0118840042786,
0.));
#198270=CARTESIAN_POINT('Ctrl Pts',(-20.7965552829908,-10.0118840042786,
12.));
#198271=CARTESIAN_POINT('Ctrl Pts',(-20.7847669117568,-10.0027060057389,
0.));
#198272=CARTESIAN_POINT('Ctrl Pts',(-20.7847669117568,-10.0027060057389,
12.));
#198273=CARTESIAN_POINT('Ctrl Pts',(-20.7730716175417,-9.9936580075464,
0.));
#198274=CARTESIAN_POINT('Ctrl Pts',(-20.7730716175417,-9.9936580075464,
12.));
#198275=CARTESIAN_POINT('Ctrl Pts',(-20.761471257499,-9.98474047926852,
0.));
#198276=CARTESIAN_POINT('Ctrl Pts',(-20.761471257499,-9.98474047926852,
12.));
#198277=CARTESIAN_POINT('Ctrl Pts',(-20.7499677289627,-9.9759538982347,
0.));
#198278=CARTESIAN_POINT('Ctrl Pts',(-20.7499677289627,-9.9759538982347,
12.));
#198279=CARTESIAN_POINT('Ctrl Pts',(-20.7385629709795,-9.96729874986201,
0.));
#198280=CARTESIAN_POINT('Ctrl Pts',(-20.7385629709795,-9.96729874986201,
12.));
#198281=CARTESIAN_POINT('Ctrl Pts',(-20.7272589658751,-9.95877552798397,
0.));
#198282=CARTESIAN_POINT('Ctrl Pts',(-20.7272589658751,-9.95877552798397,
12.));
#198283=CARTESIAN_POINT('Ctrl Pts',(-20.7160577407579,-9.95038473514948,
0.));
#198284=CARTESIAN_POINT('Ctrl Pts',(-20.7160577407579,-9.95038473514948,
12.));
#198285=CARTESIAN_POINT('Ctrl Pts',(-20.7049613692234,-9.94212688298236,
0.));
#198286=CARTESIAN_POINT('Ctrl Pts',(-20.7049613692234,-9.94212688298236,
12.));
#198287=CARTESIAN_POINT('Ctrl Pts',(-20.6939719732484,-9.93400249259729,
0.));
#198288=CARTESIAN_POINT('Ctrl Pts',(-20.6939719732484,-9.93400249259729,
12.));
#198289=CARTESIAN_POINT('Ctrl Pts',(-20.6830917250255,-9.92601209498748,
0.));
#198290=CARTESIAN_POINT('Ctrl Pts',(-20.6830917250255,-9.92601209498748,
12.));
#198291=CARTESIAN_POINT('Ctrl Pts',(-20.6723228488263,-9.91815623141288,
0.));
#198292=CARTESIAN_POINT('Ctrl Pts',(-20.6723228488263,-9.91815623141288,
12.));
#198293=CARTESIAN_POINT('Ctrl Pts',(-20.6616676228315,-9.91043545377007,
0.));
#198294=CARTESIAN_POINT('Ctrl Pts',(-20.6616676228315,-9.91043545377007,
12.));
#198295=CARTESIAN_POINT('Ctrl Pts',(-20.6511283817414,-9.90285032516692,
0.));
#198296=CARTESIAN_POINT('Ctrl Pts',(-20.6511283817414,-9.90285032516692,
12.));
#198297=CARTESIAN_POINT('Ctrl Pts',(-20.6407075193976,-9.89540142049119,
0.));
#198298=CARTESIAN_POINT('Ctrl Pts',(-20.6407075193976,-9.89540142049119,
12.));
#198299=CARTESIAN_POINT('Ctrl Pts',(-20.6304074914087,-9.88808932697306,
0.));
#198300=CARTESIAN_POINT('Ctrl Pts',(-20.6304074914087,-9.88808932697306,
12.));
#198301=CARTESIAN_POINT('Ctrl Pts',(-20.6202308177474,-9.88091464472675,
0.));
#198302=CARTESIAN_POINT('Ctrl Pts',(-20.6202308177474,-9.88091464472675,
12.));
#198303=CARTESIAN_POINT('Ctrl Pts',(-20.6101800854494,-9.87387798732956,
0.));
#198304=CARTESIAN_POINT('Ctrl Pts',(-20.6101800854494,-9.87387798732956,
12.));
#198305=CARTESIAN_POINT('Ctrl Pts',(-20.6002579513699,-9.86697998242622,
0.));
#198306=CARTESIAN_POINT('Ctrl Pts',(-20.6002579513699,-9.86697998242622,
12.));
#198307=CARTESIAN_POINT('Ctrl Pts',(-20.5904671449754,-9.86022127232747,
0.));
#198308=CARTESIAN_POINT('Ctrl Pts',(-20.5904671449754,-9.86022127232747,
12.));
#198309=CARTESIAN_POINT('Ctrl Pts',(-20.5808104710015,-9.8536025145698,
0.));
#198310=CARTESIAN_POINT('Ctrl Pts',(-20.5808104710015,-9.8536025145698,
12.));
#198311=CARTESIAN_POINT('Ctrl Pts',(-20.5712908125139,-9.84712438256277,
0.));
#198312=CARTESIAN_POINT('Ctrl Pts',(-20.5712908125139,-9.84712438256277,
12.));
#198313=CARTESIAN_POINT('Ctrl Pts',(-20.5619111362402,-9.84078756677565,
0.));
#198314=CARTESIAN_POINT('Ctrl Pts',(-20.5619111362402,-9.84078756677565,
12.));
#198315=CARTESIAN_POINT('Ctrl Pts',(-20.552674497646,-9.83459277585315,
0.));
#198316=CARTESIAN_POINT('Ctrl Pts',(-20.552674497646,-9.83459277585315,
12.));
#198317=CARTESIAN_POINT('Ctrl Pts',(-20.5435840460721,-9.82854073773877,
0.));
#198318=CARTESIAN_POINT('Ctrl Pts',(-20.5435840460721,-9.82854073773877,
12.));
#198319=CARTESIAN_POINT('Ctrl Pts',(-20.5346430299517,-9.82263220080362,
0.));
#198320=CARTESIAN_POINT('Ctrl Pts',(-20.5346430299517,-9.82263220080362,
12.));
#198321=CARTESIAN_POINT('Ctrl Pts',(-20.5258548000629,-9.81686793455942,
0.));
#198322=CARTESIAN_POINT('Ctrl Pts',(-20.5258548000629,-9.81686793455942,
12.));
#198323=CARTESIAN_POINT('Ctrl Pts',(-20.517222812284,-9.81124873025281,
0.));
#198324=CARTESIAN_POINT('Ctrl Pts',(-20.517222812284,-9.81124873025281,
12.));
#198325=CARTESIAN_POINT('Ctrl Pts',(-20.5087506310505,-9.80577540161087,
0.));
#198326=CARTESIAN_POINT('Ctrl Pts',(-20.5087506310505,-9.80577540161087,
12.));
#198327=CARTESIAN_POINT('Ctrl Pts',(-20.5004419312107,-9.80044878520948,
0.));
#198328=CARTESIAN_POINT('Ctrl Pts',(-20.5004419312107,-9.80044878520948,
12.));
#198329=CARTESIAN_POINT('Ctrl Pts',(-20.4923005087943,-9.7952697428833,
0.));
#198330=CARTESIAN_POINT('Ctrl Pts',(-20.4923005087943,-9.7952697428833,
12.));
#198331=CARTESIAN_POINT('Ctrl Pts',(-20.4843302955329,-9.79023916498655,
0.));
#198332=CARTESIAN_POINT('Ctrl Pts',(-20.4843302955329,-9.79023916498655,
12.));
#198333=CARTESIAN_POINT('Ctrl Pts',(-20.4765353711586,-9.78535797314166,
0.));
#198334=CARTESIAN_POINT('Ctrl Pts',(-20.4765353711586,-9.78535797314166,
12.));
#198335=CARTESIAN_POINT('Ctrl Pts',(-20.4689199790669,-9.7806271237332,
0.));
#198336=CARTESIAN_POINT('Ctrl Pts',(-20.4689199790669,-9.7806271237332,
12.));
#198337=CARTESIAN_POINT('Ctrl Pts',(-20.4614885274975,-9.77604760815528,
0.));
#198338=CARTESIAN_POINT('Ctrl Pts',(-20.4614885274975,-9.77604760815528,
12.));
#198339=CARTESIAN_POINT('Ctrl Pts',(-20.4542455817527,-9.77162045104069,
0.));
#198340=CARTESIAN_POINT('Ctrl Pts',(-20.4542455817527,-9.77162045104069,
12.));
#198341=CARTESIAN_POINT('Ctrl Pts',(-20.447195862298,-9.76734670980891,
0.));
#198342=CARTESIAN_POINT('Ctrl Pts',(-20.447195862298,-9.76734670980891,
12.));
#198343=CARTESIAN_POINT('Ctrl Pts',(-20.44034423294,-9.76322747195494,0.));
#198344=CARTESIAN_POINT('Ctrl Pts',(-20.44034423294,-9.76322747195494,12.));
#198345=CARTESIAN_POINT('Ctrl Pts',(-20.4336957355473,-9.75926386289922,
0.));
#198346=CARTESIAN_POINT('Ctrl Pts',(-20.4336957355473,-9.75926386289922,
12.));
#198347=CARTESIAN_POINT('Ctrl Pts',(-20.4272556476629,-9.75545705902417,
0.));
#198348=CARTESIAN_POINT('Ctrl Pts',(-20.4272556476629,-9.75545705902417,
12.));
#198349=CARTESIAN_POINT('Ctrl Pts',(-20.4210295275817,-9.7518082978643,
0.));
#198350=CARTESIAN_POINT('Ctrl Pts',(-20.4210295275817,-9.7518082978643,
12.));
#198351=CARTESIAN_POINT('Ctrl Pts',(-20.4150232777393,-9.74831889242174,
0.));
#198352=CARTESIAN_POINT('Ctrl Pts',(-20.4150232777393,-9.74831889242174,
12.));
#198353=CARTESIAN_POINT('Ctrl Pts',(-20.4092430879861,-9.74499021838537,
0.));
#198354=CARTESIAN_POINT('Ctrl Pts',(-20.4092430879861,-9.74499021838537,
12.));
#198355=CARTESIAN_POINT('Ctrl Pts',(-20.4036953576549,-9.74182369656271,
0.));
#198356=CARTESIAN_POINT('Ctrl Pts',(-20.4036953576549,-9.74182369656271,
12.));
#198357=CARTESIAN_POINT('Ctrl Pts',(-20.3983866213331,-9.738820776132,0.));
#198358=CARTESIAN_POINT('Ctrl Pts',(-20.3983866213331,-9.738820776132,12.));
#198359=CARTESIAN_POINT('Ctrl Pts',(-20.3933234845647,-9.73598292014242,
0.));
#198360=CARTESIAN_POINT('Ctrl Pts',(-20.3933234845647,-9.73598292014242,
12.));
#198361=CARTESIAN_POINT('Ctrl Pts',(-20.3885129129912,-9.73331167102807,
0.));
#198362=CARTESIAN_POINT('Ctrl Pts',(-20.3885129129912,-9.73331167102807,
12.));
#198363=CARTESIAN_POINT('Ctrl Pts',(-20.3839624556742,-9.73080870123727,
0.));
#198364=CARTESIAN_POINT('Ctrl Pts',(-20.3839624556742,-9.73080870123727,
12.));
#198365=CARTESIAN_POINT('Ctrl Pts',(-20.3796805893304,-9.72847589116541,
0.));
#198366=CARTESIAN_POINT('Ctrl Pts',(-20.3796805893304,-9.72847589116541,
12.));
#198367=CARTESIAN_POINT('Ctrl Pts',(-20.3756766651951,-9.7263153173288,
0.));
#198368=CARTESIAN_POINT('Ctrl Pts',(-20.3756766651951,-9.7263153173288,
12.));
#198369=CARTESIAN_POINT('Ctrl Pts',(-20.371960235676,-9.72432910043194,
0.));
#198370=CARTESIAN_POINT('Ctrl Pts',(-20.371960235676,-9.72432910043194,
12.));
#198371=CARTESIAN_POINT('Ctrl Pts',(-20.3685406190576,-9.72251930722489,
0.));
#198372=CARTESIAN_POINT('Ctrl Pts',(-20.3685406190576,-9.72251930722489,
12.));
#198373=CARTESIAN_POINT('Ctrl Pts',(-20.3654261611056,-9.7208877838108,
0.));
#198374=CARTESIAN_POINT('Ctrl Pts',(-20.3654261611056,-9.7208877838108,
12.));
#198375=CARTESIAN_POINT('Ctrl Pts',(-20.3626256913981,-9.71943648548099,
0.));
#198376=CARTESIAN_POINT('Ctrl Pts',(-20.3626256913981,-9.71943648548099,
12.));
#198377=CARTESIAN_POINT('Ctrl Pts',(-20.3601498764344,-9.71816778328006,
0.));
#198378=CARTESIAN_POINT('Ctrl Pts',(-20.3601498764344,-9.71816778328006,
12.));
#198379=CARTESIAN_POINT('Ctrl Pts',(-20.3580133103356,-9.71708493723096,
0.));
#198380=CARTESIAN_POINT('Ctrl Pts',(-20.3580133103356,-9.71708493723096,
12.));
#198381=CARTESIAN_POINT('Ctrl Pts',(-20.3562337557875,-9.71619192554185,
0.));
#198382=CARTESIAN_POINT('Ctrl Pts',(-20.3562337557875,-9.71619192554185,
12.));
#198383=CARTESIAN_POINT('Ctrl Pts',(-20.3548282742361,-9.71549257088172,
0.));
#198384=CARTESIAN_POINT('Ctrl Pts',(-20.3548282742361,-9.71549257088172,
12.));
#198385=CARTESIAN_POINT('Ctrl Pts',(-20.3538098605706,-9.7149897805202,
0.));
#198386=CARTESIAN_POINT('Ctrl Pts',(-20.3538098605706,-9.7149897805202,
12.));
#198387=CARTESIAN_POINT('Ctrl Pts',(-20.3533097561886,-9.7147459035068,
0.));
#198388=CARTESIAN_POINT('Ctrl Pts',(-20.3533097561886,-9.7147459035068,
12.));
#198389=CARTESIAN_POINT('Ctrl Pts',(-20.3531126095522,-9.71465227853041,
0.));
#198390=CARTESIAN_POINT('Ctrl Pts',(-20.3531126095522,-9.71465227853041,
12.));
#198391=CARTESIAN_POINT('Ctrl Pts',(-20.353060251684,-9.71462954053041,
0.));
#198392=CARTESIAN_POINT('Ctrl Pts',(-20.353060251684,-9.71462954053041,
12.));
#198393=CARTESIAN_POINT('Ctrl Pts',(-20.353053841303,-9.71462809124915,
0.));
#198394=CARTESIAN_POINT('Ctrl Pts',(-20.353053841303,-9.71462809124915,
12.));
#198395=CARTESIAN_POINT('',(-22.8400320311649,-12.4230808101438,0.));
#198396=CARTESIAN_POINT('Ctrl Pts',(-22.8400320311649,-12.4230808101438,
0.));
#198397=CARTESIAN_POINT('Ctrl Pts',(-22.8370364396459,-12.418215285186,
0.));
#198398=CARTESIAN_POINT('Ctrl Pts',(-22.8310435872748,-12.4084933766346,
0.));
#198399=CARTESIAN_POINT('Ctrl Pts',(-22.8220493007173,-12.3939379378998,
0.));
#198400=CARTESIAN_POINT('Ctrl Pts',(-22.81004690224,-12.374585536673,0.));
#198401=CARTESIAN_POINT('Ctrl Pts',(-22.795027221673,-12.3504864740319,
0.));
#198402=CARTESIAN_POINT('Ctrl Pts',(-22.7799908974768,-12.3264788926075,
0.));
#198403=CARTESIAN_POINT('Ctrl Pts',(-22.764938010105,-12.3025628601792,
0.));
#198404=CARTESIAN_POINT('Ctrl Pts',(-22.7498686970069,-12.2787384750742,
0.));
#198405=CARTESIAN_POINT('Ctrl Pts',(-22.7347831655287,-12.2550058702395,
0.));
#198406=CARTESIAN_POINT('Ctrl Pts',(-22.7196817119374,-12.2313652198061,
0.));
#198407=CARTESIAN_POINT('Ctrl Pts',(-22.7045647168747,-12.2078167360284,
0.));
#198408=CARTESIAN_POINT('Ctrl Pts',(-22.6894326205037,-12.1843606579261,
0.));
#198409=CARTESIAN_POINT('Ctrl Pts',(-22.6742859034944,-12.1609972423099,
0.));
#198410=CARTESIAN_POINT('Ctrl Pts',(-22.6591250653965,-12.1377267537145,
0.));
#198411=CARTESIAN_POINT('Ctrl Pts',(-22.6439506046605,-12.1145494550383,
0.));
#198412=CARTESIAN_POINT('Ctrl Pts',(-22.6287629967056,-12.0914655972823,
0.));
#198413=CARTESIAN_POINT('Ctrl Pts',(-22.6135626764898,-12.0684754113862,
0.));
#198414=CARTESIAN_POINT('Ctrl Pts',(-22.5983500505644,-12.0455791139128,
0.));
#198415=CARTESIAN_POINT('Ctrl Pts',(-22.5831255061282,-12.0227769113127,
0.));
#198416=CARTESIAN_POINT('Ctrl Pts',(-22.5678894211181,-12.0000690046695,
0.));
#198417=CARTESIAN_POINT('Ctrl Pts',(-22.5526421741158,-11.9774555943496,
0.));
#198418=CARTESIAN_POINT('Ctrl Pts',(-22.5373841537307,-11.9549368843997,
0.));
#198419=CARTESIAN_POINT('Ctrl Pts',(-22.5221157697883,-11.9325130877803,
0.));
#198420=CARTESIAN_POINT('Ctrl Pts',(-22.5068374513973,-11.9101844254557,
0.));
#198421=CARTESIAN_POINT('Ctrl Pts',(-22.4915496418485,-11.8879511239942,
0.));
#198422=CARTESIAN_POINT('Ctrl Pts',(-22.4762527946702,-11.8658134137019,
0.));
#198423=CARTESIAN_POINT('Ctrl Pts',(-22.4609473690471,-11.8437715264487,
0.));
#198424=CARTESIAN_POINT('Ctrl Pts',(-22.4456338258735,-11.8218256937889,
0.));
#198425=CARTESIAN_POINT('Ctrl Pts',(-22.430312622646,-11.7999761445173,
0.));
#198426=CARTESIAN_POINT('Ctrl Pts',(-22.4149842125008,-11.7782231042039,
0.));
#198427=CARTESIAN_POINT('Ctrl Pts',(-22.3996490469191,-11.7565667964764,
0.));
#198428=CARTESIAN_POINT('Ctrl Pts',(-22.3843075773899,-11.7350074437961,
0.));
#198429=CARTESIAN_POINT('Ctrl Pts',(-22.3689602575491,-11.7135452684532,
0.));
#198430=CARTESIAN_POINT('Ctrl Pts',(-22.3536075450029,-11.6921804934056,
0.));
#198431=CARTESIAN_POINT('Ctrl Pts',(-22.3382499035619,-11.6709133432985,
0.));
#198432=CARTESIAN_POINT('Ctrl Pts',(-22.3228878043976,-11.6497440449857,
0.));
#198433=CARTESIAN_POINT('Ctrl Pts',(-22.3075217249049,-11.6286728270009,
0.));
#198434=CARTESIAN_POINT('Ctrl Pts',(-22.2921521480356,-11.6076999192357,
0.));
#198435=CARTESIAN_POINT('Ctrl Pts',(-22.2767795614348,-11.5868255525188,
0.));
#198436=CARTESIAN_POINT('Ctrl Pts',(-22.2614044566898,-11.5660499582403,
0.));
#198437=CARTESIAN_POINT('Ctrl Pts',(-22.2460273284654,-11.5453733679121,
0.));
#198438=CARTESIAN_POINT('Ctrl Pts',(-22.2306486738901,-11.5247960128477,
0.));
#198439=CARTESIAN_POINT('Ctrl Pts',(-22.2152689931022,-11.5043181244242,
0.));
#198440=CARTESIAN_POINT('Ctrl Pts',(-22.1998887896436,-11.483939934259,
0.));
#198441=CARTESIAN_POINT('Ctrl Pts',(-22.184508570917,-11.463661674411,0.));
#198442=CARTESIAN_POINT('Ctrl Pts',(-22.1691288486096,-11.443483577557,
0.));
#198443=CARTESIAN_POINT('Ctrl Pts',(-22.1537501391487,-11.4234058771742,
0.));
#198444=CARTESIAN_POINT('Ctrl Pts',(-22.1383729640964,-11.4034288076908,
0.));
#198445=CARTESIAN_POINT('Ctrl Pts',(-22.1229978500186,-11.3835526044256,
0.));
#198446=CARTESIAN_POINT('Ctrl Pts',(-22.1076253283979,-11.3637775035367,
0.));
#198447=CARTESIAN_POINT('Ctrl Pts',(-22.0922559355294,-11.3441037419553,
0.));
#198448=CARTESIAN_POINT('Ctrl Pts',(-22.0768902124267,-11.3245315573168,
0.));
#198449=CARTESIAN_POINT('Ctrl Pts',(-22.0615287047179,-11.3050611878771,
0.));
#198450=CARTESIAN_POINT('Ctrl Pts',(-22.046171962566,-11.2856928724374,
0.));
#198451=CARTESIAN_POINT('Ctrl Pts',(-22.030820540835,-11.2664268504206,
0.));
#198452=CARTESIAN_POINT('Ctrl Pts',(-22.0154749992363,-11.2472633619275,
0.));
#198453=CARTESIAN_POINT('Ctrl Pts',(-22.0001359024839,-11.2282026477896,
0.));
#198454=CARTESIAN_POINT('Ctrl Pts',(-21.9848038204439,-11.2092449496125,
0.));
#198455=CARTESIAN_POINT('Ctrl Pts',(-21.9694793282914,-11.190390509811,
0.));
#198456=CARTESIAN_POINT('Ctrl Pts',(-21.9541630066506,-11.1716395716376,
0.));
#198457=CARTESIAN_POINT('Ctrl Pts',(-21.9388554416439,-11.1529923792003,
0.));
#198458=CARTESIAN_POINT('Ctrl Pts',(-21.923557224952,-11.1344491774741,
0.));
#198459=CARTESIAN_POINT('Ctrl Pts',(-21.9082689538688,-11.1160102123024,
0.));
#198460=CARTESIAN_POINT('Ctrl Pts',(-21.8929912313608,-11.0976757303944,
0.));
#198461=CARTESIAN_POINT('Ctrl Pts',(-21.877724666119,-11.0794459793057,
0.));
#198462=CARTESIAN_POINT('Ctrl Pts',(-21.8624698726318,-11.0613212074363,
0.));
#198463=CARTESIAN_POINT('Ctrl Pts',(-21.8472274713103,-11.0433016640807,
0.));
#198464=CARTESIAN_POINT('Ctrl Pts',(-21.8319980886033,-11.0253875994598,
0.));
#198465=CARTESIAN_POINT('Ctrl Pts',(-21.8167823571168,-11.0075792647477,
0.));
#198466=CARTESIAN_POINT('Ctrl Pts',(-21.8015809157301,-10.9898769120912,
0.));
#198467=CARTESIAN_POINT('Ctrl Pts',(-21.7863944097141,-10.9722807946155,
0.));
#198468=CARTESIAN_POINT('Ctrl Pts',(-21.7712234908464,-10.9547911664455,
0.));
#198469=CARTESIAN_POINT('Ctrl Pts',(-21.7560688175247,-10.9374082827444,
0.));
#198470=CARTESIAN_POINT('Ctrl Pts',(-21.7409310548797,-10.9201323997384,
0.));
#198471=CARTESIAN_POINT('Ctrl Pts',(-21.7258108748873,-10.902963774734,
0.));
#198472=CARTESIAN_POINT('Ctrl Pts',(-21.7107089564825,-10.8859026661293,
0.));
#198473=CARTESIAN_POINT('Ctrl Pts',(-21.6956259856672,-10.8689493334095,
0.));
#198474=CARTESIAN_POINT('Ctrl Pts',(-21.6805626556467,-10.8521040371835,
0.));
#198475=CARTESIAN_POINT('Ctrl Pts',(-21.6655196669732,-10.8353670392272,
0.));
#198476=CARTESIAN_POINT('Ctrl Pts',(-21.6504977276866,-10.8187386025136,
0.));
#198477=CARTESIAN_POINT('Ctrl Pts',(-21.6354975534557,-10.8022189912369,
0.));
#198478=CARTESIAN_POINT('Ctrl Pts',(-21.6205198677173,-10.7858084708261,
0.));
#198479=CARTESIAN_POINT('Ctrl Pts',(-21.6055654018176,-10.7695073079552,
0.));
#198480=CARTESIAN_POINT('Ctrl Pts',(-21.5906348951743,-10.7533157705941,
0.));
#198481=CARTESIAN_POINT('Ctrl Pts',(-21.5757290954371,-10.7372341280467,
0.));
#198482=CARTESIAN_POINT('Ctrl Pts',(-21.5608487586468,-10.7212626509816,
0.));
#198483=CARTESIAN_POINT('Ctrl Pts',(-21.5459946493955,-10.7054016114571,
0.));
#198484=CARTESIAN_POINT('Ctrl Pts',(-21.5311675409807,-10.689651282929,
0.));
#198485=CARTESIAN_POINT('Ctrl Pts',(-21.51636821558,-10.6740119402834,0.));
#198486=CARTESIAN_POINT('Ctrl Pts',(-21.5015974644449,-10.6584838598939,
0.));
#198487=CARTESIAN_POINT('Ctrl Pts',(-21.4868560880889,-10.6430673196607,
0.));
#198488=CARTESIAN_POINT('Ctrl Pts',(-21.4721448964766,-10.6277625990456,
0.));
#198489=CARTESIAN_POINT('Ctrl Pts',(-21.4574647092097,-10.6125699790961,
0.));
#198490=CARTESIAN_POINT('Ctrl Pts',(-21.4428163557144,-10.5974897424622,
0.));
#198491=CARTESIAN_POINT('Ctrl Pts',(-21.4282006754631,-10.5825221734573,
0.));
#198492=CARTESIAN_POINT('Ctrl Pts',(-21.4136185181979,-10.5676675581108,
0.));
#198493=CARTESIAN_POINT('Ctrl Pts',(-21.3990707441497,-10.5529261842108,
0.));
#198494=CARTESIAN_POINT('Ctrl Pts',(-21.3845582242602,-10.5382983413421,
0.));
#198495=CARTESIAN_POINT('Ctrl Pts',(-21.3700818403936,-10.5237843209057,
0.));
#198496=CARTESIAN_POINT('Ctrl Pts',(-21.3556424855814,-10.5093844161685,
0.));
#198497=CARTESIAN_POINT('Ctrl Pts',(-21.3412410642904,-10.4950989223337,
0.));
#198498=CARTESIAN_POINT('Ctrl Pts',(-21.3268784926819,-10.4809281365931,
0.));
#198499=CARTESIAN_POINT('Ctrl Pts',(-21.3125556988731,-10.4668723581768,
0.));
#198500=CARTESIAN_POINT('Ctrl Pts',(-21.2982736231931,-10.4529318883874,
0.));
#198501=CARTESIAN_POINT('Ctrl Pts',(-21.2840332184483,-10.4391070306391,
0.));
#198502=CARTESIAN_POINT('Ctrl Pts',(-21.2698354502403,-10.42539809054,0.));
#198503=CARTESIAN_POINT('Ctrl Pts',(-21.255681297275,-10.4118053759588,
0.));
#198504=CARTESIAN_POINT('Ctrl Pts',(-21.2415717516714,-10.3983291970846,
0.));
#198505=CARTESIAN_POINT('Ctrl Pts',(-21.22750781927,-10.3849698664786,0.));
#198506=CARTESIAN_POINT('Ctrl Pts',(-21.2134905199345,-10.371727699113,
0.));
#198507=CARTESIAN_POINT('Ctrl Pts',(-21.199520887919,-10.3586030124587,
0.));
#198508=CARTESIAN_POINT('Ctrl Pts',(-21.1855999722416,-10.34559612657,0.));
#198509=CARTESIAN_POINT('Ctrl Pts',(-21.1717288370509,-10.3327073641572,
0.));
#198510=CARTESIAN_POINT('Ctrl Pts',(-21.1579085619965,-10.3199370506544,
0.));
#198511=CARTESIAN_POINT('Ctrl Pts',(-21.1441402425843,-10.3072855142687,
0.));
#198512=CARTESIAN_POINT('Ctrl Pts',(-21.1304249906002,-10.2947530860721,
0.));
#198513=CARTESIAN_POINT('Ctrl Pts',(-21.1167639345631,-10.2823401001072,
0.));
#198514=CARTESIAN_POINT('Ctrl Pts',(-21.1031582201627,-10.2700468934744,
0.));
#198515=CARTESIAN_POINT('Ctrl Pts',(-21.0896090107063,-10.2578738064181,
0.));
#198516=CARTESIAN_POINT('Ctrl Pts',(-21.0761174875445,-10.2458211823912,
0.));
#198517=CARTESIAN_POINT('Ctrl Pts',(-21.0626848505663,-10.2338893681567,
0.));
#198518=CARTESIAN_POINT('Ctrl Pts',(-21.0493123187483,-10.2220787139154,
0.));
#198519=CARTESIAN_POINT('Ctrl Pts',(-21.0360011306815,-10.2103895734123,
0.));
#198520=CARTESIAN_POINT('Ctrl Pts',(-21.0227525451107,-10.1988223040425,
0.));
#198521=CARTESIAN_POINT('Ctrl Pts',(-21.0095678414486,-10.187377266936,
0.));
#198522=CARTESIAN_POINT('Ctrl Pts',(-20.9964483203686,-10.1760548270767,
0.));
#198523=CARTESIAN_POINT('Ctrl Pts',(-20.9833953044736,-10.1648553534568,
0.));
#198524=CARTESIAN_POINT('Ctrl Pts',(-20.9704101389369,-10.1537792192065,
0.));
#198525=CARTESIAN_POINT('Ctrl Pts',(-20.9574941921591,-10.1428268017256,
0.));
#198526=CARTESIAN_POINT('Ctrl Pts',(-20.9446488563933,-10.1319984827908,
0.));
#198527=CARTESIAN_POINT('Ctrl Pts',(-20.9318755484734,-10.1212946487057,
0.));
#198528=CARTESIAN_POINT('Ctrl Pts',(-20.919175710627,-10.1107156904836,
0.));
#198529=CARTESIAN_POINT('Ctrl Pts',(-20.9065508112557,-10.1002620040076,
0.));
#198530=CARTESIAN_POINT('Ctrl Pts',(-20.894002345737,-10.0899339901915,
0.));
#198531=CARTESIAN_POINT('Ctrl Pts',(-20.881531837184,-10.0797320551154,
0.));
#198532=CARTESIAN_POINT('Ctrl Pts',(-20.86914083737,-10.0696566102218,0.));
#198533=CARTESIAN_POINT('Ctrl Pts',(-20.8568309277316,-10.0597080725375,
0.));
#198534=CARTESIAN_POINT('Ctrl Pts',(-20.8446037203402,-10.0498868648733,
0.));
#198535=CARTESIAN_POINT('Ctrl Pts',(-20.8324608588909,-10.0401934160234,
0.));
#198536=CARTESIAN_POINT('Ctrl Pts',(-20.8204040196602,-10.0306281609435,
0.));
#198537=CARTESIAN_POINT('Ctrl Pts',(-20.8084349126888,-10.0211915410095,
0.));
#198538=CARTESIAN_POINT('Ctrl Pts',(-20.7965552829908,-10.0118840042786,
0.));
#198539=CARTESIAN_POINT('Ctrl Pts',(-20.7847669117568,-10.0027060057389,
0.));
#198540=CARTESIAN_POINT('Ctrl Pts',(-20.7730716175417,-9.9936580075464,
0.));
#198541=CARTESIAN_POINT('Ctrl Pts',(-20.761471257499,-9.98474047926852,
0.));
#198542=CARTESIAN_POINT('Ctrl Pts',(-20.7499677289627,-9.9759538982347,
0.));
#198543=CARTESIAN_POINT('Ctrl Pts',(-20.7385629709795,-9.96729874986201,
0.));
#198544=CARTESIAN_POINT('Ctrl Pts',(-20.7272589658751,-9.95877552798397,
0.));
#198545=CARTESIAN_POINT('Ctrl Pts',(-20.7160577407579,-9.95038473514948,
0.));
#198546=CARTESIAN_POINT('Ctrl Pts',(-20.7049613692234,-9.94212688298236,
0.));
#198547=CARTESIAN_POINT('Ctrl Pts',(-20.6939719732484,-9.93400249259729,
0.));
#198548=CARTESIAN_POINT('Ctrl Pts',(-20.6830917250255,-9.92601209498748,
0.));
#198549=CARTESIAN_POINT('Ctrl Pts',(-20.6723228488263,-9.91815623141288,
0.));
#198550=CARTESIAN_POINT('Ctrl Pts',(-20.6616676228315,-9.91043545377007,
0.));
#198551=CARTESIAN_POINT('Ctrl Pts',(-20.6511283817414,-9.90285032516692,
0.));
#198552=CARTESIAN_POINT('Ctrl Pts',(-20.6407075193976,-9.89540142049119,
0.));
#198553=CARTESIAN_POINT('Ctrl Pts',(-20.6304074914087,-9.88808932697306,
0.));
#198554=CARTESIAN_POINT('Ctrl Pts',(-20.6202308177474,-9.88091464472675,
0.));
#198555=CARTESIAN_POINT('Ctrl Pts',(-20.6101800854494,-9.87387798732956,
0.));
#198556=CARTESIAN_POINT('Ctrl Pts',(-20.6002579513699,-9.86697998242622,
0.));
#198557=CARTESIAN_POINT('Ctrl Pts',(-20.5904671449754,-9.86022127232747,
0.));
#198558=CARTESIAN_POINT('Ctrl Pts',(-20.5808104710015,-9.8536025145698,
0.));
#198559=CARTESIAN_POINT('Ctrl Pts',(-20.5712908125139,-9.84712438256277,
0.));
#198560=CARTESIAN_POINT('Ctrl Pts',(-20.5619111362402,-9.84078756677565,
0.));
#198561=CARTESIAN_POINT('Ctrl Pts',(-20.552674497646,-9.83459277585315,
0.));
#198562=CARTESIAN_POINT('Ctrl Pts',(-20.5435840460721,-9.82854073773877,
0.));
#198563=CARTESIAN_POINT('Ctrl Pts',(-20.5346430299517,-9.82263220080362,
0.));
#198564=CARTESIAN_POINT('Ctrl Pts',(-20.5258548000629,-9.81686793455942,
0.));
#198565=CARTESIAN_POINT('Ctrl Pts',(-20.517222812284,-9.81124873025281,
0.));
#198566=CARTESIAN_POINT('Ctrl Pts',(-20.5087506310505,-9.80577540161087,
0.));
#198567=CARTESIAN_POINT('Ctrl Pts',(-20.5004419312107,-9.80044878520948,
0.));
#198568=CARTESIAN_POINT('Ctrl Pts',(-20.4923005087943,-9.7952697428833,
0.));
#198569=CARTESIAN_POINT('Ctrl Pts',(-20.4843302955329,-9.79023916498655,
0.));
#198570=CARTESIAN_POINT('Ctrl Pts',(-20.4765353711586,-9.78535797314166,
0.));
#198571=CARTESIAN_POINT('Ctrl Pts',(-20.4689199790669,-9.7806271237332,
0.));
#198572=CARTESIAN_POINT('Ctrl Pts',(-20.4614885274975,-9.77604760815528,
0.));
#198573=CARTESIAN_POINT('Ctrl Pts',(-20.4542455817527,-9.77162045104069,
0.));
#198574=CARTESIAN_POINT('Ctrl Pts',(-20.447195862298,-9.76734670980891,
0.));
#198575=CARTESIAN_POINT('Ctrl Pts',(-20.44034423294,-9.76322747195494,0.));
#198576=CARTESIAN_POINT('Ctrl Pts',(-20.4336957355473,-9.75926386289922,
0.));
#198577=CARTESIAN_POINT('Ctrl Pts',(-20.4272556476629,-9.75545705902417,
0.));
#198578=CARTESIAN_POINT('Ctrl Pts',(-20.4210295275817,-9.7518082978643,
0.));
#198579=CARTESIAN_POINT('Ctrl Pts',(-20.4150232777393,-9.74831889242174,
0.));
#198580=CARTESIAN_POINT('Ctrl Pts',(-20.4092430879861,-9.74499021838537,
0.));
#198581=CARTESIAN_POINT('Ctrl Pts',(-20.4036953576549,-9.74182369656271,
0.));
#198582=CARTESIAN_POINT('Ctrl Pts',(-20.3983866213331,-9.738820776132,0.));
#198583=CARTESIAN_POINT('Ctrl Pts',(-20.3933234845647,-9.73598292014242,
0.));
#198584=CARTESIAN_POINT('Ctrl Pts',(-20.3885129129912,-9.73331167102807,
0.));
#198585=CARTESIAN_POINT('Ctrl Pts',(-20.3839624556742,-9.73080870123727,
0.));
#198586=CARTESIAN_POINT('Ctrl Pts',(-20.3796805893304,-9.72847589116541,
0.));
#198587=CARTESIAN_POINT('Ctrl Pts',(-20.3756766651951,-9.7263153173288,
0.));
#198588=CARTESIAN_POINT('Ctrl Pts',(-20.371960235676,-9.72432910043194,
0.));
#198589=CARTESIAN_POINT('Ctrl Pts',(-20.3685406190576,-9.72251930722489,
0.));
#198590=CARTESIAN_POINT('Ctrl Pts',(-20.3654261611056,-9.7208877838108,
0.));
#198591=CARTESIAN_POINT('Ctrl Pts',(-20.3626256913981,-9.71943648548099,
0.));
#198592=CARTESIAN_POINT('Ctrl Pts',(-20.3601498764344,-9.71816778328006,
0.));
#198593=CARTESIAN_POINT('Ctrl Pts',(-20.3580133103356,-9.71708493723096,
0.));
#198594=CARTESIAN_POINT('Ctrl Pts',(-20.3562337557875,-9.71619192554185,
0.));
#198595=CARTESIAN_POINT('Ctrl Pts',(-20.3548282742361,-9.71549257088172,
0.));
#198596=CARTESIAN_POINT('Ctrl Pts',(-20.3538098605706,-9.7149897805202,
0.));
#198597=CARTESIAN_POINT('Ctrl Pts',(-20.3533097561886,-9.7147459035068,
0.));
#198598=CARTESIAN_POINT('Ctrl Pts',(-20.3531126095522,-9.71465227853041,
0.));
#198599=CARTESIAN_POINT('Ctrl Pts',(-20.353060251684,-9.71462954053041,
0.));
#198600=CARTESIAN_POINT('Ctrl Pts',(-20.353053841303,-9.71462809124915,
0.));
#198601=CARTESIAN_POINT('',(-22.8400320311649,-12.4230808101438,0.));
#198602=CARTESIAN_POINT('Ctrl Pts',(-21.2610617890679,-7.52250298901264,
0.));
#198603=CARTESIAN_POINT('Ctrl Pts',(-21.2610617890679,-7.52250298901264,
12.));
#198604=CARTESIAN_POINT('Ctrl Pts',(-21.2610673466886,-7.5225064970397,
0.));
#198605=CARTESIAN_POINT('Ctrl Pts',(-21.2610673466886,-7.5225064970397,
12.));
#198606=CARTESIAN_POINT('Ctrl Pts',(-21.2611204474866,-7.52252744144903,
0.));
#198607=CARTESIAN_POINT('Ctrl Pts',(-21.2611204474866,-7.52252744144903,
12.));
#198608=CARTESIAN_POINT('Ctrl Pts',(-21.261326054066,-7.5226006423166,0.));
#198609=CARTESIAN_POINT('Ctrl Pts',(-21.261326054066,-7.5226006423166,12.));
#198610=CARTESIAN_POINT('Ctrl Pts',(-21.2618521283555,-7.52278182242669,
0.));
#198611=CARTESIAN_POINT('Ctrl Pts',(-21.2618521283555,-7.52278182242669,
12.));
#198612=CARTESIAN_POINT('Ctrl Pts',(-21.262927782038,-7.52314642316199,
0.));
#198613=CARTESIAN_POINT('Ctrl Pts',(-21.262927782038,-7.52314642316199,
12.));
#198614=CARTESIAN_POINT('Ctrl Pts',(-21.2644161259962,-7.52364573027552,
0.));
#198615=CARTESIAN_POINT('Ctrl Pts',(-21.2644161259962,-7.52364573027552,
12.));
#198616=CARTESIAN_POINT('Ctrl Pts',(-21.2663059157058,-7.52427261074297,
0.));
#198617=CARTESIAN_POINT('Ctrl Pts',(-21.2663059157058,-7.52427261074297,
12.));
#198618=CARTESIAN_POINT('Ctrl Pts',(-21.2685823838671,-7.5250177033353,
0.));
#198619=CARTESIAN_POINT('Ctrl Pts',(-21.2685823838671,-7.5250177033353,
12.));
#198620=CARTESIAN_POINT('Ctrl Pts',(-21.2712301573466,-7.52587126095529,
0.));
#198621=CARTESIAN_POINT('Ctrl Pts',(-21.2712301573466,-7.52587126095529,
12.));
#198622=CARTESIAN_POINT('Ctrl Pts',(-21.2742366113579,-7.5268252691854,
0.));
#198623=CARTESIAN_POINT('Ctrl Pts',(-21.2742366113579,-7.5268252691854,
12.));
#198624=CARTESIAN_POINT('Ctrl Pts',(-21.2775925269652,-7.52787386225332,
0.));
#198625=CARTESIAN_POINT('Ctrl Pts',(-21.2775925269652,-7.52787386225332,
12.));
#198626=CARTESIAN_POINT('Ctrl Pts',(-21.2812902781143,-7.52901217930407,
0.));
#198627=CARTESIAN_POINT('Ctrl Pts',(-21.2812902781143,-7.52901217930407,
12.));
#198628=CARTESIAN_POINT('Ctrl Pts',(-21.2853226580657,-7.53023562438229,
0.));
#198629=CARTESIAN_POINT('Ctrl Pts',(-21.2853226580657,-7.53023562438229,
12.));
#198630=CARTESIAN_POINT('Ctrl Pts',(-21.2896816163842,-7.53153906987855,
0.));
#198631=CARTESIAN_POINT('Ctrl Pts',(-21.2896816163842,-7.53153906987855,
12.));
#198632=CARTESIAN_POINT('Ctrl Pts',(-21.2943588989331,-7.53291726078526,
0.));
#198633=CARTESIAN_POINT('Ctrl Pts',(-21.2943588989331,-7.53291726078526,
12.));
#198634=CARTESIAN_POINT('Ctrl Pts',(-21.2993464250717,-7.53436505309942,
0.));
#198635=CARTESIAN_POINT('Ctrl Pts',(-21.2993464250717,-7.53436505309942,
12.));
#198636=CARTESIAN_POINT('Ctrl Pts',(-21.3046368712157,-7.53587778251735,
0.));
#198637=CARTESIAN_POINT('Ctrl Pts',(-21.3046368712157,-7.53587778251735,
12.));
#198638=CARTESIAN_POINT('Ctrl Pts',(-21.310223716773,-7.53745129364616,
0.));
#198639=CARTESIAN_POINT('Ctrl Pts',(-21.310223716773,-7.53745129364616,
12.));
#198640=CARTESIAN_POINT('Ctrl Pts',(-21.3161009456256,-7.53908175169898,
0.));
#198641=CARTESIAN_POINT('Ctrl Pts',(-21.3161009456256,-7.53908175169898,
12.));
#198642=CARTESIAN_POINT('Ctrl Pts',(-21.3222628524165,-7.54076552038278,
0.));
#198643=CARTESIAN_POINT('Ctrl Pts',(-21.3222628524165,-7.54076552038278,
12.));
#198644=CARTESIAN_POINT('Ctrl Pts',(-21.328703791771,-7.5424990037703,0.));
#198645=CARTESIAN_POINT('Ctrl Pts',(-21.328703791771,-7.5424990037703,12.));
#198646=CARTESIAN_POINT('Ctrl Pts',(-21.3354182340149,-7.54427868151267,
0.));
#198647=CARTESIAN_POINT('Ctrl Pts',(-21.3354182340149,-7.54427868151267,
12.));
#198648=CARTESIAN_POINT('Ctrl Pts',(-21.3424008295038,-7.54610114948346,
0.));
#198649=CARTESIAN_POINT('Ctrl Pts',(-21.3424008295038,-7.54610114948346,
12.));
#198650=CARTESIAN_POINT('Ctrl Pts',(-21.3496464761531,-7.5479631624633,
0.));
#198651=CARTESIAN_POINT('Ctrl Pts',(-21.3496464761531,-7.5479631624633,
12.));
#198652=CARTESIAN_POINT('Ctrl Pts',(-21.3571503685855,-7.54986166521309,
0.));
#198653=CARTESIAN_POINT('Ctrl Pts',(-21.3571503685855,-7.54986166521309,
12.));
#198654=CARTESIAN_POINT('Ctrl Pts',(-21.3649079431865,-7.55179375777443,
0.));
#198655=CARTESIAN_POINT('Ctrl Pts',(-21.3649079431865,-7.55179375777443,
12.));
#198656=CARTESIAN_POINT('Ctrl Pts',(-21.3729148390243,-7.55375667080028,
0.));
#198657=CARTESIAN_POINT('Ctrl Pts',(-21.3729148390243,-7.55375667080028,
12.));
#198658=CARTESIAN_POINT('Ctrl Pts',(-21.3811668478932,-7.55574773403502,
0.));
#198659=CARTESIAN_POINT('Ctrl Pts',(-21.3811668478932,-7.55574773403502,
12.));
#198660=CARTESIAN_POINT('Ctrl Pts',(-21.3896598842117,-7.55776435731416,
0.));
#198661=CARTESIAN_POINT('Ctrl Pts',(-21.3896598842117,-7.55776435731416,
12.));
#198662=CARTESIAN_POINT('Ctrl Pts',(-21.3983899952987,-7.5598040370061,
0.));
#198663=CARTESIAN_POINT('Ctrl Pts',(-21.3983899952987,-7.5598040370061,
12.));
#198664=CARTESIAN_POINT('Ctrl Pts',(-21.4073533630365,-7.56186435703621,
0.));
#198665=CARTESIAN_POINT('Ctrl Pts',(-21.4073533630365,-7.56186435703621,
12.));
#198666=CARTESIAN_POINT('Ctrl Pts',(-21.4165463106254,-7.56394299313684,
0.));
#198667=CARTESIAN_POINT('Ctrl Pts',(-21.4165463106254,-7.56394299313684,
12.));
#198668=CARTESIAN_POINT('Ctrl Pts',(-21.4259653015736,-7.56603771218712,
0.));
#198669=CARTESIAN_POINT('Ctrl Pts',(-21.4259653015736,-7.56603771218712,
12.));
#198670=CARTESIAN_POINT('Ctrl Pts',(-21.4356069261513,-7.56814636360847,
0.));
#198671=CARTESIAN_POINT('Ctrl Pts',(-21.4356069261513,-7.56814636360847,
12.));
#198672=CARTESIAN_POINT('Ctrl Pts',(-21.4454678907509,-7.57026687261165,
0.));
#198673=CARTESIAN_POINT('Ctrl Pts',(-21.4454678907509,-7.57026687261165,
12.));
#198674=CARTESIAN_POINT('Ctrl Pts',(-21.4555450053142,-7.57239723223505,
0.));
#198675=CARTESIAN_POINT('Ctrl Pts',(-21.4555450053142,-7.57239723223505,
12.));
#198676=CARTESIAN_POINT('Ctrl Pts',(-21.4658351740128,-7.57453549743411,
0.));
#198677=CARTESIAN_POINT('Ctrl Pts',(-21.4658351740128,-7.57453549743411,
12.));
#198678=CARTESIAN_POINT('Ctrl Pts',(-21.4763353936762,-7.57667978402987,
0.));
#198679=CARTESIAN_POINT('Ctrl Pts',(-21.4763353936762,-7.57667978402987,
12.));
#198680=CARTESIAN_POINT('Ctrl Pts',(-21.4870427508194,-7.57882826679131,
0.));
#198681=CARTESIAN_POINT('Ctrl Pts',(-21.4870427508194,-7.57882826679131,
12.));
#198682=CARTESIAN_POINT('Ctrl Pts',(-21.4979544192744,-7.58097917790744,
0.));
#198683=CARTESIAN_POINT('Ctrl Pts',(-21.4979544192744,-7.58097917790744,
12.));
#198684=CARTESIAN_POINT('Ctrl Pts',(-21.5090676573873,-7.58313080519179,
0.));
#198685=CARTESIAN_POINT('Ctrl Pts',(-21.5090676573873,-7.58313080519179,
12.));
#198686=CARTESIAN_POINT('Ctrl Pts',(-21.5203798035299,-7.58528148919129,
0.));
#198687=CARTESIAN_POINT('Ctrl Pts',(-21.5203798035299,-7.58528148919129,
12.));
#198688=CARTESIAN_POINT('Ctrl Pts',(-21.5318882716736,-7.58742962034833,
0.));
#198689=CARTESIAN_POINT('Ctrl Pts',(-21.5318882716736,-7.58742962034833,
12.));
#198690=CARTESIAN_POINT('Ctrl Pts',(-21.543590547011,-7.58957363620013,
0.));
#198691=CARTESIAN_POINT('Ctrl Pts',(-21.543590547011,-7.58957363620013,
12.));
#198692=CARTESIAN_POINT('Ctrl Pts',(-21.5554841813462,-7.59171201844776,
0.));
#198693=CARTESIAN_POINT('Ctrl Pts',(-21.5554841813462,-7.59171201844776,
12.));
#198694=CARTESIAN_POINT('Ctrl Pts',(-21.5675667904726,-7.59384329124918,
0.));
#198695=CARTESIAN_POINT('Ctrl Pts',(-21.5675667904726,-7.59384329124918,
12.));
#198696=CARTESIAN_POINT('Ctrl Pts',(-21.5798360518978,-7.59596601973583,
0.));
#198697=CARTESIAN_POINT('Ctrl Pts',(-21.5798360518978,-7.59596601973583,
12.));
#198698=CARTESIAN_POINT('Ctrl Pts',(-21.5922897024466,-7.59807880846194,
0.));
#198699=CARTESIAN_POINT('Ctrl Pts',(-21.5922897024466,-7.59807880846194,
12.));
#198700=CARTESIAN_POINT('Ctrl Pts',(-21.6049255358843,-7.6001802998824,
0.));
#198701=CARTESIAN_POINT('Ctrl Pts',(-21.6049255358843,-7.6001802998824,
12.));
#198702=CARTESIAN_POINT('Ctrl Pts',(-21.617741400599,-7.60226917285428,
0.));
#198703=CARTESIAN_POINT('Ctrl Pts',(-21.617741400599,-7.60226917285428,
12.));
#198704=CARTESIAN_POINT('Ctrl Pts',(-21.6307351973822,-7.60434414118295,
0.));
#198705=CARTESIAN_POINT('Ctrl Pts',(-21.6307351973822,-7.60434414118295,
12.));
#198706=CARTESIAN_POINT('Ctrl Pts',(-21.6439048771743,-7.60640395216356,
0.));
#198707=CARTESIAN_POINT('Ctrl Pts',(-21.6439048771743,-7.60640395216356,
12.));
#198708=CARTESIAN_POINT('Ctrl Pts',(-21.6572484388081,-7.60844738512873,
0.));
#198709=CARTESIAN_POINT('Ctrl Pts',(-21.6572484388081,-7.60844738512873,
12.));
#198710=CARTESIAN_POINT('Ctrl Pts',(-21.6707639267576,-7.61047325000955,
0.));
#198711=CARTESIAN_POINT('Ctrl Pts',(-21.6707639267576,-7.61047325000955,
12.));
#198712=CARTESIAN_POINT('Ctrl Pts',(-21.6844494295815,-7.61248038630268,
0.));
#198713=CARTESIAN_POINT('Ctrl Pts',(-21.6844494295815,-7.61248038630268,
12.));
#198714=CARTESIAN_POINT('Ctrl Pts',(-21.6983030783322,-7.61446766202786,
0.));
#198715=CARTESIAN_POINT('Ctrl Pts',(-21.6983030783322,-7.61446766202786,
12.));
#198716=CARTESIAN_POINT('Ctrl Pts',(-21.7123230449834,-7.6164339727042,
0.));
#198717=CARTESIAN_POINT('Ctrl Pts',(-21.7123230449834,-7.6164339727042,
12.));
#198718=CARTESIAN_POINT('Ctrl Pts',(-21.7265075407975,-7.61837824030537,
0.));
#198719=CARTESIAN_POINT('Ctrl Pts',(-21.7265075407975,-7.61837824030537,
12.));
#198720=CARTESIAN_POINT('Ctrl Pts',(-21.7408548148656,-7.62029941230854,
0.));
#198721=CARTESIAN_POINT('Ctrl Pts',(-21.7408548148656,-7.62029941230854,
12.));
#198722=CARTESIAN_POINT('Ctrl Pts',(-21.7553631528328,-7.62219646084228,
0.));
#198723=CARTESIAN_POINT('Ctrl Pts',(-21.7553631528328,-7.62219646084228,
12.));
#198724=CARTESIAN_POINT('Ctrl Pts',(-21.7700308755584,-7.62406838181166,
0.));
#198725=CARTESIAN_POINT('Ctrl Pts',(-21.7700308755584,-7.62406838181166,
12.));
#198726=CARTESIAN_POINT('Ctrl Pts',(-21.7848563378021,-7.62591419404512,
0.));
#198727=CARTESIAN_POINT('Ctrl Pts',(-21.7848563378021,-7.62591419404512,
12.));
#198728=CARTESIAN_POINT('Ctrl Pts',(-21.799837926858,-7.62773293842389,
0.));
#198729=CARTESIAN_POINT('Ctrl Pts',(-21.799837926858,-7.62773293842389,
12.));
#198730=CARTESIAN_POINT('Ctrl Pts',(-21.814974061509,-7.62952367718126,
0.));
#198731=CARTESIAN_POINT('Ctrl Pts',(-21.814974061509,-7.62952367718126,
12.));
#198732=CARTESIAN_POINT('Ctrl Pts',(-21.8302631910195,-7.63128549323022,
0.));
#198733=CARTESIAN_POINT('Ctrl Pts',(-21.8302631910195,-7.63128549323022,
12.));
#198734=CARTESIAN_POINT('Ctrl Pts',(-21.8457037941084,-7.63301748948935,
0.));
#198735=CARTESIAN_POINT('Ctrl Pts',(-21.8457037941084,-7.63301748948935,
12.));
#198736=CARTESIAN_POINT('Ctrl Pts',(-21.8612943779089,-7.63471878821225,
0.));
#198737=CARTESIAN_POINT('Ctrl Pts',(-21.8612943779089,-7.63471878821225,
12.));
#198738=CARTESIAN_POINT('Ctrl Pts',(-21.8770334769496,-7.63638853033399,
0.));
#198739=CARTESIAN_POINT('Ctrl Pts',(-21.8770334769496,-7.63638853033399,
12.));
#198740=CARTESIAN_POINT('Ctrl Pts',(-21.8929196523514,-7.63802587492034,
0.));
#198741=CARTESIAN_POINT('Ctrl Pts',(-21.8929196523514,-7.63802587492034,
12.));
#198742=CARTESIAN_POINT('Ctrl Pts',(-21.9089514909874,-7.63962999860927,
0.));
#198743=CARTESIAN_POINT('Ctrl Pts',(-21.9089514909874,-7.63962999860927,
12.));
#198744=CARTESIAN_POINT('Ctrl Pts',(-21.9251276046546,-7.64120009506531,
0.));
#198745=CARTESIAN_POINT('Ctrl Pts',(-21.9251276046546,-7.64120009506531,
12.));
#198746=CARTESIAN_POINT('Ctrl Pts',(-21.9414466292072,-7.64273537442682,
0.));
#198747=CARTESIAN_POINT('Ctrl Pts',(-21.9414466292072,-7.64273537442682,
12.));
#198748=CARTESIAN_POINT('Ctrl Pts',(-21.9579072237651,-7.64423506279122,
0.));
#198749=CARTESIAN_POINT('Ctrl Pts',(-21.9579072237651,-7.64423506279122,
12.));
#198750=CARTESIAN_POINT('Ctrl Pts',(-21.9745080700798,-7.64569840177335,
0.));
#198751=CARTESIAN_POINT('Ctrl Pts',(-21.9745080700798,-7.64569840177335,
12.));
#198752=CARTESIAN_POINT('Ctrl Pts',(-21.9912478718542,-7.64712464805249,
0.));
#198753=CARTESIAN_POINT('Ctrl Pts',(-21.9912478718542,-7.64712464805249,
12.));
#198754=CARTESIAN_POINT('Ctrl Pts',(-22.0081253540774,-7.64851307293351,
0.));
#198755=CARTESIAN_POINT('Ctrl Pts',(-22.0081253540774,-7.64851307293351,
12.));
#198756=CARTESIAN_POINT('Ctrl Pts',(-22.0251392623209,-7.64986296190168,
0.));
#198757=CARTESIAN_POINT('Ctrl Pts',(-22.0251392623209,-7.64986296190168,
12.));
#198758=CARTESIAN_POINT('Ctrl Pts',(-22.0422883621174,-7.65117361421358,
0.));
#198759=CARTESIAN_POINT('Ctrl Pts',(-22.0422883621174,-7.65117361421358,
12.));
#198760=CARTESIAN_POINT('Ctrl Pts',(-22.0595714384431,-7.65244434253112,
0.));
#198761=CARTESIAN_POINT('Ctrl Pts',(-22.0595714384431,-7.65244434253112,
12.));
#198762=CARTESIAN_POINT('Ctrl Pts',(-22.0769872951596,-7.65367447254949,
0.));
#198763=CARTESIAN_POINT('Ctrl Pts',(-22.0769872951596,-7.65367447254949,
12.));
#198764=CARTESIAN_POINT('Ctrl Pts',(-22.094534754469,-7.65486334263643,
0.));
#198765=CARTESIAN_POINT('Ctrl Pts',(-22.094534754469,-7.65486334263643,
12.));
#198766=CARTESIAN_POINT('Ctrl Pts',(-22.1122126563329,-7.65601030346806,
0.));
#198767=CARTESIAN_POINT('Ctrl Pts',(-22.1122126563329,-7.65601030346806,
12.));
#198768=CARTESIAN_POINT('Ctrl Pts',(-22.1300198579675,-7.65711471769396,
0.));
#198769=CARTESIAN_POINT('Ctrl Pts',(-22.1300198579675,-7.65711471769396,
12.));
#198770=CARTESIAN_POINT('Ctrl Pts',(-22.1479552334211,-7.65817595963349,
0.));
#198771=CARTESIAN_POINT('Ctrl Pts',(-22.1479552334211,-7.65817595963349,
12.));
#198772=CARTESIAN_POINT('Ctrl Pts',(-22.1660176731178,-7.6591934149693,
0.));
#198773=CARTESIAN_POINT('Ctrl Pts',(-22.1660176731178,-7.6591934149693,
12.));
#198774=CARTESIAN_POINT('Ctrl Pts',(-22.1842060834091,-7.66016648045004,
0.));
#198775=CARTESIAN_POINT('Ctrl Pts',(-22.1842060834091,-7.66016648045004,
12.));
#198776=CARTESIAN_POINT('Ctrl Pts',(-22.2025193860964,-7.6610945635927,
0.));
#198777=CARTESIAN_POINT('Ctrl Pts',(-22.2025193860964,-7.6610945635927,
12.));
#198778=CARTESIAN_POINT('Ctrl Pts',(-22.2209565180085,-7.66197708240399,
0.));
#198779=CARTESIAN_POINT('Ctrl Pts',(-22.2209565180085,-7.66197708240399,
12.));
#198780=CARTESIAN_POINT('Ctrl Pts',(-22.2395164306547,-7.66281346512508,
0.));
#198781=CARTESIAN_POINT('Ctrl Pts',(-22.2395164306547,-7.66281346512508,
12.));
#198782=CARTESIAN_POINT('Ctrl Pts',(-22.258198089848,-7.6636031499764,0.));
#198783=CARTESIAN_POINT('Ctrl Pts',(-22.258198089848,-7.6636031499764,12.));
#198784=CARTESIAN_POINT('Ctrl Pts',(-22.2770004753335,-7.66434558490978,
0.));
#198785=CARTESIAN_POINT('Ctrl Pts',(-22.2770004753335,-7.66434558490978,
12.));
#198786=CARTESIAN_POINT('Ctrl Pts',(-22.2959225803937,-7.66504022736298,
0.));
#198787=CARTESIAN_POINT('Ctrl Pts',(-22.2959225803937,-7.66504022736298,
12.));
#198788=CARTESIAN_POINT('Ctrl Pts',(-22.314963411484,-7.66568654402493,
0.));
#198789=CARTESIAN_POINT('Ctrl Pts',(-22.314963411484,-7.66568654402493,
12.));
#198790=CARTESIAN_POINT('Ctrl Pts',(-22.3341219879469,-7.66628401061952,
0.));
#198791=CARTESIAN_POINT('Ctrl Pts',(-22.3341219879469,-7.66628401061952,
12.));
#198792=CARTESIAN_POINT('Ctrl Pts',(-22.3533973417021,-7.66683211169158,
0.));
#198793=CARTESIAN_POINT('Ctrl Pts',(-22.3533973417021,-7.66683211169158,
12.));
#198794=CARTESIAN_POINT('Ctrl Pts',(-22.372788516936,-7.66733034039882,
0.));
#198795=CARTESIAN_POINT('Ctrl Pts',(-22.372788516936,-7.66733034039882,
12.));
#198796=CARTESIAN_POINT('Ctrl Pts',(-22.3922945697773,-7.66777819830789,
0.));
#198797=CARTESIAN_POINT('Ctrl Pts',(-22.3922945697773,-7.66777819830789,
12.));
#198798=CARTESIAN_POINT('Ctrl Pts',(-22.4119145679758,-7.66817519519639,
0.));
#198799=CARTESIAN_POINT('Ctrl Pts',(-22.4119145679758,-7.66817519519639,
12.));
#198800=CARTESIAN_POINT('Ctrl Pts',(-22.4316475906603,-7.66852084886704,
0.));
#198801=CARTESIAN_POINT('Ctrl Pts',(-22.4316475906603,-7.66852084886704,
12.));
#198802=CARTESIAN_POINT('Ctrl Pts',(-22.4514927280855,-7.66881468496634,
0.));
#198803=CARTESIAN_POINT('Ctrl Pts',(-22.4514927280855,-7.66881468496634,
12.));
#198804=CARTESIAN_POINT('Ctrl Pts',(-22.47144908137,-7.6690562368083,0.));
#198805=CARTESIAN_POINT('Ctrl Pts',(-22.47144908137,-7.6690562368083,12.));
#198806=CARTESIAN_POINT('Ctrl Pts',(-22.4915157622312,-7.66924504520314,
0.));
#198807=CARTESIAN_POINT('Ctrl Pts',(-22.4915157622312,-7.66924504520314,
12.));
#198808=CARTESIAN_POINT('Ctrl Pts',(-22.5116918927032,-7.66938065829107,
0.));
#198809=CARTESIAN_POINT('Ctrl Pts',(-22.5116918927032,-7.66938065829107,
12.));
#198810=CARTESIAN_POINT('Ctrl Pts',(-22.53197660492,-7.66946263138143,0.));
#198811=CARTESIAN_POINT('Ctrl Pts',(-22.53197660492,-7.66946263138143,12.));
#198812=CARTESIAN_POINT('Ctrl Pts',(-22.5523690409116,-7.66949052679692,
0.));
#198813=CARTESIAN_POINT('Ctrl Pts',(-22.5523690409116,-7.66949052679692,
12.));
#198814=CARTESIAN_POINT('Ctrl Pts',(-22.5728683523831,-7.66946391372305,
0.));
#198815=CARTESIAN_POINT('Ctrl Pts',(-22.5728683523831,-7.66946391372305,
12.));
#198816=CARTESIAN_POINT('Ctrl Pts',(-22.5934737004953,-7.66938236806232,
0.));
#198817=CARTESIAN_POINT('Ctrl Pts',(-22.5934737004953,-7.66938236806232,
12.));
#198818=CARTESIAN_POINT('Ctrl Pts',(-22.6141842556243,-7.66924547229413,
0.));
#198819=CARTESIAN_POINT('Ctrl Pts',(-22.6141842556243,-7.66924547229413,
12.));
#198820=CARTESIAN_POINT('Ctrl Pts',(-22.6349991971541,-7.66905281533714,
0.));
#198821=CARTESIAN_POINT('Ctrl Pts',(-22.6349991971541,-7.66905281533714,
12.));
#198822=CARTESIAN_POINT('Ctrl Pts',(-22.6559177133127,-7.66880399241322,
0.));
#198823=CARTESIAN_POINT('Ctrl Pts',(-22.6559177133127,-7.66880399241322,
12.));
#198824=CARTESIAN_POINT('Ctrl Pts',(-22.6769390009885,-7.66849860491742,
0.));
#198825=CARTESIAN_POINT('Ctrl Pts',(-22.6769390009885,-7.66849860491742,
12.));
#198826=CARTESIAN_POINT('Ctrl Pts',(-22.6980622655446,-7.66813626029274,
0.));
#198827=CARTESIAN_POINT('Ctrl Pts',(-22.6980622655446,-7.66813626029274,
12.));
#198828=CARTESIAN_POINT('Ctrl Pts',(-22.7192867206245,-7.66771657191027,
0.));
#198829=CARTESIAN_POINT('Ctrl Pts',(-22.7192867206245,-7.66771657191027,
12.));
#198830=CARTESIAN_POINT('Ctrl Pts',(-22.7406115879513,-7.66723915895439,
0.));
#198831=CARTESIAN_POINT('Ctrl Pts',(-22.7406115879513,-7.66723915895439,
12.));
#198832=CARTESIAN_POINT('Ctrl Pts',(-22.7620360971843,-7.66670364630298,
0.));
#198833=CARTESIAN_POINT('Ctrl Pts',(-22.7620360971843,-7.66670364630298,
12.));
#198834=CARTESIAN_POINT('Ctrl Pts',(-22.7835594857699,-7.66610966441272,
0.));
#198835=CARTESIAN_POINT('Ctrl Pts',(-22.7835594857699,-7.66610966441272,
12.));
#198836=CARTESIAN_POINT('Ctrl Pts',(-22.8051809987833,-7.66545684920987,
0.));
#198837=CARTESIAN_POINT('Ctrl Pts',(-22.8051809987833,-7.66545684920987,
12.));
#198838=CARTESIAN_POINT('Ctrl Pts',(-22.8268998887678,-7.66474484198548,
0.));
#198839=CARTESIAN_POINT('Ctrl Pts',(-22.8268998887678,-7.66474484198548,
12.));
#198840=CARTESIAN_POINT('Ctrl Pts',(-22.848715415557,-7.66397328929802,
0.));
#198841=CARTESIAN_POINT('Ctrl Pts',(-22.848715415557,-7.66397328929802,
12.));
#198842=CARTESIAN_POINT('Ctrl Pts',(-22.8706268461283,-7.66314184287336,
0.));
#198843=CARTESIAN_POINT('Ctrl Pts',(-22.8706268461283,-7.66314184287336,
12.));
#198844=CARTESIAN_POINT('Ctrl Pts',(-22.8926334544883,-7.66225015950155,
0.));
#198845=CARTESIAN_POINT('Ctrl Pts',(-22.8926334544883,-7.66225015950155,
12.));
#198846=CARTESIAN_POINT('Ctrl Pts',(-22.9147345215421,-7.66129790094107,
0.));
#198847=CARTESIAN_POINT('Ctrl Pts',(-22.9147345215421,-7.66129790094107,
12.));
#198848=CARTESIAN_POINT('Ctrl Pts',(-22.9369293349593,-7.66028473382777,
0.));
#198849=CARTESIAN_POINT('Ctrl Pts',(-22.9369293349593,-7.66028473382777,
12.));
#198850=CARTESIAN_POINT('Ctrl Pts',(-22.959217189033,-7.65921032958901,
0.));
#198851=CARTESIAN_POINT('Ctrl Pts',(-22.959217189033,-7.65921032958901,
12.));
#198852=CARTESIAN_POINT('Ctrl Pts',(-22.9815973845296,-7.65807436436431,
0.));
#198853=CARTESIAN_POINT('Ctrl Pts',(-22.9815973845296,-7.65807436436431,
12.));
#198854=CARTESIAN_POINT('Ctrl Pts',(-23.0040692285814,-7.65687651891304,
0.));
#198855=CARTESIAN_POINT('Ctrl Pts',(-23.0040692285814,-7.65687651891304,
12.));
#198856=CARTESIAN_POINT('Ctrl Pts',(-23.0266320345787,-7.65561647852533,
0.));
#198857=CARTESIAN_POINT('Ctrl Pts',(-23.0266320345787,-7.65561647852533,
12.));
#198858=CARTESIAN_POINT('Ctrl Pts',(-23.0492851220528,-7.65429393293945,
0.));
#198859=CARTESIAN_POINT('Ctrl Pts',(-23.0492851220528,-7.65429393293945,
12.));
#198860=CARTESIAN_POINT('Ctrl Pts',(-23.072027816555,-7.65290857626357,
0.));
#198861=CARTESIAN_POINT('Ctrl Pts',(-23.072027816555,-7.65290857626357,
12.));
#198862=CARTESIAN_POINT('Ctrl Pts',(-23.094859449525,-7.65146010690475,
0.));
#198863=CARTESIAN_POINT('Ctrl Pts',(-23.094859449525,-7.65146010690475,
12.));
#198864=CARTESIAN_POINT('Ctrl Pts',(-23.1177793581679,-7.64994822749859,
0.));
#198865=CARTESIAN_POINT('Ctrl Pts',(-23.1177793581679,-7.64994822749859,
12.));
#198866=CARTESIAN_POINT('Ctrl Pts',(-23.1407868853819,-7.64837264482942,
0.));
#198867=CARTESIAN_POINT('Ctrl Pts',(-23.1407868853819,-7.64837264482942,
12.));
#198868=CARTESIAN_POINT('Ctrl Pts',(-23.1638813796694,-7.64673306975804,
0.));
#198869=CARTESIAN_POINT('Ctrl Pts',(-23.1638813796694,-7.64673306975804,
12.));
#198870=CARTESIAN_POINT('Ctrl Pts',(-23.1870621950452,-7.64502921715482,
0.));
#198871=CARTESIAN_POINT('Ctrl Pts',(-23.1870621950452,-7.64502921715482,
12.));
#198872=CARTESIAN_POINT('Ctrl Pts',(-23.2103286909398,-7.64326080583679,
0.));
#198873=CARTESIAN_POINT('Ctrl Pts',(-23.2103286909398,-7.64326080583679,
12.));
#198874=CARTESIAN_POINT('Ctrl Pts',(-23.2336802320912,-7.64142755851504,
0.));
#198875=CARTESIAN_POINT('Ctrl Pts',(-23.2336802320912,-7.64142755851504,
12.));
#198876=CARTESIAN_POINT('Ctrl Pts',(-23.2571161884488,-7.63952920172835,
0.));
#198877=CARTESIAN_POINT('Ctrl Pts',(-23.2571161884488,-7.63952920172835,
12.));
#198878=CARTESIAN_POINT('Ctrl Pts',(-23.2806359350855,-7.63756546576374,
0.));
#198879=CARTESIAN_POINT('Ctrl Pts',(-23.2806359350855,-7.63756546576374,
12.));
#198880=CARTESIAN_POINT('Ctrl Pts',(-23.3042388521022,-7.63553608458782,
0.));
#198881=CARTESIAN_POINT('Ctrl Pts',(-23.3042388521022,-7.63553608458782,
12.));
#198882=CARTESIAN_POINT('Ctrl Pts',(-23.3279243245241,-7.63344079578161,
0.));
#198883=CARTESIAN_POINT('Ctrl Pts',(-23.3279243245241,-7.63344079578161,
12.));
#198884=CARTESIAN_POINT('Ctrl Pts',(-23.3516917421972,-7.63127934048136,
0.));
#198885=CARTESIAN_POINT('Ctrl Pts',(-23.3516917421972,-7.63127934048136,
12.));
#198886=CARTESIAN_POINT('Ctrl Pts',(-23.3755404996636,-7.62905146332592,
0.));
#198887=CARTESIAN_POINT('Ctrl Pts',(-23.3755404996636,-7.62905146332592,
12.));
#198888=CARTESIAN_POINT('Ctrl Pts',(-23.399469996112,-7.62675691240328,
0.));
#198889=CARTESIAN_POINT('Ctrl Pts',(-23.399469996112,-7.62675691240328,
12.));
#198890=CARTESIAN_POINT('Ctrl Pts',(-23.4234796353542,-7.62439543920049,
0.));
#198891=CARTESIAN_POINT('Ctrl Pts',(-23.4234796353542,-7.62439543920049,
12.));
#198892=CARTESIAN_POINT('Ctrl Pts',(-23.4475688257854,-7.62196679855954,
0.));
#198893=CARTESIAN_POINT('Ctrl Pts',(-23.4475688257854,-7.62196679855954,
12.));
#198894=CARTESIAN_POINT('Ctrl Pts',(-23.4717369803438,-7.61947074863976,
0.));
#198895=CARTESIAN_POINT('Ctrl Pts',(-23.4717369803438,-7.61947074863976,
12.));
#198896=CARTESIAN_POINT('Ctrl Pts',(-23.4959835164609,-7.61690705088318,
0.));
#198897=CARTESIAN_POINT('Ctrl Pts',(-23.4959835164609,-7.61690705088318,
12.));
#198898=CARTESIAN_POINT('Ctrl Pts',(-23.5203078560129,-7.61427546999297,
0.));
#198899=CARTESIAN_POINT('Ctrl Pts',(-23.5203078560129,-7.61427546999297,
12.));
#198900=CARTESIAN_POINT('Ctrl Pts',(-23.544709425203,-7.61157577385371,
0.));
#198901=CARTESIAN_POINT('Ctrl Pts',(-23.544709425203,-7.61157577385371,
12.));
#198902=CARTESIAN_POINT('Ctrl Pts',(-23.5691876544244,-7.60880773344599,
0.));
#198903=CARTESIAN_POINT('Ctrl Pts',(-23.5691876544244,-7.60880773344599,
12.));
#198904=CARTESIAN_POINT('Ctrl Pts',(-23.5937419781245,-7.60597112277093,
0.));
#198905=CARTESIAN_POINT('Ctrl Pts',(-23.5937419781245,-7.60597112277093,
12.));
#198906=CARTESIAN_POINT('Ctrl Pts',(-23.6183718346576,-7.60306571877805,
0.));
#198907=CARTESIAN_POINT('Ctrl Pts',(-23.6183718346576,-7.60306571877805,
12.));
#198908=CARTESIAN_POINT('Ctrl Pts',(-23.6430766661418,-7.60009130130125,
0.));
#198909=CARTESIAN_POINT('Ctrl Pts',(-23.6430766661418,-7.60009130130125,
12.));
#198910=CARTESIAN_POINT('Ctrl Pts',(-23.6678559182875,-7.59704765299566,
0.));
#198911=CARTESIAN_POINT('Ctrl Pts',(-23.6678559182875,-7.59704765299566,
12.));
#198912=CARTESIAN_POINT('Ctrl Pts',(-23.6927090405066,-7.59393455934034,
0.));
#198913=CARTESIAN_POINT('Ctrl Pts',(-23.6927090405066,-7.59393455934034,
12.));
#198914=CARTESIAN_POINT('Ctrl Pts',(-23.7176354860457,-7.5907518086532,
0.));
#198915=CARTESIAN_POINT('Ctrl Pts',(-23.7176354860457,-7.5907518086532,
12.));
#198916=CARTESIAN_POINT('Ctrl Pts',(-23.7426347121006,-7.58749919210825,
0.));
#198917=CARTESIAN_POINT('Ctrl Pts',(-23.7426347121006,-7.58749919210825,
12.));
#198918=CARTESIAN_POINT('Ctrl Pts',(-23.7677061799376,-7.5841765037627,
0.));
#198919=CARTESIAN_POINT('Ctrl Pts',(-23.7677061799376,-7.5841765037627,
12.));
#198920=CARTESIAN_POINT('Ctrl Pts',(-23.7928493549908,-7.58078354058212,
0.));
#198921=CARTESIAN_POINT('Ctrl Pts',(-23.7928493549908,-7.58078354058212,
12.));
#198922=CARTESIAN_POINT('Ctrl Pts',(-23.8180637069976,-7.57732010249065,
0.));
#198923=CARTESIAN_POINT('Ctrl Pts',(-23.8180637069976,-7.57732010249065,
12.));
#198924=CARTESIAN_POINT('Ctrl Pts',(-23.8433487096132,-7.57378599219814,
0.));
#198925=CARTESIAN_POINT('Ctrl Pts',(-23.8433487096132,-7.57378599219814,
12.));
#198926=CARTESIAN_POINT('Ctrl Pts',(-23.8687038399595,-7.57018101500709,
0.));
#198927=CARTESIAN_POINT('Ctrl Pts',(-23.8687038399595,-7.57018101500709,
12.));
#198928=CARTESIAN_POINT('Ctrl Pts',(-23.8941285782002,-7.5665049786379,
0.));
#198929=CARTESIAN_POINT('Ctrl Pts',(-23.8941285782002,-7.5665049786379,
12.));
#198930=CARTESIAN_POINT('Ctrl Pts',(-23.9196224070759,-7.56275769304772,
0.));
#198931=CARTESIAN_POINT('Ctrl Pts',(-23.9196224070759,-7.56275769304772,
12.));
#198932=CARTESIAN_POINT('Ctrl Pts',(-23.9451848115002,-7.55893897027679,
0.));
#198933=CARTESIAN_POINT('Ctrl Pts',(-23.9451848115002,-7.55893897027679,
12.));
#198934=CARTESIAN_POINT('Ctrl Pts',(-23.9708152779886,-7.55504862424807,
0.));
#198935=CARTESIAN_POINT('Ctrl Pts',(-23.9708152779886,-7.55504862424807,
12.));
#198936=CARTESIAN_POINT('Ctrl Pts',(-23.9965132953187,-7.55108647097431,
0.));
#198937=CARTESIAN_POINT('Ctrl Pts',(-23.9965132953187,-7.55108647097431,
12.));
#198938=CARTESIAN_POINT('Ctrl Pts',(-24.0222783554531,-7.54705232885894,
0.));
#198939=CARTESIAN_POINT('Ctrl Pts',(-24.0222783554531,-7.54705232885894,
12.));
#198940=CARTESIAN_POINT('Ctrl Pts',(-24.0481099543353,-7.54294601896127,
0.));
#198941=CARTESIAN_POINT('Ctrl Pts',(-24.0481099543353,-7.54294601896127,
12.));
#198942=CARTESIAN_POINT('Ctrl Pts',(-24.0740075927984,-7.53876736531004,
0.));
#198943=CARTESIAN_POINT('Ctrl Pts',(-24.0740075927984,-7.53876736531004,
12.));
#198944=CARTESIAN_POINT('Ctrl Pts',(-24.0999707772643,-7.53451619514658,
0.));
#198945=CARTESIAN_POINT('Ctrl Pts',(-24.0999707772643,-7.53451619514658,
12.));
#198946=CARTESIAN_POINT('Ctrl Pts',(-24.1259990209211,-7.53019233935536,
0.));
#198947=CARTESIAN_POINT('Ctrl Pts',(-24.1259990209211,-7.53019233935536,
12.));
#198948=CARTESIAN_POINT('Ctrl Pts',(-24.152091842537,-7.52579563201478,
0.));
#198949=CARTESIAN_POINT('Ctrl Pts',(-24.152091842537,-7.52579563201478,
12.));
#198950=CARTESIAN_POINT('Ctrl Pts',(-24.1782487641602,-7.52132590953862,
0.));
#198951=CARTESIAN_POINT('Ctrl Pts',(-24.1782487641602,-7.52132590953862,
12.));
#198952=CARTESIAN_POINT('Ctrl Pts',(-24.2044693092356,-7.51678300997997,
0.));
#198953=CARTESIAN_POINT('Ctrl Pts',(-24.2044693092356,-7.51678300997997,
12.));
#198954=CARTESIAN_POINT('Ctrl Pts',(-24.230753000389,-7.51216677222198,
0.));
#198955=CARTESIAN_POINT('Ctrl Pts',(-24.230753000389,-7.51216677222198,
12.));
#198956=CARTESIAN_POINT('Ctrl Pts',(-24.2570993577032,-7.50747703535114,
0.));
#198957=CARTESIAN_POINT('Ctrl Pts',(-24.2570993577032,-7.50747703535114,
12.));
#198958=CARTESIAN_POINT('Ctrl Pts',(-24.2835078958966,-7.50271363765098,
0.));
#198959=CARTESIAN_POINT('Ctrl Pts',(-24.2835078958966,-7.50271363765098,
12.));
#198960=CARTESIAN_POINT('Ctrl Pts',(-24.3099781253345,-7.49787641695358,
0.));
#198961=CARTESIAN_POINT('Ctrl Pts',(-24.3099781253345,-7.49787641695358,
12.));
#198962=CARTESIAN_POINT('Ctrl Pts',(-24.3365095573673,-7.49296521252329,
0.));
#198963=CARTESIAN_POINT('Ctrl Pts',(-24.3365095573673,-7.49296521252329,
12.));
#198964=CARTESIAN_POINT('Ctrl Pts',(-24.3631017084513,-7.48797986651827,
0.));
#198965=CARTESIAN_POINT('Ctrl Pts',(-24.3631017084513,-7.48797986651827,
12.));
#198966=CARTESIAN_POINT('Ctrl Pts',(-24.3897541049248,-7.48292022569253,
0.));
#198967=CARTESIAN_POINT('Ctrl Pts',(-24.3897541049248,-7.48292022569253,
12.));
#198968=CARTESIAN_POINT('Ctrl Pts',(-24.4164662871165,-7.47778614286573,
0.));
#198969=CARTESIAN_POINT('Ctrl Pts',(-24.4164662871165,-7.47778614286573,
12.));
#198970=CARTESIAN_POINT('Ctrl Pts',(-24.4432378146501,-7.47257747883318,
0.));
#198971=CARTESIAN_POINT('Ctrl Pts',(-24.4432378146501,-7.47257747883318,
12.));
#198972=CARTESIAN_POINT('Ctrl Pts',(-24.4700682684544,-7.46729410308922,
0.));
#198973=CARTESIAN_POINT('Ctrl Pts',(-24.4700682684544,-7.46729410308922,
12.));
#198974=CARTESIAN_POINT('Ctrl Pts',(-24.4969572391509,-7.46193588961641,
0.));
#198975=CARTESIAN_POINT('Ctrl Pts',(-24.4969572391509,-7.46193588961641,
12.));
#198976=CARTESIAN_POINT('Ctrl Pts',(-24.52390431731,-7.45650271336045,0.));
#198977=CARTESIAN_POINT('Ctrl Pts',(-24.52390431731,-7.45650271336045,12.));
#198978=CARTESIAN_POINT('Ctrl Pts',(-24.5509090831579,-7.45099444651295,
0.));
#198979=CARTESIAN_POINT('Ctrl Pts',(-24.5509090831579,-7.45099444651295,
12.));
#198980=CARTESIAN_POINT('Ctrl Pts',(-24.5779710960865,-7.44541095473162,
0.));
#198981=CARTESIAN_POINT('Ctrl Pts',(-24.5779710960865,-7.44541095473162,
12.));
#198982=CARTESIAN_POINT('Ctrl Pts',(-24.6050898852349,-7.43975209375374,
0.));
#198983=CARTESIAN_POINT('Ctrl Pts',(-24.6050898852349,-7.43975209375374,
12.));
#198984=CARTESIAN_POINT('Ctrl Pts',(-24.6322649369472,-7.4340177048922,
0.));
#198985=CARTESIAN_POINT('Ctrl Pts',(-24.6322649369472,-7.4340177048922,
12.));
#198986=CARTESIAN_POINT('Ctrl Pts',(-24.659495712869,-7.4282076215868,0.));
#198987=CARTESIAN_POINT('Ctrl Pts',(-24.659495712869,-7.4282076215868,12.));
#198988=CARTESIAN_POINT('Ctrl Pts',(-24.6867816727118,-7.42232167765762,
0.));
#198989=CARTESIAN_POINT('Ctrl Pts',(-24.6867816727118,-7.42232167765762,
12.));
#198990=CARTESIAN_POINT('Ctrl Pts',(-24.7141222949988,-7.41635971481243,
0.));
#198991=CARTESIAN_POINT('Ctrl Pts',(-24.7141222949988,-7.41635971481243,
12.));
#198992=CARTESIAN_POINT('Ctrl Pts',(-24.7415170994754,-7.41032159082173,
0.));
#198993=CARTESIAN_POINT('Ctrl Pts',(-24.7415170994754,-7.41032159082173,
12.));
#198994=CARTESIAN_POINT('Ctrl Pts',(-24.7689656669005,-7.40420718661754,
0.));
#198995=CARTESIAN_POINT('Ctrl Pts',(-24.7689656669005,-7.40420718661754,
12.));
#198996=CARTESIAN_POINT('Ctrl Pts',(-24.7964676646518,-7.39801641583612,
0.));
#198997=CARTESIAN_POINT('Ctrl Pts',(-24.7964676646518,-7.39801641583612,
12.));
#198998=CARTESIAN_POINT('Ctrl Pts',(-24.8240228521042,-7.39174922586841,
0.));
#198999=CARTESIAN_POINT('Ctrl Pts',(-24.8240228521042,-7.39174922586841,
12.));
#199000=CARTESIAN_POINT('Ctrl Pts',(-24.8516310625367,-7.38540558904945,
0.));
#199001=CARTESIAN_POINT('Ctrl Pts',(-24.8516310625367,-7.38540558904945,
12.));
#199002=CARTESIAN_POINT('Ctrl Pts',(-24.8792921911309,-7.3789854964161,
0.));
#199003=CARTESIAN_POINT('Ctrl Pts',(-24.8792921911309,-7.3789854964161,
12.));
#199004=CARTESIAN_POINT('Ctrl Pts',(-24.9014633826201,-7.37378825962717,
0.));
#199005=CARTESIAN_POINT('Ctrl Pts',(-24.9014633826201,-7.37378825962717,
12.));
#199006=CARTESIAN_POINT('Ctrl Pts',(-24.9181155530631,-7.36985593120696,
0.));
#199007=CARTESIAN_POINT('Ctrl Pts',(-24.9181155530631,-7.36985593120696,
12.));
#199008=CARTESIAN_POINT('Ctrl Pts',(-24.9292275670705,-7.36721909029059,
0.));
#199009=CARTESIAN_POINT('Ctrl Pts',(-24.9292275670705,-7.36721909029059,
12.));
#199010=CARTESIAN_POINT('Ctrl Pts',(-24.9347862158358,-7.36589684767343,
0.));
#199011=CARTESIAN_POINT('Ctrl Pts',(-24.9347862158358,-7.36589684767343,
12.));
#199012=CARTESIAN_POINT('',(-24.9347862158358,-7.36589684767343,0.));
#199013=CARTESIAN_POINT('Ctrl Pts',(-21.2610617890679,-7.52250298901264,
0.));
#199014=CARTESIAN_POINT('Ctrl Pts',(-21.2610673466886,-7.5225064970397,
0.));
#199015=CARTESIAN_POINT('Ctrl Pts',(-21.2611204474866,-7.52252744144903,
0.));
#199016=CARTESIAN_POINT('Ctrl Pts',(-21.261326054066,-7.5226006423166,0.));
#199017=CARTESIAN_POINT('Ctrl Pts',(-21.2618521283555,-7.52278182242669,
0.));
#199018=CARTESIAN_POINT('Ctrl Pts',(-21.262927782038,-7.52314642316199,
0.));
#199019=CARTESIAN_POINT('Ctrl Pts',(-21.2644161259962,-7.52364573027552,
0.));
#199020=CARTESIAN_POINT('Ctrl Pts',(-21.2663059157058,-7.52427261074297,
0.));
#199021=CARTESIAN_POINT('Ctrl Pts',(-21.2685823838671,-7.5250177033353,
0.));
#199022=CARTESIAN_POINT('Ctrl Pts',(-21.2712301573466,-7.52587126095529,
0.));
#199023=CARTESIAN_POINT('Ctrl Pts',(-21.2742366113579,-7.5268252691854,
0.));
#199024=CARTESIAN_POINT('Ctrl Pts',(-21.2775925269652,-7.52787386225332,
0.));
#199025=CARTESIAN_POINT('Ctrl Pts',(-21.2812902781143,-7.52901217930407,
0.));
#199026=CARTESIAN_POINT('Ctrl Pts',(-21.2853226580657,-7.53023562438229,
0.));
#199027=CARTESIAN_POINT('Ctrl Pts',(-21.2896816163842,-7.53153906987855,
0.));
#199028=CARTESIAN_POINT('Ctrl Pts',(-21.2943588989331,-7.53291726078526,
0.));
#199029=CARTESIAN_POINT('Ctrl Pts',(-21.2993464250717,-7.53436505309942,
0.));
#199030=CARTESIAN_POINT('Ctrl Pts',(-21.3046368712157,-7.53587778251735,
0.));
#199031=CARTESIAN_POINT('Ctrl Pts',(-21.310223716773,-7.53745129364616,
0.));
#199032=CARTESIAN_POINT('Ctrl Pts',(-21.3161009456256,-7.53908175169898,
0.));
#199033=CARTESIAN_POINT('Ctrl Pts',(-21.3222628524165,-7.54076552038278,
0.));
#199034=CARTESIAN_POINT('Ctrl Pts',(-21.328703791771,-7.5424990037703,0.));
#199035=CARTESIAN_POINT('Ctrl Pts',(-21.3354182340149,-7.54427868151267,
0.));
#199036=CARTESIAN_POINT('Ctrl Pts',(-21.3424008295038,-7.54610114948346,
0.));
#199037=CARTESIAN_POINT('Ctrl Pts',(-21.3496464761531,-7.5479631624633,
0.));
#199038=CARTESIAN_POINT('Ctrl Pts',(-21.3571503685855,-7.54986166521309,
0.));
#199039=CARTESIAN_POINT('Ctrl Pts',(-21.3649079431865,-7.55179375777443,
0.));
#199040=CARTESIAN_POINT('Ctrl Pts',(-21.3729148390243,-7.55375667080028,
0.));
#199041=CARTESIAN_POINT('Ctrl Pts',(-21.3811668478932,-7.55574773403502,
0.));
#199042=CARTESIAN_POINT('Ctrl Pts',(-21.3896598842117,-7.55776435731416,
0.));
#199043=CARTESIAN_POINT('Ctrl Pts',(-21.3983899952987,-7.5598040370061,
0.));
#199044=CARTESIAN_POINT('Ctrl Pts',(-21.4073533630365,-7.56186435703621,
0.));
#199045=CARTESIAN_POINT('Ctrl Pts',(-21.4165463106254,-7.56394299313684,
0.));
#199046=CARTESIAN_POINT('Ctrl Pts',(-21.4259653015736,-7.56603771218712,
0.));
#199047=CARTESIAN_POINT('Ctrl Pts',(-21.4356069261513,-7.56814636360847,
0.));
#199048=CARTESIAN_POINT('Ctrl Pts',(-21.4454678907509,-7.57026687261165,
0.));
#199049=CARTESIAN_POINT('Ctrl Pts',(-21.4555450053142,-7.57239723223505,
0.));
#199050=CARTESIAN_POINT('Ctrl Pts',(-21.4658351740128,-7.57453549743411,
0.));
#199051=CARTESIAN_POINT('Ctrl Pts',(-21.4763353936762,-7.57667978402987,
0.));
#199052=CARTESIAN_POINT('Ctrl Pts',(-21.4870427508194,-7.57882826679131,
0.));
#199053=CARTESIAN_POINT('Ctrl Pts',(-21.4979544192744,-7.58097917790744,
0.));
#199054=CARTESIAN_POINT('Ctrl Pts',(-21.5090676573873,-7.58313080519179,
0.));
#199055=CARTESIAN_POINT('Ctrl Pts',(-21.5203798035299,-7.58528148919129,
0.));
#199056=CARTESIAN_POINT('Ctrl Pts',(-21.5318882716736,-7.58742962034833,
0.));
#199057=CARTESIAN_POINT('Ctrl Pts',(-21.543590547011,-7.58957363620013,
0.));
#199058=CARTESIAN_POINT('Ctrl Pts',(-21.5554841813462,-7.59171201844776,
0.));
#199059=CARTESIAN_POINT('Ctrl Pts',(-21.5675667904726,-7.59384329124918,
0.));
#199060=CARTESIAN_POINT('Ctrl Pts',(-21.5798360518978,-7.59596601973583,
0.));
#199061=CARTESIAN_POINT('Ctrl Pts',(-21.5922897024466,-7.59807880846194,
0.));
#199062=CARTESIAN_POINT('Ctrl Pts',(-21.6049255358843,-7.6001802998824,
0.));
#199063=CARTESIAN_POINT('Ctrl Pts',(-21.617741400599,-7.60226917285428,
0.));
#199064=CARTESIAN_POINT('Ctrl Pts',(-21.6307351973822,-7.60434414118295,
0.));
#199065=CARTESIAN_POINT('Ctrl Pts',(-21.6439048771743,-7.60640395216356,
0.));
#199066=CARTESIAN_POINT('Ctrl Pts',(-21.6572484388081,-7.60844738512873,
0.));
#199067=CARTESIAN_POINT('Ctrl Pts',(-21.6707639267576,-7.61047325000955,
0.));
#199068=CARTESIAN_POINT('Ctrl Pts',(-21.6844494295815,-7.61248038630268,
0.));
#199069=CARTESIAN_POINT('Ctrl Pts',(-21.6983030783322,-7.61446766202786,
0.));
#199070=CARTESIAN_POINT('Ctrl Pts',(-21.7123230449834,-7.6164339727042,
0.));
#199071=CARTESIAN_POINT('Ctrl Pts',(-21.7265075407975,-7.61837824030537,
0.));
#199072=CARTESIAN_POINT('Ctrl Pts',(-21.7408548148656,-7.62029941230854,
0.));
#199073=CARTESIAN_POINT('Ctrl Pts',(-21.7553631528328,-7.62219646084228,
0.));
#199074=CARTESIAN_POINT('Ctrl Pts',(-21.7700308755584,-7.62406838181166,
0.));
#199075=CARTESIAN_POINT('Ctrl Pts',(-21.7848563378021,-7.62591419404512,
0.));
#199076=CARTESIAN_POINT('Ctrl Pts',(-21.799837926858,-7.62773293842389,
0.));
#199077=CARTESIAN_POINT('Ctrl Pts',(-21.814974061509,-7.62952367718126,
0.));
#199078=CARTESIAN_POINT('Ctrl Pts',(-21.8302631910195,-7.63128549323022,
0.));
#199079=CARTESIAN_POINT('Ctrl Pts',(-21.8457037941084,-7.63301748948935,
0.));
#199080=CARTESIAN_POINT('Ctrl Pts',(-21.8612943779089,-7.63471878821225,
0.));
#199081=CARTESIAN_POINT('Ctrl Pts',(-21.8770334769496,-7.63638853033399,
0.));
#199082=CARTESIAN_POINT('Ctrl Pts',(-21.8929196523514,-7.63802587492034,
0.));
#199083=CARTESIAN_POINT('Ctrl Pts',(-21.9089514909874,-7.63962999860927,
0.));
#199084=CARTESIAN_POINT('Ctrl Pts',(-21.9251276046546,-7.64120009506531,
0.));
#199085=CARTESIAN_POINT('Ctrl Pts',(-21.9414466292072,-7.64273537442682,
0.));
#199086=CARTESIAN_POINT('Ctrl Pts',(-21.9579072237651,-7.64423506279122,
0.));
#199087=CARTESIAN_POINT('Ctrl Pts',(-21.9745080700798,-7.64569840177335,
0.));
#199088=CARTESIAN_POINT('Ctrl Pts',(-21.9912478718542,-7.64712464805249,
0.));
#199089=CARTESIAN_POINT('Ctrl Pts',(-22.0081253540774,-7.64851307293351,
0.));
#199090=CARTESIAN_POINT('Ctrl Pts',(-22.0251392623209,-7.64986296190168,
0.));
#199091=CARTESIAN_POINT('Ctrl Pts',(-22.0422883621174,-7.65117361421358,
0.));
#199092=CARTESIAN_POINT('Ctrl Pts',(-22.0595714384431,-7.65244434253112,
0.));
#199093=CARTESIAN_POINT('Ctrl Pts',(-22.0769872951596,-7.65367447254949,
0.));
#199094=CARTESIAN_POINT('Ctrl Pts',(-22.094534754469,-7.65486334263643,
0.));
#199095=CARTESIAN_POINT('Ctrl Pts',(-22.1122126563329,-7.65601030346806,
0.));
#199096=CARTESIAN_POINT('Ctrl Pts',(-22.1300198579675,-7.65711471769396,
0.));
#199097=CARTESIAN_POINT('Ctrl Pts',(-22.1479552334211,-7.65817595963349,
0.));
#199098=CARTESIAN_POINT('Ctrl Pts',(-22.1660176731178,-7.6591934149693,
0.));
#199099=CARTESIAN_POINT('Ctrl Pts',(-22.1842060834091,-7.66016648045004,
0.));
#199100=CARTESIAN_POINT('Ctrl Pts',(-22.2025193860964,-7.6610945635927,
0.));
#199101=CARTESIAN_POINT('Ctrl Pts',(-22.2209565180085,-7.66197708240399,
0.));
#199102=CARTESIAN_POINT('Ctrl Pts',(-22.2395164306547,-7.66281346512508,
0.));
#199103=CARTESIAN_POINT('Ctrl Pts',(-22.258198089848,-7.6636031499764,0.));
#199104=CARTESIAN_POINT('Ctrl Pts',(-22.2770004753335,-7.66434558490978,
0.));
#199105=CARTESIAN_POINT('Ctrl Pts',(-22.2959225803937,-7.66504022736298,
0.));
#199106=CARTESIAN_POINT('Ctrl Pts',(-22.314963411484,-7.66568654402493,
0.));
#199107=CARTESIAN_POINT('Ctrl Pts',(-22.3341219879469,-7.66628401061952,
0.));
#199108=CARTESIAN_POINT('Ctrl Pts',(-22.3533973417021,-7.66683211169158,
0.));
#199109=CARTESIAN_POINT('Ctrl Pts',(-22.372788516936,-7.66733034039882,
0.));
#199110=CARTESIAN_POINT('Ctrl Pts',(-22.3922945697773,-7.66777819830789,
0.));
#199111=CARTESIAN_POINT('Ctrl Pts',(-22.4119145679758,-7.66817519519639,
0.));
#199112=CARTESIAN_POINT('Ctrl Pts',(-22.4316475906603,-7.66852084886704,
0.));
#199113=CARTESIAN_POINT('Ctrl Pts',(-22.4514927280855,-7.66881468496634,
0.));
#199114=CARTESIAN_POINT('Ctrl Pts',(-22.47144908137,-7.6690562368083,0.));
#199115=CARTESIAN_POINT('Ctrl Pts',(-22.4915157622312,-7.66924504520314,
0.));
#199116=CARTESIAN_POINT('Ctrl Pts',(-22.5116918927032,-7.66938065829107,
0.));
#199117=CARTESIAN_POINT('Ctrl Pts',(-22.53197660492,-7.66946263138143,0.));
#199118=CARTESIAN_POINT('Ctrl Pts',(-22.5523690409116,-7.66949052679692,
0.));
#199119=CARTESIAN_POINT('Ctrl Pts',(-22.5728683523831,-7.66946391372305,
0.));
#199120=CARTESIAN_POINT('Ctrl Pts',(-22.5934737004953,-7.66938236806232,
0.));
#199121=CARTESIAN_POINT('Ctrl Pts',(-22.6141842556243,-7.66924547229413,
0.));
#199122=CARTESIAN_POINT('Ctrl Pts',(-22.6349991971541,-7.66905281533714,
0.));
#199123=CARTESIAN_POINT('Ctrl Pts',(-22.6559177133127,-7.66880399241322,
0.));
#199124=CARTESIAN_POINT('Ctrl Pts',(-22.6769390009885,-7.66849860491742,
0.));
#199125=CARTESIAN_POINT('Ctrl Pts',(-22.6980622655446,-7.66813626029274,
0.));
#199126=CARTESIAN_POINT('Ctrl Pts',(-22.7192867206245,-7.66771657191027,
0.));
#199127=CARTESIAN_POINT('Ctrl Pts',(-22.7406115879513,-7.66723915895439,
0.));
#199128=CARTESIAN_POINT('Ctrl Pts',(-22.7620360971843,-7.66670364630298,
0.));
#199129=CARTESIAN_POINT('Ctrl Pts',(-22.7835594857699,-7.66610966441272,
0.));
#199130=CARTESIAN_POINT('Ctrl Pts',(-22.8051809987833,-7.66545684920987,
0.));
#199131=CARTESIAN_POINT('Ctrl Pts',(-22.8268998887678,-7.66474484198548,
0.));
#199132=CARTESIAN_POINT('Ctrl Pts',(-22.848715415557,-7.66397328929802,
0.));
#199133=CARTESIAN_POINT('Ctrl Pts',(-22.8706268461283,-7.66314184287336,
0.));
#199134=CARTESIAN_POINT('Ctrl Pts',(-22.8926334544883,-7.66225015950155,
0.));
#199135=CARTESIAN_POINT('Ctrl Pts',(-22.9147345215421,-7.66129790094107,
0.));
#199136=CARTESIAN_POINT('Ctrl Pts',(-22.9369293349593,-7.66028473382777,
0.));
#199137=CARTESIAN_POINT('Ctrl Pts',(-22.959217189033,-7.65921032958901,
0.));
#199138=CARTESIAN_POINT('Ctrl Pts',(-22.9815973845296,-7.65807436436431,
0.));
#199139=CARTESIAN_POINT('Ctrl Pts',(-23.0040692285814,-7.65687651891304,
0.));
#199140=CARTESIAN_POINT('Ctrl Pts',(-23.0266320345787,-7.65561647852533,
0.));
#199141=CARTESIAN_POINT('Ctrl Pts',(-23.0492851220528,-7.65429393293945,
0.));
#199142=CARTESIAN_POINT('Ctrl Pts',(-23.072027816555,-7.65290857626357,
0.));
#199143=CARTESIAN_POINT('Ctrl Pts',(-23.094859449525,-7.65146010690475,
0.));
#199144=CARTESIAN_POINT('Ctrl Pts',(-23.1177793581679,-7.64994822749859,
0.));
#199145=CARTESIAN_POINT('Ctrl Pts',(-23.1407868853819,-7.64837264482942,
0.));
#199146=CARTESIAN_POINT('Ctrl Pts',(-23.1638813796694,-7.64673306975804,
0.));
#199147=CARTESIAN_POINT('Ctrl Pts',(-23.1870621950452,-7.64502921715482,
0.));
#199148=CARTESIAN_POINT('Ctrl Pts',(-23.2103286909398,-7.64326080583679,
0.));
#199149=CARTESIAN_POINT('Ctrl Pts',(-23.2336802320912,-7.64142755851504,
0.));
#199150=CARTESIAN_POINT('Ctrl Pts',(-23.2571161884488,-7.63952920172835,
0.));
#199151=CARTESIAN_POINT('Ctrl Pts',(-23.2806359350855,-7.63756546576374,
0.));
#199152=CARTESIAN_POINT('Ctrl Pts',(-23.3042388521022,-7.63553608458782,
0.));
#199153=CARTESIAN_POINT('Ctrl Pts',(-23.3279243245241,-7.63344079578161,
0.));
#199154=CARTESIAN_POINT('Ctrl Pts',(-23.3516917421972,-7.63127934048136,
0.));
#199155=CARTESIAN_POINT('Ctrl Pts',(-23.3755404996636,-7.62905146332592,
0.));
#199156=CARTESIAN_POINT('Ctrl Pts',(-23.399469996112,-7.62675691240328,
0.));
#199157=CARTESIAN_POINT('Ctrl Pts',(-23.4234796353542,-7.62439543920049,
0.));
#199158=CARTESIAN_POINT('Ctrl Pts',(-23.4475688257854,-7.62196679855954,
0.));
#199159=CARTESIAN_POINT('Ctrl Pts',(-23.4717369803438,-7.61947074863976,
0.));
#199160=CARTESIAN_POINT('Ctrl Pts',(-23.4959835164609,-7.61690705088318,
0.));
#199161=CARTESIAN_POINT('Ctrl Pts',(-23.5203078560129,-7.61427546999297,
0.));
#199162=CARTESIAN_POINT('Ctrl Pts',(-23.544709425203,-7.61157577385371,
0.));
#199163=CARTESIAN_POINT('Ctrl Pts',(-23.5691876544244,-7.60880773344599,
0.));
#199164=CARTESIAN_POINT('Ctrl Pts',(-23.5937419781245,-7.60597112277093,
0.));
#199165=CARTESIAN_POINT('Ctrl Pts',(-23.6183718346576,-7.60306571877805,
0.));
#199166=CARTESIAN_POINT('Ctrl Pts',(-23.6430766661418,-7.60009130130125,
0.));
#199167=CARTESIAN_POINT('Ctrl Pts',(-23.6678559182875,-7.59704765299566,
0.));
#199168=CARTESIAN_POINT('Ctrl Pts',(-23.6927090405066,-7.59393455934034,
0.));
#199169=CARTESIAN_POINT('Ctrl Pts',(-23.7176354860457,-7.5907518086532,
0.));
#199170=CARTESIAN_POINT('Ctrl Pts',(-23.7426347121006,-7.58749919210825,
0.));
#199171=CARTESIAN_POINT('Ctrl Pts',(-23.7677061799376,-7.5841765037627,
0.));
#199172=CARTESIAN_POINT('Ctrl Pts',(-23.7928493549908,-7.58078354058212,
0.));
#199173=CARTESIAN_POINT('Ctrl Pts',(-23.8180637069976,-7.57732010249065,
0.));
#199174=CARTESIAN_POINT('Ctrl Pts',(-23.8433487096132,-7.57378599219814,
0.));
#199175=CARTESIAN_POINT('Ctrl Pts',(-23.8687038399595,-7.57018101500709,
0.));
#199176=CARTESIAN_POINT('Ctrl Pts',(-23.8941285782002,-7.5665049786379,
0.));
#199177=CARTESIAN_POINT('Ctrl Pts',(-23.9196224070759,-7.56275769304772,
0.));
#199178=CARTESIAN_POINT('Ctrl Pts',(-23.9451848115002,-7.55893897027679,
0.));
#199179=CARTESIAN_POINT('Ctrl Pts',(-23.9708152779886,-7.55504862424807,
0.));
#199180=CARTESIAN_POINT('Ctrl Pts',(-23.9965132953187,-7.55108647097431,
0.));
#199181=CARTESIAN_POINT('Ctrl Pts',(-24.0222783554531,-7.54705232885894,
0.));
#199182=CARTESIAN_POINT('Ctrl Pts',(-24.0481099543353,-7.54294601896127,
0.));
#199183=CARTESIAN_POINT('Ctrl Pts',(-24.0740075927984,-7.53876736531004,
0.));
#199184=CARTESIAN_POINT('Ctrl Pts',(-24.0999707772643,-7.53451619514658,
0.));
#199185=CARTESIAN_POINT('Ctrl Pts',(-24.1259990209211,-7.53019233935536,
0.));
#199186=CARTESIAN_POINT('Ctrl Pts',(-24.152091842537,-7.52579563201478,
0.));
#199187=CARTESIAN_POINT('Ctrl Pts',(-24.1782487641602,-7.52132590953862,
0.));
#199188=CARTESIAN_POINT('Ctrl Pts',(-24.2044693092356,-7.51678300997997,
0.));
#199189=CARTESIAN_POINT('Ctrl Pts',(-24.230753000389,-7.51216677222198,
0.));
#199190=CARTESIAN_POINT('Ctrl Pts',(-24.2570993577032,-7.50747703535114,
0.));
#199191=CARTESIAN_POINT('Ctrl Pts',(-24.2835078958966,-7.50271363765098,
0.));
#199192=CARTESIAN_POINT('Ctrl Pts',(-24.3099781253345,-7.49787641695358,
0.));
#199193=CARTESIAN_POINT('Ctrl Pts',(-24.3365095573673,-7.49296521252329,
0.));
#199194=CARTESIAN_POINT('Ctrl Pts',(-24.3631017084513,-7.48797986651827,
0.));
#199195=CARTESIAN_POINT('Ctrl Pts',(-24.3897541049248,-7.48292022569253,
0.));
#199196=CARTESIAN_POINT('Ctrl Pts',(-24.4164662871165,-7.47778614286573,
0.));
#199197=CARTESIAN_POINT('Ctrl Pts',(-24.4432378146501,-7.47257747883318,
0.));
#199198=CARTESIAN_POINT('Ctrl Pts',(-24.4700682684544,-7.46729410308922,
0.));
#199199=CARTESIAN_POINT('Ctrl Pts',(-24.4969572391509,-7.46193588961641,
0.));
#199200=CARTESIAN_POINT('Ctrl Pts',(-24.52390431731,-7.45650271336045,0.));
#199201=CARTESIAN_POINT('Ctrl Pts',(-24.5509090831579,-7.45099444651295,
0.));
#199202=CARTESIAN_POINT('Ctrl Pts',(-24.5779710960865,-7.44541095473162,
0.));
#199203=CARTESIAN_POINT('Ctrl Pts',(-24.6050898852349,-7.43975209375374,
0.));
#199204=CARTESIAN_POINT('Ctrl Pts',(-24.6322649369472,-7.4340177048922,
0.));
#199205=CARTESIAN_POINT('Ctrl Pts',(-24.659495712869,-7.4282076215868,0.));
#199206=CARTESIAN_POINT('Ctrl Pts',(-24.6867816727118,-7.42232167765762,
0.));
#199207=CARTESIAN_POINT('Ctrl Pts',(-24.7141222949988,-7.41635971481243,
0.));
#199208=CARTESIAN_POINT('Ctrl Pts',(-24.7415170994754,-7.41032159082173,
0.));
#199209=CARTESIAN_POINT('Ctrl Pts',(-24.7689656669005,-7.40420718661754,
0.));
#199210=CARTESIAN_POINT('Ctrl Pts',(-24.7964676646518,-7.39801641583612,
0.));
#199211=CARTESIAN_POINT('Ctrl Pts',(-24.8240228521042,-7.39174922586841,
0.));
#199212=CARTESIAN_POINT('Ctrl Pts',(-24.8516310625367,-7.38540558904945,
0.));
#199213=CARTESIAN_POINT('Ctrl Pts',(-24.8792921911309,-7.3789854964161,
0.));
#199214=CARTESIAN_POINT('Ctrl Pts',(-24.9014633826201,-7.37378825962717,
0.));
#199215=CARTESIAN_POINT('Ctrl Pts',(-24.9181155530631,-7.36985593120696,
0.));
#199216=CARTESIAN_POINT('Ctrl Pts',(-24.9292275670705,-7.36721909029059,
0.));
#199217=CARTESIAN_POINT('Ctrl Pts',(-24.9347862158358,-7.36589684767343,
0.));
#199218=CARTESIAN_POINT('',(-24.9347862158358,-7.36589684767343,0.));
#199219=CARTESIAN_POINT('Origin',(-21.4341755315424,-1.68110656504246,0.));
#199220=CARTESIAN_POINT('',(-22.4835757167854,-1.76341220531179,0.));
#199221=CARTESIAN_POINT('',(-22.4835757167854,-1.76341220531179,0.));
#199222=CARTESIAN_POINT('',(-10.7170877657712,-0.840553282521227,0.));
#199223=CARTESIAN_POINT('Ctrl Pts',(-25.2771067246846,-6.08833931617698,
0.));
#199224=CARTESIAN_POINT('Ctrl Pts',(-25.2771067246846,-6.08833931617698,
12.));
#199225=CARTESIAN_POINT('Ctrl Pts',(-25.2729539149479,-6.08441489609824,
0.));
#199226=CARTESIAN_POINT('Ctrl Pts',(-25.2729539149479,-6.08441489609824,
12.));
#199227=CARTESIAN_POINT('Ctrl Pts',(-25.2646490489816,-6.07657531787577,
0.));
#199228=CARTESIAN_POINT('Ctrl Pts',(-25.2646490489816,-6.07657531787577,
12.));
#199229=CARTESIAN_POINT('Ctrl Pts',(-25.2521940105523,-6.06484373634696,
0.));
#199230=CARTESIAN_POINT('Ctrl Pts',(-25.2521940105523,-6.06484373634696,
12.));
#199231=CARTESIAN_POINT('Ctrl Pts',(-25.2355918138798,-6.04925720151412,
0.));
#199232=CARTESIAN_POINT('Ctrl Pts',(-25.2355918138798,-6.04925720151412,
12.));
#199233=CARTESIAN_POINT('Ctrl Pts',(-25.2148466201368,-6.02986667390187,
0.));
#199234=CARTESIAN_POINT('Ctrl Pts',(-25.2148466201368,-6.02986667390187,
12.));
#199235=CARTESIAN_POINT('Ctrl Pts',(-25.1941090269638,-6.0105688180476,
0.));
#199236=CARTESIAN_POINT('Ctrl Pts',(-25.1941090269638,-6.0105688180476,
12.));
#199237=CARTESIAN_POINT('Ctrl Pts',(-25.1733791296154,-5.99136367859838,
0.));
#199238=CARTESIAN_POINT('Ctrl Pts',(-25.1733791296154,-5.99136367859838,
12.));
#199239=CARTESIAN_POINT('Ctrl Pts',(-25.1526570863065,-5.97225131495636,
0.));
#199240=CARTESIAN_POINT('Ctrl Pts',(-25.1526570863065,-5.97225131495636,
12.));
#199241=CARTESIAN_POINT('Ctrl Pts',(-25.1319431317273,-5.95323180187348,
0.));
#199242=CARTESIAN_POINT('Ctrl Pts',(-25.1319431317273,-5.95323180187348,
12.));
#199243=CARTESIAN_POINT('Ctrl Pts',(-25.1112375971182,-5.93430523086776,
0.));
#199244=CARTESIAN_POINT('Ctrl Pts',(-25.1112375971182,-5.93430523086776,
12.));
#199245=CARTESIAN_POINT('Ctrl Pts',(-25.0905409050863,-5.91547170844382,
0.));
#199246=CARTESIAN_POINT('Ctrl Pts',(-25.0905409050863,-5.91547170844382,
12.));
#199247=CARTESIAN_POINT('Ctrl Pts',(-25.0698535426593,-5.89673135155459,
0.));
#199248=CARTESIAN_POINT('Ctrl Pts',(-25.0698535426593,-5.89673135155459,
12.));
#199249=CARTESIAN_POINT('Ctrl Pts',(-25.0491760405965,-5.87808428385329,
0.));
#199250=CARTESIAN_POINT('Ctrl Pts',(-25.0491760405965,-5.87808428385329,
12.));
#199251=CARTESIAN_POINT('Ctrl Pts',(-25.0285089498922,-5.8595306315681,
0.));
#199252=CARTESIAN_POINT('Ctrl Pts',(-25.0285089498922,-5.8595306315681,
12.));
#199253=CARTESIAN_POINT('Ctrl Pts',(-25.0078528200558,-5.84107051963073,
0.));
#199254=CARTESIAN_POINT('Ctrl Pts',(-25.0078528200558,-5.84107051963073,
12.));
#199255=CARTESIAN_POINT('Ctrl Pts',(-24.9872081752709,-5.82270406744214,
0.));
#199256=CARTESIAN_POINT('Ctrl Pts',(-24.9872081752709,-5.82270406744214,
12.));
#199257=CARTESIAN_POINT('Ctrl Pts',(-24.9665754954462,-5.80443138549747,
0.));
#199258=CARTESIAN_POINT('Ctrl Pts',(-24.9665754954462,-5.80443138549747,
12.));
#199259=CARTESIAN_POINT('Ctrl Pts',(-24.9459552293308,-5.78625257775703,
0.));
#199260=CARTESIAN_POINT('Ctrl Pts',(-24.9459552293308,-5.78625257775703,
12.));
#199261=CARTESIAN_POINT('Ctrl Pts',(-24.9253478043632,-5.76816774342236,
0.));
#199262=CARTESIAN_POINT('Ctrl Pts',(-24.9253478043632,-5.76816774342236,
12.));
#199263=CARTESIAN_POINT('Ctrl Pts',(-24.9047536376467,-5.75017697890813,
0.));
#199264=CARTESIAN_POINT('Ctrl Pts',(-24.9047536376467,-5.75017697890813,
12.));
#199265=CARTESIAN_POINT('Ctrl Pts',(-24.8841731467219,-5.73228037976926,
0.));
#199266=CARTESIAN_POINT('Ctrl Pts',(-24.8841731467219,-5.73228037976926,
12.));
#199267=CARTESIAN_POINT('Ctrl Pts',(-24.8636067597677,-5.71447804252019,
0.));
#199268=CARTESIAN_POINT('Ctrl Pts',(-24.8636067597677,-5.71447804252019,
12.));
#199269=CARTESIAN_POINT('Ctrl Pts',(-24.8430549277634,-5.69677006679429,
0.));
#199270=CARTESIAN_POINT('Ctrl Pts',(-24.8430549277634,-5.69677006679429,
12.));
#199271=CARTESIAN_POINT('Ctrl Pts',(-24.822518122386,-5.67915655496524,
0.));
#199272=CARTESIAN_POINT('Ctrl Pts',(-24.822518122386,-5.67915655496524,
12.));
#199273=CARTESIAN_POINT('Ctrl Pts',(-24.8019968304618,-5.66163761114903,
0.));
#199274=CARTESIAN_POINT('Ctrl Pts',(-24.8019968304618,-5.66163761114903,
12.));
#199275=CARTESIAN_POINT('Ctrl Pts',(-24.7814915496728,-5.64421334042247,
0.));
#199276=CARTESIAN_POINT('Ctrl Pts',(-24.7814915496728,-5.64421334042247,
12.));
#199277=CARTESIAN_POINT('Ctrl Pts',(-24.76100278357,-5.62688384790919,0.));
#199278=CARTESIAN_POINT('Ctrl Pts',(-24.76100278357,-5.62688384790919,12.));
#199279=CARTESIAN_POINT('Ctrl Pts',(-24.7405310372736,-5.60964923798495,
0.));
#199280=CARTESIAN_POINT('Ctrl Pts',(-24.7405310372736,-5.60964923798495,
12.));
#199281=CARTESIAN_POINT('Ctrl Pts',(-24.7200768119079,-5.59250961323995,
0.));
#199282=CARTESIAN_POINT('Ctrl Pts',(-24.7200768119079,-5.59250961323995,
12.));
#199283=CARTESIAN_POINT('Ctrl Pts',(-24.6996406035507,-5.57546507427766,
0.));
#199284=CARTESIAN_POINT('Ctrl Pts',(-24.6996406035507,-5.57546507427766,
12.));
#199285=CARTESIAN_POINT('Ctrl Pts',(-24.6792229061785,-5.55851572025389,
0.));
#199286=CARTESIAN_POINT('Ctrl Pts',(-24.6792229061785,-5.55851572025389,
12.));
#199287=CARTESIAN_POINT('Ctrl Pts',(-24.6588242134733,-5.54166164919593,
0.));
#199288=CARTESIAN_POINT('Ctrl Pts',(-24.6588242134733,-5.54166164919593,
12.));
#199289=CARTESIAN_POINT('Ctrl Pts',(-24.6384450211466,-5.52490295840996,
0.));
#199290=CARTESIAN_POINT('Ctrl Pts',(-24.6384450211466,-5.52490295840996,
12.));
#199291=CARTESIAN_POINT('Ctrl Pts',(-24.618085828918,-5.50823974481959,
0.));
#199292=CARTESIAN_POINT('Ctrl Pts',(-24.618085828918,-5.50823974481959,
12.));
#199293=CARTESIAN_POINT('Ctrl Pts',(-24.5977471429365,-5.49167210537235,
0.));
#199294=CARTESIAN_POINT('Ctrl Pts',(-24.5977471429365,-5.49167210537235,
12.));
#199295=CARTESIAN_POINT('Ctrl Pts',(-24.5774294770329,-5.47520013724403,
0.));
#199296=CARTESIAN_POINT('Ctrl Pts',(-24.5774294770329,-5.47520013724403,
12.));
#199297=CARTESIAN_POINT('Ctrl Pts',(-24.5571333514841,-5.45882393762244,
0.));
#199298=CARTESIAN_POINT('Ctrl Pts',(-24.5571333514841,-5.45882393762244,
12.));
#199299=CARTESIAN_POINT('Ctrl Pts',(-24.5368592922861,-5.44254360356865,
0.));
#199300=CARTESIAN_POINT('Ctrl Pts',(-24.5368592922861,-5.44254360356865,
12.));
#199301=CARTESIAN_POINT('Ctrl Pts',(-24.5166078302107,-5.42635923183411,
0.));
#199302=CARTESIAN_POINT('Ctrl Pts',(-24.5166078302107,-5.42635923183411,
12.));
#199303=CARTESIAN_POINT('Ctrl Pts',(-24.4963794999831,-5.41027091869242,
0.));
#199304=CARTESIAN_POINT('Ctrl Pts',(-24.4963794999831,-5.41027091869242,
12.));
#199305=CARTESIAN_POINT('Ctrl Pts',(-24.4761748393322,-5.3942787597383,
0.));
#199306=CARTESIAN_POINT('Ctrl Pts',(-24.4761748393322,-5.3942787597383,
12.));
#199307=CARTESIAN_POINT('Ctrl Pts',(-24.4559943883159,-5.37838284973706,
0.));
#199308=CARTESIAN_POINT('Ctrl Pts',(-24.4559943883159,-5.37838284973706,
12.));
#199309=CARTESIAN_POINT('Ctrl Pts',(-24.4358386899152,-5.36258328273639,
0.));
#199310=CARTESIAN_POINT('Ctrl Pts',(-24.4358386899152,-5.36258328273639,
12.));
#199311=CARTESIAN_POINT('Ctrl Pts',(-24.4157082904615,-5.34688015213546,
0.));
#199312=CARTESIAN_POINT('Ctrl Pts',(-24.4157082904615,-5.34688015213546,
12.));
#199313=CARTESIAN_POINT('Ctrl Pts',(-24.3956037401293,-5.33127355076036,
0.));
#199314=CARTESIAN_POINT('Ctrl Pts',(-24.3956037401293,-5.33127355076036,
12.));
#199315=CARTESIAN_POINT('Ctrl Pts',(-24.3755255933917,-5.31576357092524,
0.));
#199316=CARTESIAN_POINT('Ctrl Pts',(-24.3755255933917,-5.31576357092524,
12.));
#199317=CARTESIAN_POINT('Ctrl Pts',(-24.3554744095075,-5.30035030449058,
0.));
#199318=CARTESIAN_POINT('Ctrl Pts',(-24.3554744095075,-5.30035030449058,
12.));
#199319=CARTESIAN_POINT('Ctrl Pts',(-24.3354507529415,-5.28503384290644,
0.));
#199320=CARTESIAN_POINT('Ctrl Pts',(-24.3354507529415,-5.28503384290644,
12.));
#199321=CARTESIAN_POINT('Ctrl Pts',(-24.3154551932222,-5.26981427718796,
0.));
#199322=CARTESIAN_POINT('Ctrl Pts',(-24.3154551932222,-5.26981427718796,
12.));
#199323=CARTESIAN_POINT('Ctrl Pts',(-24.2954883048448,-5.25469169788856,
0.));
#199324=CARTESIAN_POINT('Ctrl Pts',(-24.2954883048448,-5.25469169788856,
12.));
#199325=CARTESIAN_POINT('Ctrl Pts',(-24.2755506671526,-5.23966619506289,
0.));
#199326=CARTESIAN_POINT('Ctrl Pts',(-24.2755506671526,-5.23966619506289,
12.));
#199327=CARTESIAN_POINT('Ctrl Pts',(-24.2556428642294,-5.22473785822441,
0.));
#199328=CARTESIAN_POINT('Ctrl Pts',(-24.2556428642294,-5.22473785822441,
12.));
#199329=CARTESIAN_POINT('Ctrl Pts',(-24.2357654847765,-5.20990677629173,
0.));
#199330=CARTESIAN_POINT('Ctrl Pts',(-24.2357654847765,-5.20990677629173,
12.));
#199331=CARTESIAN_POINT('Ctrl Pts',(-24.215919122017,-5.19517303753643,
0.));
#199332=CARTESIAN_POINT('Ctrl Pts',(-24.215919122017,-5.19517303753643,
12.));
#199333=CARTESIAN_POINT('Ctrl Pts',(-24.1961043738754,-5.18053672961392,
0.));
#199334=CARTESIAN_POINT('Ctrl Pts',(-24.1961043738754,-5.18053672961392,
12.));
#199335=CARTESIAN_POINT('Ctrl Pts',(-24.1763218431343,-5.16599793957979,
0.));
#199336=CARTESIAN_POINT('Ctrl Pts',(-24.1763218431343,-5.16599793957979,
12.));
#199337=CARTESIAN_POINT('Ctrl Pts',(-24.156572137597,-5.15155675390075,
0.));
#199338=CARTESIAN_POINT('Ctrl Pts',(-24.156572137597,-5.15155675390075,
12.));
#199339=CARTESIAN_POINT('Ctrl Pts',(-24.1368558702443,-5.13721325845744,
0.));
#199340=CARTESIAN_POINT('Ctrl Pts',(-24.1368558702443,-5.13721325845744,
12.));
#199341=CARTESIAN_POINT('Ctrl Pts',(-24.117173659394,-5.12296753853859,
0.));
#199342=CARTESIAN_POINT('Ctrl Pts',(-24.117173659394,-5.12296753853859,
12.));
#199343=CARTESIAN_POINT('Ctrl Pts',(-24.0975261288446,-5.10881967883132,
0.));
#199344=CARTESIAN_POINT('Ctrl Pts',(-24.0975261288446,-5.10881967883132,
12.));
#199345=CARTESIAN_POINT('Ctrl Pts',(-24.0779139079266,-5.09476976342625,
0.));
#199346=CARTESIAN_POINT('Ctrl Pts',(-24.0779139079266,-5.09476976342625,
12.));
#199347=CARTESIAN_POINT('Ctrl Pts',(-24.0583376315638,-5.08081787581276,
0.));
#199348=CARTESIAN_POINT('Ctrl Pts',(-24.0583376315638,-5.08081787581276,
12.));
#199349=CARTESIAN_POINT('Ctrl Pts',(-24.0387979403268,-5.06696409886641,
0.));
#199350=CARTESIAN_POINT('Ctrl Pts',(-24.0387979403268,-5.06696409886641,
12.));
#199351=CARTESIAN_POINT('Ctrl Pts',(-24.0192954804896,-5.05320851483065,
0.));
#199352=CARTESIAN_POINT('Ctrl Pts',(-24.0192954804896,-5.05320851483065,
12.));
#199353=CARTESIAN_POINT('Ctrl Pts',(-23.9998309040746,-5.03955120528521,
0.));
#199354=CARTESIAN_POINT('Ctrl Pts',(-23.9998309040746,-5.03955120528521,
12.));
#199355=CARTESIAN_POINT('Ctrl Pts',(-23.9804048689227,-5.02599225112454,
0.));
#199356=CARTESIAN_POINT('Ctrl Pts',(-23.9804048689227,-5.02599225112454,
12.));
#199357=CARTESIAN_POINT('Ctrl Pts',(-23.9610180388271,-5.01253173257453,
0.));
#199358=CARTESIAN_POINT('Ctrl Pts',(-23.9610180388271,-5.01253173257453,
12.));
#199359=CARTESIAN_POINT('Ctrl Pts',(-23.9416710836529,-4.99916972919306,
0.));
#199360=CARTESIAN_POINT('Ctrl Pts',(-23.9416710836529,-4.99916972919306,
12.));
#199361=CARTESIAN_POINT('Ctrl Pts',(-23.9223646794592,-4.98590631986532,
0.));
#199362=CARTESIAN_POINT('Ctrl Pts',(-23.9223646794592,-4.98590631986532,
12.));
#199363=CARTESIAN_POINT('Ctrl Pts',(-23.9030995086163,-4.97274158279226,
0.));
#199364=CARTESIAN_POINT('Ctrl Pts',(-23.9030995086163,-4.97274158279226,
12.));
#199365=CARTESIAN_POINT('Ctrl Pts',(-23.8838762599218,-4.9596755954656,
0.));
#199366=CARTESIAN_POINT('Ctrl Pts',(-23.8838762599218,-4.9596755954656,
12.));
#199367=CARTESIAN_POINT('Ctrl Pts',(-23.8646956287168,-4.9467084346586,
0.));
#199368=CARTESIAN_POINT('Ctrl Pts',(-23.8646956287168,-4.9467084346586,
12.));
#199369=CARTESIAN_POINT('Ctrl Pts',(-23.8455583170057,-4.93384017643432,
0.));
#199370=CARTESIAN_POINT('Ctrl Pts',(-23.8455583170057,-4.93384017643432,
12.));
#199371=CARTESIAN_POINT('Ctrl Pts',(-23.8264650335717,-4.92107089613969,
0.));
#199372=CARTESIAN_POINT('Ctrl Pts',(-23.8264650335717,-4.92107089613969,
12.));
#199373=CARTESIAN_POINT('Ctrl Pts',(-23.8074164940896,-4.90840066839344,
0.));
#199374=CARTESIAN_POINT('Ctrl Pts',(-23.8074164940896,-4.90840066839344,
12.));
#199375=CARTESIAN_POINT('Ctrl Pts',(-23.7884134212384,-4.89582956706775,
0.));
#199376=CARTESIAN_POINT('Ctrl Pts',(-23.7884134212384,-4.89582956706775,
12.));
#199377=CARTESIAN_POINT('Ctrl Pts',(-23.7694565448049,-4.88335766525573,
0.));
#199378=CARTESIAN_POINT('Ctrl Pts',(-23.7694565448049,-4.88335766525573,
12.));
#199379=CARTESIAN_POINT('Ctrl Pts',(-23.7505466018245,-4.87098503527152,
0.));
#199380=CARTESIAN_POINT('Ctrl Pts',(-23.7505466018245,-4.87098503527152,
12.));
#199381=CARTESIAN_POINT('Ctrl Pts',(-23.7316843367313,-4.85871174865499,
0.));
#199382=CARTESIAN_POINT('Ctrl Pts',(-23.7316843367313,-4.85871174865499,
12.));
#199383=CARTESIAN_POINT('Ctrl Pts',(-23.7128705015017,-4.84653787616425,
0.));
#199384=CARTESIAN_POINT('Ctrl Pts',(-23.7128705015017,-4.84653787616425,
12.));
#199385=CARTESIAN_POINT('Ctrl Pts',(-23.6941058557971,-4.83446348776265,
0.));
#199386=CARTESIAN_POINT('Ctrl Pts',(-23.6941058557971,-4.83446348776265,
12.));
#199387=CARTESIAN_POINT('Ctrl Pts',(-23.675391167102,-4.82248865259562,
0.));
#199388=CARTESIAN_POINT('Ctrl Pts',(-23.675391167102,-4.82248865259562,
12.));
#199389=CARTESIAN_POINT('Ctrl Pts',(-23.6567272108628,-4.81061343896432,
0.));
#199390=CARTESIAN_POINT('Ctrl Pts',(-23.6567272108628,-4.81061343896432,
12.));
#199391=CARTESIAN_POINT('Ctrl Pts',(-23.6381147706579,-4.7988379143322,
0.));
#199392=CARTESIAN_POINT('Ctrl Pts',(-23.6381147706579,-4.7988379143322,
12.));
#199393=CARTESIAN_POINT('Ctrl Pts',(-23.6195546383624,-4.78716214532098,
0.));
#199394=CARTESIAN_POINT('Ctrl Pts',(-23.6195546383624,-4.78716214532098,
12.));
#199395=CARTESIAN_POINT('Ctrl Pts',(-23.6010476143099,-4.77558619769872,
0.));
#199396=CARTESIAN_POINT('Ctrl Pts',(-23.6010476143099,-4.77558619769872,
12.));
#199397=CARTESIAN_POINT('Ctrl Pts',(-23.5825945074535,-4.76411013636251,
0.));
#199398=CARTESIAN_POINT('Ctrl Pts',(-23.5825945074535,-4.76411013636251,
12.));
#199399=CARTESIAN_POINT('Ctrl Pts',(-23.5641961355168,-4.75273402530617,
0.));
#199400=CARTESIAN_POINT('Ctrl Pts',(-23.5641961355168,-4.75273402530617,
12.));
#199401=CARTESIAN_POINT('Ctrl Pts',(-23.545853325171,-4.74145792760698,
0.));
#199402=CARTESIAN_POINT('Ctrl Pts',(-23.545853325171,-4.74145792760698,
12.));
#199403=CARTESIAN_POINT('Ctrl Pts',(-23.5275669122372,-4.7302819054303,
0.));
#199404=CARTESIAN_POINT('Ctrl Pts',(-23.5275669122372,-4.7302819054303,
12.));
#199405=CARTESIAN_POINT('Ctrl Pts',(-23.509337741878,-4.71920602001901,
0.));
#199406=CARTESIAN_POINT('Ctrl Pts',(-23.509337741878,-4.71920602001901,
12.));
#199407=CARTESIAN_POINT('Ctrl Pts',(-23.491166668789,-4.70823033167818,
0.));
#199408=CARTESIAN_POINT('Ctrl Pts',(-23.491166668789,-4.70823033167818,
12.));
#199409=CARTESIAN_POINT('Ctrl Pts',(-23.4730545573853,-4.69735489975024,
0.));
#199410=CARTESIAN_POINT('Ctrl Pts',(-23.4730545573853,-4.69735489975024,
12.));
#199411=CARTESIAN_POINT('Ctrl Pts',(-23.455002281986,-4.68657978258303,
0.));
#199412=CARTESIAN_POINT('Ctrl Pts',(-23.455002281986,-4.68657978258303,
12.));
#199413=CARTESIAN_POINT('Ctrl Pts',(-23.4370107270451,-4.67590503753058,
0.));
#199414=CARTESIAN_POINT('Ctrl Pts',(-23.4370107270451,-4.67590503753058,
12.));
#199415=CARTESIAN_POINT('Ctrl Pts',(-23.4190807873803,-4.6653307209467,
0.));
#199416=CARTESIAN_POINT('Ctrl Pts',(-23.4190807873803,-4.6653307209467,
12.));
#199417=CARTESIAN_POINT('Ctrl Pts',(-23.4012133683959,-4.65485688816924,
0.));
#199418=CARTESIAN_POINT('Ctrl Pts',(-23.4012133683959,-4.65485688816924,
12.));
#199419=CARTESIAN_POINT('Ctrl Pts',(-23.3834093863068,-4.6444835934993,
0.));
#199420=CARTESIAN_POINT('Ctrl Pts',(-23.3834093863068,-4.6444835934993,
12.));
#199421=CARTESIAN_POINT('Ctrl Pts',(-23.3656697683489,-4.63421089016541,
0.));
#199422=CARTESIAN_POINT('Ctrl Pts',(-23.3656697683489,-4.63421089016541,
12.));
#199423=CARTESIAN_POINT('Ctrl Pts',(-23.3479954530272,-4.62403883030805,
0.));
#199424=CARTESIAN_POINT('Ctrl Pts',(-23.3479954530272,-4.62403883030805,
12.));
#199425=CARTESIAN_POINT('Ctrl Pts',(-23.3303873903938,-4.6139674649783,
0.));
#199426=CARTESIAN_POINT('Ctrl Pts',(-23.3303873903938,-4.6139674649783,
12.));
#199427=CARTESIAN_POINT('Ctrl Pts',(-23.3128465423115,-4.60399684412163,
0.));
#199428=CARTESIAN_POINT('Ctrl Pts',(-23.3128465423115,-4.60399684412163,
12.));
#199429=CARTESIAN_POINT('Ctrl Pts',(-23.2953738827191,-4.5941270165575,
0.));
#199430=CARTESIAN_POINT('Ctrl Pts',(-23.2953738827191,-4.5941270165575,
12.));
#199431=CARTESIAN_POINT('Ctrl Pts',(-23.2779703978876,-4.5843580299469,
0.));
#199432=CARTESIAN_POINT('Ctrl Pts',(-23.2779703978876,-4.5843580299469,
12.));
#199433=CARTESIAN_POINT('Ctrl Pts',(-23.2606370866866,-4.57468993076097,
0.));
#199434=CARTESIAN_POINT('Ctrl Pts',(-23.2606370866866,-4.57468993076097,
12.));
#199435=CARTESIAN_POINT('Ctrl Pts',(-23.2433749609131,-4.56512276427839,
0.));
#199436=CARTESIAN_POINT('Ctrl Pts',(-23.2433749609131,-4.56512276427839,
12.));
#199437=CARTESIAN_POINT('Ctrl Pts',(-23.2261850456064,-4.55565657456975,
0.));
#199438=CARTESIAN_POINT('Ctrl Pts',(-23.2261850456064,-4.55565657456975,
12.));
#199439=CARTESIAN_POINT('Ctrl Pts',(-23.2090683793629,-4.54629140447544,
0.));
#199440=CARTESIAN_POINT('Ctrl Pts',(-23.2090683793629,-4.54629140447544,
12.));
#199441=CARTESIAN_POINT('Ctrl Pts',(-23.1920260146465,-4.53702729557566,
0.));
#199442=CARTESIAN_POINT('Ctrl Pts',(-23.1920260146465,-4.53702729557566,
12.));
#199443=CARTESIAN_POINT('Ctrl Pts',(-23.1750590180908,-4.52786428815014,
0.));
#199444=CARTESIAN_POINT('Ctrl Pts',(-23.1750590180908,-4.52786428815014,
12.));
#199445=CARTESIAN_POINT('Ctrl Pts',(-23.1581684708761,-4.51880242116748,
0.));
#199446=CARTESIAN_POINT('Ctrl Pts',(-23.1581684708761,-4.51880242116748,
12.));
#199447=CARTESIAN_POINT('Ctrl Pts',(-23.1413554691123,-4.5098417322706,
0.));
#199448=CARTESIAN_POINT('Ctrl Pts',(-23.1413554691123,-4.5098417322706,
12.));
#199449=CARTESIAN_POINT('Ctrl Pts',(-23.1246211242115,-4.50098225775171,
0.));
#199450=CARTESIAN_POINT('Ctrl Pts',(-23.1246211242115,-4.50098225775171,
12.));
#199451=CARTESIAN_POINT('Ctrl Pts',(-23.1079665632636,-4.49222403252216,
0.));
#199452=CARTESIAN_POINT('Ctrl Pts',(-23.1079665632636,-4.49222403252216,
12.));
#199453=CARTESIAN_POINT('Ctrl Pts',(-23.0913929293922,-4.48356709006788,
0.));
#199454=CARTESIAN_POINT('Ctrl Pts',(-23.0913929293922,-4.48356709006788,
12.));
#199455=CARTESIAN_POINT('Ctrl Pts',(-23.0749013821881,-4.47501146242856,
0.));
#199456=CARTESIAN_POINT('Ctrl Pts',(-23.0749013821881,-4.47501146242856,
12.));
#199457=CARTESIAN_POINT('Ctrl Pts',(-23.0584930981732,-4.4665571801823,
0.));
#199458=CARTESIAN_POINT('Ctrl Pts',(-23.0584930981732,-4.4665571801823,
12.));
#199459=CARTESIAN_POINT('Ctrl Pts',(-23.0421692712467,-4.45820427241683,
0.));
#199460=CARTESIAN_POINT('Ctrl Pts',(-23.0421692712467,-4.45820427241683,
12.));
#199461=CARTESIAN_POINT('Ctrl Pts',(-23.0259311131392,-4.44995276669686,
0.));
#199462=CARTESIAN_POINT('Ctrl Pts',(-23.0259311131392,-4.44995276669686,
12.));
#199463=CARTESIAN_POINT('Ctrl Pts',(-23.0097798538395,-4.44180268901643,
0.));
#199464=CARTESIAN_POINT('Ctrl Pts',(-23.0097798538395,-4.44180268901643,
12.));
#199465=CARTESIAN_POINT('Ctrl Pts',(-22.9937167421006,-4.43375406376879,
0.));
#199466=CARTESIAN_POINT('Ctrl Pts',(-22.9937167421006,-4.43375406376879,
12.));
#199467=CARTESIAN_POINT('Ctrl Pts',(-22.977743046002,-4.42580691372751,
0.));
#199468=CARTESIAN_POINT('Ctrl Pts',(-22.977743046002,-4.42580691372751,
12.));
#199469=CARTESIAN_POINT('Ctrl Pts',(-22.9618600534866,-4.41796126001302,
0.));
#199470=CARTESIAN_POINT('Ctrl Pts',(-22.9618600534866,-4.41796126001302,
12.));
#199471=CARTESIAN_POINT('Ctrl Pts',(-22.9460690729093,-4.41021712205553,
0.));
#199472=CARTESIAN_POINT('Ctrl Pts',(-22.9460690729093,-4.41021712205553,
12.));
#199473=CARTESIAN_POINT('Ctrl Pts',(-22.930371433555,-4.40257451754323,
0.));
#199474=CARTESIAN_POINT('Ctrl Pts',(-22.930371433555,-4.40257451754323,
12.));
#199475=CARTESIAN_POINT('Ctrl Pts',(-22.9147684862426,-4.39503346238473,
0.));
#199476=CARTESIAN_POINT('Ctrl Pts',(-22.9147684862426,-4.39503346238473,
12.));
#199477=CARTESIAN_POINT('Ctrl Pts',(-22.8992616040108,-4.38759397068406,
0.));
#199478=CARTESIAN_POINT('Ctrl Pts',(-22.8992616040108,-4.38759397068406,
12.));
#199479=CARTESIAN_POINT('Ctrl Pts',(-22.8838521827701,-4.38025605470093,
0.));
#199480=CARTESIAN_POINT('Ctrl Pts',(-22.8838521827701,-4.38025605470093,
12.));
#199481=CARTESIAN_POINT('Ctrl Pts',(-22.8685416419725,-4.37301972480745,
0.));
#199482=CARTESIAN_POINT('Ctrl Pts',(-22.8685416419725,-4.37301972480745,
12.));
#199483=CARTESIAN_POINT('Ctrl Pts',(-22.8533314252422,-4.36588498942997,
0.));
#199484=CARTESIAN_POINT('Ctrl Pts',(-22.8533314252422,-4.36588498942997,
12.));
#199485=CARTESIAN_POINT('Ctrl Pts',(-22.8382230011184,-4.35885185500546,
0.));
#199486=CARTESIAN_POINT('Ctrl Pts',(-22.8382230011184,-4.35885185500546,
12.));
#199487=CARTESIAN_POINT('Ctrl Pts',(-22.8232178638876,-4.35192032594791,
0.));
#199488=CARTESIAN_POINT('Ctrl Pts',(-22.8232178638876,-4.35192032594791,
12.));
#199489=CARTESIAN_POINT('Ctrl Pts',(-22.8083175343791,-4.34509040460062,
0.));
#199490=CARTESIAN_POINT('Ctrl Pts',(-22.8083175343791,-4.34509040460062,
12.));
#199491=CARTESIAN_POINT('Ctrl Pts',(-22.7935235607806,-4.33836209118446,
0.));
#199492=CARTESIAN_POINT('Ctrl Pts',(-22.7935235607806,-4.33836209118446,
12.));
#199493=CARTESIAN_POINT('Ctrl Pts',(-22.7788375194076,-4.3317353837319,
0.));
#199494=CARTESIAN_POINT('Ctrl Pts',(-22.7788375194076,-4.3317353837319,
12.));
#199495=CARTESIAN_POINT('Ctrl Pts',(-22.7642610156475,-4.32521027803754,
0.));
#199496=CARTESIAN_POINT('Ctrl Pts',(-22.7642610156475,-4.32521027803754,
12.));
#199497=CARTESIAN_POINT('Ctrl Pts',(-22.7497956849848,-4.31878676761235,
0.));
#199498=CARTESIAN_POINT('Ctrl Pts',(-22.7497956849848,-4.31878676761235,
12.));
#199499=CARTESIAN_POINT('Ctrl Pts',(-22.7354431939926,-4.31246484362549,
0.));
#199500=CARTESIAN_POINT('Ctrl Pts',(-22.7354431939926,-4.31246484362549,
12.));
#199501=CARTESIAN_POINT('Ctrl Pts',(-22.7212052413386,-4.30624449484069,
0.));
#199502=CARTESIAN_POINT('Ctrl Pts',(-22.7212052413386,-4.30624449484069,
12.));
#199503=CARTESIAN_POINT('Ctrl Pts',(-22.7070835587564,-4.3001257075406,
0.));
#199504=CARTESIAN_POINT('Ctrl Pts',(-22.7070835587564,-4.3001257075406,
12.));
#199505=CARTESIAN_POINT('Ctrl Pts',(-22.6930799122548,-4.29410846547056,
0.));
#199506=CARTESIAN_POINT('Ctrl Pts',(-22.6930799122548,-4.29410846547056,
12.));
#199507=CARTESIAN_POINT('Ctrl Pts',(-22.6791961033538,-4.28819274977763,
0.));
#199508=CARTESIAN_POINT('Ctrl Pts',(-22.6791961033538,-4.28819274977763,
12.));
#199509=CARTESIAN_POINT('Ctrl Pts',(-22.6654339703109,-4.28237853894059,
0.));
#199510=CARTESIAN_POINT('Ctrl Pts',(-22.6654339703109,-4.28237853894059,
12.));
#199511=CARTESIAN_POINT('Ctrl Pts',(-22.6517953893303,-4.2766658086912,
0.));
#199512=CARTESIAN_POINT('Ctrl Pts',(-22.6517953893303,-4.2766658086912,
12.));
#199513=CARTESIAN_POINT('Ctrl Pts',(-22.6382822758172,-4.27105453193004,
0.));
#199514=CARTESIAN_POINT('Ctrl Pts',(-22.6382822758172,-4.27105453193004,
12.));
#199515=CARTESIAN_POINT('Ctrl Pts',(-22.6248965859977,-4.26554467865576,
0.));
#199516=CARTESIAN_POINT('Ctrl Pts',(-22.6248965859977,-4.26554467865576,
12.));
#199517=CARTESIAN_POINT('Ctrl Pts',(-22.6116403184821,-4.26013621588305,
0.));
#199518=CARTESIAN_POINT('Ctrl Pts',(-22.6116403184821,-4.26013621588305,
12.));
#199519=CARTESIAN_POINT('Ctrl Pts',(-22.5985155158636,-4.25482910755481,
0.));
#199520=CARTESIAN_POINT('Ctrl Pts',(-22.5985155158636,-4.25482910755481,
12.));
#199521=CARTESIAN_POINT('Ctrl Pts',(-22.5855242662477,-4.24962331444177,
0.));
#199522=CARTESIAN_POINT('Ctrl Pts',(-22.5855242662477,-4.24962331444177,
12.));
#199523=CARTESIAN_POINT('Ctrl Pts',(-22.572668704992,-4.24451879404851,
0.));
#199524=CARTESIAN_POINT('Ctrl Pts',(-22.572668704992,-4.24451879404851,
12.));
#199525=CARTESIAN_POINT('Ctrl Pts',(-22.5599510166429,-4.23951550052522,
0.));
#199526=CARTESIAN_POINT('Ctrl Pts',(-22.5599510166429,-4.23951550052522,
12.));
#199527=CARTESIAN_POINT('Ctrl Pts',(-22.5473734368086,-4.23461338456712,
0.));
#199528=CARTESIAN_POINT('Ctrl Pts',(-22.5473734368086,-4.23461338456712,
12.));
#199529=CARTESIAN_POINT('Ctrl Pts',(-22.5349382540588,-4.22981239330733,
0.));
#199530=CARTESIAN_POINT('Ctrl Pts',(-22.5349382540588,-4.22981239330733,
12.));
#199531=CARTESIAN_POINT('Ctrl Pts',(-22.5226478117886,-4.22511247020041,
0.));
#199532=CARTESIAN_POINT('Ctrl Pts',(-22.5226478117886,-4.22511247020041,
12.));
#199533=CARTESIAN_POINT('Ctrl Pts',(-22.5105045108881,-4.22051355490196,
0.));
#199534=CARTESIAN_POINT('Ctrl Pts',(-22.5105045108881,-4.22051355490196,
12.));
#199535=CARTESIAN_POINT('Ctrl Pts',(-22.4985108124228,-4.21601558313906,
0.));
#199536=CARTESIAN_POINT('Ctrl Pts',(-22.4985108124228,-4.21601558313906,
12.));
#199537=CARTESIAN_POINT('Ctrl Pts',(-22.4866692403147,-4.21161848657428,
0.));
#199538=CARTESIAN_POINT('Ctrl Pts',(-22.4866692403147,-4.21161848657428,
12.));
#199539=CARTESIAN_POINT('Ctrl Pts',(-22.4749823839917,-4.20732219265649,
0.));
#199540=CARTESIAN_POINT('Ctrl Pts',(-22.4749823839917,-4.20732219265649,
12.));
#199541=CARTESIAN_POINT('Ctrl Pts',(-22.4634529011437,-4.20312662448174,
0.));
#199542=CARTESIAN_POINT('Ctrl Pts',(-22.4634529011437,-4.20312662448174,
12.));
#199543=CARTESIAN_POINT('Ctrl Pts',(-22.4520835205422,-4.19903170066358,
0.));
#199544=CARTESIAN_POINT('Ctrl Pts',(-22.4520835205422,-4.19903170066358,
12.));
#199545=CARTESIAN_POINT('Ctrl Pts',(-22.4408770448917,-4.1950373351886,
0.));
#199546=CARTESIAN_POINT('Ctrl Pts',(-22.4408770448917,-4.1950373351886,
12.));
#199547=CARTESIAN_POINT('Ctrl Pts',(-22.4298363535416,-4.19114343726932,
0.));
#199548=CARTESIAN_POINT('Ctrl Pts',(-22.4298363535416,-4.19114343726932,
12.));
#199549=CARTESIAN_POINT('Ctrl Pts',(-22.4189644056109,-4.18734991117707,
0.));
#199550=CARTESIAN_POINT('Ctrl Pts',(-22.4189644056109,-4.18734991117707,
12.));
#199551=CARTESIAN_POINT('Ctrl Pts',(-22.4082642454448,-4.18365665600839,
0.));
#199552=CARTESIAN_POINT('Ctrl Pts',(-22.4082642454448,-4.18365665600839,
12.));
#199553=CARTESIAN_POINT('Ctrl Pts',(-22.3977390078074,-4.18006356544879,
0.));
#199554=CARTESIAN_POINT('Ctrl Pts',(-22.3977390078074,-4.18006356544879,
12.));
#199555=CARTESIAN_POINT('Ctrl Pts',(-22.3873919231339,-4.17657052752834,
0.));
#199556=CARTESIAN_POINT('Ctrl Pts',(-22.3873919231339,-4.17657052752834,
12.));
#199557=CARTESIAN_POINT('Ctrl Pts',(-22.3772263228624,-4.17317742436162,
0.));
#199558=CARTESIAN_POINT('Ctrl Pts',(-22.3772263228624,-4.17317742436162,
12.));
#199559=CARTESIAN_POINT('Ctrl Pts',(-22.3672456427605,-4.16988413199469,
0.));
#199560=CARTESIAN_POINT('Ctrl Pts',(-22.3672456427605,-4.16988413199469,
12.));
#199561=CARTESIAN_POINT('Ctrl Pts',(-22.3574534257397,-4.16669052026602,
0.));
#199562=CARTESIAN_POINT('Ctrl Pts',(-22.3574534257397,-4.16669052026602,
12.));
#199563=CARTESIAN_POINT('Ctrl Pts',(-22.3478533253886,-4.1635964526318,
0.));
#199564=CARTESIAN_POINT('Ctrl Pts',(-22.3478533253886,-4.1635964526318,
12.));
#199565=CARTESIAN_POINT('Ctrl Pts',(-22.3384491078599,-4.16060178604154,
0.));
#199566=CARTESIAN_POINT('Ctrl Pts',(-22.3384491078599,-4.16060178604154,
12.));
#199567=CARTESIAN_POINT('Ctrl Pts',(-22.3292446628957,-4.15770637047882,
0.));
#199568=CARTESIAN_POINT('Ctrl Pts',(-22.3292446628957,-4.15770637047882,
12.));
#199569=CARTESIAN_POINT('Ctrl Pts',(-22.3202440186979,-4.15491004835278,
0.));
#199570=CARTESIAN_POINT('Ctrl Pts',(-22.3202440186979,-4.15491004835278,
12.));
#199571=CARTESIAN_POINT('Ctrl Pts',(-22.3114513545186,-4.15221265396993,
0.));
#199572=CARTESIAN_POINT('Ctrl Pts',(-22.3114513545186,-4.15221265396993,
12.));
#199573=CARTESIAN_POINT('Ctrl Pts',(-22.3028710166935,-4.14961401285525,
0.));
#199574=CARTESIAN_POINT('Ctrl Pts',(-22.3028710166935,-4.14961401285525,
12.));
#199575=CARTESIAN_POINT('Ctrl Pts',(-22.2945075198468,-4.14711394168559,
0.));
#199576=CARTESIAN_POINT('Ctrl Pts',(-22.2945075198468,-4.14711394168559,
12.));
#199577=CARTESIAN_POINT('Ctrl Pts',(-22.2863655389167,-4.14471224859295,
0.));
#199578=CARTESIAN_POINT('Ctrl Pts',(-22.2863655389167,-4.14471224859295,
12.));
#199579=CARTESIAN_POINT('Ctrl Pts',(-22.2784499072026,-4.14240873321982,
0.));
#199580=CARTESIAN_POINT('Ctrl Pts',(-22.2784499072026,-4.14240873321982,
12.));
#199581=CARTESIAN_POINT('Ctrl Pts',(-22.2707656042456,-4.14020318715988,
0.));
#199582=CARTESIAN_POINT('Ctrl Pts',(-22.2707656042456,-4.14020318715988,
12.));
#199583=CARTESIAN_POINT('Ctrl Pts',(-22.263317791397,-4.13809539255418,
0.));
#199584=CARTESIAN_POINT('Ctrl Pts',(-22.263317791397,-4.13809539255418,
12.));
#199585=CARTESIAN_POINT('Ctrl Pts',(-22.2561118708422,-4.13608511977226,
0.));
#199586=CARTESIAN_POINT('Ctrl Pts',(-22.2561118708422,-4.13608511977226,
12.));
#199587=CARTESIAN_POINT('Ctrl Pts',(-22.2491535317789,-4.13417212558808,
0.));
#199588=CARTESIAN_POINT('Ctrl Pts',(-22.2491535317789,-4.13417212558808,
12.));
#199589=CARTESIAN_POINT('Ctrl Pts',(-22.2424488153523,-4.1323561506016,
0.));
#199590=CARTESIAN_POINT('Ctrl Pts',(-22.2424488153523,-4.1323561506016,
12.));
#199591=CARTESIAN_POINT('Ctrl Pts',(-22.2360040565534,-4.13063692157499,
0.));
#199592=CARTESIAN_POINT('Ctrl Pts',(-22.2360040565534,-4.13063692157499,
12.));
#199593=CARTESIAN_POINT('Ctrl Pts',(-22.2298258043947,-4.12901415463379,
0.));
#199594=CARTESIAN_POINT('Ctrl Pts',(-22.2298258043947,-4.12901415463379,
12.));
#199595=CARTESIAN_POINT('Ctrl Pts',(-22.2239207458781,-4.12748755830099,
0.));
#199596=CARTESIAN_POINT('Ctrl Pts',(-22.2239207458781,-4.12748755830099,
12.));
#199597=CARTESIAN_POINT('Ctrl Pts',(-22.2182956401341,-4.126056836133,0.));
#199598=CARTESIAN_POINT('Ctrl Pts',(-22.2182956401341,-4.126056836133,12.));
#199599=CARTESIAN_POINT('Ctrl Pts',(-22.2129576146671,-4.12472167516602,
0.));
#199600=CARTESIAN_POINT('Ctrl Pts',(-22.2129576146671,-4.12472167516602,
12.));
#199601=CARTESIAN_POINT('Ctrl Pts',(-22.2079143941719,-4.12348173702024,
0.));
#199602=CARTESIAN_POINT('Ctrl Pts',(-22.2079143941719,-4.12348173702024,
12.));
#199603=CARTESIAN_POINT('Ctrl Pts',(-22.2031746532106,-4.12233664408237,
0.));
#199604=CARTESIAN_POINT('Ctrl Pts',(-22.2031746532106,-4.12233664408237,
12.));
#199605=CARTESIAN_POINT('Ctrl Pts',(-22.1987479618246,-4.12128598183533,
0.));
#199606=CARTESIAN_POINT('Ctrl Pts',(-22.1987479618246,-4.12128598183533,
12.));
#199607=CARTESIAN_POINT('Ctrl Pts',(-22.1946440958098,-4.12032932637738,
0.));
#199608=CARTESIAN_POINT('Ctrl Pts',(-22.1946440958098,-4.12032932637738,
12.));
#199609=CARTESIAN_POINT('Ctrl Pts',(-22.1908725908525,-4.11946626228623,
0.));
#199610=CARTESIAN_POINT('Ctrl Pts',(-22.1908725908525,-4.11946626228623,
12.));
#199611=CARTESIAN_POINT('Ctrl Pts',(-22.1874419861496,-4.11869641271752,
0.));
#199612=CARTESIAN_POINT('Ctrl Pts',(-22.1874419861496,-4.11869641271752,
12.));
#199613=CARTESIAN_POINT('Ctrl Pts',(-22.1843613164855,-4.11801938107464,
0.));
#199614=CARTESIAN_POINT('Ctrl Pts',(-22.1843613164855,-4.11801938107464,
12.));
#199615=CARTESIAN_POINT('Ctrl Pts',(-22.1816414985788,-4.11743469691765,
0.));
#199616=CARTESIAN_POINT('Ctrl Pts',(-22.1816414985788,-4.11743469691765,
12.));
#199617=CARTESIAN_POINT('Ctrl Pts',(-22.179297473024,-4.11694173195041,
0.));
#199618=CARTESIAN_POINT('Ctrl Pts',(-22.179297473024,-4.11694173195041,
12.));
#199619=CARTESIAN_POINT('Ctrl Pts',(-22.177347426894,-4.11653973150558,
0.));
#199620=CARTESIAN_POINT('Ctrl Pts',(-22.177347426894,-4.11653973150558,
12.));
#199621=CARTESIAN_POINT('Ctrl Pts',(-22.1758088296598,-4.11622797217066,
0.));
#199622=CARTESIAN_POINT('Ctrl Pts',(-22.1758088296598,-4.11622797217066,
12.));
#199623=CARTESIAN_POINT('Ctrl Pts',(-22.1746949858773,-4.11600589882767,
0.));
#199624=CARTESIAN_POINT('Ctrl Pts',(-22.1746949858773,-4.11600589882767,
12.));
#199625=CARTESIAN_POINT('Ctrl Pts',(-22.174148802123,-4.11589976826061,
0.));
#199626=CARTESIAN_POINT('Ctrl Pts',(-22.174148802123,-4.11589976826061,
12.));
#199627=CARTESIAN_POINT('Ctrl Pts',(-22.1739341411684,-4.1158603587821,
0.));
#199628=CARTESIAN_POINT('Ctrl Pts',(-22.1739341411684,-4.1158603587821,
12.));
#199629=CARTESIAN_POINT('Ctrl Pts',(-22.1738776823239,-4.11585194677412,
0.));
#199630=CARTESIAN_POINT('Ctrl Pts',(-22.1738776823239,-4.11585194677412,
12.));
#199631=CARTESIAN_POINT('Ctrl Pts',(-22.1738711152697,-4.11585220600461,
0.));
#199632=CARTESIAN_POINT('Ctrl Pts',(-22.1738711152697,-4.11585220600461,
12.));
#199633=CARTESIAN_POINT('',(-25.2771067246846,-6.08833931617698,0.));
#199634=CARTESIAN_POINT('Ctrl Pts',(-25.2771067246846,-6.08833931617698,
0.));
#199635=CARTESIAN_POINT('Ctrl Pts',(-25.2729539149479,-6.08441489609824,
0.));
#199636=CARTESIAN_POINT('Ctrl Pts',(-25.2646490489816,-6.07657531787577,
0.));
#199637=CARTESIAN_POINT('Ctrl Pts',(-25.2521940105523,-6.06484373634696,
0.));
#199638=CARTESIAN_POINT('Ctrl Pts',(-25.2355918138798,-6.04925720151412,
0.));
#199639=CARTESIAN_POINT('Ctrl Pts',(-25.2148466201368,-6.02986667390187,
0.));
#199640=CARTESIAN_POINT('Ctrl Pts',(-25.1941090269638,-6.0105688180476,
0.));
#199641=CARTESIAN_POINT('Ctrl Pts',(-25.1733791296154,-5.99136367859838,
0.));
#199642=CARTESIAN_POINT('Ctrl Pts',(-25.1526570863065,-5.97225131495636,
0.));
#199643=CARTESIAN_POINT('Ctrl Pts',(-25.1319431317273,-5.95323180187348,
0.));
#199644=CARTESIAN_POINT('Ctrl Pts',(-25.1112375971182,-5.93430523086776,
0.));
#199645=CARTESIAN_POINT('Ctrl Pts',(-25.0905409050863,-5.91547170844382,
0.));
#199646=CARTESIAN_POINT('Ctrl Pts',(-25.0698535426593,-5.89673135155459,
0.));
#199647=CARTESIAN_POINT('Ctrl Pts',(-25.0491760405965,-5.87808428385329,
0.));
#199648=CARTESIAN_POINT('Ctrl Pts',(-25.0285089498922,-5.8595306315681,
0.));
#199649=CARTESIAN_POINT('Ctrl Pts',(-25.0078528200558,-5.84107051963073,
0.));
#199650=CARTESIAN_POINT('Ctrl Pts',(-24.9872081752709,-5.82270406744214,
0.));
#199651=CARTESIAN_POINT('Ctrl Pts',(-24.9665754954462,-5.80443138549747,
0.));
#199652=CARTESIAN_POINT('Ctrl Pts',(-24.9459552293308,-5.78625257775703,
0.));
#199653=CARTESIAN_POINT('Ctrl Pts',(-24.9253478043632,-5.76816774342236,
0.));
#199654=CARTESIAN_POINT('Ctrl Pts',(-24.9047536376467,-5.75017697890813,
0.));
#199655=CARTESIAN_POINT('Ctrl Pts',(-24.8841731467219,-5.73228037976926,
0.));
#199656=CARTESIAN_POINT('Ctrl Pts',(-24.8636067597677,-5.71447804252019,
0.));
#199657=CARTESIAN_POINT('Ctrl Pts',(-24.8430549277634,-5.69677006679429,
0.));
#199658=CARTESIAN_POINT('Ctrl Pts',(-24.822518122386,-5.67915655496524,
0.));
#199659=CARTESIAN_POINT('Ctrl Pts',(-24.8019968304618,-5.66163761114903,
0.));
#199660=CARTESIAN_POINT('Ctrl Pts',(-24.7814915496728,-5.64421334042247,
0.));
#199661=CARTESIAN_POINT('Ctrl Pts',(-24.76100278357,-5.62688384790919,0.));
#199662=CARTESIAN_POINT('Ctrl Pts',(-24.7405310372736,-5.60964923798495,
0.));
#199663=CARTESIAN_POINT('Ctrl Pts',(-24.7200768119079,-5.59250961323995,
0.));
#199664=CARTESIAN_POINT('Ctrl Pts',(-24.6996406035507,-5.57546507427766,
0.));
#199665=CARTESIAN_POINT('Ctrl Pts',(-24.6792229061785,-5.55851572025389,
0.));
#199666=CARTESIAN_POINT('Ctrl Pts',(-24.6588242134733,-5.54166164919593,
0.));
#199667=CARTESIAN_POINT('Ctrl Pts',(-24.6384450211466,-5.52490295840996,
0.));
#199668=CARTESIAN_POINT('Ctrl Pts',(-24.618085828918,-5.50823974481959,
0.));
#199669=CARTESIAN_POINT('Ctrl Pts',(-24.5977471429365,-5.49167210537235,
0.));
#199670=CARTESIAN_POINT('Ctrl Pts',(-24.5774294770329,-5.47520013724403,
0.));
#199671=CARTESIAN_POINT('Ctrl Pts',(-24.5571333514841,-5.45882393762244,
0.));
#199672=CARTESIAN_POINT('Ctrl Pts',(-24.5368592922861,-5.44254360356865,
0.));
#199673=CARTESIAN_POINT('Ctrl Pts',(-24.5166078302107,-5.42635923183411,
0.));
#199674=CARTESIAN_POINT('Ctrl Pts',(-24.4963794999831,-5.41027091869242,
0.));
#199675=CARTESIAN_POINT('Ctrl Pts',(-24.4761748393322,-5.3942787597383,
0.));
#199676=CARTESIAN_POINT('Ctrl Pts',(-24.4559943883159,-5.37838284973706,
0.));
#199677=CARTESIAN_POINT('Ctrl Pts',(-24.4358386899152,-5.36258328273639,
0.));
#199678=CARTESIAN_POINT('Ctrl Pts',(-24.4157082904615,-5.34688015213546,
0.));
#199679=CARTESIAN_POINT('Ctrl Pts',(-24.3956037401293,-5.33127355076036,
0.));
#199680=CARTESIAN_POINT('Ctrl Pts',(-24.3755255933917,-5.31576357092524,
0.));
#199681=CARTESIAN_POINT('Ctrl Pts',(-24.3554744095075,-5.30035030449058,
0.));
#199682=CARTESIAN_POINT('Ctrl Pts',(-24.3354507529415,-5.28503384290644,
0.));
#199683=CARTESIAN_POINT('Ctrl Pts',(-24.3154551932222,-5.26981427718796,
0.));
#199684=CARTESIAN_POINT('Ctrl Pts',(-24.2954883048448,-5.25469169788856,
0.));
#199685=CARTESIAN_POINT('Ctrl Pts',(-24.2755506671526,-5.23966619506289,
0.));
#199686=CARTESIAN_POINT('Ctrl Pts',(-24.2556428642294,-5.22473785822441,
0.));
#199687=CARTESIAN_POINT('Ctrl Pts',(-24.2357654847765,-5.20990677629173,
0.));
#199688=CARTESIAN_POINT('Ctrl Pts',(-24.215919122017,-5.19517303753643,
0.));
#199689=CARTESIAN_POINT('Ctrl Pts',(-24.1961043738754,-5.18053672961392,
0.));
#199690=CARTESIAN_POINT('Ctrl Pts',(-24.1763218431343,-5.16599793957979,
0.));
#199691=CARTESIAN_POINT('Ctrl Pts',(-24.156572137597,-5.15155675390075,
0.));
#199692=CARTESIAN_POINT('Ctrl Pts',(-24.1368558702443,-5.13721325845744,
0.));
#199693=CARTESIAN_POINT('Ctrl Pts',(-24.117173659394,-5.12296753853859,
0.));
#199694=CARTESIAN_POINT('Ctrl Pts',(-24.0975261288446,-5.10881967883132,
0.));
#199695=CARTESIAN_POINT('Ctrl Pts',(-24.0779139079266,-5.09476976342625,
0.));
#199696=CARTESIAN_POINT('Ctrl Pts',(-24.0583376315638,-5.08081787581276,
0.));
#199697=CARTESIAN_POINT('Ctrl Pts',(-24.0387979403268,-5.06696409886641,
0.));
#199698=CARTESIAN_POINT('Ctrl Pts',(-24.0192954804896,-5.05320851483065,
0.));
#199699=CARTESIAN_POINT('Ctrl Pts',(-23.9998309040746,-5.03955120528521,
0.));
#199700=CARTESIAN_POINT('Ctrl Pts',(-23.9804048689227,-5.02599225112454,
0.));
#199701=CARTESIAN_POINT('Ctrl Pts',(-23.9610180388271,-5.01253173257453,
0.));
#199702=CARTESIAN_POINT('Ctrl Pts',(-23.9416710836529,-4.99916972919306,
0.));
#199703=CARTESIAN_POINT('Ctrl Pts',(-23.9223646794592,-4.98590631986532,
0.));
#199704=CARTESIAN_POINT('Ctrl Pts',(-23.9030995086163,-4.97274158279226,
0.));
#199705=CARTESIAN_POINT('Ctrl Pts',(-23.8838762599218,-4.9596755954656,
0.));
#199706=CARTESIAN_POINT('Ctrl Pts',(-23.8646956287168,-4.9467084346586,
0.));
#199707=CARTESIAN_POINT('Ctrl Pts',(-23.8455583170057,-4.93384017643432,
0.));
#199708=CARTESIAN_POINT('Ctrl Pts',(-23.8264650335717,-4.92107089613969,
0.));
#199709=CARTESIAN_POINT('Ctrl Pts',(-23.8074164940896,-4.90840066839344,
0.));
#199710=CARTESIAN_POINT('Ctrl Pts',(-23.7884134212384,-4.89582956706775,
0.));
#199711=CARTESIAN_POINT('Ctrl Pts',(-23.7694565448049,-4.88335766525573,
0.));
#199712=CARTESIAN_POINT('Ctrl Pts',(-23.7505466018245,-4.87098503527152,
0.));
#199713=CARTESIAN_POINT('Ctrl Pts',(-23.7316843367313,-4.85871174865499,
0.));
#199714=CARTESIAN_POINT('Ctrl Pts',(-23.7128705015017,-4.84653787616425,
0.));
#199715=CARTESIAN_POINT('Ctrl Pts',(-23.6941058557971,-4.83446348776265,
0.));
#199716=CARTESIAN_POINT('Ctrl Pts',(-23.675391167102,-4.82248865259562,
0.));
#199717=CARTESIAN_POINT('Ctrl Pts',(-23.6567272108628,-4.81061343896432,
0.));
#199718=CARTESIAN_POINT('Ctrl Pts',(-23.6381147706579,-4.7988379143322,
0.));
#199719=CARTESIAN_POINT('Ctrl Pts',(-23.6195546383624,-4.78716214532098,
0.));
#199720=CARTESIAN_POINT('Ctrl Pts',(-23.6010476143099,-4.77558619769872,
0.));
#199721=CARTESIAN_POINT('Ctrl Pts',(-23.5825945074535,-4.76411013636251,
0.));
#199722=CARTESIAN_POINT('Ctrl Pts',(-23.5641961355168,-4.75273402530617,
0.));
#199723=CARTESIAN_POINT('Ctrl Pts',(-23.545853325171,-4.74145792760698,
0.));
#199724=CARTESIAN_POINT('Ctrl Pts',(-23.5275669122372,-4.7302819054303,
0.));
#199725=CARTESIAN_POINT('Ctrl Pts',(-23.509337741878,-4.71920602001901,
0.));
#199726=CARTESIAN_POINT('Ctrl Pts',(-23.491166668789,-4.70823033167818,
0.));
#199727=CARTESIAN_POINT('Ctrl Pts',(-23.4730545573853,-4.69735489975024,
0.));
#199728=CARTESIAN_POINT('Ctrl Pts',(-23.455002281986,-4.68657978258303,
0.));
#199729=CARTESIAN_POINT('Ctrl Pts',(-23.4370107270451,-4.67590503753058,
0.));
#199730=CARTESIAN_POINT('Ctrl Pts',(-23.4190807873803,-4.6653307209467,
0.));
#199731=CARTESIAN_POINT('Ctrl Pts',(-23.4012133683959,-4.65485688816924,
0.));
#199732=CARTESIAN_POINT('Ctrl Pts',(-23.3834093863068,-4.6444835934993,
0.));
#199733=CARTESIAN_POINT('Ctrl Pts',(-23.3656697683489,-4.63421089016541,
0.));
#199734=CARTESIAN_POINT('Ctrl Pts',(-23.3479954530272,-4.62403883030805,
0.));
#199735=CARTESIAN_POINT('Ctrl Pts',(-23.3303873903938,-4.6139674649783,
0.));
#199736=CARTESIAN_POINT('Ctrl Pts',(-23.3128465423115,-4.60399684412163,
0.));
#199737=CARTESIAN_POINT('Ctrl Pts',(-23.2953738827191,-4.5941270165575,
0.));
#199738=CARTESIAN_POINT('Ctrl Pts',(-23.2779703978876,-4.5843580299469,
0.));
#199739=CARTESIAN_POINT('Ctrl Pts',(-23.2606370866866,-4.57468993076097,
0.));
#199740=CARTESIAN_POINT('Ctrl Pts',(-23.2433749609131,-4.56512276427839,
0.));
#199741=CARTESIAN_POINT('Ctrl Pts',(-23.2261850456064,-4.55565657456975,
0.));
#199742=CARTESIAN_POINT('Ctrl Pts',(-23.2090683793629,-4.54629140447544,
0.));
#199743=CARTESIAN_POINT('Ctrl Pts',(-23.1920260146465,-4.53702729557566,
0.));
#199744=CARTESIAN_POINT('Ctrl Pts',(-23.1750590180908,-4.52786428815014,
0.));
#199745=CARTESIAN_POINT('Ctrl Pts',(-23.1581684708761,-4.51880242116748,
0.));
#199746=CARTESIAN_POINT('Ctrl Pts',(-23.1413554691123,-4.5098417322706,
0.));
#199747=CARTESIAN_POINT('Ctrl Pts',(-23.1246211242115,-4.50098225775171,
0.));
#199748=CARTESIAN_POINT('Ctrl Pts',(-23.1079665632636,-4.49222403252216,
0.));
#199749=CARTESIAN_POINT('Ctrl Pts',(-23.0913929293922,-4.48356709006788,
0.));
#199750=CARTESIAN_POINT('Ctrl Pts',(-23.0749013821881,-4.47501146242856,
0.));
#199751=CARTESIAN_POINT('Ctrl Pts',(-23.0584930981732,-4.4665571801823,
0.));
#199752=CARTESIAN_POINT('Ctrl Pts',(-23.0421692712467,-4.45820427241683,
0.));
#199753=CARTESIAN_POINT('Ctrl Pts',(-23.0259311131392,-4.44995276669686,
0.));
#199754=CARTESIAN_POINT('Ctrl Pts',(-23.0097798538395,-4.44180268901643,
0.));
#199755=CARTESIAN_POINT('Ctrl Pts',(-22.9937167421006,-4.43375406376879,
0.));
#199756=CARTESIAN_POINT('Ctrl Pts',(-22.977743046002,-4.42580691372751,
0.));
#199757=CARTESIAN_POINT('Ctrl Pts',(-22.9618600534866,-4.41796126001302,
0.));
#199758=CARTESIAN_POINT('Ctrl Pts',(-22.9460690729093,-4.41021712205553,
0.));
#199759=CARTESIAN_POINT('Ctrl Pts',(-22.930371433555,-4.40257451754323,
0.));
#199760=CARTESIAN_POINT('Ctrl Pts',(-22.9147684862426,-4.39503346238473,
0.));
#199761=CARTESIAN_POINT('Ctrl Pts',(-22.8992616040108,-4.38759397068406,
0.));
#199762=CARTESIAN_POINT('Ctrl Pts',(-22.8838521827701,-4.38025605470093,
0.));
#199763=CARTESIAN_POINT('Ctrl Pts',(-22.8685416419725,-4.37301972480745,
0.));
#199764=CARTESIAN_POINT('Ctrl Pts',(-22.8533314252422,-4.36588498942997,
0.));
#199765=CARTESIAN_POINT('Ctrl Pts',(-22.8382230011184,-4.35885185500546,
0.));
#199766=CARTESIAN_POINT('Ctrl Pts',(-22.8232178638876,-4.35192032594791,
0.));
#199767=CARTESIAN_POINT('Ctrl Pts',(-22.8083175343791,-4.34509040460062,
0.));
#199768=CARTESIAN_POINT('Ctrl Pts',(-22.7935235607806,-4.33836209118446,
0.));
#199769=CARTESIAN_POINT('Ctrl Pts',(-22.7788375194076,-4.3317353837319,
0.));
#199770=CARTESIAN_POINT('Ctrl Pts',(-22.7642610156475,-4.32521027803754,
0.));
#199771=CARTESIAN_POINT('Ctrl Pts',(-22.7497956849848,-4.31878676761235,
0.));
#199772=CARTESIAN_POINT('Ctrl Pts',(-22.7354431939926,-4.31246484362549,
0.));
#199773=CARTESIAN_POINT('Ctrl Pts',(-22.7212052413386,-4.30624449484069,
0.));
#199774=CARTESIAN_POINT('Ctrl Pts',(-22.7070835587564,-4.3001257075406,
0.));
#199775=CARTESIAN_POINT('Ctrl Pts',(-22.6930799122548,-4.29410846547056,
0.));
#199776=CARTESIAN_POINT('Ctrl Pts',(-22.6791961033538,-4.28819274977763,
0.));
#199777=CARTESIAN_POINT('Ctrl Pts',(-22.6654339703109,-4.28237853894059,
0.));
#199778=CARTESIAN_POINT('Ctrl Pts',(-22.6517953893303,-4.2766658086912,
0.));
#199779=CARTESIAN_POINT('Ctrl Pts',(-22.6382822758172,-4.27105453193004,
0.));
#199780=CARTESIAN_POINT('Ctrl Pts',(-22.6248965859977,-4.26554467865576,
0.));
#199781=CARTESIAN_POINT('Ctrl Pts',(-22.6116403184821,-4.26013621588305,
0.));
#199782=CARTESIAN_POINT('Ctrl Pts',(-22.5985155158636,-4.25482910755481,
0.));
#199783=CARTESIAN_POINT('Ctrl Pts',(-22.5855242662477,-4.24962331444177,
0.));
#199784=CARTESIAN_POINT('Ctrl Pts',(-22.572668704992,-4.24451879404851,
0.));
#199785=CARTESIAN_POINT('Ctrl Pts',(-22.5599510166429,-4.23951550052522,
0.));
#199786=CARTESIAN_POINT('Ctrl Pts',(-22.5473734368086,-4.23461338456712,
0.));
#199787=CARTESIAN_POINT('Ctrl Pts',(-22.5349382540588,-4.22981239330733,
0.));
#199788=CARTESIAN_POINT('Ctrl Pts',(-22.5226478117886,-4.22511247020041,
0.));
#199789=CARTESIAN_POINT('Ctrl Pts',(-22.5105045108881,-4.22051355490196,
0.));
#199790=CARTESIAN_POINT('Ctrl Pts',(-22.4985108124228,-4.21601558313906,
0.));
#199791=CARTESIAN_POINT('Ctrl Pts',(-22.4866692403147,-4.21161848657428,
0.));
#199792=CARTESIAN_POINT('Ctrl Pts',(-22.4749823839917,-4.20732219265649,
0.));
#199793=CARTESIAN_POINT('Ctrl Pts',(-22.4634529011437,-4.20312662448174,
0.));
#199794=CARTESIAN_POINT('Ctrl Pts',(-22.4520835205422,-4.19903170066358,
0.));
#199795=CARTESIAN_POINT('Ctrl Pts',(-22.4408770448917,-4.1950373351886,
0.));
#199796=CARTESIAN_POINT('Ctrl Pts',(-22.4298363535416,-4.19114343726932,
0.));
#199797=CARTESIAN_POINT('Ctrl Pts',(-22.4189644056109,-4.18734991117707,
0.));
#199798=CARTESIAN_POINT('Ctrl Pts',(-22.4082642454448,-4.18365665600839,
0.));
#199799=CARTESIAN_POINT('Ctrl Pts',(-22.3977390078074,-4.18006356544879,
0.));
#199800=CARTESIAN_POINT('Ctrl Pts',(-22.3873919231339,-4.17657052752834,
0.));
#199801=CARTESIAN_POINT('Ctrl Pts',(-22.3772263228624,-4.17317742436162,
0.));
#199802=CARTESIAN_POINT('Ctrl Pts',(-22.3672456427605,-4.16988413199469,
0.));
#199803=CARTESIAN_POINT('Ctrl Pts',(-22.3574534257397,-4.16669052026602,
0.));
#199804=CARTESIAN_POINT('Ctrl Pts',(-22.3478533253886,-4.1635964526318,
0.));
#199805=CARTESIAN_POINT('Ctrl Pts',(-22.3384491078599,-4.16060178604154,
0.));
#199806=CARTESIAN_POINT('Ctrl Pts',(-22.3292446628957,-4.15770637047882,
0.));
#199807=CARTESIAN_POINT('Ctrl Pts',(-22.3202440186979,-4.15491004835278,
0.));
#199808=CARTESIAN_POINT('Ctrl Pts',(-22.3114513545186,-4.15221265396993,
0.));
#199809=CARTESIAN_POINT('Ctrl Pts',(-22.3028710166935,-4.14961401285525,
0.));
#199810=CARTESIAN_POINT('Ctrl Pts',(-22.2945075198468,-4.14711394168559,
0.));
#199811=CARTESIAN_POINT('Ctrl Pts',(-22.2863655389167,-4.14471224859295,
0.));
#199812=CARTESIAN_POINT('Ctrl Pts',(-22.2784499072026,-4.14240873321982,
0.));
#199813=CARTESIAN_POINT('Ctrl Pts',(-22.2707656042456,-4.14020318715988,
0.));
#199814=CARTESIAN_POINT('Ctrl Pts',(-22.263317791397,-4.13809539255418,
0.));
#199815=CARTESIAN_POINT('Ctrl Pts',(-22.2561118708422,-4.13608511977226,
0.));
#199816=CARTESIAN_POINT('Ctrl Pts',(-22.2491535317789,-4.13417212558808,
0.));
#199817=CARTESIAN_POINT('Ctrl Pts',(-22.2424488153523,-4.1323561506016,
0.));
#199818=CARTESIAN_POINT('Ctrl Pts',(-22.2360040565534,-4.13063692157499,
0.));
#199819=CARTESIAN_POINT('Ctrl Pts',(-22.2298258043947,-4.12901415463379,
0.));
#199820=CARTESIAN_POINT('Ctrl Pts',(-22.2239207458781,-4.12748755830099,
0.));
#199821=CARTESIAN_POINT('Ctrl Pts',(-22.2182956401341,-4.126056836133,0.));
#199822=CARTESIAN_POINT('Ctrl Pts',(-22.2129576146671,-4.12472167516602,
0.));
#199823=CARTESIAN_POINT('Ctrl Pts',(-22.2079143941719,-4.12348173702024,
0.));
#199824=CARTESIAN_POINT('Ctrl Pts',(-22.2031746532106,-4.12233664408237,
0.));
#199825=CARTESIAN_POINT('Ctrl Pts',(-22.1987479618246,-4.12128598183533,
0.));
#199826=CARTESIAN_POINT('Ctrl Pts',(-22.1946440958098,-4.12032932637738,
0.));
#199827=CARTESIAN_POINT('Ctrl Pts',(-22.1908725908525,-4.11946626228623,
0.));
#199828=CARTESIAN_POINT('Ctrl Pts',(-22.1874419861496,-4.11869641271752,
0.));
#199829=CARTESIAN_POINT('Ctrl Pts',(-22.1843613164855,-4.11801938107464,
0.));
#199830=CARTESIAN_POINT('Ctrl Pts',(-22.1816414985788,-4.11743469691765,
0.));
#199831=CARTESIAN_POINT('Ctrl Pts',(-22.179297473024,-4.11694173195041,
0.));
#199832=CARTESIAN_POINT('Ctrl Pts',(-22.177347426894,-4.11653973150558,
0.));
#199833=CARTESIAN_POINT('Ctrl Pts',(-22.1758088296598,-4.11622797217066,
0.));
#199834=CARTESIAN_POINT('Ctrl Pts',(-22.1746949858773,-4.11600589882767,
0.));
#199835=CARTESIAN_POINT('Ctrl Pts',(-22.174148802123,-4.11589976826061,
0.));
#199836=CARTESIAN_POINT('Ctrl Pts',(-22.1739341411684,-4.1158603587821,
0.));
#199837=CARTESIAN_POINT('Ctrl Pts',(-22.1738776823239,-4.11585194677412,
0.));
#199838=CARTESIAN_POINT('Ctrl Pts',(-22.1738711152697,-4.11585220600461,
0.));
#199839=CARTESIAN_POINT('',(-25.2771067246846,-6.08833931617698,0.));
#199840=CARTESIAN_POINT('Ctrl Pts',(-22.4835757167854,-1.76341220531179,
0.));
#199841=CARTESIAN_POINT('Ctrl Pts',(-22.4835757167854,-1.76341220531179,
12.));
#199842=CARTESIAN_POINT('Ctrl Pts',(-22.483581992979,-1.76341415538764,
0.));
#199843=CARTESIAN_POINT('Ctrl Pts',(-22.483581992979,-1.76341415538764,
12.));
#199844=CARTESIAN_POINT('Ctrl Pts',(-22.4836387052232,-1.7634206426357,
0.));
#199845=CARTESIAN_POINT('Ctrl Pts',(-22.4836387052232,-1.7634206426357,
12.));
#199846=CARTESIAN_POINT('Ctrl Pts',(-22.483856251707,-1.76343813434565,
0.));
#199847=CARTESIAN_POINT('Ctrl Pts',(-22.483856251707,-1.76343813434565,
12.));
#199848=CARTESIAN_POINT('Ctrl Pts',(-22.4844112933129,-1.76347698284792,
0.));
#199849=CARTESIAN_POINT('Ctrl Pts',(-22.4844112933129,-1.76347698284792,
12.));
#199850=CARTESIAN_POINT('Ctrl Pts',(-22.4855446605991,-1.76355076045546,
0.));
#199851=CARTESIAN_POINT('Ctrl Pts',(-22.4855446605991,-1.76355076045546,
12.));
#199852=CARTESIAN_POINT('Ctrl Pts',(-22.4871115206571,-1.76364784232963,
0.));
#199853=CARTESIAN_POINT('Ctrl Pts',(-22.4871115206571,-1.76364784232963,
12.));
#199854=CARTESIAN_POINT('Ctrl Pts',(-22.4890991659478,-1.76376424879505,
0.));
#199855=CARTESIAN_POINT('Ctrl Pts',(-22.4890991659478,-1.76376424879505,
12.));
#199856=CARTESIAN_POINT('Ctrl Pts',(-22.4914909094908,-1.76389475965724,
0.));
#199857=CARTESIAN_POINT('Ctrl Pts',(-22.4914909094908,-1.76389475965724,
12.));
#199858=CARTESIAN_POINT('Ctrl Pts',(-22.4942693792449,-1.764033938803,0.));
#199859=CARTESIAN_POINT('Ctrl Pts',(-22.4942693792449,-1.764033938803,12.));
#199860=CARTESIAN_POINT('Ctrl Pts',(-22.4974203063191,-1.76417731243462,
0.));
#199861=CARTESIAN_POINT('Ctrl Pts',(-22.4974203063191,-1.76417731243462,
12.));
#199862=CARTESIAN_POINT('Ctrl Pts',(-22.5009332677316,-1.76432160068725,
0.));
#199863=CARTESIAN_POINT('Ctrl Pts',(-22.5009332677316,-1.76432160068725,
12.));
#199864=CARTESIAN_POINT('Ctrl Pts',(-22.5047996391978,-1.76446408210366,
0.));
#199865=CARTESIAN_POINT('Ctrl Pts',(-22.5047996391978,-1.76446408210366,
12.));
#199866=CARTESIAN_POINT('Ctrl Pts',(-22.5090112700212,-1.76460218257323,
0.));
#199867=CARTESIAN_POINT('Ctrl Pts',(-22.5090112700212,-1.76460218257323,
12.));
#199868=CARTESIAN_POINT('Ctrl Pts',(-22.5135590569554,-1.76473303281159,
0.));
#199869=CARTESIAN_POINT('Ctrl Pts',(-22.5135590569554,-1.76473303281159,
12.));
#199870=CARTESIAN_POINT('Ctrl Pts',(-22.5184336670207,-1.76485369319896,
0.));
#199871=CARTESIAN_POINT('Ctrl Pts',(-22.5184336670207,-1.76485369319896,
12.));
#199872=CARTESIAN_POINT('Ctrl Pts',(-22.5236259635515,-1.76496128643369,
0.));
#199873=CARTESIAN_POINT('Ctrl Pts',(-22.5236259635515,-1.76496128643369,
12.));
#199874=CARTESIAN_POINT('Ctrl Pts',(-22.529127665298,-1.76505320262751,
0.));
#199875=CARTESIAN_POINT('Ctrl Pts',(-22.529127665298,-1.76505320262751,
12.));
#199876=CARTESIAN_POINT('Ctrl Pts',(-22.5349313983571,-1.7651271156325,
0.));
#199877=CARTESIAN_POINT('Ctrl Pts',(-22.5349313983571,-1.7651271156325,
12.));
#199878=CARTESIAN_POINT('Ctrl Pts',(-22.5410303590891,-1.76518087841492,
0.));
#199879=CARTESIAN_POINT('Ctrl Pts',(-22.5410303590891,-1.76518087841492,
12.));
#199880=CARTESIAN_POINT('Ctrl Pts',(-22.5474180954006,-1.76521245524047,
0.));
#199881=CARTESIAN_POINT('Ctrl Pts',(-22.5474180954006,-1.76521245524047,
12.));
#199882=CARTESIAN_POINT('Ctrl Pts',(-22.5540882235837,-1.76521983384063,
0.));
#199883=CARTESIAN_POINT('Ctrl Pts',(-22.5540882235837,-1.76521983384063,
12.));
#199884=CARTESIAN_POINT('Ctrl Pts',(-22.5610344912501,-1.76520104500449,
0.));
#199885=CARTESIAN_POINT('Ctrl Pts',(-22.5610344912501,-1.76520104500449,
12.));
#199886=CARTESIAN_POINT('Ctrl Pts',(-22.5682508499873,-1.76515418518829,
0.));
#199887=CARTESIAN_POINT('Ctrl Pts',(-22.5682508499873,-1.76515418518829,
12.));
#199888=CARTESIAN_POINT('Ctrl Pts',(-22.5757315316355,-1.76507744026747,
0.));
#199889=CARTESIAN_POINT('Ctrl Pts',(-22.5757315316355,-1.76507744026747,
12.));
#199890=CARTESIAN_POINT('Ctrl Pts',(-22.5834711038024,-1.76496910283088,
0.));
#199891=CARTESIAN_POINT('Ctrl Pts',(-22.5834711038024,-1.76496910283088,
12.));
#199892=CARTESIAN_POINT('Ctrl Pts',(-22.5914644078106,-1.76482755288411,
0.));
#199893=CARTESIAN_POINT('Ctrl Pts',(-22.5914644078106,-1.76482755288411,
12.));
#199894=CARTESIAN_POINT('Ctrl Pts',(-22.5997065145638,-1.76465124413556,
0.));
#199895=CARTESIAN_POINT('Ctrl Pts',(-22.5997065145638,-1.76465124413556,
12.));
#199896=CARTESIAN_POINT('Ctrl Pts',(-22.6081926681342,-1.76443868648015,
0.));
#199897=CARTESIAN_POINT('Ctrl Pts',(-22.6081926681342,-1.76443868648015,
12.));
#199898=CARTESIAN_POINT('Ctrl Pts',(-22.6169182517693,-1.76418843543739,
0.));
#199899=CARTESIAN_POINT('Ctrl Pts',(-22.6169182517693,-1.76418843543739,
12.));
#199900=CARTESIAN_POINT('Ctrl Pts',(-22.6258787994847,-1.76389909571402,
0.));
#199901=CARTESIAN_POINT('Ctrl Pts',(-22.6258787994847,-1.76389909571402,
12.));
#199902=CARTESIAN_POINT('Ctrl Pts',(-22.635069997936,-1.76356932176272,
0.));
#199903=CARTESIAN_POINT('Ctrl Pts',(-22.635069997936,-1.76356932176272,
12.));
#199904=CARTESIAN_POINT('Ctrl Pts',(-22.6444876940425,-1.76319782013914,
0.));
#199905=CARTESIAN_POINT('Ctrl Pts',(-22.6444876940425,-1.76319782013914,
12.));
#199906=CARTESIAN_POINT('Ctrl Pts',(-22.6541278938413,-1.76278334912559,
0.));
#199907=CARTESIAN_POINT('Ctrl Pts',(-22.6541278938413,-1.76278334912559,
12.));
#199908=CARTESIAN_POINT('Ctrl Pts',(-22.6639867471756,-1.76232471392567,
0.));
#199909=CARTESIAN_POINT('Ctrl Pts',(-22.6639867471756,-1.76232471392567,
12.));
#199910=CARTESIAN_POINT('Ctrl Pts',(-22.6740605356699,-1.76182076289525,
0.));
#199911=CARTESIAN_POINT('Ctrl Pts',(-22.6740605356699,-1.76182076289525,
12.));
#199912=CARTESIAN_POINT('Ctrl Pts',(-22.6843456585245,-1.76127038310612,
0.));
#199913=CARTESIAN_POINT('Ctrl Pts',(-22.6843456585245,-1.76127038310612,
12.));
#199914=CARTESIAN_POINT('Ctrl Pts',(-22.6948386219843,-1.76067249704884,
0.));
#199915=CARTESIAN_POINT('Ctrl Pts',(-22.6948386219843,-1.76067249704884,
12.));
#199916=CARTESIAN_POINT('Ctrl Pts',(-22.7055360375481,-1.76002606202399,
0.));
#199917=CARTESIAN_POINT('Ctrl Pts',(-22.7055360375481,-1.76002606202399,
12.));
#199918=CARTESIAN_POINT('Ctrl Pts',(-22.7164346186007,-1.75933006905924,
0.));
#199919=CARTESIAN_POINT('Ctrl Pts',(-22.7164346186007,-1.75933006905924,
12.));
#199920=CARTESIAN_POINT('Ctrl Pts',(-22.7275311777305,-1.75858354204635,
0.));
#199921=CARTESIAN_POINT('Ctrl Pts',(-22.7275311777305,-1.75858354204635,
12.));
#199922=CARTESIAN_POINT('Ctrl Pts',(-22.7388226235565,-1.75778553673249,
0.));
#199923=CARTESIAN_POINT('Ctrl Pts',(-22.7388226235565,-1.75778553673249,
12.));
#199924=CARTESIAN_POINT('Ctrl Pts',(-22.7503059556455,-1.75693513908911,
0.));
#199925=CARTESIAN_POINT('Ctrl Pts',(-22.7503059556455,-1.75693513908911,
12.));
#199926=CARTESIAN_POINT('Ctrl Pts',(-22.7619782595013,-1.7560314637164,
0.));
#199927=CARTESIAN_POINT('Ctrl Pts',(-22.7619782595013,-1.7560314637164,
12.));
#199928=CARTESIAN_POINT('Ctrl Pts',(-22.7738367016115,-1.75507365227127,
0.));
#199929=CARTESIAN_POINT('Ctrl Pts',(-22.7738367016115,-1.75507365227127,
12.));
#199930=CARTESIAN_POINT('Ctrl Pts',(-22.7858785242358,-1.75406087182929,
0.));
#199931=CARTESIAN_POINT('Ctrl Pts',(-22.7858785242358,-1.75406087182929,
12.));
#199932=CARTESIAN_POINT('Ctrl Pts',(-22.7981010424312,-1.75299231391461,
0.));
#199933=CARTESIAN_POINT('Ctrl Pts',(-22.7981010424312,-1.75299231391461,
12.));
#199934=CARTESIAN_POINT('Ctrl Pts',(-22.8105016414712,-1.75186719365589,
0.));
#199935=CARTESIAN_POINT('Ctrl Pts',(-22.8105016414712,-1.75186719365589,
12.));
#199936=CARTESIAN_POINT('Ctrl Pts',(-22.8230777741285,-1.75068474890884,
0.));
#199937=CARTESIAN_POINT('Ctrl Pts',(-22.8230777741285,-1.75068474890884,
12.));
#199938=CARTESIAN_POINT('Ctrl Pts',(-22.8358269579854,-1.74944423940117,
0.));
#199939=CARTESIAN_POINT('Ctrl Pts',(-22.8358269579854,-1.74944423940117,
12.));
#199940=CARTESIAN_POINT('Ctrl Pts',(-22.8487467728075,-1.74814494588492,
0.));
#199941=CARTESIAN_POINT('Ctrl Pts',(-22.8487467728075,-1.74814494588492,
12.));
#199942=CARTESIAN_POINT('Ctrl Pts',(-22.8618348580234,-1.74678616930663,
0.));
#199943=CARTESIAN_POINT('Ctrl Pts',(-22.8618348580234,-1.74678616930663,
12.));
#199944=CARTESIAN_POINT('Ctrl Pts',(-22.8750889101696,-1.745367229982,0.));
#199945=CARTESIAN_POINT('Ctrl Pts',(-22.8750889101696,-1.745367229982,12.));
#199946=CARTESIAN_POINT('Ctrl Pts',(-22.8885066803351,-1.74388746677702,
0.));
#199947=CARTESIAN_POINT('Ctrl Pts',(-22.8885066803351,-1.74388746677702,
12.));
#199948=CARTESIAN_POINT('Ctrl Pts',(-22.9020859716144,-1.74234623630079,
0.));
#199949=CARTESIAN_POINT('Ctrl Pts',(-22.9020859716144,-1.74234623630079,
12.));
#199950=CARTESIAN_POINT('Ctrl Pts',(-22.9158246373365,-1.74074291231057,
0.));
#199951=CARTESIAN_POINT('Ctrl Pts',(-22.9158246373365,-1.74074291231057,
12.));
#199952=CARTESIAN_POINT('Ctrl Pts',(-22.9297205792587,-1.73907688511664,
0.));
#199953=CARTESIAN_POINT('Ctrl Pts',(-22.9297205792587,-1.73907688511664,
12.));
#199954=CARTESIAN_POINT('Ctrl Pts',(-22.9437717457825,-1.73734756100038,
0.));
#199955=CARTESIAN_POINT('Ctrl Pts',(-22.9437717457825,-1.73734756100038,
12.));
#199956=CARTESIAN_POINT('Ctrl Pts',(-22.9579761301062,-1.73555436162771,
0.));
#199957=CARTESIAN_POINT('Ctrl Pts',(-22.9579761301062,-1.73555436162771,
12.));
#199958=CARTESIAN_POINT('Ctrl Pts',(-22.9723317685688,-1.73369672350817,
0.));
#199959=CARTESIAN_POINT('Ctrl Pts',(-22.9723317685688,-1.73369672350817,
12.));
#199960=CARTESIAN_POINT('Ctrl Pts',(-22.9868367391978,-1.73177409750193,
0.));
#199961=CARTESIAN_POINT('Ctrl Pts',(-22.9868367391978,-1.73177409750193,
12.));
#199962=CARTESIAN_POINT('Ctrl Pts',(-23.0014891601891,-1.72978594832137,
0.));
#199963=CARTESIAN_POINT('Ctrl Pts',(-23.0014891601891,-1.72978594832137,
12.));
#199964=CARTESIAN_POINT('Ctrl Pts',(-23.0162871884167,-1.72773175404702,
0.));
#199965=CARTESIAN_POINT('Ctrl Pts',(-23.0162871884167,-1.72773175404702,
12.));
#199966=CARTESIAN_POINT('Ctrl Pts',(-23.031229017888,-1.72561100564033,
0.));
#199967=CARTESIAN_POINT('Ctrl Pts',(-23.031229017888,-1.72561100564033,
12.));
#199968=CARTESIAN_POINT('Ctrl Pts',(-23.0463128785528,-1.72342320653731,
0.));
#199969=CARTESIAN_POINT('Ctrl Pts',(-23.0463128785528,-1.72342320653731,
12.));
#199970=CARTESIAN_POINT('Ctrl Pts',(-23.061537035156,-1.7211678722598,0.));
#199971=CARTESIAN_POINT('Ctrl Pts',(-23.061537035156,-1.7211678722598,12.));
#199972=CARTESIAN_POINT('Ctrl Pts',(-23.0768997860709,-1.71884453003027,
0.));
#199973=CARTESIAN_POINT('Ctrl Pts',(-23.0768997860709,-1.71884453003027,
12.));
#199974=CARTESIAN_POINT('Ctrl Pts',(-23.0923994621216,-1.71645271839311,
0.));
#199975=CARTESIAN_POINT('Ctrl Pts',(-23.0923994621216,-1.71645271839311,
12.));
#199976=CARTESIAN_POINT('Ctrl Pts',(-23.1080344254291,-1.71399198684724,
0.));
#199977=CARTESIAN_POINT('Ctrl Pts',(-23.1080344254291,-1.71399198684724,
12.));
#199978=CARTESIAN_POINT('Ctrl Pts',(-23.1238030684929,-1.71146189552192,
0.));
#199979=CARTESIAN_POINT('Ctrl Pts',(-23.1238030684929,-1.71146189552192,
12.));
#199980=CARTESIAN_POINT('Ctrl Pts',(-23.1397038132358,-1.7088620148546,
0.));
#199981=CARTESIAN_POINT('Ctrl Pts',(-23.1397038132358,-1.7088620148546,
12.));
#199982=CARTESIAN_POINT('Ctrl Pts',(-23.1557351100613,-1.70619192527847,
0.));
#199983=CARTESIAN_POINT('Ctrl Pts',(-23.1557351100613,-1.70619192527847,
12.));
#199984=CARTESIAN_POINT('Ctrl Pts',(-23.1718954368749,-1.70345121691259,
0.));
#199985=CARTESIAN_POINT('Ctrl Pts',(-23.1718954368749,-1.70345121691259,
12.));
#199986=CARTESIAN_POINT('Ctrl Pts',(-23.1881832981848,-1.70063948926987,
0.));
#199987=CARTESIAN_POINT('Ctrl Pts',(-23.1881832981848,-1.70063948926987,
12.));
#199988=CARTESIAN_POINT('Ctrl Pts',(-23.2045972243765,-1.69775635099425,
0.));
#199989=CARTESIAN_POINT('Ctrl Pts',(-23.2045972243765,-1.69775635099425,
12.));
#199990=CARTESIAN_POINT('Ctrl Pts',(-23.2211357709374,-1.69480141959945,
0.));
#199991=CARTESIAN_POINT('Ctrl Pts',(-23.2211357709374,-1.69480141959945,
12.));
#199992=CARTESIAN_POINT('Ctrl Pts',(-23.2377975177014,-1.69177432121716,
0.));
#199993=CARTESIAN_POINT('Ctrl Pts',(-23.2377975177014,-1.69177432121716,
12.));
#199994=CARTESIAN_POINT('Ctrl Pts',(-23.2545810680536,-1.6886746903491,
0.));
#199995=CARTESIAN_POINT('Ctrl Pts',(-23.2545810680536,-1.6886746903491,
12.));
#199996=CARTESIAN_POINT('Ctrl Pts',(-23.2714850482245,-1.68550216963275,
0.));
#199997=CARTESIAN_POINT('Ctrl Pts',(-23.2714850482245,-1.68550216963275,
12.));
#199998=CARTESIAN_POINT('Ctrl Pts',(-23.2885081066949,-1.68225640962181,
0.));
#199999=CARTESIAN_POINT('Ctrl Pts',(-23.2885081066949,-1.68225640962181,
12.));
#200000=CARTESIAN_POINT('Ctrl Pts',(-23.3056489135611,-1.67893706857123,
0.));
#200001=CARTESIAN_POINT('Ctrl Pts',(-23.3056489135611,-1.67893706857123,
12.));
#200002=CARTESIAN_POINT('Ctrl Pts',(-23.3229061599145,-1.67554381222987,
0.));
#200003=CARTESIAN_POINT('Ctrl Pts',(-23.3229061599145,-1.67554381222987,
12.));
#200004=CARTESIAN_POINT('Ctrl Pts',(-23.3402785571866,-1.67207631363905,
0.));
#200005=CARTESIAN_POINT('Ctrl Pts',(-23.3402785571866,-1.67207631363905,
12.));
#200006=CARTESIAN_POINT('Ctrl Pts',(-23.3577648365747,-1.66853425293977,
0.));
#200007=CARTESIAN_POINT('Ctrl Pts',(-23.3577648365747,-1.66853425293977,
12.));
#200008=CARTESIAN_POINT('Ctrl Pts',(-23.375363748555,-1.66491731718864,
0.));
#200009=CARTESIAN_POINT('Ctrl Pts',(-23.375363748555,-1.66491731718864,
12.));
#200010=CARTESIAN_POINT('Ctrl Pts',(-23.3930740623622,-1.66122520018008,
0.));
#200011=CARTESIAN_POINT('Ctrl Pts',(-23.3930740623622,-1.66122520018008,
12.));
#200012=CARTESIAN_POINT('Ctrl Pts',(-23.4108945654803,-1.65745760227507,
0.));
#200013=CARTESIAN_POINT('Ctrl Pts',(-23.4108945654803,-1.65745760227507,
12.));
#200014=CARTESIAN_POINT('Ctrl Pts',(-23.4288240631034,-1.6536142302373,
0.));
#200015=CARTESIAN_POINT('Ctrl Pts',(-23.4288240631034,-1.6536142302373,
12.));
#200016=CARTESIAN_POINT('Ctrl Pts',(-23.446861377656,-1.64969479707339,
0.));
#200017=CARTESIAN_POINT('Ctrl Pts',(-23.446861377656,-1.64969479707339,
12.));
#200018=CARTESIAN_POINT('Ctrl Pts',(-23.4650053483919,-1.64569902187608,
0.));
#200019=CARTESIAN_POINT('Ctrl Pts',(-23.4650053483919,-1.64569902187608,
12.));
#200020=CARTESIAN_POINT('Ctrl Pts',(-23.4832548309638,-1.64162662967524,
0.));
#200021=CARTESIAN_POINT('Ctrl Pts',(-23.4832548309638,-1.64162662967524,
12.));
#200022=CARTESIAN_POINT('Ctrl Pts',(-23.5016086970006,-1.63747735129474,
0.));
#200023=CARTESIAN_POINT('Ctrl Pts',(-23.5016086970006,-1.63747735129474,
12.));
#200024=CARTESIAN_POINT('Ctrl Pts',(-23.5200658336624,-1.63325092321731,
0.));
#200025=CARTESIAN_POINT('Ctrl Pts',(-23.5200658336624,-1.63325092321731,
12.));
#200026=CARTESIAN_POINT('Ctrl Pts',(-23.5386251432278,-1.62894708745231,
0.));
#200027=CARTESIAN_POINT('Ctrl Pts',(-23.5386251432278,-1.62894708745231,
12.));
#200028=CARTESIAN_POINT('Ctrl Pts',(-23.5572855427617,-1.62456559140072,
0.));
#200029=CARTESIAN_POINT('Ctrl Pts',(-23.5572855427617,-1.62456559140072,
12.));
#200030=CARTESIAN_POINT('Ctrl Pts',(-23.5760459637608,-1.62010618772869,
0.));
#200031=CARTESIAN_POINT('Ctrl Pts',(-23.5760459637608,-1.62010618772869,
12.));
#200032=CARTESIAN_POINT('Ctrl Pts',(-23.5949053517996,-1.61556863424697,
0.));
#200033=CARTESIAN_POINT('Ctrl Pts',(-23.5949053517996,-1.61556863424697,
12.));
#200034=CARTESIAN_POINT('Ctrl Pts',(-23.6138626661644,-1.61095269379773,
0.));
#200035=CARTESIAN_POINT('Ctrl Pts',(-23.6138626661644,-1.61095269379773,
12.));
#200036=CARTESIAN_POINT('Ctrl Pts',(-23.6329168794916,-1.60625813414666,
0.));
#200037=CARTESIAN_POINT('Ctrl Pts',(-23.6329168794916,-1.60625813414666,
12.));
#200038=CARTESIAN_POINT('Ctrl Pts',(-23.6520669774863,-1.60148472786588,
0.));
#200039=CARTESIAN_POINT('Ctrl Pts',(-23.6520669774863,-1.60148472786588,
12.));
#200040=CARTESIAN_POINT('Ctrl Pts',(-23.6713119586302,-1.59663225222458,
0.));
#200041=CARTESIAN_POINT('Ctrl Pts',(-23.6713119586302,-1.59663225222458,
12.));
#200042=CARTESIAN_POINT('Ctrl Pts',(-23.6906508338833,-1.59170048908631,
0.));
#200043=CARTESIAN_POINT('Ctrl Pts',(-23.6906508338833,-1.59170048908631,
12.));
#200044=CARTESIAN_POINT('Ctrl Pts',(-23.7100826263835,-1.58668922481222,
0.));
#200045=CARTESIAN_POINT('Ctrl Pts',(-23.7100826263835,-1.58668922481222,
12.));
#200046=CARTESIAN_POINT('Ctrl Pts',(-23.7296063711308,-1.58159825017362,
0.));
#200047=CARTESIAN_POINT('Ctrl Pts',(-23.7296063711308,-1.58159825017362,
12.));
#200048=CARTESIAN_POINT('Ctrl Pts',(-23.7492211147369,-1.57642736025251,
0.));
#200049=CARTESIAN_POINT('Ctrl Pts',(-23.7492211147369,-1.57642736025251,
12.));
#200050=CARTESIAN_POINT('Ctrl Pts',(-23.7689259151869,-1.57117635434412,
0.));
#200051=CARTESIAN_POINT('Ctrl Pts',(-23.7689259151869,-1.57117635434412,
12.));
#200052=CARTESIAN_POINT('Ctrl Pts',(-23.788719841588,-1.56584503586844,
0.));
#200053=CARTESIAN_POINT('Ctrl Pts',(-23.788719841588,-1.56584503586844,
12.));
#200054=CARTESIAN_POINT('Ctrl Pts',(-23.8086019739192,-1.56043321228631,
0.));
#200055=CARTESIAN_POINT('Ctrl Pts',(-23.8086019739192,-1.56043321228631,
12.));
#200056=CARTESIAN_POINT('Ctrl Pts',(-23.8285714027631,-1.55494069502628,
0.));
#200057=CARTESIAN_POINT('Ctrl Pts',(-23.8285714027631,-1.55494069502628,
12.));
#200058=CARTESIAN_POINT('Ctrl Pts',(-23.8486272290698,-1.5493672994053,
0.));
#200059=CARTESIAN_POINT('Ctrl Pts',(-23.8486272290698,-1.5493672994053,
12.));
#200060=CARTESIAN_POINT('Ctrl Pts',(-23.8687685639635,-1.54371284453978,
0.));
#200061=CARTESIAN_POINT('Ctrl Pts',(-23.8687685639635,-1.54371284453978,
12.));
#200062=CARTESIAN_POINT('Ctrl Pts',(-23.8889945285313,-1.53797715326748,
0.));
#200063=CARTESIAN_POINT('Ctrl Pts',(-23.8889945285313,-1.53797715326748,
12.));
#200064=CARTESIAN_POINT('Ctrl Pts',(-23.9093042536119,-1.53216005207462,
0.));
#200065=CARTESIAN_POINT('Ctrl Pts',(-23.9093042536119,-1.53216005207462,
12.));
#200066=CARTESIAN_POINT('Ctrl Pts',(-23.9296968795761,-1.52626137103039,
0.));
#200067=CARTESIAN_POINT('Ctrl Pts',(-23.9296968795761,-1.52626137103039,
12.));
#200068=CARTESIAN_POINT('Ctrl Pts',(-23.9501715561038,-1.52028094372806,
0.));
#200069=CARTESIAN_POINT('Ctrl Pts',(-23.9501715561038,-1.52028094372806,
12.));
#200070=CARTESIAN_POINT('Ctrl Pts',(-23.9707274420145,-1.51421860720628,
0.));
#200071=CARTESIAN_POINT('Ctrl Pts',(-23.9707274420145,-1.51421860720628,
12.));
#200072=CARTESIAN_POINT('Ctrl Pts',(-23.991363705093,-1.50807420187702,
0.));
#200073=CARTESIAN_POINT('Ctrl Pts',(-23.991363705093,-1.50807420187702,
12.));
#200074=CARTESIAN_POINT('Ctrl Pts',(-24.0120795219086,-1.50184757146099,
0.));
#200075=CARTESIAN_POINT('Ctrl Pts',(-24.0120795219086,-1.50184757146099,
12.));
#200076=CARTESIAN_POINT('Ctrl Pts',(-24.0328740776331,-1.49553856292798,
0.));
#200077=CARTESIAN_POINT('Ctrl Pts',(-24.0328740776331,-1.49553856292798,
12.));
#200078=CARTESIAN_POINT('Ctrl Pts',(-24.053746565843,-1.48914702644883,
0.));
#200079=CARTESIAN_POINT('Ctrl Pts',(-24.053746565843,-1.48914702644883,
12.));
#200080=CARTESIAN_POINT('Ctrl Pts',(-24.074696188353,-1.4826728153368,0.));
#200081=CARTESIAN_POINT('Ctrl Pts',(-24.074696188353,-1.4826728153368,12.));
#200082=CARTESIAN_POINT('Ctrl Pts',(-24.0957221550782,-1.47611578597741,
0.));
#200083=CARTESIAN_POINT('Ctrl Pts',(-24.0957221550782,-1.47611578597741,
12.));
#200084=CARTESIAN_POINT('Ctrl Pts',(-24.1168236838827,-1.46947579776992,
0.));
#200085=CARTESIAN_POINT('Ctrl Pts',(-24.1168236838827,-1.46947579776992,
12.));
#200086=CARTESIAN_POINT('Ctrl Pts',(-24.1380000004272,-1.46275271307398,
0.));
#200087=CARTESIAN_POINT('Ctrl Pts',(-24.1380000004272,-1.46275271307398,
12.));
#200088=CARTESIAN_POINT('Ctrl Pts',(-24.1592503380105,-1.45594639716314,
0.));
#200089=CARTESIAN_POINT('Ctrl Pts',(-24.1592503380105,-1.45594639716314,
12.));
#200090=CARTESIAN_POINT('Ctrl Pts',(-24.1805739374033,-1.44905671818721,
0.));
#200091=CARTESIAN_POINT('Ctrl Pts',(-24.1805739374033,-1.44905671818721,
12.));
#200092=CARTESIAN_POINT('Ctrl Pts',(-24.2019700467214,-1.44208354711074,
0.));
#200093=CARTESIAN_POINT('Ctrl Pts',(-24.2019700467214,-1.44208354711074,
12.));
#200094=CARTESIAN_POINT('Ctrl Pts',(-24.2234379212978,-1.43502675765502,
0.));
#200095=CARTESIAN_POINT('Ctrl Pts',(-24.2234379212978,-1.43502675765502,
12.));
#200096=CARTESIAN_POINT('Ctrl Pts',(-24.2449768235485,-1.42788622624851,
0.));
#200097=CARTESIAN_POINT('Ctrl Pts',(-24.2449768235485,-1.42788622624851,
12.));
#200098=CARTESIAN_POINT('Ctrl Pts',(-24.2665860228357,-1.42066183198252,
0.));
#200099=CARTESIAN_POINT('Ctrl Pts',(-24.2665860228357,-1.42066183198252,
12.));
#200100=CARTESIAN_POINT('Ctrl Pts',(-24.2882647953214,-1.41335345657685,
0.));
#200101=CARTESIAN_POINT('Ctrl Pts',(-24.2882647953214,-1.41335345657685,
12.));
#200102=CARTESIAN_POINT('Ctrl Pts',(-24.3100124238316,-1.4059609843434,
0.));
#200103=CARTESIAN_POINT('Ctrl Pts',(-24.3100124238316,-1.4059609843434,
12.));
#200104=CARTESIAN_POINT('Ctrl Pts',(-24.3318281977647,-1.3984843021281,
0.));
#200105=CARTESIAN_POINT('Ctrl Pts',(-24.3318281977647,-1.3984843021281,
12.));
#200106=CARTESIAN_POINT('Ctrl Pts',(-24.3537114129877,-1.3909232992639,
0.));
#200107=CARTESIAN_POINT('Ctrl Pts',(-24.3537114129877,-1.3909232992639,
12.));
#200108=CARTESIAN_POINT('Ctrl Pts',(-24.37566137173,-1.38327786752998,0.));
#200109=CARTESIAN_POINT('Ctrl Pts',(-24.37566137173,-1.38327786752998,12.));
#200110=CARTESIAN_POINT('Ctrl Pts',(-24.3976773824731,-1.37554790111607,
0.));
#200111=CARTESIAN_POINT('Ctrl Pts',(-24.3976773824731,-1.37554790111607,
12.));
#200112=CARTESIAN_POINT('Ctrl Pts',(-24.4197587598337,-1.36773329659954,
0.));
#200113=CARTESIAN_POINT('Ctrl Pts',(-24.4197587598337,-1.36773329659954,
12.));
#200114=CARTESIAN_POINT('Ctrl Pts',(-24.4419048244524,-1.35983395290624,
0.));
#200115=CARTESIAN_POINT('Ctrl Pts',(-24.4419048244524,-1.35983395290624,
12.));
#200116=CARTESIAN_POINT('Ctrl Pts',(-24.4641149028894,-1.35184977125644,
0.));
#200117=CARTESIAN_POINT('Ctrl Pts',(-24.4641149028894,-1.35184977125644,
12.));
#200118=CARTESIAN_POINT('Ctrl Pts',(-24.4863883275135,-1.34378065512335,
0.));
#200119=CARTESIAN_POINT('Ctrl Pts',(-24.4863883275135,-1.34378065512335,
12.));
#200120=CARTESIAN_POINT('Ctrl Pts',(-24.5087244363856,-1.33562651019684,
0.));
#200121=CARTESIAN_POINT('Ctrl Pts',(-24.5087244363856,-1.33562651019684,
12.));
#200122=CARTESIAN_POINT('Ctrl Pts',(-24.5311225731434,-1.32738724435326,
0.));
#200123=CARTESIAN_POINT('Ctrl Pts',(-24.5311225731434,-1.32738724435326,
12.));
#200124=CARTESIAN_POINT('Ctrl Pts',(-24.5535820868671,-1.31906276763669,
0.));
#200125=CARTESIAN_POINT('Ctrl Pts',(-24.5535820868671,-1.31906276763669,
12.));
#200126=CARTESIAN_POINT('Ctrl Pts',(-24.576102332018,-1.31065299222023,
0.));
#200127=CARTESIAN_POINT('Ctrl Pts',(-24.576102332018,-1.31065299222023,
12.));
#200128=CARTESIAN_POINT('Ctrl Pts',(-24.5986826684025,-1.30215783236364,
0.));
#200129=CARTESIAN_POINT('Ctrl Pts',(-24.5986826684025,-1.30215783236364,
12.));
#200130=CARTESIAN_POINT('Ctrl Pts',(-24.6213224611228,-1.29357720438107,
0.));
#200131=CARTESIAN_POINT('Ctrl Pts',(-24.6213224611228,-1.29357720438107,
12.));
#200132=CARTESIAN_POINT('Ctrl Pts',(-24.6440210805278,-1.28491102661513,
0.));
#200133=CARTESIAN_POINT('Ctrl Pts',(-24.6440210805278,-1.28491102661513,
12.));
#200134=CARTESIAN_POINT('Ctrl Pts',(-24.666777902156,-1.2761592194164,0.));
#200135=CARTESIAN_POINT('Ctrl Pts',(-24.666777902156,-1.2761592194164,12.));
#200136=CARTESIAN_POINT('Ctrl Pts',(-24.6895923066837,-1.26732170513497,
0.));
#200137=CARTESIAN_POINT('Ctrl Pts',(-24.6895923066837,-1.26732170513497,
12.));
#200138=CARTESIAN_POINT('Ctrl Pts',(-24.7124636797895,-1.25839840807415,
0.));
#200139=CARTESIAN_POINT('Ctrl Pts',(-24.7124636797895,-1.25839840807415,
12.));
#200140=CARTESIAN_POINT('Ctrl Pts',(-24.7353914120012,-1.24938925444323,
0.));
#200141=CARTESIAN_POINT('Ctrl Pts',(-24.7353914120012,-1.24938925444323,
12.));
#200142=CARTESIAN_POINT('Ctrl Pts',(-24.7583748985439,-1.24029417231988,
0.));
#200143=CARTESIAN_POINT('Ctrl Pts',(-24.7583748985439,-1.24029417231988,
12.));
#200144=CARTESIAN_POINT('Ctrl Pts',(-24.78141353918,-1.23111309161843,0.));
#200145=CARTESIAN_POINT('Ctrl Pts',(-24.78141353918,-1.23111309161843,12.));
#200146=CARTESIAN_POINT('Ctrl Pts',(-24.8045067380536,-1.22184594406526,
0.));
#200147=CARTESIAN_POINT('Ctrl Pts',(-24.8045067380536,-1.22184594406526,
12.));
#200148=CARTESIAN_POINT('Ctrl Pts',(-24.8276539035092,-1.21249266318205,
0.));
#200149=CARTESIAN_POINT('Ctrl Pts',(-24.8276539035092,-1.21249266318205,
12.));
#200150=CARTESIAN_POINT('Ctrl Pts',(-24.8508544481973,-1.20305318426015,
0.));
#200151=CARTESIAN_POINT('Ctrl Pts',(-24.8508544481973,-1.20305318426015,
12.));
#200152=CARTESIAN_POINT('Ctrl Pts',(-24.8741077892074,-1.19352744434059,
0.));
#200153=CARTESIAN_POINT('Ctrl Pts',(-24.8741077892074,-1.19352744434059,
12.));
#200154=CARTESIAN_POINT('Ctrl Pts',(-24.8974133481829,-1.18391538220098,
0.));
#200155=CARTESIAN_POINT('Ctrl Pts',(-24.8974133481829,-1.18391538220098,
12.));
#200156=CARTESIAN_POINT('Ctrl Pts',(-24.9207705514449,-1.17421693835039,
0.));
#200157=CARTESIAN_POINT('Ctrl Pts',(-24.9207705514449,-1.17421693835039,
12.));
#200158=CARTESIAN_POINT('Ctrl Pts',(-24.9441788300932,-1.16443205502852,
0.));
#200159=CARTESIAN_POINT('Ctrl Pts',(-24.9441788300932,-1.16443205502852,
12.));
#200160=CARTESIAN_POINT('Ctrl Pts',(-24.9676376201501,-1.15456067621894,
0.));
#200161=CARTESIAN_POINT('Ctrl Pts',(-24.9676376201501,-1.15456067621894,
12.));
#200162=CARTESIAN_POINT('Ctrl Pts',(-24.9911463621431,-1.14460274758206,
0.));
#200163=CARTESIAN_POINT('Ctrl Pts',(-24.9911463621431,-1.14460274758206,
12.));
#200164=CARTESIAN_POINT('Ctrl Pts',(-25.0147045006193,-1.13455821638535,
0.));
#200165=CARTESIAN_POINT('Ctrl Pts',(-25.0147045006193,-1.13455821638535,
12.));
#200166=CARTESIAN_POINT('Ctrl Pts',(-25.0383114836898,-1.12442703144455,
0.));
#200167=CARTESIAN_POINT('Ctrl Pts',(-25.0383114836898,-1.12442703144455,
12.));
#200168=CARTESIAN_POINT('Ctrl Pts',(-25.0619667625336,-1.1142091430689,
0.));
#200169=CARTESIAN_POINT('Ctrl Pts',(-25.0619667625336,-1.1142091430689,
12.));
#200170=CARTESIAN_POINT('Ctrl Pts',(-25.085669790968,-1.1039045030174,0.));
#200171=CARTESIAN_POINT('Ctrl Pts',(-25.085669790968,-1.1039045030174,12.));
#200172=CARTESIAN_POINT('Ctrl Pts',(-25.1094200248448,-1.09351306445299,
0.));
#200173=CARTESIAN_POINT('Ctrl Pts',(-25.1094200248448,-1.09351306445299,
12.));
#200174=CARTESIAN_POINT('Ctrl Pts',(-25.1332169227415,-1.08303478197174,
0.));
#200175=CARTESIAN_POINT('Ctrl Pts',(-25.1332169227415,-1.08303478197174,
12.));
#200176=CARTESIAN_POINT('Ctrl Pts',(-25.1570599469311,-1.0724696116546,
0.));
#200177=CARTESIAN_POINT('Ctrl Pts',(-25.1570599469311,-1.0724696116546,
12.));
#200178=CARTESIAN_POINT('Ctrl Pts',(-25.1809485642191,-1.06181751111754,
0.));
#200179=CARTESIAN_POINT('Ctrl Pts',(-25.1809485642191,-1.06181751111754,
12.));
#200180=CARTESIAN_POINT('Ctrl Pts',(-25.2048822469027,-1.05107843957925,
0.));
#200181=CARTESIAN_POINT('Ctrl Pts',(-25.2048822469027,-1.05107843957925,
12.));
#200182=CARTESIAN_POINT('Ctrl Pts',(-25.2288604735087,-1.04025235791515,
0.));
#200183=CARTESIAN_POINT('Ctrl Pts',(-25.2288604735087,-1.04025235791515,
12.));
#200184=CARTESIAN_POINT('Ctrl Pts',(-25.2528827300427,-1.0293392287683,
0.));
#200185=CARTESIAN_POINT('Ctrl Pts',(-25.2528827300427,-1.0293392287683,
12.));
#200186=CARTESIAN_POINT('Ctrl Pts',(-25.2769485087268,-1.01833901642272,
0.));
#200187=CARTESIAN_POINT('Ctrl Pts',(-25.2769485087268,-1.01833901642272,
12.));
#200188=CARTESIAN_POINT('Ctrl Pts',(-25.3010573055557,-1.00725168656933,
0.));
#200189=CARTESIAN_POINT('Ctrl Pts',(-25.3010573055557,-1.00725168656933,
12.));
#200190=CARTESIAN_POINT('Ctrl Pts',(-25.3252086182976,-0.996077206120919,
0.));
#200191=CARTESIAN_POINT('Ctrl Pts',(-25.3252086182976,-0.996077206120919,
12.));
#200192=CARTESIAN_POINT('Ctrl Pts',(-25.3494019441444,-0.984815543004089,
0.));
#200193=CARTESIAN_POINT('Ctrl Pts',(-25.3494019441444,-0.984815543004089,
12.));
#200194=CARTESIAN_POINT('Ctrl Pts',(-25.3736367778842,-0.973466666000048,
0.));
#200195=CARTESIAN_POINT('Ctrl Pts',(-25.3736367778842,-0.973466666000048,
12.));
#200196=CARTESIAN_POINT('Ctrl Pts',(-25.3979126089155,-0.962030544502802,
0.));
#200197=CARTESIAN_POINT('Ctrl Pts',(-25.3979126089155,-0.962030544502802,
12.));
#200198=CARTESIAN_POINT('Ctrl Pts',(-25.4222289223155,-0.950507148596968,
0.));
#200199=CARTESIAN_POINT('Ctrl Pts',(-25.4222289223155,-0.950507148596968,
12.));
#200200=CARTESIAN_POINT('Ctrl Pts',(-25.4465852044835,-0.938896449495632,
0.));
#200201=CARTESIAN_POINT('Ctrl Pts',(-25.4465852044835,-0.938896449495632,
12.));
#200202=CARTESIAN_POINT('Ctrl Pts',(-25.4709809474996,-0.927198419885604,
0.));
#200203=CARTESIAN_POINT('Ctrl Pts',(-25.4709809474996,-0.927198419885604,
12.));
#200204=CARTESIAN_POINT('Ctrl Pts',(-25.4954156541787,-0.915413034335333,
0.));
#200205=CARTESIAN_POINT('Ctrl Pts',(-25.4954156541787,-0.915413034335333,
12.));
#200206=CARTESIAN_POINT('Ctrl Pts',(-25.5198888424195,-0.903540269651154,
0.));
#200207=CARTESIAN_POINT('Ctrl Pts',(-25.5198888424195,-0.903540269651154,
12.));
#200208=CARTESIAN_POINT('Ctrl Pts',(-25.5444000508223,-0.891580105349467,
0.));
#200209=CARTESIAN_POINT('Ctrl Pts',(-25.5444000508223,-0.891580105349467,
12.));
#200210=CARTESIAN_POINT('Ctrl Pts',(-25.568948840818,-0.87953252383509,
0.));
#200211=CARTESIAN_POINT('Ctrl Pts',(-25.568948840818,-0.87953252383509,
12.));
#200212=CARTESIAN_POINT('Ctrl Pts',(-25.5935347843616,-0.86739750933947,
0.));
#200213=CARTESIAN_POINT('Ctrl Pts',(-25.5935347843616,-0.86739750933947,
12.));
#200214=CARTESIAN_POINT('Ctrl Pts',(-25.618157453608,-0.855175047037614,
0.));
#200215=CARTESIAN_POINT('Ctrl Pts',(-25.618157453608,-0.855175047037614,
12.));
#200216=CARTESIAN_POINT('Ctrl Pts',(-25.6428164100078,-0.842865122121544,
0.));
#200217=CARTESIAN_POINT('Ctrl Pts',(-25.6428164100078,-0.842865122121544,
12.));
#200218=CARTESIAN_POINT('Ctrl Pts',(-25.6675111931957,-0.830467718864367,
0.));
#200219=CARTESIAN_POINT('Ctrl Pts',(-25.6675111931957,-0.830467718864367,
12.));
#200220=CARTESIAN_POINT('Ctrl Pts',(-25.6922413110172,-0.817982819786719,
0.));
#200221=CARTESIAN_POINT('Ctrl Pts',(-25.6922413110172,-0.817982819786719,
12.));
#200222=CARTESIAN_POINT('Ctrl Pts',(-25.7170062262474,-0.805410404552594,
0.));
#200223=CARTESIAN_POINT('Ctrl Pts',(-25.7170062262474,-0.805410404552594,
12.));
#200224=CARTESIAN_POINT('Ctrl Pts',(-25.7418053757671,-0.792750451613534,
0.));
#200225=CARTESIAN_POINT('Ctrl Pts',(-25.7418053757671,-0.792750451613534,
12.));
#200226=CARTESIAN_POINT('Ctrl Pts',(-25.7666381946871,-0.780002940289025,
0.));
#200227=CARTESIAN_POINT('Ctrl Pts',(-25.7666381946871,-0.780002940289025,
12.));
#200228=CARTESIAN_POINT('Ctrl Pts',(-25.7915041383304,-0.767167852648639,
0.));
#200229=CARTESIAN_POINT('Ctrl Pts',(-25.7915041383304,-0.767167852648639,
12.));
#200230=CARTESIAN_POINT('Ctrl Pts',(-25.816402705995,-0.754245175608288,
0.));
#200231=CARTESIAN_POINT('Ctrl Pts',(-25.816402705995,-0.754245175608288,
12.));
#200232=CARTESIAN_POINT('Ctrl Pts',(-25.841333461908,-0.741234902664697,
0.));
#200233=CARTESIAN_POINT('Ctrl Pts',(-25.841333461908,-0.741234902664697,
12.));
#200234=CARTESIAN_POINT('Ctrl Pts',(-25.8662960624285,-0.728137036485877,
0.));
#200235=CARTESIAN_POINT('Ctrl Pts',(-25.8662960624285,-0.728137036485877,
12.));
#200236=CARTESIAN_POINT('Ctrl Pts',(-25.8912902615141,-0.714951588533753,
0.));
#200237=CARTESIAN_POINT('Ctrl Pts',(-25.8912902615141,-0.714951588533753,
12.));
#200238=CARTESIAN_POINT('Ctrl Pts',(-25.9163158909645,-0.701678575236602,
0.));
#200239=CARTESIAN_POINT('Ctrl Pts',(-25.9163158909645,-0.701678575236602,
12.));
#200240=CARTESIAN_POINT('Ctrl Pts',(-25.941372847213,-0.688318015065678,
0.));
#200241=CARTESIAN_POINT('Ctrl Pts',(-25.941372847213,-0.688318015065678,
12.));
#200242=CARTESIAN_POINT('Ctrl Pts',(-25.9614434298092,-0.677559543215902,
0.));
#200243=CARTESIAN_POINT('Ctrl Pts',(-25.9614434298092,-0.677559543215902,
12.));
#200244=CARTESIAN_POINT('Ctrl Pts',(-25.9765104298171,-0.669451306784415,
0.));
#200245=CARTESIAN_POINT('Ctrl Pts',(-25.9765104298171,-0.669451306784415,
12.));
#200246=CARTESIAN_POINT('Ctrl Pts',(-25.9865613464809,-0.664028313188912,
0.));
#200247=CARTESIAN_POINT('Ctrl Pts',(-25.9865613464809,-0.664028313188912,
12.));
#200248=CARTESIAN_POINT('Ctrl Pts',(-25.991588367311,-0.661312440730891,
0.));
#200249=CARTESIAN_POINT('Ctrl Pts',(-25.991588367311,-0.661312440730891,
12.));
#200250=CARTESIAN_POINT('',(-25.991588367311,-0.661312440730891,0.));
#200251=CARTESIAN_POINT('Ctrl Pts',(-22.4835757167854,-1.76341220531179,
0.));
#200252=CARTESIAN_POINT('Ctrl Pts',(-22.483581992979,-1.76341415538764,
0.));
#200253=CARTESIAN_POINT('Ctrl Pts',(-22.4836387052232,-1.7634206426357,
0.));
#200254=CARTESIAN_POINT('Ctrl Pts',(-22.483856251707,-1.76343813434565,
0.));
#200255=CARTESIAN_POINT('Ctrl Pts',(-22.4844112933129,-1.76347698284792,
0.));
#200256=CARTESIAN_POINT('Ctrl Pts',(-22.4855446605991,-1.76355076045546,
0.));
#200257=CARTESIAN_POINT('Ctrl Pts',(-22.4871115206571,-1.76364784232963,
0.));
#200258=CARTESIAN_POINT('Ctrl Pts',(-22.4890991659478,-1.76376424879505,
0.));
#200259=CARTESIAN_POINT('Ctrl Pts',(-22.4914909094908,-1.76389475965724,
0.));
#200260=CARTESIAN_POINT('Ctrl Pts',(-22.4942693792449,-1.764033938803,0.));
#200261=CARTESIAN_POINT('Ctrl Pts',(-22.4974203063191,-1.76417731243462,
0.));
#200262=CARTESIAN_POINT('Ctrl Pts',(-22.5009332677316,-1.76432160068725,
0.));
#200263=CARTESIAN_POINT('Ctrl Pts',(-22.5047996391978,-1.76446408210366,
0.));
#200264=CARTESIAN_POINT('Ctrl Pts',(-22.5090112700212,-1.76460218257323,
0.));
#200265=CARTESIAN_POINT('Ctrl Pts',(-22.5135590569554,-1.76473303281159,
0.));
#200266=CARTESIAN_POINT('Ctrl Pts',(-22.5184336670207,-1.76485369319896,
0.));
#200267=CARTESIAN_POINT('Ctrl Pts',(-22.5236259635515,-1.76496128643369,
0.));
#200268=CARTESIAN_POINT('Ctrl Pts',(-22.529127665298,-1.76505320262751,
0.));
#200269=CARTESIAN_POINT('Ctrl Pts',(-22.5349313983571,-1.7651271156325,
0.));
#200270=CARTESIAN_POINT('Ctrl Pts',(-22.5410303590891,-1.76518087841492,
0.));
#200271=CARTESIAN_POINT('Ctrl Pts',(-22.5474180954006,-1.76521245524047,
0.));
#200272=CARTESIAN_POINT('Ctrl Pts',(-22.5540882235837,-1.76521983384063,
0.));
#200273=CARTESIAN_POINT('Ctrl Pts',(-22.5610344912501,-1.76520104500449,
0.));
#200274=CARTESIAN_POINT('Ctrl Pts',(-22.5682508499873,-1.76515418518829,
0.));
#200275=CARTESIAN_POINT('Ctrl Pts',(-22.5757315316355,-1.76507744026747,
0.));
#200276=CARTESIAN_POINT('Ctrl Pts',(-22.5834711038024,-1.76496910283088,
0.));
#200277=CARTESIAN_POINT('Ctrl Pts',(-22.5914644078106,-1.76482755288411,
0.));
#200278=CARTESIAN_POINT('Ctrl Pts',(-22.5997065145638,-1.76465124413556,
0.));
#200279=CARTESIAN_POINT('Ctrl Pts',(-22.6081926681342,-1.76443868648015,
0.));
#200280=CARTESIAN_POINT('Ctrl Pts',(-22.6169182517693,-1.76418843543739,
0.));
#200281=CARTESIAN_POINT('Ctrl Pts',(-22.6258787994847,-1.76389909571402,
0.));
#200282=CARTESIAN_POINT('Ctrl Pts',(-22.635069997936,-1.76356932176272,
0.));
#200283=CARTESIAN_POINT('Ctrl Pts',(-22.6444876940425,-1.76319782013914,
0.));
#200284=CARTESIAN_POINT('Ctrl Pts',(-22.6541278938413,-1.76278334912559,
0.));
#200285=CARTESIAN_POINT('Ctrl Pts',(-22.6639867471756,-1.76232471392567,
0.));
#200286=CARTESIAN_POINT('Ctrl Pts',(-22.6740605356699,-1.76182076289525,
0.));
#200287=CARTESIAN_POINT('Ctrl Pts',(-22.6843456585245,-1.76127038310612,
0.));
#200288=CARTESIAN_POINT('Ctrl Pts',(-22.6948386219843,-1.76067249704884,
0.));
#200289=CARTESIAN_POINT('Ctrl Pts',(-22.7055360375481,-1.76002606202399,
0.));
#200290=CARTESIAN_POINT('Ctrl Pts',(-22.7164346186007,-1.75933006905924,
0.));
#200291=CARTESIAN_POINT('Ctrl Pts',(-22.7275311777305,-1.75858354204635,
0.));
#200292=CARTESIAN_POINT('Ctrl Pts',(-22.7388226235565,-1.75778553673249,
0.));
#200293=CARTESIAN_POINT('Ctrl Pts',(-22.7503059556455,-1.75693513908911,
0.));
#200294=CARTESIAN_POINT('Ctrl Pts',(-22.7619782595013,-1.7560314637164,
0.));
#200295=CARTESIAN_POINT('Ctrl Pts',(-22.7738367016115,-1.75507365227127,
0.));
#200296=CARTESIAN_POINT('Ctrl Pts',(-22.7858785242358,-1.75406087182929,
0.));
#200297=CARTESIAN_POINT('Ctrl Pts',(-22.7981010424312,-1.75299231391461,
0.));
#200298=CARTESIAN_POINT('Ctrl Pts',(-22.8105016414712,-1.75186719365589,
0.));
#200299=CARTESIAN_POINT('Ctrl Pts',(-22.8230777741285,-1.75068474890884,
0.));
#200300=CARTESIAN_POINT('Ctrl Pts',(-22.8358269579854,-1.74944423940117,
0.));
#200301=CARTESIAN_POINT('Ctrl Pts',(-22.8487467728075,-1.74814494588492,
0.));
#200302=CARTESIAN_POINT('Ctrl Pts',(-22.8618348580234,-1.74678616930663,
0.));
#200303=CARTESIAN_POINT('Ctrl Pts',(-22.8750889101696,-1.745367229982,0.));
#200304=CARTESIAN_POINT('Ctrl Pts',(-22.8885066803351,-1.74388746677702,
0.));
#200305=CARTESIAN_POINT('Ctrl Pts',(-22.9020859716144,-1.74234623630079,
0.));
#200306=CARTESIAN_POINT('Ctrl Pts',(-22.9158246373365,-1.74074291231057,
0.));
#200307=CARTESIAN_POINT('Ctrl Pts',(-22.9297205792587,-1.73907688511664,
0.));
#200308=CARTESIAN_POINT('Ctrl Pts',(-22.9437717457825,-1.73734756100038,
0.));
#200309=CARTESIAN_POINT('Ctrl Pts',(-22.9579761301062,-1.73555436162771,
0.));
#200310=CARTESIAN_POINT('Ctrl Pts',(-22.9723317685688,-1.73369672350817,
0.));
#200311=CARTESIAN_POINT('Ctrl Pts',(-22.9868367391978,-1.73177409750193,
0.));
#200312=CARTESIAN_POINT('Ctrl Pts',(-23.0014891601891,-1.72978594832137,
0.));
#200313=CARTESIAN_POINT('Ctrl Pts',(-23.0162871884167,-1.72773175404702,
0.));
#200314=CARTESIAN_POINT('Ctrl Pts',(-23.031229017888,-1.72561100564033,
0.));
#200315=CARTESIAN_POINT('Ctrl Pts',(-23.0463128785528,-1.72342320653731,
0.));
#200316=CARTESIAN_POINT('Ctrl Pts',(-23.061537035156,-1.7211678722598,0.));
#200317=CARTESIAN_POINT('Ctrl Pts',(-23.0768997860709,-1.71884453003027,
0.));
#200318=CARTESIAN_POINT('Ctrl Pts',(-23.0923994621216,-1.71645271839311,
0.));
#200319=CARTESIAN_POINT('Ctrl Pts',(-23.1080344254291,-1.71399198684724,
0.));
#200320=CARTESIAN_POINT('Ctrl Pts',(-23.1238030684929,-1.71146189552192,
0.));
#200321=CARTESIAN_POINT('Ctrl Pts',(-23.1397038132358,-1.7088620148546,
0.));
#200322=CARTESIAN_POINT('Ctrl Pts',(-23.1557351100613,-1.70619192527847,
0.));
#200323=CARTESIAN_POINT('Ctrl Pts',(-23.1718954368749,-1.70345121691259,
0.));
#200324=CARTESIAN_POINT('Ctrl Pts',(-23.1881832981848,-1.70063948926987,
0.));
#200325=CARTESIAN_POINT('Ctrl Pts',(-23.2045972243765,-1.69775635099425,
0.));
#200326=CARTESIAN_POINT('Ctrl Pts',(-23.2211357709374,-1.69480141959945,
0.));
#200327=CARTESIAN_POINT('Ctrl Pts',(-23.2377975177014,-1.69177432121716,
0.));
#200328=CARTESIAN_POINT('Ctrl Pts',(-23.2545810680536,-1.6886746903491,
0.));
#200329=CARTESIAN_POINT('Ctrl Pts',(-23.2714850482245,-1.68550216963275,
0.));
#200330=CARTESIAN_POINT('Ctrl Pts',(-23.2885081066949,-1.68225640962181,
0.));
#200331=CARTESIAN_POINT('Ctrl Pts',(-23.3056489135611,-1.67893706857123,
0.));
#200332=CARTESIAN_POINT('Ctrl Pts',(-23.3229061599145,-1.67554381222987,
0.));
#200333=CARTESIAN_POINT('Ctrl Pts',(-23.3402785571866,-1.67207631363905,
0.));
#200334=CARTESIAN_POINT('Ctrl Pts',(-23.3577648365747,-1.66853425293977,
0.));
#200335=CARTESIAN_POINT('Ctrl Pts',(-23.375363748555,-1.66491731718864,
0.));
#200336=CARTESIAN_POINT('Ctrl Pts',(-23.3930740623622,-1.66122520018008,
0.));
#200337=CARTESIAN_POINT('Ctrl Pts',(-23.4108945654803,-1.65745760227507,
0.));
#200338=CARTESIAN_POINT('Ctrl Pts',(-23.4288240631034,-1.6536142302373,
0.));
#200339=CARTESIAN_POINT('Ctrl Pts',(-23.446861377656,-1.64969479707339,
0.));
#200340=CARTESIAN_POINT('Ctrl Pts',(-23.4650053483919,-1.64569902187608,
0.));
#200341=CARTESIAN_POINT('Ctrl Pts',(-23.4832548309638,-1.64162662967524,
0.));
#200342=CARTESIAN_POINT('Ctrl Pts',(-23.5016086970006,-1.63747735129474,
0.));
#200343=CARTESIAN_POINT('Ctrl Pts',(-23.5200658336624,-1.63325092321731,
0.));
#200344=CARTESIAN_POINT('Ctrl Pts',(-23.5386251432278,-1.62894708745231,
0.));
#200345=CARTESIAN_POINT('Ctrl Pts',(-23.5572855427617,-1.62456559140072,
0.));
#200346=CARTESIAN_POINT('Ctrl Pts',(-23.5760459637608,-1.62010618772869,
0.));
#200347=CARTESIAN_POINT('Ctrl Pts',(-23.5949053517996,-1.61556863424697,
0.));
#200348=CARTESIAN_POINT('Ctrl Pts',(-23.6138626661644,-1.61095269379773,
0.));
#200349=CARTESIAN_POINT('Ctrl Pts',(-23.6329168794916,-1.60625813414666,
0.));
#200350=CARTESIAN_POINT('Ctrl Pts',(-23.6520669774863,-1.60148472786588,
0.));
#200351=CARTESIAN_POINT('Ctrl Pts',(-23.6713119586302,-1.59663225222458,
0.));
#200352=CARTESIAN_POINT('Ctrl Pts',(-23.6906508338833,-1.59170048908631,
0.));
#200353=CARTESIAN_POINT('Ctrl Pts',(-23.7100826263835,-1.58668922481222,
0.));
#200354=CARTESIAN_POINT('Ctrl Pts',(-23.7296063711308,-1.58159825017362,
0.));
#200355=CARTESIAN_POINT('Ctrl Pts',(-23.7492211147369,-1.57642736025251,
0.));
#200356=CARTESIAN_POINT('Ctrl Pts',(-23.7689259151869,-1.57117635434412,
0.));
#200357=CARTESIAN_POINT('Ctrl Pts',(-23.788719841588,-1.56584503586844,
0.));
#200358=CARTESIAN_POINT('Ctrl Pts',(-23.8086019739192,-1.56043321228631,
0.));
#200359=CARTESIAN_POINT('Ctrl Pts',(-23.8285714027631,-1.55494069502628,
0.));
#200360=CARTESIAN_POINT('Ctrl Pts',(-23.8486272290698,-1.5493672994053,
0.));
#200361=CARTESIAN_POINT('Ctrl Pts',(-23.8687685639635,-1.54371284453978,
0.));
#200362=CARTESIAN_POINT('Ctrl Pts',(-23.8889945285313,-1.53797715326748,
0.));
#200363=CARTESIAN_POINT('Ctrl Pts',(-23.9093042536119,-1.53216005207462,
0.));
#200364=CARTESIAN_POINT('Ctrl Pts',(-23.9296968795761,-1.52626137103039,
0.));
#200365=CARTESIAN_POINT('Ctrl Pts',(-23.9501715561038,-1.52028094372806,
0.));
#200366=CARTESIAN_POINT('Ctrl Pts',(-23.9707274420145,-1.51421860720628,
0.));
#200367=CARTESIAN_POINT('Ctrl Pts',(-23.991363705093,-1.50807420187702,
0.));
#200368=CARTESIAN_POINT('Ctrl Pts',(-24.0120795219086,-1.50184757146099,
0.));
#200369=CARTESIAN_POINT('Ctrl Pts',(-24.0328740776331,-1.49553856292798,
0.));
#200370=CARTESIAN_POINT('Ctrl Pts',(-24.053746565843,-1.48914702644883,
0.));
#200371=CARTESIAN_POINT('Ctrl Pts',(-24.074696188353,-1.4826728153368,0.));
#200372=CARTESIAN_POINT('Ctrl Pts',(-24.0957221550782,-1.47611578597741,
0.));
#200373=CARTESIAN_POINT('Ctrl Pts',(-24.1168236838827,-1.46947579776992,
0.));
#200374=CARTESIAN_POINT('Ctrl Pts',(-24.1380000004272,-1.46275271307398,
0.));
#200375=CARTESIAN_POINT('Ctrl Pts',(-24.1592503380105,-1.45594639716314,
0.));
#200376=CARTESIAN_POINT('Ctrl Pts',(-24.1805739374033,-1.44905671818721,
0.));
#200377=CARTESIAN_POINT('Ctrl Pts',(-24.2019700467214,-1.44208354711074,
0.));
#200378=CARTESIAN_POINT('Ctrl Pts',(-24.2234379212978,-1.43502675765502,
0.));
#200379=CARTESIAN_POINT('Ctrl Pts',(-24.2449768235485,-1.42788622624851,
0.));
#200380=CARTESIAN_POINT('Ctrl Pts',(-24.2665860228357,-1.42066183198252,
0.));
#200381=CARTESIAN_POINT('Ctrl Pts',(-24.2882647953214,-1.41335345657685,
0.));
#200382=CARTESIAN_POINT('Ctrl Pts',(-24.3100124238316,-1.4059609843434,
0.));
#200383=CARTESIAN_POINT('Ctrl Pts',(-24.3318281977647,-1.3984843021281,
0.));
#200384=CARTESIAN_POINT('Ctrl Pts',(-24.3537114129877,-1.3909232992639,
0.));
#200385=CARTESIAN_POINT('Ctrl Pts',(-24.37566137173,-1.38327786752998,0.));
#200386=CARTESIAN_POINT('Ctrl Pts',(-24.3976773824731,-1.37554790111607,
0.));
#200387=CARTESIAN_POINT('Ctrl Pts',(-24.4197587598337,-1.36773329659954,
0.));
#200388=CARTESIAN_POINT('Ctrl Pts',(-24.4419048244524,-1.35983395290624,
0.));
#200389=CARTESIAN_POINT('Ctrl Pts',(-24.4641149028894,-1.35184977125644,
0.));
#200390=CARTESIAN_POINT('Ctrl Pts',(-24.4863883275135,-1.34378065512335,
0.));
#200391=CARTESIAN_POINT('Ctrl Pts',(-24.5087244363856,-1.33562651019684,
0.));
#200392=CARTESIAN_POINT('Ctrl Pts',(-24.5311225731434,-1.32738724435326,
0.));
#200393=CARTESIAN_POINT('Ctrl Pts',(-24.5535820868671,-1.31906276763669,
0.));
#200394=CARTESIAN_POINT('Ctrl Pts',(-24.576102332018,-1.31065299222023,
0.));
#200395=CARTESIAN_POINT('Ctrl Pts',(-24.5986826684025,-1.30215783236364,
0.));
#200396=CARTESIAN_POINT('Ctrl Pts',(-24.6213224611228,-1.29357720438107,
0.));
#200397=CARTESIAN_POINT('Ctrl Pts',(-24.6440210805278,-1.28491102661513,
0.));
#200398=CARTESIAN_POINT('Ctrl Pts',(-24.666777902156,-1.2761592194164,0.));
#200399=CARTESIAN_POINT('Ctrl Pts',(-24.6895923066837,-1.26732170513497,
0.));
#200400=CARTESIAN_POINT('Ctrl Pts',(-24.7124636797895,-1.25839840807415,
0.));
#200401=CARTESIAN_POINT('Ctrl Pts',(-24.7353914120012,-1.24938925444323,
0.));
#200402=CARTESIAN_POINT('Ctrl Pts',(-24.7583748985439,-1.24029417231988,
0.));
#200403=CARTESIAN_POINT('Ctrl Pts',(-24.78141353918,-1.23111309161843,0.));
#200404=CARTESIAN_POINT('Ctrl Pts',(-24.8045067380536,-1.22184594406526,
0.));
#200405=CARTESIAN_POINT('Ctrl Pts',(-24.8276539035092,-1.21249266318205,
0.));
#200406=CARTESIAN_POINT('Ctrl Pts',(-24.8508544481973,-1.20305318426015,
0.));
#200407=CARTESIAN_POINT('Ctrl Pts',(-24.8741077892074,-1.19352744434059,
0.));
#200408=CARTESIAN_POINT('Ctrl Pts',(-24.8974133481829,-1.18391538220098,
0.));
#200409=CARTESIAN_POINT('Ctrl Pts',(-24.9207705514449,-1.17421693835039,
0.));
#200410=CARTESIAN_POINT('Ctrl Pts',(-24.9441788300932,-1.16443205502852,
0.));
#200411=CARTESIAN_POINT('Ctrl Pts',(-24.9676376201501,-1.15456067621894,
0.));
#200412=CARTESIAN_POINT('Ctrl Pts',(-24.9911463621431,-1.14460274758206,
0.));
#200413=CARTESIAN_POINT('Ctrl Pts',(-25.0147045006193,-1.13455821638535,
0.));
#200414=CARTESIAN_POINT('Ctrl Pts',(-25.0383114836898,-1.12442703144455,
0.));
#200415=CARTESIAN_POINT('Ctrl Pts',(-25.0619667625336,-1.1142091430689,
0.));
#200416=CARTESIAN_POINT('Ctrl Pts',(-25.085669790968,-1.1039045030174,0.));
#200417=CARTESIAN_POINT('Ctrl Pts',(-25.1094200248448,-1.09351306445299,
0.));
#200418=CARTESIAN_POINT('Ctrl Pts',(-25.1332169227415,-1.08303478197174,
0.));
#200419=CARTESIAN_POINT('Ctrl Pts',(-25.1570599469311,-1.0724696116546,
0.));
#200420=CARTESIAN_POINT('Ctrl Pts',(-25.1809485642191,-1.06181751111754,
0.));
#200421=CARTESIAN_POINT('Ctrl Pts',(-25.2048822469027,-1.05107843957925,
0.));
#200422=CARTESIAN_POINT('Ctrl Pts',(-25.2288604735087,-1.04025235791515,
0.));
#200423=CARTESIAN_POINT('Ctrl Pts',(-25.2528827300427,-1.0293392287683,
0.));
#200424=CARTESIAN_POINT('Ctrl Pts',(-25.2769485087268,-1.01833901642272,
0.));
#200425=CARTESIAN_POINT('Ctrl Pts',(-25.3010573055557,-1.00725168656933,
0.));
#200426=CARTESIAN_POINT('Ctrl Pts',(-25.3252086182976,-0.996077206120919,
0.));
#200427=CARTESIAN_POINT('Ctrl Pts',(-25.3494019441444,-0.984815543004089,
0.));
#200428=CARTESIAN_POINT('Ctrl Pts',(-25.3736367778842,-0.973466666000048,
0.));
#200429=CARTESIAN_POINT('Ctrl Pts',(-25.3979126089155,-0.962030544502802,
0.));
#200430=CARTESIAN_POINT('Ctrl Pts',(-25.4222289223155,-0.950507148596968,
0.));
#200431=CARTESIAN_POINT('Ctrl Pts',(-25.4465852044835,-0.938896449495632,
0.));
#200432=CARTESIAN_POINT('Ctrl Pts',(-25.4709809474996,-0.927198419885604,
0.));
#200433=CARTESIAN_POINT('Ctrl Pts',(-25.4954156541787,-0.915413034335333,
0.));
#200434=CARTESIAN_POINT('Ctrl Pts',(-25.5198888424195,-0.903540269651154,
0.));
#200435=CARTESIAN_POINT('Ctrl Pts',(-25.5444000508223,-0.891580105349467,
0.));
#200436=CARTESIAN_POINT('Ctrl Pts',(-25.568948840818,-0.87953252383509,
0.));
#200437=CARTESIAN_POINT('Ctrl Pts',(-25.5935347843616,-0.86739750933947,
0.));
#200438=CARTESIAN_POINT('Ctrl Pts',(-25.618157453608,-0.855175047037614,
0.));
#200439=CARTESIAN_POINT('Ctrl Pts',(-25.6428164100078,-0.842865122121544,
0.));
#200440=CARTESIAN_POINT('Ctrl Pts',(-25.6675111931957,-0.830467718864367,
0.));
#200441=CARTESIAN_POINT('Ctrl Pts',(-25.6922413110172,-0.817982819786719,
0.));
#200442=CARTESIAN_POINT('Ctrl Pts',(-25.7170062262474,-0.805410404552594,
0.));
#200443=CARTESIAN_POINT('Ctrl Pts',(-25.7418053757671,-0.792750451613534,
0.));
#200444=CARTESIAN_POINT('Ctrl Pts',(-25.7666381946871,-0.780002940289025,
0.));
#200445=CARTESIAN_POINT('Ctrl Pts',(-25.7915041383304,-0.767167852648639,
0.));
#200446=CARTESIAN_POINT('Ctrl Pts',(-25.816402705995,-0.754245175608288,
0.));
#200447=CARTESIAN_POINT('Ctrl Pts',(-25.841333461908,-0.741234902664697,
0.));
#200448=CARTESIAN_POINT('Ctrl Pts',(-25.8662960624285,-0.728137036485877,
0.));
#200449=CARTESIAN_POINT('Ctrl Pts',(-25.8912902615141,-0.714951588533753,
0.));
#200450=CARTESIAN_POINT('Ctrl Pts',(-25.9163158909645,-0.701678575236602,
0.));
#200451=CARTESIAN_POINT('Ctrl Pts',(-25.941372847213,-0.688318015065678,
0.));
#200452=CARTESIAN_POINT('Ctrl Pts',(-25.9614434298092,-0.677559543215902,
0.));
#200453=CARTESIAN_POINT('Ctrl Pts',(-25.9765104298171,-0.669451306784415,
0.));
#200454=CARTESIAN_POINT('Ctrl Pts',(-25.9865613464809,-0.664028313188912,
0.));
#200455=CARTESIAN_POINT('Ctrl Pts',(-25.991588367311,-0.661312440730891,
0.));
#200456=CARTESIAN_POINT('',(-25.991588367311,-0.661312440730891,0.));
#200457=CARTESIAN_POINT('Origin',(-21.1389261070099,3.92374859571501,0.));
#200458=CARTESIAN_POINT('',(-22.1738711152697,4.11585220600461,0.));
#200459=CARTESIAN_POINT('',(-22.1738711152697,4.11585220600461,0.));
#200460=CARTESIAN_POINT('',(-10.5694630535049,1.96187429785751,0.));
#200461=CARTESIAN_POINT('Ctrl Pts',(-25.991588367311,0.661312440730901,
0.));
#200462=CARTESIAN_POINT('Ctrl Pts',(-25.991588367311,0.661312440730901,
12.));
#200463=CARTESIAN_POINT('Ctrl Pts',(-25.9865613464773,0.664028313187627,
0.));
#200464=CARTESIAN_POINT('Ctrl Pts',(-25.9865613464773,0.664028313187627,
12.));
#200465=CARTESIAN_POINT('Ctrl Pts',(-25.9765104298071,0.669451306780825,
0.));
#200466=CARTESIAN_POINT('Ctrl Pts',(-25.9765104298071,0.669451306780825,
12.));
#200467=CARTESIAN_POINT('Ctrl Pts',(-25.9614434297919,0.677559543209725,
0.));
#200468=CARTESIAN_POINT('Ctrl Pts',(-25.9614434297919,0.677559543209725,
12.));
#200469=CARTESIAN_POINT('Ctrl Pts',(-25.9413728471909,0.688318015057729,
0.));
#200470=CARTESIAN_POINT('Ctrl Pts',(-25.9413728471909,0.688318015057729,
12.));
#200471=CARTESIAN_POINT('Ctrl Pts',(-25.9163158909426,0.701678575228756,
0.));
#200472=CARTESIAN_POINT('Ctrl Pts',(-25.9163158909426,0.701678575228756,
12.));
#200473=CARTESIAN_POINT('Ctrl Pts',(-25.891290261497,0.714951588527638,
0.));
#200474=CARTESIAN_POINT('Ctrl Pts',(-25.891290261497,0.714951588527638,
12.));
#200475=CARTESIAN_POINT('Ctrl Pts',(-25.8662960624185,0.728137036482335,
0.));
#200476=CARTESIAN_POINT('Ctrl Pts',(-25.8662960624185,0.728137036482335,
12.));
#200477=CARTESIAN_POINT('Ctrl Pts',(-25.8413334619055,0.741234902663807,
0.));
#200478=CARTESIAN_POINT('Ctrl Pts',(-25.8413334619055,0.741234902663807,
12.));
#200479=CARTESIAN_POINT('Ctrl Pts',(-25.8164027059984,0.754245175609524,
0.));
#200480=CARTESIAN_POINT('Ctrl Pts',(-25.8164027059984,0.754245175609524,
12.));
#200481=CARTESIAN_POINT('Ctrl Pts',(-25.7915041383376,0.767167852651168,
0.));
#200482=CARTESIAN_POINT('Ctrl Pts',(-25.7915041383376,0.767167852651168,
12.));
#200483=CARTESIAN_POINT('Ctrl Pts',(-25.7666381946955,0.780002940291965,
0.));
#200484=CARTESIAN_POINT('Ctrl Pts',(-25.7666381946955,0.780002940291965,
12.));
#200485=CARTESIAN_POINT('Ctrl Pts',(-25.7418053757746,0.792750451616127,
0.));
#200486=CARTESIAN_POINT('Ctrl Pts',(-25.7418053757746,0.792750451616127,
12.));
#200487=CARTESIAN_POINT('Ctrl Pts',(-25.7170062262525,0.805410404554352,
0.));
#200488=CARTESIAN_POINT('Ctrl Pts',(-25.7170062262525,0.805410404554352,
12.));
#200489=CARTESIAN_POINT('Ctrl Pts',(-25.6922413110194,0.817982819787464,
0.));
#200490=CARTESIAN_POINT('Ctrl Pts',(-25.6922413110194,0.817982819787464,
12.));
#200491=CARTESIAN_POINT('Ctrl Pts',(-25.6675111931952,0.830467718864205,
0.));
#200492=CARTESIAN_POINT('Ctrl Pts',(-25.6675111931952,0.830467718864205,
12.));
#200493=CARTESIAN_POINT('Ctrl Pts',(-25.6428164100055,0.842865122120758,
0.));
#200494=CARTESIAN_POINT('Ctrl Pts',(-25.6428164100055,0.842865122120758,
12.));
#200495=CARTESIAN_POINT('Ctrl Pts',(-25.6181574536049,0.855175047036549,
0.));
#200496=CARTESIAN_POINT('Ctrl Pts',(-25.6181574536049,0.855175047036549,
12.));
#200497=CARTESIAN_POINT('Ctrl Pts',(-25.5935347843585,0.867397509338431,
0.));
#200498=CARTESIAN_POINT('Ctrl Pts',(-25.5935347843585,0.867397509338431,
12.));
#200499=CARTESIAN_POINT('Ctrl Pts',(-25.5689488408156,0.879532523834294,
0.));
#200500=CARTESIAN_POINT('Ctrl Pts',(-25.5689488408156,0.879532523834294,
12.));
#200501=CARTESIAN_POINT('Ctrl Pts',(-25.5444000508211,0.89158010534904,
0.));
#200502=CARTESIAN_POINT('Ctrl Pts',(-25.5444000508211,0.89158010534904,
12.));
#200503=CARTESIAN_POINT('Ctrl Pts',(-25.5198888424194,0.903540269651106,
0.));
#200504=CARTESIAN_POINT('Ctrl Pts',(-25.5198888424194,0.903540269651106,
12.));
#200505=CARTESIAN_POINT('Ctrl Pts',(-25.4954156541795,0.915413034335613,
0.));
#200506=CARTESIAN_POINT('Ctrl Pts',(-25.4954156541795,0.915413034335613,
12.));
#200507=CARTESIAN_POINT('Ctrl Pts',(-25.4709809475009,0.927198419886094,
0.));
#200508=CARTESIAN_POINT('Ctrl Pts',(-25.4709809475009,0.927198419886094,
12.));
#200509=CARTESIAN_POINT('Ctrl Pts',(-25.4465852044849,0.938896449496192,
0.));
#200510=CARTESIAN_POINT('Ctrl Pts',(-25.4465852044849,0.938896449496192,
12.));
#200511=CARTESIAN_POINT('Ctrl Pts',(-25.4222289223167,0.950507148597468,
0.));
#200512=CARTESIAN_POINT('Ctrl Pts',(-25.4222289223167,0.950507148597468,
12.));
#200513=CARTESIAN_POINT('Ctrl Pts',(-25.3979126089163,0.962030544503142,
0.));
#200514=CARTESIAN_POINT('Ctrl Pts',(-25.3979126089163,0.962030544503142,
12.));
#200515=CARTESIAN_POINT('Ctrl Pts',(-25.3736367778845,0.973466666000163,
0.));
#200516=CARTESIAN_POINT('Ctrl Pts',(-25.3736367778845,0.973466666000163,
12.));
#200517=CARTESIAN_POINT('Ctrl Pts',(-25.3494019441441,0.984815543003973,
0.));
#200518=CARTESIAN_POINT('Ctrl Pts',(-25.3494019441441,0.984815543003973,
12.));
#200519=CARTESIAN_POINT('Ctrl Pts',(-25.3252086182968,0.996077206120624,
0.));
#200520=CARTESIAN_POINT('Ctrl Pts',(-25.3252086182968,0.996077206120624,
12.));
#200521=CARTESIAN_POINT('Ctrl Pts',(-25.3010573055547,1.00725168656896,
0.));
#200522=CARTESIAN_POINT('Ctrl Pts',(-25.3010573055547,1.00725168656896,
12.));
#200523=CARTESIAN_POINT('Ctrl Pts',(-25.276948508726,1.01833901642237,0.));
#200524=CARTESIAN_POINT('Ctrl Pts',(-25.276948508726,1.01833901642237,12.));
#200525=CARTESIAN_POINT('Ctrl Pts',(-25.2528827300422,1.02933922876806,
0.));
#200526=CARTESIAN_POINT('Ctrl Pts',(-25.2528827300422,1.02933922876806,
12.));
#200527=CARTESIAN_POINT('Ctrl Pts',(-25.2288604735086,1.04025235791507,
0.));
#200528=CARTESIAN_POINT('Ctrl Pts',(-25.2288604735086,1.04025235791507,
12.));
#200529=CARTESIAN_POINT('Ctrl Pts',(-25.2048822469028,1.05107843957931,
0.));
#200530=CARTESIAN_POINT('Ctrl Pts',(-25.2048822469028,1.05107843957931,
12.));
#200531=CARTESIAN_POINT('Ctrl Pts',(-25.1809485642192,1.06181751111768,
0.));
#200532=CARTESIAN_POINT('Ctrl Pts',(-25.1809485642192,1.06181751111768,
12.));
#200533=CARTESIAN_POINT('Ctrl Pts',(-25.157059946931,1.07246961165475,0.));
#200534=CARTESIAN_POINT('Ctrl Pts',(-25.157059946931,1.07246961165475,12.));
#200535=CARTESIAN_POINT('Ctrl Pts',(-25.1332169227413,1.08303478197187,
0.));
#200536=CARTESIAN_POINT('Ctrl Pts',(-25.1332169227413,1.08303478197187,
12.));
#200537=CARTESIAN_POINT('Ctrl Pts',(-25.1094200248446,1.09351306445308,
0.));
#200538=CARTESIAN_POINT('Ctrl Pts',(-25.1094200248446,1.09351306445308,
12.));
#200539=CARTESIAN_POINT('Ctrl Pts',(-25.0856697909679,1.10390450301745,
0.));
#200540=CARTESIAN_POINT('Ctrl Pts',(-25.0856697909679,1.10390450301745,
12.));
#200541=CARTESIAN_POINT('Ctrl Pts',(-25.0619667625336,1.11420914306889,
0.));
#200542=CARTESIAN_POINT('Ctrl Pts',(-25.0619667625336,1.11420914306889,
12.));
#200543=CARTESIAN_POINT('Ctrl Pts',(-25.0383114836899,1.12442703144451,
0.));
#200544=CARTESIAN_POINT('Ctrl Pts',(-25.0383114836899,1.12442703144451,
12.));
#200545=CARTESIAN_POINT('Ctrl Pts',(-25.0147045006196,1.1345582163853,0.));
#200546=CARTESIAN_POINT('Ctrl Pts',(-25.0147045006196,1.1345582163853,12.));
#200547=CARTESIAN_POINT('Ctrl Pts',(-24.9911463621433,1.144602747582,0.));
#200548=CARTESIAN_POINT('Ctrl Pts',(-24.9911463621433,1.144602747582,12.));
#200549=CARTESIAN_POINT('Ctrl Pts',(-24.9676376201502,1.15456067621889,
0.));
#200550=CARTESIAN_POINT('Ctrl Pts',(-24.9676376201502,1.15456067621889,
12.));
#200551=CARTESIAN_POINT('Ctrl Pts',(-24.9441788300932,1.16443205502849,
0.));
#200552=CARTESIAN_POINT('Ctrl Pts',(-24.9441788300932,1.16443205502849,
12.));
#200553=CARTESIAN_POINT('Ctrl Pts',(-24.9207705514449,1.17421693835041,
0.));
#200554=CARTESIAN_POINT('Ctrl Pts',(-24.9207705514449,1.17421693835041,
12.));
#200555=CARTESIAN_POINT('Ctrl Pts',(-24.8974133481829,1.18391538220103,
0.));
#200556=CARTESIAN_POINT('Ctrl Pts',(-24.8974133481829,1.18391538220103,
12.));
#200557=CARTESIAN_POINT('Ctrl Pts',(-24.8741077892075,1.19352744434064,
0.));
#200558=CARTESIAN_POINT('Ctrl Pts',(-24.8741077892075,1.19352744434064,
12.));
#200559=CARTESIAN_POINT('Ctrl Pts',(-24.8508544481974,1.2030531842602,0.));
#200560=CARTESIAN_POINT('Ctrl Pts',(-24.8508544481974,1.2030531842602,12.));
#200561=CARTESIAN_POINT('Ctrl Pts',(-24.8276539035092,1.21249266318208,
0.));
#200562=CARTESIAN_POINT('Ctrl Pts',(-24.8276539035092,1.21249266318208,
12.));
#200563=CARTESIAN_POINT('Ctrl Pts',(-24.8045067380536,1.22184594406528,
0.));
#200564=CARTESIAN_POINT('Ctrl Pts',(-24.8045067380536,1.22184594406528,
12.));
#200565=CARTESIAN_POINT('Ctrl Pts',(-24.7814135391799,1.23111309161843,
0.));
#200566=CARTESIAN_POINT('Ctrl Pts',(-24.7814135391799,1.23111309161843,
12.));
#200567=CARTESIAN_POINT('Ctrl Pts',(-24.7583748985438,1.24029417231989,
0.));
#200568=CARTESIAN_POINT('Ctrl Pts',(-24.7583748985438,1.24029417231989,
12.));
#200569=CARTESIAN_POINT('Ctrl Pts',(-24.7353914120011,1.24938925444325,
0.));
#200570=CARTESIAN_POINT('Ctrl Pts',(-24.7353914120011,1.24938925444325,
12.));
#200571=CARTESIAN_POINT('Ctrl Pts',(-24.7124636797894,1.25839840807418,
0.));
#200572=CARTESIAN_POINT('Ctrl Pts',(-24.7124636797894,1.25839840807418,
12.));
#200573=CARTESIAN_POINT('Ctrl Pts',(-24.6895923066836,1.267321705135,0.));
#200574=CARTESIAN_POINT('Ctrl Pts',(-24.6895923066836,1.267321705135,12.));
#200575=CARTESIAN_POINT('Ctrl Pts',(-24.666777902156,1.27615921941642,0.));
#200576=CARTESIAN_POINT('Ctrl Pts',(-24.666777902156,1.27615921941642,12.));
#200577=CARTESIAN_POINT('Ctrl Pts',(-24.6440210805278,1.28491102661514,
0.));
#200578=CARTESIAN_POINT('Ctrl Pts',(-24.6440210805278,1.28491102661514,
12.));
#200579=CARTESIAN_POINT('Ctrl Pts',(-24.6213224611229,1.29357720438107,
0.));
#200580=CARTESIAN_POINT('Ctrl Pts',(-24.6213224611229,1.29357720438107,
12.));
#200581=CARTESIAN_POINT('Ctrl Pts',(-24.5986826684027,1.30215783236362,
0.));
#200582=CARTESIAN_POINT('Ctrl Pts',(-24.5986826684027,1.30215783236362,
12.));
#200583=CARTESIAN_POINT('Ctrl Pts',(-24.5761023320183,1.31065299222021,
0.));
#200584=CARTESIAN_POINT('Ctrl Pts',(-24.5761023320183,1.31065299222021,
12.));
#200585=CARTESIAN_POINT('Ctrl Pts',(-24.5535820868674,1.31906276763668,
0.));
#200586=CARTESIAN_POINT('Ctrl Pts',(-24.5535820868674,1.31906276763668,
12.));
#200587=CARTESIAN_POINT('Ctrl Pts',(-24.5311225731435,1.32738724435326,
0.));
#200588=CARTESIAN_POINT('Ctrl Pts',(-24.5311225731435,1.32738724435326,
12.));
#200589=CARTESIAN_POINT('Ctrl Pts',(-24.5087244363856,1.33562651019686,
0.));
#200590=CARTESIAN_POINT('Ctrl Pts',(-24.5087244363856,1.33562651019686,
12.));
#200591=CARTESIAN_POINT('Ctrl Pts',(-24.4863883275134,1.34378065512337,
0.));
#200592=CARTESIAN_POINT('Ctrl Pts',(-24.4863883275134,1.34378065512337,
12.));
#200593=CARTESIAN_POINT('Ctrl Pts',(-24.4641149028892,1.35184977125648,
0.));
#200594=CARTESIAN_POINT('Ctrl Pts',(-24.4641149028892,1.35184977125648,
12.));
#200595=CARTESIAN_POINT('Ctrl Pts',(-24.4419048244523,1.35983395290627,
0.));
#200596=CARTESIAN_POINT('Ctrl Pts',(-24.4419048244523,1.35983395290627,
12.));
#200597=CARTESIAN_POINT('Ctrl Pts',(-24.4197587598337,1.36773329659956,
0.));
#200598=CARTESIAN_POINT('Ctrl Pts',(-24.4197587598337,1.36773329659956,
12.));
#200599=CARTESIAN_POINT('Ctrl Pts',(-24.3976773824732,1.37554790111609,
0.));
#200600=CARTESIAN_POINT('Ctrl Pts',(-24.3976773824732,1.37554790111609,
12.));
#200601=CARTESIAN_POINT('Ctrl Pts',(-24.3756613717299,1.38327786752998,
0.));
#200602=CARTESIAN_POINT('Ctrl Pts',(-24.3756613717299,1.38327786752998,
12.));
#200603=CARTESIAN_POINT('Ctrl Pts',(-24.3537114129875,1.39092329926388,
0.));
#200604=CARTESIAN_POINT('Ctrl Pts',(-24.3537114129875,1.39092329926388,
12.));
#200605=CARTESIAN_POINT('Ctrl Pts',(-24.3318281977643,1.39848430212807,
0.));
#200606=CARTESIAN_POINT('Ctrl Pts',(-24.3318281977643,1.39848430212807,
12.));
#200607=CARTESIAN_POINT('Ctrl Pts',(-24.3100124238311,1.40596098434337,
0.));
#200608=CARTESIAN_POINT('Ctrl Pts',(-24.3100124238311,1.40596098434337,
12.));
#200609=CARTESIAN_POINT('Ctrl Pts',(-24.288264795321,1.41335345657682,0.));
#200610=CARTESIAN_POINT('Ctrl Pts',(-24.288264795321,1.41335345657682,12.));
#200611=CARTESIAN_POINT('Ctrl Pts',(-24.2665860228356,1.42066183198252,
0.));
#200612=CARTESIAN_POINT('Ctrl Pts',(-24.2665860228356,1.42066183198252,
12.));
#200613=CARTESIAN_POINT('Ctrl Pts',(-24.2449768235488,1.42788622624854,
0.));
#200614=CARTESIAN_POINT('Ctrl Pts',(-24.2449768235488,1.42788622624854,
12.));
#200615=CARTESIAN_POINT('Ctrl Pts',(-24.2234379212984,1.43502675765508,
0.));
#200616=CARTESIAN_POINT('Ctrl Pts',(-24.2234379212984,1.43502675765508,
12.));
#200617=CARTESIAN_POINT('Ctrl Pts',(-24.201970046722,1.44208354711082,0.));
#200618=CARTESIAN_POINT('Ctrl Pts',(-24.201970046722,1.44208354711082,12.));
#200619=CARTESIAN_POINT('Ctrl Pts',(-24.1805739374038,1.44905671818727,
0.));
#200620=CARTESIAN_POINT('Ctrl Pts',(-24.1805739374038,1.44905671818727,
12.));
#200621=CARTESIAN_POINT('Ctrl Pts',(-24.1592503380107,1.45594639716317,
0.));
#200622=CARTESIAN_POINT('Ctrl Pts',(-24.1592503380107,1.45594639716317,
12.));
#200623=CARTESIAN_POINT('Ctrl Pts',(-24.1380000004272,1.46275271307397,
0.));
#200624=CARTESIAN_POINT('Ctrl Pts',(-24.1380000004272,1.46275271307397,
12.));
#200625=CARTESIAN_POINT('Ctrl Pts',(-24.1168236838824,1.46947579776991,
0.));
#200626=CARTESIAN_POINT('Ctrl Pts',(-24.1168236838824,1.46947579776991,
12.));
#200627=CARTESIAN_POINT('Ctrl Pts',(-24.0957221550778,1.47611578597742,
0.));
#200628=CARTESIAN_POINT('Ctrl Pts',(-24.0957221550778,1.47611578597742,
12.));
#200629=CARTESIAN_POINT('Ctrl Pts',(-24.0746961883528,1.48267281533683,
0.));
#200630=CARTESIAN_POINT('Ctrl Pts',(-24.0746961883528,1.48267281533683,
12.));
#200631=CARTESIAN_POINT('Ctrl Pts',(-24.0537465658429,1.48914702644887,
0.));
#200632=CARTESIAN_POINT('Ctrl Pts',(-24.0537465658429,1.48914702644887,
12.));
#200633=CARTESIAN_POINT('Ctrl Pts',(-24.0328740776331,1.49553856292801,
0.));
#200634=CARTESIAN_POINT('Ctrl Pts',(-24.0328740776331,1.49553856292801,
12.));
#200635=CARTESIAN_POINT('Ctrl Pts',(-24.0120795219086,1.50184757146098,
0.));
#200636=CARTESIAN_POINT('Ctrl Pts',(-24.0120795219086,1.50184757146098,
12.));
#200637=CARTESIAN_POINT('Ctrl Pts',(-23.9913637050927,1.50807420187694,
0.));
#200638=CARTESIAN_POINT('Ctrl Pts',(-23.9913637050927,1.50807420187694,
12.));
#200639=CARTESIAN_POINT('Ctrl Pts',(-23.970727442014,1.51421860720614,0.));
#200640=CARTESIAN_POINT('Ctrl Pts',(-23.970727442014,1.51421860720614,12.));
#200641=CARTESIAN_POINT('Ctrl Pts',(-23.9501715561033,1.52028094372792,
0.));
#200642=CARTESIAN_POINT('Ctrl Pts',(-23.9501715561033,1.52028094372792,
12.));
#200643=CARTESIAN_POINT('Ctrl Pts',(-23.9296968795757,1.52626137103032,
0.));
#200644=CARTESIAN_POINT('Ctrl Pts',(-23.9296968795757,1.52626137103032,
12.));
#200645=CARTESIAN_POINT('Ctrl Pts',(-23.9093042536119,1.53216005207463,
0.));
#200646=CARTESIAN_POINT('Ctrl Pts',(-23.9093042536119,1.53216005207463,
12.));
#200647=CARTESIAN_POINT('Ctrl Pts',(-23.8889945285318,1.53797715326758,
0.));
#200648=CARTESIAN_POINT('Ctrl Pts',(-23.8889945285318,1.53797715326758,
12.));
#200649=CARTESIAN_POINT('Ctrl Pts',(-23.8687685639642,1.5437128445399,0.));
#200650=CARTESIAN_POINT('Ctrl Pts',(-23.8687685639642,1.5437128445399,12.));
#200651=CARTESIAN_POINT('Ctrl Pts',(-23.8486272290705,1.54936729940541,
0.));
#200652=CARTESIAN_POINT('Ctrl Pts',(-23.8486272290705,1.54936729940541,
12.));
#200653=CARTESIAN_POINT('Ctrl Pts',(-23.8285714027636,1.55494069502635,
0.));
#200654=CARTESIAN_POINT('Ctrl Pts',(-23.8285714027636,1.55494069502635,
12.));
#200655=CARTESIAN_POINT('Ctrl Pts',(-23.8086019739194,1.56043321228633,
0.));
#200656=CARTESIAN_POINT('Ctrl Pts',(-23.8086019739194,1.56043321228633,
12.));
#200657=CARTESIAN_POINT('Ctrl Pts',(-23.7887198415878,1.56584503586843,
0.));
#200658=CARTESIAN_POINT('Ctrl Pts',(-23.7887198415878,1.56584503586843,
12.));
#200659=CARTESIAN_POINT('Ctrl Pts',(-23.7689259151862,1.57117635434408,
0.));
#200660=CARTESIAN_POINT('Ctrl Pts',(-23.7689259151862,1.57117635434408,
12.));
#200661=CARTESIAN_POINT('Ctrl Pts',(-23.749221114736,1.57642736025246,0.));
#200662=CARTESIAN_POINT('Ctrl Pts',(-23.749221114736,1.57642736025246,12.));
#200663=CARTESIAN_POINT('Ctrl Pts',(-23.72960637113,1.58159825017358,0.));
#200664=CARTESIAN_POINT('Ctrl Pts',(-23.72960637113,1.58159825017358,12.));
#200665=CARTESIAN_POINT('Ctrl Pts',(-23.710082626383,1.58668922481221,0.));
#200666=CARTESIAN_POINT('Ctrl Pts',(-23.710082626383,1.58668922481221,12.));
#200667=CARTESIAN_POINT('Ctrl Pts',(-23.6906508338833,1.59170048908633,
0.));
#200668=CARTESIAN_POINT('Ctrl Pts',(-23.6906508338833,1.59170048908633,
12.));
#200669=CARTESIAN_POINT('Ctrl Pts',(-23.671311958631,1.59663225222463,0.));
#200670=CARTESIAN_POINT('Ctrl Pts',(-23.671311958631,1.59663225222463,12.));
#200671=CARTESIAN_POINT('Ctrl Pts',(-23.6520669774876,1.60148472786595,
0.));
#200672=CARTESIAN_POINT('Ctrl Pts',(-23.6520669774876,1.60148472786595,
12.));
#200673=CARTESIAN_POINT('Ctrl Pts',(-23.6329168794929,1.60625813414672,
0.));
#200674=CARTESIAN_POINT('Ctrl Pts',(-23.6329168794929,1.60625813414672,
12.));
#200675=CARTESIAN_POINT('Ctrl Pts',(-23.6138626661653,1.61095269379778,
0.));
#200676=CARTESIAN_POINT('Ctrl Pts',(-23.6138626661653,1.61095269379778,
12.));
#200677=CARTESIAN_POINT('Ctrl Pts',(-23.5949053517997,1.61556863424698,
0.));
#200678=CARTESIAN_POINT('Ctrl Pts',(-23.5949053517997,1.61556863424698,
12.));
#200679=CARTESIAN_POINT('Ctrl Pts',(-23.57604596376,1.62010618772866,0.));
#200680=CARTESIAN_POINT('Ctrl Pts',(-23.57604596376,1.62010618772866,12.));
#200681=CARTESIAN_POINT('Ctrl Pts',(-23.5572855427601,1.62456559140064,
0.));
#200682=CARTESIAN_POINT('Ctrl Pts',(-23.5572855427601,1.62456559140064,
12.));
#200683=CARTESIAN_POINT('Ctrl Pts',(-23.538625143226,1.62894708745223,0.));
#200684=CARTESIAN_POINT('Ctrl Pts',(-23.538625143226,1.62894708745223,12.));
#200685=CARTESIAN_POINT('Ctrl Pts',(-23.5200658336612,1.63325092321725,
0.));
#200686=CARTESIAN_POINT('Ctrl Pts',(-23.5200658336612,1.63325092321725,
12.));
#200687=CARTESIAN_POINT('Ctrl Pts',(-23.5016086970003,1.63747735129474,
0.));
#200688=CARTESIAN_POINT('Ctrl Pts',(-23.5016086970003,1.63747735129474,
12.));
#200689=CARTESIAN_POINT('Ctrl Pts',(-23.4832548309645,1.64162662967528,
0.));
#200690=CARTESIAN_POINT('Ctrl Pts',(-23.4832548309645,1.64162662967528,
12.));
#200691=CARTESIAN_POINT('Ctrl Pts',(-23.4650053483932,1.64569902187611,
0.));
#200692=CARTESIAN_POINT('Ctrl Pts',(-23.4650053483932,1.64569902187611,
12.));
#200693=CARTESIAN_POINT('Ctrl Pts',(-23.4468613776574,1.6496947970734,0.));
#200694=CARTESIAN_POINT('Ctrl Pts',(-23.4468613776574,1.6496947970734,12.));
#200695=CARTESIAN_POINT('Ctrl Pts',(-23.4288240631043,1.65361423023728,
0.));
#200696=CARTESIAN_POINT('Ctrl Pts',(-23.4288240631043,1.65361423023728,
12.));
#200697=CARTESIAN_POINT('Ctrl Pts',(-23.4108945654805,1.65745760227505,
0.));
#200698=CARTESIAN_POINT('Ctrl Pts',(-23.4108945654805,1.65745760227505,
12.));
#200699=CARTESIAN_POINT('Ctrl Pts',(-23.3930740623619,1.66122520018011,
0.));
#200700=CARTESIAN_POINT('Ctrl Pts',(-23.3930740623619,1.66122520018011,
12.));
#200701=CARTESIAN_POINT('Ctrl Pts',(-23.3753637485545,1.66491731718876,
0.));
#200702=CARTESIAN_POINT('Ctrl Pts',(-23.3753637485545,1.66491731718876,
12.));
#200703=CARTESIAN_POINT('Ctrl Pts',(-23.3577648365744,1.66853425293995,
0.));
#200704=CARTESIAN_POINT('Ctrl Pts',(-23.3577648365744,1.66853425293995,
12.));
#200705=CARTESIAN_POINT('Ctrl Pts',(-23.3402785571865,1.67207631363921,
0.));
#200706=CARTESIAN_POINT('Ctrl Pts',(-23.3402785571865,1.67207631363921,
12.));
#200707=CARTESIAN_POINT('Ctrl Pts',(-23.3229061599145,1.67554381222994,
0.));
#200708=CARTESIAN_POINT('Ctrl Pts',(-23.3229061599145,1.67554381222994,
12.));
#200709=CARTESIAN_POINT('Ctrl Pts',(-23.3056489135611,1.67893706857117,
0.));
#200710=CARTESIAN_POINT('Ctrl Pts',(-23.3056489135611,1.67893706857117,
12.));
#200711=CARTESIAN_POINT('Ctrl Pts',(-23.2885081066951,1.68225640962168,
0.));
#200712=CARTESIAN_POINT('Ctrl Pts',(-23.2885081066951,1.68225640962168,
12.));
#200713=CARTESIAN_POINT('Ctrl Pts',(-23.2714850482246,1.68550216963258,
0.));
#200714=CARTESIAN_POINT('Ctrl Pts',(-23.2714850482246,1.68550216963258,
12.));
#200715=CARTESIAN_POINT('Ctrl Pts',(-23.2545810680537,1.68867469034896,
0.));
#200716=CARTESIAN_POINT('Ctrl Pts',(-23.2545810680537,1.68867469034896,
12.));
#200717=CARTESIAN_POINT('Ctrl Pts',(-23.2377975177013,1.69177432121711,
0.));
#200718=CARTESIAN_POINT('Ctrl Pts',(-23.2377975177013,1.69177432121711,
12.));
#200719=CARTESIAN_POINT('Ctrl Pts',(-23.2211357709374,1.69480141959953,
0.));
#200720=CARTESIAN_POINT('Ctrl Pts',(-23.2211357709374,1.69480141959953,
12.));
#200721=CARTESIAN_POINT('Ctrl Pts',(-23.2045972243767,1.69775635099443,
0.));
#200722=CARTESIAN_POINT('Ctrl Pts',(-23.2045972243767,1.69775635099443,
12.));
#200723=CARTESIAN_POINT('Ctrl Pts',(-23.1881832981851,1.7006394892701,0.));
#200724=CARTESIAN_POINT('Ctrl Pts',(-23.1881832981851,1.7006394892701,12.));
#200725=CARTESIAN_POINT('Ctrl Pts',(-23.1718954368751,1.70345121691276,
0.));
#200726=CARTESIAN_POINT('Ctrl Pts',(-23.1718954368751,1.70345121691276,
12.));
#200727=CARTESIAN_POINT('Ctrl Pts',(-23.1557351100614,1.70619192527852,
0.));
#200728=CARTESIAN_POINT('Ctrl Pts',(-23.1557351100614,1.70619192527852,
12.));
#200729=CARTESIAN_POINT('Ctrl Pts',(-23.1397038132356,1.70886201485452,
0.));
#200730=CARTESIAN_POINT('Ctrl Pts',(-23.1397038132356,1.70886201485452,
12.));
#200731=CARTESIAN_POINT('Ctrl Pts',(-23.1238030684925,1.71146189552174,
0.));
#200732=CARTESIAN_POINT('Ctrl Pts',(-23.1238030684925,1.71146189552174,
12.));
#200733=CARTESIAN_POINT('Ctrl Pts',(-23.1080344254286,1.71399198684704,
0.));
#200734=CARTESIAN_POINT('Ctrl Pts',(-23.1080344254286,1.71399198684704,
12.));
#200735=CARTESIAN_POINT('Ctrl Pts',(-23.0923994621213,1.71645271839296,
0.));
#200736=CARTESIAN_POINT('Ctrl Pts',(-23.0923994621213,1.71645271839296,
12.));
#200737=CARTESIAN_POINT('Ctrl Pts',(-23.0768997860709,1.71884453003027,
0.));
#200738=CARTESIAN_POINT('Ctrl Pts',(-23.0768997860709,1.71884453003027,
12.));
#200739=CARTESIAN_POINT('Ctrl Pts',(-23.0615370351562,1.72116787225991,
0.));
#200740=CARTESIAN_POINT('Ctrl Pts',(-23.0615370351562,1.72116787225991,
12.));
#200741=CARTESIAN_POINT('Ctrl Pts',(-23.0463128785531,1.72342320653746,
0.));
#200742=CARTESIAN_POINT('Ctrl Pts',(-23.0463128785531,1.72342320653746,
12.));
#200743=CARTESIAN_POINT('Ctrl Pts',(-23.0312290178883,1.72561100564045,
0.));
#200744=CARTESIAN_POINT('Ctrl Pts',(-23.0312290178883,1.72561100564045,
12.));
#200745=CARTESIAN_POINT('Ctrl Pts',(-23.0162871884168,1.72773175404708,
0.));
#200746=CARTESIAN_POINT('Ctrl Pts',(-23.0162871884168,1.72773175404708,
12.));
#200747=CARTESIAN_POINT('Ctrl Pts',(-23.001489160189,1.72978594832136,0.));
#200748=CARTESIAN_POINT('Ctrl Pts',(-23.001489160189,1.72978594832136,12.));
#200749=CARTESIAN_POINT('Ctrl Pts',(-22.9868367391978,1.7317740975019,0.));
#200750=CARTESIAN_POINT('Ctrl Pts',(-22.9868367391978,1.7317740975019,12.));
#200751=CARTESIAN_POINT('Ctrl Pts',(-22.9723317685688,1.73369672350814,
0.));
#200752=CARTESIAN_POINT('Ctrl Pts',(-22.9723317685688,1.73369672350814,
12.));
#200753=CARTESIAN_POINT('Ctrl Pts',(-22.9579761301063,1.73555436162769,
0.));
#200754=CARTESIAN_POINT('Ctrl Pts',(-22.9579761301063,1.73555436162769,
12.));
#200755=CARTESIAN_POINT('Ctrl Pts',(-22.9437717457826,1.73734756100039,
0.));
#200756=CARTESIAN_POINT('Ctrl Pts',(-22.9437717457826,1.73734756100039,
12.));
#200757=CARTESIAN_POINT('Ctrl Pts',(-22.9297205792586,1.73907688511666,
0.));
#200758=CARTESIAN_POINT('Ctrl Pts',(-22.9297205792586,1.73907688511666,
12.));
#200759=CARTESIAN_POINT('Ctrl Pts',(-22.9158246373363,1.74074291231058,
0.));
#200760=CARTESIAN_POINT('Ctrl Pts',(-22.9158246373363,1.74074291231058,
12.));
#200761=CARTESIAN_POINT('Ctrl Pts',(-22.9020859716141,1.7423462363008,0.));
#200762=CARTESIAN_POINT('Ctrl Pts',(-22.9020859716141,1.7423462363008,12.));
#200763=CARTESIAN_POINT('Ctrl Pts',(-22.888506680335,1.74388746677702,0.));
#200764=CARTESIAN_POINT('Ctrl Pts',(-22.888506680335,1.74388746677702,12.));
#200765=CARTESIAN_POINT('Ctrl Pts',(-22.8750889101696,1.74536722998201,
0.));
#200766=CARTESIAN_POINT('Ctrl Pts',(-22.8750889101696,1.74536722998201,
12.));
#200767=CARTESIAN_POINT('Ctrl Pts',(-22.8618348580235,1.74678616930664,
0.));
#200768=CARTESIAN_POINT('Ctrl Pts',(-22.8618348580235,1.74678616930664,
12.));
#200769=CARTESIAN_POINT('Ctrl Pts',(-22.8487467728076,1.74814494588492,
0.));
#200770=CARTESIAN_POINT('Ctrl Pts',(-22.8487467728076,1.74814494588492,
12.));
#200771=CARTESIAN_POINT('Ctrl Pts',(-22.8358269579853,1.74944423940115,
0.));
#200772=CARTESIAN_POINT('Ctrl Pts',(-22.8358269579853,1.74944423940115,
12.));
#200773=CARTESIAN_POINT('Ctrl Pts',(-22.8230777741284,1.75068474890883,
0.));
#200774=CARTESIAN_POINT('Ctrl Pts',(-22.8230777741284,1.75068474890883,
12.));
#200775=CARTESIAN_POINT('Ctrl Pts',(-22.8105016414713,1.75186719365592,
0.));
#200776=CARTESIAN_POINT('Ctrl Pts',(-22.8105016414713,1.75186719365592,
12.));
#200777=CARTESIAN_POINT('Ctrl Pts',(-22.7981010424314,1.75299231391466,
0.));
#200778=CARTESIAN_POINT('Ctrl Pts',(-22.7981010424314,1.75299231391466,
12.));
#200779=CARTESIAN_POINT('Ctrl Pts',(-22.7858785242361,1.75406087182936,
0.));
#200780=CARTESIAN_POINT('Ctrl Pts',(-22.7858785242361,1.75406087182936,
12.));
#200781=CARTESIAN_POINT('Ctrl Pts',(-22.7738367016118,1.75507365227131,
0.));
#200782=CARTESIAN_POINT('Ctrl Pts',(-22.7738367016118,1.75507365227131,
12.));
#200783=CARTESIAN_POINT('Ctrl Pts',(-22.7619782595013,1.75603146371641,
0.));
#200784=CARTESIAN_POINT('Ctrl Pts',(-22.7619782595013,1.75603146371641,
12.));
#200785=CARTESIAN_POINT('Ctrl Pts',(-22.750305955645,1.75693513908907,0.));
#200786=CARTESIAN_POINT('Ctrl Pts',(-22.750305955645,1.75693513908907,12.));
#200787=CARTESIAN_POINT('Ctrl Pts',(-22.7388226235559,1.75778553673244,
0.));
#200788=CARTESIAN_POINT('Ctrl Pts',(-22.7388226235559,1.75778553673244,
12.));
#200789=CARTESIAN_POINT('Ctrl Pts',(-22.72753117773,1.75858354204633,0.));
#200790=CARTESIAN_POINT('Ctrl Pts',(-22.72753117773,1.75858354204633,12.));
#200791=CARTESIAN_POINT('Ctrl Pts',(-22.7164346186006,1.75933006905925,
0.));
#200792=CARTESIAN_POINT('Ctrl Pts',(-22.7164346186006,1.75933006905925,
12.));
#200793=CARTESIAN_POINT('Ctrl Pts',(-22.7055360375485,1.76002606202401,
0.));
#200794=CARTESIAN_POINT('Ctrl Pts',(-22.7055360375485,1.76002606202401,
12.));
#200795=CARTESIAN_POINT('Ctrl Pts',(-22.6948386219851,1.76067249704886,
0.));
#200796=CARTESIAN_POINT('Ctrl Pts',(-22.6948386219851,1.76067249704886,
12.));
#200797=CARTESIAN_POINT('Ctrl Pts',(-22.684345658525,1.76127038310614,0.));
#200798=CARTESIAN_POINT('Ctrl Pts',(-22.684345658525,1.76127038310614,12.));
#200799=CARTESIAN_POINT('Ctrl Pts',(-22.67406053567,1.76182076289525,0.));
#200800=CARTESIAN_POINT('Ctrl Pts',(-22.67406053567,1.76182076289525,12.));
#200801=CARTESIAN_POINT('Ctrl Pts',(-22.6639867471753,1.76232471392568,
0.));
#200802=CARTESIAN_POINT('Ctrl Pts',(-22.6639867471753,1.76232471392568,
12.));
#200803=CARTESIAN_POINT('Ctrl Pts',(-22.6541278938409,1.76278334912561,
0.));
#200804=CARTESIAN_POINT('Ctrl Pts',(-22.6541278938409,1.76278334912561,
12.));
#200805=CARTESIAN_POINT('Ctrl Pts',(-22.6444876940423,1.76319782013916,
0.));
#200806=CARTESIAN_POINT('Ctrl Pts',(-22.6444876940423,1.76319782013916,
12.));
#200807=CARTESIAN_POINT('Ctrl Pts',(-22.6350699979359,1.76356932176273,
0.));
#200808=CARTESIAN_POINT('Ctrl Pts',(-22.6350699979359,1.76356932176273,
12.));
#200809=CARTESIAN_POINT('Ctrl Pts',(-22.6258787994848,1.76389909571403,
0.));
#200810=CARTESIAN_POINT('Ctrl Pts',(-22.6258787994848,1.76389909571403,
12.));
#200811=CARTESIAN_POINT('Ctrl Pts',(-22.6169182517694,1.76418843543739,
0.));
#200812=CARTESIAN_POINT('Ctrl Pts',(-22.6169182517694,1.76418843543739,
12.));
#200813=CARTESIAN_POINT('Ctrl Pts',(-22.6081926681343,1.76443868648015,
0.));
#200814=CARTESIAN_POINT('Ctrl Pts',(-22.6081926681343,1.76443868648015,
12.));
#200815=CARTESIAN_POINT('Ctrl Pts',(-22.5997065145638,1.76465124413557,
0.));
#200816=CARTESIAN_POINT('Ctrl Pts',(-22.5997065145638,1.76465124413557,
12.));
#200817=CARTESIAN_POINT('Ctrl Pts',(-22.5914644078106,1.76482755288411,
0.));
#200818=CARTESIAN_POINT('Ctrl Pts',(-22.5914644078106,1.76482755288411,
12.));
#200819=CARTESIAN_POINT('Ctrl Pts',(-22.5834711038022,1.76496910283088,
0.));
#200820=CARTESIAN_POINT('Ctrl Pts',(-22.5834711038022,1.76496910283088,
12.));
#200821=CARTESIAN_POINT('Ctrl Pts',(-22.5757315316353,1.76507744026746,
0.));
#200822=CARTESIAN_POINT('Ctrl Pts',(-22.5757315316353,1.76507744026746,
12.));
#200823=CARTESIAN_POINT('Ctrl Pts',(-22.5682508499873,1.76515418518831,
0.));
#200824=CARTESIAN_POINT('Ctrl Pts',(-22.5682508499873,1.76515418518831,
12.));
#200825=CARTESIAN_POINT('Ctrl Pts',(-22.5610344912501,1.7652010450045,0.));
#200826=CARTESIAN_POINT('Ctrl Pts',(-22.5610344912501,1.7652010450045,12.));
#200827=CARTESIAN_POINT('Ctrl Pts',(-22.5540882235837,1.76521983384062,
0.));
#200828=CARTESIAN_POINT('Ctrl Pts',(-22.5540882235837,1.76521983384062,
12.));
#200829=CARTESIAN_POINT('Ctrl Pts',(-22.5474180954006,1.76521245524047,
0.));
#200830=CARTESIAN_POINT('Ctrl Pts',(-22.5474180954006,1.76521245524047,
12.));
#200831=CARTESIAN_POINT('Ctrl Pts',(-22.5410303590892,1.76518087841493,
0.));
#200832=CARTESIAN_POINT('Ctrl Pts',(-22.5410303590892,1.76518087841493,
12.));
#200833=CARTESIAN_POINT('Ctrl Pts',(-22.5349313983571,1.76512711563254,
0.));
#200834=CARTESIAN_POINT('Ctrl Pts',(-22.5349313983571,1.76512711563254,
12.));
#200835=CARTESIAN_POINT('Ctrl Pts',(-22.529127665298,1.76505320262759,0.));
#200836=CARTESIAN_POINT('Ctrl Pts',(-22.529127665298,1.76505320262759,12.));
#200837=CARTESIAN_POINT('Ctrl Pts',(-22.5236259635515,1.76496128643375,
0.));
#200838=CARTESIAN_POINT('Ctrl Pts',(-22.5236259635515,1.76496128643375,
12.));
#200839=CARTESIAN_POINT('Ctrl Pts',(-22.5184336670207,1.76485369319895,
0.));
#200840=CARTESIAN_POINT('Ctrl Pts',(-22.5184336670207,1.76485369319895,
12.));
#200841=CARTESIAN_POINT('Ctrl Pts',(-22.5135590569554,1.76473303281149,
0.));
#200842=CARTESIAN_POINT('Ctrl Pts',(-22.5135590569554,1.76473303281149,
12.));
#200843=CARTESIAN_POINT('Ctrl Pts',(-22.5090112700212,1.76460218257313,
0.));
#200844=CARTESIAN_POINT('Ctrl Pts',(-22.5090112700212,1.76460218257313,
12.));
#200845=CARTESIAN_POINT('Ctrl Pts',(-22.5047996391978,1.76446408210364,
0.));
#200846=CARTESIAN_POINT('Ctrl Pts',(-22.5047996391978,1.76446408210364,
12.));
#200847=CARTESIAN_POINT('Ctrl Pts',(-22.5009332677316,1.76432160068737,
0.));
#200848=CARTESIAN_POINT('Ctrl Pts',(-22.5009332677316,1.76432160068737,
12.));
#200849=CARTESIAN_POINT('Ctrl Pts',(-22.4974203063191,1.76417731243483,
0.));
#200850=CARTESIAN_POINT('Ctrl Pts',(-22.4974203063191,1.76417731243483,
12.));
#200851=CARTESIAN_POINT('Ctrl Pts',(-22.4942693792449,1.76403393880316,
0.));
#200852=CARTESIAN_POINT('Ctrl Pts',(-22.4942693792449,1.76403393880316,
12.));
#200853=CARTESIAN_POINT('Ctrl Pts',(-22.4914909094908,1.76389475965714,
0.));
#200854=CARTESIAN_POINT('Ctrl Pts',(-22.4914909094908,1.76389475965714,
12.));
#200855=CARTESIAN_POINT('Ctrl Pts',(-22.4890991659479,1.76376424879468,
0.));
#200856=CARTESIAN_POINT('Ctrl Pts',(-22.4890991659479,1.76376424879468,
12.));
#200857=CARTESIAN_POINT('Ctrl Pts',(-22.4871115206572,1.76364784232925,
0.));
#200858=CARTESIAN_POINT('Ctrl Pts',(-22.4871115206572,1.76364784232925,
12.));
#200859=CARTESIAN_POINT('Ctrl Pts',(-22.4855446605991,1.76355076045549,
0.));
#200860=CARTESIAN_POINT('Ctrl Pts',(-22.4855446605991,1.76355076045549,
12.));
#200861=CARTESIAN_POINT('Ctrl Pts',(-22.4844112933125,1.76347698284861,
0.));
#200862=CARTESIAN_POINT('Ctrl Pts',(-22.4844112933125,1.76347698284861,
12.));
#200863=CARTESIAN_POINT('Ctrl Pts',(-22.4838562517064,1.76343813434659,
0.));
#200864=CARTESIAN_POINT('Ctrl Pts',(-22.4838562517064,1.76343813434659,
12.));
#200865=CARTESIAN_POINT('Ctrl Pts',(-22.4836387052228,1.76342064263637,
0.));
#200866=CARTESIAN_POINT('Ctrl Pts',(-22.4836387052228,1.76342064263637,
12.));
#200867=CARTESIAN_POINT('Ctrl Pts',(-22.4835819929788,1.7634141553879,0.));
#200868=CARTESIAN_POINT('Ctrl Pts',(-22.4835819929788,1.7634141553879,12.));
#200869=CARTESIAN_POINT('Ctrl Pts',(-22.4835757167854,1.7634122053118,0.));
#200870=CARTESIAN_POINT('Ctrl Pts',(-22.4835757167854,1.7634122053118,12.));
#200871=CARTESIAN_POINT('',(-25.991588367311,0.661312440730901,0.));
#200872=CARTESIAN_POINT('Ctrl Pts',(-25.991588367311,0.661312440730901,
0.));
#200873=CARTESIAN_POINT('Ctrl Pts',(-25.9865613464773,0.664028313187627,
0.));
#200874=CARTESIAN_POINT('Ctrl Pts',(-25.9765104298071,0.669451306780825,
0.));
#200875=CARTESIAN_POINT('Ctrl Pts',(-25.9614434297919,0.677559543209725,
0.));
#200876=CARTESIAN_POINT('Ctrl Pts',(-25.9413728471909,0.688318015057729,
0.));
#200877=CARTESIAN_POINT('Ctrl Pts',(-25.9163158909426,0.701678575228756,
0.));
#200878=CARTESIAN_POINT('Ctrl Pts',(-25.891290261497,0.714951588527638,
0.));
#200879=CARTESIAN_POINT('Ctrl Pts',(-25.8662960624185,0.728137036482335,
0.));
#200880=CARTESIAN_POINT('Ctrl Pts',(-25.8413334619055,0.741234902663807,
0.));
#200881=CARTESIAN_POINT('Ctrl Pts',(-25.8164027059984,0.754245175609524,
0.));
#200882=CARTESIAN_POINT('Ctrl Pts',(-25.7915041383376,0.767167852651168,
0.));
#200883=CARTESIAN_POINT('Ctrl Pts',(-25.7666381946955,0.780002940291965,
0.));
#200884=CARTESIAN_POINT('Ctrl Pts',(-25.7418053757746,0.792750451616127,
0.));
#200885=CARTESIAN_POINT('Ctrl Pts',(-25.7170062262525,0.805410404554352,
0.));
#200886=CARTESIAN_POINT('Ctrl Pts',(-25.6922413110194,0.817982819787464,
0.));
#200887=CARTESIAN_POINT('Ctrl Pts',(-25.6675111931952,0.830467718864205,
0.));
#200888=CARTESIAN_POINT('Ctrl Pts',(-25.6428164100055,0.842865122120758,
0.));
#200889=CARTESIAN_POINT('Ctrl Pts',(-25.6181574536049,0.855175047036549,
0.));
#200890=CARTESIAN_POINT('Ctrl Pts',(-25.5935347843585,0.867397509338431,
0.));
#200891=CARTESIAN_POINT('Ctrl Pts',(-25.5689488408156,0.879532523834294,
0.));
#200892=CARTESIAN_POINT('Ctrl Pts',(-25.5444000508211,0.89158010534904,
0.));
#200893=CARTESIAN_POINT('Ctrl Pts',(-25.5198888424194,0.903540269651106,
0.));
#200894=CARTESIAN_POINT('Ctrl Pts',(-25.4954156541795,0.915413034335613,
0.));
#200895=CARTESIAN_POINT('Ctrl Pts',(-25.4709809475009,0.927198419886094,
0.));
#200896=CARTESIAN_POINT('Ctrl Pts',(-25.4465852044849,0.938896449496192,
0.));
#200897=CARTESIAN_POINT('Ctrl Pts',(-25.4222289223167,0.950507148597468,
0.));
#200898=CARTESIAN_POINT('Ctrl Pts',(-25.3979126089163,0.962030544503142,
0.));
#200899=CARTESIAN_POINT('Ctrl Pts',(-25.3736367778845,0.973466666000163,
0.));
#200900=CARTESIAN_POINT('Ctrl Pts',(-25.3494019441441,0.984815543003973,
0.));
#200901=CARTESIAN_POINT('Ctrl Pts',(-25.3252086182968,0.996077206120624,
0.));
#200902=CARTESIAN_POINT('Ctrl Pts',(-25.3010573055547,1.00725168656896,
0.));
#200903=CARTESIAN_POINT('Ctrl Pts',(-25.276948508726,1.01833901642237,0.));
#200904=CARTESIAN_POINT('Ctrl Pts',(-25.2528827300422,1.02933922876806,
0.));
#200905=CARTESIAN_POINT('Ctrl Pts',(-25.2288604735086,1.04025235791507,
0.));
#200906=CARTESIAN_POINT('Ctrl Pts',(-25.2048822469028,1.05107843957931,
0.));
#200907=CARTESIAN_POINT('Ctrl Pts',(-25.1809485642192,1.06181751111768,
0.));
#200908=CARTESIAN_POINT('Ctrl Pts',(-25.157059946931,1.07246961165475,0.));
#200909=CARTESIAN_POINT('Ctrl Pts',(-25.1332169227413,1.08303478197187,
0.));
#200910=CARTESIAN_POINT('Ctrl Pts',(-25.1094200248446,1.09351306445308,
0.));
#200911=CARTESIAN_POINT('Ctrl Pts',(-25.0856697909679,1.10390450301745,
0.));
#200912=CARTESIAN_POINT('Ctrl Pts',(-25.0619667625336,1.11420914306889,
0.));
#200913=CARTESIAN_POINT('Ctrl Pts',(-25.0383114836899,1.12442703144451,
0.));
#200914=CARTESIAN_POINT('Ctrl Pts',(-25.0147045006196,1.1345582163853,0.));
#200915=CARTESIAN_POINT('Ctrl Pts',(-24.9911463621433,1.144602747582,0.));
#200916=CARTESIAN_POINT('Ctrl Pts',(-24.9676376201502,1.15456067621889,
0.));
#200917=CARTESIAN_POINT('Ctrl Pts',(-24.9441788300932,1.16443205502849,
0.));
#200918=CARTESIAN_POINT('Ctrl Pts',(-24.9207705514449,1.17421693835041,
0.));
#200919=CARTESIAN_POINT('Ctrl Pts',(-24.8974133481829,1.18391538220103,
0.));
#200920=CARTESIAN_POINT('Ctrl Pts',(-24.8741077892075,1.19352744434064,
0.));
#200921=CARTESIAN_POINT('Ctrl Pts',(-24.8508544481974,1.2030531842602,0.));
#200922=CARTESIAN_POINT('Ctrl Pts',(-24.8276539035092,1.21249266318208,
0.));
#200923=CARTESIAN_POINT('Ctrl Pts',(-24.8045067380536,1.22184594406528,
0.));
#200924=CARTESIAN_POINT('Ctrl Pts',(-24.7814135391799,1.23111309161843,
0.));
#200925=CARTESIAN_POINT('Ctrl Pts',(-24.7583748985438,1.24029417231989,
0.));
#200926=CARTESIAN_POINT('Ctrl Pts',(-24.7353914120011,1.24938925444325,
0.));
#200927=CARTESIAN_POINT('Ctrl Pts',(-24.7124636797894,1.25839840807418,
0.));
#200928=CARTESIAN_POINT('Ctrl Pts',(-24.6895923066836,1.267321705135,0.));
#200929=CARTESIAN_POINT('Ctrl Pts',(-24.666777902156,1.27615921941642,0.));
#200930=CARTESIAN_POINT('Ctrl Pts',(-24.6440210805278,1.28491102661514,
0.));
#200931=CARTESIAN_POINT('Ctrl Pts',(-24.6213224611229,1.29357720438107,
0.));
#200932=CARTESIAN_POINT('Ctrl Pts',(-24.5986826684027,1.30215783236362,
0.));
#200933=CARTESIAN_POINT('Ctrl Pts',(-24.5761023320183,1.31065299222021,
0.));
#200934=CARTESIAN_POINT('Ctrl Pts',(-24.5535820868674,1.31906276763668,
0.));
#200935=CARTESIAN_POINT('Ctrl Pts',(-24.5311225731435,1.32738724435326,
0.));
#200936=CARTESIAN_POINT('Ctrl Pts',(-24.5087244363856,1.33562651019686,
0.));
#200937=CARTESIAN_POINT('Ctrl Pts',(-24.4863883275134,1.34378065512337,
0.));
#200938=CARTESIAN_POINT('Ctrl Pts',(-24.4641149028892,1.35184977125648,
0.));
#200939=CARTESIAN_POINT('Ctrl Pts',(-24.4419048244523,1.35983395290627,
0.));
#200940=CARTESIAN_POINT('Ctrl Pts',(-24.4197587598337,1.36773329659956,
0.));
#200941=CARTESIAN_POINT('Ctrl Pts',(-24.3976773824732,1.37554790111609,
0.));
#200942=CARTESIAN_POINT('Ctrl Pts',(-24.3756613717299,1.38327786752998,
0.));
#200943=CARTESIAN_POINT('Ctrl Pts',(-24.3537114129875,1.39092329926388,
0.));
#200944=CARTESIAN_POINT('Ctrl Pts',(-24.3318281977643,1.39848430212807,
0.));
#200945=CARTESIAN_POINT('Ctrl Pts',(-24.3100124238311,1.40596098434337,
0.));
#200946=CARTESIAN_POINT('Ctrl Pts',(-24.288264795321,1.41335345657682,0.));
#200947=CARTESIAN_POINT('Ctrl Pts',(-24.2665860228356,1.42066183198252,
0.));
#200948=CARTESIAN_POINT('Ctrl Pts',(-24.2449768235488,1.42788622624854,
0.));
#200949=CARTESIAN_POINT('Ctrl Pts',(-24.2234379212984,1.43502675765508,
0.));
#200950=CARTESIAN_POINT('Ctrl Pts',(-24.201970046722,1.44208354711082,0.));
#200951=CARTESIAN_POINT('Ctrl Pts',(-24.1805739374038,1.44905671818727,
0.));
#200952=CARTESIAN_POINT('Ctrl Pts',(-24.1592503380107,1.45594639716317,
0.));
#200953=CARTESIAN_POINT('Ctrl Pts',(-24.1380000004272,1.46275271307397,
0.));
#200954=CARTESIAN_POINT('Ctrl Pts',(-24.1168236838824,1.46947579776991,
0.));
#200955=CARTESIAN_POINT('Ctrl Pts',(-24.0957221550778,1.47611578597742,
0.));
#200956=CARTESIAN_POINT('Ctrl Pts',(-24.0746961883528,1.48267281533683,
0.));
#200957=CARTESIAN_POINT('Ctrl Pts',(-24.0537465658429,1.48914702644887,
0.));
#200958=CARTESIAN_POINT('Ctrl Pts',(-24.0328740776331,1.49553856292801,
0.));
#200959=CARTESIAN_POINT('Ctrl Pts',(-24.0120795219086,1.50184757146098,
0.));
#200960=CARTESIAN_POINT('Ctrl Pts',(-23.9913637050927,1.50807420187694,
0.));
#200961=CARTESIAN_POINT('Ctrl Pts',(-23.970727442014,1.51421860720614,0.));
#200962=CARTESIAN_POINT('Ctrl Pts',(-23.9501715561033,1.52028094372792,
0.));
#200963=CARTESIAN_POINT('Ctrl Pts',(-23.9296968795757,1.52626137103032,
0.));
#200964=CARTESIAN_POINT('Ctrl Pts',(-23.9093042536119,1.53216005207463,
0.));
#200965=CARTESIAN_POINT('Ctrl Pts',(-23.8889945285318,1.53797715326758,
0.));
#200966=CARTESIAN_POINT('Ctrl Pts',(-23.8687685639642,1.5437128445399,0.));
#200967=CARTESIAN_POINT('Ctrl Pts',(-23.8486272290705,1.54936729940541,
0.));
#200968=CARTESIAN_POINT('Ctrl Pts',(-23.8285714027636,1.55494069502635,
0.));
#200969=CARTESIAN_POINT('Ctrl Pts',(-23.8086019739194,1.56043321228633,
0.));
#200970=CARTESIAN_POINT('Ctrl Pts',(-23.7887198415878,1.56584503586843,
0.));
#200971=CARTESIAN_POINT('Ctrl Pts',(-23.7689259151862,1.57117635434408,
0.));
#200972=CARTESIAN_POINT('Ctrl Pts',(-23.749221114736,1.57642736025246,0.));
#200973=CARTESIAN_POINT('Ctrl Pts',(-23.72960637113,1.58159825017358,0.));
#200974=CARTESIAN_POINT('Ctrl Pts',(-23.710082626383,1.58668922481221,0.));
#200975=CARTESIAN_POINT('Ctrl Pts',(-23.6906508338833,1.59170048908633,
0.));
#200976=CARTESIAN_POINT('Ctrl Pts',(-23.671311958631,1.59663225222463,0.));
#200977=CARTESIAN_POINT('Ctrl Pts',(-23.6520669774876,1.60148472786595,
0.));
#200978=CARTESIAN_POINT('Ctrl Pts',(-23.6329168794929,1.60625813414672,
0.));
#200979=CARTESIAN_POINT('Ctrl Pts',(-23.6138626661653,1.61095269379778,
0.));
#200980=CARTESIAN_POINT('Ctrl Pts',(-23.5949053517997,1.61556863424698,
0.));
#200981=CARTESIAN_POINT('Ctrl Pts',(-23.57604596376,1.62010618772866,0.));
#200982=CARTESIAN_POINT('Ctrl Pts',(-23.5572855427601,1.62456559140064,
0.));
#200983=CARTESIAN_POINT('Ctrl Pts',(-23.538625143226,1.62894708745223,0.));
#200984=CARTESIAN_POINT('Ctrl Pts',(-23.5200658336612,1.63325092321725,
0.));
#200985=CARTESIAN_POINT('Ctrl Pts',(-23.5016086970003,1.63747735129474,
0.));
#200986=CARTESIAN_POINT('Ctrl Pts',(-23.4832548309645,1.64162662967528,
0.));
#200987=CARTESIAN_POINT('Ctrl Pts',(-23.4650053483932,1.64569902187611,
0.));
#200988=CARTESIAN_POINT('Ctrl Pts',(-23.4468613776574,1.6496947970734,0.));
#200989=CARTESIAN_POINT('Ctrl Pts',(-23.4288240631043,1.65361423023728,
0.));
#200990=CARTESIAN_POINT('Ctrl Pts',(-23.4108945654805,1.65745760227505,
0.));
#200991=CARTESIAN_POINT('Ctrl Pts',(-23.3930740623619,1.66122520018011,
0.));
#200992=CARTESIAN_POINT('Ctrl Pts',(-23.3753637485545,1.66491731718876,
0.));
#200993=CARTESIAN_POINT('Ctrl Pts',(-23.3577648365744,1.66853425293995,
0.));
#200994=CARTESIAN_POINT('Ctrl Pts',(-23.3402785571865,1.67207631363921,
0.));
#200995=CARTESIAN_POINT('Ctrl Pts',(-23.3229061599145,1.67554381222994,
0.));
#200996=CARTESIAN_POINT('Ctrl Pts',(-23.3056489135611,1.67893706857117,
0.));
#200997=CARTESIAN_POINT('Ctrl Pts',(-23.2885081066951,1.68225640962168,
0.));
#200998=CARTESIAN_POINT('Ctrl Pts',(-23.2714850482246,1.68550216963258,
0.));
#200999=CARTESIAN_POINT('Ctrl Pts',(-23.2545810680537,1.68867469034896,
0.));
#201000=CARTESIAN_POINT('Ctrl Pts',(-23.2377975177013,1.69177432121711,
0.));
#201001=CARTESIAN_POINT('Ctrl Pts',(-23.2211357709374,1.69480141959953,
0.));
#201002=CARTESIAN_POINT('Ctrl Pts',(-23.2045972243767,1.69775635099443,
0.));
#201003=CARTESIAN_POINT('Ctrl Pts',(-23.1881832981851,1.7006394892701,0.));
#201004=CARTESIAN_POINT('Ctrl Pts',(-23.1718954368751,1.70345121691276,
0.));
#201005=CARTESIAN_POINT('Ctrl Pts',(-23.1557351100614,1.70619192527852,
0.));
#201006=CARTESIAN_POINT('Ctrl Pts',(-23.1397038132356,1.70886201485452,
0.));
#201007=CARTESIAN_POINT('Ctrl Pts',(-23.1238030684925,1.71146189552174,
0.));
#201008=CARTESIAN_POINT('Ctrl Pts',(-23.1080344254286,1.71399198684704,
0.));
#201009=CARTESIAN_POINT('Ctrl Pts',(-23.0923994621213,1.71645271839296,
0.));
#201010=CARTESIAN_POINT('Ctrl Pts',(-23.0768997860709,1.71884453003027,
0.));
#201011=CARTESIAN_POINT('Ctrl Pts',(-23.0615370351562,1.72116787225991,
0.));
#201012=CARTESIAN_POINT('Ctrl Pts',(-23.0463128785531,1.72342320653746,
0.));
#201013=CARTESIAN_POINT('Ctrl Pts',(-23.0312290178883,1.72561100564045,
0.));
#201014=CARTESIAN_POINT('Ctrl Pts',(-23.0162871884168,1.72773175404708,
0.));
#201015=CARTESIAN_POINT('Ctrl Pts',(-23.001489160189,1.72978594832136,0.));
#201016=CARTESIAN_POINT('Ctrl Pts',(-22.9868367391978,1.7317740975019,0.));
#201017=CARTESIAN_POINT('Ctrl Pts',(-22.9723317685688,1.73369672350814,
0.));
#201018=CARTESIAN_POINT('Ctrl Pts',(-22.9579761301063,1.73555436162769,
0.));
#201019=CARTESIAN_POINT('Ctrl Pts',(-22.9437717457826,1.73734756100039,
0.));
#201020=CARTESIAN_POINT('Ctrl Pts',(-22.9297205792586,1.73907688511666,
0.));
#201021=CARTESIAN_POINT('Ctrl Pts',(-22.9158246373363,1.74074291231058,
0.));
#201022=CARTESIAN_POINT('Ctrl Pts',(-22.9020859716141,1.7423462363008,0.));
#201023=CARTESIAN_POINT('Ctrl Pts',(-22.888506680335,1.74388746677702,0.));
#201024=CARTESIAN_POINT('Ctrl Pts',(-22.8750889101696,1.74536722998201,
0.));
#201025=CARTESIAN_POINT('Ctrl Pts',(-22.8618348580235,1.74678616930664,
0.));
#201026=CARTESIAN_POINT('Ctrl Pts',(-22.8487467728076,1.74814494588492,
0.));
#201027=CARTESIAN_POINT('Ctrl Pts',(-22.8358269579853,1.74944423940115,
0.));
#201028=CARTESIAN_POINT('Ctrl Pts',(-22.8230777741284,1.75068474890883,
0.));
#201029=CARTESIAN_POINT('Ctrl Pts',(-22.8105016414713,1.75186719365592,
0.));
#201030=CARTESIAN_POINT('Ctrl Pts',(-22.7981010424314,1.75299231391466,
0.));
#201031=CARTESIAN_POINT('Ctrl Pts',(-22.7858785242361,1.75406087182936,
0.));
#201032=CARTESIAN_POINT('Ctrl Pts',(-22.7738367016118,1.75507365227131,
0.));
#201033=CARTESIAN_POINT('Ctrl Pts',(-22.7619782595013,1.75603146371641,
0.));
#201034=CARTESIAN_POINT('Ctrl Pts',(-22.750305955645,1.75693513908907,0.));
#201035=CARTESIAN_POINT('Ctrl Pts',(-22.7388226235559,1.75778553673244,
0.));
#201036=CARTESIAN_POINT('Ctrl Pts',(-22.72753117773,1.75858354204633,0.));
#201037=CARTESIAN_POINT('Ctrl Pts',(-22.7164346186006,1.75933006905925,
0.));
#201038=CARTESIAN_POINT('Ctrl Pts',(-22.7055360375485,1.76002606202401,
0.));
#201039=CARTESIAN_POINT('Ctrl Pts',(-22.6948386219851,1.76067249704886,
0.));
#201040=CARTESIAN_POINT('Ctrl Pts',(-22.684345658525,1.76127038310614,0.));
#201041=CARTESIAN_POINT('Ctrl Pts',(-22.67406053567,1.76182076289525,0.));
#201042=CARTESIAN_POINT('Ctrl Pts',(-22.6639867471753,1.76232471392568,
0.));
#201043=CARTESIAN_POINT('Ctrl Pts',(-22.6541278938409,1.76278334912561,
0.));
#201044=CARTESIAN_POINT('Ctrl Pts',(-22.6444876940423,1.76319782013916,
0.));
#201045=CARTESIAN_POINT('Ctrl Pts',(-22.6350699979359,1.76356932176273,
0.));
#201046=CARTESIAN_POINT('Ctrl Pts',(-22.6258787994848,1.76389909571403,
0.));
#201047=CARTESIAN_POINT('Ctrl Pts',(-22.6169182517694,1.76418843543739,
0.));
#201048=CARTESIAN_POINT('Ctrl Pts',(-22.6081926681343,1.76443868648015,
0.));
#201049=CARTESIAN_POINT('Ctrl Pts',(-22.5997065145638,1.76465124413557,
0.));
#201050=CARTESIAN_POINT('Ctrl Pts',(-22.5914644078106,1.76482755288411,
0.));
#201051=CARTESIAN_POINT('Ctrl Pts',(-22.5834711038022,1.76496910283088,
0.));
#201052=CARTESIAN_POINT('Ctrl Pts',(-22.5757315316353,1.76507744026746,
0.));
#201053=CARTESIAN_POINT('Ctrl Pts',(-22.5682508499873,1.76515418518831,
0.));
#201054=CARTESIAN_POINT('Ctrl Pts',(-22.5610344912501,1.7652010450045,0.));
#201055=CARTESIAN_POINT('Ctrl Pts',(-22.5540882235837,1.76521983384062,
0.));
#201056=CARTESIAN_POINT('Ctrl Pts',(-22.5474180954006,1.76521245524047,
0.));
#201057=CARTESIAN_POINT('Ctrl Pts',(-22.5410303590892,1.76518087841493,
0.));
#201058=CARTESIAN_POINT('Ctrl Pts',(-22.5349313983571,1.76512711563254,
0.));
#201059=CARTESIAN_POINT('Ctrl Pts',(-22.529127665298,1.76505320262759,0.));
#201060=CARTESIAN_POINT('Ctrl Pts',(-22.5236259635515,1.76496128643375,
0.));
#201061=CARTESIAN_POINT('Ctrl Pts',(-22.5184336670207,1.76485369319895,
0.));
#201062=CARTESIAN_POINT('Ctrl Pts',(-22.5135590569554,1.76473303281149,
0.));
#201063=CARTESIAN_POINT('Ctrl Pts',(-22.5090112700212,1.76460218257313,
0.));
#201064=CARTESIAN_POINT('Ctrl Pts',(-22.5047996391978,1.76446408210364,
0.));
#201065=CARTESIAN_POINT('Ctrl Pts',(-22.5009332677316,1.76432160068737,
0.));
#201066=CARTESIAN_POINT('Ctrl Pts',(-22.4974203063191,1.76417731243483,
0.));
#201067=CARTESIAN_POINT('Ctrl Pts',(-22.4942693792449,1.76403393880316,
0.));
#201068=CARTESIAN_POINT('Ctrl Pts',(-22.4914909094908,1.76389475965714,
0.));
#201069=CARTESIAN_POINT('Ctrl Pts',(-22.4890991659479,1.76376424879468,
0.));
#201070=CARTESIAN_POINT('Ctrl Pts',(-22.4871115206572,1.76364784232925,
0.));
#201071=CARTESIAN_POINT('Ctrl Pts',(-22.4855446605991,1.76355076045549,
0.));
#201072=CARTESIAN_POINT('Ctrl Pts',(-22.4844112933125,1.76347698284861,
0.));
#201073=CARTESIAN_POINT('Ctrl Pts',(-22.4838562517064,1.76343813434659,
0.));
#201074=CARTESIAN_POINT('Ctrl Pts',(-22.4836387052228,1.76342064263637,
0.));
#201075=CARTESIAN_POINT('Ctrl Pts',(-22.4835819929788,1.7634141553879,0.));
#201076=CARTESIAN_POINT('Ctrl Pts',(-22.4835757167854,1.7634122053118,0.));
#201077=CARTESIAN_POINT('',(-25.991588367311,0.661312440730901,0.));
#201078=CARTESIAN_POINT('Ctrl Pts',(-22.1738711152697,4.11585220600461,
0.));
#201079=CARTESIAN_POINT('Ctrl Pts',(-22.1738711152697,4.11585220600461,
12.));
#201080=CARTESIAN_POINT('Ctrl Pts',(-22.173877682324,4.11585194677442,0.));
#201081=CARTESIAN_POINT('Ctrl Pts',(-22.173877682324,4.11585194677442,12.));
#201082=CARTESIAN_POINT('Ctrl Pts',(-22.1739341411687,4.11586035878287,
0.));
#201083=CARTESIAN_POINT('Ctrl Pts',(-22.1739341411687,4.11586035878287,
12.));
#201084=CARTESIAN_POINT('Ctrl Pts',(-22.1741488021234,4.11589976826166,
0.));
#201085=CARTESIAN_POINT('Ctrl Pts',(-22.1741488021234,4.11589976826166,
12.));
#201086=CARTESIAN_POINT('Ctrl Pts',(-22.1746949858775,4.11600589882845,
0.));
#201087=CARTESIAN_POINT('Ctrl Pts',(-22.1746949858775,4.11600589882845,
12.));
#201088=CARTESIAN_POINT('Ctrl Pts',(-22.1758088296598,4.11622797217068,
0.));
#201089=CARTESIAN_POINT('Ctrl Pts',(-22.1758088296598,4.11622797217068,
12.));
#201090=CARTESIAN_POINT('Ctrl Pts',(-22.177347426894,4.11653973150518,0.));
#201091=CARTESIAN_POINT('Ctrl Pts',(-22.177347426894,4.11653973150518,12.));
#201092=CARTESIAN_POINT('Ctrl Pts',(-22.179297473024,4.11694173195003,0.));
#201093=CARTESIAN_POINT('Ctrl Pts',(-22.179297473024,4.11694173195003,12.));
#201094=CARTESIAN_POINT('Ctrl Pts',(-22.1816414985788,4.11743469691756,
0.));
#201095=CARTESIAN_POINT('Ctrl Pts',(-22.1816414985788,4.11743469691756,
12.));
#201096=CARTESIAN_POINT('Ctrl Pts',(-22.1843613164855,4.11801938107479,
0.));
#201097=CARTESIAN_POINT('Ctrl Pts',(-22.1843613164855,4.11801938107479,
12.));
#201098=CARTESIAN_POINT('Ctrl Pts',(-22.1874419861496,4.11869641271773,
0.));
#201099=CARTESIAN_POINT('Ctrl Pts',(-22.1874419861496,4.11869641271773,
12.));
#201100=CARTESIAN_POINT('Ctrl Pts',(-22.1908725908525,4.11946626228636,
0.));
#201101=CARTESIAN_POINT('Ctrl Pts',(-22.1908725908525,4.11946626228636,
12.));
#201102=CARTESIAN_POINT('Ctrl Pts',(-22.1946440958098,4.12032932637736,
0.));
#201103=CARTESIAN_POINT('Ctrl Pts',(-22.1946440958098,4.12032932637736,
12.));
#201104=CARTESIAN_POINT('Ctrl Pts',(-22.1987479618246,4.12128598183522,
0.));
#201105=CARTESIAN_POINT('Ctrl Pts',(-22.1987479618246,4.12128598183522,
12.));
#201106=CARTESIAN_POINT('Ctrl Pts',(-22.2031746532106,4.12233664408227,
0.));
#201107=CARTESIAN_POINT('Ctrl Pts',(-22.2031746532106,4.12233664408227,
12.));
#201108=CARTESIAN_POINT('Ctrl Pts',(-22.2079143941719,4.12348173702023,
0.));
#201109=CARTESIAN_POINT('Ctrl Pts',(-22.2079143941719,4.12348173702023,
12.));
#201110=CARTESIAN_POINT('Ctrl Pts',(-22.2129576146671,4.12472167516607,
0.));
#201111=CARTESIAN_POINT('Ctrl Pts',(-22.2129576146671,4.12472167516607,
12.));
#201112=CARTESIAN_POINT('Ctrl Pts',(-22.2182956401341,4.12605683613307,
0.));
#201113=CARTESIAN_POINT('Ctrl Pts',(-22.2182956401341,4.12605683613307,
12.));
#201114=CARTESIAN_POINT('Ctrl Pts',(-22.2239207458781,4.12748755830104,
0.));
#201115=CARTESIAN_POINT('Ctrl Pts',(-22.2239207458781,4.12748755830104,
12.));
#201116=CARTESIAN_POINT('Ctrl Pts',(-22.2298258043947,4.12901415463379,
0.));
#201117=CARTESIAN_POINT('Ctrl Pts',(-22.2298258043947,4.12901415463379,
12.));
#201118=CARTESIAN_POINT('Ctrl Pts',(-22.2360040565533,4.13063692157498,
0.));
#201119=CARTESIAN_POINT('Ctrl Pts',(-22.2360040565533,4.13063692157498,
12.));
#201120=CARTESIAN_POINT('Ctrl Pts',(-22.2424488153523,4.1323561506016,0.));
#201121=CARTESIAN_POINT('Ctrl Pts',(-22.2424488153523,4.1323561506016,12.));
#201122=CARTESIAN_POINT('Ctrl Pts',(-22.249153531779,4.1341721255881,0.));
#201123=CARTESIAN_POINT('Ctrl Pts',(-22.249153531779,4.1341721255881,12.));
#201124=CARTESIAN_POINT('Ctrl Pts',(-22.2561118708421,4.13608511977225,
0.));
#201125=CARTESIAN_POINT('Ctrl Pts',(-22.2561118708421,4.13608511977225,
12.));
#201126=CARTESIAN_POINT('Ctrl Pts',(-22.2633177913972,4.13809539255421,
0.));
#201127=CARTESIAN_POINT('Ctrl Pts',(-22.2633177913972,4.13809539255421,
12.));
#201128=CARTESIAN_POINT('Ctrl Pts',(-22.2707656042457,4.14020318715991,
0.));
#201129=CARTESIAN_POINT('Ctrl Pts',(-22.2707656042457,4.14020318715991,
12.));
#201130=CARTESIAN_POINT('Ctrl Pts',(-22.2784499072027,4.14240873321984,
0.));
#201131=CARTESIAN_POINT('Ctrl Pts',(-22.2784499072027,4.14240873321984,
12.));
#201132=CARTESIAN_POINT('Ctrl Pts',(-22.2863655389166,4.14471224859295,
0.));
#201133=CARTESIAN_POINT('Ctrl Pts',(-22.2863655389166,4.14471224859295,
12.));
#201134=CARTESIAN_POINT('Ctrl Pts',(-22.2945075198467,4.14711394168556,
0.));
#201135=CARTESIAN_POINT('Ctrl Pts',(-22.2945075198467,4.14711394168556,
12.));
#201136=CARTESIAN_POINT('Ctrl Pts',(-22.3028710166933,4.14961401285522,
0.));
#201137=CARTESIAN_POINT('Ctrl Pts',(-22.3028710166933,4.14961401285522,
12.));
#201138=CARTESIAN_POINT('Ctrl Pts',(-22.3114513545185,4.1522126539699,0.));
#201139=CARTESIAN_POINT('Ctrl Pts',(-22.3114513545185,4.1522126539699,12.));
#201140=CARTESIAN_POINT('Ctrl Pts',(-22.3202440186979,4.15491004835281,
0.));
#201141=CARTESIAN_POINT('Ctrl Pts',(-22.3202440186979,4.15491004835281,
12.));
#201142=CARTESIAN_POINT('Ctrl Pts',(-22.3292446628959,4.15770637047889,
0.));
#201143=CARTESIAN_POINT('Ctrl Pts',(-22.3292446628959,4.15770637047889,
12.));
#201144=CARTESIAN_POINT('Ctrl Pts',(-22.3384491078602,4.16060178604164,
0.));
#201145=CARTESIAN_POINT('Ctrl Pts',(-22.3384491078602,4.16060178604164,
12.));
#201146=CARTESIAN_POINT('Ctrl Pts',(-22.3478533253889,4.16359645263187,
0.));
#201147=CARTESIAN_POINT('Ctrl Pts',(-22.3478533253889,4.16359645263187,
12.));
#201148=CARTESIAN_POINT('Ctrl Pts',(-22.3574534257396,4.166690520266,0.));
#201149=CARTESIAN_POINT('Ctrl Pts',(-22.3574534257396,4.166690520266,12.));
#201150=CARTESIAN_POINT('Ctrl Pts',(-22.36724564276,4.16988413199457,0.));
#201151=CARTESIAN_POINT('Ctrl Pts',(-22.36724564276,4.16988413199457,12.));
#201152=CARTESIAN_POINT('Ctrl Pts',(-22.3772263228617,4.17317742436145,
0.));
#201153=CARTESIAN_POINT('Ctrl Pts',(-22.3772263228617,4.17317742436145,
12.));
#201154=CARTESIAN_POINT('Ctrl Pts',(-22.3873919231334,4.17657052752825,
0.));
#201155=CARTESIAN_POINT('Ctrl Pts',(-22.3873919231334,4.17657052752825,
12.));
#201156=CARTESIAN_POINT('Ctrl Pts',(-22.3977390078075,4.18006356544882,
0.));
#201157=CARTESIAN_POINT('Ctrl Pts',(-22.3977390078075,4.18006356544882,
12.));
#201158=CARTESIAN_POINT('Ctrl Pts',(-22.4082642454453,4.1836566560085,0.));
#201159=CARTESIAN_POINT('Ctrl Pts',(-22.4082642454453,4.1836566560085,12.));
#201160=CARTESIAN_POINT('Ctrl Pts',(-22.4189644056115,4.1873499111772,0.));
#201161=CARTESIAN_POINT('Ctrl Pts',(-22.4189644056115,4.1873499111772,12.));
#201162=CARTESIAN_POINT('Ctrl Pts',(-22.4298363535421,4.19114343726941,
0.));
#201163=CARTESIAN_POINT('Ctrl Pts',(-22.4298363535421,4.19114343726941,
12.));
#201164=CARTESIAN_POINT('Ctrl Pts',(-22.4408770448917,4.1950373351886,0.));
#201165=CARTESIAN_POINT('Ctrl Pts',(-22.4408770448917,4.1950373351886,12.));
#201166=CARTESIAN_POINT('Ctrl Pts',(-22.4520835205419,4.19903170066354,
0.));
#201167=CARTESIAN_POINT('Ctrl Pts',(-22.4520835205419,4.19903170066354,
12.));
#201168=CARTESIAN_POINT('Ctrl Pts',(-22.4634529011433,4.2031266244817,0.));
#201169=CARTESIAN_POINT('Ctrl Pts',(-22.4634529011433,4.2031266244817,12.));
#201170=CARTESIAN_POINT('Ctrl Pts',(-22.4749823839915,4.20732219265648,
0.));
#201171=CARTESIAN_POINT('Ctrl Pts',(-22.4749823839915,4.20732219265648,
12.));
#201172=CARTESIAN_POINT('Ctrl Pts',(-22.4866692403147,4.21161848657428,
0.));
#201173=CARTESIAN_POINT('Ctrl Pts',(-22.4866692403147,4.21161848657428,
12.));
#201174=CARTESIAN_POINT('Ctrl Pts',(-22.4985108124229,4.21601558313908,
0.));
#201175=CARTESIAN_POINT('Ctrl Pts',(-22.4985108124229,4.21601558313908,
12.));
#201176=CARTESIAN_POINT('Ctrl Pts',(-22.5105045108882,4.22051355490196,
0.));
#201177=CARTESIAN_POINT('Ctrl Pts',(-22.5105045108882,4.22051355490196,
12.));
#201178=CARTESIAN_POINT('Ctrl Pts',(-22.5226478117885,4.2251124702004,0.));
#201179=CARTESIAN_POINT('Ctrl Pts',(-22.5226478117885,4.2251124702004,12.));
#201180=CARTESIAN_POINT('Ctrl Pts',(-22.5349382540587,4.22981239330731,
0.));
#201181=CARTESIAN_POINT('Ctrl Pts',(-22.5349382540587,4.22981239330731,
12.));
#201182=CARTESIAN_POINT('Ctrl Pts',(-22.5473734368086,4.23461338456713,
0.));
#201183=CARTESIAN_POINT('Ctrl Pts',(-22.5473734368086,4.23461338456713,
12.));
#201184=CARTESIAN_POINT('Ctrl Pts',(-22.559951016643,4.23951550052526,0.));
#201185=CARTESIAN_POINT('Ctrl Pts',(-22.559951016643,4.23951550052526,12.));
#201186=CARTESIAN_POINT('Ctrl Pts',(-22.5726687049922,4.24451879404858,
0.));
#201187=CARTESIAN_POINT('Ctrl Pts',(-22.5726687049922,4.24451879404858,
12.));
#201188=CARTESIAN_POINT('Ctrl Pts',(-22.5855242662479,4.24962331444184,
0.));
#201189=CARTESIAN_POINT('Ctrl Pts',(-22.5855242662479,4.24962331444184,
12.));
#201190=CARTESIAN_POINT('Ctrl Pts',(-22.5985155158637,4.25482910755485,
0.));
#201191=CARTESIAN_POINT('Ctrl Pts',(-22.5985155158637,4.25482910755485,
12.));
#201192=CARTESIAN_POINT('Ctrl Pts',(-22.611640318482,4.26013621588303,0.));
#201193=CARTESIAN_POINT('Ctrl Pts',(-22.611640318482,4.26013621588303,12.));
#201194=CARTESIAN_POINT('Ctrl Pts',(-22.6248965859975,4.26554467865571,
0.));
#201195=CARTESIAN_POINT('Ctrl Pts',(-22.6248965859975,4.26554467865571,
12.));
#201196=CARTESIAN_POINT('Ctrl Pts',(-22.6382822758171,4.27105453192999,
0.));
#201197=CARTESIAN_POINT('Ctrl Pts',(-22.6382822758171,4.27105453192999,
12.));
#201198=CARTESIAN_POINT('Ctrl Pts',(-22.6517953893303,4.27666580869117,
0.));
#201199=CARTESIAN_POINT('Ctrl Pts',(-22.6517953893303,4.27666580869117,
12.));
#201200=CARTESIAN_POINT('Ctrl Pts',(-22.665433970311,4.28237853894059,0.));
#201201=CARTESIAN_POINT('Ctrl Pts',(-22.665433970311,4.28237853894059,12.));
#201202=CARTESIAN_POINT('Ctrl Pts',(-22.6791961033537,4.28819274977766,
0.));
#201203=CARTESIAN_POINT('Ctrl Pts',(-22.6791961033537,4.28819274977766,
12.));
#201204=CARTESIAN_POINT('Ctrl Pts',(-22.6930799122545,4.29410846547061,
0.));
#201205=CARTESIAN_POINT('Ctrl Pts',(-22.6930799122545,4.29410846547061,
12.));
#201206=CARTESIAN_POINT('Ctrl Pts',(-22.707083558756,4.30012570754066,0.));
#201207=CARTESIAN_POINT('Ctrl Pts',(-22.707083558756,4.30012570754066,12.));
#201208=CARTESIAN_POINT('Ctrl Pts',(-22.7212052413384,4.30624449484074,
0.));
#201209=CARTESIAN_POINT('Ctrl Pts',(-22.7212052413384,4.30624449484074,
12.));
#201210=CARTESIAN_POINT('Ctrl Pts',(-22.7354431939927,4.3124648436255,0.));
#201211=CARTESIAN_POINT('Ctrl Pts',(-22.7354431939927,4.3124648436255,12.));
#201212=CARTESIAN_POINT('Ctrl Pts',(-22.7497956849852,4.3187867676123,0.));
#201213=CARTESIAN_POINT('Ctrl Pts',(-22.7497956849852,4.3187867676123,12.));
#201214=CARTESIAN_POINT('Ctrl Pts',(-22.764261015648,4.32521027803747,0.));
#201215=CARTESIAN_POINT('Ctrl Pts',(-22.764261015648,4.32521027803747,12.));
#201216=CARTESIAN_POINT('Ctrl Pts',(-22.7788375194081,4.33173538373182,
0.));
#201217=CARTESIAN_POINT('Ctrl Pts',(-22.7788375194081,4.33173538373182,
12.));
#201218=CARTESIAN_POINT('Ctrl Pts',(-22.7935235607807,4.33836209118442,
0.));
#201219=CARTESIAN_POINT('Ctrl Pts',(-22.7935235607807,4.33836209118442,
12.));
#201220=CARTESIAN_POINT('Ctrl Pts',(-22.808317534379,4.34509040460065,0.));
#201221=CARTESIAN_POINT('Ctrl Pts',(-22.808317534379,4.34509040460065,12.));
#201222=CARTESIAN_POINT('Ctrl Pts',(-22.8232178638873,4.35192032594801,
0.));
#201223=CARTESIAN_POINT('Ctrl Pts',(-22.8232178638873,4.35192032594801,
12.));
#201224=CARTESIAN_POINT('Ctrl Pts',(-22.838223001118,4.35885185500559,0.));
#201225=CARTESIAN_POINT('Ctrl Pts',(-22.838223001118,4.35885185500559,12.));
#201226=CARTESIAN_POINT('Ctrl Pts',(-22.8533314252419,4.36588498943009,
0.));
#201227=CARTESIAN_POINT('Ctrl Pts',(-22.8533314252419,4.36588498943009,
12.));
#201228=CARTESIAN_POINT('Ctrl Pts',(-22.8685416419725,4.37301972480752,
0.));
#201229=CARTESIAN_POINT('Ctrl Pts',(-22.8685416419725,4.37301972480752,
12.));
#201230=CARTESIAN_POINT('Ctrl Pts',(-22.8838521827702,4.38025605470089,
0.));
#201231=CARTESIAN_POINT('Ctrl Pts',(-22.8838521827702,4.38025605470089,
12.));
#201232=CARTESIAN_POINT('Ctrl Pts',(-22.8992616040108,4.38759397068391,
0.));
#201233=CARTESIAN_POINT('Ctrl Pts',(-22.8992616040108,4.38759397068391,
12.));
#201234=CARTESIAN_POINT('Ctrl Pts',(-22.9147684862425,4.39503346238454,
0.));
#201235=CARTESIAN_POINT('Ctrl Pts',(-22.9147684862425,4.39503346238454,
12.));
#201236=CARTESIAN_POINT('Ctrl Pts',(-22.9303714335549,4.40257451754307,
0.));
#201237=CARTESIAN_POINT('Ctrl Pts',(-22.9303714335549,4.40257451754307,
12.));
#201238=CARTESIAN_POINT('Ctrl Pts',(-22.9460690729093,4.41021712205547,
0.));
#201239=CARTESIAN_POINT('Ctrl Pts',(-22.9460690729093,4.41021712205547,
12.));
#201240=CARTESIAN_POINT('Ctrl Pts',(-22.9618600534866,4.41796126001309,
0.));
#201241=CARTESIAN_POINT('Ctrl Pts',(-22.9618600534866,4.41796126001309,
12.));
#201242=CARTESIAN_POINT('Ctrl Pts',(-22.9777430460021,4.42580691372771,
0.));
#201243=CARTESIAN_POINT('Ctrl Pts',(-22.9777430460021,4.42580691372771,
12.));
#201244=CARTESIAN_POINT('Ctrl Pts',(-22.9937167421009,4.43375406376904,
0.));
#201245=CARTESIAN_POINT('Ctrl Pts',(-22.9937167421009,4.43375406376904,
12.));
#201246=CARTESIAN_POINT('Ctrl Pts',(-23.0097798538399,4.44180268901666,
0.));
#201247=CARTESIAN_POINT('Ctrl Pts',(-23.0097798538399,4.44180268901666,
12.));
#201248=CARTESIAN_POINT('Ctrl Pts',(-23.0259311131395,4.44995276669698,
0.));
#201249=CARTESIAN_POINT('Ctrl Pts',(-23.0259311131395,4.44995276669698,
12.));
#201250=CARTESIAN_POINT('Ctrl Pts',(-23.0421692712466,4.45820427241676,
0.));
#201251=CARTESIAN_POINT('Ctrl Pts',(-23.0421692712466,4.45820427241676,
12.));
#201252=CARTESIAN_POINT('Ctrl Pts',(-23.0584930981723,4.46655718018205,
0.));
#201253=CARTESIAN_POINT('Ctrl Pts',(-23.0584930981723,4.46655718018205,
12.));
#201254=CARTESIAN_POINT('Ctrl Pts',(-23.0749013821868,4.47501146242821,
0.));
#201255=CARTESIAN_POINT('Ctrl Pts',(-23.0749013821868,4.47501146242821,
12.));
#201256=CARTESIAN_POINT('Ctrl Pts',(-23.0913929293909,4.48356709006756,
0.));
#201257=CARTESIAN_POINT('Ctrl Pts',(-23.0913929293909,4.48356709006756,
12.));
#201258=CARTESIAN_POINT('Ctrl Pts',(-23.1079665632629,4.49222403252201,
0.));
#201259=CARTESIAN_POINT('Ctrl Pts',(-23.1079665632629,4.49222403252201,
12.));
#201260=CARTESIAN_POINT('Ctrl Pts',(-23.1246211242117,4.50098225775178,
0.));
#201261=CARTESIAN_POINT('Ctrl Pts',(-23.1246211242117,4.50098225775178,
12.));
#201262=CARTESIAN_POINT('Ctrl Pts',(-23.1413554691136,4.50984173227087,
0.));
#201263=CARTESIAN_POINT('Ctrl Pts',(-23.1413554691136,4.50984173227087,
12.));
#201264=CARTESIAN_POINT('Ctrl Pts',(-23.1581684708778,4.51880242116785,
0.));
#201265=CARTESIAN_POINT('Ctrl Pts',(-23.1581684708778,4.51880242116785,
12.));
#201266=CARTESIAN_POINT('Ctrl Pts',(-23.1750590180923,4.52786428815047,
0.));
#201267=CARTESIAN_POINT('Ctrl Pts',(-23.1750590180923,4.52786428815047,
12.));
#201268=CARTESIAN_POINT('Ctrl Pts',(-23.1920260146474,4.53702729557585,
0.));
#201269=CARTESIAN_POINT('Ctrl Pts',(-23.1920260146474,4.53702729557585,
12.));
#201270=CARTESIAN_POINT('Ctrl Pts',(-23.2090683793627,4.54629140447542,
0.));
#201271=CARTESIAN_POINT('Ctrl Pts',(-23.2090683793627,4.54629140447542,
12.));
#201272=CARTESIAN_POINT('Ctrl Pts',(-23.2261850456055,4.55565657456956,
0.));
#201273=CARTESIAN_POINT('Ctrl Pts',(-23.2261850456055,4.55565657456956,
12.));
#201274=CARTESIAN_POINT('Ctrl Pts',(-23.2433749609117,4.5651227642781,0.));
#201275=CARTESIAN_POINT('Ctrl Pts',(-23.2433749609117,4.5651227642781,12.));
#201276=CARTESIAN_POINT('Ctrl Pts',(-23.2606370866853,4.5746899307607,0.));
#201277=CARTESIAN_POINT('Ctrl Pts',(-23.2606370866853,4.5746899307607,12.));
#201278=CARTESIAN_POINT('Ctrl Pts',(-23.2779703978868,4.58435802994674,
0.));
#201279=CARTESIAN_POINT('Ctrl Pts',(-23.2779703978868,4.58435802994674,
12.));
#201280=CARTESIAN_POINT('Ctrl Pts',(-23.295373882719,4.59412701655749,0.));
#201281=CARTESIAN_POINT('Ctrl Pts',(-23.295373882719,4.59412701655749,12.));
#201282=CARTESIAN_POINT('Ctrl Pts',(-23.3128465423119,4.60399684412174,
0.));
#201283=CARTESIAN_POINT('Ctrl Pts',(-23.3128465423119,4.60399684412174,
12.));
#201284=CARTESIAN_POINT('Ctrl Pts',(-23.3303873903947,4.61396746497848,
0.));
#201285=CARTESIAN_POINT('Ctrl Pts',(-23.3303873903947,4.61396746497848,
12.));
#201286=CARTESIAN_POINT('Ctrl Pts',(-23.3479954530281,4.62403883030823,
0.));
#201287=CARTESIAN_POINT('Ctrl Pts',(-23.3479954530281,4.62403883030823,
12.));
#201288=CARTESIAN_POINT('Ctrl Pts',(-23.3656697683496,4.63421089016554,
0.));
#201289=CARTESIAN_POINT('Ctrl Pts',(-23.3656697683496,4.63421089016554,
12.));
#201290=CARTESIAN_POINT('Ctrl Pts',(-23.383409386307,4.64448359349935,0.));
#201291=CARTESIAN_POINT('Ctrl Pts',(-23.383409386307,4.64448359349935,12.));
#201292=CARTESIAN_POINT('Ctrl Pts',(-23.4012133683957,4.65485688816921,
0.));
#201293=CARTESIAN_POINT('Ctrl Pts',(-23.4012133683957,4.65485688816921,
12.));
#201294=CARTESIAN_POINT('Ctrl Pts',(-23.4190807873798,4.66533072094663,
0.));
#201295=CARTESIAN_POINT('Ctrl Pts',(-23.4190807873798,4.66533072094663,
12.));
#201296=CARTESIAN_POINT('Ctrl Pts',(-23.4370107270444,4.6759050375305,0.));
#201297=CARTESIAN_POINT('Ctrl Pts',(-23.4370107270444,4.6759050375305,12.));
#201298=CARTESIAN_POINT('Ctrl Pts',(-23.4550022819853,4.68657978258297,
0.));
#201299=CARTESIAN_POINT('Ctrl Pts',(-23.4550022819853,4.68657978258297,
12.));
#201300=CARTESIAN_POINT('Ctrl Pts',(-23.4730545573849,4.69735489975023,
0.));
#201301=CARTESIAN_POINT('Ctrl Pts',(-23.4730545573849,4.69735489975023,
12.));
#201302=CARTESIAN_POINT('Ctrl Pts',(-23.491166668789,4.7082303316782,0.));
#201303=CARTESIAN_POINT('Ctrl Pts',(-23.491166668789,4.7082303316782,12.));
#201304=CARTESIAN_POINT('Ctrl Pts',(-23.5093377418784,4.71920602001904,
0.));
#201305=CARTESIAN_POINT('Ctrl Pts',(-23.5093377418784,4.71920602001904,
12.));
#201306=CARTESIAN_POINT('Ctrl Pts',(-23.5275669122378,4.73028190543031,
0.));
#201307=CARTESIAN_POINT('Ctrl Pts',(-23.5275669122378,4.73028190543031,
12.));
#201308=CARTESIAN_POINT('Ctrl Pts',(-23.5458533251715,4.74145792760698,
0.));
#201309=CARTESIAN_POINT('Ctrl Pts',(-23.5458533251715,4.74145792760698,
12.));
#201310=CARTESIAN_POINT('Ctrl Pts',(-23.564196135517,4.75273402530615,0.));
#201311=CARTESIAN_POINT('Ctrl Pts',(-23.564196135517,4.75273402530615,12.));
#201312=CARTESIAN_POINT('Ctrl Pts',(-23.5825945074535,4.7641101363625,0.));
#201313=CARTESIAN_POINT('Ctrl Pts',(-23.5825945074535,4.7641101363625,12.));
#201314=CARTESIAN_POINT('Ctrl Pts',(-23.6010476143099,4.77558619769875,
0.));
#201315=CARTESIAN_POINT('Ctrl Pts',(-23.6010476143099,4.77558619769875,
12.));
#201316=CARTESIAN_POINT('Ctrl Pts',(-23.6195546383625,4.78716214532104,
0.));
#201317=CARTESIAN_POINT('Ctrl Pts',(-23.6195546383625,4.78716214532104,
12.));
#201318=CARTESIAN_POINT('Ctrl Pts',(-23.6381147706581,4.79883791433229,
0.));
#201319=CARTESIAN_POINT('Ctrl Pts',(-23.6381147706581,4.79883791433229,
12.));
#201320=CARTESIAN_POINT('Ctrl Pts',(-23.6567272108631,4.81061343896442,
0.));
#201321=CARTESIAN_POINT('Ctrl Pts',(-23.6567272108631,4.81061343896442,
12.));
#201322=CARTESIAN_POINT('Ctrl Pts',(-23.6753911671023,4.82248865259569,
0.));
#201323=CARTESIAN_POINT('Ctrl Pts',(-23.6753911671023,4.82248865259569,
12.));
#201324=CARTESIAN_POINT('Ctrl Pts',(-23.6941058557971,4.83446348776267,
0.));
#201325=CARTESIAN_POINT('Ctrl Pts',(-23.6941058557971,4.83446348776267,
12.));
#201326=CARTESIAN_POINT('Ctrl Pts',(-23.7128705015014,4.84653787616422,
0.));
#201327=CARTESIAN_POINT('Ctrl Pts',(-23.7128705015014,4.84653787616422,
12.));
#201328=CARTESIAN_POINT('Ctrl Pts',(-23.7316843367308,4.85871174865491,
0.));
#201329=CARTESIAN_POINT('Ctrl Pts',(-23.7316843367308,4.85871174865491,
12.));
#201330=CARTESIAN_POINT('Ctrl Pts',(-23.7505466018239,4.87098503527142,
0.));
#201331=CARTESIAN_POINT('Ctrl Pts',(-23.7505466018239,4.87098503527142,
12.));
#201332=CARTESIAN_POINT('Ctrl Pts',(-23.7694565448044,4.88335766525565,
0.));
#201333=CARTESIAN_POINT('Ctrl Pts',(-23.7694565448044,4.88335766525565,
12.));
#201334=CARTESIAN_POINT('Ctrl Pts',(-23.7884134212381,4.89582956706771,
0.));
#201335=CARTESIAN_POINT('Ctrl Pts',(-23.7884134212381,4.89582956706771,
12.));
#201336=CARTESIAN_POINT('Ctrl Pts',(-23.8074164940897,4.90840066839346,
0.));
#201337=CARTESIAN_POINT('Ctrl Pts',(-23.8074164940897,4.90840066839346,
12.));
#201338=CARTESIAN_POINT('Ctrl Pts',(-23.8264650335721,4.92107089613976,
0.));
#201339=CARTESIAN_POINT('Ctrl Pts',(-23.8264650335721,4.92107089613976,
12.));
#201340=CARTESIAN_POINT('Ctrl Pts',(-23.8455583170062,4.93384017643441,
0.));
#201341=CARTESIAN_POINT('Ctrl Pts',(-23.8455583170062,4.93384017643441,
12.));
#201342=CARTESIAN_POINT('Ctrl Pts',(-23.8646956287172,4.94670843465868,
0.));
#201343=CARTESIAN_POINT('Ctrl Pts',(-23.8646956287172,4.94670843465868,
12.));
#201344=CARTESIAN_POINT('Ctrl Pts',(-23.883876259922,4.95967559546565,0.));
#201345=CARTESIAN_POINT('Ctrl Pts',(-23.883876259922,4.95967559546565,12.));
#201346=CARTESIAN_POINT('Ctrl Pts',(-23.9030995086164,4.97274158279228,
0.));
#201347=CARTESIAN_POINT('Ctrl Pts',(-23.9030995086164,4.97274158279228,
12.));
#201348=CARTESIAN_POINT('Ctrl Pts',(-23.9223646794591,4.98590631986532,
0.));
#201349=CARTESIAN_POINT('Ctrl Pts',(-23.9223646794591,4.98590631986532,
12.));
#201350=CARTESIAN_POINT('Ctrl Pts',(-23.9416710836529,4.99916972919309,
0.));
#201351=CARTESIAN_POINT('Ctrl Pts',(-23.9416710836529,4.99916972919309,
12.));
#201352=CARTESIAN_POINT('Ctrl Pts',(-23.9610180388271,5.01253173257458,
0.));
#201353=CARTESIAN_POINT('Ctrl Pts',(-23.9610180388271,5.01253173257458,
12.));
#201354=CARTESIAN_POINT('Ctrl Pts',(-23.9804048689228,5.02599225112461,
0.));
#201355=CARTESIAN_POINT('Ctrl Pts',(-23.9804048689228,5.02599225112461,
12.));
#201356=CARTESIAN_POINT('Ctrl Pts',(-23.9998309040747,5.03955120528527,
0.));
#201357=CARTESIAN_POINT('Ctrl Pts',(-23.9998309040747,5.03955120528527,
12.));
#201358=CARTESIAN_POINT('Ctrl Pts',(-24.0192954804896,5.05320851483068,
0.));
#201359=CARTESIAN_POINT('Ctrl Pts',(-24.0192954804896,5.05320851483068,
12.));
#201360=CARTESIAN_POINT('Ctrl Pts',(-24.0387979403268,5.06696409886639,
0.));
#201361=CARTESIAN_POINT('Ctrl Pts',(-24.0387979403268,5.06696409886639,
12.));
#201362=CARTESIAN_POINT('Ctrl Pts',(-24.0583376315636,5.0808178758127,0.));
#201363=CARTESIAN_POINT('Ctrl Pts',(-24.0583376315636,5.0808178758127,12.));
#201364=CARTESIAN_POINT('Ctrl Pts',(-24.0779139079264,5.09476976342616,
0.));
#201365=CARTESIAN_POINT('Ctrl Pts',(-24.0779139079264,5.09476976342616,
12.));
#201366=CARTESIAN_POINT('Ctrl Pts',(-24.0975261288444,5.10881967883124,
0.));
#201367=CARTESIAN_POINT('Ctrl Pts',(-24.0975261288444,5.10881967883124,
12.));
#201368=CARTESIAN_POINT('Ctrl Pts',(-24.117173659394,5.12296753853857,0.));
#201369=CARTESIAN_POINT('Ctrl Pts',(-24.117173659394,5.12296753853857,12.));
#201370=CARTESIAN_POINT('Ctrl Pts',(-24.1368558702443,5.13721325845745,
0.));
#201371=CARTESIAN_POINT('Ctrl Pts',(-24.1368558702443,5.13721325845745,
12.));
#201372=CARTESIAN_POINT('Ctrl Pts',(-24.1565721375971,5.15155675390079,
0.));
#201373=CARTESIAN_POINT('Ctrl Pts',(-24.1565721375971,5.15155675390079,
12.));
#201374=CARTESIAN_POINT('Ctrl Pts',(-24.1763218431344,5.16599793957985,
0.));
#201375=CARTESIAN_POINT('Ctrl Pts',(-24.1763218431344,5.16599793957985,
12.));
#201376=CARTESIAN_POINT('Ctrl Pts',(-24.1961043738756,5.18053672961398,
0.));
#201377=CARTESIAN_POINT('Ctrl Pts',(-24.1961043738756,5.18053672961398,
12.));
#201378=CARTESIAN_POINT('Ctrl Pts',(-24.2159191220171,5.19517303753647,
0.));
#201379=CARTESIAN_POINT('Ctrl Pts',(-24.2159191220171,5.19517303753647,
12.));
#201380=CARTESIAN_POINT('Ctrl Pts',(-24.2357654847766,5.20990677629176,
0.));
#201381=CARTESIAN_POINT('Ctrl Pts',(-24.2357654847766,5.20990677629176,
12.));
#201382=CARTESIAN_POINT('Ctrl Pts',(-24.2556428642294,5.22473785822442,
0.));
#201383=CARTESIAN_POINT('Ctrl Pts',(-24.2556428642294,5.22473785822442,
12.));
#201384=CARTESIAN_POINT('Ctrl Pts',(-24.2755506671525,5.23966619506289,
0.));
#201385=CARTESIAN_POINT('Ctrl Pts',(-24.2755506671525,5.23966619506289,
12.));
#201386=CARTESIAN_POINT('Ctrl Pts',(-24.2954883048447,5.25469169788856,
0.));
#201387=CARTESIAN_POINT('Ctrl Pts',(-24.2954883048447,5.25469169788856,
12.));
#201388=CARTESIAN_POINT('Ctrl Pts',(-24.3154551932221,5.26981427718798,
0.));
#201389=CARTESIAN_POINT('Ctrl Pts',(-24.3154551932221,5.26981427718798,
12.));
#201390=CARTESIAN_POINT('Ctrl Pts',(-24.3354507529414,5.28503384290648,
0.));
#201391=CARTESIAN_POINT('Ctrl Pts',(-24.3354507529414,5.28503384290648,
12.));
#201392=CARTESIAN_POINT('Ctrl Pts',(-24.3554744095075,5.30035030449063,
0.));
#201393=CARTESIAN_POINT('Ctrl Pts',(-24.3554744095075,5.30035030449063,
12.));
#201394=CARTESIAN_POINT('Ctrl Pts',(-24.3755255933917,5.31576357092526,
0.));
#201395=CARTESIAN_POINT('Ctrl Pts',(-24.3755255933917,5.31576357092526,
12.));
#201396=CARTESIAN_POINT('Ctrl Pts',(-24.3956037401293,5.33127355076033,
0.));
#201397=CARTESIAN_POINT('Ctrl Pts',(-24.3956037401293,5.33127355076033,
12.));
#201398=CARTESIAN_POINT('Ctrl Pts',(-24.4157082904614,5.34688015213537,
0.));
#201399=CARTESIAN_POINT('Ctrl Pts',(-24.4157082904614,5.34688015213537,
12.));
#201400=CARTESIAN_POINT('Ctrl Pts',(-24.435838689915,5.36258328273627,0.));
#201401=CARTESIAN_POINT('Ctrl Pts',(-24.435838689915,5.36258328273627,12.));
#201402=CARTESIAN_POINT('Ctrl Pts',(-24.4559943883157,5.37838284973695,
0.));
#201403=CARTESIAN_POINT('Ctrl Pts',(-24.4559943883157,5.37838284973695,
12.));
#201404=CARTESIAN_POINT('Ctrl Pts',(-24.4761748393321,5.39427875973824,
0.));
#201405=CARTESIAN_POINT('Ctrl Pts',(-24.4761748393321,5.39427875973824,
12.));
#201406=CARTESIAN_POINT('Ctrl Pts',(-24.4963794999831,5.41027091869241,
0.));
#201407=CARTESIAN_POINT('Ctrl Pts',(-24.4963794999831,5.41027091869241,
12.));
#201408=CARTESIAN_POINT('Ctrl Pts',(-24.5166078302108,5.42635923183419,
0.));
#201409=CARTESIAN_POINT('Ctrl Pts',(-24.5166078302108,5.42635923183419,
12.));
#201410=CARTESIAN_POINT('Ctrl Pts',(-24.5368592922863,5.4425436035688,0.));
#201411=CARTESIAN_POINT('Ctrl Pts',(-24.5368592922863,5.4425436035688,12.));
#201412=CARTESIAN_POINT('Ctrl Pts',(-24.5571333514842,5.45882393762261,
0.));
#201413=CARTESIAN_POINT('Ctrl Pts',(-24.5571333514842,5.45882393762261,
12.));
#201414=CARTESIAN_POINT('Ctrl Pts',(-24.5774294770329,5.47520013724419,
0.));
#201415=CARTESIAN_POINT('Ctrl Pts',(-24.5774294770329,5.47520013724419,
12.));
#201416=CARTESIAN_POINT('Ctrl Pts',(-24.5977471429364,5.49167210537246,
0.));
#201417=CARTESIAN_POINT('Ctrl Pts',(-24.5977471429364,5.49167210537246,
12.));
#201418=CARTESIAN_POINT('Ctrl Pts',(-24.6180858289179,5.50823974481962,
0.));
#201419=CARTESIAN_POINT('Ctrl Pts',(-24.6180858289179,5.50823974481962,
12.));
#201420=CARTESIAN_POINT('Ctrl Pts',(-24.6384450211467,5.52490295840991,
0.));
#201421=CARTESIAN_POINT('Ctrl Pts',(-24.6384450211467,5.52490295840991,
12.));
#201422=CARTESIAN_POINT('Ctrl Pts',(-24.6588242134738,5.54166164919583,
0.));
#201423=CARTESIAN_POINT('Ctrl Pts',(-24.6588242134738,5.54166164919583,
12.));
#201424=CARTESIAN_POINT('Ctrl Pts',(-24.6792229061794,5.55851572025376,
0.));
#201425=CARTESIAN_POINT('Ctrl Pts',(-24.6792229061794,5.55851572025376,
12.));
#201426=CARTESIAN_POINT('Ctrl Pts',(-24.6996406035517,5.57546507427754,
0.));
#201427=CARTESIAN_POINT('Ctrl Pts',(-24.6996406035517,5.57546507427754,
12.));
#201428=CARTESIAN_POINT('Ctrl Pts',(-24.7200768119088,5.59250961323987,
0.));
#201429=CARTESIAN_POINT('Ctrl Pts',(-24.7200768119088,5.59250961323987,
12.));
#201430=CARTESIAN_POINT('Ctrl Pts',(-24.7405310372739,5.60964923798491,
0.));
#201431=CARTESIAN_POINT('Ctrl Pts',(-24.7405310372739,5.60964923798491,
12.));
#201432=CARTESIAN_POINT('Ctrl Pts',(-24.7610027835697,5.62688384790923,
0.));
#201433=CARTESIAN_POINT('Ctrl Pts',(-24.7610027835697,5.62688384790923,
12.));
#201434=CARTESIAN_POINT('Ctrl Pts',(-24.781491549672,5.6442133404226,0.));
#201435=CARTESIAN_POINT('Ctrl Pts',(-24.781491549672,5.6442133404226,12.));
#201436=CARTESIAN_POINT('Ctrl Pts',(-24.8019968304605,5.66163761114921,
0.));
#201437=CARTESIAN_POINT('Ctrl Pts',(-24.8019968304605,5.66163761114921,
12.));
#201438=CARTESIAN_POINT('Ctrl Pts',(-24.8225181223845,5.67915655496542,
0.));
#201439=CARTESIAN_POINT('Ctrl Pts',(-24.8225181223845,5.67915655496542,
12.));
#201440=CARTESIAN_POINT('Ctrl Pts',(-24.8430549277621,5.69677006679444,
0.));
#201441=CARTESIAN_POINT('Ctrl Pts',(-24.8430549277621,5.69677006679444,
12.));
#201442=CARTESIAN_POINT('Ctrl Pts',(-24.8636067597669,5.71447804252027,
0.));
#201443=CARTESIAN_POINT('Ctrl Pts',(-24.8636067597669,5.71447804252027,
12.));
#201444=CARTESIAN_POINT('Ctrl Pts',(-24.884173146722,5.73228037976926,0.));
#201445=CARTESIAN_POINT('Ctrl Pts',(-24.884173146722,5.73228037976926,12.));
#201446=CARTESIAN_POINT('Ctrl Pts',(-24.904753637648,5.75017697890804,0.));
#201447=CARTESIAN_POINT('Ctrl Pts',(-24.904753637648,5.75017697890804,12.));
#201448=CARTESIAN_POINT('Ctrl Pts',(-24.9253478043656,5.76816774342219,
0.));
#201449=CARTESIAN_POINT('Ctrl Pts',(-24.9253478043656,5.76816774342219,
12.));
#201450=CARTESIAN_POINT('Ctrl Pts',(-24.945955229334,5.78625257775681,0.));
#201451=CARTESIAN_POINT('Ctrl Pts',(-24.945955229334,5.78625257775681,12.));
#201452=CARTESIAN_POINT('Ctrl Pts',(-24.9665754954496,5.80443138549726,
0.));
#201453=CARTESIAN_POINT('Ctrl Pts',(-24.9665754954496,5.80443138549726,
12.));
#201454=CARTESIAN_POINT('Ctrl Pts',(-24.9872081752734,5.82270406744198,
0.));
#201455=CARTESIAN_POINT('Ctrl Pts',(-24.9872081752734,5.82270406744198,
12.));
#201456=CARTESIAN_POINT('Ctrl Pts',(-25.0078528200564,5.84107051963071,
0.));
#201457=CARTESIAN_POINT('Ctrl Pts',(-25.0078528200564,5.84107051963071,
12.));
#201458=CARTESIAN_POINT('Ctrl Pts',(-25.0285089498899,5.85953063156826,
0.));
#201459=CARTESIAN_POINT('Ctrl Pts',(-25.0285089498899,5.85953063156826,
12.));
#201460=CARTESIAN_POINT('Ctrl Pts',(-25.0491760405911,5.87808428385365,
0.));
#201461=CARTESIAN_POINT('Ctrl Pts',(-25.0491760405911,5.87808428385365,
12.));
#201462=CARTESIAN_POINT('Ctrl Pts',(-25.0698535426514,5.89673135155514,
0.));
#201463=CARTESIAN_POINT('Ctrl Pts',(-25.0698535426514,5.89673135155514,
12.));
#201464=CARTESIAN_POINT('Ctrl Pts',(-25.0905409050773,5.91547170844447,
0.));
#201465=CARTESIAN_POINT('Ctrl Pts',(-25.0905409050773,5.91547170844447,
12.));
#201466=CARTESIAN_POINT('Ctrl Pts',(-25.1112375971106,5.93430523086834,
0.));
#201467=CARTESIAN_POINT('Ctrl Pts',(-25.1112375971106,5.93430523086834,
12.));
#201468=CARTESIAN_POINT('Ctrl Pts',(-25.1319431317237,5.95323180187378,
0.));
#201469=CARTESIAN_POINT('Ctrl Pts',(-25.1319431317237,5.95323180187378,
12.));
#201470=CARTESIAN_POINT('Ctrl Pts',(-25.1526570863092,5.97225131495616,
0.));
#201471=CARTESIAN_POINT('Ctrl Pts',(-25.1526570863092,5.97225131495616,
12.));
#201472=CARTESIAN_POINT('Ctrl Pts',(-25.1733791296259,5.99136367859754,
0.));
#201473=CARTESIAN_POINT('Ctrl Pts',(-25.1733791296259,5.99136367859754,
12.));
#201474=CARTESIAN_POINT('Ctrl Pts',(-25.1941090269819,6.01056881804612,
0.));
#201475=CARTESIAN_POINT('Ctrl Pts',(-25.1941090269819,6.01056881804612,
12.));
#201476=CARTESIAN_POINT('Ctrl Pts',(-25.21484662016,6.02986667389996,0.));
#201477=CARTESIAN_POINT('Ctrl Pts',(-25.21484662016,6.02986667389996,12.));
#201478=CARTESIAN_POINT('Ctrl Pts',(-25.2355918139032,6.04925720151218,
0.));
#201479=CARTESIAN_POINT('Ctrl Pts',(-25.2355918139032,6.04925720151218,
12.));
#201480=CARTESIAN_POINT('Ctrl Pts',(-25.2521940105705,6.06484373634546,
0.));
#201481=CARTESIAN_POINT('Ctrl Pts',(-25.2521940105705,6.06484373634546,
12.));
#201482=CARTESIAN_POINT('Ctrl Pts',(-25.2646490489923,6.0765753178749,0.));
#201483=CARTESIAN_POINT('Ctrl Pts',(-25.2646490489923,6.0765753178749,12.));
#201484=CARTESIAN_POINT('Ctrl Pts',(-25.2729539149517,6.08441489609793,
0.));
#201485=CARTESIAN_POINT('Ctrl Pts',(-25.2729539149517,6.08441489609793,
12.));
#201486=CARTESIAN_POINT('Ctrl Pts',(-25.2771067246846,6.08833931617699,
0.));
#201487=CARTESIAN_POINT('Ctrl Pts',(-25.2771067246846,6.08833931617699,
12.));
#201488=CARTESIAN_POINT('',(-25.2771067246846,6.08833931617699,0.));
#201489=CARTESIAN_POINT('Ctrl Pts',(-22.1738711152697,4.11585220600461,
0.));
#201490=CARTESIAN_POINT('Ctrl Pts',(-22.173877682324,4.11585194677442,0.));
#201491=CARTESIAN_POINT('Ctrl Pts',(-22.1739341411687,4.11586035878287,
0.));
#201492=CARTESIAN_POINT('Ctrl Pts',(-22.1741488021234,4.11589976826166,
0.));
#201493=CARTESIAN_POINT('Ctrl Pts',(-22.1746949858775,4.11600589882845,
0.));
#201494=CARTESIAN_POINT('Ctrl Pts',(-22.1758088296598,4.11622797217068,
0.));
#201495=CARTESIAN_POINT('Ctrl Pts',(-22.177347426894,4.11653973150518,0.));
#201496=CARTESIAN_POINT('Ctrl Pts',(-22.179297473024,4.11694173195003,0.));
#201497=CARTESIAN_POINT('Ctrl Pts',(-22.1816414985788,4.11743469691756,
0.));
#201498=CARTESIAN_POINT('Ctrl Pts',(-22.1843613164855,4.11801938107479,
0.));
#201499=CARTESIAN_POINT('Ctrl Pts',(-22.1874419861496,4.11869641271773,
0.));
#201500=CARTESIAN_POINT('Ctrl Pts',(-22.1908725908525,4.11946626228636,
0.));
#201501=CARTESIAN_POINT('Ctrl Pts',(-22.1946440958098,4.12032932637736,
0.));
#201502=CARTESIAN_POINT('Ctrl Pts',(-22.1987479618246,4.12128598183522,
0.));
#201503=CARTESIAN_POINT('Ctrl Pts',(-22.2031746532106,4.12233664408227,
0.));
#201504=CARTESIAN_POINT('Ctrl Pts',(-22.2079143941719,4.12348173702023,
0.));
#201505=CARTESIAN_POINT('Ctrl Pts',(-22.2129576146671,4.12472167516607,
0.));
#201506=CARTESIAN_POINT('Ctrl Pts',(-22.2182956401341,4.12605683613307,
0.));
#201507=CARTESIAN_POINT('Ctrl Pts',(-22.2239207458781,4.12748755830104,
0.));
#201508=CARTESIAN_POINT('Ctrl Pts',(-22.2298258043947,4.12901415463379,
0.));
#201509=CARTESIAN_POINT('Ctrl Pts',(-22.2360040565533,4.13063692157498,
0.));
#201510=CARTESIAN_POINT('Ctrl Pts',(-22.2424488153523,4.1323561506016,0.));
#201511=CARTESIAN_POINT('Ctrl Pts',(-22.249153531779,4.1341721255881,0.));
#201512=CARTESIAN_POINT('Ctrl Pts',(-22.2561118708421,4.13608511977225,
0.));
#201513=CARTESIAN_POINT('Ctrl Pts',(-22.2633177913972,4.13809539255421,
0.));
#201514=CARTESIAN_POINT('Ctrl Pts',(-22.2707656042457,4.14020318715991,
0.));
#201515=CARTESIAN_POINT('Ctrl Pts',(-22.2784499072027,4.14240873321984,
0.));
#201516=CARTESIAN_POINT('Ctrl Pts',(-22.2863655389166,4.14471224859295,
0.));
#201517=CARTESIAN_POINT('Ctrl Pts',(-22.2945075198467,4.14711394168556,
0.));
#201518=CARTESIAN_POINT('Ctrl Pts',(-22.3028710166933,4.14961401285522,
0.));
#201519=CARTESIAN_POINT('Ctrl Pts',(-22.3114513545185,4.1522126539699,0.));
#201520=CARTESIAN_POINT('Ctrl Pts',(-22.3202440186979,4.15491004835281,
0.));
#201521=CARTESIAN_POINT('Ctrl Pts',(-22.3292446628959,4.15770637047889,
0.));
#201522=CARTESIAN_POINT('Ctrl Pts',(-22.3384491078602,4.16060178604164,
0.));
#201523=CARTESIAN_POINT('Ctrl Pts',(-22.3478533253889,4.16359645263187,
0.));
#201524=CARTESIAN_POINT('Ctrl Pts',(-22.3574534257396,4.166690520266,0.));
#201525=CARTESIAN_POINT('Ctrl Pts',(-22.36724564276,4.16988413199457,0.));
#201526=CARTESIAN_POINT('Ctrl Pts',(-22.3772263228617,4.17317742436145,
0.));
#201527=CARTESIAN_POINT('Ctrl Pts',(-22.3873919231334,4.17657052752825,
0.));
#201528=CARTESIAN_POINT('Ctrl Pts',(-22.3977390078075,4.18006356544882,
0.));
#201529=CARTESIAN_POINT('Ctrl Pts',(-22.4082642454453,4.1836566560085,0.));
#201530=CARTESIAN_POINT('Ctrl Pts',(-22.4189644056115,4.1873499111772,0.));
#201531=CARTESIAN_POINT('Ctrl Pts',(-22.4298363535421,4.19114343726941,
0.));
#201532=CARTESIAN_POINT('Ctrl Pts',(-22.4408770448917,4.1950373351886,0.));
#201533=CARTESIAN_POINT('Ctrl Pts',(-22.4520835205419,4.19903170066354,
0.));
#201534=CARTESIAN_POINT('Ctrl Pts',(-22.4634529011433,4.2031266244817,0.));
#201535=CARTESIAN_POINT('Ctrl Pts',(-22.4749823839915,4.20732219265648,
0.));
#201536=CARTESIAN_POINT('Ctrl Pts',(-22.4866692403147,4.21161848657428,
0.));
#201537=CARTESIAN_POINT('Ctrl Pts',(-22.4985108124229,4.21601558313908,
0.));
#201538=CARTESIAN_POINT('Ctrl Pts',(-22.5105045108882,4.22051355490196,
0.));
#201539=CARTESIAN_POINT('Ctrl Pts',(-22.5226478117885,4.2251124702004,0.));
#201540=CARTESIAN_POINT('Ctrl Pts',(-22.5349382540587,4.22981239330731,
0.));
#201541=CARTESIAN_POINT('Ctrl Pts',(-22.5473734368086,4.23461338456713,
0.));
#201542=CARTESIAN_POINT('Ctrl Pts',(-22.559951016643,4.23951550052526,0.));
#201543=CARTESIAN_POINT('Ctrl Pts',(-22.5726687049922,4.24451879404858,
0.));
#201544=CARTESIAN_POINT('Ctrl Pts',(-22.5855242662479,4.24962331444184,
0.));
#201545=CARTESIAN_POINT('Ctrl Pts',(-22.5985155158637,4.25482910755485,
0.));
#201546=CARTESIAN_POINT('Ctrl Pts',(-22.611640318482,4.26013621588303,0.));
#201547=CARTESIAN_POINT('Ctrl Pts',(-22.6248965859975,4.26554467865571,
0.));
#201548=CARTESIAN_POINT('Ctrl Pts',(-22.6382822758171,4.27105453192999,
0.));
#201549=CARTESIAN_POINT('Ctrl Pts',(-22.6517953893303,4.27666580869117,
0.));
#201550=CARTESIAN_POINT('Ctrl Pts',(-22.665433970311,4.28237853894059,0.));
#201551=CARTESIAN_POINT('Ctrl Pts',(-22.6791961033537,4.28819274977766,
0.));
#201552=CARTESIAN_POINT('Ctrl Pts',(-22.6930799122545,4.29410846547061,
0.));
#201553=CARTESIAN_POINT('Ctrl Pts',(-22.707083558756,4.30012570754066,0.));
#201554=CARTESIAN_POINT('Ctrl Pts',(-22.7212052413384,4.30624449484074,
0.));
#201555=CARTESIAN_POINT('Ctrl Pts',(-22.7354431939927,4.3124648436255,0.));
#201556=CARTESIAN_POINT('Ctrl Pts',(-22.7497956849852,4.3187867676123,0.));
#201557=CARTESIAN_POINT('Ctrl Pts',(-22.764261015648,4.32521027803747,0.));
#201558=CARTESIAN_POINT('Ctrl Pts',(-22.7788375194081,4.33173538373182,
0.));
#201559=CARTESIAN_POINT('Ctrl Pts',(-22.7935235607807,4.33836209118442,
0.));
#201560=CARTESIAN_POINT('Ctrl Pts',(-22.808317534379,4.34509040460065,0.));
#201561=CARTESIAN_POINT('Ctrl Pts',(-22.8232178638873,4.35192032594801,
0.));
#201562=CARTESIAN_POINT('Ctrl Pts',(-22.838223001118,4.35885185500559,0.));
#201563=CARTESIAN_POINT('Ctrl Pts',(-22.8533314252419,4.36588498943009,
0.));
#201564=CARTESIAN_POINT('Ctrl Pts',(-22.8685416419725,4.37301972480752,
0.));
#201565=CARTESIAN_POINT('Ctrl Pts',(-22.8838521827702,4.38025605470089,
0.));
#201566=CARTESIAN_POINT('Ctrl Pts',(-22.8992616040108,4.38759397068391,
0.));
#201567=CARTESIAN_POINT('Ctrl Pts',(-22.9147684862425,4.39503346238454,
0.));
#201568=CARTESIAN_POINT('Ctrl Pts',(-22.9303714335549,4.40257451754307,
0.));
#201569=CARTESIAN_POINT('Ctrl Pts',(-22.9460690729093,4.41021712205547,
0.));
#201570=CARTESIAN_POINT('Ctrl Pts',(-22.9618600534866,4.41796126001309,
0.));
#201571=CARTESIAN_POINT('Ctrl Pts',(-22.9777430460021,4.42580691372771,
0.));
#201572=CARTESIAN_POINT('Ctrl Pts',(-22.9937167421009,4.43375406376904,
0.));
#201573=CARTESIAN_POINT('Ctrl Pts',(-23.0097798538399,4.44180268901666,
0.));
#201574=CARTESIAN_POINT('Ctrl Pts',(-23.0259311131395,4.44995276669698,
0.));
#201575=CARTESIAN_POINT('Ctrl Pts',(-23.0421692712466,4.45820427241676,
0.));
#201576=CARTESIAN_POINT('Ctrl Pts',(-23.0584930981723,4.46655718018205,
0.));
#201577=CARTESIAN_POINT('Ctrl Pts',(-23.0749013821868,4.47501146242821,
0.));
#201578=CARTESIAN_POINT('Ctrl Pts',(-23.0913929293909,4.48356709006756,
0.));
#201579=CARTESIAN_POINT('Ctrl Pts',(-23.1079665632629,4.49222403252201,
0.));
#201580=CARTESIAN_POINT('Ctrl Pts',(-23.1246211242117,4.50098225775178,
0.));
#201581=CARTESIAN_POINT('Ctrl Pts',(-23.1413554691136,4.50984173227087,
0.));
#201582=CARTESIAN_POINT('Ctrl Pts',(-23.1581684708778,4.51880242116785,
0.));
#201583=CARTESIAN_POINT('Ctrl Pts',(-23.1750590180923,4.52786428815047,
0.));
#201584=CARTESIAN_POINT('Ctrl Pts',(-23.1920260146474,4.53702729557585,
0.));
#201585=CARTESIAN_POINT('Ctrl Pts',(-23.2090683793627,4.54629140447542,
0.));
#201586=CARTESIAN_POINT('Ctrl Pts',(-23.2261850456055,4.55565657456956,
0.));
#201587=CARTESIAN_POINT('Ctrl Pts',(-23.2433749609117,4.5651227642781,0.));
#201588=CARTESIAN_POINT('Ctrl Pts',(-23.2606370866853,4.5746899307607,0.));
#201589=CARTESIAN_POINT('Ctrl Pts',(-23.2779703978868,4.58435802994674,
0.));
#201590=CARTESIAN_POINT('Ctrl Pts',(-23.295373882719,4.59412701655749,0.));
#201591=CARTESIAN_POINT('Ctrl Pts',(-23.3128465423119,4.60399684412174,
0.));
#201592=CARTESIAN_POINT('Ctrl Pts',(-23.3303873903947,4.61396746497848,
0.));
#201593=CARTESIAN_POINT('Ctrl Pts',(-23.3479954530281,4.62403883030823,
0.));
#201594=CARTESIAN_POINT('Ctrl Pts',(-23.3656697683496,4.63421089016554,
0.));
#201595=CARTESIAN_POINT('Ctrl Pts',(-23.383409386307,4.64448359349935,0.));
#201596=CARTESIAN_POINT('Ctrl Pts',(-23.4012133683957,4.65485688816921,
0.));
#201597=CARTESIAN_POINT('Ctrl Pts',(-23.4190807873798,4.66533072094663,
0.));
#201598=CARTESIAN_POINT('Ctrl Pts',(-23.4370107270444,4.6759050375305,0.));
#201599=CARTESIAN_POINT('Ctrl Pts',(-23.4550022819853,4.68657978258297,
0.));
#201600=CARTESIAN_POINT('Ctrl Pts',(-23.4730545573849,4.69735489975023,
0.));
#201601=CARTESIAN_POINT('Ctrl Pts',(-23.491166668789,4.7082303316782,0.));
#201602=CARTESIAN_POINT('Ctrl Pts',(-23.5093377418784,4.71920602001904,
0.));
#201603=CARTESIAN_POINT('Ctrl Pts',(-23.5275669122378,4.73028190543031,
0.));
#201604=CARTESIAN_POINT('Ctrl Pts',(-23.5458533251715,4.74145792760698,
0.));
#201605=CARTESIAN_POINT('Ctrl Pts',(-23.564196135517,4.75273402530615,0.));
#201606=CARTESIAN_POINT('Ctrl Pts',(-23.5825945074535,4.7641101363625,0.));
#201607=CARTESIAN_POINT('Ctrl Pts',(-23.6010476143099,4.77558619769875,
0.));
#201608=CARTESIAN_POINT('Ctrl Pts',(-23.6195546383625,4.78716214532104,
0.));
#201609=CARTESIAN_POINT('Ctrl Pts',(-23.6381147706581,4.79883791433229,
0.));
#201610=CARTESIAN_POINT('Ctrl Pts',(-23.6567272108631,4.81061343896442,
0.));
#201611=CARTESIAN_POINT('Ctrl Pts',(-23.6753911671023,4.82248865259569,
0.));
#201612=CARTESIAN_POINT('Ctrl Pts',(-23.6941058557971,4.83446348776267,
0.));
#201613=CARTESIAN_POINT('Ctrl Pts',(-23.7128705015014,4.84653787616422,
0.));
#201614=CARTESIAN_POINT('Ctrl Pts',(-23.7316843367308,4.85871174865491,
0.));
#201615=CARTESIAN_POINT('Ctrl Pts',(-23.7505466018239,4.87098503527142,
0.));
#201616=CARTESIAN_POINT('Ctrl Pts',(-23.7694565448044,4.88335766525565,
0.));
#201617=CARTESIAN_POINT('Ctrl Pts',(-23.7884134212381,4.89582956706771,
0.));
#201618=CARTESIAN_POINT('Ctrl Pts',(-23.8074164940897,4.90840066839346,
0.));
#201619=CARTESIAN_POINT('Ctrl Pts',(-23.8264650335721,4.92107089613976,
0.));
#201620=CARTESIAN_POINT('Ctrl Pts',(-23.8455583170062,4.93384017643441,
0.));
#201621=CARTESIAN_POINT('Ctrl Pts',(-23.8646956287172,4.94670843465868,
0.));
#201622=CARTESIAN_POINT('Ctrl Pts',(-23.883876259922,4.95967559546565,0.));
#201623=CARTESIAN_POINT('Ctrl Pts',(-23.9030995086164,4.97274158279228,
0.));
#201624=CARTESIAN_POINT('Ctrl Pts',(-23.9223646794591,4.98590631986532,
0.));
#201625=CARTESIAN_POINT('Ctrl Pts',(-23.9416710836529,4.99916972919309,
0.));
#201626=CARTESIAN_POINT('Ctrl Pts',(-23.9610180388271,5.01253173257458,
0.));
#201627=CARTESIAN_POINT('Ctrl Pts',(-23.9804048689228,5.02599225112461,
0.));
#201628=CARTESIAN_POINT('Ctrl Pts',(-23.9998309040747,5.03955120528527,
0.));
#201629=CARTESIAN_POINT('Ctrl Pts',(-24.0192954804896,5.05320851483068,
0.));
#201630=CARTESIAN_POINT('Ctrl Pts',(-24.0387979403268,5.06696409886639,
0.));
#201631=CARTESIAN_POINT('Ctrl Pts',(-24.0583376315636,5.0808178758127,0.));
#201632=CARTESIAN_POINT('Ctrl Pts',(-24.0779139079264,5.09476976342616,
0.));
#201633=CARTESIAN_POINT('Ctrl Pts',(-24.0975261288444,5.10881967883124,
0.));
#201634=CARTESIAN_POINT('Ctrl Pts',(-24.117173659394,5.12296753853857,0.));
#201635=CARTESIAN_POINT('Ctrl Pts',(-24.1368558702443,5.13721325845745,
0.));
#201636=CARTESIAN_POINT('Ctrl Pts',(-24.1565721375971,5.15155675390079,
0.));
#201637=CARTESIAN_POINT('Ctrl Pts',(-24.1763218431344,5.16599793957985,
0.));
#201638=CARTESIAN_POINT('Ctrl Pts',(-24.1961043738756,5.18053672961398,
0.));
#201639=CARTESIAN_POINT('Ctrl Pts',(-24.2159191220171,5.19517303753647,
0.));
#201640=CARTESIAN_POINT('Ctrl Pts',(-24.2357654847766,5.20990677629176,
0.));
#201641=CARTESIAN_POINT('Ctrl Pts',(-24.2556428642294,5.22473785822442,
0.));
#201642=CARTESIAN_POINT('Ctrl Pts',(-24.2755506671525,5.23966619506289,
0.));
#201643=CARTESIAN_POINT('Ctrl Pts',(-24.2954883048447,5.25469169788856,
0.));
#201644=CARTESIAN_POINT('Ctrl Pts',(-24.3154551932221,5.26981427718798,
0.));
#201645=CARTESIAN_POINT('Ctrl Pts',(-24.3354507529414,5.28503384290648,
0.));
#201646=CARTESIAN_POINT('Ctrl Pts',(-24.3554744095075,5.30035030449063,
0.));
#201647=CARTESIAN_POINT('Ctrl Pts',(-24.3755255933917,5.31576357092526,
0.));
#201648=CARTESIAN_POINT('Ctrl Pts',(-24.3956037401293,5.33127355076033,
0.));
#201649=CARTESIAN_POINT('Ctrl Pts',(-24.4157082904614,5.34688015213537,
0.));
#201650=CARTESIAN_POINT('Ctrl Pts',(-24.435838689915,5.36258328273627,0.));
#201651=CARTESIAN_POINT('Ctrl Pts',(-24.4559943883157,5.37838284973695,
0.));
#201652=CARTESIAN_POINT('Ctrl Pts',(-24.4761748393321,5.39427875973824,
0.));
#201653=CARTESIAN_POINT('Ctrl Pts',(-24.4963794999831,5.41027091869241,
0.));
#201654=CARTESIAN_POINT('Ctrl Pts',(-24.5166078302108,5.42635923183419,
0.));
#201655=CARTESIAN_POINT('Ctrl Pts',(-24.5368592922863,5.4425436035688,0.));
#201656=CARTESIAN_POINT('Ctrl Pts',(-24.5571333514842,5.45882393762261,
0.));
#201657=CARTESIAN_POINT('Ctrl Pts',(-24.5774294770329,5.47520013724419,
0.));
#201658=CARTESIAN_POINT('Ctrl Pts',(-24.5977471429364,5.49167210537246,
0.));
#201659=CARTESIAN_POINT('Ctrl Pts',(-24.6180858289179,5.50823974481962,
0.));
#201660=CARTESIAN_POINT('Ctrl Pts',(-24.6384450211467,5.52490295840991,
0.));
#201661=CARTESIAN_POINT('Ctrl Pts',(-24.6588242134738,5.54166164919583,
0.));
#201662=CARTESIAN_POINT('Ctrl Pts',(-24.6792229061794,5.55851572025376,
0.));
#201663=CARTESIAN_POINT('Ctrl Pts',(-24.6996406035517,5.57546507427754,
0.));
#201664=CARTESIAN_POINT('Ctrl Pts',(-24.7200768119088,5.59250961323987,
0.));
#201665=CARTESIAN_POINT('Ctrl Pts',(-24.7405310372739,5.60964923798491,
0.));
#201666=CARTESIAN_POINT('Ctrl Pts',(-24.7610027835697,5.62688384790923,
0.));
#201667=CARTESIAN_POINT('Ctrl Pts',(-24.781491549672,5.6442133404226,0.));
#201668=CARTESIAN_POINT('Ctrl Pts',(-24.8019968304605,5.66163761114921,
0.));
#201669=CARTESIAN_POINT('Ctrl Pts',(-24.8225181223845,5.67915655496542,
0.));
#201670=CARTESIAN_POINT('Ctrl Pts',(-24.8430549277621,5.69677006679444,
0.));
#201671=CARTESIAN_POINT('Ctrl Pts',(-24.8636067597669,5.71447804252027,
0.));
#201672=CARTESIAN_POINT('Ctrl Pts',(-24.884173146722,5.73228037976926,0.));
#201673=CARTESIAN_POINT('Ctrl Pts',(-24.904753637648,5.75017697890804,0.));
#201674=CARTESIAN_POINT('Ctrl Pts',(-24.9253478043656,5.76816774342219,
0.));
#201675=CARTESIAN_POINT('Ctrl Pts',(-24.945955229334,5.78625257775681,0.));
#201676=CARTESIAN_POINT('Ctrl Pts',(-24.9665754954496,5.80443138549726,
0.));
#201677=CARTESIAN_POINT('Ctrl Pts',(-24.9872081752734,5.82270406744198,
0.));
#201678=CARTESIAN_POINT('Ctrl Pts',(-25.0078528200564,5.84107051963071,
0.));
#201679=CARTESIAN_POINT('Ctrl Pts',(-25.0285089498899,5.85953063156826,
0.));
#201680=CARTESIAN_POINT('Ctrl Pts',(-25.0491760405911,5.87808428385365,
0.));
#201681=CARTESIAN_POINT('Ctrl Pts',(-25.0698535426514,5.89673135155514,
0.));
#201682=CARTESIAN_POINT('Ctrl Pts',(-25.0905409050773,5.91547170844447,
0.));
#201683=CARTESIAN_POINT('Ctrl Pts',(-25.1112375971106,5.93430523086834,
0.));
#201684=CARTESIAN_POINT('Ctrl Pts',(-25.1319431317237,5.95323180187378,
0.));
#201685=CARTESIAN_POINT('Ctrl Pts',(-25.1526570863092,5.97225131495616,
0.));
#201686=CARTESIAN_POINT('Ctrl Pts',(-25.1733791296259,5.99136367859754,
0.));
#201687=CARTESIAN_POINT('Ctrl Pts',(-25.1941090269819,6.01056881804612,
0.));
#201688=CARTESIAN_POINT('Ctrl Pts',(-25.21484662016,6.02986667389996,0.));
#201689=CARTESIAN_POINT('Ctrl Pts',(-25.2355918139032,6.04925720151218,
0.));
#201690=CARTESIAN_POINT('Ctrl Pts',(-25.2521940105705,6.06484373634546,
0.));
#201691=CARTESIAN_POINT('Ctrl Pts',(-25.2646490489923,6.0765753178749,0.));
#201692=CARTESIAN_POINT('Ctrl Pts',(-25.2729539149517,6.08441489609793,
0.));
#201693=CARTESIAN_POINT('Ctrl Pts',(-25.2771067246846,6.08833931617699,
0.));
#201694=CARTESIAN_POINT('',(-25.2771067246846,6.08833931617699,0.));
#201695=CARTESIAN_POINT('Origin',(-19.4030938020118,9.26120677397565,0.));
#201696=CARTESIAN_POINT('',(-20.353053841303,9.71462809124917,0.));
#201697=CARTESIAN_POINT('',(-20.353053841303,9.71462809124917,0.));
#201698=CARTESIAN_POINT('',(-9.70154690100589,4.63060338698782,0.));
#201699=CARTESIAN_POINT('Ctrl Pts',(-24.9347862158358,7.36589684767345,
0.));
#201700=CARTESIAN_POINT('Ctrl Pts',(-24.9347862158358,7.36589684767345,
12.));
#201701=CARTESIAN_POINT('Ctrl Pts',(-24.9292275670674,7.36721909028843,
0.));
#201702=CARTESIAN_POINT('Ctrl Pts',(-24.9292275670674,7.36721909028843,
12.));
#201703=CARTESIAN_POINT('Ctrl Pts',(-24.9181155530543,7.3698559312009,0.));
#201704=CARTESIAN_POINT('Ctrl Pts',(-24.9181155530543,7.3698559312009,12.));
#201705=CARTESIAN_POINT('Ctrl Pts',(-24.901463382605,7.37378825961676,0.));
#201706=CARTESIAN_POINT('Ctrl Pts',(-24.901463382605,7.37378825961676,12.));
#201707=CARTESIAN_POINT('Ctrl Pts',(-24.8792921911115,7.3789854964027,0.));
#201708=CARTESIAN_POINT('Ctrl Pts',(-24.8792921911115,7.3789854964027,12.));
#201709=CARTESIAN_POINT('Ctrl Pts',(-24.8516310625176,7.38540558903621,
0.));
#201710=CARTESIAN_POINT('Ctrl Pts',(-24.8516310625176,7.38540558903621,
12.));
#201711=CARTESIAN_POINT('Ctrl Pts',(-24.8240228520893,7.39174922585808,
0.));
#201712=CARTESIAN_POINT('Ctrl Pts',(-24.8240228520893,7.39174922585808,
12.));
#201713=CARTESIAN_POINT('Ctrl Pts',(-24.7964676646431,7.39801641583013,
0.));
#201714=CARTESIAN_POINT('Ctrl Pts',(-24.7964676646431,7.39801641583013,
12.));
#201715=CARTESIAN_POINT('Ctrl Pts',(-24.7689656668983,7.40420718661603,
0.));
#201716=CARTESIAN_POINT('Ctrl Pts',(-24.7689656668983,7.40420718661603,
12.));
#201717=CARTESIAN_POINT('Ctrl Pts',(-24.7415170994784,7.41032159082382,
0.));
#201718=CARTESIAN_POINT('Ctrl Pts',(-24.7415170994784,7.41032159082382,
12.));
#201719=CARTESIAN_POINT('Ctrl Pts',(-24.7141222950051,7.41635971481674,
0.));
#201720=CARTESIAN_POINT('Ctrl Pts',(-24.7141222950051,7.41635971481674,
12.));
#201721=CARTESIAN_POINT('Ctrl Pts',(-24.6867816727192,7.42232167766265,
0.));
#201722=CARTESIAN_POINT('Ctrl Pts',(-24.6867816727192,7.42232167766265,
12.));
#201723=CARTESIAN_POINT('Ctrl Pts',(-24.6594957128756,7.42820762159126,
0.));
#201724=CARTESIAN_POINT('Ctrl Pts',(-24.6594957128756,7.42820762159126,
12.));
#201725=CARTESIAN_POINT('Ctrl Pts',(-24.6322649369517,7.43401770489524,
0.));
#201726=CARTESIAN_POINT('Ctrl Pts',(-24.6322649369517,7.43401770489524,
12.));
#201727=CARTESIAN_POINT('Ctrl Pts',(-24.6050898852368,7.43975209375504,
0.));
#201728=CARTESIAN_POINT('Ctrl Pts',(-24.6050898852368,7.43975209375504,
12.));
#201729=CARTESIAN_POINT('Ctrl Pts',(-24.577971096086,7.44541095473134,0.));
#201730=CARTESIAN_POINT('Ctrl Pts',(-24.577971096086,7.44541095473134,12.));
#201731=CARTESIAN_POINT('Ctrl Pts',(-24.5509090831559,7.4509944465116,0.));
#201732=CARTESIAN_POINT('Ctrl Pts',(-24.5509090831559,7.4509944465116,12.));
#201733=CARTESIAN_POINT('Ctrl Pts',(-24.5239043173072,7.45650271335862,
0.));
#201734=CARTESIAN_POINT('Ctrl Pts',(-24.5239043173072,7.45650271335862,
12.));
#201735=CARTESIAN_POINT('Ctrl Pts',(-24.4969572391483,7.46193588961463,
0.));
#201736=CARTESIAN_POINT('Ctrl Pts',(-24.4969572391483,7.46193588961463,
12.));
#201737=CARTESIAN_POINT('Ctrl Pts',(-24.4700682684524,7.46729410308786,
0.));
#201738=CARTESIAN_POINT('Ctrl Pts',(-24.4700682684524,7.46729410308786,
12.));
#201739=CARTESIAN_POINT('Ctrl Pts',(-24.443237814649,7.47257747883246,0.));
#201740=CARTESIAN_POINT('Ctrl Pts',(-24.443237814649,7.47257747883246,12.));
#201741=CARTESIAN_POINT('Ctrl Pts',(-24.4164662871163,7.47778614286565,
0.));
#201742=CARTESIAN_POINT('Ctrl Pts',(-24.4164662871163,7.47778614286565,
12.));
#201743=CARTESIAN_POINT('Ctrl Pts',(-24.3897541049254,7.48292022569301,
0.));
#201744=CARTESIAN_POINT('Ctrl Pts',(-24.3897541049254,7.48292022569301,
12.));
#201745=CARTESIAN_POINT('Ctrl Pts',(-24.3631017084524,7.48797986651908,
0.));
#201746=CARTESIAN_POINT('Ctrl Pts',(-24.3631017084524,7.48797986651908,
12.));
#201747=CARTESIAN_POINT('Ctrl Pts',(-24.3365095573685,7.4929652125242,0.));
#201748=CARTESIAN_POINT('Ctrl Pts',(-24.3365095573685,7.4929652125242,12.));
#201749=CARTESIAN_POINT('Ctrl Pts',(-24.3099781253355,7.49787641695439,
0.));
#201750=CARTESIAN_POINT('Ctrl Pts',(-24.3099781253355,7.49787641695439,
12.));
#201751=CARTESIAN_POINT('Ctrl Pts',(-24.2835078958973,7.50271363765152,
0.));
#201752=CARTESIAN_POINT('Ctrl Pts',(-24.2835078958973,7.50271363765152,
12.));
#201753=CARTESIAN_POINT('Ctrl Pts',(-24.2570993577034,7.50747703535133,
0.));
#201754=CARTESIAN_POINT('Ctrl Pts',(-24.2570993577034,7.50747703535133,
12.));
#201755=CARTESIAN_POINT('Ctrl Pts',(-24.2307530003887,7.51216677222181,
0.));
#201756=CARTESIAN_POINT('Ctrl Pts',(-24.2307530003887,7.51216677222181,
12.));
#201757=CARTESIAN_POINT('Ctrl Pts',(-24.2044693092349,7.51678300997949,
0.));
#201758=CARTESIAN_POINT('Ctrl Pts',(-24.2044693092349,7.51678300997949,
12.));
#201759=CARTESIAN_POINT('Ctrl Pts',(-24.1782487641594,7.52132590953802,
0.));
#201760=CARTESIAN_POINT('Ctrl Pts',(-24.1782487641594,7.52132590953802,
12.));
#201761=CARTESIAN_POINT('Ctrl Pts',(-24.1520918425364,7.52579563201424,
0.));
#201762=CARTESIAN_POINT('Ctrl Pts',(-24.1520918425364,7.52579563201424,
12.));
#201763=CARTESIAN_POINT('Ctrl Pts',(-24.1259990209207,7.53019233935501,
0.));
#201764=CARTESIAN_POINT('Ctrl Pts',(-24.1259990209207,7.53019233935501,
12.));
#201765=CARTESIAN_POINT('Ctrl Pts',(-24.0999707772642,7.53451619514649,
0.));
#201766=CARTESIAN_POINT('Ctrl Pts',(-24.0999707772642,7.53451619514649,
12.));
#201767=CARTESIAN_POINT('Ctrl Pts',(-24.0740075927985,7.53876736531014,
0.));
#201768=CARTESIAN_POINT('Ctrl Pts',(-24.0740075927985,7.53876736531014,
12.));
#201769=CARTESIAN_POINT('Ctrl Pts',(-24.0481099543353,7.54294601896144,
0.));
#201770=CARTESIAN_POINT('Ctrl Pts',(-24.0481099543353,7.54294601896144,
12.));
#201771=CARTESIAN_POINT('Ctrl Pts',(-24.022278355453,7.5470523288591,0.));
#201772=CARTESIAN_POINT('Ctrl Pts',(-24.022278355453,7.5470523288591,12.));
#201773=CARTESIAN_POINT('Ctrl Pts',(-23.9965132953185,7.55108647097441,
0.));
#201774=CARTESIAN_POINT('Ctrl Pts',(-23.9965132953185,7.55108647097441,
12.));
#201775=CARTESIAN_POINT('Ctrl Pts',(-23.9708152779884,7.55504862424812,
0.));
#201776=CARTESIAN_POINT('Ctrl Pts',(-23.9708152779884,7.55504862424812,
12.));
#201777=CARTESIAN_POINT('Ctrl Pts',(-23.9451848115,7.55893897027682,0.));
#201778=CARTESIAN_POINT('Ctrl Pts',(-23.9451848115,7.55893897027682,12.));
#201779=CARTESIAN_POINT('Ctrl Pts',(-23.9196224070759,7.56275769304773,
0.));
#201780=CARTESIAN_POINT('Ctrl Pts',(-23.9196224070759,7.56275769304773,
12.));
#201781=CARTESIAN_POINT('Ctrl Pts',(-23.8941285782003,7.56650497863792,
0.));
#201782=CARTESIAN_POINT('Ctrl Pts',(-23.8941285782003,7.56650497863792,
12.));
#201783=CARTESIAN_POINT('Ctrl Pts',(-23.8687038399598,7.57018101500711,
0.));
#201784=CARTESIAN_POINT('Ctrl Pts',(-23.8687038399598,7.57018101500711,
12.));
#201785=CARTESIAN_POINT('Ctrl Pts',(-23.8433487096134,7.57378599219816,
0.));
#201786=CARTESIAN_POINT('Ctrl Pts',(-23.8433487096134,7.57378599219816,
12.));
#201787=CARTESIAN_POINT('Ctrl Pts',(-23.8180637069977,7.57732010249066,
0.));
#201788=CARTESIAN_POINT('Ctrl Pts',(-23.8180637069977,7.57732010249066,
12.));
#201789=CARTESIAN_POINT('Ctrl Pts',(-23.7928493549908,7.58078354058212,
0.));
#201790=CARTESIAN_POINT('Ctrl Pts',(-23.7928493549908,7.58078354058212,
12.));
#201791=CARTESIAN_POINT('Ctrl Pts',(-23.7677061799376,7.58417650376272,
0.));
#201792=CARTESIAN_POINT('Ctrl Pts',(-23.7677061799376,7.58417650376272,
12.));
#201793=CARTESIAN_POINT('Ctrl Pts',(-23.7426347121006,7.58749919210832,
0.));
#201794=CARTESIAN_POINT('Ctrl Pts',(-23.7426347121006,7.58749919210832,
12.));
#201795=CARTESIAN_POINT('Ctrl Pts',(-23.7176354860457,7.59075180865327,
0.));
#201796=CARTESIAN_POINT('Ctrl Pts',(-23.7176354860457,7.59075180865327,
12.));
#201797=CARTESIAN_POINT('Ctrl Pts',(-23.6927090405067,7.59393455934042,
0.));
#201798=CARTESIAN_POINT('Ctrl Pts',(-23.6927090405067,7.59393455934042,
12.));
#201799=CARTESIAN_POINT('Ctrl Pts',(-23.6678559182876,7.59704765299572,
0.));
#201800=CARTESIAN_POINT('Ctrl Pts',(-23.6678559182876,7.59704765299572,
12.));
#201801=CARTESIAN_POINT('Ctrl Pts',(-23.6430766661419,7.60009130130129,
0.));
#201802=CARTESIAN_POINT('Ctrl Pts',(-23.6430766661419,7.60009130130129,
12.));
#201803=CARTESIAN_POINT('Ctrl Pts',(-23.6183718346576,7.60306571877806,
0.));
#201804=CARTESIAN_POINT('Ctrl Pts',(-23.6183718346576,7.60306571877806,
12.));
#201805=CARTESIAN_POINT('Ctrl Pts',(-23.5937419781244,7.60597112277094,
0.));
#201806=CARTESIAN_POINT('Ctrl Pts',(-23.5937419781244,7.60597112277094,
12.));
#201807=CARTESIAN_POINT('Ctrl Pts',(-23.5691876544243,7.60880773344599,
0.));
#201808=CARTESIAN_POINT('Ctrl Pts',(-23.5691876544243,7.60880773344599,
12.));
#201809=CARTESIAN_POINT('Ctrl Pts',(-23.5447094252029,7.61157577385372,
0.));
#201810=CARTESIAN_POINT('Ctrl Pts',(-23.5447094252029,7.61157577385372,
12.));
#201811=CARTESIAN_POINT('Ctrl Pts',(-23.5203078560128,7.61427546999299,
0.));
#201812=CARTESIAN_POINT('Ctrl Pts',(-23.5203078560128,7.61427546999299,
12.));
#201813=CARTESIAN_POINT('Ctrl Pts',(-23.4959835164608,7.61690705088319,
0.));
#201814=CARTESIAN_POINT('Ctrl Pts',(-23.4959835164608,7.61690705088319,
12.));
#201815=CARTESIAN_POINT('Ctrl Pts',(-23.4717369803438,7.61947074863977,
0.));
#201816=CARTESIAN_POINT('Ctrl Pts',(-23.4717369803438,7.61947074863977,
12.));
#201817=CARTESIAN_POINT('Ctrl Pts',(-23.4475688257854,7.62196679855957,
0.));
#201818=CARTESIAN_POINT('Ctrl Pts',(-23.4475688257854,7.62196679855957,
12.));
#201819=CARTESIAN_POINT('Ctrl Pts',(-23.4234796353544,7.62439543920054,
0.));
#201820=CARTESIAN_POINT('Ctrl Pts',(-23.4234796353544,7.62439543920054,
12.));
#201821=CARTESIAN_POINT('Ctrl Pts',(-23.3994699961122,7.62675691240335,
0.));
#201822=CARTESIAN_POINT('Ctrl Pts',(-23.3994699961122,7.62675691240335,
12.));
#201823=CARTESIAN_POINT('Ctrl Pts',(-23.3755404996638,7.62905146332598,
0.));
#201824=CARTESIAN_POINT('Ctrl Pts',(-23.3755404996638,7.62905146332598,
12.));
#201825=CARTESIAN_POINT('Ctrl Pts',(-23.3516917421973,7.63127934048139,
0.));
#201826=CARTESIAN_POINT('Ctrl Pts',(-23.3516917421973,7.63127934048139,
12.));
#201827=CARTESIAN_POINT('Ctrl Pts',(-23.3279243245241,7.63344079578162,
0.));
#201828=CARTESIAN_POINT('Ctrl Pts',(-23.3279243245241,7.63344079578162,
12.));
#201829=CARTESIAN_POINT('Ctrl Pts',(-23.3042388521021,7.63553608458784,
0.));
#201830=CARTESIAN_POINT('Ctrl Pts',(-23.3042388521021,7.63553608458784,
12.));
#201831=CARTESIAN_POINT('Ctrl Pts',(-23.2806359350853,7.63756546576375,
0.));
#201832=CARTESIAN_POINT('Ctrl Pts',(-23.2806359350853,7.63756546576375,
12.));
#201833=CARTESIAN_POINT('Ctrl Pts',(-23.2571161884487,7.63952920172837,
0.));
#201834=CARTESIAN_POINT('Ctrl Pts',(-23.2571161884487,7.63952920172837,
12.));
#201835=CARTESIAN_POINT('Ctrl Pts',(-23.2336802320912,7.64142755851508,
0.));
#201836=CARTESIAN_POINT('Ctrl Pts',(-23.2336802320912,7.64142755851508,
12.));
#201837=CARTESIAN_POINT('Ctrl Pts',(-23.2103286909399,7.64326080583684,
0.));
#201838=CARTESIAN_POINT('Ctrl Pts',(-23.2103286909399,7.64326080583684,
12.));
#201839=CARTESIAN_POINT('Ctrl Pts',(-23.1870621950452,7.64502921715483,
0.));
#201840=CARTESIAN_POINT('Ctrl Pts',(-23.1870621950452,7.64502921715483,
12.));
#201841=CARTESIAN_POINT('Ctrl Pts',(-23.1638813796691,7.64673306975797,
0.));
#201842=CARTESIAN_POINT('Ctrl Pts',(-23.1638813796691,7.64673306975797,
12.));
#201843=CARTESIAN_POINT('Ctrl Pts',(-23.1407868853815,7.64837264482929,
0.));
#201844=CARTESIAN_POINT('Ctrl Pts',(-23.1407868853815,7.64837264482929,
12.));
#201845=CARTESIAN_POINT('Ctrl Pts',(-23.1177793581674,7.64994822749845,
0.));
#201846=CARTESIAN_POINT('Ctrl Pts',(-23.1177793581674,7.64994822749845,
12.));
#201847=CARTESIAN_POINT('Ctrl Pts',(-23.0948594495246,7.65146010690464,
0.));
#201848=CARTESIAN_POINT('Ctrl Pts',(-23.0948594495246,7.65146010690464,
12.));
#201849=CARTESIAN_POINT('Ctrl Pts',(-23.072027816555,7.65290857626356,0.));
#201850=CARTESIAN_POINT('Ctrl Pts',(-23.072027816555,7.65290857626356,12.));
#201851=CARTESIAN_POINT('Ctrl Pts',(-23.049285122053,7.65429393293955,0.));
#201852=CARTESIAN_POINT('Ctrl Pts',(-23.049285122053,7.65429393293955,12.));
#201853=CARTESIAN_POINT('Ctrl Pts',(-23.0266320345792,7.65561647852555,
0.));
#201854=CARTESIAN_POINT('Ctrl Pts',(-23.0266320345792,7.65561647852555,
12.));
#201855=CARTESIAN_POINT('Ctrl Pts',(-23.004069228582,7.6568765189133,0.));
#201856=CARTESIAN_POINT('Ctrl Pts',(-23.004069228582,7.6568765189133,12.));
#201857=CARTESIAN_POINT('Ctrl Pts',(-22.9815973845301,7.65807436436453,
0.));
#201858=CARTESIAN_POINT('Ctrl Pts',(-22.9815973845301,7.65807436436453,
12.));
#201859=CARTESIAN_POINT('Ctrl Pts',(-22.9592171890332,7.65921032958912,
0.));
#201860=CARTESIAN_POINT('Ctrl Pts',(-22.9592171890332,7.65921032958912,
12.));
#201861=CARTESIAN_POINT('Ctrl Pts',(-22.9369293349592,7.66028473382777,
0.));
#201862=CARTESIAN_POINT('Ctrl Pts',(-22.9369293349592,7.66028473382777,
12.));
#201863=CARTESIAN_POINT('Ctrl Pts',(-22.9147345215418,7.661297900941,0.));
#201864=CARTESIAN_POINT('Ctrl Pts',(-22.9147345215418,7.661297900941,12.));
#201865=CARTESIAN_POINT('Ctrl Pts',(-22.8926334544879,7.66225015950147,
0.));
#201866=CARTESIAN_POINT('Ctrl Pts',(-22.8926334544879,7.66225015950147,
12.));
#201867=CARTESIAN_POINT('Ctrl Pts',(-22.870626846128,7.66314184287334,0.));
#201868=CARTESIAN_POINT('Ctrl Pts',(-22.870626846128,7.66314184287334,12.));
#201869=CARTESIAN_POINT('Ctrl Pts',(-22.8487154155569,7.66397328929805,
0.));
#201870=CARTESIAN_POINT('Ctrl Pts',(-22.8487154155569,7.66397328929805,
12.));
#201871=CARTESIAN_POINT('Ctrl Pts',(-22.8268998887679,7.66474484198553,
0.));
#201872=CARTESIAN_POINT('Ctrl Pts',(-22.8268998887679,7.66474484198553,
12.));
#201873=CARTESIAN_POINT('Ctrl Pts',(-22.8051809987834,7.66545684920987,
0.));
#201874=CARTESIAN_POINT('Ctrl Pts',(-22.8051809987834,7.66545684920987,
12.));
#201875=CARTESIAN_POINT('Ctrl Pts',(-22.7835594857697,7.66610966441259,
0.));
#201876=CARTESIAN_POINT('Ctrl Pts',(-22.7835594857697,7.66610966441259,
12.));
#201877=CARTESIAN_POINT('Ctrl Pts',(-22.7620360971839,7.66670364630273,
0.));
#201878=CARTESIAN_POINT('Ctrl Pts',(-22.7620360971839,7.66670364630273,
12.));
#201879=CARTESIAN_POINT('Ctrl Pts',(-22.7406115879508,7.66723915895412,
0.));
#201880=CARTESIAN_POINT('Ctrl Pts',(-22.7406115879508,7.66723915895412,
12.));
#201881=CARTESIAN_POINT('Ctrl Pts',(-22.7192867206242,7.6677165719101,0.));
#201882=CARTESIAN_POINT('Ctrl Pts',(-22.7192867206242,7.6677165719101,12.));
#201883=CARTESIAN_POINT('Ctrl Pts',(-22.6980622655446,7.66813626029276,
0.));
#201884=CARTESIAN_POINT('Ctrl Pts',(-22.6980622655446,7.66813626029276,
12.));
#201885=CARTESIAN_POINT('Ctrl Pts',(-22.6769390009889,7.66849860491763,
0.));
#201886=CARTESIAN_POINT('Ctrl Pts',(-22.6769390009889,7.66849860491763,
12.));
#201887=CARTESIAN_POINT('Ctrl Pts',(-22.6559177133133,7.66880399241354,
0.));
#201888=CARTESIAN_POINT('Ctrl Pts',(-22.6559177133133,7.66880399241354,
12.));
#201889=CARTESIAN_POINT('Ctrl Pts',(-22.6349991971547,7.66905281533745,
0.));
#201890=CARTESIAN_POINT('Ctrl Pts',(-22.6349991971547,7.66905281533745,
12.));
#201891=CARTESIAN_POINT('Ctrl Pts',(-22.6141842556248,7.66924547229435,
0.));
#201892=CARTESIAN_POINT('Ctrl Pts',(-22.6141842556248,7.66924547229435,
12.));
#201893=CARTESIAN_POINT('Ctrl Pts',(-22.5934737004955,7.66938236806241,
0.));
#201894=CARTESIAN_POINT('Ctrl Pts',(-22.5934737004955,7.66938236806241,
12.));
#201895=CARTESIAN_POINT('Ctrl Pts',(-22.5728683523829,7.66946391372299,
0.));
#201896=CARTESIAN_POINT('Ctrl Pts',(-22.5728683523829,7.66946391372299,
12.));
#201897=CARTESIAN_POINT('Ctrl Pts',(-22.5523690409109,7.66949052679671,
0.));
#201898=CARTESIAN_POINT('Ctrl Pts',(-22.5523690409109,7.66949052679671,
12.));
#201899=CARTESIAN_POINT('Ctrl Pts',(-22.5319766049191,7.66946263138116,
0.));
#201900=CARTESIAN_POINT('Ctrl Pts',(-22.5319766049191,7.66946263138116,
12.));
#201901=CARTESIAN_POINT('Ctrl Pts',(-22.5116918927023,7.66938065829082,
0.));
#201902=CARTESIAN_POINT('Ctrl Pts',(-22.5116918927023,7.66938065829082,
12.));
#201903=CARTESIAN_POINT('Ctrl Pts',(-22.4915157622308,7.66924504520302,
0.));
#201904=CARTESIAN_POINT('Ctrl Pts',(-22.4915157622308,7.66924504520302,
12.));
#201905=CARTESIAN_POINT('Ctrl Pts',(-22.47144908137,7.66905623680835,0.));
#201906=CARTESIAN_POINT('Ctrl Pts',(-22.47144908137,7.66905623680835,12.));
#201907=CARTESIAN_POINT('Ctrl Pts',(-22.4514927280863,7.6688146849666,0.));
#201908=CARTESIAN_POINT('Ctrl Pts',(-22.4514927280863,7.6688146849666,12.));
#201909=CARTESIAN_POINT('Ctrl Pts',(-22.4316475906616,7.66852084886745,
0.));
#201910=CARTESIAN_POINT('Ctrl Pts',(-22.4316475906616,7.66852084886745,
12.));
#201911=CARTESIAN_POINT('Ctrl Pts',(-22.411914567977,7.66817519519682,0.));
#201912=CARTESIAN_POINT('Ctrl Pts',(-22.411914567977,7.66817519519682,12.));
#201913=CARTESIAN_POINT('Ctrl Pts',(-22.3922945697782,7.66777819830819,
0.));
#201914=CARTESIAN_POINT('Ctrl Pts',(-22.3922945697782,7.66777819830819,
12.));
#201915=CARTESIAN_POINT('Ctrl Pts',(-22.3727885169361,7.66733034039887,
0.));
#201916=CARTESIAN_POINT('Ctrl Pts',(-22.3727885169361,7.66733034039887,
12.));
#201917=CARTESIAN_POINT('Ctrl Pts',(-22.3533973417013,7.66683211169134,
0.));
#201918=CARTESIAN_POINT('Ctrl Pts',(-22.3533973417013,7.66683211169134,
12.));
#201919=CARTESIAN_POINT('Ctrl Pts',(-22.3341219879454,7.66628401061905,
0.));
#201920=CARTESIAN_POINT('Ctrl Pts',(-22.3341219879454,7.66628401061905,
12.));
#201921=CARTESIAN_POINT('Ctrl Pts',(-22.3149634114823,7.66568654402441,
0.));
#201922=CARTESIAN_POINT('Ctrl Pts',(-22.3149634114823,7.66568654402441,
12.));
#201923=CARTESIAN_POINT('Ctrl Pts',(-22.2959225803925,7.66504022736262,
0.));
#201924=CARTESIAN_POINT('Ctrl Pts',(-22.2959225803925,7.66504022736262,
12.));
#201925=CARTESIAN_POINT('Ctrl Pts',(-22.2770004753332,7.66434558490972,
0.));
#201926=CARTESIAN_POINT('Ctrl Pts',(-22.2770004753332,7.66434558490972,
12.));
#201927=CARTESIAN_POINT('Ctrl Pts',(-22.2581980898487,7.66360314997662,
0.));
#201928=CARTESIAN_POINT('Ctrl Pts',(-22.2581980898487,7.66360314997662,
12.));
#201929=CARTESIAN_POINT('Ctrl Pts',(-22.239516430656,7.66281346512545,0.));
#201930=CARTESIAN_POINT('Ctrl Pts',(-22.239516430656,7.66281346512545,12.));
#201931=CARTESIAN_POINT('Ctrl Pts',(-22.2209565180098,7.66197708240435,
0.));
#201932=CARTESIAN_POINT('Ctrl Pts',(-22.2209565180098,7.66197708240435,
12.));
#201933=CARTESIAN_POINT('Ctrl Pts',(-22.2025193860972,7.66109456359292,
0.));
#201934=CARTESIAN_POINT('Ctrl Pts',(-22.2025193860972,7.66109456359292,
12.));
#201935=CARTESIAN_POINT('Ctrl Pts',(-22.1842060834092,7.66016648045008,
0.));
#201936=CARTESIAN_POINT('Ctrl Pts',(-22.1842060834092,7.66016648045008,
12.));
#201937=CARTESIAN_POINT('Ctrl Pts',(-22.1660176731174,7.65919341496925,
0.));
#201938=CARTESIAN_POINT('Ctrl Pts',(-22.1660176731174,7.65919341496925,
12.));
#201939=CARTESIAN_POINT('Ctrl Pts',(-22.1479552334206,7.65817595963351,
0.));
#201940=CARTESIAN_POINT('Ctrl Pts',(-22.1479552334206,7.65817595963351,
12.));
#201941=CARTESIAN_POINT('Ctrl Pts',(-22.1300198579671,7.65711471769407,
0.));
#201942=CARTESIAN_POINT('Ctrl Pts',(-22.1300198579671,7.65711471769407,
12.));
#201943=CARTESIAN_POINT('Ctrl Pts',(-22.1122126563327,7.65601030346819,
0.));
#201944=CARTESIAN_POINT('Ctrl Pts',(-22.1122126563327,7.65601030346819,
12.));
#201945=CARTESIAN_POINT('Ctrl Pts',(-22.094534754469,7.6548633426365,0.));
#201946=CARTESIAN_POINT('Ctrl Pts',(-22.094534754469,7.6548633426365,12.));
#201947=CARTESIAN_POINT('Ctrl Pts',(-22.0769872951596,7.65367447254945,
0.));
#201948=CARTESIAN_POINT('Ctrl Pts',(-22.0769872951596,7.65367447254945,
12.));
#201949=CARTESIAN_POINT('Ctrl Pts',(-22.0595714384432,7.65244434253104,
0.));
#201950=CARTESIAN_POINT('Ctrl Pts',(-22.0595714384432,7.65244434253104,
12.));
#201951=CARTESIAN_POINT('Ctrl Pts',(-22.0422883621176,7.65117361421346,
0.));
#201952=CARTESIAN_POINT('Ctrl Pts',(-22.0422883621176,7.65117361421346,
12.));
#201953=CARTESIAN_POINT('Ctrl Pts',(-22.0251392623209,7.64986296190156,
0.));
#201954=CARTESIAN_POINT('Ctrl Pts',(-22.0251392623209,7.64986296190156,
12.));
#201955=CARTESIAN_POINT('Ctrl Pts',(-22.0081253540773,7.64851307293346,
0.));
#201956=CARTESIAN_POINT('Ctrl Pts',(-22.0081253540773,7.64851307293346,
12.));
#201957=CARTESIAN_POINT('Ctrl Pts',(-21.9912478718542,7.64712464805258,
0.));
#201958=CARTESIAN_POINT('Ctrl Pts',(-21.9912478718542,7.64712464805258,
12.));
#201959=CARTESIAN_POINT('Ctrl Pts',(-21.97450807008,7.64569840177359,0.));
#201960=CARTESIAN_POINT('Ctrl Pts',(-21.97450807008,7.64569840177359,12.));
#201961=CARTESIAN_POINT('Ctrl Pts',(-21.9579072237653,7.64423506279153,
0.));
#201962=CARTESIAN_POINT('Ctrl Pts',(-21.9579072237653,7.64423506279153,
12.));
#201963=CARTESIAN_POINT('Ctrl Pts',(-21.9414466292074,7.64273537442706,
0.));
#201964=CARTESIAN_POINT('Ctrl Pts',(-21.9414466292074,7.64273537442706,
12.));
#201965=CARTESIAN_POINT('Ctrl Pts',(-21.9251276046546,7.6412000950654,0.));
#201966=CARTESIAN_POINT('Ctrl Pts',(-21.9251276046546,7.6412000950654,12.));
#201967=CARTESIAN_POINT('Ctrl Pts',(-21.9089514909873,7.63962999860916,
0.));
#201968=CARTESIAN_POINT('Ctrl Pts',(-21.9089514909873,7.63962999860916,
12.));
#201969=CARTESIAN_POINT('Ctrl Pts',(-21.8929196523511,7.63802587492007,
0.));
#201970=CARTESIAN_POINT('Ctrl Pts',(-21.8929196523511,7.63802587492007,
12.));
#201971=CARTESIAN_POINT('Ctrl Pts',(-21.8770334769492,7.63638853033367,
0.));
#201972=CARTESIAN_POINT('Ctrl Pts',(-21.8770334769492,7.63638853033367,
12.));
#201973=CARTESIAN_POINT('Ctrl Pts',(-21.8612943779086,7.63471878821203,
0.));
#201974=CARTESIAN_POINT('Ctrl Pts',(-21.8612943779086,7.63471878821203,
12.));
#201975=CARTESIAN_POINT('Ctrl Pts',(-21.8457037941084,7.63301748948936,
0.));
#201976=CARTESIAN_POINT('Ctrl Pts',(-21.8457037941084,7.63301748948936,
12.));
#201977=CARTESIAN_POINT('Ctrl Pts',(-21.8302631910197,7.6312854932304,0.));
#201978=CARTESIAN_POINT('Ctrl Pts',(-21.8302631910197,7.6312854932304,12.));
#201979=CARTESIAN_POINT('Ctrl Pts',(-21.8149740615093,7.62952367718151,
0.));
#201980=CARTESIAN_POINT('Ctrl Pts',(-21.8149740615093,7.62952367718151,
12.));
#201981=CARTESIAN_POINT('Ctrl Pts',(-21.7998379268583,7.62773293842409,
0.));
#201982=CARTESIAN_POINT('Ctrl Pts',(-21.7998379268583,7.62773293842409,
12.));
#201983=CARTESIAN_POINT('Ctrl Pts',(-21.7848563378022,7.62591419404521,
0.));
#201984=CARTESIAN_POINT('Ctrl Pts',(-21.7848563378022,7.62591419404521,
12.));
#201985=CARTESIAN_POINT('Ctrl Pts',(-21.7700308755583,7.62406838181164,
0.));
#201986=CARTESIAN_POINT('Ctrl Pts',(-21.7700308755583,7.62406838181164,
12.));
#201987=CARTESIAN_POINT('Ctrl Pts',(-21.7553631528329,7.62219646084226,
0.));
#201988=CARTESIAN_POINT('Ctrl Pts',(-21.7553631528329,7.62219646084226,
12.));
#201989=CARTESIAN_POINT('Ctrl Pts',(-21.7408548148657,7.62029941230855,
0.));
#201990=CARTESIAN_POINT('Ctrl Pts',(-21.7408548148657,7.62029941230855,
12.));
#201991=CARTESIAN_POINT('Ctrl Pts',(-21.7265075407977,7.61837824030541,
0.));
#201992=CARTESIAN_POINT('Ctrl Pts',(-21.7265075407977,7.61837824030541,
12.));
#201993=CARTESIAN_POINT('Ctrl Pts',(-21.7123230449835,7.61643397270425,
0.));
#201994=CARTESIAN_POINT('Ctrl Pts',(-21.7123230449835,7.61643397270425,
12.));
#201995=CARTESIAN_POINT('Ctrl Pts',(-21.6983030783321,7.61446766202787,
0.));
#201996=CARTESIAN_POINT('Ctrl Pts',(-21.6983030783321,7.61446766202787,
12.));
#201997=CARTESIAN_POINT('Ctrl Pts',(-21.6844494295813,7.61248038630265,
0.));
#201998=CARTESIAN_POINT('Ctrl Pts',(-21.6844494295813,7.61248038630265,
12.));
#201999=CARTESIAN_POINT('Ctrl Pts',(-21.6707639267573,7.6104732500095,0.));
#202000=CARTESIAN_POINT('Ctrl Pts',(-21.6707639267573,7.6104732500095,12.));
#202001=CARTESIAN_POINT('Ctrl Pts',(-21.6572484388079,7.60844738512872,
0.));
#202002=CARTESIAN_POINT('Ctrl Pts',(-21.6572484388079,7.60844738512872,
12.));
#202003=CARTESIAN_POINT('Ctrl Pts',(-21.6439048771743,7.60640395216358,
0.));
#202004=CARTESIAN_POINT('Ctrl Pts',(-21.6439048771743,7.60640395216358,
12.));
#202005=CARTESIAN_POINT('Ctrl Pts',(-21.6307351973823,7.604344141183,0.));
#202006=CARTESIAN_POINT('Ctrl Pts',(-21.6307351973823,7.604344141183,12.));
#202007=CARTESIAN_POINT('Ctrl Pts',(-21.6177414005991,7.60226917285432,
0.));
#202008=CARTESIAN_POINT('Ctrl Pts',(-21.6177414005991,7.60226917285432,
12.));
#202009=CARTESIAN_POINT('Ctrl Pts',(-21.6049255358843,7.60018029988238,
0.));
#202010=CARTESIAN_POINT('Ctrl Pts',(-21.6049255358843,7.60018029988238,
12.));
#202011=CARTESIAN_POINT('Ctrl Pts',(-21.5922897024466,7.59807880846192,
0.));
#202012=CARTESIAN_POINT('Ctrl Pts',(-21.5922897024466,7.59807880846192,
12.));
#202013=CARTESIAN_POINT('Ctrl Pts',(-21.5798360518978,7.59596601973588,
0.));
#202014=CARTESIAN_POINT('Ctrl Pts',(-21.5798360518978,7.59596601973588,
12.));
#202015=CARTESIAN_POINT('Ctrl Pts',(-21.5675667904728,7.5938432912493,0.));
#202016=CARTESIAN_POINT('Ctrl Pts',(-21.5675667904728,7.5938432912493,12.));
#202017=CARTESIAN_POINT('Ctrl Pts',(-21.5554841813465,7.59171201844793,
0.));
#202018=CARTESIAN_POINT('Ctrl Pts',(-21.5554841813465,7.59171201844793,
12.));
#202019=CARTESIAN_POINT('Ctrl Pts',(-21.5435905470113,7.58957363620026,
0.));
#202020=CARTESIAN_POINT('Ctrl Pts',(-21.5435905470113,7.58957363620026,
12.));
#202021=CARTESIAN_POINT('Ctrl Pts',(-21.5318882716735,7.58742962034834,
0.));
#202022=CARTESIAN_POINT('Ctrl Pts',(-21.5318882716735,7.58742962034834,
12.));
#202023=CARTESIAN_POINT('Ctrl Pts',(-21.5203798035294,7.58528148919113,
0.));
#202024=CARTESIAN_POINT('Ctrl Pts',(-21.5203798035294,7.58528148919113,
12.));
#202025=CARTESIAN_POINT('Ctrl Pts',(-21.5090676573866,7.58313080519158,
0.));
#202026=CARTESIAN_POINT('Ctrl Pts',(-21.5090676573866,7.58313080519158,
12.));
#202027=CARTESIAN_POINT('Ctrl Pts',(-21.497954419274,7.5809791779073,0.));
#202028=CARTESIAN_POINT('Ctrl Pts',(-21.497954419274,7.5809791779073,12.));
#202029=CARTESIAN_POINT('Ctrl Pts',(-21.4870427508193,7.57882826679131,
0.));
#202030=CARTESIAN_POINT('Ctrl Pts',(-21.4870427508193,7.57882826679131,
12.));
#202031=CARTESIAN_POINT('Ctrl Pts',(-21.4763353936766,7.57667978403002,
0.));
#202032=CARTESIAN_POINT('Ctrl Pts',(-21.4763353936766,7.57667978403002,
12.));
#202033=CARTESIAN_POINT('Ctrl Pts',(-21.4658351740135,7.57453549743435,
0.));
#202034=CARTESIAN_POINT('Ctrl Pts',(-21.4658351740135,7.57453549743435,
12.));
#202035=CARTESIAN_POINT('Ctrl Pts',(-21.4555450053147,7.57239723223521,
0.));
#202036=CARTESIAN_POINT('Ctrl Pts',(-21.4555450053147,7.57239723223521,
12.));
#202037=CARTESIAN_POINT('Ctrl Pts',(-21.445467890751,7.57026687261169,0.));
#202038=CARTESIAN_POINT('Ctrl Pts',(-21.445467890751,7.57026687261169,12.));
#202039=CARTESIAN_POINT('Ctrl Pts',(-21.435606926151,7.56814636360842,0.));
#202040=CARTESIAN_POINT('Ctrl Pts',(-21.435606926151,7.56814636360842,12.));
#202041=CARTESIAN_POINT('Ctrl Pts',(-21.4259653015732,7.56603771218706,
0.));
#202042=CARTESIAN_POINT('Ctrl Pts',(-21.4259653015732,7.56603771218706,
12.));
#202043=CARTESIAN_POINT('Ctrl Pts',(-21.4165463106252,7.56394299313682,
0.));
#202044=CARTESIAN_POINT('Ctrl Pts',(-21.4165463106252,7.56394299313682,
12.));
#202045=CARTESIAN_POINT('Ctrl Pts',(-21.4073533630364,7.56186435703622,
0.));
#202046=CARTESIAN_POINT('Ctrl Pts',(-21.4073533630364,7.56186435703622,
12.));
#202047=CARTESIAN_POINT('Ctrl Pts',(-21.3983899952988,7.55980403700615,
0.));
#202048=CARTESIAN_POINT('Ctrl Pts',(-21.3983899952988,7.55980403700615,
12.));
#202049=CARTESIAN_POINT('Ctrl Pts',(-21.3896598842119,7.55776435731422,
0.));
#202050=CARTESIAN_POINT('Ctrl Pts',(-21.3896598842119,7.55776435731422,
12.));
#202051=CARTESIAN_POINT('Ctrl Pts',(-21.3811668478933,7.55574773403507,
0.));
#202052=CARTESIAN_POINT('Ctrl Pts',(-21.3811668478933,7.55574773403507,
12.));
#202053=CARTESIAN_POINT('Ctrl Pts',(-21.3729148390244,7.55375667080032,
0.));
#202054=CARTESIAN_POINT('Ctrl Pts',(-21.3729148390244,7.55375667080032,
12.));
#202055=CARTESIAN_POINT('Ctrl Pts',(-21.3649079431864,7.55179375777441,
0.));
#202056=CARTESIAN_POINT('Ctrl Pts',(-21.3649079431864,7.55179375777441,
12.));
#202057=CARTESIAN_POINT('Ctrl Pts',(-21.3571503685853,7.54986166521306,
0.));
#202058=CARTESIAN_POINT('Ctrl Pts',(-21.3571503685853,7.54986166521306,
12.));
#202059=CARTESIAN_POINT('Ctrl Pts',(-21.349646476153,7.54796316246327,0.));
#202060=CARTESIAN_POINT('Ctrl Pts',(-21.349646476153,7.54796316246327,12.));
#202061=CARTESIAN_POINT('Ctrl Pts',(-21.3424008295038,7.54610114948351,
0.));
#202062=CARTESIAN_POINT('Ctrl Pts',(-21.3424008295038,7.54610114948351,
12.));
#202063=CARTESIAN_POINT('Ctrl Pts',(-21.3354182340149,7.54427868151268,
0.));
#202064=CARTESIAN_POINT('Ctrl Pts',(-21.3354182340149,7.54427868151268,
12.));
#202065=CARTESIAN_POINT('Ctrl Pts',(-21.328703791771,7.54249900377031,0.));
#202066=CARTESIAN_POINT('Ctrl Pts',(-21.328703791771,7.54249900377031,12.));
#202067=CARTESIAN_POINT('Ctrl Pts',(-21.3222628524165,7.5407655203828,0.));
#202068=CARTESIAN_POINT('Ctrl Pts',(-21.3222628524165,7.5407655203828,12.));
#202069=CARTESIAN_POINT('Ctrl Pts',(-21.3161009456256,7.53908175169899,
0.));
#202070=CARTESIAN_POINT('Ctrl Pts',(-21.3161009456256,7.53908175169899,
12.));
#202071=CARTESIAN_POINT('Ctrl Pts',(-21.3102237167729,7.53745129364619,
0.));
#202072=CARTESIAN_POINT('Ctrl Pts',(-21.3102237167729,7.53745129364619,
12.));
#202073=CARTESIAN_POINT('Ctrl Pts',(-21.3046368712156,7.53587778251743,
0.));
#202074=CARTESIAN_POINT('Ctrl Pts',(-21.3046368712156,7.53587778251743,
12.));
#202075=CARTESIAN_POINT('Ctrl Pts',(-21.2993464250717,7.53436505309949,
0.));
#202076=CARTESIAN_POINT('Ctrl Pts',(-21.2993464250717,7.53436505309949,
12.));
#202077=CARTESIAN_POINT('Ctrl Pts',(-21.2943588989331,7.53291726078526,
0.));
#202078=CARTESIAN_POINT('Ctrl Pts',(-21.2943588989331,7.53291726078526,
12.));
#202079=CARTESIAN_POINT('Ctrl Pts',(-21.2896816163843,7.53153906987847,
0.));
#202080=CARTESIAN_POINT('Ctrl Pts',(-21.2896816163843,7.53153906987847,
12.));
#202081=CARTESIAN_POINT('Ctrl Pts',(-21.2853226580658,7.53023562438221,
0.));
#202082=CARTESIAN_POINT('Ctrl Pts',(-21.2853226580658,7.53023562438221,
12.));
#202083=CARTESIAN_POINT('Ctrl Pts',(-21.2812902781143,7.52901217930407,
0.));
#202084=CARTESIAN_POINT('Ctrl Pts',(-21.2812902781143,7.52901217930407,
12.));
#202085=CARTESIAN_POINT('Ctrl Pts',(-21.2775925269651,7.52787386225343,
0.));
#202086=CARTESIAN_POINT('Ctrl Pts',(-21.2775925269651,7.52787386225343,
12.));
#202087=CARTESIAN_POINT('Ctrl Pts',(-21.2742366113578,7.5268252691856,0.));
#202088=CARTESIAN_POINT('Ctrl Pts',(-21.2742366113578,7.5268252691856,12.));
#202089=CARTESIAN_POINT('Ctrl Pts',(-21.2712301573465,7.52587126095544,
0.));
#202090=CARTESIAN_POINT('Ctrl Pts',(-21.2712301573465,7.52587126095544,
12.));
#202091=CARTESIAN_POINT('Ctrl Pts',(-21.2685823838672,7.52501770333522,
0.));
#202092=CARTESIAN_POINT('Ctrl Pts',(-21.2685823838672,7.52501770333522,
12.));
#202093=CARTESIAN_POINT('Ctrl Pts',(-21.266305915706,7.52427261074264,0.));
#202094=CARTESIAN_POINT('Ctrl Pts',(-21.266305915706,7.52427261074264,12.));
#202095=CARTESIAN_POINT('Ctrl Pts',(-21.2644161259965,7.52364573027521,
0.));
#202096=CARTESIAN_POINT('Ctrl Pts',(-21.2644161259965,7.52364573027521,
12.));
#202097=CARTESIAN_POINT('Ctrl Pts',(-21.262927782038,7.52314642316202,0.));
#202098=CARTESIAN_POINT('Ctrl Pts',(-21.262927782038,7.52314642316202,12.));
#202099=CARTESIAN_POINT('Ctrl Pts',(-21.261852128355,7.52278182242727,0.));
#202100=CARTESIAN_POINT('Ctrl Pts',(-21.261852128355,7.52278182242727,12.));
#202101=CARTESIAN_POINT('Ctrl Pts',(-21.2613260540651,7.52260064231736,
0.));
#202102=CARTESIAN_POINT('Ctrl Pts',(-21.2613260540651,7.52260064231736,
12.));
#202103=CARTESIAN_POINT('Ctrl Pts',(-21.261120447486,7.52252744144958,0.));
#202104=CARTESIAN_POINT('Ctrl Pts',(-21.261120447486,7.52252744144958,12.));
#202105=CARTESIAN_POINT('Ctrl Pts',(-21.2610673466883,7.52250649703992,
0.));
#202106=CARTESIAN_POINT('Ctrl Pts',(-21.2610673466883,7.52250649703992,
12.));
#202107=CARTESIAN_POINT('Ctrl Pts',(-21.2610617890679,7.52250298901265,
0.));
#202108=CARTESIAN_POINT('Ctrl Pts',(-21.2610617890679,7.52250298901265,
12.));
#202109=CARTESIAN_POINT('',(-24.9347862158358,7.36589684767345,0.));
#202110=CARTESIAN_POINT('Ctrl Pts',(-24.9347862158358,7.36589684767345,
0.));
#202111=CARTESIAN_POINT('Ctrl Pts',(-24.9292275670674,7.36721909028843,
0.));
#202112=CARTESIAN_POINT('Ctrl Pts',(-24.9181155530543,7.3698559312009,0.));
#202113=CARTESIAN_POINT('Ctrl Pts',(-24.901463382605,7.37378825961676,0.));
#202114=CARTESIAN_POINT('Ctrl Pts',(-24.8792921911115,7.3789854964027,0.));
#202115=CARTESIAN_POINT('Ctrl Pts',(-24.8516310625176,7.38540558903621,
0.));
#202116=CARTESIAN_POINT('Ctrl Pts',(-24.8240228520893,7.39174922585808,
0.));
#202117=CARTESIAN_POINT('Ctrl Pts',(-24.7964676646431,7.39801641583013,
0.));
#202118=CARTESIAN_POINT('Ctrl Pts',(-24.7689656668983,7.40420718661603,
0.));
#202119=CARTESIAN_POINT('Ctrl Pts',(-24.7415170994784,7.41032159082382,
0.));
#202120=CARTESIAN_POINT('Ctrl Pts',(-24.7141222950051,7.41635971481674,
0.));
#202121=CARTESIAN_POINT('Ctrl Pts',(-24.6867816727192,7.42232167766265,
0.));
#202122=CARTESIAN_POINT('Ctrl Pts',(-24.6594957128756,7.42820762159126,
0.));
#202123=CARTESIAN_POINT('Ctrl Pts',(-24.6322649369517,7.43401770489524,
0.));
#202124=CARTESIAN_POINT('Ctrl Pts',(-24.6050898852368,7.43975209375504,
0.));
#202125=CARTESIAN_POINT('Ctrl Pts',(-24.577971096086,7.44541095473134,0.));
#202126=CARTESIAN_POINT('Ctrl Pts',(-24.5509090831559,7.4509944465116,0.));
#202127=CARTESIAN_POINT('Ctrl Pts',(-24.5239043173072,7.45650271335862,
0.));
#202128=CARTESIAN_POINT('Ctrl Pts',(-24.4969572391483,7.46193588961463,
0.));
#202129=CARTESIAN_POINT('Ctrl Pts',(-24.4700682684524,7.46729410308786,
0.));
#202130=CARTESIAN_POINT('Ctrl Pts',(-24.443237814649,7.47257747883246,0.));
#202131=CARTESIAN_POINT('Ctrl Pts',(-24.4164662871163,7.47778614286565,
0.));
#202132=CARTESIAN_POINT('Ctrl Pts',(-24.3897541049254,7.48292022569301,
0.));
#202133=CARTESIAN_POINT('Ctrl Pts',(-24.3631017084524,7.48797986651908,
0.));
#202134=CARTESIAN_POINT('Ctrl Pts',(-24.3365095573685,7.4929652125242,0.));
#202135=CARTESIAN_POINT('Ctrl Pts',(-24.3099781253355,7.49787641695439,
0.));
#202136=CARTESIAN_POINT('Ctrl Pts',(-24.2835078958973,7.50271363765152,
0.));
#202137=CARTESIAN_POINT('Ctrl Pts',(-24.2570993577034,7.50747703535133,
0.));
#202138=CARTESIAN_POINT('Ctrl Pts',(-24.2307530003887,7.51216677222181,
0.));
#202139=CARTESIAN_POINT('Ctrl Pts',(-24.2044693092349,7.51678300997949,
0.));
#202140=CARTESIAN_POINT('Ctrl Pts',(-24.1782487641594,7.52132590953802,
0.));
#202141=CARTESIAN_POINT('Ctrl Pts',(-24.1520918425364,7.52579563201424,
0.));
#202142=CARTESIAN_POINT('Ctrl Pts',(-24.1259990209207,7.53019233935501,
0.));
#202143=CARTESIAN_POINT('Ctrl Pts',(-24.0999707772642,7.53451619514649,
0.));
#202144=CARTESIAN_POINT('Ctrl Pts',(-24.0740075927985,7.53876736531014,
0.));
#202145=CARTESIAN_POINT('Ctrl Pts',(-24.0481099543353,7.54294601896144,
0.));
#202146=CARTESIAN_POINT('Ctrl Pts',(-24.022278355453,7.5470523288591,0.));
#202147=CARTESIAN_POINT('Ctrl Pts',(-23.9965132953185,7.55108647097441,
0.));
#202148=CARTESIAN_POINT('Ctrl Pts',(-23.9708152779884,7.55504862424812,
0.));
#202149=CARTESIAN_POINT('Ctrl Pts',(-23.9451848115,7.55893897027682,0.));
#202150=CARTESIAN_POINT('Ctrl Pts',(-23.9196224070759,7.56275769304773,
0.));
#202151=CARTESIAN_POINT('Ctrl Pts',(-23.8941285782003,7.56650497863792,
0.));
#202152=CARTESIAN_POINT('Ctrl Pts',(-23.8687038399598,7.57018101500711,
0.));
#202153=CARTESIAN_POINT('Ctrl Pts',(-23.8433487096134,7.57378599219816,
0.));
#202154=CARTESIAN_POINT('Ctrl Pts',(-23.8180637069977,7.57732010249066,
0.));
#202155=CARTESIAN_POINT('Ctrl Pts',(-23.7928493549908,7.58078354058212,
0.));
#202156=CARTESIAN_POINT('Ctrl Pts',(-23.7677061799376,7.58417650376272,
0.));
#202157=CARTESIAN_POINT('Ctrl Pts',(-23.7426347121006,7.58749919210832,
0.));
#202158=CARTESIAN_POINT('Ctrl Pts',(-23.7176354860457,7.59075180865327,
0.));
#202159=CARTESIAN_POINT('Ctrl Pts',(-23.6927090405067,7.59393455934042,
0.));
#202160=CARTESIAN_POINT('Ctrl Pts',(-23.6678559182876,7.59704765299572,
0.));
#202161=CARTESIAN_POINT('Ctrl Pts',(-23.6430766661419,7.60009130130129,
0.));
#202162=CARTESIAN_POINT('Ctrl Pts',(-23.6183718346576,7.60306571877806,
0.));
#202163=CARTESIAN_POINT('Ctrl Pts',(-23.5937419781244,7.60597112277094,
0.));
#202164=CARTESIAN_POINT('Ctrl Pts',(-23.5691876544243,7.60880773344599,
0.));
#202165=CARTESIAN_POINT('Ctrl Pts',(-23.5447094252029,7.61157577385372,
0.));
#202166=CARTESIAN_POINT('Ctrl Pts',(-23.5203078560128,7.61427546999299,
0.));
#202167=CARTESIAN_POINT('Ctrl Pts',(-23.4959835164608,7.61690705088319,
0.));
#202168=CARTESIAN_POINT('Ctrl Pts',(-23.4717369803438,7.61947074863977,
0.));
#202169=CARTESIAN_POINT('Ctrl Pts',(-23.4475688257854,7.62196679855957,
0.));
#202170=CARTESIAN_POINT('Ctrl Pts',(-23.4234796353544,7.62439543920054,
0.));
#202171=CARTESIAN_POINT('Ctrl Pts',(-23.3994699961122,7.62675691240335,
0.));
#202172=CARTESIAN_POINT('Ctrl Pts',(-23.3755404996638,7.62905146332598,
0.));
#202173=CARTESIAN_POINT('Ctrl Pts',(-23.3516917421973,7.63127934048139,
0.));
#202174=CARTESIAN_POINT('Ctrl Pts',(-23.3279243245241,7.63344079578162,
0.));
#202175=CARTESIAN_POINT('Ctrl Pts',(-23.3042388521021,7.63553608458784,
0.));
#202176=CARTESIAN_POINT('Ctrl Pts',(-23.2806359350853,7.63756546576375,
0.));
#202177=CARTESIAN_POINT('Ctrl Pts',(-23.2571161884487,7.63952920172837,
0.));
#202178=CARTESIAN_POINT('Ctrl Pts',(-23.2336802320912,7.64142755851508,
0.));
#202179=CARTESIAN_POINT('Ctrl Pts',(-23.2103286909399,7.64326080583684,
0.));
#202180=CARTESIAN_POINT('Ctrl Pts',(-23.1870621950452,7.64502921715483,
0.));
#202181=CARTESIAN_POINT('Ctrl Pts',(-23.1638813796691,7.64673306975797,
0.));
#202182=CARTESIAN_POINT('Ctrl Pts',(-23.1407868853815,7.64837264482929,
0.));
#202183=CARTESIAN_POINT('Ctrl Pts',(-23.1177793581674,7.64994822749845,
0.));
#202184=CARTESIAN_POINT('Ctrl Pts',(-23.0948594495246,7.65146010690464,
0.));
#202185=CARTESIAN_POINT('Ctrl Pts',(-23.072027816555,7.65290857626356,0.));
#202186=CARTESIAN_POINT('Ctrl Pts',(-23.049285122053,7.65429393293955,0.));
#202187=CARTESIAN_POINT('Ctrl Pts',(-23.0266320345792,7.65561647852555,
0.));
#202188=CARTESIAN_POINT('Ctrl Pts',(-23.004069228582,7.6568765189133,0.));
#202189=CARTESIAN_POINT('Ctrl Pts',(-22.9815973845301,7.65807436436453,
0.));
#202190=CARTESIAN_POINT('Ctrl Pts',(-22.9592171890332,7.65921032958912,
0.));
#202191=CARTESIAN_POINT('Ctrl Pts',(-22.9369293349592,7.66028473382777,
0.));
#202192=CARTESIAN_POINT('Ctrl Pts',(-22.9147345215418,7.661297900941,0.));
#202193=CARTESIAN_POINT('Ctrl Pts',(-22.8926334544879,7.66225015950147,
0.));
#202194=CARTESIAN_POINT('Ctrl Pts',(-22.870626846128,7.66314184287334,0.));
#202195=CARTESIAN_POINT('Ctrl Pts',(-22.8487154155569,7.66397328929805,
0.));
#202196=CARTESIAN_POINT('Ctrl Pts',(-22.8268998887679,7.66474484198553,
0.));
#202197=CARTESIAN_POINT('Ctrl Pts',(-22.8051809987834,7.66545684920987,
0.));
#202198=CARTESIAN_POINT('Ctrl Pts',(-22.7835594857697,7.66610966441259,
0.));
#202199=CARTESIAN_POINT('Ctrl Pts',(-22.7620360971839,7.66670364630273,
0.));
#202200=CARTESIAN_POINT('Ctrl Pts',(-22.7406115879508,7.66723915895412,
0.));
#202201=CARTESIAN_POINT('Ctrl Pts',(-22.7192867206242,7.6677165719101,0.));
#202202=CARTESIAN_POINT('Ctrl Pts',(-22.6980622655446,7.66813626029276,
0.));
#202203=CARTESIAN_POINT('Ctrl Pts',(-22.6769390009889,7.66849860491763,
0.));
#202204=CARTESIAN_POINT('Ctrl Pts',(-22.6559177133133,7.66880399241354,
0.));
#202205=CARTESIAN_POINT('Ctrl Pts',(-22.6349991971547,7.66905281533745,
0.));
#202206=CARTESIAN_POINT('Ctrl Pts',(-22.6141842556248,7.66924547229435,
0.));
#202207=CARTESIAN_POINT('Ctrl Pts',(-22.5934737004955,7.66938236806241,
0.));
#202208=CARTESIAN_POINT('Ctrl Pts',(-22.5728683523829,7.66946391372299,
0.));
#202209=CARTESIAN_POINT('Ctrl Pts',(-22.5523690409109,7.66949052679671,
0.));
#202210=CARTESIAN_POINT('Ctrl Pts',(-22.5319766049191,7.66946263138116,
0.));
#202211=CARTESIAN_POINT('Ctrl Pts',(-22.5116918927023,7.66938065829082,
0.));
#202212=CARTESIAN_POINT('Ctrl Pts',(-22.4915157622308,7.66924504520302,
0.));
#202213=CARTESIAN_POINT('Ctrl Pts',(-22.47144908137,7.66905623680835,0.));
#202214=CARTESIAN_POINT('Ctrl Pts',(-22.4514927280863,7.6688146849666,0.));
#202215=CARTESIAN_POINT('Ctrl Pts',(-22.4316475906616,7.66852084886745,
0.));
#202216=CARTESIAN_POINT('Ctrl Pts',(-22.411914567977,7.66817519519682,0.));
#202217=CARTESIAN_POINT('Ctrl Pts',(-22.3922945697782,7.66777819830819,
0.));
#202218=CARTESIAN_POINT('Ctrl Pts',(-22.3727885169361,7.66733034039887,
0.));
#202219=CARTESIAN_POINT('Ctrl Pts',(-22.3533973417013,7.66683211169134,
0.));
#202220=CARTESIAN_POINT('Ctrl Pts',(-22.3341219879454,7.66628401061905,
0.));
#202221=CARTESIAN_POINT('Ctrl Pts',(-22.3149634114823,7.66568654402441,
0.));
#202222=CARTESIAN_POINT('Ctrl Pts',(-22.2959225803925,7.66504022736262,
0.));
#202223=CARTESIAN_POINT('Ctrl Pts',(-22.2770004753332,7.66434558490972,
0.));
#202224=CARTESIAN_POINT('Ctrl Pts',(-22.2581980898487,7.66360314997662,
0.));
#202225=CARTESIAN_POINT('Ctrl Pts',(-22.239516430656,7.66281346512545,0.));
#202226=CARTESIAN_POINT('Ctrl Pts',(-22.2209565180098,7.66197708240435,
0.));
#202227=CARTESIAN_POINT('Ctrl Pts',(-22.2025193860972,7.66109456359292,
0.));
#202228=CARTESIAN_POINT('Ctrl Pts',(-22.1842060834092,7.66016648045008,
0.));
#202229=CARTESIAN_POINT('Ctrl Pts',(-22.1660176731174,7.65919341496925,
0.));
#202230=CARTESIAN_POINT('Ctrl Pts',(-22.1479552334206,7.65817595963351,
0.));
#202231=CARTESIAN_POINT('Ctrl Pts',(-22.1300198579671,7.65711471769407,
0.));
#202232=CARTESIAN_POINT('Ctrl Pts',(-22.1122126563327,7.65601030346819,
0.));
#202233=CARTESIAN_POINT('Ctrl Pts',(-22.094534754469,7.6548633426365,0.));
#202234=CARTESIAN_POINT('Ctrl Pts',(-22.0769872951596,7.65367447254945,
0.));
#202235=CARTESIAN_POINT('Ctrl Pts',(-22.0595714384432,7.65244434253104,
0.));
#202236=CARTESIAN_POINT('Ctrl Pts',(-22.0422883621176,7.65117361421346,
0.));
#202237=CARTESIAN_POINT('Ctrl Pts',(-22.0251392623209,7.64986296190156,
0.));
#202238=CARTESIAN_POINT('Ctrl Pts',(-22.0081253540773,7.64851307293346,
0.));
#202239=CARTESIAN_POINT('Ctrl Pts',(-21.9912478718542,7.64712464805258,
0.));
#202240=CARTESIAN_POINT('Ctrl Pts',(-21.97450807008,7.64569840177359,0.));
#202241=CARTESIAN_POINT('Ctrl Pts',(-21.9579072237653,7.64423506279153,
0.));
#202242=CARTESIAN_POINT('Ctrl Pts',(-21.9414466292074,7.64273537442706,
0.));
#202243=CARTESIAN_POINT('Ctrl Pts',(-21.9251276046546,7.6412000950654,0.));
#202244=CARTESIAN_POINT('Ctrl Pts',(-21.9089514909873,7.63962999860916,
0.));
#202245=CARTESIAN_POINT('Ctrl Pts',(-21.8929196523511,7.63802587492007,
0.));
#202246=CARTESIAN_POINT('Ctrl Pts',(-21.8770334769492,7.63638853033367,
0.));
#202247=CARTESIAN_POINT('Ctrl Pts',(-21.8612943779086,7.63471878821203,
0.));
#202248=CARTESIAN_POINT('Ctrl Pts',(-21.8457037941084,7.63301748948936,
0.));
#202249=CARTESIAN_POINT('Ctrl Pts',(-21.8302631910197,7.6312854932304,0.));
#202250=CARTESIAN_POINT('Ctrl Pts',(-21.8149740615093,7.62952367718151,
0.));
#202251=CARTESIAN_POINT('Ctrl Pts',(-21.7998379268583,7.62773293842409,
0.));
#202252=CARTESIAN_POINT('Ctrl Pts',(-21.7848563378022,7.62591419404521,
0.));
#202253=CARTESIAN_POINT('Ctrl Pts',(-21.7700308755583,7.62406838181164,
0.));
#202254=CARTESIAN_POINT('Ctrl Pts',(-21.7553631528329,7.62219646084226,
0.));
#202255=CARTESIAN_POINT('Ctrl Pts',(-21.7408548148657,7.62029941230855,
0.));
#202256=CARTESIAN_POINT('Ctrl Pts',(-21.7265075407977,7.61837824030541,
0.));
#202257=CARTESIAN_POINT('Ctrl Pts',(-21.7123230449835,7.61643397270425,
0.));
#202258=CARTESIAN_POINT('Ctrl Pts',(-21.6983030783321,7.61446766202787,
0.));
#202259=CARTESIAN_POINT('Ctrl Pts',(-21.6844494295813,7.61248038630265,
0.));
#202260=CARTESIAN_POINT('Ctrl Pts',(-21.6707639267573,7.6104732500095,0.));
#202261=CARTESIAN_POINT('Ctrl Pts',(-21.6572484388079,7.60844738512872,
0.));
#202262=CARTESIAN_POINT('Ctrl Pts',(-21.6439048771743,7.60640395216358,
0.));
#202263=CARTESIAN_POINT('Ctrl Pts',(-21.6307351973823,7.604344141183,0.));
#202264=CARTESIAN_POINT('Ctrl Pts',(-21.6177414005991,7.60226917285432,
0.));
#202265=CARTESIAN_POINT('Ctrl Pts',(-21.6049255358843,7.60018029988238,
0.));
#202266=CARTESIAN_POINT('Ctrl Pts',(-21.5922897024466,7.59807880846192,
0.));
#202267=CARTESIAN_POINT('Ctrl Pts',(-21.5798360518978,7.59596601973588,
0.));
#202268=CARTESIAN_POINT('Ctrl Pts',(-21.5675667904728,7.5938432912493,0.));
#202269=CARTESIAN_POINT('Ctrl Pts',(-21.5554841813465,7.59171201844793,
0.));
#202270=CARTESIAN_POINT('Ctrl Pts',(-21.5435905470113,7.58957363620026,
0.));
#202271=CARTESIAN_POINT('Ctrl Pts',(-21.5318882716735,7.58742962034834,
0.));
#202272=CARTESIAN_POINT('Ctrl Pts',(-21.5203798035294,7.58528148919113,
0.));
#202273=CARTESIAN_POINT('Ctrl Pts',(-21.5090676573866,7.58313080519158,
0.));
#202274=CARTESIAN_POINT('Ctrl Pts',(-21.497954419274,7.5809791779073,0.));
#202275=CARTESIAN_POINT('Ctrl Pts',(-21.4870427508193,7.57882826679131,
0.));
#202276=CARTESIAN_POINT('Ctrl Pts',(-21.4763353936766,7.57667978403002,
0.));
#202277=CARTESIAN_POINT('Ctrl Pts',(-21.4658351740135,7.57453549743435,
0.));
#202278=CARTESIAN_POINT('Ctrl Pts',(-21.4555450053147,7.57239723223521,
0.));
#202279=CARTESIAN_POINT('Ctrl Pts',(-21.445467890751,7.57026687261169,0.));
#202280=CARTESIAN_POINT('Ctrl Pts',(-21.435606926151,7.56814636360842,0.));
#202281=CARTESIAN_POINT('Ctrl Pts',(-21.4259653015732,7.56603771218706,
0.));
#202282=CARTESIAN_POINT('Ctrl Pts',(-21.4165463106252,7.56394299313682,
0.));
#202283=CARTESIAN_POINT('Ctrl Pts',(-21.4073533630364,7.56186435703622,
0.));
#202284=CARTESIAN_POINT('Ctrl Pts',(-21.3983899952988,7.55980403700615,
0.));
#202285=CARTESIAN_POINT('Ctrl Pts',(-21.3896598842119,7.55776435731422,
0.));
#202286=CARTESIAN_POINT('Ctrl Pts',(-21.3811668478933,7.55574773403507,
0.));
#202287=CARTESIAN_POINT('Ctrl Pts',(-21.3729148390244,7.55375667080032,
0.));
#202288=CARTESIAN_POINT('Ctrl Pts',(-21.3649079431864,7.55179375777441,
0.));
#202289=CARTESIAN_POINT('Ctrl Pts',(-21.3571503685853,7.54986166521306,
0.));
#202290=CARTESIAN_POINT('Ctrl Pts',(-21.349646476153,7.54796316246327,0.));
#202291=CARTESIAN_POINT('Ctrl Pts',(-21.3424008295038,7.54610114948351,
0.));
#202292=CARTESIAN_POINT('Ctrl Pts',(-21.3354182340149,7.54427868151268,
0.));
#202293=CARTESIAN_POINT('Ctrl Pts',(-21.328703791771,7.54249900377031,0.));
#202294=CARTESIAN_POINT('Ctrl Pts',(-21.3222628524165,7.5407655203828,0.));
#202295=CARTESIAN_POINT('Ctrl Pts',(-21.3161009456256,7.53908175169899,
0.));
#202296=CARTESIAN_POINT('Ctrl Pts',(-21.3102237167729,7.53745129364619,
0.));
#202297=CARTESIAN_POINT('Ctrl Pts',(-21.3046368712156,7.53587778251743,
0.));
#202298=CARTESIAN_POINT('Ctrl Pts',(-21.2993464250717,7.53436505309949,
0.));
#202299=CARTESIAN_POINT('Ctrl Pts',(-21.2943588989331,7.53291726078526,
0.));
#202300=CARTESIAN_POINT('Ctrl Pts',(-21.2896816163843,7.53153906987847,
0.));
#202301=CARTESIAN_POINT('Ctrl Pts',(-21.2853226580658,7.53023562438221,
0.));
#202302=CARTESIAN_POINT('Ctrl Pts',(-21.2812902781143,7.52901217930407,
0.));
#202303=CARTESIAN_POINT('Ctrl Pts',(-21.2775925269651,7.52787386225343,
0.));
#202304=CARTESIAN_POINT('Ctrl Pts',(-21.2742366113578,7.5268252691856,0.));
#202305=CARTESIAN_POINT('Ctrl Pts',(-21.2712301573465,7.52587126095544,
0.));
#202306=CARTESIAN_POINT('Ctrl Pts',(-21.2685823838672,7.52501770333522,
0.));
#202307=CARTESIAN_POINT('Ctrl Pts',(-21.266305915706,7.52427261074264,0.));
#202308=CARTESIAN_POINT('Ctrl Pts',(-21.2644161259965,7.52364573027521,
0.));
#202309=CARTESIAN_POINT('Ctrl Pts',(-21.262927782038,7.52314642316202,0.));
#202310=CARTESIAN_POINT('Ctrl Pts',(-21.261852128355,7.52278182242727,0.));
#202311=CARTESIAN_POINT('Ctrl Pts',(-21.2613260540651,7.52260064231736,
0.));
#202312=CARTESIAN_POINT('Ctrl Pts',(-21.261120447486,7.52252744144958,0.));
#202313=CARTESIAN_POINT('Ctrl Pts',(-21.2610673466883,7.52250649703992,
0.));
#202314=CARTESIAN_POINT('Ctrl Pts',(-21.2610617890679,7.52250298901265,
0.));
#202315=CARTESIAN_POINT('',(-24.9347862158358,7.36589684767345,0.));
#202316=CARTESIAN_POINT('Ctrl Pts',(-20.353053841303,9.71462809124917,0.));
#202317=CARTESIAN_POINT('Ctrl Pts',(-20.353053841303,9.71462809124917,12.));
#202318=CARTESIAN_POINT('Ctrl Pts',(-20.353060251684,9.71462954053074,0.));
#202319=CARTESIAN_POINT('Ctrl Pts',(-20.353060251684,9.71462954053074,12.));
#202320=CARTESIAN_POINT('Ctrl Pts',(-20.3531126095522,9.71465227853122,
0.));
#202321=CARTESIAN_POINT('Ctrl Pts',(-20.3531126095522,9.71465227853122,
12.));
#202322=CARTESIAN_POINT('Ctrl Pts',(-20.3533097561886,9.71474590350791,
0.));
#202323=CARTESIAN_POINT('Ctrl Pts',(-20.3533097561886,9.71474590350791,
12.));
#202324=CARTESIAN_POINT('Ctrl Pts',(-20.3538098605706,9.71498978052101,
0.));
#202325=CARTESIAN_POINT('Ctrl Pts',(-20.3538098605706,9.71498978052101,
12.));
#202326=CARTESIAN_POINT('Ctrl Pts',(-20.3548282742361,9.71549257088175,
0.));
#202327=CARTESIAN_POINT('Ctrl Pts',(-20.3548282742361,9.71549257088175,
12.));
#202328=CARTESIAN_POINT('Ctrl Pts',(-20.3562337557875,9.71619192554147,
0.));
#202329=CARTESIAN_POINT('Ctrl Pts',(-20.3562337557875,9.71619192554147,
12.));
#202330=CARTESIAN_POINT('Ctrl Pts',(-20.3580133103357,9.71708493723061,
0.));
#202331=CARTESIAN_POINT('Ctrl Pts',(-20.3580133103357,9.71708493723061,
12.));
#202332=CARTESIAN_POINT('Ctrl Pts',(-20.3601498764344,9.71816778327999,
0.));
#202333=CARTESIAN_POINT('Ctrl Pts',(-20.3601498764344,9.71816778327999,
12.));
#202334=CARTESIAN_POINT('Ctrl Pts',(-20.362625691398,9.71943648548114,0.));
#202335=CARTESIAN_POINT('Ctrl Pts',(-20.362625691398,9.71943648548114,12.));
#202336=CARTESIAN_POINT('Ctrl Pts',(-20.3654261611055,9.72088778381102,
0.));
#202337=CARTESIAN_POINT('Ctrl Pts',(-20.3654261611055,9.72088778381102,
12.));
#202338=CARTESIAN_POINT('Ctrl Pts',(-20.3685406190576,9.72251930722504,
0.));
#202339=CARTESIAN_POINT('Ctrl Pts',(-20.3685406190576,9.72251930722504,
12.));
#202340=CARTESIAN_POINT('Ctrl Pts',(-20.371960235676,9.72432910043193,0.));
#202341=CARTESIAN_POINT('Ctrl Pts',(-20.371960235676,9.72432910043193,12.));
#202342=CARTESIAN_POINT('Ctrl Pts',(-20.3756766651952,9.72631531732871,
0.));
#202343=CARTESIAN_POINT('Ctrl Pts',(-20.3756766651952,9.72631531732871,
12.));
#202344=CARTESIAN_POINT('Ctrl Pts',(-20.3796805893304,9.72847589116533,
0.));
#202345=CARTESIAN_POINT('Ctrl Pts',(-20.3796805893304,9.72847589116533,
12.));
#202346=CARTESIAN_POINT('Ctrl Pts',(-20.3839624556742,9.73080870123726,
0.));
#202347=CARTESIAN_POINT('Ctrl Pts',(-20.3839624556742,9.73080870123726,
12.));
#202348=CARTESIAN_POINT('Ctrl Pts',(-20.3885129129912,9.73331167102812,
0.));
#202349=CARTESIAN_POINT('Ctrl Pts',(-20.3885129129912,9.73331167102812,
12.));
#202350=CARTESIAN_POINT('Ctrl Pts',(-20.3933234845646,9.7359829201425,0.));
#202351=CARTESIAN_POINT('Ctrl Pts',(-20.3933234845646,9.7359829201425,12.));
#202352=CARTESIAN_POINT('Ctrl Pts',(-20.3983866213331,9.73882077613206,
0.));
#202353=CARTESIAN_POINT('Ctrl Pts',(-20.3983866213331,9.73882077613206,
12.));
#202354=CARTESIAN_POINT('Ctrl Pts',(-20.4036953576549,9.74182369656272,
0.));
#202355=CARTESIAN_POINT('Ctrl Pts',(-20.4036953576549,9.74182369656272,
12.));
#202356=CARTESIAN_POINT('Ctrl Pts',(-20.4092430879861,9.74499021838536,
0.));
#202357=CARTESIAN_POINT('Ctrl Pts',(-20.4092430879861,9.74499021838536,
12.));
#202358=CARTESIAN_POINT('Ctrl Pts',(-20.4150232777393,9.74831889242175,
0.));
#202359=CARTESIAN_POINT('Ctrl Pts',(-20.4150232777393,9.74831889242175,
12.));
#202360=CARTESIAN_POINT('Ctrl Pts',(-20.4210295275818,9.75180829786433,
0.));
#202361=CARTESIAN_POINT('Ctrl Pts',(-20.4210295275818,9.75180829786433,
12.));
#202362=CARTESIAN_POINT('Ctrl Pts',(-20.4272556476629,9.75545705902416,
0.));
#202363=CARTESIAN_POINT('Ctrl Pts',(-20.4272556476629,9.75545705902416,
12.));
#202364=CARTESIAN_POINT('Ctrl Pts',(-20.4336957355474,9.7592638628993,0.));
#202365=CARTESIAN_POINT('Ctrl Pts',(-20.4336957355474,9.7592638628993,12.));
#202366=CARTESIAN_POINT('Ctrl Pts',(-20.4403442329401,9.76322747195502,
0.));
#202367=CARTESIAN_POINT('Ctrl Pts',(-20.4403442329401,9.76322747195502,
12.));
#202368=CARTESIAN_POINT('Ctrl Pts',(-20.447195862298,9.76734670980897,0.));
#202369=CARTESIAN_POINT('Ctrl Pts',(-20.447195862298,9.76734670980897,12.));
#202370=CARTESIAN_POINT('Ctrl Pts',(-20.4542455817527,9.7716204510407,0.));
#202371=CARTESIAN_POINT('Ctrl Pts',(-20.4542455817527,9.7716204510407,12.));
#202372=CARTESIAN_POINT('Ctrl Pts',(-20.4614885274973,9.77604760815523,
0.));
#202373=CARTESIAN_POINT('Ctrl Pts',(-20.4614885274973,9.77604760815523,
12.));
#202374=CARTESIAN_POINT('Ctrl Pts',(-20.4689199790668,9.78062712373313,
0.));
#202375=CARTESIAN_POINT('Ctrl Pts',(-20.4689199790668,9.78062712373313,
12.));
#202376=CARTESIAN_POINT('Ctrl Pts',(-20.4765353711585,9.78535797314162,
0.));
#202377=CARTESIAN_POINT('Ctrl Pts',(-20.4765353711585,9.78535797314162,
12.));
#202378=CARTESIAN_POINT('Ctrl Pts',(-20.4843302955329,9.7902391649866,0.));
#202379=CARTESIAN_POINT('Ctrl Pts',(-20.4843302955329,9.7902391649866,12.));
#202380=CARTESIAN_POINT('Ctrl Pts',(-20.4923005087945,9.79526974288344,
0.));
#202381=CARTESIAN_POINT('Ctrl Pts',(-20.4923005087945,9.79526974288344,
12.));
#202382=CARTESIAN_POINT('Ctrl Pts',(-20.500441931211,9.80044878520967,0.));
#202383=CARTESIAN_POINT('Ctrl Pts',(-20.500441931211,9.80044878520967,12.));
#202384=CARTESIAN_POINT('Ctrl Pts',(-20.5087506310507,9.80577540161103,
0.));
#202385=CARTESIAN_POINT('Ctrl Pts',(-20.5087506310507,9.80577540161103,
12.));
#202386=CARTESIAN_POINT('Ctrl Pts',(-20.5172228122839,9.81124873025278,
0.));
#202387=CARTESIAN_POINT('Ctrl Pts',(-20.5172228122839,9.81124873025278,
12.));
#202388=CARTESIAN_POINT('Ctrl Pts',(-20.5258548000625,9.81686793455918,
0.));
#202389=CARTESIAN_POINT('Ctrl Pts',(-20.5258548000625,9.81686793455918,
12.));
#202390=CARTESIAN_POINT('Ctrl Pts',(-20.534643029951,9.82263220080328,0.));
#202391=CARTESIAN_POINT('Ctrl Pts',(-20.534643029951,9.82263220080328,12.));
#202392=CARTESIAN_POINT('Ctrl Pts',(-20.5435840460717,9.82854073773857,
0.));
#202393=CARTESIAN_POINT('Ctrl Pts',(-20.5435840460717,9.82854073773857,
12.));
#202394=CARTESIAN_POINT('Ctrl Pts',(-20.5526744976461,9.83459277585321,
0.));
#202395=CARTESIAN_POINT('Ctrl Pts',(-20.5526744976461,9.83459277585321,
12.));
#202396=CARTESIAN_POINT('Ctrl Pts',(-20.5619111362406,9.84078756677589,
0.));
#202397=CARTESIAN_POINT('Ctrl Pts',(-20.5619111362406,9.84078756677589,
12.));
#202398=CARTESIAN_POINT('Ctrl Pts',(-20.5712908125145,9.84712438256308,
0.));
#202399=CARTESIAN_POINT('Ctrl Pts',(-20.5712908125145,9.84712438256308,
12.));
#202400=CARTESIAN_POINT('Ctrl Pts',(-20.580810471002,9.85360251457004,0.));
#202401=CARTESIAN_POINT('Ctrl Pts',(-20.580810471002,9.85360251457004,12.));
#202402=CARTESIAN_POINT('Ctrl Pts',(-20.5904671449754,9.86022127232749,
0.));
#202403=CARTESIAN_POINT('Ctrl Pts',(-20.5904671449754,9.86022127232749,
12.));
#202404=CARTESIAN_POINT('Ctrl Pts',(-20.6002579513696,9.86697998242612,
0.));
#202405=CARTESIAN_POINT('Ctrl Pts',(-20.6002579513696,9.86697998242612,
12.));
#202406=CARTESIAN_POINT('Ctrl Pts',(-20.6101800854491,9.87387798732944,
0.));
#202407=CARTESIAN_POINT('Ctrl Pts',(-20.6101800854491,9.87387798732944,
12.));
#202408=CARTESIAN_POINT('Ctrl Pts',(-20.6202308177472,9.88091464472669,
0.));
#202409=CARTESIAN_POINT('Ctrl Pts',(-20.6202308177472,9.88091464472669,
12.));
#202410=CARTESIAN_POINT('Ctrl Pts',(-20.6304074914086,9.88808932697305,
0.));
#202411=CARTESIAN_POINT('Ctrl Pts',(-20.6304074914086,9.88808932697305,
12.));
#202412=CARTESIAN_POINT('Ctrl Pts',(-20.6407075193977,9.89540142049124,
0.));
#202413=CARTESIAN_POINT('Ctrl Pts',(-20.6407075193977,9.89540142049124,
12.));
#202414=CARTESIAN_POINT('Ctrl Pts',(-20.6511283817415,9.90285032516696,
0.));
#202415=CARTESIAN_POINT('Ctrl Pts',(-20.6511283817415,9.90285032516696,
12.));
#202416=CARTESIAN_POINT('Ctrl Pts',(-20.6616676228315,9.91043545377004,
0.));
#202417=CARTESIAN_POINT('Ctrl Pts',(-20.6616676228315,9.91043545377004,
12.));
#202418=CARTESIAN_POINT('Ctrl Pts',(-20.6723228488262,9.91815623141284,
0.));
#202419=CARTESIAN_POINT('Ctrl Pts',(-20.6723228488262,9.91815623141284,
12.));
#202420=CARTESIAN_POINT('Ctrl Pts',(-20.6830917250255,9.9260120949875,0.));
#202421=CARTESIAN_POINT('Ctrl Pts',(-20.6830917250255,9.9260120949875,12.));
#202422=CARTESIAN_POINT('Ctrl Pts',(-20.6939719732485,9.93400249259736,
0.));
#202423=CARTESIAN_POINT('Ctrl Pts',(-20.6939719732485,9.93400249259736,
12.));
#202424=CARTESIAN_POINT('Ctrl Pts',(-20.7049613692237,9.94212688298251,
0.));
#202425=CARTESIAN_POINT('Ctrl Pts',(-20.7049613692237,9.94212688298251,
12.));
#202426=CARTESIAN_POINT('Ctrl Pts',(-20.716057740758,9.95038473514962,0.));
#202427=CARTESIAN_POINT('Ctrl Pts',(-20.716057740758,9.95038473514962,12.));
#202428=CARTESIAN_POINT('Ctrl Pts',(-20.7272589658752,9.95877552798403,
0.));
#202429=CARTESIAN_POINT('Ctrl Pts',(-20.7272589658752,9.95877552798403,
12.));
#202430=CARTESIAN_POINT('Ctrl Pts',(-20.7385629709795,9.96729874986198,
0.));
#202431=CARTESIAN_POINT('Ctrl Pts',(-20.7385629709795,9.96729874986198,
12.));
#202432=CARTESIAN_POINT('Ctrl Pts',(-20.7499677289625,9.97595389823461,
0.));
#202433=CARTESIAN_POINT('Ctrl Pts',(-20.7499677289625,9.97595389823461,
12.));
#202434=CARTESIAN_POINT('Ctrl Pts',(-20.7614712574989,9.98474047926846,
0.));
#202435=CARTESIAN_POINT('Ctrl Pts',(-20.7614712574989,9.98474047926846,
12.));
#202436=CARTESIAN_POINT('Ctrl Pts',(-20.7730716175417,9.99365800754638,
0.));
#202437=CARTESIAN_POINT('Ctrl Pts',(-20.7730716175417,9.99365800754638,
12.));
#202438=CARTESIAN_POINT('Ctrl Pts',(-20.7847669117568,10.0027060057389,
0.));
#202439=CARTESIAN_POINT('Ctrl Pts',(-20.7847669117568,10.0027060057389,
12.));
#202440=CARTESIAN_POINT('Ctrl Pts',(-20.7965552829907,10.0118840042786,
0.));
#202441=CARTESIAN_POINT('Ctrl Pts',(-20.7965552829907,10.0118840042786,
12.));
#202442=CARTESIAN_POINT('Ctrl Pts',(-20.8084349126885,10.0211915410095,
0.));
#202443=CARTESIAN_POINT('Ctrl Pts',(-20.8084349126885,10.0211915410095,
12.));
#202444=CARTESIAN_POINT('Ctrl Pts',(-20.8204040196599,10.0306281609435,
0.));
#202445=CARTESIAN_POINT('Ctrl Pts',(-20.8204040196599,10.0306281609435,
12.));
#202446=CARTESIAN_POINT('Ctrl Pts',(-20.8324608588906,10.0401934160234,
0.));
#202447=CARTESIAN_POINT('Ctrl Pts',(-20.8324608588906,10.0401934160234,
12.));
#202448=CARTESIAN_POINT('Ctrl Pts',(-20.8446037203402,10.0498868648733,
0.));
#202449=CARTESIAN_POINT('Ctrl Pts',(-20.8446037203402,10.0498868648733,
12.));
#202450=CARTESIAN_POINT('Ctrl Pts',(-20.856830927732,10.0597080725375,0.));
#202451=CARTESIAN_POINT('Ctrl Pts',(-20.856830927732,10.0597080725375,12.));
#202452=CARTESIAN_POINT('Ctrl Pts',(-20.8691408373705,10.0696566102219,
0.));
#202453=CARTESIAN_POINT('Ctrl Pts',(-20.8691408373705,10.0696566102219,
12.));
#202454=CARTESIAN_POINT('Ctrl Pts',(-20.8815318371844,10.0797320551154,
0.));
#202455=CARTESIAN_POINT('Ctrl Pts',(-20.8815318371844,10.0797320551154,
12.));
#202456=CARTESIAN_POINT('Ctrl Pts',(-20.8940023457371,10.0899339901916,
0.));
#202457=CARTESIAN_POINT('Ctrl Pts',(-20.8940023457371,10.0899339901916,
12.));
#202458=CARTESIAN_POINT('Ctrl Pts',(-20.9065508112556,10.1002620040076,
0.));
#202459=CARTESIAN_POINT('Ctrl Pts',(-20.9065508112556,10.1002620040076,
12.));
#202460=CARTESIAN_POINT('Ctrl Pts',(-20.9191757106266,10.1107156904836,
0.));
#202461=CARTESIAN_POINT('Ctrl Pts',(-20.9191757106266,10.1107156904836,
12.));
#202462=CARTESIAN_POINT('Ctrl Pts',(-20.931875548473,10.1212946487057,0.));
#202463=CARTESIAN_POINT('Ctrl Pts',(-20.931875548473,10.1212946487057,12.));
#202464=CARTESIAN_POINT('Ctrl Pts',(-20.944648856393,10.1319984827909,0.));
#202465=CARTESIAN_POINT('Ctrl Pts',(-20.944648856393,10.1319984827909,12.));
#202466=CARTESIAN_POINT('Ctrl Pts',(-20.9574941921591,10.1428268017257,
0.));
#202467=CARTESIAN_POINT('Ctrl Pts',(-20.9574941921591,10.1428268017257,
12.));
#202468=CARTESIAN_POINT('Ctrl Pts',(-20.970410138937,10.1537792192065,0.));
#202469=CARTESIAN_POINT('Ctrl Pts',(-20.970410138937,10.1537792192065,12.));
#202470=CARTESIAN_POINT('Ctrl Pts',(-20.9833953044737,10.1648553534567,
0.));
#202471=CARTESIAN_POINT('Ctrl Pts',(-20.9833953044737,10.1648553534567,
12.));
#202472=CARTESIAN_POINT('Ctrl Pts',(-20.9964483203685,10.1760548270765,
0.));
#202473=CARTESIAN_POINT('Ctrl Pts',(-20.9964483203685,10.1760548270765,
12.));
#202474=CARTESIAN_POINT('Ctrl Pts',(-21.0095678414486,10.1873772669358,
0.));
#202475=CARTESIAN_POINT('Ctrl Pts',(-21.0095678414486,10.1873772669358,
12.));
#202476=CARTESIAN_POINT('Ctrl Pts',(-21.0227525451107,10.1988223040425,
0.));
#202477=CARTESIAN_POINT('Ctrl Pts',(-21.0227525451107,10.1988223040425,
12.));
#202478=CARTESIAN_POINT('Ctrl Pts',(-21.0360011306814,10.2103895734123,
0.));
#202479=CARTESIAN_POINT('Ctrl Pts',(-21.0360011306814,10.2103895734123,
12.));
#202480=CARTESIAN_POINT('Ctrl Pts',(-21.0493123187483,10.2220787139157,
0.));
#202481=CARTESIAN_POINT('Ctrl Pts',(-21.0493123187483,10.2220787139157,
12.));
#202482=CARTESIAN_POINT('Ctrl Pts',(-21.0626848505665,10.233889368157,0.));
#202483=CARTESIAN_POINT('Ctrl Pts',(-21.0626848505665,10.233889368157,12.));
#202484=CARTESIAN_POINT('Ctrl Pts',(-21.0761174875448,10.2458211823915,
0.));
#202485=CARTESIAN_POINT('Ctrl Pts',(-21.0761174875448,10.2458211823915,
12.));
#202486=CARTESIAN_POINT('Ctrl Pts',(-21.0896090107066,10.2578738064183,
0.));
#202487=CARTESIAN_POINT('Ctrl Pts',(-21.0896090107066,10.2578738064183,
12.));
#202488=CARTESIAN_POINT('Ctrl Pts',(-21.1031582201625,10.2700468934743,
0.));
#202489=CARTESIAN_POINT('Ctrl Pts',(-21.1031582201625,10.2700468934743,
12.));
#202490=CARTESIAN_POINT('Ctrl Pts',(-21.1167639345623,10.2823401001067,
0.));
#202491=CARTESIAN_POINT('Ctrl Pts',(-21.1167639345623,10.2823401001067,
12.));
#202492=CARTESIAN_POINT('Ctrl Pts',(-21.130424990599,10.2947530860714,0.));
#202493=CARTESIAN_POINT('Ctrl Pts',(-21.130424990599,10.2947530860714,12.));
#202494=CARTESIAN_POINT('Ctrl Pts',(-21.1441402425831,10.307285514268,0.));
#202495=CARTESIAN_POINT('Ctrl Pts',(-21.1441402425831,10.307285514268,12.));
#202496=CARTESIAN_POINT('Ctrl Pts',(-21.1579085619959,10.3199370506541,
0.));
#202497=CARTESIAN_POINT('Ctrl Pts',(-21.1579085619959,10.3199370506541,
12.));
#202498=CARTESIAN_POINT('Ctrl Pts',(-21.1717288370512,10.3327073641574,
0.));
#202499=CARTESIAN_POINT('Ctrl Pts',(-21.1717288370512,10.3327073641574,
12.));
#202500=CARTESIAN_POINT('Ctrl Pts',(-21.1855999722427,10.3455961265706,
0.));
#202501=CARTESIAN_POINT('Ctrl Pts',(-21.1855999722427,10.3455961265706,
12.));
#202502=CARTESIAN_POINT('Ctrl Pts',(-21.1995208879205,10.3586030124595,
0.));
#202503=CARTESIAN_POINT('Ctrl Pts',(-21.1995208879205,10.3586030124595,
12.));
#202504=CARTESIAN_POINT('Ctrl Pts',(-21.2134905199359,10.3717276991137,
0.));
#202505=CARTESIAN_POINT('Ctrl Pts',(-21.2134905199359,10.3717276991137,
12.));
#202506=CARTESIAN_POINT('Ctrl Pts',(-21.2275078192708,10.384969866479,0.));
#202507=CARTESIAN_POINT('Ctrl Pts',(-21.2275078192708,10.384969866479,12.));
#202508=CARTESIAN_POINT('Ctrl Pts',(-21.2415717516713,10.3983291970846,
0.));
#202509=CARTESIAN_POINT('Ctrl Pts',(-21.2415717516713,10.3983291970846,
12.));
#202510=CARTESIAN_POINT('Ctrl Pts',(-21.2556812972741,10.4118053759584,
0.));
#202511=CARTESIAN_POINT('Ctrl Pts',(-21.2556812972741,10.4118053759584,
12.));
#202512=CARTESIAN_POINT('Ctrl Pts',(-21.2698354502391,10.4253980905394,
0.));
#202513=CARTESIAN_POINT('Ctrl Pts',(-21.2698354502391,10.4253980905394,
12.));
#202514=CARTESIAN_POINT('Ctrl Pts',(-21.2840332184471,10.4391070306385,
0.));
#202515=CARTESIAN_POINT('Ctrl Pts',(-21.2840332184471,10.4391070306385,
12.));
#202516=CARTESIAN_POINT('Ctrl Pts',(-21.2982736231924,10.452931888387,0.));
#202517=CARTESIAN_POINT('Ctrl Pts',(-21.2982736231924,10.452931888387,12.));
#202518=CARTESIAN_POINT('Ctrl Pts',(-21.312555698873,10.4668723581768,0.));
#202519=CARTESIAN_POINT('Ctrl Pts',(-21.312555698873,10.4668723581768,12.));
#202520=CARTESIAN_POINT('Ctrl Pts',(-21.3268784926823,10.4809281365933,
0.));
#202521=CARTESIAN_POINT('Ctrl Pts',(-21.3268784926823,10.4809281365933,
12.));
#202522=CARTESIAN_POINT('Ctrl Pts',(-21.3412410642912,10.4950989223341,
0.));
#202523=CARTESIAN_POINT('Ctrl Pts',(-21.3412410642912,10.4950989223341,
12.));
#202524=CARTESIAN_POINT('Ctrl Pts',(-21.3556424855822,10.5093844161689,
0.));
#202525=CARTESIAN_POINT('Ctrl Pts',(-21.3556424855822,10.5093844161689,
12.));
#202526=CARTESIAN_POINT('Ctrl Pts',(-21.3700818403942,10.523784320906,0.));
#202527=CARTESIAN_POINT('Ctrl Pts',(-21.3700818403942,10.523784320906,12.));
#202528=CARTESIAN_POINT('Ctrl Pts',(-21.3845582242604,10.5382983413422,
0.));
#202529=CARTESIAN_POINT('Ctrl Pts',(-21.3845582242604,10.5382983413422,
12.));
#202530=CARTESIAN_POINT('Ctrl Pts',(-21.3990707441495,10.5529261842107,
0.));
#202531=CARTESIAN_POINT('Ctrl Pts',(-21.3990707441495,10.5529261842107,
12.));
#202532=CARTESIAN_POINT('Ctrl Pts',(-21.4136185181974,10.5676675581106,
0.));
#202533=CARTESIAN_POINT('Ctrl Pts',(-21.4136185181974,10.5676675581106,
12.));
#202534=CARTESIAN_POINT('Ctrl Pts',(-21.4282006754624,10.582522173457,0.));
#202535=CARTESIAN_POINT('Ctrl Pts',(-21.4282006754624,10.582522173457,12.));
#202536=CARTESIAN_POINT('Ctrl Pts',(-21.4428163557137,10.597489742462,0.));
#202537=CARTESIAN_POINT('Ctrl Pts',(-21.4428163557137,10.597489742462,12.));
#202538=CARTESIAN_POINT('Ctrl Pts',(-21.4574647092093,10.612569979096,0.));
#202539=CARTESIAN_POINT('Ctrl Pts',(-21.4574647092093,10.612569979096,12.));
#202540=CARTESIAN_POINT('Ctrl Pts',(-21.4721448964766,10.6277625990457,
0.));
#202541=CARTESIAN_POINT('Ctrl Pts',(-21.4721448964766,10.6277625990457,
12.));
#202542=CARTESIAN_POINT('Ctrl Pts',(-21.4868560880893,10.6430673196609,
0.));
#202543=CARTESIAN_POINT('Ctrl Pts',(-21.4868560880893,10.6430673196609,
12.));
#202544=CARTESIAN_POINT('Ctrl Pts',(-21.5015974644454,10.658483859894,0.));
#202545=CARTESIAN_POINT('Ctrl Pts',(-21.5015974644454,10.658483859894,12.));
#202546=CARTESIAN_POINT('Ctrl Pts',(-21.5163682155805,10.6740119402835,
0.));
#202547=CARTESIAN_POINT('Ctrl Pts',(-21.5163682155805,10.6740119402835,
12.));
#202548=CARTESIAN_POINT('Ctrl Pts',(-21.531167540981,10.689651282929,0.));
#202549=CARTESIAN_POINT('Ctrl Pts',(-21.531167540981,10.689651282929,12.));
#202550=CARTESIAN_POINT('Ctrl Pts',(-21.5459946493955,10.7054016114571,
0.));
#202551=CARTESIAN_POINT('Ctrl Pts',(-21.5459946493955,10.7054016114571,
12.));
#202552=CARTESIAN_POINT('Ctrl Pts',(-21.5608487586467,10.7212626509816,
0.));
#202553=CARTESIAN_POINT('Ctrl Pts',(-21.5608487586467,10.7212626509816,
12.));
#202554=CARTESIAN_POINT('Ctrl Pts',(-21.5757290954372,10.7372341280468,
0.));
#202555=CARTESIAN_POINT('Ctrl Pts',(-21.5757290954372,10.7372341280468,
12.));
#202556=CARTESIAN_POINT('Ctrl Pts',(-21.5906348951745,10.7533157705943,
0.));
#202557=CARTESIAN_POINT('Ctrl Pts',(-21.5906348951745,10.7533157705943,
12.));
#202558=CARTESIAN_POINT('Ctrl Pts',(-21.6055654018179,10.7695073079554,
0.));
#202559=CARTESIAN_POINT('Ctrl Pts',(-21.6055654018179,10.7695073079554,
12.));
#202560=CARTESIAN_POINT('Ctrl Pts',(-21.6205198677176,10.7858084708262,
0.));
#202561=CARTESIAN_POINT('Ctrl Pts',(-21.6205198677176,10.7858084708262,
12.));
#202562=CARTESIAN_POINT('Ctrl Pts',(-21.6354975534557,10.8022189912369,
0.));
#202563=CARTESIAN_POINT('Ctrl Pts',(-21.6354975534557,10.8022189912369,
12.));
#202564=CARTESIAN_POINT('Ctrl Pts',(-21.6504977276864,10.8187386025135,
0.));
#202565=CARTESIAN_POINT('Ctrl Pts',(-21.6504977276864,10.8187386025135,
12.));
#202566=CARTESIAN_POINT('Ctrl Pts',(-21.6655196669727,10.835367039227,0.));
#202567=CARTESIAN_POINT('Ctrl Pts',(-21.6655196669727,10.835367039227,12.));
#202568=CARTESIAN_POINT('Ctrl Pts',(-21.6805626556461,10.8521040371832,
0.));
#202569=CARTESIAN_POINT('Ctrl Pts',(-21.6805626556461,10.8521040371832,
12.));
#202570=CARTESIAN_POINT('Ctrl Pts',(-21.6956259856667,10.8689493334093,
0.));
#202571=CARTESIAN_POINT('Ctrl Pts',(-21.6956259856667,10.8689493334093,
12.));
#202572=CARTESIAN_POINT('Ctrl Pts',(-21.7107089564822,10.8859026661292,
0.));
#202573=CARTESIAN_POINT('Ctrl Pts',(-21.7107089564822,10.8859026661292,
12.));
#202574=CARTESIAN_POINT('Ctrl Pts',(-21.7258108748874,10.9029637747341,
0.));
#202575=CARTESIAN_POINT('Ctrl Pts',(-21.7258108748874,10.9029637747341,
12.));
#202576=CARTESIAN_POINT('Ctrl Pts',(-21.74093105488,10.9201323997386,0.));
#202577=CARTESIAN_POINT('Ctrl Pts',(-21.74093105488,10.9201323997386,12.));
#202578=CARTESIAN_POINT('Ctrl Pts',(-21.7560688175252,10.9374082827446,
0.));
#202579=CARTESIAN_POINT('Ctrl Pts',(-21.7560688175252,10.9374082827446,
12.));
#202580=CARTESIAN_POINT('Ctrl Pts',(-21.7712234908468,10.9547911664457,
0.));
#202581=CARTESIAN_POINT('Ctrl Pts',(-21.7712234908468,10.9547911664457,
12.));
#202582=CARTESIAN_POINT('Ctrl Pts',(-21.7863944097143,10.9722807946157,
0.));
#202583=CARTESIAN_POINT('Ctrl Pts',(-21.7863944097143,10.9722807946157,
12.));
#202584=CARTESIAN_POINT('Ctrl Pts',(-21.8015809157302,10.9898769120913,
0.));
#202585=CARTESIAN_POINT('Ctrl Pts',(-21.8015809157302,10.9898769120913,
12.));
#202586=CARTESIAN_POINT('Ctrl Pts',(-21.8167823571168,11.0075792647477,
0.));
#202587=CARTESIAN_POINT('Ctrl Pts',(-21.8167823571168,11.0075792647477,
12.));
#202588=CARTESIAN_POINT('Ctrl Pts',(-21.8319980886033,11.0253875994598,
0.));
#202589=CARTESIAN_POINT('Ctrl Pts',(-21.8319980886033,11.0253875994598,
12.));
#202590=CARTESIAN_POINT('Ctrl Pts',(-21.8472274713103,11.0433016640808,
0.));
#202591=CARTESIAN_POINT('Ctrl Pts',(-21.8472274713103,11.0433016640808,
12.));
#202592=CARTESIAN_POINT('Ctrl Pts',(-21.8624698726319,11.0613212074364,
0.));
#202593=CARTESIAN_POINT('Ctrl Pts',(-21.8624698726319,11.0613212074364,
12.));
#202594=CARTESIAN_POINT('Ctrl Pts',(-21.8777246661191,11.0794459793058,
0.));
#202595=CARTESIAN_POINT('Ctrl Pts',(-21.8777246661191,11.0794459793058,
12.));
#202596=CARTESIAN_POINT('Ctrl Pts',(-21.8929912313608,11.0976757303944,
0.));
#202597=CARTESIAN_POINT('Ctrl Pts',(-21.8929912313608,11.0976757303944,
12.));
#202598=CARTESIAN_POINT('Ctrl Pts',(-21.9082689538687,11.1160102123024,
0.));
#202599=CARTESIAN_POINT('Ctrl Pts',(-21.9082689538687,11.1160102123024,
12.));
#202600=CARTESIAN_POINT('Ctrl Pts',(-21.9235572249518,11.134449177474,0.));
#202601=CARTESIAN_POINT('Ctrl Pts',(-21.9235572249518,11.134449177474,12.));
#202602=CARTESIAN_POINT('Ctrl Pts',(-21.9388554416437,11.1529923792002,
0.));
#202603=CARTESIAN_POINT('Ctrl Pts',(-21.9388554416437,11.1529923792002,
12.));
#202604=CARTESIAN_POINT('Ctrl Pts',(-21.9541630066504,11.1716395716375,
0.));
#202605=CARTESIAN_POINT('Ctrl Pts',(-21.9541630066504,11.1716395716375,
12.));
#202606=CARTESIAN_POINT('Ctrl Pts',(-21.9694793282913,11.1903905098109,
0.));
#202607=CARTESIAN_POINT('Ctrl Pts',(-21.9694793282913,11.1903905098109,
12.));
#202608=CARTESIAN_POINT('Ctrl Pts',(-21.9848038204439,11.2092449496125,
0.));
#202609=CARTESIAN_POINT('Ctrl Pts',(-21.9848038204439,11.2092449496125,
12.));
#202610=CARTESIAN_POINT('Ctrl Pts',(-22.0001359024839,11.2282026477897,
0.));
#202611=CARTESIAN_POINT('Ctrl Pts',(-22.0001359024839,11.2282026477897,
12.));
#202612=CARTESIAN_POINT('Ctrl Pts',(-22.0154749992364,11.2472633619276,
0.));
#202613=CARTESIAN_POINT('Ctrl Pts',(-22.0154749992364,11.2472633619276,
12.));
#202614=CARTESIAN_POINT('Ctrl Pts',(-22.0308205408351,11.2664268504207,
0.));
#202615=CARTESIAN_POINT('Ctrl Pts',(-22.0308205408351,11.2664268504207,
12.));
#202616=CARTESIAN_POINT('Ctrl Pts',(-22.046171962566,11.2856928724374,0.));
#202617=CARTESIAN_POINT('Ctrl Pts',(-22.046171962566,11.2856928724374,12.));
#202618=CARTESIAN_POINT('Ctrl Pts',(-22.0615287047179,11.3050611878771,
0.));
#202619=CARTESIAN_POINT('Ctrl Pts',(-22.0615287047179,11.3050611878771,
12.));
#202620=CARTESIAN_POINT('Ctrl Pts',(-22.0768902124267,11.3245315573168,
0.));
#202621=CARTESIAN_POINT('Ctrl Pts',(-22.0768902124267,11.3245315573168,
12.));
#202622=CARTESIAN_POINT('Ctrl Pts',(-22.0922559355293,11.3441037419553,
0.));
#202623=CARTESIAN_POINT('Ctrl Pts',(-22.0922559355293,11.3441037419553,
12.));
#202624=CARTESIAN_POINT('Ctrl Pts',(-22.1076253283978,11.3637775035367,
0.));
#202625=CARTESIAN_POINT('Ctrl Pts',(-22.1076253283978,11.3637775035367,
12.));
#202626=CARTESIAN_POINT('Ctrl Pts',(-22.1229978500185,11.3835526044256,
0.));
#202627=CARTESIAN_POINT('Ctrl Pts',(-22.1229978500185,11.3835526044256,
12.));
#202628=CARTESIAN_POINT('Ctrl Pts',(-22.1383729640963,11.4034288076908,
0.));
#202629=CARTESIAN_POINT('Ctrl Pts',(-22.1383729640963,11.4034288076908,
12.));
#202630=CARTESIAN_POINT('Ctrl Pts',(-22.1537501391486,11.4234058771742,
0.));
#202631=CARTESIAN_POINT('Ctrl Pts',(-22.1537501391486,11.4234058771742,
12.));
#202632=CARTESIAN_POINT('Ctrl Pts',(-22.1691288486096,11.443483577557,0.));
#202633=CARTESIAN_POINT('Ctrl Pts',(-22.1691288486096,11.443483577557,12.));
#202634=CARTESIAN_POINT('Ctrl Pts',(-22.184508570917,11.463661674411,0.));
#202635=CARTESIAN_POINT('Ctrl Pts',(-22.184508570917,11.463661674411,12.));
#202636=CARTESIAN_POINT('Ctrl Pts',(-22.1998887896435,11.4839399342589,
0.));
#202637=CARTESIAN_POINT('Ctrl Pts',(-22.1998887896435,11.4839399342589,
12.));
#202638=CARTESIAN_POINT('Ctrl Pts',(-22.215268993102,11.504318124424,0.));
#202639=CARTESIAN_POINT('Ctrl Pts',(-22.215268993102,11.504318124424,12.));
#202640=CARTESIAN_POINT('Ctrl Pts',(-22.2306486738899,11.5247960128476,
0.));
#202641=CARTESIAN_POINT('Ctrl Pts',(-22.2306486738899,11.5247960128476,
12.));
#202642=CARTESIAN_POINT('Ctrl Pts',(-22.2460273284653,11.545373367912,0.));
#202643=CARTESIAN_POINT('Ctrl Pts',(-22.2460273284653,11.545373367912,12.));
#202644=CARTESIAN_POINT('Ctrl Pts',(-22.2614044566898,11.5660499582403,
0.));
#202645=CARTESIAN_POINT('Ctrl Pts',(-22.2614044566898,11.5660499582403,
12.));
#202646=CARTESIAN_POINT('Ctrl Pts',(-22.2767795614349,11.5868255525189,
0.));
#202647=CARTESIAN_POINT('Ctrl Pts',(-22.2767795614349,11.5868255525189,
12.));
#202648=CARTESIAN_POINT('Ctrl Pts',(-22.2921521480358,11.6076999192359,
0.));
#202649=CARTESIAN_POINT('Ctrl Pts',(-22.2921521480358,11.6076999192359,
12.));
#202650=CARTESIAN_POINT('Ctrl Pts',(-22.3075217249049,11.6286728270011,
0.));
#202651=CARTESIAN_POINT('Ctrl Pts',(-22.3075217249049,11.6286728270011,
12.));
#202652=CARTESIAN_POINT('Ctrl Pts',(-22.3228878043976,11.6497440449858,
0.));
#202653=CARTESIAN_POINT('Ctrl Pts',(-22.3228878043976,11.6497440449858,
12.));
#202654=CARTESIAN_POINT('Ctrl Pts',(-22.3382499035618,11.6709133432986,
0.));
#202655=CARTESIAN_POINT('Ctrl Pts',(-22.3382499035618,11.6709133432986,
12.));
#202656=CARTESIAN_POINT('Ctrl Pts',(-22.3536075450028,11.6921804934056,
0.));
#202657=CARTESIAN_POINT('Ctrl Pts',(-22.3536075450028,11.6921804934056,
12.));
#202658=CARTESIAN_POINT('Ctrl Pts',(-22.3689602575492,11.7135452684532,
0.));
#202659=CARTESIAN_POINT('Ctrl Pts',(-22.3689602575492,11.7135452684532,
12.));
#202660=CARTESIAN_POINT('Ctrl Pts',(-22.3843075773905,11.7350074437961,
0.));
#202661=CARTESIAN_POINT('Ctrl Pts',(-22.3843075773905,11.7350074437961,
12.));
#202662=CARTESIAN_POINT('Ctrl Pts',(-22.39964904692,11.7565667964765,0.));
#202663=CARTESIAN_POINT('Ctrl Pts',(-22.39964904692,11.7565667964765,12.));
#202664=CARTESIAN_POINT('Ctrl Pts',(-22.4149842125018,11.7782231042041,
0.));
#202665=CARTESIAN_POINT('Ctrl Pts',(-22.4149842125018,11.7782231042041,
12.));
#202666=CARTESIAN_POINT('Ctrl Pts',(-22.4303126226468,11.7999761445175,
0.));
#202667=CARTESIAN_POINT('Ctrl Pts',(-22.4303126226468,11.7999761445175,
12.));
#202668=CARTESIAN_POINT('Ctrl Pts',(-22.4456338258738,11.8218256937889,
0.));
#202669=CARTESIAN_POINT('Ctrl Pts',(-22.4456338258738,11.8218256937889,
12.));
#202670=CARTESIAN_POINT('Ctrl Pts',(-22.4609473690469,11.8437715264487,
0.));
#202671=CARTESIAN_POINT('Ctrl Pts',(-22.4609473690469,11.8437715264487,
12.));
#202672=CARTESIAN_POINT('Ctrl Pts',(-22.4762527946694,11.8658134137018,
0.));
#202673=CARTESIAN_POINT('Ctrl Pts',(-22.4762527946694,11.8658134137018,
12.));
#202674=CARTESIAN_POINT('Ctrl Pts',(-22.4915496418472,11.8879511239941,
0.));
#202675=CARTESIAN_POINT('Ctrl Pts',(-22.4915496418472,11.8879511239941,
12.));
#202676=CARTESIAN_POINT('Ctrl Pts',(-22.5068374513958,11.9101844254555,
0.));
#202677=CARTESIAN_POINT('Ctrl Pts',(-22.5068374513958,11.9101844254555,
12.));
#202678=CARTESIAN_POINT('Ctrl Pts',(-22.5221157697869,11.9325130877801,
0.));
#202679=CARTESIAN_POINT('Ctrl Pts',(-22.5221157697869,11.9325130877801,
12.));
#202680=CARTESIAN_POINT('Ctrl Pts',(-22.5373841537299,11.9549368843996,
0.));
#202681=CARTESIAN_POINT('Ctrl Pts',(-22.5373841537299,11.9549368843996,
12.));
#202682=CARTESIAN_POINT('Ctrl Pts',(-22.5526421741159,11.9774555943496,
0.));
#202683=CARTESIAN_POINT('Ctrl Pts',(-22.5526421741159,11.9774555943496,
12.));
#202684=CARTESIAN_POINT('Ctrl Pts',(-22.5678894211194,12.0000690046697,
0.));
#202685=CARTESIAN_POINT('Ctrl Pts',(-22.5678894211194,12.0000690046697,
12.));
#202686=CARTESIAN_POINT('Ctrl Pts',(-22.5831255061306,12.0227769113132,
0.));
#202687=CARTESIAN_POINT('Ctrl Pts',(-22.5831255061306,12.0227769113132,
12.));
#202688=CARTESIAN_POINT('Ctrl Pts',(-22.5983500505675,12.0455791139135,
0.));
#202689=CARTESIAN_POINT('Ctrl Pts',(-22.5983500505675,12.0455791139135,
12.));
#202690=CARTESIAN_POINT('Ctrl Pts',(-22.613562676493,12.0684754113869,0.));
#202691=CARTESIAN_POINT('Ctrl Pts',(-22.613562676493,12.0684754113869,12.));
#202692=CARTESIAN_POINT('Ctrl Pts',(-22.628762996708,12.0914655972828,0.));
#202693=CARTESIAN_POINT('Ctrl Pts',(-22.628762996708,12.0914655972828,12.));
#202694=CARTESIAN_POINT('Ctrl Pts',(-22.6439506046611,12.1145494550384,
0.));
#202695=CARTESIAN_POINT('Ctrl Pts',(-22.6439506046611,12.1145494550384,
12.));
#202696=CARTESIAN_POINT('Ctrl Pts',(-22.6591250653942,12.1377267537141,
0.));
#202697=CARTESIAN_POINT('Ctrl Pts',(-22.6591250653942,12.1377267537141,
12.));
#202698=CARTESIAN_POINT('Ctrl Pts',(-22.6742859034891,12.1609972423088,
0.));
#202699=CARTESIAN_POINT('Ctrl Pts',(-22.6742859034891,12.1609972423088,
12.));
#202700=CARTESIAN_POINT('Ctrl Pts',(-22.6894326204959,12.1843606579246,
0.));
#202701=CARTESIAN_POINT('Ctrl Pts',(-22.6894326204959,12.1843606579246,
12.));
#202702=CARTESIAN_POINT('Ctrl Pts',(-22.7045647168659,12.2078167360267,
0.));
#202703=CARTESIAN_POINT('Ctrl Pts',(-22.7045647168659,12.2078167360267,
12.));
#202704=CARTESIAN_POINT('Ctrl Pts',(-22.7196817119299,12.2313652198047,
0.));
#202705=CARTESIAN_POINT('Ctrl Pts',(-22.7196817119299,12.2313652198047,
12.));
#202706=CARTESIAN_POINT('Ctrl Pts',(-22.7347831655251,12.2550058702389,
0.));
#202707=CARTESIAN_POINT('Ctrl Pts',(-22.7347831655251,12.2550058702389,
12.));
#202708=CARTESIAN_POINT('Ctrl Pts',(-22.7498686970096,12.2787384750747,
0.));
#202709=CARTESIAN_POINT('Ctrl Pts',(-22.7498686970096,12.2787384750747,
12.));
#202710=CARTESIAN_POINT('Ctrl Pts',(-22.7649380101154,12.3025628601812,
0.));
#202711=CARTESIAN_POINT('Ctrl Pts',(-22.7649380101154,12.3025628601812,
12.));
#202712=CARTESIAN_POINT('Ctrl Pts',(-22.7799908974947,12.3264788926108,
0.));
#202713=CARTESIAN_POINT('Ctrl Pts',(-22.7799908974947,12.3264788926108,
12.));
#202714=CARTESIAN_POINT('Ctrl Pts',(-22.7950272216959,12.3504864740361,
0.));
#202715=CARTESIAN_POINT('Ctrl Pts',(-22.7950272216959,12.3504864740361,
12.));
#202716=CARTESIAN_POINT('Ctrl Pts',(-22.8100469022632,12.3745855366772,
0.));
#202717=CARTESIAN_POINT('Ctrl Pts',(-22.8100469022632,12.3745855366772,
12.));
#202718=CARTESIAN_POINT('Ctrl Pts',(-22.8220493007353,12.393937937903,0.));
#202719=CARTESIAN_POINT('Ctrl Pts',(-22.8220493007353,12.393937937903,12.));
#202720=CARTESIAN_POINT('Ctrl Pts',(-22.8310435872852,12.4084933766366,
0.));
#202721=CARTESIAN_POINT('Ctrl Pts',(-22.8310435872852,12.4084933766366,
12.));
#202722=CARTESIAN_POINT('Ctrl Pts',(-22.8370364396497,12.4182152851867,
0.));
#202723=CARTESIAN_POINT('Ctrl Pts',(-22.8370364396497,12.4182152851867,
12.));
#202724=CARTESIAN_POINT('Ctrl Pts',(-22.8400320311648,12.4230808101438,
0.));
#202725=CARTESIAN_POINT('Ctrl Pts',(-22.8400320311648,12.4230808101438,
12.));
#202726=CARTESIAN_POINT('',(-22.8400320311648,12.4230808101438,0.));
#202727=CARTESIAN_POINT('Ctrl Pts',(-20.353053841303,9.71462809124917,0.));
#202728=CARTESIAN_POINT('Ctrl Pts',(-20.353060251684,9.71462954053074,0.));
#202729=CARTESIAN_POINT('Ctrl Pts',(-20.3531126095522,9.71465227853122,
0.));
#202730=CARTESIAN_POINT('Ctrl Pts',(-20.3533097561886,9.71474590350791,
0.));
#202731=CARTESIAN_POINT('Ctrl Pts',(-20.3538098605706,9.71498978052101,
0.));
#202732=CARTESIAN_POINT('Ctrl Pts',(-20.3548282742361,9.71549257088175,
0.));
#202733=CARTESIAN_POINT('Ctrl Pts',(-20.3562337557875,9.71619192554147,
0.));
#202734=CARTESIAN_POINT('Ctrl Pts',(-20.3580133103357,9.71708493723061,
0.));
#202735=CARTESIAN_POINT('Ctrl Pts',(-20.3601498764344,9.71816778327999,
0.));
#202736=CARTESIAN_POINT('Ctrl Pts',(-20.362625691398,9.71943648548114,0.));
#202737=CARTESIAN_POINT('Ctrl Pts',(-20.3654261611055,9.72088778381102,
0.));
#202738=CARTESIAN_POINT('Ctrl Pts',(-20.3685406190576,9.72251930722504,
0.));
#202739=CARTESIAN_POINT('Ctrl Pts',(-20.371960235676,9.72432910043193,0.));
#202740=CARTESIAN_POINT('Ctrl Pts',(-20.3756766651952,9.72631531732871,
0.));
#202741=CARTESIAN_POINT('Ctrl Pts',(-20.3796805893304,9.72847589116533,
0.));
#202742=CARTESIAN_POINT('Ctrl Pts',(-20.3839624556742,9.73080870123726,
0.));
#202743=CARTESIAN_POINT('Ctrl Pts',(-20.3885129129912,9.73331167102812,
0.));
#202744=CARTESIAN_POINT('Ctrl Pts',(-20.3933234845646,9.7359829201425,0.));
#202745=CARTESIAN_POINT('Ctrl Pts',(-20.3983866213331,9.73882077613206,
0.));
#202746=CARTESIAN_POINT('Ctrl Pts',(-20.4036953576549,9.74182369656272,
0.));
#202747=CARTESIAN_POINT('Ctrl Pts',(-20.4092430879861,9.74499021838536,
0.));
#202748=CARTESIAN_POINT('Ctrl Pts',(-20.4150232777393,9.74831889242175,
0.));
#202749=CARTESIAN_POINT('Ctrl Pts',(-20.4210295275818,9.75180829786433,
0.));
#202750=CARTESIAN_POINT('Ctrl Pts',(-20.4272556476629,9.75545705902416,
0.));
#202751=CARTESIAN_POINT('Ctrl Pts',(-20.4336957355474,9.7592638628993,0.));
#202752=CARTESIAN_POINT('Ctrl Pts',(-20.4403442329401,9.76322747195502,
0.));
#202753=CARTESIAN_POINT('Ctrl Pts',(-20.447195862298,9.76734670980897,0.));
#202754=CARTESIAN_POINT('Ctrl Pts',(-20.4542455817527,9.7716204510407,0.));
#202755=CARTESIAN_POINT('Ctrl Pts',(-20.4614885274973,9.77604760815523,
0.));
#202756=CARTESIAN_POINT('Ctrl Pts',(-20.4689199790668,9.78062712373313,
0.));
#202757=CARTESIAN_POINT('Ctrl Pts',(-20.4765353711585,9.78535797314162,
0.));
#202758=CARTESIAN_POINT('Ctrl Pts',(-20.4843302955329,9.7902391649866,0.));
#202759=CARTESIAN_POINT('Ctrl Pts',(-20.4923005087945,9.79526974288344,
0.));
#202760=CARTESIAN_POINT('Ctrl Pts',(-20.500441931211,9.80044878520967,0.));
#202761=CARTESIAN_POINT('Ctrl Pts',(-20.5087506310507,9.80577540161103,
0.));
#202762=CARTESIAN_POINT('Ctrl Pts',(-20.5172228122839,9.81124873025278,
0.));
#202763=CARTESIAN_POINT('Ctrl Pts',(-20.5258548000625,9.81686793455918,
0.));
#202764=CARTESIAN_POINT('Ctrl Pts',(-20.534643029951,9.82263220080328,0.));
#202765=CARTESIAN_POINT('Ctrl Pts',(-20.5435840460717,9.82854073773857,
0.));
#202766=CARTESIAN_POINT('Ctrl Pts',(-20.5526744976461,9.83459277585321,
0.));
#202767=CARTESIAN_POINT('Ctrl Pts',(-20.5619111362406,9.84078756677589,
0.));
#202768=CARTESIAN_POINT('Ctrl Pts',(-20.5712908125145,9.84712438256308,
0.));
#202769=CARTESIAN_POINT('Ctrl Pts',(-20.580810471002,9.85360251457004,0.));
#202770=CARTESIAN_POINT('Ctrl Pts',(-20.5904671449754,9.86022127232749,
0.));
#202771=CARTESIAN_POINT('Ctrl Pts',(-20.6002579513696,9.86697998242612,
0.));
#202772=CARTESIAN_POINT('Ctrl Pts',(-20.6101800854491,9.87387798732944,
0.));
#202773=CARTESIAN_POINT('Ctrl Pts',(-20.6202308177472,9.88091464472669,
0.));
#202774=CARTESIAN_POINT('Ctrl Pts',(-20.6304074914086,9.88808932697305,
0.));
#202775=CARTESIAN_POINT('Ctrl Pts',(-20.6407075193977,9.89540142049124,
0.));
#202776=CARTESIAN_POINT('Ctrl Pts',(-20.6511283817415,9.90285032516696,
0.));
#202777=CARTESIAN_POINT('Ctrl Pts',(-20.6616676228315,9.91043545377004,
0.));
#202778=CARTESIAN_POINT('Ctrl Pts',(-20.6723228488262,9.91815623141284,
0.));
#202779=CARTESIAN_POINT('Ctrl Pts',(-20.6830917250255,9.9260120949875,0.));
#202780=CARTESIAN_POINT('Ctrl Pts',(-20.6939719732485,9.93400249259736,
0.));
#202781=CARTESIAN_POINT('Ctrl Pts',(-20.7049613692237,9.94212688298251,
0.));
#202782=CARTESIAN_POINT('Ctrl Pts',(-20.716057740758,9.95038473514962,0.));
#202783=CARTESIAN_POINT('Ctrl Pts',(-20.7272589658752,9.95877552798403,
0.));
#202784=CARTESIAN_POINT('Ctrl Pts',(-20.7385629709795,9.96729874986198,
0.));
#202785=CARTESIAN_POINT('Ctrl Pts',(-20.7499677289625,9.97595389823461,
0.));
#202786=CARTESIAN_POINT('Ctrl Pts',(-20.7614712574989,9.98474047926846,
0.));
#202787=CARTESIAN_POINT('Ctrl Pts',(-20.7730716175417,9.99365800754638,
0.));
#202788=CARTESIAN_POINT('Ctrl Pts',(-20.7847669117568,10.0027060057389,
0.));
#202789=CARTESIAN_POINT('Ctrl Pts',(-20.7965552829907,10.0118840042786,
0.));
#202790=CARTESIAN_POINT('Ctrl Pts',(-20.8084349126885,10.0211915410095,
0.));
#202791=CARTESIAN_POINT('Ctrl Pts',(-20.8204040196599,10.0306281609435,
0.));
#202792=CARTESIAN_POINT('Ctrl Pts',(-20.8324608588906,10.0401934160234,
0.));
#202793=CARTESIAN_POINT('Ctrl Pts',(-20.8446037203402,10.0498868648733,
0.));
#202794=CARTESIAN_POINT('Ctrl Pts',(-20.856830927732,10.0597080725375,0.));
#202795=CARTESIAN_POINT('Ctrl Pts',(-20.8691408373705,10.0696566102219,
0.));
#202796=CARTESIAN_POINT('Ctrl Pts',(-20.8815318371844,10.0797320551154,
0.));
#202797=CARTESIAN_POINT('Ctrl Pts',(-20.8940023457371,10.0899339901916,
0.));
#202798=CARTESIAN_POINT('Ctrl Pts',(-20.9065508112556,10.1002620040076,
0.));
#202799=CARTESIAN_POINT('Ctrl Pts',(-20.9191757106266,10.1107156904836,
0.));
#202800=CARTESIAN_POINT('Ctrl Pts',(-20.931875548473,10.1212946487057,0.));
#202801=CARTESIAN_POINT('Ctrl Pts',(-20.944648856393,10.1319984827909,0.));
#202802=CARTESIAN_POINT('Ctrl Pts',(-20.9574941921591,10.1428268017257,
0.));
#202803=CARTESIAN_POINT('Ctrl Pts',(-20.970410138937,10.1537792192065,0.));
#202804=CARTESIAN_POINT('Ctrl Pts',(-20.9833953044737,10.1648553534567,
0.));
#202805=CARTESIAN_POINT('Ctrl Pts',(-20.9964483203685,10.1760548270765,
0.));
#202806=CARTESIAN_POINT('Ctrl Pts',(-21.0095678414486,10.1873772669358,
0.));
#202807=CARTESIAN_POINT('Ctrl Pts',(-21.0227525451107,10.1988223040425,
0.));
#202808=CARTESIAN_POINT('Ctrl Pts',(-21.0360011306814,10.2103895734123,
0.));
#202809=CARTESIAN_POINT('Ctrl Pts',(-21.0493123187483,10.2220787139157,
0.));
#202810=CARTESIAN_POINT('Ctrl Pts',(-21.0626848505665,10.233889368157,0.));
#202811=CARTESIAN_POINT('Ctrl Pts',(-21.0761174875448,10.2458211823915,
0.));
#202812=CARTESIAN_POINT('Ctrl Pts',(-21.0896090107066,10.2578738064183,
0.));
#202813=CARTESIAN_POINT('Ctrl Pts',(-21.1031582201625,10.2700468934743,
0.));
#202814=CARTESIAN_POINT('Ctrl Pts',(-21.1167639345623,10.2823401001067,
0.));
#202815=CARTESIAN_POINT('Ctrl Pts',(-21.130424990599,10.2947530860714,0.));
#202816=CARTESIAN_POINT('Ctrl Pts',(-21.1441402425831,10.307285514268,0.));
#202817=CARTESIAN_POINT('Ctrl Pts',(-21.1579085619959,10.3199370506541,
0.));
#202818=CARTESIAN_POINT('Ctrl Pts',(-21.1717288370512,10.3327073641574,
0.));
#202819=CARTESIAN_POINT('Ctrl Pts',(-21.1855999722427,10.3455961265706,
0.));
#202820=CARTESIAN_POINT('Ctrl Pts',(-21.1995208879205,10.3586030124595,
0.));
#202821=CARTESIAN_POINT('Ctrl Pts',(-21.2134905199359,10.3717276991137,
0.));
#202822=CARTESIAN_POINT('Ctrl Pts',(-21.2275078192708,10.384969866479,0.));
#202823=CARTESIAN_POINT('Ctrl Pts',(-21.2415717516713,10.3983291970846,
0.));
#202824=CARTESIAN_POINT('Ctrl Pts',(-21.2556812972741,10.4118053759584,
0.));
#202825=CARTESIAN_POINT('Ctrl Pts',(-21.2698354502391,10.4253980905394,
0.));
#202826=CARTESIAN_POINT('Ctrl Pts',(-21.2840332184471,10.4391070306385,
0.));
#202827=CARTESIAN_POINT('Ctrl Pts',(-21.2982736231924,10.452931888387,0.));
#202828=CARTESIAN_POINT('Ctrl Pts',(-21.312555698873,10.4668723581768,0.));
#202829=CARTESIAN_POINT('Ctrl Pts',(-21.3268784926823,10.4809281365933,
0.));
#202830=CARTESIAN_POINT('Ctrl Pts',(-21.3412410642912,10.4950989223341,
0.));
#202831=CARTESIAN_POINT('Ctrl Pts',(-21.3556424855822,10.5093844161689,
0.));
#202832=CARTESIAN_POINT('Ctrl Pts',(-21.3700818403942,10.523784320906,0.));
#202833=CARTESIAN_POINT('Ctrl Pts',(-21.3845582242604,10.5382983413422,
0.));
#202834=CARTESIAN_POINT('Ctrl Pts',(-21.3990707441495,10.5529261842107,
0.));
#202835=CARTESIAN_POINT('Ctrl Pts',(-21.4136185181974,10.5676675581106,
0.));
#202836=CARTESIAN_POINT('Ctrl Pts',(-21.4282006754624,10.582522173457,0.));
#202837=CARTESIAN_POINT('Ctrl Pts',(-21.4428163557137,10.597489742462,0.));
#202838=CARTESIAN_POINT('Ctrl Pts',(-21.4574647092093,10.612569979096,0.));
#202839=CARTESIAN_POINT('Ctrl Pts',(-21.4721448964766,10.6277625990457,
0.));
#202840=CARTESIAN_POINT('Ctrl Pts',(-21.4868560880893,10.6430673196609,
0.));
#202841=CARTESIAN_POINT('Ctrl Pts',(-21.5015974644454,10.658483859894,0.));
#202842=CARTESIAN_POINT('Ctrl Pts',(-21.5163682155805,10.6740119402835,
0.));
#202843=CARTESIAN_POINT('Ctrl Pts',(-21.531167540981,10.689651282929,0.));
#202844=CARTESIAN_POINT('Ctrl Pts',(-21.5459946493955,10.7054016114571,
0.));
#202845=CARTESIAN_POINT('Ctrl Pts',(-21.5608487586467,10.7212626509816,
0.));
#202846=CARTESIAN_POINT('Ctrl Pts',(-21.5757290954372,10.7372341280468,
0.));
#202847=CARTESIAN_POINT('Ctrl Pts',(-21.5906348951745,10.7533157705943,
0.));
#202848=CARTESIAN_POINT('Ctrl Pts',(-21.6055654018179,10.7695073079554,
0.));
#202849=CARTESIAN_POINT('Ctrl Pts',(-21.6205198677176,10.7858084708262,
0.));
#202850=CARTESIAN_POINT('Ctrl Pts',(-21.6354975534557,10.8022189912369,
0.));
#202851=CARTESIAN_POINT('Ctrl Pts',(-21.6504977276864,10.8187386025135,
0.));
#202852=CARTESIAN_POINT('Ctrl Pts',(-21.6655196669727,10.835367039227,0.));
#202853=CARTESIAN_POINT('Ctrl Pts',(-21.6805626556461,10.8521040371832,
0.));
#202854=CARTESIAN_POINT('Ctrl Pts',(-21.6956259856667,10.8689493334093,
0.));
#202855=CARTESIAN_POINT('Ctrl Pts',(-21.7107089564822,10.8859026661292,
0.));
#202856=CARTESIAN_POINT('Ctrl Pts',(-21.7258108748874,10.9029637747341,
0.));
#202857=CARTESIAN_POINT('Ctrl Pts',(-21.74093105488,10.9201323997386,0.));
#202858=CARTESIAN_POINT('Ctrl Pts',(-21.7560688175252,10.9374082827446,
0.));
#202859=CARTESIAN_POINT('Ctrl Pts',(-21.7712234908468,10.9547911664457,
0.));
#202860=CARTESIAN_POINT('Ctrl Pts',(-21.7863944097143,10.9722807946157,
0.));
#202861=CARTESIAN_POINT('Ctrl Pts',(-21.8015809157302,10.9898769120913,
0.));
#202862=CARTESIAN_POINT('Ctrl Pts',(-21.8167823571168,11.0075792647477,
0.));
#202863=CARTESIAN_POINT('Ctrl Pts',(-21.8319980886033,11.0253875994598,
0.));
#202864=CARTESIAN_POINT('Ctrl Pts',(-21.8472274713103,11.0433016640808,
0.));
#202865=CARTESIAN_POINT('Ctrl Pts',(-21.8624698726319,11.0613212074364,
0.));
#202866=CARTESIAN_POINT('Ctrl Pts',(-21.8777246661191,11.0794459793058,
0.));
#202867=CARTESIAN_POINT('Ctrl Pts',(-21.8929912313608,11.0976757303944,
0.));
#202868=CARTESIAN_POINT('Ctrl Pts',(-21.9082689538687,11.1160102123024,
0.));
#202869=CARTESIAN_POINT('Ctrl Pts',(-21.9235572249518,11.134449177474,0.));
#202870=CARTESIAN_POINT('Ctrl Pts',(-21.9388554416437,11.1529923792002,
0.));
#202871=CARTESIAN_POINT('Ctrl Pts',(-21.9541630066504,11.1716395716375,
0.));
#202872=CARTESIAN_POINT('Ctrl Pts',(-21.9694793282913,11.1903905098109,
0.));
#202873=CARTESIAN_POINT('Ctrl Pts',(-21.9848038204439,11.2092449496125,
0.));
#202874=CARTESIAN_POINT('Ctrl Pts',(-22.0001359024839,11.2282026477897,
0.));
#202875=CARTESIAN_POINT('Ctrl Pts',(-22.0154749992364,11.2472633619276,
0.));
#202876=CARTESIAN_POINT('Ctrl Pts',(-22.0308205408351,11.2664268504207,
0.));
#202877=CARTESIAN_POINT('Ctrl Pts',(-22.046171962566,11.2856928724374,0.));
#202878=CARTESIAN_POINT('Ctrl Pts',(-22.0615287047179,11.3050611878771,
0.));
#202879=CARTESIAN_POINT('Ctrl Pts',(-22.0768902124267,11.3245315573168,
0.));
#202880=CARTESIAN_POINT('Ctrl Pts',(-22.0922559355293,11.3441037419553,
0.));
#202881=CARTESIAN_POINT('Ctrl Pts',(-22.1076253283978,11.3637775035367,
0.));
#202882=CARTESIAN_POINT('Ctrl Pts',(-22.1229978500185,11.3835526044256,
0.));
#202883=CARTESIAN_POINT('Ctrl Pts',(-22.1383729640963,11.4034288076908,
0.));
#202884=CARTESIAN_POINT('Ctrl Pts',(-22.1537501391486,11.4234058771742,
0.));
#202885=CARTESIAN_POINT('Ctrl Pts',(-22.1691288486096,11.443483577557,0.));
#202886=CARTESIAN_POINT('Ctrl Pts',(-22.184508570917,11.463661674411,0.));
#202887=CARTESIAN_POINT('Ctrl Pts',(-22.1998887896435,11.4839399342589,
0.));
#202888=CARTESIAN_POINT('Ctrl Pts',(-22.215268993102,11.504318124424,0.));
#202889=CARTESIAN_POINT('Ctrl Pts',(-22.2306486738899,11.5247960128476,
0.));
#202890=CARTESIAN_POINT('Ctrl Pts',(-22.2460273284653,11.545373367912,0.));
#202891=CARTESIAN_POINT('Ctrl Pts',(-22.2614044566898,11.5660499582403,
0.));
#202892=CARTESIAN_POINT('Ctrl Pts',(-22.2767795614349,11.5868255525189,
0.));
#202893=CARTESIAN_POINT('Ctrl Pts',(-22.2921521480358,11.6076999192359,
0.));
#202894=CARTESIAN_POINT('Ctrl Pts',(-22.3075217249049,11.6286728270011,
0.));
#202895=CARTESIAN_POINT('Ctrl Pts',(-22.3228878043976,11.6497440449858,
0.));
#202896=CARTESIAN_POINT('Ctrl Pts',(-22.3382499035618,11.6709133432986,
0.));
#202897=CARTESIAN_POINT('Ctrl Pts',(-22.3536075450028,11.6921804934056,
0.));
#202898=CARTESIAN_POINT('Ctrl Pts',(-22.3689602575492,11.7135452684532,
0.));
#202899=CARTESIAN_POINT('Ctrl Pts',(-22.3843075773905,11.7350074437961,
0.));
#202900=CARTESIAN_POINT('Ctrl Pts',(-22.39964904692,11.7565667964765,0.));
#202901=CARTESIAN_POINT('Ctrl Pts',(-22.4149842125018,11.7782231042041,
0.));
#202902=CARTESIAN_POINT('Ctrl Pts',(-22.4303126226468,11.7999761445175,
0.));
#202903=CARTESIAN_POINT('Ctrl Pts',(-22.4456338258738,11.8218256937889,
0.));
#202904=CARTESIAN_POINT('Ctrl Pts',(-22.4609473690469,11.8437715264487,
0.));
#202905=CARTESIAN_POINT('Ctrl Pts',(-22.4762527946694,11.8658134137018,
0.));
#202906=CARTESIAN_POINT('Ctrl Pts',(-22.4915496418472,11.8879511239941,
0.));
#202907=CARTESIAN_POINT('Ctrl Pts',(-22.5068374513958,11.9101844254555,
0.));
#202908=CARTESIAN_POINT('Ctrl Pts',(-22.5221157697869,11.9325130877801,
0.));
#202909=CARTESIAN_POINT('Ctrl Pts',(-22.5373841537299,11.9549368843996,
0.));
#202910=CARTESIAN_POINT('Ctrl Pts',(-22.5526421741159,11.9774555943496,
0.));
#202911=CARTESIAN_POINT('Ctrl Pts',(-22.5678894211194,12.0000690046697,
0.));
#202912=CARTESIAN_POINT('Ctrl Pts',(-22.5831255061306,12.0227769113132,
0.));
#202913=CARTESIAN_POINT('Ctrl Pts',(-22.5983500505675,12.0455791139135,
0.));
#202914=CARTESIAN_POINT('Ctrl Pts',(-22.613562676493,12.0684754113869,0.));
#202915=CARTESIAN_POINT('Ctrl Pts',(-22.628762996708,12.0914655972828,0.));
#202916=CARTESIAN_POINT('Ctrl Pts',(-22.6439506046611,12.1145494550384,
0.));
#202917=CARTESIAN_POINT('Ctrl Pts',(-22.6591250653942,12.1377267537141,
0.));
#202918=CARTESIAN_POINT('Ctrl Pts',(-22.6742859034891,12.1609972423088,
0.));
#202919=CARTESIAN_POINT('Ctrl Pts',(-22.6894326204959,12.1843606579246,
0.));
#202920=CARTESIAN_POINT('Ctrl Pts',(-22.7045647168659,12.2078167360267,
0.));
#202921=CARTESIAN_POINT('Ctrl Pts',(-22.7196817119299,12.2313652198047,
0.));
#202922=CARTESIAN_POINT('Ctrl Pts',(-22.7347831655251,12.2550058702389,
0.));
#202923=CARTESIAN_POINT('Ctrl Pts',(-22.7498686970096,12.2787384750747,
0.));
#202924=CARTESIAN_POINT('Ctrl Pts',(-22.7649380101154,12.3025628601812,
0.));
#202925=CARTESIAN_POINT('Ctrl Pts',(-22.7799908974947,12.3264788926108,
0.));
#202926=CARTESIAN_POINT('Ctrl Pts',(-22.7950272216959,12.3504864740361,
0.));
#202927=CARTESIAN_POINT('Ctrl Pts',(-22.8100469022632,12.3745855366772,
0.));
#202928=CARTESIAN_POINT('Ctrl Pts',(-22.8220493007353,12.393937937903,0.));
#202929=CARTESIAN_POINT('Ctrl Pts',(-22.8310435872852,12.4084933766366,
0.));
#202930=CARTESIAN_POINT('Ctrl Pts',(-22.8370364396497,12.4182152851867,
0.));
#202931=CARTESIAN_POINT('Ctrl Pts',(-22.8400320311648,12.4230808101438,
0.));
#202932=CARTESIAN_POINT('',(-22.8400320311648,12.4230808101438,0.));
#202933=CARTESIAN_POINT('Origin',(-16.3449727195352,13.9675290154577,0.));
#202934=CARTESIAN_POINT('',(-17.1452095830633,14.6513681262571,0.));
#202935=CARTESIAN_POINT('',(-17.1452095830633,14.6513681262571,0.));
#202936=CARTESIAN_POINT('',(-8.17248635976757,6.98376450772883,0.));
#202937=CARTESIAN_POINT('Ctrl Pts',(-22.1787195904339,13.5685075571671,
0.));
#202938=CARTESIAN_POINT('Ctrl Pts',(-22.1787195904339,13.5685075571671,
12.));
#202939=CARTESIAN_POINT('Ctrl Pts',(-22.1730081264583,13.5683460612913,
0.));
#202940=CARTESIAN_POINT('Ctrl Pts',(-22.1730081264583,13.5683460612913,
12.));
#202941=CARTESIAN_POINT('Ctrl Pts',(-22.1615922804939,13.5680170531724,
0.));
#202942=CARTESIAN_POINT('Ctrl Pts',(-22.1615922804939,13.5680170531724,
12.));
#202943=CARTESIAN_POINT('Ctrl Pts',(-22.1444897575076,13.5675054918922,
0.));
#202944=CARTESIAN_POINT('Ctrl Pts',(-22.1444897575076,13.5675054918922,
12.));
#202945=CARTESIAN_POINT('Ctrl Pts',(-22.1217288871823,13.5667873105179,
0.));
#202946=CARTESIAN_POINT('Ctrl Pts',(-22.1217288871823,13.5667873105179,
12.));
#202947=CARTESIAN_POINT('Ctrl Pts',(-22.0933486464442,13.5658294169106,
0.));
#202948=CARTESIAN_POINT('Ctrl Pts',(-22.0933486464442,13.5658294169106,
12.));
#202949=CARTESIAN_POINT('Ctrl Pts',(-22.0650393089492,13.5648113688894,
0.));
#202950=CARTESIAN_POINT('Ctrl Pts',(-22.0650393089492,13.5648113688894,
12.));
#202951=CARTESIAN_POINT('Ctrl Pts',(-22.0368009736227,13.5637332022393,
0.));
#202952=CARTESIAN_POINT('Ctrl Pts',(-22.0368009736227,13.5637332022393,
12.));
#202953=CARTESIAN_POINT('Ctrl Pts',(-22.0086337943431,13.5625949868313,
0.));
#202954=CARTESIAN_POINT('Ctrl Pts',(-22.0086337943431,13.5625949868313,
12.));
#202955=CARTESIAN_POINT('Ctrl Pts',(-21.9805379899192,13.5613968357589,
0.));
#202956=CARTESIAN_POINT('Ctrl Pts',(-21.9805379899192,13.5613968357589,
12.));
#202957=CARTESIAN_POINT('Ctrl Pts',(-21.9525138592862,13.5601389185315,
0.));
#202958=CARTESIAN_POINT('Ctrl Pts',(-21.9525138592862,13.5601389185315,
12.));
#202959=CARTESIAN_POINT('Ctrl Pts',(-21.9245617765827,13.5588214586672,
0.));
#202960=CARTESIAN_POINT('Ctrl Pts',(-21.9245617765827,13.5588214586672,
12.));
#202961=CARTESIAN_POINT('Ctrl Pts',(-21.8966821688876,13.5574447178484,
0.));
#202962=CARTESIAN_POINT('Ctrl Pts',(-21.8966821688876,13.5574447178484,
12.));
#202963=CARTESIAN_POINT('Ctrl Pts',(-21.8688754989401,13.5560089839426,
0.));
#202964=CARTESIAN_POINT('Ctrl Pts',(-21.8688754989401,13.5560089839426,
12.));
#202965=CARTESIAN_POINT('Ctrl Pts',(-21.841142245609,13.5545145573048,0.));
#202966=CARTESIAN_POINT('Ctrl Pts',(-21.841142245609,13.5545145573048,12.));
#202967=CARTESIAN_POINT('Ctrl Pts',(-21.8134828857963,13.5529617381569,
0.));
#202968=CARTESIAN_POINT('Ctrl Pts',(-21.8134828857963,13.5529617381569,
12.));
#202969=CARTESIAN_POINT('Ctrl Pts',(-21.7858978745848,13.5513508127232,
0.));
#202970=CARTESIAN_POINT('Ctrl Pts',(-21.7858978745848,13.5513508127232,
12.));
#202971=CARTESIAN_POINT('Ctrl Pts',(-21.7583876294532,13.5496820422186,
0.));
#202972=CARTESIAN_POINT('Ctrl Pts',(-21.7583876294532,13.5496820422186,
12.));
#202973=CARTESIAN_POINT('Ctrl Pts',(-21.730952541226,13.5479556704457,0.));
#202974=CARTESIAN_POINT('Ctrl Pts',(-21.730952541226,13.5479556704457,12.));
#202975=CARTESIAN_POINT('Ctrl Pts',(-21.7035929822939,13.546171929503,0.));
#202976=CARTESIAN_POINT('Ctrl Pts',(-21.7035929822939,13.546171929503,12.));
#202977=CARTESIAN_POINT('Ctrl Pts',(-21.676309315769,13.5443310461516,0.));
#202978=CARTESIAN_POINT('Ctrl Pts',(-21.676309315769,13.5443310461516,12.));
#202979=CARTESIAN_POINT('Ctrl Pts',(-21.6491019044647,13.5424332480698,
0.));
#202980=CARTESIAN_POINT('Ctrl Pts',(-21.6491019044647,13.5424332480698,
12.));
#202981=CARTESIAN_POINT('Ctrl Pts',(-21.6219711193951,13.5404787697798,
0.));
#202982=CARTESIAN_POINT('Ctrl Pts',(-21.6219711193951,13.5404787697798,
12.));
#202983=CARTESIAN_POINT('Ctrl Pts',(-21.5949173499022,13.5384678597206,
0.));
#202984=CARTESIAN_POINT('Ctrl Pts',(-21.5949173499022,13.5384678597206,
12.));
#202985=CARTESIAN_POINT('Ctrl Pts',(-21.5679410019011,13.5364007790292,
0.));
#202986=CARTESIAN_POINT('Ctrl Pts',(-21.5679410019011,13.5364007790292,
12.));
#202987=CARTESIAN_POINT('Ctrl Pts',(-21.5410424932511,13.5342777983225,
0.));
#202988=CARTESIAN_POINT('Ctrl Pts',(-21.5410424932511,13.5342777983225,
12.));
#202989=CARTESIAN_POINT('Ctrl Pts',(-21.5142222501671,13.5320991952145,
0.));
#202990=CARTESIAN_POINT('Ctrl Pts',(-21.5142222501671,13.5320991952145,
12.));
#202991=CARTESIAN_POINT('Ctrl Pts',(-21.487480703047,13.5298652514357,0.));
#202992=CARTESIAN_POINT('Ctrl Pts',(-21.487480703047,13.5298652514357,12.));
#202993=CARTESIAN_POINT('Ctrl Pts',(-21.4608182828695,13.5275762503553,
0.));
#202994=CARTESIAN_POINT('Ctrl Pts',(-21.4608182828695,13.5275762503553,
12.));
#202995=CARTESIAN_POINT('Ctrl Pts',(-21.4342354165254,13.5252324737795,
0.));
#202996=CARTESIAN_POINT('Ctrl Pts',(-21.4342354165254,13.5252324737795,
12.));
#202997=CARTESIAN_POINT('Ctrl Pts',(-21.4077325259318,13.5228342013508,
0.));
#202998=CARTESIAN_POINT('Ctrl Pts',(-21.4077325259318,13.5228342013508,
12.));
#202999=CARTESIAN_POINT('Ctrl Pts',(-21.3813100304967,13.5203817122496,
0.));
#203000=CARTESIAN_POINT('Ctrl Pts',(-21.3813100304967,13.5203817122496,
12.));
#203001=CARTESIAN_POINT('Ctrl Pts',(-21.3549683486219,13.5178752862461,
0.));
#203002=CARTESIAN_POINT('Ctrl Pts',(-21.3549683486219,13.5178752862461,
12.));
#203003=CARTESIAN_POINT('Ctrl Pts',(-21.328707899634,13.5153152050554,0.));
#203004=CARTESIAN_POINT('Ctrl Pts',(-21.328707899634,13.5153152050554,12.));
#203005=CARTESIAN_POINT('Ctrl Pts',(-21.3025291054236,13.5127017534972,
0.));
#203006=CARTESIAN_POINT('Ctrl Pts',(-21.3025291054236,13.5127017534972,
12.));
#203007=CARTESIAN_POINT('Ctrl Pts',(-21.2764323924442,13.5100352209207,
0.));
#203008=CARTESIAN_POINT('Ctrl Pts',(-21.2764323924442,13.5100352209207,
12.));
#203009=CARTESIAN_POINT('Ctrl Pts',(-21.2504181927429,13.5073159019454,
0.));
#203010=CARTESIAN_POINT('Ctrl Pts',(-21.2504181927429,13.5073159019454,
12.));
#203011=CARTESIAN_POINT('Ctrl Pts',(-21.224486942933,13.5045440957404,0.));
#203012=CARTESIAN_POINT('Ctrl Pts',(-21.224486942933,13.5045440957404,12.));
#203013=CARTESIAN_POINT('Ctrl Pts',(-21.1986390835825,13.5017201056088,
0.));
#203014=CARTESIAN_POINT('Ctrl Pts',(-21.1986390835825,13.5017201056088,
12.));
#203015=CARTESIAN_POINT('Ctrl Pts',(-21.1728750584173,13.4988442384491,
0.));
#203016=CARTESIAN_POINT('Ctrl Pts',(-21.1728750584173,13.4988442384491,
12.));
#203017=CARTESIAN_POINT('Ctrl Pts',(-21.1471953136209,13.4959168042934,
0.));
#203018=CARTESIAN_POINT('Ctrl Pts',(-21.1471953136209,13.4959168042934,
12.));
#203019=CARTESIAN_POINT('Ctrl Pts',(-21.1216002970209,13.4929381157778,
0.));
#203020=CARTESIAN_POINT('Ctrl Pts',(-21.1216002970209,13.4929381157778,
12.));
#203021=CARTESIAN_POINT('Ctrl Pts',(-21.0960904575048,13.4899084877718,
0.));
#203022=CARTESIAN_POINT('Ctrl Pts',(-21.0960904575048,13.4899084877718,
12.));
#203023=CARTESIAN_POINT('Ctrl Pts',(-21.0706662455202,13.4868282377191,
0.));
#203024=CARTESIAN_POINT('Ctrl Pts',(-21.0706662455202,13.4868282377191,
12.));
#203025=CARTESIAN_POINT('Ctrl Pts',(-21.0453281134247,13.4836976858912,
0.));
#203026=CARTESIAN_POINT('Ctrl Pts',(-21.0453281134247,13.4836976858912,
12.));
#203027=CARTESIAN_POINT('Ctrl Pts',(-21.0200765158885,13.4805171556822,
0.));
#203028=CARTESIAN_POINT('Ctrl Pts',(-21.0200765158885,13.4805171556822,
12.));
#203029=CARTESIAN_POINT('Ctrl Pts',(-20.9949119102592,13.4772869738879,
0.));
#203030=CARTESIAN_POINT('Ctrl Pts',(-20.9949119102592,13.4772869738879,
12.));
#203031=CARTESIAN_POINT('Ctrl Pts',(-20.9698347569476,13.4740074710087,
0.));
#203032=CARTESIAN_POINT('Ctrl Pts',(-20.9698347569476,13.4740074710087,
12.));
#203033=CARTESIAN_POINT('Ctrl Pts',(-20.9448455197557,13.4706789815166,
0.));
#203034=CARTESIAN_POINT('Ctrl Pts',(-20.9448455197557,13.4706789815166,
12.));
#203035=CARTESIAN_POINT('Ctrl Pts',(-20.9199446657584,13.4673018437718,
0.));
#203036=CARTESIAN_POINT('Ctrl Pts',(-20.9199446657584,13.4673018437718,
12.));
#203037=CARTESIAN_POINT('Ctrl Pts',(-20.8951326652158,13.4638763999725,
0.));
#203038=CARTESIAN_POINT('Ctrl Pts',(-20.8951326652158,13.4638763999725,
12.));
#203039=CARTESIAN_POINT('Ctrl Pts',(-20.8704099914641,13.4604029960983,
0.));
#203040=CARTESIAN_POINT('Ctrl Pts',(-20.8704099914641,13.4604029960983,
12.));
#203041=CARTESIAN_POINT('Ctrl Pts',(-20.8457771208082,13.4568819818631,
0.));
#203042=CARTESIAN_POINT('Ctrl Pts',(-20.8457771208082,13.4568819818631,
12.));
#203043=CARTESIAN_POINT('Ctrl Pts',(-20.821234532398,13.4533137106667,0.));
#203044=CARTESIAN_POINT('Ctrl Pts',(-20.821234532398,13.4533137106667,12.));
#203045=CARTESIAN_POINT('Ctrl Pts',(-20.7967827081227,13.4496985395637,
0.));
#203046=CARTESIAN_POINT('Ctrl Pts',(-20.7967827081227,13.4496985395637,
12.));
#203047=CARTESIAN_POINT('Ctrl Pts',(-20.7724221327608,13.4460368293688,
0.));
#203048=CARTESIAN_POINT('Ctrl Pts',(-20.7724221327608,13.4460368293688,
12.));
#203049=CARTESIAN_POINT('Ctrl Pts',(-20.7481532941013,13.4423289447561,
0.));
#203050=CARTESIAN_POINT('Ctrl Pts',(-20.7481532941013,13.4423289447561,
12.));
#203051=CARTESIAN_POINT('Ctrl Pts',(-20.7239766830675,13.4385752543663,
0.));
#203052=CARTESIAN_POINT('Ctrl Pts',(-20.7239766830675,13.4385752543663,
12.));
#203053=CARTESIAN_POINT('Ctrl Pts',(-20.6998927938288,13.4347761309154,
0.));
#203054=CARTESIAN_POINT('Ctrl Pts',(-20.6998927938288,13.4347761309154,
12.));
#203055=CARTESIAN_POINT('Ctrl Pts',(-20.6759021239103,13.4309319513119,
0.));
#203056=CARTESIAN_POINT('Ctrl Pts',(-20.6759021239103,13.4309319513119,
12.));
#203057=CARTESIAN_POINT('Ctrl Pts',(-20.6520051742869,13.4270430967651,
0.));
#203058=CARTESIAN_POINT('Ctrl Pts',(-20.6520051742869,13.4270430967651,
12.));
#203059=CARTESIAN_POINT('Ctrl Pts',(-20.6282024494237,13.4231099528179,
0.));
#203060=CARTESIAN_POINT('Ctrl Pts',(-20.6282024494237,13.4231099528179,
12.));
#203061=CARTESIAN_POINT('Ctrl Pts',(-20.6044944573153,13.4191329093932,
0.));
#203062=CARTESIAN_POINT('Ctrl Pts',(-20.6044944573153,13.4191329093932,
12.));
#203063=CARTESIAN_POINT('Ctrl Pts',(-20.5808817095155,13.4151123608411,
0.));
#203064=CARTESIAN_POINT('Ctrl Pts',(-20.5808817095155,13.4151123608411,
12.));
#203065=CARTESIAN_POINT('Ctrl Pts',(-20.5573647211639,13.4110487059912,
0.));
#203066=CARTESIAN_POINT('Ctrl Pts',(-20.5573647211639,13.4110487059912,
12.));
#203067=CARTESIAN_POINT('Ctrl Pts',(-20.5339440109956,13.4069423482076,
0.));
#203068=CARTESIAN_POINT('Ctrl Pts',(-20.5339440109956,13.4069423482076,
12.));
#203069=CARTESIAN_POINT('Ctrl Pts',(-20.5106201013753,13.4027936954529,
0.));
#203070=CARTESIAN_POINT('Ctrl Pts',(-20.5106201013753,13.4027936954529,
12.));
#203071=CARTESIAN_POINT('Ctrl Pts',(-20.487393518404,13.3986031603716,0.));
#203072=CARTESIAN_POINT('Ctrl Pts',(-20.487393518404,13.3986031603716,12.));
#203073=CARTESIAN_POINT('Ctrl Pts',(-20.4642647920038,13.3943711603739,
0.));
#203074=CARTESIAN_POINT('Ctrl Pts',(-20.4642647920038,13.3943711603739,
12.));
#203075=CARTESIAN_POINT('Ctrl Pts',(-20.4412344560008,13.3900981177255,
0.));
#203076=CARTESIAN_POINT('Ctrl Pts',(-20.4412344560008,13.3900981177255,
12.));
#203077=CARTESIAN_POINT('Ctrl Pts',(-20.4183030482002,13.3857844596387,
0.));
#203078=CARTESIAN_POINT('Ctrl Pts',(-20.4183030482002,13.3857844596387,
12.));
#203079=CARTESIAN_POINT('Ctrl Pts',(-20.3954711104502,13.3814306183719,
0.));
#203080=CARTESIAN_POINT('Ctrl Pts',(-20.3954711104502,13.3814306183719,
12.));
#203081=CARTESIAN_POINT('Ctrl Pts',(-20.3727391887184,13.3770370313188,
0.));
#203082=CARTESIAN_POINT('Ctrl Pts',(-20.3727391887184,13.3770370313188,
12.));
#203083=CARTESIAN_POINT('Ctrl Pts',(-20.3501078331814,13.3726041410867,
0.));
#203084=CARTESIAN_POINT('Ctrl Pts',(-20.3501078331814,13.3726041410867,
12.));
#203085=CARTESIAN_POINT('Ctrl Pts',(-20.3275775983029,13.3681323955826,
0.));
#203086=CARTESIAN_POINT('Ctrl Pts',(-20.3275775983029,13.3681323955826,
12.));
#203087=CARTESIAN_POINT('Ctrl Pts',(-20.3051490429048,13.3636222481016,
0.));
#203088=CARTESIAN_POINT('Ctrl Pts',(-20.3051490429048,13.3636222481016,
12.));
#203089=CARTESIAN_POINT('Ctrl Pts',(-20.2828227302339,13.3590741574195,
0.));
#203090=CARTESIAN_POINT('Ctrl Pts',(-20.2828227302339,13.3590741574195,
12.));
#203091=CARTESIAN_POINT('Ctrl Pts',(-20.2605992280122,13.3544885878889,
0.));
#203092=CARTESIAN_POINT('Ctrl Pts',(-20.2605992280122,13.3544885878889,
12.));
#203093=CARTESIAN_POINT('Ctrl Pts',(-20.2384791085359,13.3498660095386,
0.));
#203094=CARTESIAN_POINT('Ctrl Pts',(-20.2384791085359,13.3498660095386,
12.));
#203095=CARTESIAN_POINT('Ctrl Pts',(-20.216462948786,13.3452068981766,0.));
#203096=CARTESIAN_POINT('Ctrl Pts',(-20.216462948786,13.3452068981766,12.));
#203097=CARTESIAN_POINT('Ctrl Pts',(-20.1945513305235,13.3405117354971,
0.));
#203098=CARTESIAN_POINT('Ctrl Pts',(-20.1945513305235,13.3405117354971,
12.));
#203099=CARTESIAN_POINT('Ctrl Pts',(-20.1727448403817,13.3357810091903,
0.));
#203100=CARTESIAN_POINT('Ctrl Pts',(-20.1727448403817,13.3357810091903,
12.));
#203101=CARTESIAN_POINT('Ctrl Pts',(-20.1510440699474,13.3310152130564,
0.));
#203102=CARTESIAN_POINT('Ctrl Pts',(-20.1510440699474,13.3310152130564,
12.));
#203103=CARTESIAN_POINT('Ctrl Pts',(-20.1294496158402,13.3262148471226,
0.));
#203104=CARTESIAN_POINT('Ctrl Pts',(-20.1294496158402,13.3262148471226,
12.));
#203105=CARTESIAN_POINT('Ctrl Pts',(-20.1079620798375,13.3213804177587,
0.));
#203106=CARTESIAN_POINT('Ctrl Pts',(-20.1079620798375,13.3213804177587,
12.));
#203107=CARTESIAN_POINT('Ctrl Pts',(-20.0865820689883,13.3165124377962,
0.));
#203108=CARTESIAN_POINT('Ctrl Pts',(-20.0865820689883,13.3165124377962,
12.));
#203109=CARTESIAN_POINT('Ctrl Pts',(-20.0653101957188,13.3116114266515,
0.));
#203110=CARTESIAN_POINT('Ctrl Pts',(-20.0653101957188,13.3116114266515,
12.));
#203111=CARTESIAN_POINT('Ctrl Pts',(-20.0441470779345,13.3066779104515,
0.));
#203112=CARTESIAN_POINT('Ctrl Pts',(-20.0441470779345,13.3066779104515,
12.));
#203113=CARTESIAN_POINT('Ctrl Pts',(-20.0230933391038,13.3017124221637,
0.));
#203114=CARTESIAN_POINT('Ctrl Pts',(-20.0230933391038,13.3017124221637,
12.));
#203115=CARTESIAN_POINT('Ctrl Pts',(-20.0021496083738,13.2967155017306,
0.));
#203116=CARTESIAN_POINT('Ctrl Pts',(-20.0021496083738,13.2967155017306,
12.));
#203117=CARTESIAN_POINT('Ctrl Pts',(-19.981316520717,13.2916876962094,0.));
#203118=CARTESIAN_POINT('Ctrl Pts',(-19.981316520717,13.2916876962094,12.));
#203119=CARTESIAN_POINT('Ctrl Pts',(-19.9605947170586,13.286629559915,0.));
#203120=CARTESIAN_POINT('Ctrl Pts',(-19.9605947170586,13.286629559915,12.));
#203121=CARTESIAN_POINT('Ctrl Pts',(-19.9399848444019,13.2815416545663,
0.));
#203122=CARTESIAN_POINT('Ctrl Pts',(-19.9399848444019,13.2815416545663,
12.));
#203123=CARTESIAN_POINT('Ctrl Pts',(-19.9194875559422,13.2764245494357,
0.));
#203124=CARTESIAN_POINT('Ctrl Pts',(-19.9194875559422,13.2764245494357,
12.));
#203125=CARTESIAN_POINT('Ctrl Pts',(-19.8991035111745,13.271278821502,0.));
#203126=CARTESIAN_POINT('Ctrl Pts',(-19.8991035111745,13.271278821502,12.));
#203127=CARTESIAN_POINT('Ctrl Pts',(-19.8788333760577,13.2661050556132,
0.));
#203128=CARTESIAN_POINT('Ctrl Pts',(-19.8788333760577,13.2661050556132,
12.));
#203129=CARTESIAN_POINT('Ctrl Pts',(-19.8586778231715,13.2609038446529,
0.));
#203130=CARTESIAN_POINT('Ctrl Pts',(-19.8586778231715,13.2609038446529,
12.));
#203131=CARTESIAN_POINT('Ctrl Pts',(-19.8386375318634,13.2556757897086,
0.));
#203132=CARTESIAN_POINT('Ctrl Pts',(-19.8386375318634,13.2556757897086,
12.));
#203133=CARTESIAN_POINT('Ctrl Pts',(-19.8187131883917,13.2504215002457,
0.));
#203134=CARTESIAN_POINT('Ctrl Pts',(-19.8187131883917,13.2504215002457,
12.));
#203135=CARTESIAN_POINT('Ctrl Pts',(-19.7989054860495,13.2451415942805,
0.));
#203136=CARTESIAN_POINT('Ctrl Pts',(-19.7989054860495,13.2451415942805,
12.));
#203137=CARTESIAN_POINT('Ctrl Pts',(-19.7792151253289,13.2398366985675,
0.));
#203138=CARTESIAN_POINT('Ctrl Pts',(-19.7792151253289,13.2398366985675,
12.));
#203139=CARTESIAN_POINT('Ctrl Pts',(-19.7596428141168,13.2345074487963,
0.));
#203140=CARTESIAN_POINT('Ctrl Pts',(-19.7596428141168,13.2345074487963,
12.));
#203141=CARTESIAN_POINT('Ctrl Pts',(-19.7401892678697,13.2291544897899,
0.));
#203142=CARTESIAN_POINT('Ctrl Pts',(-19.7401892678697,13.2291544897899,
12.));
#203143=CARTESIAN_POINT('Ctrl Pts',(-19.7208552097868,13.2237784757065,
0.));
#203144=CARTESIAN_POINT('Ctrl Pts',(-19.7208552097868,13.2237784757065,
12.));
#203145=CARTESIAN_POINT('Ctrl Pts',(-19.7016413709685,13.2183800702436,
0.));
#203146=CARTESIAN_POINT('Ctrl Pts',(-19.7016413709685,13.2183800702436,
12.));
#203147=CARTESIAN_POINT('Ctrl Pts',(-19.6825484905823,13.2129599468485,
0.));
#203148=CARTESIAN_POINT('Ctrl Pts',(-19.6825484905823,13.2129599468485,
12.));
#203149=CARTESIAN_POINT('Ctrl Pts',(-19.6635773160936,13.2075187889529,
0.));
#203150=CARTESIAN_POINT('Ctrl Pts',(-19.6635773160936,13.2075187889529,
12.));
#203151=CARTESIAN_POINT('Ctrl Pts',(-19.6447286034772,13.2020572902065,
0.));
#203152=CARTESIAN_POINT('Ctrl Pts',(-19.6447286034772,13.2020572902065,
12.));
#203153=CARTESIAN_POINT('Ctrl Pts',(-19.6260031174244,13.1965761547151,
0.));
#203154=CARTESIAN_POINT('Ctrl Pts',(-19.6260031174244,13.1965761547151,
12.));
#203155=CARTESIAN_POINT('Ctrl Pts',(-19.6074016315414,13.1910760972814,
0.));
#203156=CARTESIAN_POINT('Ctrl Pts',(-19.6074016315414,13.1910760972814,
12.));
#203157=CARTESIAN_POINT('Ctrl Pts',(-19.5889249285338,13.1855578436471,
0.));
#203158=CARTESIAN_POINT('Ctrl Pts',(-19.5889249285338,13.1855578436471,
12.));
#203159=CARTESIAN_POINT('Ctrl Pts',(-19.5705738004667,13.1800221307673,
0.));
#203160=CARTESIAN_POINT('Ctrl Pts',(-19.5705738004667,13.1800221307673,
12.));
#203161=CARTESIAN_POINT('Ctrl Pts',(-19.5523490490244,13.1744697070911,
0.));
#203162=CARTESIAN_POINT('Ctrl Pts',(-19.5523490490244,13.1744697070911,
12.));
#203163=CARTESIAN_POINT('Ctrl Pts',(-19.5342514857562,13.168901332843,0.));
#203164=CARTESIAN_POINT('Ctrl Pts',(-19.5342514857562,13.168901332843,12.));
#203165=CARTESIAN_POINT('Ctrl Pts',(-19.5162819323213,13.1633177803101,
0.));
#203166=CARTESIAN_POINT('Ctrl Pts',(-19.5162819323213,13.1633177803101,
12.));
#203167=CARTESIAN_POINT('Ctrl Pts',(-19.4984412207082,13.1577198341245,
0.));
#203168=CARTESIAN_POINT('Ctrl Pts',(-19.4984412207082,13.1577198341245,
12.));
#203169=CARTESIAN_POINT('Ctrl Pts',(-19.4807301935268,13.1521082915853,
0.));
#203170=CARTESIAN_POINT('Ctrl Pts',(-19.4807301935268,13.1521082915853,
12.));
#203171=CARTESIAN_POINT('Ctrl Pts',(-19.4631497043258,13.1464839629971,
0.));
#203172=CARTESIAN_POINT('Ctrl Pts',(-19.4631497043258,13.1464839629971,
12.));
#203173=CARTESIAN_POINT('Ctrl Pts',(-19.4457006178876,13.1408476720061,
0.));
#203174=CARTESIAN_POINT('Ctrl Pts',(-19.4457006178876,13.1408476720061,
12.));
#203175=CARTESIAN_POINT('Ctrl Pts',(-19.4283838105262,13.1352002559438,
0.));
#203176=CARTESIAN_POINT('Ctrl Pts',(-19.4283838105262,13.1352002559438,
12.));
#203177=CARTESIAN_POINT('Ctrl Pts',(-19.4112001703557,13.1295425661634,
0.));
#203178=CARTESIAN_POINT('Ctrl Pts',(-19.4112001703557,13.1295425661634,
12.));
#203179=CARTESIAN_POINT('Ctrl Pts',(-19.3941505976263,13.1238754684177,
0.));
#203180=CARTESIAN_POINT('Ctrl Pts',(-19.3941505976263,13.1238754684177,
12.));
#203181=CARTESIAN_POINT('Ctrl Pts',(-19.3772360051091,13.118199843271,0.));
#203182=CARTESIAN_POINT('Ctrl Pts',(-19.3772360051091,13.118199843271,12.));
#203183=CARTESIAN_POINT('Ctrl Pts',(-19.3604573184515,13.1125165865022,
0.));
#203184=CARTESIAN_POINT('Ctrl Pts',(-19.3604573184515,13.1125165865022,
12.));
#203185=CARTESIAN_POINT('Ctrl Pts',(-19.3438154765395,13.1068266095186,
0.));
#203186=CARTESIAN_POINT('Ctrl Pts',(-19.3438154765395,13.1068266095186,
12.));
#203187=CARTESIAN_POINT('Ctrl Pts',(-19.3273114318269,13.1011308397591,
0.));
#203188=CARTESIAN_POINT('Ctrl Pts',(-19.3273114318269,13.1011308397591,
12.));
#203189=CARTESIAN_POINT('Ctrl Pts',(-19.310946150736,13.0954302211479,0.));
#203190=CARTESIAN_POINT('Ctrl Pts',(-19.310946150736,13.0954302211479,12.));
#203191=CARTESIAN_POINT('Ctrl Pts',(-19.2947206141247,13.0897257145968,
0.));
#203192=CARTESIAN_POINT('Ctrl Pts',(-19.2947206141247,13.0897257145968,
12.));
#203193=CARTESIAN_POINT('Ctrl Pts',(-19.2786358177198,13.0840182984949,
0.));
#203194=CARTESIAN_POINT('Ctrl Pts',(-19.2786358177198,13.0840182984949,
12.));
#203195=CARTESIAN_POINT('Ctrl Pts',(-19.2626927725596,13.0783089692118,
0.));
#203196=CARTESIAN_POINT('Ctrl Pts',(-19.2626927725596,13.0783089692118,
12.));
#203197=CARTESIAN_POINT('Ctrl Pts',(-19.2468925053989,13.0725987415859,
0.));
#203198=CARTESIAN_POINT('Ctrl Pts',(-19.2468925053989,13.0725987415859,
12.));
#203199=CARTESIAN_POINT('Ctrl Pts',(-19.2312360592033,13.0668886494795,
0.));
#203200=CARTESIAN_POINT('Ctrl Pts',(-19.2312360592033,13.0668886494795,
12.));
#203201=CARTESIAN_POINT('Ctrl Pts',(-19.2157244937142,13.0611797463915,
0.));
#203202=CARTESIAN_POINT('Ctrl Pts',(-19.2157244937142,13.0611797463915,
12.));
#203203=CARTESIAN_POINT('Ctrl Pts',(-19.2003588859772,13.0554731060538,
0.));
#203204=CARTESIAN_POINT('Ctrl Pts',(-19.2003588859772,13.0554731060538,
12.));
#203205=CARTESIAN_POINT('Ctrl Pts',(-19.1851403308825,13.0497698230441,
0.));
#203206=CARTESIAN_POINT('Ctrl Pts',(-19.1851403308825,13.0497698230441,
12.));
#203207=CARTESIAN_POINT('Ctrl Pts',(-19.1700699416622,13.0440710133772,
0.));
#203208=CARTESIAN_POINT('Ctrl Pts',(-19.1700699416622,13.0440710133772,
12.));
#203209=CARTESIAN_POINT('Ctrl Pts',(-19.155148850523,13.0383778152068,0.));
#203210=CARTESIAN_POINT('Ctrl Pts',(-19.155148850523,13.0383778152068,12.));
#203211=CARTESIAN_POINT('Ctrl Pts',(-19.1403782093386,13.0326913895838,
0.));
#203212=CARTESIAN_POINT('Ctrl Pts',(-19.1403782093386,13.0326913895838,
12.));
#203213=CARTESIAN_POINT('Ctrl Pts',(-19.1257591903099,13.0270129211976,
0.));
#203214=CARTESIAN_POINT('Ctrl Pts',(-19.1257591903099,13.0270129211976,
12.));
#203215=CARTESIAN_POINT('Ctrl Pts',(-19.111292986631,13.0213436191328,0.));
#203216=CARTESIAN_POINT('Ctrl Pts',(-19.111292986631,13.0213436191328,12.));
#203217=CARTESIAN_POINT('Ctrl Pts',(-19.0969808131228,13.0156847176096,
0.));
#203218=CARTESIAN_POINT('Ctrl Pts',(-19.0969808131228,13.0156847176096,
12.));
#203219=CARTESIAN_POINT('Ctrl Pts',(-19.0828239070484,13.0100374768788,
0.));
#203220=CARTESIAN_POINT('Ctrl Pts',(-19.0828239070484,13.0100374768788,
12.));
#203221=CARTESIAN_POINT('Ctrl Pts',(-19.0688235289437,13.0044031841382,
0.));
#203222=CARTESIAN_POINT('Ctrl Pts',(-19.0688235289437,13.0044031841382,
12.));
#203223=CARTESIAN_POINT('Ctrl Pts',(-19.0549809634354,12.9987831544502,
0.));
#203224=CARTESIAN_POINT('Ctrl Pts',(-19.0549809634354,12.9987831544502,
12.));
#203225=CARTESIAN_POINT('Ctrl Pts',(-19.0412975200398,12.9931787316514,
0.));
#203226=CARTESIAN_POINT('Ctrl Pts',(-19.0412975200398,12.9931787316514,
12.));
#203227=CARTESIAN_POINT('Ctrl Pts',(-19.0277745339909,12.9875912893003,
0.));
#203228=CARTESIAN_POINT('Ctrl Pts',(-19.0277745339909,12.9875912893003,
12.));
#203229=CARTESIAN_POINT('Ctrl Pts',(-19.014413367335,12.9820222318716,0.));
#203230=CARTESIAN_POINT('Ctrl Pts',(-19.014413367335,12.9820222318716,12.));
#203231=CARTESIAN_POINT('Ctrl Pts',(-19.0012154099792,12.9764729959206,
0.));
#203232=CARTESIAN_POINT('Ctrl Pts',(-19.0012154099792,12.9764729959206,
12.));
#203233=CARTESIAN_POINT('Ctrl Pts',(-18.9881820807585,12.9709450512747,
0.));
#203234=CARTESIAN_POINT('Ctrl Pts',(-18.9881820807585,12.9709450512747,
12.));
#203235=CARTESIAN_POINT('Ctrl Pts',(-18.9753148284473,12.9654399021868,
0.));
#203236=CARTESIAN_POINT('Ctrl Pts',(-18.9753148284473,12.9654399021868,
12.));
#203237=CARTESIAN_POINT('Ctrl Pts',(-18.9626151329226,12.9599590886317,
0.));
#203238=CARTESIAN_POINT('Ctrl Pts',(-18.9626151329226,12.9599590886317,
12.));
#203239=CARTESIAN_POINT('Ctrl Pts',(-18.9500845064714,12.9545041877377,
0.));
#203240=CARTESIAN_POINT('Ctrl Pts',(-18.9500845064714,12.9545041877377,
12.));
#203241=CARTESIAN_POINT('Ctrl Pts',(-18.9377244950435,12.9490768151821,
0.));
#203242=CARTESIAN_POINT('Ctrl Pts',(-18.9377244950435,12.9490768151821,
12.));
#203243=CARTESIAN_POINT('Ctrl Pts',(-18.9255366795196,12.9436786266106,
0.));
#203244=CARTESIAN_POINT('Ctrl Pts',(-18.9255366795196,12.9436786266106,
12.));
#203245=CARTESIAN_POINT('Ctrl Pts',(-18.9135226769466,12.9383113190375,
0.));
#203246=CARTESIAN_POINT('Ctrl Pts',(-18.9135226769466,12.9383113190375,
12.));
#203247=CARTESIAN_POINT('Ctrl Pts',(-18.9016841423402,12.9329766328184,
0.));
#203248=CARTESIAN_POINT('Ctrl Pts',(-18.9016841423402,12.9329766328184,
12.));
#203249=CARTESIAN_POINT('Ctrl Pts',(-18.8900227704888,12.9276763536372,
0.));
#203250=CARTESIAN_POINT('Ctrl Pts',(-18.8900227704888,12.9276763536372,
12.));
#203251=CARTESIAN_POINT('Ctrl Pts',(-18.8785402977528,12.9224123144982,
0.));
#203252=CARTESIAN_POINT('Ctrl Pts',(-18.8785402977528,12.9224123144982,
12.));
#203253=CARTESIAN_POINT('Ctrl Pts',(-18.8672385038328,12.9171863977047,
0.));
#203254=CARTESIAN_POINT('Ctrl Pts',(-18.8672385038328,12.9171863977047,
12.));
#203255=CARTESIAN_POINT('Ctrl Pts',(-18.8561192136201,12.9120005369066,
0.));
#203256=CARTESIAN_POINT('Ctrl Pts',(-18.8561192136201,12.9120005369066,
12.));
#203257=CARTESIAN_POINT('Ctrl Pts',(-18.8451842990986,12.9068567191856,
0.));
#203258=CARTESIAN_POINT('Ctrl Pts',(-18.8451842990986,12.9068567191856,
12.));
#203259=CARTESIAN_POINT('Ctrl Pts',(-18.834435681259,12.9017569871738,0.));
#203260=CARTESIAN_POINT('Ctrl Pts',(-18.834435681259,12.9017569871738,12.));
#203261=CARTESIAN_POINT('Ctrl Pts',(-18.8238753319124,12.8967034410752,
0.));
#203262=CARTESIAN_POINT('Ctrl Pts',(-18.8238753319124,12.8967034410752,
12.));
#203263=CARTESIAN_POINT('Ctrl Pts',(-18.8135052757815,12.8916982409931,
0.));
#203264=CARTESIAN_POINT('Ctrl Pts',(-18.8135052757815,12.8916982409931,
12.));
#203265=CARTESIAN_POINT('Ctrl Pts',(-18.8033275941939,12.8867436109543,
0.));
#203266=CARTESIAN_POINT('Ctrl Pts',(-18.8033275941939,12.8867436109543,
12.));
#203267=CARTESIAN_POINT('Ctrl Pts',(-18.7933444285867,12.8818418427474,
0.));
#203268=CARTESIAN_POINT('Ctrl Pts',(-18.7933444285867,12.8818418427474,
12.));
#203269=CARTESIAN_POINT('Ctrl Pts',(-18.7835579840481,12.8769952998097,
0.));
#203270=CARTESIAN_POINT('Ctrl Pts',(-18.7835579840481,12.8769952998097,
12.));
#203271=CARTESIAN_POINT('Ctrl Pts',(-18.7739705329029,12.8722064211814,
0.));
#203272=CARTESIAN_POINT('Ctrl Pts',(-18.7739705329029,12.8722064211814,
12.));
#203273=CARTESIAN_POINT('Ctrl Pts',(-18.7645844169568,12.8674777239656,
0.));
#203274=CARTESIAN_POINT('Ctrl Pts',(-18.7645844169568,12.8674777239656,
12.));
#203275=CARTESIAN_POINT('Ctrl Pts',(-18.7554020493888,12.8628118054172,
0.));
#203276=CARTESIAN_POINT('Ctrl Pts',(-18.7554020493888,12.8628118054172,
12.));
#203277=CARTESIAN_POINT('Ctrl Pts',(-18.7464259171248,12.8582113455644,
0.));
#203278=CARTESIAN_POINT('Ctrl Pts',(-18.7464259171248,12.8582113455644,
12.));
#203279=CARTESIAN_POINT('Ctrl Pts',(-18.7376585820851,12.8536791086315,
0.));
#203280=CARTESIAN_POINT('Ctrl Pts',(-18.7376585820851,12.8536791086315,
12.));
#203281=CARTESIAN_POINT('Ctrl Pts',(-18.7291026886552,12.849217951159,0.));
#203282=CARTESIAN_POINT('Ctrl Pts',(-18.7291026886552,12.849217951159,12.));
#203283=CARTESIAN_POINT('Ctrl Pts',(-18.7207609737701,12.8448308329494,
0.));
#203284=CARTESIAN_POINT('Ctrl Pts',(-18.7207609737701,12.8448308329494,
12.));
#203285=CARTESIAN_POINT('Ctrl Pts',(-18.7126362754446,12.8405208263432,
0.));
#203286=CARTESIAN_POINT('Ctrl Pts',(-18.7126362754446,12.8405208263432,
12.));
#203287=CARTESIAN_POINT('Ctrl Pts',(-18.7047315436296,12.8362911280362,
0.));
#203288=CARTESIAN_POINT('Ctrl Pts',(-18.7047315436296,12.8362911280362,
12.));
#203289=CARTESIAN_POINT('Ctrl Pts',(-18.6970498410173,12.832145059979,0.));
#203290=CARTESIAN_POINT('Ctrl Pts',(-18.6970498410173,12.832145059979,12.));
#203291=CARTESIAN_POINT('Ctrl Pts',(-18.6895943376172,12.8280860635231,
0.));
#203292=CARTESIAN_POINT('Ctrl Pts',(-18.6895943376172,12.8280860635231,
12.));
#203293=CARTESIAN_POINT('Ctrl Pts',(-18.6823683094139,12.8241176980016,
0.));
#203294=CARTESIAN_POINT('Ctrl Pts',(-18.6823683094139,12.8241176980016,
12.));
#203295=CARTESIAN_POINT('Ctrl Pts',(-18.6753751301091,12.8202436318473,
0.));
#203296=CARTESIAN_POINT('Ctrl Pts',(-18.6753751301091,12.8202436318473,
12.));
#203297=CARTESIAN_POINT('Ctrl Pts',(-18.6686182952798,12.8164676687361,
0.));
#203298=CARTESIAN_POINT('Ctrl Pts',(-18.6686182952798,12.8164676687361,
12.));
#203299=CARTESIAN_POINT('Ctrl Pts',(-18.6621014624746,12.8127937909632,
0.));
#203300=CARTESIAN_POINT('Ctrl Pts',(-18.6621014624746,12.8127937909632,
12.));
#203301=CARTESIAN_POINT('Ctrl Pts',(-18.6558284825772,12.8092261933858,
0.));
#203302=CARTESIAN_POINT('Ctrl Pts',(-18.6558284825772,12.8092261933858,
12.));
#203303=CARTESIAN_POINT('Ctrl Pts',(-18.6498034438986,12.805769331162,0.));
#203304=CARTESIAN_POINT('Ctrl Pts',(-18.6498034438986,12.805769331162,12.));
#203305=CARTESIAN_POINT('Ctrl Pts',(-18.6440306327457,12.8024278770153,
0.));
#203306=CARTESIAN_POINT('Ctrl Pts',(-18.6440306327457,12.8024278770153,
12.));
#203307=CARTESIAN_POINT('Ctrl Pts',(-18.63851447924,12.7992066625264,0.));
#203308=CARTESIAN_POINT('Ctrl Pts',(-18.63851447924,12.7992066625264,12.));
#203309=CARTESIAN_POINT('Ctrl Pts',(-18.6332595057005,12.7961106222251,
0.));
#203310=CARTESIAN_POINT('Ctrl Pts',(-18.6332595057005,12.7961106222251,
12.));
#203311=CARTESIAN_POINT('Ctrl Pts',(-18.6282702819371,12.7931447451556,
0.));
#203312=CARTESIAN_POINT('Ctrl Pts',(-18.6282702819371,12.7931447451556,
12.));
#203313=CARTESIAN_POINT('Ctrl Pts',(-18.6235516265575,12.7903142925234,
0.));
#203314=CARTESIAN_POINT('Ctrl Pts',(-18.6235516265575,12.7903142925234,
12.));
#203315=CARTESIAN_POINT('Ctrl Pts',(-18.6191087624752,12.7876249657834,
0.));
#203316=CARTESIAN_POINT('Ctrl Pts',(-18.6191087624752,12.7876249657834,
12.));
#203317=CARTESIAN_POINT('Ctrl Pts',(-18.6149475565189,12.78508316579,0.));
#203318=CARTESIAN_POINT('Ctrl Pts',(-18.6149475565189,12.78508316579,12.));
#203319=CARTESIAN_POINT('Ctrl Pts',(-18.611074482622,12.7826959526924,0.));
#203320=CARTESIAN_POINT('Ctrl Pts',(-18.611074482622,12.7826959526924,12.));
#203321=CARTESIAN_POINT('Ctrl Pts',(-18.6074961535723,12.7804705387658,
0.));
#203322=CARTESIAN_POINT('Ctrl Pts',(-18.6074961535723,12.7804705387658,
12.));
#203323=CARTESIAN_POINT('Ctrl Pts',(-18.6042190183703,12.7784139605067,
0.));
#203324=CARTESIAN_POINT('Ctrl Pts',(-18.6042190183703,12.7784139605067,
12.));
#203325=CARTESIAN_POINT('Ctrl Pts',(-18.6012488486708,12.7765325225082,
0.));
#203326=CARTESIAN_POINT('Ctrl Pts',(-18.6012488486708,12.7765325225082,
12.));
#203327=CARTESIAN_POINT('Ctrl Pts',(-18.5985917525949,12.7748328937639,
0.));
#203328=CARTESIAN_POINT('Ctrl Pts',(-18.5985917525949,12.7748328937639,
12.));
#203329=CARTESIAN_POINT('Ctrl Pts',(-18.5962551167772,12.7733231262107,
0.));
#203330=CARTESIAN_POINT('Ctrl Pts',(-18.5962551167772,12.7733231262107,
12.));
#203331=CARTESIAN_POINT('Ctrl Pts',(-18.5942490615409,12.7720142287169,
0.));
#203332=CARTESIAN_POINT('Ctrl Pts',(-18.5942490615409,12.7720142287169,
12.));
#203333=CARTESIAN_POINT('Ctrl Pts',(-18.5925859134582,12.7709195951153,
0.));
#203334=CARTESIAN_POINT('Ctrl Pts',(-18.5925859134582,12.7709195951153,
12.));
#203335=CARTESIAN_POINT('Ctrl Pts',(-18.5912775137806,12.7700520897174,
0.));
#203336=CARTESIAN_POINT('Ctrl Pts',(-18.5912775137806,12.7700520897174,
12.));
#203337=CARTESIAN_POINT('Ctrl Pts',(-18.590332877722,12.7694215127923,0.));
#203338=CARTESIAN_POINT('Ctrl Pts',(-18.590332877722,12.7694215127923,12.));
#203339=CARTESIAN_POINT('Ctrl Pts',(-18.589871621842,12.7691103481996,0.));
#203340=CARTESIAN_POINT('Ctrl Pts',(-18.589871621842,12.7691103481996,12.));
#203341=CARTESIAN_POINT('Ctrl Pts',(-18.5896919669158,12.7689864266924,
0.));
#203342=CARTESIAN_POINT('Ctrl Pts',(-18.5896919669158,12.7689864266924,
12.));
#203343=CARTESIAN_POINT('Ctrl Pts',(-18.5896460962961,12.7689524524484,
0.));
#203344=CARTESIAN_POINT('Ctrl Pts',(-18.5896460962961,12.7689524524484,
12.));
#203345=CARTESIAN_POINT('Ctrl Pts',(-18.5896416359912,12.7689476255363,
0.));
#203346=CARTESIAN_POINT('Ctrl Pts',(-18.5896416359912,12.7689476255363,
12.));
#203347=CARTESIAN_POINT('',(-22.1787195904339,13.5685075571671,0.));
#203348=CARTESIAN_POINT('Ctrl Pts',(-22.1787195904339,13.5685075571671,
0.));
#203349=CARTESIAN_POINT('Ctrl Pts',(-22.1730081264583,13.5683460612913,
0.));
#203350=CARTESIAN_POINT('Ctrl Pts',(-22.1615922804939,13.5680170531724,
0.));
#203351=CARTESIAN_POINT('Ctrl Pts',(-22.1444897575076,13.5675054918922,
0.));
#203352=CARTESIAN_POINT('Ctrl Pts',(-22.1217288871823,13.5667873105179,
0.));
#203353=CARTESIAN_POINT('Ctrl Pts',(-22.0933486464442,13.5658294169106,
0.));
#203354=CARTESIAN_POINT('Ctrl Pts',(-22.0650393089492,13.5648113688894,
0.));
#203355=CARTESIAN_POINT('Ctrl Pts',(-22.0368009736227,13.5637332022393,
0.));
#203356=CARTESIAN_POINT('Ctrl Pts',(-22.0086337943431,13.5625949868313,
0.));
#203357=CARTESIAN_POINT('Ctrl Pts',(-21.9805379899192,13.5613968357589,
0.));
#203358=CARTESIAN_POINT('Ctrl Pts',(-21.9525138592862,13.5601389185315,
0.));
#203359=CARTESIAN_POINT('Ctrl Pts',(-21.9245617765827,13.5588214586672,
0.));
#203360=CARTESIAN_POINT('Ctrl Pts',(-21.8966821688876,13.5574447178484,
0.));
#203361=CARTESIAN_POINT('Ctrl Pts',(-21.8688754989401,13.5560089839426,
0.));
#203362=CARTESIAN_POINT('Ctrl Pts',(-21.841142245609,13.5545145573048,0.));
#203363=CARTESIAN_POINT('Ctrl Pts',(-21.8134828857963,13.5529617381569,
0.));
#203364=CARTESIAN_POINT('Ctrl Pts',(-21.7858978745848,13.5513508127232,
0.));
#203365=CARTESIAN_POINT('Ctrl Pts',(-21.7583876294532,13.5496820422186,
0.));
#203366=CARTESIAN_POINT('Ctrl Pts',(-21.730952541226,13.5479556704457,0.));
#203367=CARTESIAN_POINT('Ctrl Pts',(-21.7035929822939,13.546171929503,0.));
#203368=CARTESIAN_POINT('Ctrl Pts',(-21.676309315769,13.5443310461516,0.));
#203369=CARTESIAN_POINT('Ctrl Pts',(-21.6491019044647,13.5424332480698,
0.));
#203370=CARTESIAN_POINT('Ctrl Pts',(-21.6219711193951,13.5404787697798,
0.));
#203371=CARTESIAN_POINT('Ctrl Pts',(-21.5949173499022,13.5384678597206,
0.));
#203372=CARTESIAN_POINT('Ctrl Pts',(-21.5679410019011,13.5364007790292,
0.));
#203373=CARTESIAN_POINT('Ctrl Pts',(-21.5410424932511,13.5342777983225,
0.));
#203374=CARTESIAN_POINT('Ctrl Pts',(-21.5142222501671,13.5320991952145,
0.));
#203375=CARTESIAN_POINT('Ctrl Pts',(-21.487480703047,13.5298652514357,0.));
#203376=CARTESIAN_POINT('Ctrl Pts',(-21.4608182828695,13.5275762503553,
0.));
#203377=CARTESIAN_POINT('Ctrl Pts',(-21.4342354165254,13.5252324737795,
0.));
#203378=CARTESIAN_POINT('Ctrl Pts',(-21.4077325259318,13.5228342013508,
0.));
#203379=CARTESIAN_POINT('Ctrl Pts',(-21.3813100304967,13.5203817122496,
0.));
#203380=CARTESIAN_POINT('Ctrl Pts',(-21.3549683486219,13.5178752862461,
0.));
#203381=CARTESIAN_POINT('Ctrl Pts',(-21.328707899634,13.5153152050554,0.));
#203382=CARTESIAN_POINT('Ctrl Pts',(-21.3025291054236,13.5127017534972,
0.));
#203383=CARTESIAN_POINT('Ctrl Pts',(-21.2764323924442,13.5100352209207,
0.));
#203384=CARTESIAN_POINT('Ctrl Pts',(-21.2504181927429,13.5073159019454,
0.));
#203385=CARTESIAN_POINT('Ctrl Pts',(-21.224486942933,13.5045440957404,0.));
#203386=CARTESIAN_POINT('Ctrl Pts',(-21.1986390835825,13.5017201056088,
0.));
#203387=CARTESIAN_POINT('Ctrl Pts',(-21.1728750584173,13.4988442384491,
0.));
#203388=CARTESIAN_POINT('Ctrl Pts',(-21.1471953136209,13.4959168042934,
0.));
#203389=CARTESIAN_POINT('Ctrl Pts',(-21.1216002970209,13.4929381157778,
0.));
#203390=CARTESIAN_POINT('Ctrl Pts',(-21.0960904575048,13.4899084877718,
0.));
#203391=CARTESIAN_POINT('Ctrl Pts',(-21.0706662455202,13.4868282377191,
0.));
#203392=CARTESIAN_POINT('Ctrl Pts',(-21.0453281134247,13.4836976858912,
0.));
#203393=CARTESIAN_POINT('Ctrl Pts',(-21.0200765158885,13.4805171556822,
0.));
#203394=CARTESIAN_POINT('Ctrl Pts',(-20.9949119102592,13.4772869738879,
0.));
#203395=CARTESIAN_POINT('Ctrl Pts',(-20.9698347569476,13.4740074710087,
0.));
#203396=CARTESIAN_POINT('Ctrl Pts',(-20.9448455197557,13.4706789815166,
0.));
#203397=CARTESIAN_POINT('Ctrl Pts',(-20.9199446657584,13.4673018437718,
0.));
#203398=CARTESIAN_POINT('Ctrl Pts',(-20.8951326652158,13.4638763999725,
0.));
#203399=CARTESIAN_POINT('Ctrl Pts',(-20.8704099914641,13.4604029960983,
0.));
#203400=CARTESIAN_POINT('Ctrl Pts',(-20.8457771208082,13.4568819818631,
0.));
#203401=CARTESIAN_POINT('Ctrl Pts',(-20.821234532398,13.4533137106667,0.));
#203402=CARTESIAN_POINT('Ctrl Pts',(-20.7967827081227,13.4496985395637,
0.));
#203403=CARTESIAN_POINT('Ctrl Pts',(-20.7724221327608,13.4460368293688,
0.));
#203404=CARTESIAN_POINT('Ctrl Pts',(-20.7481532941013,13.4423289447561,
0.));
#203405=CARTESIAN_POINT('Ctrl Pts',(-20.7239766830675,13.4385752543663,
0.));
#203406=CARTESIAN_POINT('Ctrl Pts',(-20.6998927938288,13.4347761309154,
0.));
#203407=CARTESIAN_POINT('Ctrl Pts',(-20.6759021239103,13.4309319513119,
0.));
#203408=CARTESIAN_POINT('Ctrl Pts',(-20.6520051742869,13.4270430967651,
0.));
#203409=CARTESIAN_POINT('Ctrl Pts',(-20.6282024494237,13.4231099528179,
0.));
#203410=CARTESIAN_POINT('Ctrl Pts',(-20.6044944573153,13.4191329093932,
0.));
#203411=CARTESIAN_POINT('Ctrl Pts',(-20.5808817095155,13.4151123608411,
0.));
#203412=CARTESIAN_POINT('Ctrl Pts',(-20.5573647211639,13.4110487059912,
0.));
#203413=CARTESIAN_POINT('Ctrl Pts',(-20.5339440109956,13.4069423482076,
0.));
#203414=CARTESIAN_POINT('Ctrl Pts',(-20.5106201013753,13.4027936954529,
0.));
#203415=CARTESIAN_POINT('Ctrl Pts',(-20.487393518404,13.3986031603716,0.));
#203416=CARTESIAN_POINT('Ctrl Pts',(-20.4642647920038,13.3943711603739,
0.));
#203417=CARTESIAN_POINT('Ctrl Pts',(-20.4412344560008,13.3900981177255,
0.));
#203418=CARTESIAN_POINT('Ctrl Pts',(-20.4183030482002,13.3857844596387,
0.));
#203419=CARTESIAN_POINT('Ctrl Pts',(-20.3954711104502,13.3814306183719,
0.));
#203420=CARTESIAN_POINT('Ctrl Pts',(-20.3727391887184,13.3770370313188,
0.));
#203421=CARTESIAN_POINT('Ctrl Pts',(-20.3501078331814,13.3726041410867,
0.));
#203422=CARTESIAN_POINT('Ctrl Pts',(-20.3275775983029,13.3681323955826,
0.));
#203423=CARTESIAN_POINT('Ctrl Pts',(-20.3051490429048,13.3636222481016,
0.));
#203424=CARTESIAN_POINT('Ctrl Pts',(-20.2828227302339,13.3590741574195,
0.));
#203425=CARTESIAN_POINT('Ctrl Pts',(-20.2605992280122,13.3544885878889,
0.));
#203426=CARTESIAN_POINT('Ctrl Pts',(-20.2384791085359,13.3498660095386,
0.));
#203427=CARTESIAN_POINT('Ctrl Pts',(-20.216462948786,13.3452068981766,0.));
#203428=CARTESIAN_POINT('Ctrl Pts',(-20.1945513305235,13.3405117354971,
0.));
#203429=CARTESIAN_POINT('Ctrl Pts',(-20.1727448403817,13.3357810091903,
0.));
#203430=CARTESIAN_POINT('Ctrl Pts',(-20.1510440699474,13.3310152130564,
0.));
#203431=CARTESIAN_POINT('Ctrl Pts',(-20.1294496158402,13.3262148471226,
0.));
#203432=CARTESIAN_POINT('Ctrl Pts',(-20.1079620798375,13.3213804177587,
0.));
#203433=CARTESIAN_POINT('Ctrl Pts',(-20.0865820689883,13.3165124377962,
0.));
#203434=CARTESIAN_POINT('Ctrl Pts',(-20.0653101957188,13.3116114266515,
0.));
#203435=CARTESIAN_POINT('Ctrl Pts',(-20.0441470779345,13.3066779104515,
0.));
#203436=CARTESIAN_POINT('Ctrl Pts',(-20.0230933391038,13.3017124221637,
0.));
#203437=CARTESIAN_POINT('Ctrl Pts',(-20.0021496083738,13.2967155017306,
0.));
#203438=CARTESIAN_POINT('Ctrl Pts',(-19.981316520717,13.2916876962094,0.));
#203439=CARTESIAN_POINT('Ctrl Pts',(-19.9605947170586,13.286629559915,0.));
#203440=CARTESIAN_POINT('Ctrl Pts',(-19.9399848444019,13.2815416545663,
0.));
#203441=CARTESIAN_POINT('Ctrl Pts',(-19.9194875559422,13.2764245494357,
0.));
#203442=CARTESIAN_POINT('Ctrl Pts',(-19.8991035111745,13.271278821502,0.));
#203443=CARTESIAN_POINT('Ctrl Pts',(-19.8788333760577,13.2661050556132,
0.));
#203444=CARTESIAN_POINT('Ctrl Pts',(-19.8586778231715,13.2609038446529,
0.));
#203445=CARTESIAN_POINT('Ctrl Pts',(-19.8386375318634,13.2556757897086,
0.));
#203446=CARTESIAN_POINT('Ctrl Pts',(-19.8187131883917,13.2504215002457,
0.));
#203447=CARTESIAN_POINT('Ctrl Pts',(-19.7989054860495,13.2451415942805,
0.));
#203448=CARTESIAN_POINT('Ctrl Pts',(-19.7792151253289,13.2398366985675,
0.));
#203449=CARTESIAN_POINT('Ctrl Pts',(-19.7596428141168,13.2345074487963,
0.));
#203450=CARTESIAN_POINT('Ctrl Pts',(-19.7401892678697,13.2291544897899,
0.));
#203451=CARTESIAN_POINT('Ctrl Pts',(-19.7208552097868,13.2237784757065,
0.));
#203452=CARTESIAN_POINT('Ctrl Pts',(-19.7016413709685,13.2183800702436,
0.));
#203453=CARTESIAN_POINT('Ctrl Pts',(-19.6825484905823,13.2129599468485,
0.));
#203454=CARTESIAN_POINT('Ctrl Pts',(-19.6635773160936,13.2075187889529,
0.));
#203455=CARTESIAN_POINT('Ctrl Pts',(-19.6447286034772,13.2020572902065,
0.));
#203456=CARTESIAN_POINT('Ctrl Pts',(-19.6260031174244,13.1965761547151,
0.));
#203457=CARTESIAN_POINT('Ctrl Pts',(-19.6074016315414,13.1910760972814,
0.));
#203458=CARTESIAN_POINT('Ctrl Pts',(-19.5889249285338,13.1855578436471,
0.));
#203459=CARTESIAN_POINT('Ctrl Pts',(-19.5705738004667,13.1800221307673,
0.));
#203460=CARTESIAN_POINT('Ctrl Pts',(-19.5523490490244,13.1744697070911,
0.));
#203461=CARTESIAN_POINT('Ctrl Pts',(-19.5342514857562,13.168901332843,0.));
#203462=CARTESIAN_POINT('Ctrl Pts',(-19.5162819323213,13.1633177803101,
0.));
#203463=CARTESIAN_POINT('Ctrl Pts',(-19.4984412207082,13.1577198341245,
0.));
#203464=CARTESIAN_POINT('Ctrl Pts',(-19.4807301935268,13.1521082915853,
0.));
#203465=CARTESIAN_POINT('Ctrl Pts',(-19.4631497043258,13.1464839629971,
0.));
#203466=CARTESIAN_POINT('Ctrl Pts',(-19.4457006178876,13.1408476720061,
0.));
#203467=CARTESIAN_POINT('Ctrl Pts',(-19.4283838105262,13.1352002559438,
0.));
#203468=CARTESIAN_POINT('Ctrl Pts',(-19.4112001703557,13.1295425661634,
0.));
#203469=CARTESIAN_POINT('Ctrl Pts',(-19.3941505976263,13.1238754684177,
0.));
#203470=CARTESIAN_POINT('Ctrl Pts',(-19.3772360051091,13.118199843271,0.));
#203471=CARTESIAN_POINT('Ctrl Pts',(-19.3604573184515,13.1125165865022,
0.));
#203472=CARTESIAN_POINT('Ctrl Pts',(-19.3438154765395,13.1068266095186,
0.));
#203473=CARTESIAN_POINT('Ctrl Pts',(-19.3273114318269,13.1011308397591,
0.));
#203474=CARTESIAN_POINT('Ctrl Pts',(-19.310946150736,13.0954302211479,0.));
#203475=CARTESIAN_POINT('Ctrl Pts',(-19.2947206141247,13.0897257145968,
0.));
#203476=CARTESIAN_POINT('Ctrl Pts',(-19.2786358177198,13.0840182984949,
0.));
#203477=CARTESIAN_POINT('Ctrl Pts',(-19.2626927725596,13.0783089692118,
0.));
#203478=CARTESIAN_POINT('Ctrl Pts',(-19.2468925053989,13.0725987415859,
0.));
#203479=CARTESIAN_POINT('Ctrl Pts',(-19.2312360592033,13.0668886494795,
0.));
#203480=CARTESIAN_POINT('Ctrl Pts',(-19.2157244937142,13.0611797463915,
0.));
#203481=CARTESIAN_POINT('Ctrl Pts',(-19.2003588859772,13.0554731060538,
0.));
#203482=CARTESIAN_POINT('Ctrl Pts',(-19.1851403308825,13.0497698230441,
0.));
#203483=CARTESIAN_POINT('Ctrl Pts',(-19.1700699416622,13.0440710133772,
0.));
#203484=CARTESIAN_POINT('Ctrl Pts',(-19.155148850523,13.0383778152068,0.));
#203485=CARTESIAN_POINT('Ctrl Pts',(-19.1403782093386,13.0326913895838,
0.));
#203486=CARTESIAN_POINT('Ctrl Pts',(-19.1257591903099,13.0270129211976,
0.));
#203487=CARTESIAN_POINT('Ctrl Pts',(-19.111292986631,13.0213436191328,0.));
#203488=CARTESIAN_POINT('Ctrl Pts',(-19.0969808131228,13.0156847176096,
0.));
#203489=CARTESIAN_POINT('Ctrl Pts',(-19.0828239070484,13.0100374768788,
0.));
#203490=CARTESIAN_POINT('Ctrl Pts',(-19.0688235289437,13.0044031841382,
0.));
#203491=CARTESIAN_POINT('Ctrl Pts',(-19.0549809634354,12.9987831544502,
0.));
#203492=CARTESIAN_POINT('Ctrl Pts',(-19.0412975200398,12.9931787316514,
0.));
#203493=CARTESIAN_POINT('Ctrl Pts',(-19.0277745339909,12.9875912893003,
0.));
#203494=CARTESIAN_POINT('Ctrl Pts',(-19.014413367335,12.9820222318716,0.));
#203495=CARTESIAN_POINT('Ctrl Pts',(-19.0012154099792,12.9764729959206,
0.));
#203496=CARTESIAN_POINT('Ctrl Pts',(-18.9881820807585,12.9709450512747,
0.));
#203497=CARTESIAN_POINT('Ctrl Pts',(-18.9753148284473,12.9654399021868,
0.));
#203498=CARTESIAN_POINT('Ctrl Pts',(-18.9626151329226,12.9599590886317,
0.));
#203499=CARTESIAN_POINT('Ctrl Pts',(-18.9500845064714,12.9545041877377,
0.));
#203500=CARTESIAN_POINT('Ctrl Pts',(-18.9377244950435,12.9490768151821,
0.));
#203501=CARTESIAN_POINT('Ctrl Pts',(-18.9255366795196,12.9436786266106,
0.));
#203502=CARTESIAN_POINT('Ctrl Pts',(-18.9135226769466,12.9383113190375,
0.));
#203503=CARTESIAN_POINT('Ctrl Pts',(-18.9016841423402,12.9329766328184,
0.));
#203504=CARTESIAN_POINT('Ctrl Pts',(-18.8900227704888,12.9276763536372,
0.));
#203505=CARTESIAN_POINT('Ctrl Pts',(-18.8785402977528,12.9224123144982,
0.));
#203506=CARTESIAN_POINT('Ctrl Pts',(-18.8672385038328,12.9171863977047,
0.));
#203507=CARTESIAN_POINT('Ctrl Pts',(-18.8561192136201,12.9120005369066,
0.));
#203508=CARTESIAN_POINT('Ctrl Pts',(-18.8451842990986,12.9068567191856,
0.));
#203509=CARTESIAN_POINT('Ctrl Pts',(-18.834435681259,12.9017569871738,0.));
#203510=CARTESIAN_POINT('Ctrl Pts',(-18.8238753319124,12.8967034410752,
0.));
#203511=CARTESIAN_POINT('Ctrl Pts',(-18.8135052757815,12.8916982409931,
0.));
#203512=CARTESIAN_POINT('Ctrl Pts',(-18.8033275941939,12.8867436109543,
0.));
#203513=CARTESIAN_POINT('Ctrl Pts',(-18.7933444285867,12.8818418427474,
0.));
#203514=CARTESIAN_POINT('Ctrl Pts',(-18.7835579840481,12.8769952998097,
0.));
#203515=CARTESIAN_POINT('Ctrl Pts',(-18.7739705329029,12.8722064211814,
0.));
#203516=CARTESIAN_POINT('Ctrl Pts',(-18.7645844169568,12.8674777239656,
0.));
#203517=CARTESIAN_POINT('Ctrl Pts',(-18.7554020493888,12.8628118054172,
0.));
#203518=CARTESIAN_POINT('Ctrl Pts',(-18.7464259171248,12.8582113455644,
0.));
#203519=CARTESIAN_POINT('Ctrl Pts',(-18.7376585820851,12.8536791086315,
0.));
#203520=CARTESIAN_POINT('Ctrl Pts',(-18.7291026886552,12.849217951159,0.));
#203521=CARTESIAN_POINT('Ctrl Pts',(-18.7207609737701,12.8448308329494,
0.));
#203522=CARTESIAN_POINT('Ctrl Pts',(-18.7126362754446,12.8405208263432,
0.));
#203523=CARTESIAN_POINT('Ctrl Pts',(-18.7047315436296,12.8362911280362,
0.));
#203524=CARTESIAN_POINT('Ctrl Pts',(-18.6970498410173,12.832145059979,0.));
#203525=CARTESIAN_POINT('Ctrl Pts',(-18.6895943376172,12.8280860635231,
0.));
#203526=CARTESIAN_POINT('Ctrl Pts',(-18.6823683094139,12.8241176980016,
0.));
#203527=CARTESIAN_POINT('Ctrl Pts',(-18.6753751301091,12.8202436318473,
0.));
#203528=CARTESIAN_POINT('Ctrl Pts',(-18.6686182952798,12.8164676687361,
0.));
#203529=CARTESIAN_POINT('Ctrl Pts',(-18.6621014624746,12.8127937909632,
0.));
#203530=CARTESIAN_POINT('Ctrl Pts',(-18.6558284825772,12.8092261933858,
0.));
#203531=CARTESIAN_POINT('Ctrl Pts',(-18.6498034438986,12.805769331162,0.));
#203532=CARTESIAN_POINT('Ctrl Pts',(-18.6440306327457,12.8024278770153,
0.));
#203533=CARTESIAN_POINT('Ctrl Pts',(-18.63851447924,12.7992066625264,0.));
#203534=CARTESIAN_POINT('Ctrl Pts',(-18.6332595057005,12.7961106222251,
0.));
#203535=CARTESIAN_POINT('Ctrl Pts',(-18.6282702819371,12.7931447451556,
0.));
#203536=CARTESIAN_POINT('Ctrl Pts',(-18.6235516265575,12.7903142925234,
0.));
#203537=CARTESIAN_POINT('Ctrl Pts',(-18.6191087624752,12.7876249657834,
0.));
#203538=CARTESIAN_POINT('Ctrl Pts',(-18.6149475565189,12.78508316579,0.));
#203539=CARTESIAN_POINT('Ctrl Pts',(-18.611074482622,12.7826959526924,0.));
#203540=CARTESIAN_POINT('Ctrl Pts',(-18.6074961535723,12.7804705387658,
0.));
#203541=CARTESIAN_POINT('Ctrl Pts',(-18.6042190183703,12.7784139605067,
0.));
#203542=CARTESIAN_POINT('Ctrl Pts',(-18.6012488486708,12.7765325225082,
0.));
#203543=CARTESIAN_POINT('Ctrl Pts',(-18.5985917525949,12.7748328937639,
0.));
#203544=CARTESIAN_POINT('Ctrl Pts',(-18.5962551167772,12.7733231262107,
0.));
#203545=CARTESIAN_POINT('Ctrl Pts',(-18.5942490615409,12.7720142287169,
0.));
#203546=CARTESIAN_POINT('Ctrl Pts',(-18.5925859134582,12.7709195951153,
0.));
#203547=CARTESIAN_POINT('Ctrl Pts',(-18.5912775137806,12.7700520897174,
0.));
#203548=CARTESIAN_POINT('Ctrl Pts',(-18.590332877722,12.7694215127923,0.));
#203549=CARTESIAN_POINT('Ctrl Pts',(-18.589871621842,12.7691103481996,0.));
#203550=CARTESIAN_POINT('Ctrl Pts',(-18.5896919669158,12.7689864266924,
0.));
#203551=CARTESIAN_POINT('Ctrl Pts',(-18.5896460962961,12.7689524524484,
0.));
#203552=CARTESIAN_POINT('Ctrl Pts',(-18.5896416359912,12.7689476255363,
0.));
#203553=CARTESIAN_POINT('',(-22.1787195904339,13.5685075571671,0.));
#203554=CARTESIAN_POINT('Ctrl Pts',(-17.1452095830633,14.6513681262571,
0.));
#203555=CARTESIAN_POINT('Ctrl Pts',(-17.1452095830633,14.6513681262571,
12.));
#203556=CARTESIAN_POINT('Ctrl Pts',(-17.1452153999142,14.6513711852843,
0.));
#203557=CARTESIAN_POINT('Ctrl Pts',(-17.1452153999142,14.6513711852843,
12.));
#203558=CARTESIAN_POINT('Ctrl Pts',(-17.1452600887037,14.6514066997196,
0.));
#203559=CARTESIAN_POINT('Ctrl Pts',(-17.1452600887037,14.6514066997196,
12.));
#203560=CARTESIAN_POINT('Ctrl Pts',(-17.1454262858043,14.6515481598068,
0.));
#203561=CARTESIAN_POINT('Ctrl Pts',(-17.1454262858043,14.6515481598068,
12.));
#203562=CARTESIAN_POINT('Ctrl Pts',(-17.1458462295271,14.6519131634508,
0.));
#203563=CARTESIAN_POINT('Ctrl Pts',(-17.1458462295271,14.6519131634508,
12.));
#203564=CARTESIAN_POINT('Ctrl Pts',(-17.1466998098673,14.6526624064978,
0.));
#203565=CARTESIAN_POINT('Ctrl Pts',(-17.1466998098673,14.6526624064978,
12.));
#203566=CARTESIAN_POINT('Ctrl Pts',(-17.147876394491,14.6537016966184,0.));
#203567=CARTESIAN_POINT('Ctrl Pts',(-17.147876394491,14.6537016966184,12.));
#203568=CARTESIAN_POINT('Ctrl Pts',(-17.1493641837558,14.655024862281,0.));
#203569=CARTESIAN_POINT('Ctrl Pts',(-17.1493641837558,14.655024862281,12.));
#203570=CARTESIAN_POINT('Ctrl Pts',(-17.1511476869496,14.6566237952435,
0.));
#203571=CARTESIAN_POINT('Ctrl Pts',(-17.1511476869496,14.6566237952435,
12.));
#203572=CARTESIAN_POINT('Ctrl Pts',(-17.1532107762718,14.6584900555302,
0.));
#203573=CARTESIAN_POINT('Ctrl Pts',(-17.1532107762718,14.6584900555302,
12.));
#203574=CARTESIAN_POINT('Ctrl Pts',(-17.1555401986401,14.6606167169642,
0.));
#203575=CARTESIAN_POINT('Ctrl Pts',(-17.1555401986401,14.6606167169642,
12.));
#203576=CARTESIAN_POINT('Ctrl Pts',(-17.1581262646789,14.6629987285992,
0.));
#203577=CARTESIAN_POINT('Ctrl Pts',(-17.1581262646789,14.6629987285992,
12.));
#203578=CARTESIAN_POINT('Ctrl Pts',(-17.1609609517369,14.6656319165057,
0.));
#203579=CARTESIAN_POINT('Ctrl Pts',(-17.1609609517369,14.6656319165057,
12.));
#203580=CARTESIAN_POINT('Ctrl Pts',(-17.1640366762305,14.6685123374423,
0.));
#203581=CARTESIAN_POINT('Ctrl Pts',(-17.1640366762305,14.6685123374423,
12.));
#203582=CARTESIAN_POINT('Ctrl Pts',(-17.167344972302,14.671635583332,0.));
#203583=CARTESIAN_POINT('Ctrl Pts',(-17.167344972302,14.671635583332,12.));
#203584=CARTESIAN_POINT('Ctrl Pts',(-17.1708771619129,14.6749971333867,
0.));
#203585=CARTESIAN_POINT('Ctrl Pts',(-17.1708771619129,14.6749971333867,
12.));
#203586=CARTESIAN_POINT('Ctrl Pts',(-17.1746247499057,14.6785925615677,
0.));
#203587=CARTESIAN_POINT('Ctrl Pts',(-17.1746247499057,14.6785925615677,
12.));
#203588=CARTESIAN_POINT('Ctrl Pts',(-17.1785800350826,14.6824178576167,
0.));
#203589=CARTESIAN_POINT('Ctrl Pts',(-17.1785800350826,14.6824178576167,
12.));
#203590=CARTESIAN_POINT('Ctrl Pts',(-17.182736158472,14.686469452232,0.));
#203591=CARTESIAN_POINT('Ctrl Pts',(-17.182736158472,14.686469452232,12.));
#203592=CARTESIAN_POINT('Ctrl Pts',(-17.1870867909918,14.6907440526958,
0.));
#203593=CARTESIAN_POINT('Ctrl Pts',(-17.1870867909918,14.6907440526958,
12.));
#203594=CARTESIAN_POINT('Ctrl Pts',(-17.1916259308415,14.6952385361705,
0.));
#203595=CARTESIAN_POINT('Ctrl Pts',(-17.1916259308415,14.6952385361705,
12.));
#203596=CARTESIAN_POINT('Ctrl Pts',(-17.1963476411694,14.699949811582,0.));
#203597=CARTESIAN_POINT('Ctrl Pts',(-17.1963476411694,14.699949811582,12.));
#203598=CARTESIAN_POINT('Ctrl Pts',(-17.2012461084268,14.7048748502663,
0.));
#203599=CARTESIAN_POINT('Ctrl Pts',(-17.2012461084268,14.7048748502663,
12.));
#203600=CARTESIAN_POINT('Ctrl Pts',(-17.2063157097315,14.7100107213586,
0.));
#203601=CARTESIAN_POINT('Ctrl Pts',(-17.2063157097315,14.7100107213586,
12.));
#203602=CARTESIAN_POINT('Ctrl Pts',(-17.2115510835989,14.7153546289339,
0.));
#203603=CARTESIAN_POINT('Ctrl Pts',(-17.2115510835989,14.7153546289339,
12.));
#203604=CARTESIAN_POINT('Ctrl Pts',(-17.2169471814256,14.7209039390327,
0.));
#203605=CARTESIAN_POINT('Ctrl Pts',(-17.2169471814256,14.7209039390327,
12.));
#203606=CARTESIAN_POINT('Ctrl Pts',(-17.2224992099667,14.7266561494282,
0.));
#203607=CARTESIAN_POINT('Ctrl Pts',(-17.2224992099667,14.7266561494282,
12.));
#203608=CARTESIAN_POINT('Ctrl Pts',(-17.2282025904314,14.7326088681163,
0.));
#203609=CARTESIAN_POINT('Ctrl Pts',(-17.2282025904314,14.7326088681163,
12.));
#203610=CARTESIAN_POINT('Ctrl Pts',(-17.2340529062076,14.7387597858116,
0.));
#203611=CARTESIAN_POINT('Ctrl Pts',(-17.2340529062076,14.7387597858116,
12.));
#203612=CARTESIAN_POINT('Ctrl Pts',(-17.2400458713565,14.7451066593792,
0.));
#203613=CARTESIAN_POINT('Ctrl Pts',(-17.2400458713565,14.7451066593792,
12.));
#203614=CARTESIAN_POINT('Ctrl Pts',(-17.2461773413288,14.7516473175124,
0.));
#203615=CARTESIAN_POINT('Ctrl Pts',(-17.2461773413288,14.7516473175124,
12.));
#203616=CARTESIAN_POINT('Ctrl Pts',(-17.2524433146837,14.7583796616617,
0.));
#203617=CARTESIAN_POINT('Ctrl Pts',(-17.2524433146837,14.7583796616617,
12.));
#203618=CARTESIAN_POINT('Ctrl Pts',(-17.2588399401465,14.7653016697591,
0.));
#203619=CARTESIAN_POINT('Ctrl Pts',(-17.2588399401465,14.7653016697591,
12.));
#203620=CARTESIAN_POINT('Ctrl Pts',(-17.2653635155319,14.7724113956731,
0.));
#203621=CARTESIAN_POINT('Ctrl Pts',(-17.2653635155319,14.7724113956731,
12.));
#203622=CARTESIAN_POINT('Ctrl Pts',(-17.2720104735194,14.7797069617804,
0.));
#203623=CARTESIAN_POINT('Ctrl Pts',(-17.2720104735194,14.7797069617804,
12.));
#203624=CARTESIAN_POINT('Ctrl Pts',(-17.2787773704849,14.787186553128,0.));
#203625=CARTESIAN_POINT('Ctrl Pts',(-17.2787773704849,14.787186553128,12.));
#203626=CARTESIAN_POINT('Ctrl Pts',(-17.2856608733196,14.7948484105249,
0.));
#203627=CARTESIAN_POINT('Ctrl Pts',(-17.2856608733196,14.7948484105249,
12.));
#203628=CARTESIAN_POINT('Ctrl Pts',(-17.2926577496513,14.8026908254276,
0.));
#203629=CARTESIAN_POINT('Ctrl Pts',(-17.2926577496513,14.8026908254276,
12.));
#203630=CARTESIAN_POINT('Ctrl Pts',(-17.299764866148,14.8107121391035,0.));
#203631=CARTESIAN_POINT('Ctrl Pts',(-17.299764866148,14.8107121391035,12.));
#203632=CARTESIAN_POINT('Ctrl Pts',(-17.3069791853706,14.8189107410162,
0.));
#203633=CARTESIAN_POINT('Ctrl Pts',(-17.3069791853706,14.8189107410162,
12.));
#203634=CARTESIAN_POINT('Ctrl Pts',(-17.3142977632659,14.8272850675379,
0.));
#203635=CARTESIAN_POINT('Ctrl Pts',(-17.3142977632659,14.8272850675379,
12.));
#203636=CARTESIAN_POINT('Ctrl Pts',(-17.3217177462101,14.8358336004197,
0.));
#203637=CARTESIAN_POINT('Ctrl Pts',(-17.3217177462101,14.8358336004197,
12.));
#203638=CARTESIAN_POINT('Ctrl Pts',(-17.3292363662605,14.8445548643508,
0.));
#203639=CARTESIAN_POINT('Ctrl Pts',(-17.3292363662605,14.8445548643508,
12.));
#203640=CARTESIAN_POINT('Ctrl Pts',(-17.336850936485,14.8534474245433,0.));
#203641=CARTESIAN_POINT('Ctrl Pts',(-17.336850936485,14.8534474245433,12.));
#203642=CARTESIAN_POINT('Ctrl Pts',(-17.3445588463475,14.8625098843417,
0.));
#203643=CARTESIAN_POINT('Ctrl Pts',(-17.3445588463475,14.8625098843417,
12.));
#203644=CARTESIAN_POINT('Ctrl Pts',(-17.3523575568645,14.8717408826955,
0.));
#203645=CARTESIAN_POINT('Ctrl Pts',(-17.3523575568645,14.8717408826955,
12.));
#203646=CARTESIAN_POINT('Ctrl Pts',(-17.3602445978161,14.8811390927423,
0.));
#203647=CARTESIAN_POINT('Ctrl Pts',(-17.3602445978161,14.8811390927423,
12.));
#203648=CARTESIAN_POINT('Ctrl Pts',(-17.3682175653235,14.8907032205788,
0.));
#203649=CARTESIAN_POINT('Ctrl Pts',(-17.3682175653235,14.8907032205788,
12.));
#203650=CARTESIAN_POINT('Ctrl Pts',(-17.3762741193076,14.900432003961,0.));
#203651=CARTESIAN_POINT('Ctrl Pts',(-17.3762741193076,14.900432003961,12.));
#203652=CARTESIAN_POINT('Ctrl Pts',(-17.3844119809824,14.9103242110057,
0.));
#203653=CARTESIAN_POINT('Ctrl Pts',(-17.3844119809824,14.9103242110057,
12.));
#203654=CARTESIAN_POINT('Ctrl Pts',(-17.3926289303986,14.9203786389342,
0.));
#203655=CARTESIAN_POINT('Ctrl Pts',(-17.3926289303986,14.9203786389342,
12.));
#203656=CARTESIAN_POINT('Ctrl Pts',(-17.4009228040749,14.9305941128757,
0.));
#203657=CARTESIAN_POINT('Ctrl Pts',(-17.4009228040749,14.9305941128757,
12.));
#203658=CARTESIAN_POINT('Ctrl Pts',(-17.4092914926071,14.940969484645,0.));
#203659=CARTESIAN_POINT('Ctrl Pts',(-17.4092914926071,14.940969484645,12.));
#203660=CARTESIAN_POINT('Ctrl Pts',(-17.4177329382828,14.9515036315143,
0.));
#203661=CARTESIAN_POINT('Ctrl Pts',(-17.4177329382828,14.9515036315143,
12.));
#203662=CARTESIAN_POINT('Ctrl Pts',(-17.426245132709,14.9621954549827,0.));
#203663=CARTESIAN_POINT('Ctrl Pts',(-17.426245132709,14.9621954549827,12.));
#203664=CARTESIAN_POINT('Ctrl Pts',(-17.4348261151396,14.9730438799452,
0.));
#203665=CARTESIAN_POINT('Ctrl Pts',(-17.4348261151396,14.9730438799452,
12.));
#203666=CARTESIAN_POINT('Ctrl Pts',(-17.4434739707773,14.9840478538358,
0.));
#203667=CARTESIAN_POINT('Ctrl Pts',(-17.4434739707773,14.9840478538358,
12.));
#203668=CARTESIAN_POINT('Ctrl Pts',(-17.4521868291004,14.9952063457778,
0.));
#203669=CARTESIAN_POINT('Ctrl Pts',(-17.4521868291004,14.9952063457778,
12.));
#203670=CARTESIAN_POINT('Ctrl Pts',(-17.4609628621418,15.0065183456921,
0.));
#203671=CARTESIAN_POINT('Ctrl Pts',(-17.4609628621418,15.0065183456921,
12.));
#203672=CARTESIAN_POINT('Ctrl Pts',(-17.4698002829357,15.0179828635086,
0.));
#203673=CARTESIAN_POINT('Ctrl Pts',(-17.4698002829357,15.0179828635086,
12.));
#203674=CARTESIAN_POINT('Ctrl Pts',(-17.4786973441417,15.029598928488,0.));
#203675=CARTESIAN_POINT('Ctrl Pts',(-17.4786973441417,15.029598928488,12.));
#203676=CARTESIAN_POINT('Ctrl Pts',(-17.4876523366178,15.0413655884993,
0.));
#203677=CARTESIAN_POINT('Ctrl Pts',(-17.4876523366178,15.0413655884993,
12.));
#203678=CARTESIAN_POINT('Ctrl Pts',(-17.4966635880245,15.0532819093085,
0.));
#203679=CARTESIAN_POINT('Ctrl Pts',(-17.4966635880245,15.0532819093085,
12.));
#203680=CARTESIAN_POINT('Ctrl Pts',(-17.5057294613874,15.0653469738306,
0.));
#203681=CARTESIAN_POINT('Ctrl Pts',(-17.5057294613874,15.0653469738306,
12.));
#203682=CARTESIAN_POINT('Ctrl Pts',(-17.5148483539684,15.0775598815748,
0.));
#203683=CARTESIAN_POINT('Ctrl Pts',(-17.5148483539684,15.0775598815748,
12.));
#203684=CARTESIAN_POINT('Ctrl Pts',(-17.5240186961788,15.0899197481082,
0.));
#203685=CARTESIAN_POINT('Ctrl Pts',(-17.5240186961788,15.0899197481082,
12.));
#203686=CARTESIAN_POINT('Ctrl Pts',(-17.5332389504829,15.1024257045033,
0.));
#203687=CARTESIAN_POINT('Ctrl Pts',(-17.5332389504829,15.1024257045033,
12.));
#203688=CARTESIAN_POINT('Ctrl Pts',(-17.5425076102966,15.1150768967729,
0.));
#203689=CARTESIAN_POINT('Ctrl Pts',(-17.5425076102966,15.1150768967729,
12.));
#203690=CARTESIAN_POINT('Ctrl Pts',(-17.5518231989122,15.127872485314,0.));
#203691=CARTESIAN_POINT('Ctrl Pts',(-17.5518231989122,15.127872485314,12.));
#203692=CARTESIAN_POINT('Ctrl Pts',(-17.5611842686196,15.1408116444877,
0.));
#203693=CARTESIAN_POINT('Ctrl Pts',(-17.5611842686196,15.1408116444877,
12.));
#203694=CARTESIAN_POINT('Ctrl Pts',(-17.570589399803,15.1538935621714,0.));
#203695=CARTESIAN_POINT('Ctrl Pts',(-17.570589399803,15.1538935621714,12.));
#203696=CARTESIAN_POINT('Ctrl Pts',(-17.5800372000539,15.1671174393136,
0.));
#203697=CARTESIAN_POINT('Ctrl Pts',(-17.5800372000539,15.1671174393136,
12.));
#203698=CARTESIAN_POINT('Ctrl Pts',(-17.5895263032592,15.1804824894605,
0.));
#203699=CARTESIAN_POINT('Ctrl Pts',(-17.5895263032592,15.1804824894605,
12.));
#203700=CARTESIAN_POINT('Ctrl Pts',(-17.5990553687595,15.1939879383268,
0.));
#203701=CARTESIAN_POINT('Ctrl Pts',(-17.5990553687595,15.1939879383268,
12.));
#203702=CARTESIAN_POINT('Ctrl Pts',(-17.6086230806497,15.2076330234686,
0.));
#203703=CARTESIAN_POINT('Ctrl Pts',(-17.6086230806497,15.2076330234686,
12.));
#203704=CARTESIAN_POINT('Ctrl Pts',(-17.6182281470467,15.22141699392,0.));
#203705=CARTESIAN_POINT('Ctrl Pts',(-17.6182281470467,15.22141699392,12.));
#203706=CARTESIAN_POINT('Ctrl Pts',(-17.6278692993765,15.2353391098367,
0.));
#203707=CARTESIAN_POINT('Ctrl Pts',(-17.6278692993765,15.2353391098367,
12.));
#203708=CARTESIAN_POINT('Ctrl Pts',(-17.637545291637,15.2493986421091,0.));
#203709=CARTESIAN_POINT('Ctrl Pts',(-17.637545291637,15.2493986421091,12.));
#203710=CARTESIAN_POINT('Ctrl Pts',(-17.6472548997329,15.263594872029,0.));
#203711=CARTESIAN_POINT('Ctrl Pts',(-17.6472548997329,15.263594872029,12.));
#203712=CARTESIAN_POINT('Ctrl Pts',(-17.6569969209,15.2779270910238,0.));
#203713=CARTESIAN_POINT('Ctrl Pts',(-17.6569969209,15.2779270910238,12.));
#203714=CARTESIAN_POINT('Ctrl Pts',(-17.6667701731041,15.2923946003598,
0.));
#203715=CARTESIAN_POINT('Ctrl Pts',(-17.6667701731041,15.2923946003598,
12.));
#203716=CARTESIAN_POINT('Ctrl Pts',(-17.6765734944559,15.3069967108501,
0.));
#203717=CARTESIAN_POINT('Ctrl Pts',(-17.6765734944559,15.3069967108501,
12.));
#203718=CARTESIAN_POINT('Ctrl Pts',(-17.6864057426052,15.3217327425341,
0.));
#203719=CARTESIAN_POINT('Ctrl Pts',(-17.6864057426052,15.3217327425341,
12.));
#203720=CARTESIAN_POINT('Ctrl Pts',(-17.6962657941984,15.3366020244069,
0.));
#203721=CARTESIAN_POINT('Ctrl Pts',(-17.6962657941984,15.3366020244069,
12.));
#203722=CARTESIAN_POINT('Ctrl Pts',(-17.7061525444044,15.3516038942064,
0.));
#203723=CARTESIAN_POINT('Ctrl Pts',(-17.7061525444044,15.3516038942064,
12.));
#203724=CARTESIAN_POINT('Ctrl Pts',(-17.7160649064208,15.3667376981702,
0.));
#203725=CARTESIAN_POINT('Ctrl Pts',(-17.7160649064208,15.3667376981702,
12.));
#203726=CARTESIAN_POINT('Ctrl Pts',(-17.7260018109923,15.3820027907965,
0.));
#203727=CARTESIAN_POINT('Ctrl Pts',(-17.7260018109923,15.3820027907965,
12.));
#203728=CARTESIAN_POINT('Ctrl Pts',(-17.7359622059143,15.3973985345796,
0.));
#203729=CARTESIAN_POINT('Ctrl Pts',(-17.7359622059143,15.3973985345796,
12.));
#203730=CARTESIAN_POINT('Ctrl Pts',(-17.7459450555803,15.4129242997828,
0.));
#203731=CARTESIAN_POINT('Ctrl Pts',(-17.7459450555803,15.4129242997828,
12.));
#203732=CARTESIAN_POINT('Ctrl Pts',(-17.7559493405871,15.4285794642658,
0.));
#203733=CARTESIAN_POINT('Ctrl Pts',(-17.7559493405871,15.4285794642658,
12.));
#203734=CARTESIAN_POINT('Ctrl Pts',(-17.765974057326,15.4443634132865,0.));
#203735=CARTESIAN_POINT('Ctrl Pts',(-17.765974057326,15.4443634132865,12.));
#203736=CARTESIAN_POINT('Ctrl Pts',(-17.7760182175817,15.4602755393019,
0.));
#203737=CARTESIAN_POINT('Ctrl Pts',(-17.7760182175817,15.4602755393019,
12.));
#203738=CARTESIAN_POINT('Ctrl Pts',(-17.7860808481229,15.4763152417506,
0.));
#203739=CARTESIAN_POINT('Ctrl Pts',(-17.7860808481229,15.4763152417506,
12.));
#203740=CARTESIAN_POINT('Ctrl Pts',(-17.7961609903161,15.4924819268529,
0.));
#203741=CARTESIAN_POINT('Ctrl Pts',(-17.7961609903161,15.4924819268529,
12.));
#203742=CARTESIAN_POINT('Ctrl Pts',(-17.8062576997964,15.5087750074728,
0.));
#203743=CARTESIAN_POINT('Ctrl Pts',(-17.8062576997964,15.5087750074728,
12.));
#203744=CARTESIAN_POINT('Ctrl Pts',(-17.8163700461263,15.5251939029558,
0.));
#203745=CARTESIAN_POINT('Ctrl Pts',(-17.8163700461263,15.5251939029558,
12.));
#203746=CARTESIAN_POINT('Ctrl Pts',(-17.8264971124606,15.5417380389639,
0.));
#203747=CARTESIAN_POINT('Ctrl Pts',(-17.8264971124606,15.5417380389639,
12.));
#203748=CARTESIAN_POINT('Ctrl Pts',(-17.8366379952078,15.5584068472976,
0.));
#203749=CARTESIAN_POINT('Ctrl Pts',(-17.8366379952078,15.5584068472976,
12.));
#203750=CARTESIAN_POINT('Ctrl Pts',(-17.8467918036977,15.5751997657153,
0.));
#203751=CARTESIAN_POINT('Ctrl Pts',(-17.8467918036977,15.5751997657153,
12.));
#203752=CARTESIAN_POINT('Ctrl Pts',(-17.8569576598996,15.5921162378183,
0.));
#203753=CARTESIAN_POINT('Ctrl Pts',(-17.8569576598996,15.5921162378183,
12.));
#203754=CARTESIAN_POINT('Ctrl Pts',(-17.8671346981388,15.6091557129205,
0.));
#203755=CARTESIAN_POINT('Ctrl Pts',(-17.8671346981388,15.6091557129205,
12.));
#203756=CARTESIAN_POINT('Ctrl Pts',(-17.8773220648125,15.6263176459107,
0.));
#203757=CARTESIAN_POINT('Ctrl Pts',(-17.8773220648125,15.6263176459107,
12.));
#203758=CARTESIAN_POINT('Ctrl Pts',(-17.8875189181095,15.6436014971088,
0.));
#203759=CARTESIAN_POINT('Ctrl Pts',(-17.8875189181095,15.6436014971088,
12.));
#203760=CARTESIAN_POINT('Ctrl Pts',(-17.8977244277247,15.6610067321036,
0.));
#203761=CARTESIAN_POINT('Ctrl Pts',(-17.8977244277247,15.6610067321036,
12.));
#203762=CARTESIAN_POINT('Ctrl Pts',(-17.9079377746118,15.6785328216467,
0.));
#203763=CARTESIAN_POINT('Ctrl Pts',(-17.9079377746118,15.6785328216467,
12.));
#203764=CARTESIAN_POINT('Ctrl Pts',(-17.918158150746,15.6961792415526,0.));
#203765=CARTESIAN_POINT('Ctrl Pts',(-17.918158150746,15.6961792415526,12.));
#203766=CARTESIAN_POINT('Ctrl Pts',(-17.9283847588837,15.713945472584,0.));
#203767=CARTESIAN_POINT('Ctrl Pts',(-17.9283847588837,15.713945472584,12.));
#203768=CARTESIAN_POINT('Ctrl Pts',(-17.9386168123261,15.7318310003334,
0.));
#203769=CARTESIAN_POINT('Ctrl Pts',(-17.9386168123261,15.7318310003334,
12.));
#203770=CARTESIAN_POINT('Ctrl Pts',(-17.9488535346776,15.7498353150856,
0.));
#203771=CARTESIAN_POINT('Ctrl Pts',(-17.9488535346776,15.7498353150856,
12.));
#203772=CARTESIAN_POINT('Ctrl Pts',(-17.9590941596236,15.7679579117072,
0.));
#203773=CARTESIAN_POINT('Ctrl Pts',(-17.9590941596236,15.7679579117072,
12.));
#203774=CARTESIAN_POINT('Ctrl Pts',(-17.9693379307297,15.786198289572,0.));
#203775=CARTESIAN_POINT('Ctrl Pts',(-17.9693379307297,15.786198289572,12.));
#203776=CARTESIAN_POINT('Ctrl Pts',(-17.9795841012383,15.8045559524674,
0.));
#203777=CARTESIAN_POINT('Ctrl Pts',(-17.9795841012383,15.8045559524674,
12.));
#203778=CARTESIAN_POINT('Ctrl Pts',(-17.9898319338664,15.8230304084963,
0.));
#203779=CARTESIAN_POINT('Ctrl Pts',(-17.9898319338664,15.8230304084963,
12.));
#203780=CARTESIAN_POINT('Ctrl Pts',(-18.0000807006055,15.8416211699681,
0.));
#203781=CARTESIAN_POINT('Ctrl Pts',(-18.0000807006055,15.8416211699681,
12.));
#203782=CARTESIAN_POINT('Ctrl Pts',(-18.010329682521,15.8603277532834,0.));
#203783=CARTESIAN_POINT('Ctrl Pts',(-18.010329682521,15.8603277532834,12.));
#203784=CARTESIAN_POINT('Ctrl Pts',(-18.0205781695773,15.8791496788685,
0.));
#203785=CARTESIAN_POINT('Ctrl Pts',(-18.0205781695773,15.8791496788685,
12.));
#203786=CARTESIAN_POINT('Ctrl Pts',(-18.0308254604638,15.8980864711043,
0.));
#203787=CARTESIAN_POINT('Ctrl Pts',(-18.0308254604638,15.8980864711043,
12.));
#203788=CARTESIAN_POINT('Ctrl Pts',(-18.0410708624208,15.9171376582436,
0.));
#203789=CARTESIAN_POINT('Ctrl Pts',(-18.0410708624208,15.9171376582436,
12.));
#203790=CARTESIAN_POINT('Ctrl Pts',(-18.0513136910691,15.9363027723244,
0.));
#203791=CARTESIAN_POINT('Ctrl Pts',(-18.0513136910691,15.9363027723244,
12.));
#203792=CARTESIAN_POINT('Ctrl Pts',(-18.061553270236,15.9555813490645,0.));
#203793=CARTESIAN_POINT('Ctrl Pts',(-18.061553270236,15.9555813490645,12.));
#203794=CARTESIAN_POINT('Ctrl Pts',(-18.071788931796,15.9749729277848,0.));
#203795=CARTESIAN_POINT('Ctrl Pts',(-18.071788931796,15.9749729277848,12.));
#203796=CARTESIAN_POINT('Ctrl Pts',(-18.0820200155239,15.9944770513616,
0.));
#203797=CARTESIAN_POINT('Ctrl Pts',(-18.0820200155239,15.9944770513616,
12.));
#203798=CARTESIAN_POINT('Ctrl Pts',(-18.0922458689464,16.0140932661612,
0.));
#203799=CARTESIAN_POINT('Ctrl Pts',(-18.0922458689464,16.0140932661612,
12.));
#203800=CARTESIAN_POINT('Ctrl Pts',(-18.1024658471966,16.0338211219693,
0.));
#203801=CARTESIAN_POINT('Ctrl Pts',(-18.1024658471966,16.0338211219693,
12.));
#203802=CARTESIAN_POINT('Ctrl Pts',(-18.1126793128688,16.0536601719124,
0.));
#203803=CARTESIAN_POINT('Ctrl Pts',(-18.1126793128688,16.0536601719124,
12.));
#203804=CARTESIAN_POINT('Ctrl Pts',(-18.1228856358746,16.0736099723664,
0.));
#203805=CARTESIAN_POINT('Ctrl Pts',(-18.1228856358746,16.0736099723664,
12.));
#203806=CARTESIAN_POINT('Ctrl Pts',(-18.1330841933099,16.0936700829108,
0.));
#203807=CARTESIAN_POINT('Ctrl Pts',(-18.1330841933099,16.0936700829108,
12.));
#203808=CARTESIAN_POINT('Ctrl Pts',(-18.1432743693231,16.113840066279,0.));
#203809=CARTESIAN_POINT('Ctrl Pts',(-18.1432743693231,16.113840066279,12.));
#203810=CARTESIAN_POINT('Ctrl Pts',(-18.1534555549851,16.1341194882987,
0.));
#203811=CARTESIAN_POINT('Ctrl Pts',(-18.1534555549851,16.1341194882987,
12.));
#203812=CARTESIAN_POINT('Ctrl Pts',(-18.1636271481616,16.1545079178261,
0.));
#203813=CARTESIAN_POINT('Ctrl Pts',(-18.1636271481616,16.1545079178261,
12.));
#203814=CARTESIAN_POINT('Ctrl Pts',(-18.1737885533852,16.1750049266673,
0.));
#203815=CARTESIAN_POINT('Ctrl Pts',(-18.1737885533852,16.1750049266673,
12.));
#203816=CARTESIAN_POINT('Ctrl Pts',(-18.1839391817335,16.1956100895076,
0.));
#203817=CARTESIAN_POINT('Ctrl Pts',(-18.1839391817335,16.1956100895076,
12.));
#203818=CARTESIAN_POINT('Ctrl Pts',(-18.1940784507232,16.2163229838878,
0.));
#203819=CARTESIAN_POINT('Ctrl Pts',(-18.1940784507232,16.2163229838878,
12.));
#203820=CARTESIAN_POINT('Ctrl Pts',(-18.2042057842037,16.237143190164,0.));
#203821=CARTESIAN_POINT('Ctrl Pts',(-18.2042057842037,16.237143190164,12.));
#203822=CARTESIAN_POINT('Ctrl Pts',(-18.214320612253,16.2580702914615,0.));
#203823=CARTESIAN_POINT('Ctrl Pts',(-18.214320612253,16.2580702914615,12.));
#203824=CARTESIAN_POINT('Ctrl Pts',(-18.2244223710745,16.2791038736223,
0.));
#203825=CARTESIAN_POINT('Ctrl Pts',(-18.2244223710745,16.2791038736223,
12.));
#203826=CARTESIAN_POINT('Ctrl Pts',(-18.2345105028981,16.3002435251378,
0.));
#203827=CARTESIAN_POINT('Ctrl Pts',(-18.2345105028981,16.3002435251378,
12.));
#203828=CARTESIAN_POINT('Ctrl Pts',(-18.2445844558742,16.3214888370988,
0.));
#203829=CARTESIAN_POINT('Ctrl Pts',(-18.2445844558742,16.3214888370988,
12.));
#203830=CARTESIAN_POINT('Ctrl Pts',(-18.2546436839609,16.342839403159,0.));
#203831=CARTESIAN_POINT('Ctrl Pts',(-18.2546436839609,16.342839403159,12.));
#203832=CARTESIAN_POINT('Ctrl Pts',(-18.2646876468169,16.3642948194869,
0.));
#203833=CARTESIAN_POINT('Ctrl Pts',(-18.2646876468169,16.3642948194869,
12.));
#203834=CARTESIAN_POINT('Ctrl Pts',(-18.2747158096934,16.385854684708,0.));
#203835=CARTESIAN_POINT('Ctrl Pts',(-18.2747158096934,16.385854684708,12.));
#203836=CARTESIAN_POINT('Ctrl Pts',(-18.2847276433308,16.4075185998454,
0.));
#203837=CARTESIAN_POINT('Ctrl Pts',(-18.2847276433308,16.4075185998454,
12.));
#203838=CARTESIAN_POINT('Ctrl Pts',(-18.2947226238509,16.4292861682377,
0.));
#203839=CARTESIAN_POINT('Ctrl Pts',(-18.2947226238509,16.4292861682377,
12.));
#203840=CARTESIAN_POINT('Ctrl Pts',(-18.3047002326858,16.4511569955231,
0.));
#203841=CARTESIAN_POINT('Ctrl Pts',(-18.3047002326858,16.4511569955231,
12.));
#203842=CARTESIAN_POINT('Ctrl Pts',(-18.3146599565229,16.4731306896439,
0.));
#203843=CARTESIAN_POINT('Ctrl Pts',(-18.3146599565229,16.4731306896439,
12.));
#203844=CARTESIAN_POINT('Ctrl Pts',(-18.3246012872468,16.4952068608344,
0.));
#203845=CARTESIAN_POINT('Ctrl Pts',(-18.3246012872468,16.4952068608344,
12.));
#203846=CARTESIAN_POINT('Ctrl Pts',(-18.3345237218864,16.5173851216045,
0.));
#203847=CARTESIAN_POINT('Ctrl Pts',(-18.3345237218864,16.5173851216045,
12.));
#203848=CARTESIAN_POINT('Ctrl Pts',(-18.3444267625601,16.5396650867139,
0.));
#203849=CARTESIAN_POINT('Ctrl Pts',(-18.3444267625601,16.5396650867139,
12.));
#203850=CARTESIAN_POINT('Ctrl Pts',(-18.3543099164331,16.5620463731414,
0.));
#203851=CARTESIAN_POINT('Ctrl Pts',(-18.3543099164331,16.5620463731414,
12.));
#203852=CARTESIAN_POINT('Ctrl Pts',(-18.364172695589,16.5845286000218,0.));
#203853=CARTESIAN_POINT('Ctrl Pts',(-18.364172695589,16.5845286000218,12.));
#203854=CARTESIAN_POINT('Ctrl Pts',(-18.3740146168879,16.6071113885711,
0.));
#203855=CARTESIAN_POINT('Ctrl Pts',(-18.3740146168879,16.6071113885711,
12.));
#203856=CARTESIAN_POINT('Ctrl Pts',(-18.3838352018327,16.6297943620056,
0.));
#203857=CARTESIAN_POINT('Ctrl Pts',(-18.3838352018327,16.6297943620056,
12.));
#203858=CARTESIAN_POINT('Ctrl Pts',(-18.3936339764332,16.6525771454513,
0.));
#203859=CARTESIAN_POINT('Ctrl Pts',(-18.3936339764332,16.6525771454513,
12.));
#203860=CARTESIAN_POINT('Ctrl Pts',(-18.4034104710789,16.6754593658513,
0.));
#203861=CARTESIAN_POINT('Ctrl Pts',(-18.4034104710789,16.6754593658513,
12.));
#203862=CARTESIAN_POINT('Ctrl Pts',(-18.413164220399,16.698440651849,0.));
#203863=CARTESIAN_POINT('Ctrl Pts',(-18.413164220399,16.698440651849,12.));
#203864=CARTESIAN_POINT('Ctrl Pts',(-18.4228947633186,16.7215206338818,
0.));
#203865=CARTESIAN_POINT('Ctrl Pts',(-18.4228947633186,16.7215206338818,
12.));
#203866=CARTESIAN_POINT('Ctrl Pts',(-18.4326016431392,16.7446989442882,
0.));
#203867=CARTESIAN_POINT('Ctrl Pts',(-18.4326016431392,16.7446989442882,
12.));
#203868=CARTESIAN_POINT('Ctrl Pts',(-18.4422844076099,16.7679752173992,
0.));
#203869=CARTESIAN_POINT('Ctrl Pts',(-18.4422844076099,16.7679752173992,
12.));
#203870=CARTESIAN_POINT('Ctrl Pts',(-18.4519426090124,16.791349089629,0.));
#203871=CARTESIAN_POINT('Ctrl Pts',(-18.4519426090124,16.791349089629,12.));
#203872=CARTESIAN_POINT('Ctrl Pts',(-18.4615758042305,16.8148201995472,
0.));
#203873=CARTESIAN_POINT('Ctrl Pts',(-18.4615758042305,16.8148201995472,
12.));
#203874=CARTESIAN_POINT('Ctrl Pts',(-18.4711835548622,16.8383881879707,
0.));
#203875=CARTESIAN_POINT('Ctrl Pts',(-18.4711835548622,16.8383881879707,
12.));
#203876=CARTESIAN_POINT('Ctrl Pts',(-18.4807654268769,16.8620526977169,
0.));
#203877=CARTESIAN_POINT('Ctrl Pts',(-18.4807654268769,16.8620526977169,
12.));
#203878=CARTESIAN_POINT('Ctrl Pts',(-18.4903209902226,16.8858133733086,
0.));
#203879=CARTESIAN_POINT('Ctrl Pts',(-18.4903209902226,16.8858133733086,
12.));
#203880=CARTESIAN_POINT('Ctrl Pts',(-18.4998498184619,16.9096698606942,
0.));
#203881=CARTESIAN_POINT('Ctrl Pts',(-18.4998498184619,16.9096698606942,
12.));
#203882=CARTESIAN_POINT('Ctrl Pts',(-18.5093514883835,16.9336218069353,
0.));
#203883=CARTESIAN_POINT('Ctrl Pts',(-18.5093514883835,16.9336218069353,
12.));
#203884=CARTESIAN_POINT('Ctrl Pts',(-18.518825579666,16.957668859934,0.));
#203885=CARTESIAN_POINT('Ctrl Pts',(-18.518825579666,16.957668859934,12.));
#203886=CARTESIAN_POINT('Ctrl Pts',(-18.5282716744198,16.9818106680382,
0.));
#203887=CARTESIAN_POINT('Ctrl Pts',(-18.5282716744198,16.9818106680382,
12.));
#203888=CARTESIAN_POINT('Ctrl Pts',(-18.5376893576961,17.0060468805099,
0.));
#203889=CARTESIAN_POINT('Ctrl Pts',(-18.5376893576961,17.0060468805099,
12.));
#203890=CARTESIAN_POINT('Ctrl Pts',(-18.5470782182089,17.030377148174,0.));
#203891=CARTESIAN_POINT('Ctrl Pts',(-18.5470782182089,17.030377148174,12.));
#203892=CARTESIAN_POINT('Ctrl Pts',(-18.5564378489628,17.0548011239751,
0.));
#203893=CARTESIAN_POINT('Ctrl Pts',(-18.5564378489628,17.0548011239751,
12.));
#203894=CARTESIAN_POINT('Ctrl Pts',(-18.5657678479788,17.0793184636079,
0.));
#203895=CARTESIAN_POINT('Ctrl Pts',(-18.5657678479788,17.0793184636079,
12.));
#203896=CARTESIAN_POINT('Ctrl Pts',(-18.5750678188543,17.1039288260001,
0.));
#203897=CARTESIAN_POINT('Ctrl Pts',(-18.5750678188543,17.1039288260001,
12.));
#203898=CARTESIAN_POINT('Ctrl Pts',(-18.5843373717253,17.1286318741185,
0.));
#203899=CARTESIAN_POINT('Ctrl Pts',(-18.5843373717253,17.1286318741185,
12.));
#203900=CARTESIAN_POINT('Ctrl Pts',(-18.5935761222833,17.1534272741646,
0.));
#203901=CARTESIAN_POINT('Ctrl Pts',(-18.5935761222833,17.1534272741646,
12.));
#203902=CARTESIAN_POINT('Ctrl Pts',(-18.6027836898826,17.1783146940131,
0.));
#203903=CARTESIAN_POINT('Ctrl Pts',(-18.6027836898826,17.1783146940131,
12.));
#203904=CARTESIAN_POINT('Ctrl Pts',(-18.6119596959957,17.2032938019288,
0.));
#203905=CARTESIAN_POINT('Ctrl Pts',(-18.6119596959957,17.2032938019288,
12.));
#203906=CARTESIAN_POINT('Ctrl Pts',(-18.6211037624041,17.2283642650519,
0.));
#203907=CARTESIAN_POINT('Ctrl Pts',(-18.6211037624041,17.2283642650519,
12.));
#203908=CARTESIAN_POINT('Ctrl Pts',(-18.630215509794,17.2535257482186,0.));
#203909=CARTESIAN_POINT('Ctrl Pts',(-18.630215509794,17.2535257482186,12.));
#203910=CARTESIAN_POINT('Ctrl Pts',(-18.639294555474,17.278777912021,0.));
#203911=CARTESIAN_POINT('Ctrl Pts',(-18.639294555474,17.278777912021,12.));
#203912=CARTESIAN_POINT('Ctrl Pts',(-18.6483405141853,17.3041204135069,
0.));
#203913=CARTESIAN_POINT('Ctrl Pts',(-18.6483405141853,17.3041204135069,
12.));
#203914=CARTESIAN_POINT('Ctrl Pts',(-18.6573530024019,17.3295529098612,
0.));
#203915=CARTESIAN_POINT('Ctrl Pts',(-18.6573530024019,17.3295529098612,
12.));
#203916=CARTESIAN_POINT('Ctrl Pts',(-18.6663316416569,17.3550750612438,
0.));
#203917=CARTESIAN_POINT('Ctrl Pts',(-18.6663316416569,17.3550750612438,
12.));
#203918=CARTESIAN_POINT('Ctrl Pts',(-18.6752760624045,17.3806865340744,
0.));
#203919=CARTESIAN_POINT('Ctrl Pts',(-18.6752760624045,17.3806865340744,
12.));
#203920=CARTESIAN_POINT('Ctrl Pts',(-18.6841859073472,17.4063870038563,
0.));
#203921=CARTESIAN_POINT('Ctrl Pts',(-18.6841859073472,17.4063870038563,
12.));
#203922=CARTESIAN_POINT('Ctrl Pts',(-18.6930608357421,17.4321761588148,
0.));
#203923=CARTESIAN_POINT('Ctrl Pts',(-18.6930608357421,17.4321761588148,
12.));
#203924=CARTESIAN_POINT('Ctrl Pts',(-18.7019005250322,17.4580537012764,
0.));
#203925=CARTESIAN_POINT('Ctrl Pts',(-18.7019005250322,17.4580537012764,
12.));
#203926=CARTESIAN_POINT('Ctrl Pts',(-18.7107046613941,17.4840193397176,
0.));
#203927=CARTESIAN_POINT('Ctrl Pts',(-18.7107046613941,17.4840193397176,
12.));
#203928=CARTESIAN_POINT('Ctrl Pts',(-18.7194729318128,17.5100727820891,
0.));
#203929=CARTESIAN_POINT('Ctrl Pts',(-18.7194729318128,17.5100727820891,
12.));
#203930=CARTESIAN_POINT('Ctrl Pts',(-18.728205015716,17.5362137287604,0.));
#203931=CARTESIAN_POINT('Ctrl Pts',(-18.728205015716,17.5362137287604,12.));
#203932=CARTESIAN_POINT('Ctrl Pts',(-18.7369005764558,17.5624418653248,
0.));
#203933=CARTESIAN_POINT('Ctrl Pts',(-18.7369005764558,17.5624418653248,
12.));
#203934=CARTESIAN_POINT('Ctrl Pts',(-18.7455592536667,17.5887568561361,
0.));
#203935=CARTESIAN_POINT('Ctrl Pts',(-18.7455592536667,17.5887568561361,
12.));
#203936=CARTESIAN_POINT('Ctrl Pts',(-18.7541806530935,17.6151583356988,
0.));
#203937=CARTESIAN_POINT('Ctrl Pts',(-18.7541806530935,17.6151583356988,
12.));
#203938=CARTESIAN_POINT('Ctrl Pts',(-18.7627643613139,17.6416459210646,
0.));
#203939=CARTESIAN_POINT('Ctrl Pts',(-18.7627643613139,17.6416459210646,
12.));
#203940=CARTESIAN_POINT('Ctrl Pts',(-18.7713099642673,17.6682192274197,
0.));
#203941=CARTESIAN_POINT('Ctrl Pts',(-18.7713099642673,17.6682192274197,
12.));
#203942=CARTESIAN_POINT('Ctrl Pts',(-18.7798170641305,17.6948778822981,
0.));
#203943=CARTESIAN_POINT('Ctrl Pts',(-18.7798170641305,17.6948778822981,
12.));
#203944=CARTESIAN_POINT('Ctrl Pts',(-18.7882852976016,17.7216215409019,
0.));
#203945=CARTESIAN_POINT('Ctrl Pts',(-18.7882852976016,17.7216215409019,
12.));
#203946=CARTESIAN_POINT('Ctrl Pts',(-18.7967143519444,17.7484498996916,
0.));
#203947=CARTESIAN_POINT('Ctrl Pts',(-18.7967143519444,17.7484498996916,
12.));
#203948=CARTESIAN_POINT('Ctrl Pts',(-18.8051039860543,17.7753627137898,
0.));
#203949=CARTESIAN_POINT('Ctrl Pts',(-18.8051039860543,17.7753627137898,
12.));
#203950=CARTESIAN_POINT('Ctrl Pts',(-18.8134540340581,17.8023598011135,
0.));
#203951=CARTESIAN_POINT('Ctrl Pts',(-18.8134540340581,17.8023598011135,
12.));
#203952=CARTESIAN_POINT('Ctrl Pts',(-18.8217643886368,17.8294410311105,
0.));
#203953=CARTESIAN_POINT('Ctrl Pts',(-18.8217643886368,17.8294410311105,
12.));
#203954=CARTESIAN_POINT('Ctrl Pts',(-18.8300349896187,17.8566063174871,
0.));
#203955=CARTESIAN_POINT('Ctrl Pts',(-18.8300349896187,17.8566063174871,
12.));
#203956=CARTESIAN_POINT('Ctrl Pts',(-18.8366196462746,17.8784057509434,
0.));
#203957=CARTESIAN_POINT('Ctrl Pts',(-18.8366196462746,17.8784057509434,
12.));
#203958=CARTESIAN_POINT('Ctrl Pts',(-18.8415402351882,17.8947931177853,
0.));
#203959=CARTESIAN_POINT('Ctrl Pts',(-18.8415402351882,17.8947931177853,
12.));
#203960=CARTESIAN_POINT('Ctrl Pts',(-18.8448126709726,17.9057348246611,
0.));
#203961=CARTESIAN_POINT('Ctrl Pts',(-18.8448126709726,17.9057348246611,
12.));
#203962=CARTESIAN_POINT('Ctrl Pts',(-18.8464468996588,17.9112098770111,
0.));
#203963=CARTESIAN_POINT('Ctrl Pts',(-18.8464468996588,17.9112098770111,
12.));
#203964=CARTESIAN_POINT('',(-18.8464468996588,17.9112098770111,0.));
#203965=CARTESIAN_POINT('Ctrl Pts',(-17.1452095830633,14.6513681262571,
0.));
#203966=CARTESIAN_POINT('Ctrl Pts',(-17.1452153999142,14.6513711852843,
0.));
#203967=CARTESIAN_POINT('Ctrl Pts',(-17.1452600887037,14.6514066997196,
0.));
#203968=CARTESIAN_POINT('Ctrl Pts',(-17.1454262858043,14.6515481598068,
0.));
#203969=CARTESIAN_POINT('Ctrl Pts',(-17.1458462295271,14.6519131634508,
0.));
#203970=CARTESIAN_POINT('Ctrl Pts',(-17.1466998098673,14.6526624064978,
0.));
#203971=CARTESIAN_POINT('Ctrl Pts',(-17.147876394491,14.6537016966184,0.));
#203972=CARTESIAN_POINT('Ctrl Pts',(-17.1493641837558,14.655024862281,0.));
#203973=CARTESIAN_POINT('Ctrl Pts',(-17.1511476869496,14.6566237952435,
0.));
#203974=CARTESIAN_POINT('Ctrl Pts',(-17.1532107762718,14.6584900555302,
0.));
#203975=CARTESIAN_POINT('Ctrl Pts',(-17.1555401986401,14.6606167169642,
0.));
#203976=CARTESIAN_POINT('Ctrl Pts',(-17.1581262646789,14.6629987285992,
0.));
#203977=CARTESIAN_POINT('Ctrl Pts',(-17.1609609517369,14.6656319165057,
0.));
#203978=CARTESIAN_POINT('Ctrl Pts',(-17.1640366762305,14.6685123374423,
0.));
#203979=CARTESIAN_POINT('Ctrl Pts',(-17.167344972302,14.671635583332,0.));
#203980=CARTESIAN_POINT('Ctrl Pts',(-17.1708771619129,14.6749971333867,
0.));
#203981=CARTESIAN_POINT('Ctrl Pts',(-17.1746247499057,14.6785925615677,
0.));
#203982=CARTESIAN_POINT('Ctrl Pts',(-17.1785800350826,14.6824178576167,
0.));
#203983=CARTESIAN_POINT('Ctrl Pts',(-17.182736158472,14.686469452232,0.));
#203984=CARTESIAN_POINT('Ctrl Pts',(-17.1870867909918,14.6907440526958,
0.));
#203985=CARTESIAN_POINT('Ctrl Pts',(-17.1916259308415,14.6952385361705,
0.));
#203986=CARTESIAN_POINT('Ctrl Pts',(-17.1963476411694,14.699949811582,0.));
#203987=CARTESIAN_POINT('Ctrl Pts',(-17.2012461084268,14.7048748502663,
0.));
#203988=CARTESIAN_POINT('Ctrl Pts',(-17.2063157097315,14.7100107213586,
0.));
#203989=CARTESIAN_POINT('Ctrl Pts',(-17.2115510835989,14.7153546289339,
0.));
#203990=CARTESIAN_POINT('Ctrl Pts',(-17.2169471814256,14.7209039390327,
0.));
#203991=CARTESIAN_POINT('Ctrl Pts',(-17.2224992099667,14.7266561494282,
0.));
#203992=CARTESIAN_POINT('Ctrl Pts',(-17.2282025904314,14.7326088681163,
0.));
#203993=CARTESIAN_POINT('Ctrl Pts',(-17.2340529062076,14.7387597858116,
0.));
#203994=CARTESIAN_POINT('Ctrl Pts',(-17.2400458713565,14.7451066593792,
0.));
#203995=CARTESIAN_POINT('Ctrl Pts',(-17.2461773413288,14.7516473175124,
0.));
#203996=CARTESIAN_POINT('Ctrl Pts',(-17.2524433146837,14.7583796616617,
0.));
#203997=CARTESIAN_POINT('Ctrl Pts',(-17.2588399401465,14.7653016697591,
0.));
#203998=CARTESIAN_POINT('Ctrl Pts',(-17.2653635155319,14.7724113956731,
0.));
#203999=CARTESIAN_POINT('Ctrl Pts',(-17.2720104735194,14.7797069617804,
0.));
#204000=CARTESIAN_POINT('Ctrl Pts',(-17.2787773704849,14.787186553128,0.));
#204001=CARTESIAN_POINT('Ctrl Pts',(-17.2856608733196,14.7948484105249,
0.));
#204002=CARTESIAN_POINT('Ctrl Pts',(-17.2926577496513,14.8026908254276,
0.));
#204003=CARTESIAN_POINT('Ctrl Pts',(-17.299764866148,14.8107121391035,0.));
#204004=CARTESIAN_POINT('Ctrl Pts',(-17.3069791853706,14.8189107410162,
0.));
#204005=CARTESIAN_POINT('Ctrl Pts',(-17.3142977632659,14.8272850675379,
0.));
#204006=CARTESIAN_POINT('Ctrl Pts',(-17.3217177462101,14.8358336004197,
0.));
#204007=CARTESIAN_POINT('Ctrl Pts',(-17.3292363662605,14.8445548643508,
0.));
#204008=CARTESIAN_POINT('Ctrl Pts',(-17.336850936485,14.8534474245433,0.));
#204009=CARTESIAN_POINT('Ctrl Pts',(-17.3445588463475,14.8625098843417,
0.));
#204010=CARTESIAN_POINT('Ctrl Pts',(-17.3523575568645,14.8717408826955,
0.));
#204011=CARTESIAN_POINT('Ctrl Pts',(-17.3602445978161,14.8811390927423,
0.));
#204012=CARTESIAN_POINT('Ctrl Pts',(-17.3682175653235,14.8907032205788,
0.));
#204013=CARTESIAN_POINT('Ctrl Pts',(-17.3762741193076,14.900432003961,0.));
#204014=CARTESIAN_POINT('Ctrl Pts',(-17.3844119809824,14.9103242110057,
0.));
#204015=CARTESIAN_POINT('Ctrl Pts',(-17.3926289303986,14.9203786389342,
0.));
#204016=CARTESIAN_POINT('Ctrl Pts',(-17.4009228040749,14.9305941128757,
0.));
#204017=CARTESIAN_POINT('Ctrl Pts',(-17.4092914926071,14.940969484645,0.));
#204018=CARTESIAN_POINT('Ctrl Pts',(-17.4177329382828,14.9515036315143,
0.));
#204019=CARTESIAN_POINT('Ctrl Pts',(-17.426245132709,14.9621954549827,0.));
#204020=CARTESIAN_POINT('Ctrl Pts',(-17.4348261151396,14.9730438799452,
0.));
#204021=CARTESIAN_POINT('Ctrl Pts',(-17.4434739707773,14.9840478538358,
0.));
#204022=CARTESIAN_POINT('Ctrl Pts',(-17.4521868291004,14.9952063457778,
0.));
#204023=CARTESIAN_POINT('Ctrl Pts',(-17.4609628621418,15.0065183456921,
0.));
#204024=CARTESIAN_POINT('Ctrl Pts',(-17.4698002829357,15.0179828635086,
0.));
#204025=CARTESIAN_POINT('Ctrl Pts',(-17.4786973441417,15.029598928488,0.));
#204026=CARTESIAN_POINT('Ctrl Pts',(-17.4876523366178,15.0413655884993,
0.));
#204027=CARTESIAN_POINT('Ctrl Pts',(-17.4966635880245,15.0532819093085,
0.));
#204028=CARTESIAN_POINT('Ctrl Pts',(-17.5057294613874,15.0653469738306,
0.));
#204029=CARTESIAN_POINT('Ctrl Pts',(-17.5148483539684,15.0775598815748,
0.));
#204030=CARTESIAN_POINT('Ctrl Pts',(-17.5240186961788,15.0899197481082,
0.));
#204031=CARTESIAN_POINT('Ctrl Pts',(-17.5332389504829,15.1024257045033,
0.));
#204032=CARTESIAN_POINT('Ctrl Pts',(-17.5425076102966,15.1150768967729,
0.));
#204033=CARTESIAN_POINT('Ctrl Pts',(-17.5518231989122,15.127872485314,0.));
#204034=CARTESIAN_POINT('Ctrl Pts',(-17.5611842686196,15.1408116444877,
0.));
#204035=CARTESIAN_POINT('Ctrl Pts',(-17.570589399803,15.1538935621714,0.));
#204036=CARTESIAN_POINT('Ctrl Pts',(-17.5800372000539,15.1671174393136,
0.));
#204037=CARTESIAN_POINT('Ctrl Pts',(-17.5895263032592,15.1804824894605,
0.));
#204038=CARTESIAN_POINT('Ctrl Pts',(-17.5990553687595,15.1939879383268,
0.));
#204039=CARTESIAN_POINT('Ctrl Pts',(-17.6086230806497,15.2076330234686,
0.));
#204040=CARTESIAN_POINT('Ctrl Pts',(-17.6182281470467,15.22141699392,0.));
#204041=CARTESIAN_POINT('Ctrl Pts',(-17.6278692993765,15.2353391098367,
0.));
#204042=CARTESIAN_POINT('Ctrl Pts',(-17.637545291637,15.2493986421091,0.));
#204043=CARTESIAN_POINT('Ctrl Pts',(-17.6472548997329,15.263594872029,0.));
#204044=CARTESIAN_POINT('Ctrl Pts',(-17.6569969209,15.2779270910238,0.));
#204045=CARTESIAN_POINT('Ctrl Pts',(-17.6667701731041,15.2923946003598,
0.));
#204046=CARTESIAN_POINT('Ctrl Pts',(-17.6765734944559,15.3069967108501,
0.));
#204047=CARTESIAN_POINT('Ctrl Pts',(-17.6864057426052,15.3217327425341,
0.));
#204048=CARTESIAN_POINT('Ctrl Pts',(-17.6962657941984,15.3366020244069,
0.));
#204049=CARTESIAN_POINT('Ctrl Pts',(-17.7061525444044,15.3516038942064,
0.));
#204050=CARTESIAN_POINT('Ctrl Pts',(-17.7160649064208,15.3667376981702,
0.));
#204051=CARTESIAN_POINT('Ctrl Pts',(-17.7260018109923,15.3820027907965,
0.));
#204052=CARTESIAN_POINT('Ctrl Pts',(-17.7359622059143,15.3973985345796,
0.));
#204053=CARTESIAN_POINT('Ctrl Pts',(-17.7459450555803,15.4129242997828,
0.));
#204054=CARTESIAN_POINT('Ctrl Pts',(-17.7559493405871,15.4285794642658,
0.));
#204055=CARTESIAN_POINT('Ctrl Pts',(-17.765974057326,15.4443634132865,0.));
#204056=CARTESIAN_POINT('Ctrl Pts',(-17.7760182175817,15.4602755393019,
0.));
#204057=CARTESIAN_POINT('Ctrl Pts',(-17.7860808481229,15.4763152417506,
0.));
#204058=CARTESIAN_POINT('Ctrl Pts',(-17.7961609903161,15.4924819268529,
0.));
#204059=CARTESIAN_POINT('Ctrl Pts',(-17.8062576997964,15.5087750074728,
0.));
#204060=CARTESIAN_POINT('Ctrl Pts',(-17.8163700461263,15.5251939029558,
0.));
#204061=CARTESIAN_POINT('Ctrl Pts',(-17.8264971124606,15.5417380389639,
0.));
#204062=CARTESIAN_POINT('Ctrl Pts',(-17.8366379952078,15.5584068472976,
0.));
#204063=CARTESIAN_POINT('Ctrl Pts',(-17.8467918036977,15.5751997657153,
0.));
#204064=CARTESIAN_POINT('Ctrl Pts',(-17.8569576598996,15.5921162378183,
0.));
#204065=CARTESIAN_POINT('Ctrl Pts',(-17.8671346981388,15.6091557129205,
0.));
#204066=CARTESIAN_POINT('Ctrl Pts',(-17.8773220648125,15.6263176459107,
0.));
#204067=CARTESIAN_POINT('Ctrl Pts',(-17.8875189181095,15.6436014971088,
0.));
#204068=CARTESIAN_POINT('Ctrl Pts',(-17.8977244277247,15.6610067321036,
0.));
#204069=CARTESIAN_POINT('Ctrl Pts',(-17.9079377746118,15.6785328216467,
0.));
#204070=CARTESIAN_POINT('Ctrl Pts',(-17.918158150746,15.6961792415526,0.));
#204071=CARTESIAN_POINT('Ctrl Pts',(-17.9283847588837,15.713945472584,0.));
#204072=CARTESIAN_POINT('Ctrl Pts',(-17.9386168123261,15.7318310003334,
0.));
#204073=CARTESIAN_POINT('Ctrl Pts',(-17.9488535346776,15.7498353150856,
0.));
#204074=CARTESIAN_POINT('Ctrl Pts',(-17.9590941596236,15.7679579117072,
0.));
#204075=CARTESIAN_POINT('Ctrl Pts',(-17.9693379307297,15.786198289572,0.));
#204076=CARTESIAN_POINT('Ctrl Pts',(-17.9795841012383,15.8045559524674,
0.));
#204077=CARTESIAN_POINT('Ctrl Pts',(-17.9898319338664,15.8230304084963,
0.));
#204078=CARTESIAN_POINT('Ctrl Pts',(-18.0000807006055,15.8416211699681,
0.));
#204079=CARTESIAN_POINT('Ctrl Pts',(-18.010329682521,15.8603277532834,0.));
#204080=CARTESIAN_POINT('Ctrl Pts',(-18.0205781695773,15.8791496788685,
0.));
#204081=CARTESIAN_POINT('Ctrl Pts',(-18.0308254604638,15.8980864711043,
0.));
#204082=CARTESIAN_POINT('Ctrl Pts',(-18.0410708624208,15.9171376582436,
0.));
#204083=CARTESIAN_POINT('Ctrl Pts',(-18.0513136910691,15.9363027723244,
0.));
#204084=CARTESIAN_POINT('Ctrl Pts',(-18.061553270236,15.9555813490645,0.));
#204085=CARTESIAN_POINT('Ctrl Pts',(-18.071788931796,15.9749729277848,0.));
#204086=CARTESIAN_POINT('Ctrl Pts',(-18.0820200155239,15.9944770513616,
0.));
#204087=CARTESIAN_POINT('Ctrl Pts',(-18.0922458689464,16.0140932661612,
0.));
#204088=CARTESIAN_POINT('Ctrl Pts',(-18.1024658471966,16.0338211219693,
0.));
#204089=CARTESIAN_POINT('Ctrl Pts',(-18.1126793128688,16.0536601719124,
0.));
#204090=CARTESIAN_POINT('Ctrl Pts',(-18.1228856358746,16.0736099723664,
0.));
#204091=CARTESIAN_POINT('Ctrl Pts',(-18.1330841933099,16.0936700829108,
0.));
#204092=CARTESIAN_POINT('Ctrl Pts',(-18.1432743693231,16.113840066279,0.));
#204093=CARTESIAN_POINT('Ctrl Pts',(-18.1534555549851,16.1341194882987,
0.));
#204094=CARTESIAN_POINT('Ctrl Pts',(-18.1636271481616,16.1545079178261,
0.));
#204095=CARTESIAN_POINT('Ctrl Pts',(-18.1737885533852,16.1750049266673,
0.));
#204096=CARTESIAN_POINT('Ctrl Pts',(-18.1839391817335,16.1956100895076,
0.));
#204097=CARTESIAN_POINT('Ctrl Pts',(-18.1940784507232,16.2163229838878,
0.));
#204098=CARTESIAN_POINT('Ctrl Pts',(-18.2042057842037,16.237143190164,0.));
#204099=CARTESIAN_POINT('Ctrl Pts',(-18.214320612253,16.2580702914615,0.));
#204100=CARTESIAN_POINT('Ctrl Pts',(-18.2244223710745,16.2791038736223,
0.));
#204101=CARTESIAN_POINT('Ctrl Pts',(-18.2345105028981,16.3002435251378,
0.));
#204102=CARTESIAN_POINT('Ctrl Pts',(-18.2445844558742,16.3214888370988,
0.));
#204103=CARTESIAN_POINT('Ctrl Pts',(-18.2546436839609,16.342839403159,0.));
#204104=CARTESIAN_POINT('Ctrl Pts',(-18.2646876468169,16.3642948194869,
0.));
#204105=CARTESIAN_POINT('Ctrl Pts',(-18.2747158096934,16.385854684708,0.));
#204106=CARTESIAN_POINT('Ctrl Pts',(-18.2847276433308,16.4075185998454,
0.));
#204107=CARTESIAN_POINT('Ctrl Pts',(-18.2947226238509,16.4292861682377,
0.));
#204108=CARTESIAN_POINT('Ctrl Pts',(-18.3047002326858,16.4511569955231,
0.));
#204109=CARTESIAN_POINT('Ctrl Pts',(-18.3146599565229,16.4731306896439,
0.));
#204110=CARTESIAN_POINT('Ctrl Pts',(-18.3246012872468,16.4952068608344,
0.));
#204111=CARTESIAN_POINT('Ctrl Pts',(-18.3345237218864,16.5173851216045,
0.));
#204112=CARTESIAN_POINT('Ctrl Pts',(-18.3444267625601,16.5396650867139,
0.));
#204113=CARTESIAN_POINT('Ctrl Pts',(-18.3543099164331,16.5620463731414,
0.));
#204114=CARTESIAN_POINT('Ctrl Pts',(-18.364172695589,16.5845286000218,0.));
#204115=CARTESIAN_POINT('Ctrl Pts',(-18.3740146168879,16.6071113885711,
0.));
#204116=CARTESIAN_POINT('Ctrl Pts',(-18.3838352018327,16.6297943620056,
0.));
#204117=CARTESIAN_POINT('Ctrl Pts',(-18.3936339764332,16.6525771454513,
0.));
#204118=CARTESIAN_POINT('Ctrl Pts',(-18.4034104710789,16.6754593658513,
0.));
#204119=CARTESIAN_POINT('Ctrl Pts',(-18.413164220399,16.698440651849,0.));
#204120=CARTESIAN_POINT('Ctrl Pts',(-18.4228947633186,16.7215206338818,
0.));
#204121=CARTESIAN_POINT('Ctrl Pts',(-18.4326016431392,16.7446989442882,
0.));
#204122=CARTESIAN_POINT('Ctrl Pts',(-18.4422844076099,16.7679752173992,
0.));
#204123=CARTESIAN_POINT('Ctrl Pts',(-18.4519426090124,16.791349089629,0.));
#204124=CARTESIAN_POINT('Ctrl Pts',(-18.4615758042305,16.8148201995472,
0.));
#204125=CARTESIAN_POINT('Ctrl Pts',(-18.4711835548622,16.8383881879707,
0.));
#204126=CARTESIAN_POINT('Ctrl Pts',(-18.4807654268769,16.8620526977169,
0.));
#204127=CARTESIAN_POINT('Ctrl Pts',(-18.4903209902226,16.8858133733086,
0.));
#204128=CARTESIAN_POINT('Ctrl Pts',(-18.4998498184619,16.9096698606942,
0.));
#204129=CARTESIAN_POINT('Ctrl Pts',(-18.5093514883835,16.9336218069353,
0.));
#204130=CARTESIAN_POINT('Ctrl Pts',(-18.518825579666,16.957668859934,0.));
#204131=CARTESIAN_POINT('Ctrl Pts',(-18.5282716744198,16.9818106680382,
0.));
#204132=CARTESIAN_POINT('Ctrl Pts',(-18.5376893576961,17.0060468805099,
0.));
#204133=CARTESIAN_POINT('Ctrl Pts',(-18.5470782182089,17.030377148174,0.));
#204134=CARTESIAN_POINT('Ctrl Pts',(-18.5564378489628,17.0548011239751,
0.));
#204135=CARTESIAN_POINT('Ctrl Pts',(-18.5657678479788,17.0793184636079,
0.));
#204136=CARTESIAN_POINT('Ctrl Pts',(-18.5750678188543,17.1039288260001,
0.));
#204137=CARTESIAN_POINT('Ctrl Pts',(-18.5843373717253,17.1286318741185,
0.));
#204138=CARTESIAN_POINT('Ctrl Pts',(-18.5935761222833,17.1534272741646,
0.));
#204139=CARTESIAN_POINT('Ctrl Pts',(-18.6027836898826,17.1783146940131,
0.));
#204140=CARTESIAN_POINT('Ctrl Pts',(-18.6119596959957,17.2032938019288,
0.));
#204141=CARTESIAN_POINT('Ctrl Pts',(-18.6211037624041,17.2283642650519,
0.));
#204142=CARTESIAN_POINT('Ctrl Pts',(-18.630215509794,17.2535257482186,0.));
#204143=CARTESIAN_POINT('Ctrl Pts',(-18.639294555474,17.278777912021,0.));
#204144=CARTESIAN_POINT('Ctrl Pts',(-18.6483405141853,17.3041204135069,
0.));
#204145=CARTESIAN_POINT('Ctrl Pts',(-18.6573530024019,17.3295529098612,
0.));
#204146=CARTESIAN_POINT('Ctrl Pts',(-18.6663316416569,17.3550750612438,
0.));
#204147=CARTESIAN_POINT('Ctrl Pts',(-18.6752760624045,17.3806865340744,
0.));
#204148=CARTESIAN_POINT('Ctrl Pts',(-18.6841859073472,17.4063870038563,
0.));
#204149=CARTESIAN_POINT('Ctrl Pts',(-18.6930608357421,17.4321761588148,
0.));
#204150=CARTESIAN_POINT('Ctrl Pts',(-18.7019005250322,17.4580537012764,
0.));
#204151=CARTESIAN_POINT('Ctrl Pts',(-18.7107046613941,17.4840193397176,
0.));
#204152=CARTESIAN_POINT('Ctrl Pts',(-18.7194729318128,17.5100727820891,
0.));
#204153=CARTESIAN_POINT('Ctrl Pts',(-18.728205015716,17.5362137287604,0.));
#204154=CARTESIAN_POINT('Ctrl Pts',(-18.7369005764558,17.5624418653248,
0.));
#204155=CARTESIAN_POINT('Ctrl Pts',(-18.7455592536667,17.5887568561361,
0.));
#204156=CARTESIAN_POINT('Ctrl Pts',(-18.7541806530935,17.6151583356988,
0.));
#204157=CARTESIAN_POINT('Ctrl Pts',(-18.7627643613139,17.6416459210646,
0.));
#204158=CARTESIAN_POINT('Ctrl Pts',(-18.7713099642673,17.6682192274197,
0.));
#204159=CARTESIAN_POINT('Ctrl Pts',(-18.7798170641305,17.6948778822981,
0.));
#204160=CARTESIAN_POINT('Ctrl Pts',(-18.7882852976016,17.7216215409019,
0.));
#204161=CARTESIAN_POINT('Ctrl Pts',(-18.7967143519444,17.7484498996916,
0.));
#204162=CARTESIAN_POINT('Ctrl Pts',(-18.8051039860543,17.7753627137898,
0.));
#204163=CARTESIAN_POINT('Ctrl Pts',(-18.8134540340581,17.8023598011135,
0.));
#204164=CARTESIAN_POINT('Ctrl Pts',(-18.8217643886368,17.8294410311105,
0.));
#204165=CARTESIAN_POINT('Ctrl Pts',(-18.8300349896187,17.8566063174871,
0.));
#204166=CARTESIAN_POINT('Ctrl Pts',(-18.8366196462746,17.8784057509434,
0.));
#204167=CARTESIAN_POINT('Ctrl Pts',(-18.8415402351882,17.8947931177853,
0.));
#204168=CARTESIAN_POINT('Ctrl Pts',(-18.8448126709726,17.9057348246611,
0.));
#204169=CARTESIAN_POINT('Ctrl Pts',(-18.8464468996588,17.9112098770111,
0.));
#204170=CARTESIAN_POINT('',(-18.8464468996588,17.9112098770111,0.));
#204171=CARTESIAN_POINT('Origin',(-12.1729687575668,17.7219872369693,0.));
#204172=CARTESIAN_POINT('',(-12.7689476255363,18.5896416359912,0.));
#204173=CARTESIAN_POINT('',(-12.7689476255363,18.5896416359912,0.));
#204174=CARTESIAN_POINT('',(-6.08648437878338,8.86099361848466,0.));
#204175=CARTESIAN_POINT('Ctrl Pts',(-17.9112098770111,18.8464468996588,
0.));
#204176=CARTESIAN_POINT('Ctrl Pts',(-17.9112098770111,18.8464468996588,
12.));
#204177=CARTESIAN_POINT('Ctrl Pts',(-17.9057348246595,18.8448126709691,
0.));
#204178=CARTESIAN_POINT('Ctrl Pts',(-17.9057348246595,18.8448126709691,
12.));
#204179=CARTESIAN_POINT('Ctrl Pts',(-17.8947931177807,18.8415402351786,
0.));
#204180=CARTESIAN_POINT('Ctrl Pts',(-17.8947931177807,18.8415402351786,
12.));
#204181=CARTESIAN_POINT('Ctrl Pts',(-17.8784057509356,18.8366196462581,
0.));
#204182=CARTESIAN_POINT('Ctrl Pts',(-17.8784057509356,18.8366196462581,
12.));
#204183=CARTESIAN_POINT('Ctrl Pts',(-17.8566063174771,18.8300349895974,
0.));
#204184=CARTESIAN_POINT('Ctrl Pts',(-17.8566063174771,18.8300349895974,
12.));
#204185=CARTESIAN_POINT('Ctrl Pts',(-17.8294410311006,18.8217643886157,
0.));
#204186=CARTESIAN_POINT('Ctrl Pts',(-17.8294410311006,18.8217643886157,
12.));
#204187=CARTESIAN_POINT('Ctrl Pts',(-17.8023598011057,18.8134540340417,
0.));
#204188=CARTESIAN_POINT('Ctrl Pts',(-17.8023598011057,18.8134540340417,
12.));
#204189=CARTESIAN_POINT('Ctrl Pts',(-17.7753627137853,18.8051039860448,
0.));
#204190=CARTESIAN_POINT('Ctrl Pts',(-17.7753627137853,18.8051039860448,
12.));
#204191=CARTESIAN_POINT('Ctrl Pts',(-17.7484498996905,18.7967143519419,
0.));
#204192=CARTESIAN_POINT('Ctrl Pts',(-17.7484498996905,18.7967143519419,
12.));
#204193=CARTESIAN_POINT('Ctrl Pts',(-17.7216215409035,18.7882852976049,
0.));
#204194=CARTESIAN_POINT('Ctrl Pts',(-17.7216215409035,18.7882852976049,
12.));
#204195=CARTESIAN_POINT('Ctrl Pts',(-17.6948778823014,18.7798170641374,
0.));
#204196=CARTESIAN_POINT('Ctrl Pts',(-17.6948778823014,18.7798170641374,
12.));
#204197=CARTESIAN_POINT('Ctrl Pts',(-17.6682192274236,18.7713099642754,
0.));
#204198=CARTESIAN_POINT('Ctrl Pts',(-17.6682192274236,18.7713099642754,
12.));
#204199=CARTESIAN_POINT('Ctrl Pts',(-17.6416459210681,18.762764361321,0.));
#204200=CARTESIAN_POINT('Ctrl Pts',(-17.6416459210681,18.762764361321,12.));
#204201=CARTESIAN_POINT('Ctrl Pts',(-17.6151583357012,18.7541806530984,
0.));
#204202=CARTESIAN_POINT('Ctrl Pts',(-17.6151583357012,18.7541806530984,
12.));
#204203=CARTESIAN_POINT('Ctrl Pts',(-17.5887568561371,18.7455592536687,
0.));
#204204=CARTESIAN_POINT('Ctrl Pts',(-17.5887568561371,18.7455592536687,
12.));
#204205=CARTESIAN_POINT('Ctrl Pts',(-17.5624418653245,18.7369005764553,
0.));
#204206=CARTESIAN_POINT('Ctrl Pts',(-17.5624418653245,18.7369005764553,
12.));
#204207=CARTESIAN_POINT('Ctrl Pts',(-17.5362137287593,18.7282050157138,
0.));
#204208=CARTESIAN_POINT('Ctrl Pts',(-17.5362137287593,18.7282050157138,
12.));
#204209=CARTESIAN_POINT('Ctrl Pts',(-17.5100727820876,18.7194729318098,
0.));
#204210=CARTESIAN_POINT('Ctrl Pts',(-17.5100727820876,18.7194729318098,
12.));
#204211=CARTESIAN_POINT('Ctrl Pts',(-17.4840193397162,18.7107046613912,
0.));
#204212=CARTESIAN_POINT('Ctrl Pts',(-17.4840193397162,18.7107046613912,
12.));
#204213=CARTESIAN_POINT('Ctrl Pts',(-17.4580537012753,18.70190052503,0.));
#204214=CARTESIAN_POINT('Ctrl Pts',(-17.4580537012753,18.70190052503,12.));
#204215=CARTESIAN_POINT('Ctrl Pts',(-17.4321761588142,18.6930608357409,
0.));
#204216=CARTESIAN_POINT('Ctrl Pts',(-17.4321761588142,18.6930608357409,
12.));
#204217=CARTESIAN_POINT('Ctrl Pts',(-17.4063870038562,18.6841859073471,
0.));
#204218=CARTESIAN_POINT('Ctrl Pts',(-17.4063870038562,18.6841859073471,
12.));
#204219=CARTESIAN_POINT('Ctrl Pts',(-17.3806865340747,18.6752760624052,
0.));
#204220=CARTESIAN_POINT('Ctrl Pts',(-17.3806865340747,18.6752760624052,
12.));
#204221=CARTESIAN_POINT('Ctrl Pts',(-17.3550750612443,18.6663316416582,
0.));
#204222=CARTESIAN_POINT('Ctrl Pts',(-17.3550750612443,18.6663316416582,
12.));
#204223=CARTESIAN_POINT('Ctrl Pts',(-17.3295529098618,18.6573530024033,
0.));
#204224=CARTESIAN_POINT('Ctrl Pts',(-17.3295529098618,18.6573530024033,
12.));
#204225=CARTESIAN_POINT('Ctrl Pts',(-17.3041204135074,18.6483405141865,
0.));
#204226=CARTESIAN_POINT('Ctrl Pts',(-17.3041204135074,18.6483405141865,
12.));
#204227=CARTESIAN_POINT('Ctrl Pts',(-17.2787779120213,18.6392945554748,
0.));
#204228=CARTESIAN_POINT('Ctrl Pts',(-17.2787779120213,18.6392945554748,
12.));
#204229=CARTESIAN_POINT('Ctrl Pts',(-17.2535257482187,18.6302155097943,
0.));
#204230=CARTESIAN_POINT('Ctrl Pts',(-17.2535257482187,18.6302155097943,
12.));
#204231=CARTESIAN_POINT('Ctrl Pts',(-17.2283642650518,18.6211037624038,
0.));
#204232=CARTESIAN_POINT('Ctrl Pts',(-17.2283642650518,18.6211037624038,
12.));
#204233=CARTESIAN_POINT('Ctrl Pts',(-17.2032938019284,18.6119596959949,
0.));
#204234=CARTESIAN_POINT('Ctrl Pts',(-17.2032938019284,18.6119596959949,
12.));
#204235=CARTESIAN_POINT('Ctrl Pts',(-17.1783146940127,18.6027836898817,
0.));
#204236=CARTESIAN_POINT('Ctrl Pts',(-17.1783146940127,18.6027836898817,
12.));
#204237=CARTESIAN_POINT('Ctrl Pts',(-17.1534272741643,18.5935761222825,
0.));
#204238=CARTESIAN_POINT('Ctrl Pts',(-17.1534272741643,18.5935761222825,
12.));
#204239=CARTESIAN_POINT('Ctrl Pts',(-17.1286318741183,18.5843373717247,
0.));
#204240=CARTESIAN_POINT('Ctrl Pts',(-17.1286318741183,18.5843373717247,
12.));
#204241=CARTESIAN_POINT('Ctrl Pts',(-17.1039288260001,18.5750678188542,
0.));
#204242=CARTESIAN_POINT('Ctrl Pts',(-17.1039288260001,18.5750678188542,
12.));
#204243=CARTESIAN_POINT('Ctrl Pts',(-17.0793184636079,18.5657678479789,
0.));
#204244=CARTESIAN_POINT('Ctrl Pts',(-17.0793184636079,18.5657678479789,
12.));
#204245=CARTESIAN_POINT('Ctrl Pts',(-17.0548011239751,18.556437848963,0.));
#204246=CARTESIAN_POINT('Ctrl Pts',(-17.0548011239751,18.556437848963,12.));
#204247=CARTESIAN_POINT('Ctrl Pts',(-17.0303771481738,18.547078218209,0.));
#204248=CARTESIAN_POINT('Ctrl Pts',(-17.0303771481738,18.547078218209,12.));
#204249=CARTESIAN_POINT('Ctrl Pts',(-17.0060468805097,18.5376893576961,
0.));
#204250=CARTESIAN_POINT('Ctrl Pts',(-17.0060468805097,18.5376893576961,
12.));
#204251=CARTESIAN_POINT('Ctrl Pts',(-16.981810668038,18.5282716744197,0.));
#204252=CARTESIAN_POINT('Ctrl Pts',(-16.981810668038,18.5282716744197,12.));
#204253=CARTESIAN_POINT('Ctrl Pts',(-16.9576688599339,18.5188255796659,
0.));
#204254=CARTESIAN_POINT('Ctrl Pts',(-16.9576688599339,18.5188255796659,
12.));
#204255=CARTESIAN_POINT('Ctrl Pts',(-16.9336218069353,18.5093514883835,
0.));
#204256=CARTESIAN_POINT('Ctrl Pts',(-16.9336218069353,18.5093514883835,
12.));
#204257=CARTESIAN_POINT('Ctrl Pts',(-16.9096698606943,18.499849818462,0.));
#204258=CARTESIAN_POINT('Ctrl Pts',(-16.9096698606943,18.499849818462,12.));
#204259=CARTESIAN_POINT('Ctrl Pts',(-16.8858133733088,18.4903209902227,
0.));
#204260=CARTESIAN_POINT('Ctrl Pts',(-16.8858133733088,18.4903209902227,
12.));
#204261=CARTESIAN_POINT('Ctrl Pts',(-16.8620526977171,18.480765426877,0.));
#204262=CARTESIAN_POINT('Ctrl Pts',(-16.8620526977171,18.480765426877,12.));
#204263=CARTESIAN_POINT('Ctrl Pts',(-16.8383881879709,18.4711835548623,
0.));
#204264=CARTESIAN_POINT('Ctrl Pts',(-16.8383881879709,18.4711835548623,
12.));
#204265=CARTESIAN_POINT('Ctrl Pts',(-16.8148201995472,18.4615758042305,
0.));
#204266=CARTESIAN_POINT('Ctrl Pts',(-16.8148201995472,18.4615758042305,
12.));
#204267=CARTESIAN_POINT('Ctrl Pts',(-16.791349089629,18.4519426090123,0.));
#204268=CARTESIAN_POINT('Ctrl Pts',(-16.791349089629,18.4519426090123,12.));
#204269=CARTESIAN_POINT('Ctrl Pts',(-16.7679752173992,18.44228440761,0.));
#204270=CARTESIAN_POINT('Ctrl Pts',(-16.7679752173992,18.44228440761,12.));
#204271=CARTESIAN_POINT('Ctrl Pts',(-16.7446989442882,18.4326016431392,
0.));
#204272=CARTESIAN_POINT('Ctrl Pts',(-16.7446989442882,18.4326016431392,
12.));
#204273=CARTESIAN_POINT('Ctrl Pts',(-16.7215206338818,18.4228947633187,
0.));
#204274=CARTESIAN_POINT('Ctrl Pts',(-16.7215206338818,18.4228947633187,
12.));
#204275=CARTESIAN_POINT('Ctrl Pts',(-16.6984406518491,18.413164220399,0.));
#204276=CARTESIAN_POINT('Ctrl Pts',(-16.6984406518491,18.413164220399,12.));
#204277=CARTESIAN_POINT('Ctrl Pts',(-16.6754593658513,18.403410471079,0.));
#204278=CARTESIAN_POINT('Ctrl Pts',(-16.6754593658513,18.403410471079,12.));
#204279=CARTESIAN_POINT('Ctrl Pts',(-16.6525771454513,18.3936339764332,
0.));
#204280=CARTESIAN_POINT('Ctrl Pts',(-16.6525771454513,18.3936339764332,
12.));
#204281=CARTESIAN_POINT('Ctrl Pts',(-16.6297943620056,18.3838352018327,
0.));
#204282=CARTESIAN_POINT('Ctrl Pts',(-16.6297943620056,18.3838352018327,
12.));
#204283=CARTESIAN_POINT('Ctrl Pts',(-16.607111388571,18.3740146168879,0.));
#204284=CARTESIAN_POINT('Ctrl Pts',(-16.607111388571,18.3740146168879,12.));
#204285=CARTESIAN_POINT('Ctrl Pts',(-16.5845286000217,18.3641726955889,
0.));
#204286=CARTESIAN_POINT('Ctrl Pts',(-16.5845286000217,18.3641726955889,
12.));
#204287=CARTESIAN_POINT('Ctrl Pts',(-16.5620463731413,18.354309916433,0.));
#204288=CARTESIAN_POINT('Ctrl Pts',(-16.5620463731413,18.354309916433,12.));
#204289=CARTESIAN_POINT('Ctrl Pts',(-16.5396650867139,18.34442676256,0.));
#204290=CARTESIAN_POINT('Ctrl Pts',(-16.5396650867139,18.34442676256,12.));
#204291=CARTESIAN_POINT('Ctrl Pts',(-16.5173851216045,18.3345237218864,
0.));
#204292=CARTESIAN_POINT('Ctrl Pts',(-16.5173851216045,18.3345237218864,
12.));
#204293=CARTESIAN_POINT('Ctrl Pts',(-16.4952068608345,18.3246012872469,
0.));
#204294=CARTESIAN_POINT('Ctrl Pts',(-16.4952068608345,18.3246012872469,
12.));
#204295=CARTESIAN_POINT('Ctrl Pts',(-16.4731306896441,18.3146599565231,
0.));
#204296=CARTESIAN_POINT('Ctrl Pts',(-16.4731306896441,18.3146599565231,
12.));
#204297=CARTESIAN_POINT('Ctrl Pts',(-16.4511569955233,18.304700232686,0.));
#204298=CARTESIAN_POINT('Ctrl Pts',(-16.4511569955233,18.304700232686,12.));
#204299=CARTESIAN_POINT('Ctrl Pts',(-16.4292861682379,18.294722623851,0.));
#204300=CARTESIAN_POINT('Ctrl Pts',(-16.4292861682379,18.294722623851,12.));
#204301=CARTESIAN_POINT('Ctrl Pts',(-16.4075185998455,18.2847276433309,
0.));
#204302=CARTESIAN_POINT('Ctrl Pts',(-16.4075185998455,18.2847276433309,
12.));
#204303=CARTESIAN_POINT('Ctrl Pts',(-16.385854684708,18.2747158096934,0.));
#204304=CARTESIAN_POINT('Ctrl Pts',(-16.385854684708,18.2747158096934,12.));
#204305=CARTESIAN_POINT('Ctrl Pts',(-16.3642948194868,18.2646876468169,
0.));
#204306=CARTESIAN_POINT('Ctrl Pts',(-16.3642948194868,18.2646876468169,
12.));
#204307=CARTESIAN_POINT('Ctrl Pts',(-16.3428394031589,18.2546436839608,
0.));
#204308=CARTESIAN_POINT('Ctrl Pts',(-16.3428394031589,18.2546436839608,
12.));
#204309=CARTESIAN_POINT('Ctrl Pts',(-16.3214888370987,18.2445844558741,
0.));
#204310=CARTESIAN_POINT('Ctrl Pts',(-16.3214888370987,18.2445844558741,
12.));
#204311=CARTESIAN_POINT('Ctrl Pts',(-16.3002435251378,18.2345105028982,
0.));
#204312=CARTESIAN_POINT('Ctrl Pts',(-16.3002435251378,18.2345105028982,
12.));
#204313=CARTESIAN_POINT('Ctrl Pts',(-16.2791038736223,18.2244223710745,
0.));
#204314=CARTESIAN_POINT('Ctrl Pts',(-16.2791038736223,18.2244223710745,
12.));
#204315=CARTESIAN_POINT('Ctrl Pts',(-16.2580702914615,18.2143206122529,
0.));
#204316=CARTESIAN_POINT('Ctrl Pts',(-16.2580702914615,18.2143206122529,
12.));
#204317=CARTESIAN_POINT('Ctrl Pts',(-16.2371431901638,18.2042057842035,
0.));
#204318=CARTESIAN_POINT('Ctrl Pts',(-16.2371431901638,18.2042057842035,
12.));
#204319=CARTESIAN_POINT('Ctrl Pts',(-16.2163229838875,18.1940784507229,
0.));
#204320=CARTESIAN_POINT('Ctrl Pts',(-16.2163229838875,18.1940784507229,
12.));
#204321=CARTESIAN_POINT('Ctrl Pts',(-16.1956100895073,18.1839391817331,
0.));
#204322=CARTESIAN_POINT('Ctrl Pts',(-16.1956100895073,18.1839391817331,
12.));
#204323=CARTESIAN_POINT('Ctrl Pts',(-16.1750049266671,18.1737885533849,
0.));
#204324=CARTESIAN_POINT('Ctrl Pts',(-16.1750049266671,18.1737885533849,
12.));
#204325=CARTESIAN_POINT('Ctrl Pts',(-16.154507917826,18.1636271481615,0.));
#204326=CARTESIAN_POINT('Ctrl Pts',(-16.154507917826,18.1636271481615,12.));
#204327=CARTESIAN_POINT('Ctrl Pts',(-16.1341194882988,18.1534555549852,
0.));
#204328=CARTESIAN_POINT('Ctrl Pts',(-16.1341194882988,18.1534555549852,
12.));
#204329=CARTESIAN_POINT('Ctrl Pts',(-16.1138400662794,18.1432743693235,
0.));
#204330=CARTESIAN_POINT('Ctrl Pts',(-16.1138400662794,18.1432743693235,
12.));
#204331=CARTESIAN_POINT('Ctrl Pts',(-16.0936700829112,18.1330841933105,
0.));
#204332=CARTESIAN_POINT('Ctrl Pts',(-16.0936700829112,18.1330841933105,
12.));
#204333=CARTESIAN_POINT('Ctrl Pts',(-16.0736099723668,18.1228856358751,
0.));
#204334=CARTESIAN_POINT('Ctrl Pts',(-16.0736099723668,18.1228856358751,
12.));
#204335=CARTESIAN_POINT('Ctrl Pts',(-16.0536601719126,18.112679312869,0.));
#204336=CARTESIAN_POINT('Ctrl Pts',(-16.0536601719126,18.112679312869,12.));
#204337=CARTESIAN_POINT('Ctrl Pts',(-16.0338211219693,18.1024658471966,
0.));
#204338=CARTESIAN_POINT('Ctrl Pts',(-16.0338211219693,18.1024658471966,
12.));
#204339=CARTESIAN_POINT('Ctrl Pts',(-16.014093266161,18.0922458689462,0.));
#204340=CARTESIAN_POINT('Ctrl Pts',(-16.014093266161,18.0922458689462,12.));
#204341=CARTESIAN_POINT('Ctrl Pts',(-15.9944770513613,18.0820200155236,
0.));
#204342=CARTESIAN_POINT('Ctrl Pts',(-15.9944770513613,18.0820200155236,
12.));
#204343=CARTESIAN_POINT('Ctrl Pts',(-15.9749729277846,18.0717889317958,
0.));
#204344=CARTESIAN_POINT('Ctrl Pts',(-15.9749729277846,18.0717889317958,
12.));
#204345=CARTESIAN_POINT('Ctrl Pts',(-15.9555813490644,18.0615532702359,
0.));
#204346=CARTESIAN_POINT('Ctrl Pts',(-15.9555813490644,18.0615532702359,
12.));
#204347=CARTESIAN_POINT('Ctrl Pts',(-15.9363027723244,18.0513136910691,
0.));
#204348=CARTESIAN_POINT('Ctrl Pts',(-15.9363027723244,18.0513136910691,
12.));
#204349=CARTESIAN_POINT('Ctrl Pts',(-15.9171376582436,18.0410708624208,
0.));
#204350=CARTESIAN_POINT('Ctrl Pts',(-15.9171376582436,18.0410708624208,
12.));
#204351=CARTESIAN_POINT('Ctrl Pts',(-15.8980864711042,18.0308254604636,
0.));
#204352=CARTESIAN_POINT('Ctrl Pts',(-15.8980864711042,18.0308254604636,
12.));
#204353=CARTESIAN_POINT('Ctrl Pts',(-15.8791496788683,18.0205781695769,
0.));
#204354=CARTESIAN_POINT('Ctrl Pts',(-15.8791496788683,18.0205781695769,
12.));
#204355=CARTESIAN_POINT('Ctrl Pts',(-15.8603277532831,18.0103296825205,
0.));
#204356=CARTESIAN_POINT('Ctrl Pts',(-15.8603277532831,18.0103296825205,
12.));
#204357=CARTESIAN_POINT('Ctrl Pts',(-15.8416211699679,18.0000807006052,
0.));
#204358=CARTESIAN_POINT('Ctrl Pts',(-15.8416211699679,18.0000807006052,
12.));
#204359=CARTESIAN_POINT('Ctrl Pts',(-15.8230304084962,17.9898319338664,
0.));
#204360=CARTESIAN_POINT('Ctrl Pts',(-15.8230304084962,17.9898319338664,
12.));
#204361=CARTESIAN_POINT('Ctrl Pts',(-15.8045559524676,17.9795841012386,
0.));
#204362=CARTESIAN_POINT('Ctrl Pts',(-15.8045559524676,17.9795841012386,
12.));
#204363=CARTESIAN_POINT('Ctrl Pts',(-15.7861982895724,17.9693379307303,
0.));
#204364=CARTESIAN_POINT('Ctrl Pts',(-15.7861982895724,17.9693379307303,
12.));
#204365=CARTESIAN_POINT('Ctrl Pts',(-15.7679579117077,17.9590941596242,
0.));
#204366=CARTESIAN_POINT('Ctrl Pts',(-15.7679579117077,17.9590941596242,
12.));
#204367=CARTESIAN_POINT('Ctrl Pts',(-15.749835315086,17.9488535346781,0.));
#204368=CARTESIAN_POINT('Ctrl Pts',(-15.749835315086,17.9488535346781,12.));
#204369=CARTESIAN_POINT('Ctrl Pts',(-15.7318310003335,17.9386168123262,
0.));
#204370=CARTESIAN_POINT('Ctrl Pts',(-15.7318310003335,17.9386168123262,
12.));
#204371=CARTESIAN_POINT('Ctrl Pts',(-15.7139454725838,17.9283847588835,
0.));
#204372=CARTESIAN_POINT('Ctrl Pts',(-15.7139454725838,17.9283847588835,
12.));
#204373=CARTESIAN_POINT('Ctrl Pts',(-15.6961792415522,17.9181581507455,
0.));
#204374=CARTESIAN_POINT('Ctrl Pts',(-15.6961792415522,17.9181581507455,
12.));
#204375=CARTESIAN_POINT('Ctrl Pts',(-15.678532821646,17.9079377746111,0.));
#204376=CARTESIAN_POINT('Ctrl Pts',(-15.678532821646,17.9079377746111,12.));
#204377=CARTESIAN_POINT('Ctrl Pts',(-15.661006732103,17.897724427724,0.));
#204378=CARTESIAN_POINT('Ctrl Pts',(-15.661006732103,17.897724427724,12.));
#204379=CARTESIAN_POINT('Ctrl Pts',(-15.6436014971084,17.8875189181091,
0.));
#204380=CARTESIAN_POINT('Ctrl Pts',(-15.6436014971084,17.8875189181091,
12.));
#204381=CARTESIAN_POINT('Ctrl Pts',(-15.6263176459108,17.8773220648125,
0.));
#204382=CARTESIAN_POINT('Ctrl Pts',(-15.6263176459108,17.8773220648125,
12.));
#204383=CARTESIAN_POINT('Ctrl Pts',(-15.609155712921,17.8671346981394,0.));
#204384=CARTESIAN_POINT('Ctrl Pts',(-15.609155712921,17.8671346981394,12.));
#204385=CARTESIAN_POINT('Ctrl Pts',(-15.5921162378192,17.8569576599006,
0.));
#204386=CARTESIAN_POINT('Ctrl Pts',(-15.5921162378192,17.8569576599006,
12.));
#204387=CARTESIAN_POINT('Ctrl Pts',(-15.5751997657163,17.8467918036987,
0.));
#204388=CARTESIAN_POINT('Ctrl Pts',(-15.5751997657163,17.8467918036987,
12.));
#204389=CARTESIAN_POINT('Ctrl Pts',(-15.5584068472982,17.8366379952085,
0.));
#204390=CARTESIAN_POINT('Ctrl Pts',(-15.5584068472982,17.8366379952085,
12.));
#204391=CARTESIAN_POINT('Ctrl Pts',(-15.541738038964,17.8264971124606,0.));
#204392=CARTESIAN_POINT('Ctrl Pts',(-15.541738038964,17.8264971124606,12.));
#204393=CARTESIAN_POINT('Ctrl Pts',(-15.5251939029552,17.8163700461256,
0.));
#204394=CARTESIAN_POINT('Ctrl Pts',(-15.5251939029552,17.8163700461256,
12.));
#204395=CARTESIAN_POINT('Ctrl Pts',(-15.5087750074718,17.8062576997952,
0.));
#204396=CARTESIAN_POINT('Ctrl Pts',(-15.5087750074718,17.8062576997952,
12.));
#204397=CARTESIAN_POINT('Ctrl Pts',(-15.4924819268517,17.7961609903148,
0.));
#204398=CARTESIAN_POINT('Ctrl Pts',(-15.4924819268517,17.7961609903148,
12.));
#204399=CARTESIAN_POINT('Ctrl Pts',(-15.4763152417497,17.7860808481219,
0.));
#204400=CARTESIAN_POINT('Ctrl Pts',(-15.4763152417497,17.7860808481219,
12.));
#204401=CARTESIAN_POINT('Ctrl Pts',(-15.4602755393017,17.7760182175815,
0.));
#204402=CARTESIAN_POINT('Ctrl Pts',(-15.4602755393017,17.7760182175815,
12.));
#204403=CARTESIAN_POINT('Ctrl Pts',(-15.4443634132869,17.7659740573265,
0.));
#204404=CARTESIAN_POINT('Ctrl Pts',(-15.4443634132869,17.7659740573265,
12.));
#204405=CARTESIAN_POINT('Ctrl Pts',(-15.4285794642668,17.7559493405881,
0.));
#204406=CARTESIAN_POINT('Ctrl Pts',(-15.4285794642668,17.7559493405881,
12.));
#204407=CARTESIAN_POINT('Ctrl Pts',(-15.4129242997837,17.7459450555812,
0.));
#204408=CARTESIAN_POINT('Ctrl Pts',(-15.4129242997837,17.7459450555812,
12.));
#204409=CARTESIAN_POINT('Ctrl Pts',(-15.3973985345802,17.7359622059149,
0.));
#204410=CARTESIAN_POINT('Ctrl Pts',(-15.3973985345802,17.7359622059149,
12.));
#204411=CARTESIAN_POINT('Ctrl Pts',(-15.3820027907967,17.7260018109924,
0.));
#204412=CARTESIAN_POINT('Ctrl Pts',(-15.3820027907967,17.7260018109924,
12.));
#204413=CARTESIAN_POINT('Ctrl Pts',(-15.3667376981699,17.7160649064206,
0.));
#204414=CARTESIAN_POINT('Ctrl Pts',(-15.3667376981699,17.7160649064206,
12.));
#204415=CARTESIAN_POINT('Ctrl Pts',(-15.351603894206,17.7061525444042,0.));
#204416=CARTESIAN_POINT('Ctrl Pts',(-15.351603894206,17.7061525444042,12.));
#204417=CARTESIAN_POINT('Ctrl Pts',(-15.3366020244066,17.6962657941983,
0.));
#204418=CARTESIAN_POINT('Ctrl Pts',(-15.3366020244066,17.6962657941983,
12.));
#204419=CARTESIAN_POINT('Ctrl Pts',(-15.3217327425338,17.6864057426052,
0.));
#204420=CARTESIAN_POINT('Ctrl Pts',(-15.3217327425338,17.6864057426052,
12.));
#204421=CARTESIAN_POINT('Ctrl Pts',(-15.3069967108501,17.676573494456,0.));
#204422=CARTESIAN_POINT('Ctrl Pts',(-15.3069967108501,17.676573494456,12.));
#204423=CARTESIAN_POINT('Ctrl Pts',(-15.2923946003598,17.6667701731041,
0.));
#204424=CARTESIAN_POINT('Ctrl Pts',(-15.2923946003598,17.6667701731041,
12.));
#204425=CARTESIAN_POINT('Ctrl Pts',(-15.2779270910239,17.6569969209,0.));
#204426=CARTESIAN_POINT('Ctrl Pts',(-15.2779270910239,17.6569969209,12.));
#204427=CARTESIAN_POINT('Ctrl Pts',(-15.2635948720292,17.6472548997328,
0.));
#204428=CARTESIAN_POINT('Ctrl Pts',(-15.2635948720292,17.6472548997328,
12.));
#204429=CARTESIAN_POINT('Ctrl Pts',(-15.2493986421092,17.6375452916369,
0.));
#204430=CARTESIAN_POINT('Ctrl Pts',(-15.2493986421092,17.6375452916369,
12.));
#204431=CARTESIAN_POINT('Ctrl Pts',(-15.2353391098366,17.6278692993764,
0.));
#204432=CARTESIAN_POINT('Ctrl Pts',(-15.2353391098366,17.6278692993764,
12.));
#204433=CARTESIAN_POINT('Ctrl Pts',(-15.2214169939199,17.6182281470468,
0.));
#204434=CARTESIAN_POINT('Ctrl Pts',(-15.2214169939199,17.6182281470468,
12.));
#204435=CARTESIAN_POINT('Ctrl Pts',(-15.2076330234686,17.60862308065,0.));
#204436=CARTESIAN_POINT('Ctrl Pts',(-15.2076330234686,17.60862308065,12.));
#204437=CARTESIAN_POINT('Ctrl Pts',(-15.1939879383268,17.5990553687599,
0.));
#204438=CARTESIAN_POINT('Ctrl Pts',(-15.1939879383268,17.5990553687599,
12.));
#204439=CARTESIAN_POINT('Ctrl Pts',(-15.1804824894605,17.5895263032595,
0.));
#204440=CARTESIAN_POINT('Ctrl Pts',(-15.1804824894605,17.5895263032595,
12.));
#204441=CARTESIAN_POINT('Ctrl Pts',(-15.1671174393137,17.580037200054,0.));
#204442=CARTESIAN_POINT('Ctrl Pts',(-15.1671174393137,17.580037200054,12.));
#204443=CARTESIAN_POINT('Ctrl Pts',(-15.1538935621714,17.5705893998029,
0.));
#204444=CARTESIAN_POINT('Ctrl Pts',(-15.1538935621714,17.5705893998029,
12.));
#204445=CARTESIAN_POINT('Ctrl Pts',(-15.1408116444876,17.5611842686192,
0.));
#204446=CARTESIAN_POINT('Ctrl Pts',(-15.1408116444876,17.5611842686192,
12.));
#204447=CARTESIAN_POINT('Ctrl Pts',(-15.1278724853138,17.5518231989117,
0.));
#204448=CARTESIAN_POINT('Ctrl Pts',(-15.1278724853138,17.5518231989117,
12.));
#204449=CARTESIAN_POINT('Ctrl Pts',(-15.1150768967728,17.5425076102963,
0.));
#204450=CARTESIAN_POINT('Ctrl Pts',(-15.1150768967728,17.5425076102963,
12.));
#204451=CARTESIAN_POINT('Ctrl Pts',(-15.1024257045033,17.5332389504829,
0.));
#204452=CARTESIAN_POINT('Ctrl Pts',(-15.1024257045033,17.5332389504829,
12.));
#204453=CARTESIAN_POINT('Ctrl Pts',(-15.0899197481082,17.524018696179,0.));
#204454=CARTESIAN_POINT('Ctrl Pts',(-15.0899197481082,17.524018696179,12.));
#204455=CARTESIAN_POINT('Ctrl Pts',(-15.0775598815749,17.5148483539687,
0.));
#204456=CARTESIAN_POINT('Ctrl Pts',(-15.0775598815749,17.5148483539687,
12.));
#204457=CARTESIAN_POINT('Ctrl Pts',(-15.0653469738307,17.5057294613877,
0.));
#204458=CARTESIAN_POINT('Ctrl Pts',(-15.0653469738307,17.5057294613877,
12.));
#204459=CARTESIAN_POINT('Ctrl Pts',(-15.0532819093085,17.4966635880246,
0.));
#204460=CARTESIAN_POINT('Ctrl Pts',(-15.0532819093085,17.4966635880246,
12.));
#204461=CARTESIAN_POINT('Ctrl Pts',(-15.0413655884993,17.4876523366178,
0.));
#204462=CARTESIAN_POINT('Ctrl Pts',(-15.0413655884993,17.4876523366178,
12.));
#204463=CARTESIAN_POINT('Ctrl Pts',(-15.029598928488,17.4786973441417,0.));
#204464=CARTESIAN_POINT('Ctrl Pts',(-15.029598928488,17.4786973441417,12.));
#204465=CARTESIAN_POINT('Ctrl Pts',(-15.0179828635087,17.4698002829357,
0.));
#204466=CARTESIAN_POINT('Ctrl Pts',(-15.0179828635087,17.4698002829357,
12.));
#204467=CARTESIAN_POINT('Ctrl Pts',(-15.0065183456922,17.4609628621419,
0.));
#204468=CARTESIAN_POINT('Ctrl Pts',(-15.0065183456922,17.4609628621419,
12.));
#204469=CARTESIAN_POINT('Ctrl Pts',(-14.9952063457779,17.4521868291005,
0.));
#204470=CARTESIAN_POINT('Ctrl Pts',(-14.9952063457779,17.4521868291005,
12.));
#204471=CARTESIAN_POINT('Ctrl Pts',(-14.9840478538357,17.4434739707773,
0.));
#204472=CARTESIAN_POINT('Ctrl Pts',(-14.9840478538357,17.4434739707773,
12.));
#204473=CARTESIAN_POINT('Ctrl Pts',(-14.973043879945,17.4348261151395,0.));
#204474=CARTESIAN_POINT('Ctrl Pts',(-14.973043879945,17.4348261151395,12.));
#204475=CARTESIAN_POINT('Ctrl Pts',(-14.9621954549825,17.4262451327088,
0.));
#204476=CARTESIAN_POINT('Ctrl Pts',(-14.9621954549825,17.4262451327088,
12.));
#204477=CARTESIAN_POINT('Ctrl Pts',(-14.9515036315142,17.4177329382827,
0.));
#204478=CARTESIAN_POINT('Ctrl Pts',(-14.9515036315142,17.4177329382827,
12.));
#204479=CARTESIAN_POINT('Ctrl Pts',(-14.940969484645,17.4092914926071,0.));
#204480=CARTESIAN_POINT('Ctrl Pts',(-14.940969484645,17.4092914926071,12.));
#204481=CARTESIAN_POINT('Ctrl Pts',(-14.9305941128758,17.400922804075,0.));
#204482=CARTESIAN_POINT('Ctrl Pts',(-14.9305941128758,17.400922804075,12.));
#204483=CARTESIAN_POINT('Ctrl Pts',(-14.9203786389343,17.3926289303987,
0.));
#204484=CARTESIAN_POINT('Ctrl Pts',(-14.9203786389343,17.3926289303987,
12.));
#204485=CARTESIAN_POINT('Ctrl Pts',(-14.9103242110057,17.3844119809823,
0.));
#204486=CARTESIAN_POINT('Ctrl Pts',(-14.9103242110057,17.3844119809823,
12.));
#204487=CARTESIAN_POINT('Ctrl Pts',(-14.9004320039609,17.3762741193075,
0.));
#204488=CARTESIAN_POINT('Ctrl Pts',(-14.9004320039609,17.3762741193075,
12.));
#204489=CARTESIAN_POINT('Ctrl Pts',(-14.8907032205789,17.3682175653236,
0.));
#204490=CARTESIAN_POINT('Ctrl Pts',(-14.8907032205789,17.3682175653236,
12.));
#204491=CARTESIAN_POINT('Ctrl Pts',(-14.8811390927424,17.3602445978163,
0.));
#204492=CARTESIAN_POINT('Ctrl Pts',(-14.8811390927424,17.3602445978163,
12.));
#204493=CARTESIAN_POINT('Ctrl Pts',(-14.8717408826958,17.3523575568648,
0.));
#204494=CARTESIAN_POINT('Ctrl Pts',(-14.8717408826958,17.3523575568648,
12.));
#204495=CARTESIAN_POINT('Ctrl Pts',(-14.8625098843419,17.3445588463477,
0.));
#204496=CARTESIAN_POINT('Ctrl Pts',(-14.8625098843419,17.3445588463477,
12.));
#204497=CARTESIAN_POINT('Ctrl Pts',(-14.8534474245433,17.336850936485,0.));
#204498=CARTESIAN_POINT('Ctrl Pts',(-14.8534474245433,17.336850936485,12.));
#204499=CARTESIAN_POINT('Ctrl Pts',(-14.8445548643504,17.3292363662601,
0.));
#204500=CARTESIAN_POINT('Ctrl Pts',(-14.8445548643504,17.3292363662601,
12.));
#204501=CARTESIAN_POINT('Ctrl Pts',(-14.8358336004193,17.3217177462096,
0.));
#204502=CARTESIAN_POINT('Ctrl Pts',(-14.8358336004193,17.3217177462096,
12.));
#204503=CARTESIAN_POINT('Ctrl Pts',(-14.8272850675375,17.3142977632656,
0.));
#204504=CARTESIAN_POINT('Ctrl Pts',(-14.8272850675375,17.3142977632656,
12.));
#204505=CARTESIAN_POINT('Ctrl Pts',(-14.8189107410161,17.3069791853705,
0.));
#204506=CARTESIAN_POINT('Ctrl Pts',(-14.8189107410161,17.3069791853705,
12.));
#204507=CARTESIAN_POINT('Ctrl Pts',(-14.8107121391038,17.2997648661483,
0.));
#204508=CARTESIAN_POINT('Ctrl Pts',(-14.8107121391038,17.2997648661483,
12.));
#204509=CARTESIAN_POINT('Ctrl Pts',(-14.8026908254281,17.2926577496519,
0.));
#204510=CARTESIAN_POINT('Ctrl Pts',(-14.8026908254281,17.2926577496519,
12.));
#204511=CARTESIAN_POINT('Ctrl Pts',(-14.7948484105253,17.28566087332,0.));
#204512=CARTESIAN_POINT('Ctrl Pts',(-14.7948484105253,17.28566087332,12.));
#204513=CARTESIAN_POINT('Ctrl Pts',(-14.787186553128,17.278777370485,0.));
#204514=CARTESIAN_POINT('Ctrl Pts',(-14.787186553128,17.278777370485,12.));
#204515=CARTESIAN_POINT('Ctrl Pts',(-14.7797069617802,17.2720104735192,
0.));
#204516=CARTESIAN_POINT('Ctrl Pts',(-14.7797069617802,17.2720104735192,
12.));
#204517=CARTESIAN_POINT('Ctrl Pts',(-14.7724113956728,17.2653635155317,
0.));
#204518=CARTESIAN_POINT('Ctrl Pts',(-14.7724113956728,17.2653635155317,
12.));
#204519=CARTESIAN_POINT('Ctrl Pts',(-14.7653016697589,17.2588399401464,
0.));
#204520=CARTESIAN_POINT('Ctrl Pts',(-14.7653016697589,17.2588399401464,
12.));
#204521=CARTESIAN_POINT('Ctrl Pts',(-14.7583796616617,17.2524433146837,
0.));
#204522=CARTESIAN_POINT('Ctrl Pts',(-14.7583796616617,17.2524433146837,
12.));
#204523=CARTESIAN_POINT('Ctrl Pts',(-14.7516473175125,17.2461773413289,
0.));
#204524=CARTESIAN_POINT('Ctrl Pts',(-14.7516473175125,17.2461773413289,
12.));
#204525=CARTESIAN_POINT('Ctrl Pts',(-14.7451066593793,17.2400458713566,
0.));
#204526=CARTESIAN_POINT('Ctrl Pts',(-14.7451066593793,17.2400458713566,
12.));
#204527=CARTESIAN_POINT('Ctrl Pts',(-14.7387597858117,17.2340529062077,
0.));
#204528=CARTESIAN_POINT('Ctrl Pts',(-14.7387597858117,17.2340529062077,
12.));
#204529=CARTESIAN_POINT('Ctrl Pts',(-14.7326088681163,17.2282025904314,
0.));
#204530=CARTESIAN_POINT('Ctrl Pts',(-14.7326088681163,17.2282025904314,
12.));
#204531=CARTESIAN_POINT('Ctrl Pts',(-14.7266561494282,17.2224992099666,
0.));
#204532=CARTESIAN_POINT('Ctrl Pts',(-14.7266561494282,17.2224992099666,
12.));
#204533=CARTESIAN_POINT('Ctrl Pts',(-14.7209039390326,17.2169471814255,
0.));
#204534=CARTESIAN_POINT('Ctrl Pts',(-14.7209039390326,17.2169471814255,
12.));
#204535=CARTESIAN_POINT('Ctrl Pts',(-14.7153546289338,17.2115510835988,
0.));
#204536=CARTESIAN_POINT('Ctrl Pts',(-14.7153546289338,17.2115510835988,
12.));
#204537=CARTESIAN_POINT('Ctrl Pts',(-14.7100107213586,17.2063157097316,
0.));
#204538=CARTESIAN_POINT('Ctrl Pts',(-14.7100107213586,17.2063157097316,
12.));
#204539=CARTESIAN_POINT('Ctrl Pts',(-14.7048748502663,17.2012461084268,
0.));
#204540=CARTESIAN_POINT('Ctrl Pts',(-14.7048748502663,17.2012461084268,
12.));
#204541=CARTESIAN_POINT('Ctrl Pts',(-14.699949811582,17.1963476411694,0.));
#204542=CARTESIAN_POINT('Ctrl Pts',(-14.699949811582,17.1963476411694,12.));
#204543=CARTESIAN_POINT('Ctrl Pts',(-14.6952385361706,17.1916259308415,
0.));
#204544=CARTESIAN_POINT('Ctrl Pts',(-14.6952385361706,17.1916259308415,
12.));
#204545=CARTESIAN_POINT('Ctrl Pts',(-14.6907440526958,17.1870867909918,
0.));
#204546=CARTESIAN_POINT('Ctrl Pts',(-14.6907440526958,17.1870867909918,
12.));
#204547=CARTESIAN_POINT('Ctrl Pts',(-14.6864694522319,17.182736158472,0.));
#204548=CARTESIAN_POINT('Ctrl Pts',(-14.6864694522319,17.182736158472,12.));
#204549=CARTESIAN_POINT('Ctrl Pts',(-14.6824178576167,17.1785800350827,
0.));
#204550=CARTESIAN_POINT('Ctrl Pts',(-14.6824178576167,17.1785800350827,
12.));
#204551=CARTESIAN_POINT('Ctrl Pts',(-14.6785925615676,17.1746247499057,
0.));
#204552=CARTESIAN_POINT('Ctrl Pts',(-14.6785925615676,17.1746247499057,
12.));
#204553=CARTESIAN_POINT('Ctrl Pts',(-14.6749971333867,17.1708771619129,
0.));
#204554=CARTESIAN_POINT('Ctrl Pts',(-14.6749971333867,17.1708771619129,
12.));
#204555=CARTESIAN_POINT('Ctrl Pts',(-14.6716355833321,17.1673449723019,
0.));
#204556=CARTESIAN_POINT('Ctrl Pts',(-14.6716355833321,17.1673449723019,
12.));
#204557=CARTESIAN_POINT('Ctrl Pts',(-14.6685123374424,17.1640366762304,
0.));
#204558=CARTESIAN_POINT('Ctrl Pts',(-14.6685123374424,17.1640366762304,
12.));
#204559=CARTESIAN_POINT('Ctrl Pts',(-14.6656319165057,17.1609609517369,
0.));
#204560=CARTESIAN_POINT('Ctrl Pts',(-14.6656319165057,17.1609609517369,
12.));
#204561=CARTESIAN_POINT('Ctrl Pts',(-14.662998728599,17.1581262646789,0.));
#204562=CARTESIAN_POINT('Ctrl Pts',(-14.662998728599,17.1581262646789,12.));
#204563=CARTESIAN_POINT('Ctrl Pts',(-14.660616716964,17.1555401986403,0.));
#204564=CARTESIAN_POINT('Ctrl Pts',(-14.660616716964,17.1555401986403,12.));
#204565=CARTESIAN_POINT('Ctrl Pts',(-14.6584900555301,17.1532107762719,
0.));
#204566=CARTESIAN_POINT('Ctrl Pts',(-14.6584900555301,17.1532107762719,
12.));
#204567=CARTESIAN_POINT('Ctrl Pts',(-14.6566237952435,17.1511476869495,
0.));
#204568=CARTESIAN_POINT('Ctrl Pts',(-14.6566237952435,17.1511476869495,
12.));
#204569=CARTESIAN_POINT('Ctrl Pts',(-14.6550248622813,17.1493641837556,
0.));
#204570=CARTESIAN_POINT('Ctrl Pts',(-14.6550248622813,17.1493641837556,
12.));
#204571=CARTESIAN_POINT('Ctrl Pts',(-14.6537016966188,17.1478763944909,
0.));
#204572=CARTESIAN_POINT('Ctrl Pts',(-14.6537016966188,17.1478763944909,
12.));
#204573=CARTESIAN_POINT('Ctrl Pts',(-14.6526624064978,17.1466998098673,
0.));
#204574=CARTESIAN_POINT('Ctrl Pts',(-14.6526624064978,17.1466998098673,
12.));
#204575=CARTESIAN_POINT('Ctrl Pts',(-14.65191316345,17.1458462295273,0.));
#204576=CARTESIAN_POINT('Ctrl Pts',(-14.65191316345,17.1458462295273,12.));
#204577=CARTESIAN_POINT('Ctrl Pts',(-14.6515481598057,17.1454262858045,
0.));
#204578=CARTESIAN_POINT('Ctrl Pts',(-14.6515481598057,17.1454262858045,
12.));
#204579=CARTESIAN_POINT('Ctrl Pts',(-14.6514066997188,17.1452600887039,
0.));
#204580=CARTESIAN_POINT('Ctrl Pts',(-14.6514066997188,17.1452600887039,
12.));
#204581=CARTESIAN_POINT('Ctrl Pts',(-14.651371185284,17.1452153999142,0.));
#204582=CARTESIAN_POINT('Ctrl Pts',(-14.651371185284,17.1452153999142,12.));
#204583=CARTESIAN_POINT('Ctrl Pts',(-14.6513681262571,17.1452095830633,
0.));
#204584=CARTESIAN_POINT('Ctrl Pts',(-14.6513681262571,17.1452095830633,
12.));
#204585=CARTESIAN_POINT('',(-17.9112098770111,18.8464468996588,0.));
#204586=CARTESIAN_POINT('Ctrl Pts',(-17.9112098770111,18.8464468996588,
0.));
#204587=CARTESIAN_POINT('Ctrl Pts',(-17.9057348246595,18.8448126709691,
0.));
#204588=CARTESIAN_POINT('Ctrl Pts',(-17.8947931177807,18.8415402351786,
0.));
#204589=CARTESIAN_POINT('Ctrl Pts',(-17.8784057509356,18.8366196462581,
0.));
#204590=CARTESIAN_POINT('Ctrl Pts',(-17.8566063174771,18.8300349895974,
0.));
#204591=CARTESIAN_POINT('Ctrl Pts',(-17.8294410311006,18.8217643886157,
0.));
#204592=CARTESIAN_POINT('Ctrl Pts',(-17.8023598011057,18.8134540340417,
0.));
#204593=CARTESIAN_POINT('Ctrl Pts',(-17.7753627137853,18.8051039860448,
0.));
#204594=CARTESIAN_POINT('Ctrl Pts',(-17.7484498996905,18.7967143519419,
0.));
#204595=CARTESIAN_POINT('Ctrl Pts',(-17.7216215409035,18.7882852976049,
0.));
#204596=CARTESIAN_POINT('Ctrl Pts',(-17.6948778823014,18.7798170641374,
0.));
#204597=CARTESIAN_POINT('Ctrl Pts',(-17.6682192274236,18.7713099642754,
0.));
#204598=CARTESIAN_POINT('Ctrl Pts',(-17.6416459210681,18.762764361321,0.));
#204599=CARTESIAN_POINT('Ctrl Pts',(-17.6151583357012,18.7541806530984,
0.));
#204600=CARTESIAN_POINT('Ctrl Pts',(-17.5887568561371,18.7455592536687,
0.));
#204601=CARTESIAN_POINT('Ctrl Pts',(-17.5624418653245,18.7369005764553,
0.));
#204602=CARTESIAN_POINT('Ctrl Pts',(-17.5362137287593,18.7282050157138,
0.));
#204603=CARTESIAN_POINT('Ctrl Pts',(-17.5100727820876,18.7194729318098,
0.));
#204604=CARTESIAN_POINT('Ctrl Pts',(-17.4840193397162,18.7107046613912,
0.));
#204605=CARTESIAN_POINT('Ctrl Pts',(-17.4580537012753,18.70190052503,0.));
#204606=CARTESIAN_POINT('Ctrl Pts',(-17.4321761588142,18.6930608357409,
0.));
#204607=CARTESIAN_POINT('Ctrl Pts',(-17.4063870038562,18.6841859073471,
0.));
#204608=CARTESIAN_POINT('Ctrl Pts',(-17.3806865340747,18.6752760624052,
0.));
#204609=CARTESIAN_POINT('Ctrl Pts',(-17.3550750612443,18.6663316416582,
0.));
#204610=CARTESIAN_POINT('Ctrl Pts',(-17.3295529098618,18.6573530024033,
0.));
#204611=CARTESIAN_POINT('Ctrl Pts',(-17.3041204135074,18.6483405141865,
0.));
#204612=CARTESIAN_POINT('Ctrl Pts',(-17.2787779120213,18.6392945554748,
0.));
#204613=CARTESIAN_POINT('Ctrl Pts',(-17.2535257482187,18.6302155097943,
0.));
#204614=CARTESIAN_POINT('Ctrl Pts',(-17.2283642650518,18.6211037624038,
0.));
#204615=CARTESIAN_POINT('Ctrl Pts',(-17.2032938019284,18.6119596959949,
0.));
#204616=CARTESIAN_POINT('Ctrl Pts',(-17.1783146940127,18.6027836898817,
0.));
#204617=CARTESIAN_POINT('Ctrl Pts',(-17.1534272741643,18.5935761222825,
0.));
#204618=CARTESIAN_POINT('Ctrl Pts',(-17.1286318741183,18.5843373717247,
0.));
#204619=CARTESIAN_POINT('Ctrl Pts',(-17.1039288260001,18.5750678188542,
0.));
#204620=CARTESIAN_POINT('Ctrl Pts',(-17.0793184636079,18.5657678479789,
0.));
#204621=CARTESIAN_POINT('Ctrl Pts',(-17.0548011239751,18.556437848963,0.));
#204622=CARTESIAN_POINT('Ctrl Pts',(-17.0303771481738,18.547078218209,0.));
#204623=CARTESIAN_POINT('Ctrl Pts',(-17.0060468805097,18.5376893576961,
0.));
#204624=CARTESIAN_POINT('Ctrl Pts',(-16.981810668038,18.5282716744197,0.));
#204625=CARTESIAN_POINT('Ctrl Pts',(-16.9576688599339,18.5188255796659,
0.));
#204626=CARTESIAN_POINT('Ctrl Pts',(-16.9336218069353,18.5093514883835,
0.));
#204627=CARTESIAN_POINT('Ctrl Pts',(-16.9096698606943,18.499849818462,0.));
#204628=CARTESIAN_POINT('Ctrl Pts',(-16.8858133733088,18.4903209902227,
0.));
#204629=CARTESIAN_POINT('Ctrl Pts',(-16.8620526977171,18.480765426877,0.));
#204630=CARTESIAN_POINT('Ctrl Pts',(-16.8383881879709,18.4711835548623,
0.));
#204631=CARTESIAN_POINT('Ctrl Pts',(-16.8148201995472,18.4615758042305,
0.));
#204632=CARTESIAN_POINT('Ctrl Pts',(-16.791349089629,18.4519426090123,0.));
#204633=CARTESIAN_POINT('Ctrl Pts',(-16.7679752173992,18.44228440761,0.));
#204634=CARTESIAN_POINT('Ctrl Pts',(-16.7446989442882,18.4326016431392,
0.));
#204635=CARTESIAN_POINT('Ctrl Pts',(-16.7215206338818,18.4228947633187,
0.));
#204636=CARTESIAN_POINT('Ctrl Pts',(-16.6984406518491,18.413164220399,0.));
#204637=CARTESIAN_POINT('Ctrl Pts',(-16.6754593658513,18.403410471079,0.));
#204638=CARTESIAN_POINT('Ctrl Pts',(-16.6525771454513,18.3936339764332,
0.));
#204639=CARTESIAN_POINT('Ctrl Pts',(-16.6297943620056,18.3838352018327,
0.));
#204640=CARTESIAN_POINT('Ctrl Pts',(-16.607111388571,18.3740146168879,0.));
#204641=CARTESIAN_POINT('Ctrl Pts',(-16.5845286000217,18.3641726955889,
0.));
#204642=CARTESIAN_POINT('Ctrl Pts',(-16.5620463731413,18.354309916433,0.));
#204643=CARTESIAN_POINT('Ctrl Pts',(-16.5396650867139,18.34442676256,0.));
#204644=CARTESIAN_POINT('Ctrl Pts',(-16.5173851216045,18.3345237218864,
0.));
#204645=CARTESIAN_POINT('Ctrl Pts',(-16.4952068608345,18.3246012872469,
0.));
#204646=CARTESIAN_POINT('Ctrl Pts',(-16.4731306896441,18.3146599565231,
0.));
#204647=CARTESIAN_POINT('Ctrl Pts',(-16.4511569955233,18.304700232686,0.));
#204648=CARTESIAN_POINT('Ctrl Pts',(-16.4292861682379,18.294722623851,0.));
#204649=CARTESIAN_POINT('Ctrl Pts',(-16.4075185998455,18.2847276433309,
0.));
#204650=CARTESIAN_POINT('Ctrl Pts',(-16.385854684708,18.2747158096934,0.));
#204651=CARTESIAN_POINT('Ctrl Pts',(-16.3642948194868,18.2646876468169,
0.));
#204652=CARTESIAN_POINT('Ctrl Pts',(-16.3428394031589,18.2546436839608,
0.));
#204653=CARTESIAN_POINT('Ctrl Pts',(-16.3214888370987,18.2445844558741,
0.));
#204654=CARTESIAN_POINT('Ctrl Pts',(-16.3002435251378,18.2345105028982,
0.));
#204655=CARTESIAN_POINT('Ctrl Pts',(-16.2791038736223,18.2244223710745,
0.));
#204656=CARTESIAN_POINT('Ctrl Pts',(-16.2580702914615,18.2143206122529,
0.));
#204657=CARTESIAN_POINT('Ctrl Pts',(-16.2371431901638,18.2042057842035,
0.));
#204658=CARTESIAN_POINT('Ctrl Pts',(-16.2163229838875,18.1940784507229,
0.));
#204659=CARTESIAN_POINT('Ctrl Pts',(-16.1956100895073,18.1839391817331,
0.));
#204660=CARTESIAN_POINT('Ctrl Pts',(-16.1750049266671,18.1737885533849,
0.));
#204661=CARTESIAN_POINT('Ctrl Pts',(-16.154507917826,18.1636271481615,0.));
#204662=CARTESIAN_POINT('Ctrl Pts',(-16.1341194882988,18.1534555549852,
0.));
#204663=CARTESIAN_POINT('Ctrl Pts',(-16.1138400662794,18.1432743693235,
0.));
#204664=CARTESIAN_POINT('Ctrl Pts',(-16.0936700829112,18.1330841933105,
0.));
#204665=CARTESIAN_POINT('Ctrl Pts',(-16.0736099723668,18.1228856358751,
0.));
#204666=CARTESIAN_POINT('Ctrl Pts',(-16.0536601719126,18.112679312869,0.));
#204667=CARTESIAN_POINT('Ctrl Pts',(-16.0338211219693,18.1024658471966,
0.));
#204668=CARTESIAN_POINT('Ctrl Pts',(-16.014093266161,18.0922458689462,0.));
#204669=CARTESIAN_POINT('Ctrl Pts',(-15.9944770513613,18.0820200155236,
0.));
#204670=CARTESIAN_POINT('Ctrl Pts',(-15.9749729277846,18.0717889317958,
0.));
#204671=CARTESIAN_POINT('Ctrl Pts',(-15.9555813490644,18.0615532702359,
0.));
#204672=CARTESIAN_POINT('Ctrl Pts',(-15.9363027723244,18.0513136910691,
0.));
#204673=CARTESIAN_POINT('Ctrl Pts',(-15.9171376582436,18.0410708624208,
0.));
#204674=CARTESIAN_POINT('Ctrl Pts',(-15.8980864711042,18.0308254604636,
0.));
#204675=CARTESIAN_POINT('Ctrl Pts',(-15.8791496788683,18.0205781695769,
0.));
#204676=CARTESIAN_POINT('Ctrl Pts',(-15.8603277532831,18.0103296825205,
0.));
#204677=CARTESIAN_POINT('Ctrl Pts',(-15.8416211699679,18.0000807006052,
0.));
#204678=CARTESIAN_POINT('Ctrl Pts',(-15.8230304084962,17.9898319338664,
0.));
#204679=CARTESIAN_POINT('Ctrl Pts',(-15.8045559524676,17.9795841012386,
0.));
#204680=CARTESIAN_POINT('Ctrl Pts',(-15.7861982895724,17.9693379307303,
0.));
#204681=CARTESIAN_POINT('Ctrl Pts',(-15.7679579117077,17.9590941596242,
0.));
#204682=CARTESIAN_POINT('Ctrl Pts',(-15.749835315086,17.9488535346781,0.));
#204683=CARTESIAN_POINT('Ctrl Pts',(-15.7318310003335,17.9386168123262,
0.));
#204684=CARTESIAN_POINT('Ctrl Pts',(-15.7139454725838,17.9283847588835,
0.));
#204685=CARTESIAN_POINT('Ctrl Pts',(-15.6961792415522,17.9181581507455,
0.));
#204686=CARTESIAN_POINT('Ctrl Pts',(-15.678532821646,17.9079377746111,0.));
#204687=CARTESIAN_POINT('Ctrl Pts',(-15.661006732103,17.897724427724,0.));
#204688=CARTESIAN_POINT('Ctrl Pts',(-15.6436014971084,17.8875189181091,
0.));
#204689=CARTESIAN_POINT('Ctrl Pts',(-15.6263176459108,17.8773220648125,
0.));
#204690=CARTESIAN_POINT('Ctrl Pts',(-15.609155712921,17.8671346981394,0.));
#204691=CARTESIAN_POINT('Ctrl Pts',(-15.5921162378192,17.8569576599006,
0.));
#204692=CARTESIAN_POINT('Ctrl Pts',(-15.5751997657163,17.8467918036987,
0.));
#204693=CARTESIAN_POINT('Ctrl Pts',(-15.5584068472982,17.8366379952085,
0.));
#204694=CARTESIAN_POINT('Ctrl Pts',(-15.541738038964,17.8264971124606,0.));
#204695=CARTESIAN_POINT('Ctrl Pts',(-15.5251939029552,17.8163700461256,
0.));
#204696=CARTESIAN_POINT('Ctrl Pts',(-15.5087750074718,17.8062576997952,
0.));
#204697=CARTESIAN_POINT('Ctrl Pts',(-15.4924819268517,17.7961609903148,
0.));
#204698=CARTESIAN_POINT('Ctrl Pts',(-15.4763152417497,17.7860808481219,
0.));
#204699=CARTESIAN_POINT('Ctrl Pts',(-15.4602755393017,17.7760182175815,
0.));
#204700=CARTESIAN_POINT('Ctrl Pts',(-15.4443634132869,17.7659740573265,
0.));
#204701=CARTESIAN_POINT('Ctrl Pts',(-15.4285794642668,17.7559493405881,
0.));
#204702=CARTESIAN_POINT('Ctrl Pts',(-15.4129242997837,17.7459450555812,
0.));
#204703=CARTESIAN_POINT('Ctrl Pts',(-15.3973985345802,17.7359622059149,
0.));
#204704=CARTESIAN_POINT('Ctrl Pts',(-15.3820027907967,17.7260018109924,
0.));
#204705=CARTESIAN_POINT('Ctrl Pts',(-15.3667376981699,17.7160649064206,
0.));
#204706=CARTESIAN_POINT('Ctrl Pts',(-15.351603894206,17.7061525444042,0.));
#204707=CARTESIAN_POINT('Ctrl Pts',(-15.3366020244066,17.6962657941983,
0.));
#204708=CARTESIAN_POINT('Ctrl Pts',(-15.3217327425338,17.6864057426052,
0.));
#204709=CARTESIAN_POINT('Ctrl Pts',(-15.3069967108501,17.676573494456,0.));
#204710=CARTESIAN_POINT('Ctrl Pts',(-15.2923946003598,17.6667701731041,
0.));
#204711=CARTESIAN_POINT('Ctrl Pts',(-15.2779270910239,17.6569969209,0.));
#204712=CARTESIAN_POINT('Ctrl Pts',(-15.2635948720292,17.6472548997328,
0.));
#204713=CARTESIAN_POINT('Ctrl Pts',(-15.2493986421092,17.6375452916369,
0.));
#204714=CARTESIAN_POINT('Ctrl Pts',(-15.2353391098366,17.6278692993764,
0.));
#204715=CARTESIAN_POINT('Ctrl Pts',(-15.2214169939199,17.6182281470468,
0.));
#204716=CARTESIAN_POINT('Ctrl Pts',(-15.2076330234686,17.60862308065,0.));
#204717=CARTESIAN_POINT('Ctrl Pts',(-15.1939879383268,17.5990553687599,
0.));
#204718=CARTESIAN_POINT('Ctrl Pts',(-15.1804824894605,17.5895263032595,
0.));
#204719=CARTESIAN_POINT('Ctrl Pts',(-15.1671174393137,17.580037200054,0.));
#204720=CARTESIAN_POINT('Ctrl Pts',(-15.1538935621714,17.5705893998029,
0.));
#204721=CARTESIAN_POINT('Ctrl Pts',(-15.1408116444876,17.5611842686192,
0.));
#204722=CARTESIAN_POINT('Ctrl Pts',(-15.1278724853138,17.5518231989117,
0.));
#204723=CARTESIAN_POINT('Ctrl Pts',(-15.1150768967728,17.5425076102963,
0.));
#204724=CARTESIAN_POINT('Ctrl Pts',(-15.1024257045033,17.5332389504829,
0.));
#204725=CARTESIAN_POINT('Ctrl Pts',(-15.0899197481082,17.524018696179,0.));
#204726=CARTESIAN_POINT('Ctrl Pts',(-15.0775598815749,17.5148483539687,
0.));
#204727=CARTESIAN_POINT('Ctrl Pts',(-15.0653469738307,17.5057294613877,
0.));
#204728=CARTESIAN_POINT('Ctrl Pts',(-15.0532819093085,17.4966635880246,
0.));
#204729=CARTESIAN_POINT('Ctrl Pts',(-15.0413655884993,17.4876523366178,
0.));
#204730=CARTESIAN_POINT('Ctrl Pts',(-15.029598928488,17.4786973441417,0.));
#204731=CARTESIAN_POINT('Ctrl Pts',(-15.0179828635087,17.4698002829357,
0.));
#204732=CARTESIAN_POINT('Ctrl Pts',(-15.0065183456922,17.4609628621419,
0.));
#204733=CARTESIAN_POINT('Ctrl Pts',(-14.9952063457779,17.4521868291005,
0.));
#204734=CARTESIAN_POINT('Ctrl Pts',(-14.9840478538357,17.4434739707773,
0.));
#204735=CARTESIAN_POINT('Ctrl Pts',(-14.973043879945,17.4348261151395,0.));
#204736=CARTESIAN_POINT('Ctrl Pts',(-14.9621954549825,17.4262451327088,
0.));
#204737=CARTESIAN_POINT('Ctrl Pts',(-14.9515036315142,17.4177329382827,
0.));
#204738=CARTESIAN_POINT('Ctrl Pts',(-14.940969484645,17.4092914926071,0.));
#204739=CARTESIAN_POINT('Ctrl Pts',(-14.9305941128758,17.400922804075,0.));
#204740=CARTESIAN_POINT('Ctrl Pts',(-14.9203786389343,17.3926289303987,
0.));
#204741=CARTESIAN_POINT('Ctrl Pts',(-14.9103242110057,17.3844119809823,
0.));
#204742=CARTESIAN_POINT('Ctrl Pts',(-14.9004320039609,17.3762741193075,
0.));
#204743=CARTESIAN_POINT('Ctrl Pts',(-14.8907032205789,17.3682175653236,
0.));
#204744=CARTESIAN_POINT('Ctrl Pts',(-14.8811390927424,17.3602445978163,
0.));
#204745=CARTESIAN_POINT('Ctrl Pts',(-14.8717408826958,17.3523575568648,
0.));
#204746=CARTESIAN_POINT('Ctrl Pts',(-14.8625098843419,17.3445588463477,
0.));
#204747=CARTESIAN_POINT('Ctrl Pts',(-14.8534474245433,17.336850936485,0.));
#204748=CARTESIAN_POINT('Ctrl Pts',(-14.8445548643504,17.3292363662601,
0.));
#204749=CARTESIAN_POINT('Ctrl Pts',(-14.8358336004193,17.3217177462096,
0.));
#204750=CARTESIAN_POINT('Ctrl Pts',(-14.8272850675375,17.3142977632656,
0.));
#204751=CARTESIAN_POINT('Ctrl Pts',(-14.8189107410161,17.3069791853705,
0.));
#204752=CARTESIAN_POINT('Ctrl Pts',(-14.8107121391038,17.2997648661483,
0.));
#204753=CARTESIAN_POINT('Ctrl Pts',(-14.8026908254281,17.2926577496519,
0.));
#204754=CARTESIAN_POINT('Ctrl Pts',(-14.7948484105253,17.28566087332,0.));
#204755=CARTESIAN_POINT('Ctrl Pts',(-14.787186553128,17.278777370485,0.));
#204756=CARTESIAN_POINT('Ctrl Pts',(-14.7797069617802,17.2720104735192,
0.));
#204757=CARTESIAN_POINT('Ctrl Pts',(-14.7724113956728,17.2653635155317,
0.));
#204758=CARTESIAN_POINT('Ctrl Pts',(-14.7653016697589,17.2588399401464,
0.));
#204759=CARTESIAN_POINT('Ctrl Pts',(-14.7583796616617,17.2524433146837,
0.));
#204760=CARTESIAN_POINT('Ctrl Pts',(-14.7516473175125,17.2461773413289,
0.));
#204761=CARTESIAN_POINT('Ctrl Pts',(-14.7451066593793,17.2400458713566,
0.));
#204762=CARTESIAN_POINT('Ctrl Pts',(-14.7387597858117,17.2340529062077,
0.));
#204763=CARTESIAN_POINT('Ctrl Pts',(-14.7326088681163,17.2282025904314,
0.));
#204764=CARTESIAN_POINT('Ctrl Pts',(-14.7266561494282,17.2224992099666,
0.));
#204765=CARTESIAN_POINT('Ctrl Pts',(-14.7209039390326,17.2169471814255,
0.));
#204766=CARTESIAN_POINT('Ctrl Pts',(-14.7153546289338,17.2115510835988,
0.));
#204767=CARTESIAN_POINT('Ctrl Pts',(-14.7100107213586,17.2063157097316,
0.));
#204768=CARTESIAN_POINT('Ctrl Pts',(-14.7048748502663,17.2012461084268,
0.));
#204769=CARTESIAN_POINT('Ctrl Pts',(-14.699949811582,17.1963476411694,0.));
#204770=CARTESIAN_POINT('Ctrl Pts',(-14.6952385361706,17.1916259308415,
0.));
#204771=CARTESIAN_POINT('Ctrl Pts',(-14.6907440526958,17.1870867909918,
0.));
#204772=CARTESIAN_POINT('Ctrl Pts',(-14.6864694522319,17.182736158472,0.));
#204773=CARTESIAN_POINT('Ctrl Pts',(-14.6824178576167,17.1785800350827,
0.));
#204774=CARTESIAN_POINT('Ctrl Pts',(-14.6785925615676,17.1746247499057,
0.));
#204775=CARTESIAN_POINT('Ctrl Pts',(-14.6749971333867,17.1708771619129,
0.));
#204776=CARTESIAN_POINT('Ctrl Pts',(-14.6716355833321,17.1673449723019,
0.));
#204777=CARTESIAN_POINT('Ctrl Pts',(-14.6685123374424,17.1640366762304,
0.));
#204778=CARTESIAN_POINT('Ctrl Pts',(-14.6656319165057,17.1609609517369,
0.));
#204779=CARTESIAN_POINT('Ctrl Pts',(-14.662998728599,17.1581262646789,0.));
#204780=CARTESIAN_POINT('Ctrl Pts',(-14.660616716964,17.1555401986403,0.));
#204781=CARTESIAN_POINT('Ctrl Pts',(-14.6584900555301,17.1532107762719,
0.));
#204782=CARTESIAN_POINT('Ctrl Pts',(-14.6566237952435,17.1511476869495,
0.));
#204783=CARTESIAN_POINT('Ctrl Pts',(-14.6550248622813,17.1493641837556,
0.));
#204784=CARTESIAN_POINT('Ctrl Pts',(-14.6537016966188,17.1478763944909,
0.));
#204785=CARTESIAN_POINT('Ctrl Pts',(-14.6526624064978,17.1466998098673,
0.));
#204786=CARTESIAN_POINT('Ctrl Pts',(-14.65191316345,17.1458462295273,0.));
#204787=CARTESIAN_POINT('Ctrl Pts',(-14.6515481598057,17.1454262858045,
0.));
#204788=CARTESIAN_POINT('Ctrl Pts',(-14.6514066997188,17.1452600887039,
0.));
#204789=CARTESIAN_POINT('Ctrl Pts',(-14.651371185284,17.1452153999142,0.));
#204790=CARTESIAN_POINT('Ctrl Pts',(-14.6513681262571,17.1452095830633,
0.));
#204791=CARTESIAN_POINT('',(-17.9112098770111,18.8464468996588,0.));
#204792=CARTESIAN_POINT('Ctrl Pts',(-12.7689476255363,18.5896416359912,
0.));
#204793=CARTESIAN_POINT('Ctrl Pts',(-12.7689476255363,18.5896416359912,
12.));
#204794=CARTESIAN_POINT('Ctrl Pts',(-12.7689524524483,18.5896460962964,
0.));
#204795=CARTESIAN_POINT('Ctrl Pts',(-12.7689524524483,18.5896460962964,
12.));
#204796=CARTESIAN_POINT('Ctrl Pts',(-12.768986426692,18.5896919669165,0.));
#204797=CARTESIAN_POINT('Ctrl Pts',(-12.768986426692,18.5896919669165,12.));
#204798=CARTESIAN_POINT('Ctrl Pts',(-12.769110348199,18.589871621843,0.));
#204799=CARTESIAN_POINT('Ctrl Pts',(-12.769110348199,18.589871621843,12.));
#204800=CARTESIAN_POINT('Ctrl Pts',(-12.7694215127919,18.5903328777227,
0.));
#204801=CARTESIAN_POINT('Ctrl Pts',(-12.7694215127919,18.5903328777227,
12.));
#204802=CARTESIAN_POINT('Ctrl Pts',(-12.7700520897173,18.5912775137806,
0.));
#204803=CARTESIAN_POINT('Ctrl Pts',(-12.7700520897173,18.5912775137806,
12.));
#204804=CARTESIAN_POINT('Ctrl Pts',(-12.7709195951156,18.5925859134579,
0.));
#204805=CARTESIAN_POINT('Ctrl Pts',(-12.7709195951156,18.5925859134579,
12.));
#204806=CARTESIAN_POINT('Ctrl Pts',(-12.7720142287172,18.5942490615407,
0.));
#204807=CARTESIAN_POINT('Ctrl Pts',(-12.7720142287172,18.5942490615407,
12.));
#204808=CARTESIAN_POINT('Ctrl Pts',(-12.7733231262108,18.5962551167772,
0.));
#204809=CARTESIAN_POINT('Ctrl Pts',(-12.7733231262108,18.5962551167772,
12.));
#204810=CARTESIAN_POINT('Ctrl Pts',(-12.7748328937638,18.598591752595,0.));
#204811=CARTESIAN_POINT('Ctrl Pts',(-12.7748328937638,18.598591752595,12.));
#204812=CARTESIAN_POINT('Ctrl Pts',(-12.7765325225081,18.6012488486709,
0.));
#204813=CARTESIAN_POINT('Ctrl Pts',(-12.7765325225081,18.6012488486709,
12.));
#204814=CARTESIAN_POINT('Ctrl Pts',(-12.7784139605066,18.6042190183704,
0.));
#204815=CARTESIAN_POINT('Ctrl Pts',(-12.7784139605066,18.6042190183704,
12.));
#204816=CARTESIAN_POINT('Ctrl Pts',(-12.7804705387658,18.6074961535723,
0.));
#204817=CARTESIAN_POINT('Ctrl Pts',(-12.7804705387658,18.6074961535723,
12.));
#204818=CARTESIAN_POINT('Ctrl Pts',(-12.7826959526925,18.6110744826219,
0.));
#204819=CARTESIAN_POINT('Ctrl Pts',(-12.7826959526925,18.6110744826219,
12.));
#204820=CARTESIAN_POINT('Ctrl Pts',(-12.7850831657901,18.6149475565188,
0.));
#204821=CARTESIAN_POINT('Ctrl Pts',(-12.7850831657901,18.6149475565188,
12.));
#204822=CARTESIAN_POINT('Ctrl Pts',(-12.7876249657834,18.6191087624752,
0.));
#204823=CARTESIAN_POINT('Ctrl Pts',(-12.7876249657834,18.6191087624752,
12.));
#204824=CARTESIAN_POINT('Ctrl Pts',(-12.7903142925234,18.6235516265575,
0.));
#204825=CARTESIAN_POINT('Ctrl Pts',(-12.7903142925234,18.6235516265575,
12.));
#204826=CARTESIAN_POINT('Ctrl Pts',(-12.7931447451555,18.6282702819371,
0.));
#204827=CARTESIAN_POINT('Ctrl Pts',(-12.7931447451555,18.6282702819371,
12.));
#204828=CARTESIAN_POINT('Ctrl Pts',(-12.7961106222251,18.6332595057006,
0.));
#204829=CARTESIAN_POINT('Ctrl Pts',(-12.7961106222251,18.6332595057006,
12.));
#204830=CARTESIAN_POINT('Ctrl Pts',(-12.7992066625264,18.63851447924,0.));
#204831=CARTESIAN_POINT('Ctrl Pts',(-12.7992066625264,18.63851447924,12.));
#204832=CARTESIAN_POINT('Ctrl Pts',(-12.8024278770152,18.6440306327456,
0.));
#204833=CARTESIAN_POINT('Ctrl Pts',(-12.8024278770152,18.6440306327456,
12.));
#204834=CARTESIAN_POINT('Ctrl Pts',(-12.805769331162,18.6498034438986,0.));
#204835=CARTESIAN_POINT('Ctrl Pts',(-12.805769331162,18.6498034438986,12.));
#204836=CARTESIAN_POINT('Ctrl Pts',(-12.8092261933858,18.6558284825773,
0.));
#204837=CARTESIAN_POINT('Ctrl Pts',(-12.8092261933858,18.6558284825773,
12.));
#204838=CARTESIAN_POINT('Ctrl Pts',(-12.8127937909631,18.6621014624746,
0.));
#204839=CARTESIAN_POINT('Ctrl Pts',(-12.8127937909631,18.6621014624746,
12.));
#204840=CARTESIAN_POINT('Ctrl Pts',(-12.8164676687362,18.6686182952799,
0.));
#204841=CARTESIAN_POINT('Ctrl Pts',(-12.8164676687362,18.6686182952799,
12.));
#204842=CARTESIAN_POINT('Ctrl Pts',(-12.8202436318474,18.6753751301092,
0.));
#204843=CARTESIAN_POINT('Ctrl Pts',(-12.8202436318474,18.6753751301092,
12.));
#204844=CARTESIAN_POINT('Ctrl Pts',(-12.8241176980017,18.6823683094139,
0.));
#204845=CARTESIAN_POINT('Ctrl Pts',(-12.8241176980017,18.6823683094139,
12.));
#204846=CARTESIAN_POINT('Ctrl Pts',(-12.8280860635231,18.6895943376171,
0.));
#204847=CARTESIAN_POINT('Ctrl Pts',(-12.8280860635231,18.6895943376171,
12.));
#204848=CARTESIAN_POINT('Ctrl Pts',(-12.8321450599789,18.6970498410172,
0.));
#204849=CARTESIAN_POINT('Ctrl Pts',(-12.8321450599789,18.6970498410172,
12.));
#204850=CARTESIAN_POINT('Ctrl Pts',(-12.8362911280361,18.7047315436294,
0.));
#204851=CARTESIAN_POINT('Ctrl Pts',(-12.8362911280361,18.7047315436294,
12.));
#204852=CARTESIAN_POINT('Ctrl Pts',(-12.8405208263431,18.7126362754445,
0.));
#204853=CARTESIAN_POINT('Ctrl Pts',(-12.8405208263431,18.7126362754445,
12.));
#204854=CARTESIAN_POINT('Ctrl Pts',(-12.8448308329494,18.7207609737702,
0.));
#204855=CARTESIAN_POINT('Ctrl Pts',(-12.8448308329494,18.7207609737702,
12.));
#204856=CARTESIAN_POINT('Ctrl Pts',(-12.8492179511591,18.7291026886554,
0.));
#204857=CARTESIAN_POINT('Ctrl Pts',(-12.8492179511591,18.7291026886554,
12.));
#204858=CARTESIAN_POINT('Ctrl Pts',(-12.8536791086316,18.7376585820854,
0.));
#204859=CARTESIAN_POINT('Ctrl Pts',(-12.8536791086316,18.7376585820854,
12.));
#204860=CARTESIAN_POINT('Ctrl Pts',(-12.8582113455646,18.7464259171251,
0.));
#204861=CARTESIAN_POINT('Ctrl Pts',(-12.8582113455646,18.7464259171251,
12.));
#204862=CARTESIAN_POINT('Ctrl Pts',(-12.8628118054171,18.7554020493887,
0.));
#204863=CARTESIAN_POINT('Ctrl Pts',(-12.8628118054171,18.7554020493887,
12.));
#204864=CARTESIAN_POINT('Ctrl Pts',(-12.8674777239653,18.7645844169564,
0.));
#204865=CARTESIAN_POINT('Ctrl Pts',(-12.8674777239653,18.7645844169564,
12.));
#204866=CARTESIAN_POINT('Ctrl Pts',(-12.872206421181,18.7739705329022,0.));
#204867=CARTESIAN_POINT('Ctrl Pts',(-12.872206421181,18.7739705329022,12.));
#204868=CARTESIAN_POINT('Ctrl Pts',(-12.8769952998095,18.7835579840477,
0.));
#204869=CARTESIAN_POINT('Ctrl Pts',(-12.8769952998095,18.7835579840477,
12.));
#204870=CARTESIAN_POINT('Ctrl Pts',(-12.8818418427475,18.7933444285868,
0.));
#204871=CARTESIAN_POINT('Ctrl Pts',(-12.8818418427475,18.7933444285868,
12.));
#204872=CARTESIAN_POINT('Ctrl Pts',(-12.8867436109546,18.8033275941943,
0.));
#204873=CARTESIAN_POINT('Ctrl Pts',(-12.8867436109546,18.8033275941943,
12.));
#204874=CARTESIAN_POINT('Ctrl Pts',(-12.8916982409935,18.813505275782,0.));
#204875=CARTESIAN_POINT('Ctrl Pts',(-12.8916982409935,18.813505275782,12.));
#204876=CARTESIAN_POINT('Ctrl Pts',(-12.8967034410755,18.8238753319128,
0.));
#204877=CARTESIAN_POINT('Ctrl Pts',(-12.8967034410755,18.8238753319128,
12.));
#204878=CARTESIAN_POINT('Ctrl Pts',(-12.9017569871738,18.834435681259,0.));
#204879=CARTESIAN_POINT('Ctrl Pts',(-12.9017569871738,18.834435681259,12.));
#204880=CARTESIAN_POINT('Ctrl Pts',(-12.9068567191854,18.8451842990984,
0.));
#204881=CARTESIAN_POINT('Ctrl Pts',(-12.9068567191854,18.8451842990984,
12.));
#204882=CARTESIAN_POINT('Ctrl Pts',(-12.9120005369063,18.8561192136198,
0.));
#204883=CARTESIAN_POINT('Ctrl Pts',(-12.9120005369063,18.8561192136198,
12.));
#204884=CARTESIAN_POINT('Ctrl Pts',(-12.9171863977045,18.8672385038326,
0.));
#204885=CARTESIAN_POINT('Ctrl Pts',(-12.9171863977045,18.8672385038326,
12.));
#204886=CARTESIAN_POINT('Ctrl Pts',(-12.9224123144982,18.8785402977527,
0.));
#204887=CARTESIAN_POINT('Ctrl Pts',(-12.9224123144982,18.8785402977527,
12.));
#204888=CARTESIAN_POINT('Ctrl Pts',(-12.9276763536373,18.8900227704889,
0.));
#204889=CARTESIAN_POINT('Ctrl Pts',(-12.9276763536373,18.8900227704889,
12.));
#204890=CARTESIAN_POINT('Ctrl Pts',(-12.9329766328185,18.9016841423403,
0.));
#204891=CARTESIAN_POINT('Ctrl Pts',(-12.9329766328185,18.9016841423403,
12.));
#204892=CARTESIAN_POINT('Ctrl Pts',(-12.9383113190375,18.9135226769465,
0.));
#204893=CARTESIAN_POINT('Ctrl Pts',(-12.9383113190375,18.9135226769465,
12.));
#204894=CARTESIAN_POINT('Ctrl Pts',(-12.9436786266105,18.9255366795195,
0.));
#204895=CARTESIAN_POINT('Ctrl Pts',(-12.9436786266105,18.9255366795195,
12.));
#204896=CARTESIAN_POINT('Ctrl Pts',(-12.9490768151821,18.9377244950435,
0.));
#204897=CARTESIAN_POINT('Ctrl Pts',(-12.9490768151821,18.9377244950435,
12.));
#204898=CARTESIAN_POINT('Ctrl Pts',(-12.9545041877377,18.9500845064715,
0.));
#204899=CARTESIAN_POINT('Ctrl Pts',(-12.9545041877377,18.9500845064715,
12.));
#204900=CARTESIAN_POINT('Ctrl Pts',(-12.9599590886319,18.9626151329229,
0.));
#204901=CARTESIAN_POINT('Ctrl Pts',(-12.9599590886319,18.9626151329229,
12.));
#204902=CARTESIAN_POINT('Ctrl Pts',(-12.9654399021869,18.9753148284475,
0.));
#204903=CARTESIAN_POINT('Ctrl Pts',(-12.9654399021869,18.9753148284475,
12.));
#204904=CARTESIAN_POINT('Ctrl Pts',(-12.9709450512747,18.9881820807585,
0.));
#204905=CARTESIAN_POINT('Ctrl Pts',(-12.9709450512747,18.9881820807585,
12.));
#204906=CARTESIAN_POINT('Ctrl Pts',(-12.9764729959205,19.0012154099791,
0.));
#204907=CARTESIAN_POINT('Ctrl Pts',(-12.9764729959205,19.0012154099791,
12.));
#204908=CARTESIAN_POINT('Ctrl Pts',(-12.9820222318716,19.0144133673348,
0.));
#204909=CARTESIAN_POINT('Ctrl Pts',(-12.9820222318716,19.0144133673348,
12.));
#204910=CARTESIAN_POINT('Ctrl Pts',(-12.9875912893003,19.0277745339908,
0.));
#204911=CARTESIAN_POINT('Ctrl Pts',(-12.9875912893003,19.0277745339908,
12.));
#204912=CARTESIAN_POINT('Ctrl Pts',(-12.9931787316515,19.0412975200398,
0.));
#204913=CARTESIAN_POINT('Ctrl Pts',(-12.9931787316515,19.0412975200398,
12.));
#204914=CARTESIAN_POINT('Ctrl Pts',(-12.9987831544502,19.0549809634355,
0.));
#204915=CARTESIAN_POINT('Ctrl Pts',(-12.9987831544502,19.0549809634355,
12.));
#204916=CARTESIAN_POINT('Ctrl Pts',(-13.0044031841381,19.0688235289437,
0.));
#204917=CARTESIAN_POINT('Ctrl Pts',(-13.0044031841381,19.0688235289437,
12.));
#204918=CARTESIAN_POINT('Ctrl Pts',(-13.0100374768785,19.0828239070482,
0.));
#204919=CARTESIAN_POINT('Ctrl Pts',(-13.0100374768785,19.0828239070482,
12.));
#204920=CARTESIAN_POINT('Ctrl Pts',(-13.0156847176093,19.0969808131225,
0.));
#204921=CARTESIAN_POINT('Ctrl Pts',(-13.0156847176093,19.0969808131225,
12.));
#204922=CARTESIAN_POINT('Ctrl Pts',(-13.0213436191326,19.1112929866308,
0.));
#204923=CARTESIAN_POINT('Ctrl Pts',(-13.0213436191326,19.1112929866308,
12.));
#204924=CARTESIAN_POINT('Ctrl Pts',(-13.0270129211976,19.1257591903099,
0.));
#204925=CARTESIAN_POINT('Ctrl Pts',(-13.0270129211976,19.1257591903099,
12.));
#204926=CARTESIAN_POINT('Ctrl Pts',(-13.0326913895841,19.1403782093389,
0.));
#204927=CARTESIAN_POINT('Ctrl Pts',(-13.0326913895841,19.1403782093389,
12.));
#204928=CARTESIAN_POINT('Ctrl Pts',(-13.0383778152072,19.1551488505233,
0.));
#204929=CARTESIAN_POINT('Ctrl Pts',(-13.0383778152072,19.1551488505233,
12.));
#204930=CARTESIAN_POINT('Ctrl Pts',(-13.0440710133775,19.1700699416625,
0.));
#204931=CARTESIAN_POINT('Ctrl Pts',(-13.0440710133775,19.1700699416625,
12.));
#204932=CARTESIAN_POINT('Ctrl Pts',(-13.0497698230442,19.1851403308825,
0.));
#204933=CARTESIAN_POINT('Ctrl Pts',(-13.0497698230442,19.1851403308825,
12.));
#204934=CARTESIAN_POINT('Ctrl Pts',(-13.0554731060537,19.2003588859771,
0.));
#204935=CARTESIAN_POINT('Ctrl Pts',(-13.0554731060537,19.2003588859771,
12.));
#204936=CARTESIAN_POINT('Ctrl Pts',(-13.0611797463913,19.2157244937141,
0.));
#204937=CARTESIAN_POINT('Ctrl Pts',(-13.0611797463913,19.2157244937141,
12.));
#204938=CARTESIAN_POINT('Ctrl Pts',(-13.0668886494791,19.2312360592031,
0.));
#204939=CARTESIAN_POINT('Ctrl Pts',(-13.0668886494791,19.2312360592031,
12.));
#204940=CARTESIAN_POINT('Ctrl Pts',(-13.0725987415856,19.2468925053988,
0.));
#204941=CARTESIAN_POINT('Ctrl Pts',(-13.0725987415856,19.2468925053988,
12.));
#204942=CARTESIAN_POINT('Ctrl Pts',(-13.0783089692118,19.2626927725596,
0.));
#204943=CARTESIAN_POINT('Ctrl Pts',(-13.0783089692118,19.2626927725596,
12.));
#204944=CARTESIAN_POINT('Ctrl Pts',(-13.0840182984949,19.2786358177198,
0.));
#204945=CARTESIAN_POINT('Ctrl Pts',(-13.0840182984949,19.2786358177198,
12.));
#204946=CARTESIAN_POINT('Ctrl Pts',(-13.089725714597,19.2947206141246,0.));
#204947=CARTESIAN_POINT('Ctrl Pts',(-13.089725714597,19.2947206141246,12.));
#204948=CARTESIAN_POINT('Ctrl Pts',(-13.095430221148,19.3109461507358,0.));
#204949=CARTESIAN_POINT('Ctrl Pts',(-13.095430221148,19.3109461507358,12.));
#204950=CARTESIAN_POINT('Ctrl Pts',(-13.1011308397592,19.3273114318268,
0.));
#204951=CARTESIAN_POINT('Ctrl Pts',(-13.1011308397592,19.3273114318268,
12.));
#204952=CARTESIAN_POINT('Ctrl Pts',(-13.1068266095186,19.3438154765395,
0.));
#204953=CARTESIAN_POINT('Ctrl Pts',(-13.1068266095186,19.3438154765395,
12.));
#204954=CARTESIAN_POINT('Ctrl Pts',(-13.1125165865021,19.3604573184516,
0.));
#204955=CARTESIAN_POINT('Ctrl Pts',(-13.1125165865021,19.3604573184516,
12.));
#204956=CARTESIAN_POINT('Ctrl Pts',(-13.118199843271,19.3772360051093,0.));
#204957=CARTESIAN_POINT('Ctrl Pts',(-13.118199843271,19.3772360051093,12.));
#204958=CARTESIAN_POINT('Ctrl Pts',(-13.1238754684177,19.3941505976267,
0.));
#204959=CARTESIAN_POINT('Ctrl Pts',(-13.1238754684177,19.3941505976267,
12.));
#204960=CARTESIAN_POINT('Ctrl Pts',(-13.1295425661635,19.4112001703561,
0.));
#204961=CARTESIAN_POINT('Ctrl Pts',(-13.1295425661635,19.4112001703561,
12.));
#204962=CARTESIAN_POINT('Ctrl Pts',(-13.1352002559439,19.4283838105265,
0.));
#204963=CARTESIAN_POINT('Ctrl Pts',(-13.1352002559439,19.4283838105265,
12.));
#204964=CARTESIAN_POINT('Ctrl Pts',(-13.140847672006,19.4457006178875,0.));
#204965=CARTESIAN_POINT('Ctrl Pts',(-13.140847672006,19.4457006178875,12.));
#204966=CARTESIAN_POINT('Ctrl Pts',(-13.1464839629966,19.463149704325,0.));
#204967=CARTESIAN_POINT('Ctrl Pts',(-13.1464839629966,19.463149704325,12.));
#204968=CARTESIAN_POINT('Ctrl Pts',(-13.1521082915846,19.4807301935256,
0.));
#204969=CARTESIAN_POINT('Ctrl Pts',(-13.1521082915846,19.4807301935256,
12.));
#204970=CARTESIAN_POINT('Ctrl Pts',(-13.1577198341238,19.498441220707,0.));
#204971=CARTESIAN_POINT('Ctrl Pts',(-13.1577198341238,19.498441220707,12.));
#204972=CARTESIAN_POINT('Ctrl Pts',(-13.1633177803097,19.5162819323207,
0.));
#204973=CARTESIAN_POINT('Ctrl Pts',(-13.1633177803097,19.5162819323207,
12.));
#204974=CARTESIAN_POINT('Ctrl Pts',(-13.1689013328432,19.5342514857564,
0.));
#204975=CARTESIAN_POINT('Ctrl Pts',(-13.1689013328432,19.5342514857564,
12.));
#204976=CARTESIAN_POINT('Ctrl Pts',(-13.1744697070918,19.5523490490254,
0.));
#204977=CARTESIAN_POINT('Ctrl Pts',(-13.1744697070918,19.5523490490254,
12.));
#204978=CARTESIAN_POINT('Ctrl Pts',(-13.1800221307683,19.5705738004682,
0.));
#204979=CARTESIAN_POINT('Ctrl Pts',(-13.1800221307683,19.5705738004682,
12.));
#204980=CARTESIAN_POINT('Ctrl Pts',(-13.1855578436479,19.5889249285351,
0.));
#204981=CARTESIAN_POINT('Ctrl Pts',(-13.1855578436479,19.5889249285351,
12.));
#204982=CARTESIAN_POINT('Ctrl Pts',(-13.1910760972818,19.6074016315421,
0.));
#204983=CARTESIAN_POINT('Ctrl Pts',(-13.1910760972818,19.6074016315421,
12.));
#204984=CARTESIAN_POINT('Ctrl Pts',(-13.196576154715,19.6260031174244,0.));
#204985=CARTESIAN_POINT('Ctrl Pts',(-13.196576154715,19.6260031174244,12.));
#204986=CARTESIAN_POINT('Ctrl Pts',(-13.202057290206,19.6447286034764,0.));
#204987=CARTESIAN_POINT('Ctrl Pts',(-13.202057290206,19.6447286034764,12.));
#204988=CARTESIAN_POINT('Ctrl Pts',(-13.2075187889522,19.6635773160924,
0.));
#204989=CARTESIAN_POINT('Ctrl Pts',(-13.2075187889522,19.6635773160924,
12.));
#204990=CARTESIAN_POINT('Ctrl Pts',(-13.2129599468478,19.6825484905812,
0.));
#204991=CARTESIAN_POINT('Ctrl Pts',(-13.2129599468478,19.6825484905812,
12.));
#204992=CARTESIAN_POINT('Ctrl Pts',(-13.2183800702431,19.7016413709678,
0.));
#204993=CARTESIAN_POINT('Ctrl Pts',(-13.2183800702431,19.7016413709678,
12.));
#204994=CARTESIAN_POINT('Ctrl Pts',(-13.2237784757065,19.7208552097867,
0.));
#204995=CARTESIAN_POINT('Ctrl Pts',(-13.2237784757065,19.7208552097867,
12.));
#204996=CARTESIAN_POINT('Ctrl Pts',(-13.2291544897902,19.7401892678701,
0.));
#204997=CARTESIAN_POINT('Ctrl Pts',(-13.2291544897902,19.7401892678701,
12.));
#204998=CARTESIAN_POINT('Ctrl Pts',(-13.2345074487968,19.7596428141176,
0.));
#204999=CARTESIAN_POINT('Ctrl Pts',(-13.2345074487968,19.7596428141176,
12.));
#205000=CARTESIAN_POINT('Ctrl Pts',(-13.239836698568,19.7792151253297,0.));
#205001=CARTESIAN_POINT('Ctrl Pts',(-13.239836698568,19.7792151253297,12.));
#205002=CARTESIAN_POINT('Ctrl Pts',(-13.2451415942809,19.7989054860501,
0.));
#205003=CARTESIAN_POINT('Ctrl Pts',(-13.2451415942809,19.7989054860501,
12.));
#205004=CARTESIAN_POINT('Ctrl Pts',(-13.2504215002458,19.8187131883919,
0.));
#205005=CARTESIAN_POINT('Ctrl Pts',(-13.2504215002458,19.8187131883919,
12.));
#205006=CARTESIAN_POINT('Ctrl Pts',(-13.2556757897085,19.8386375318632,
0.));
#205007=CARTESIAN_POINT('Ctrl Pts',(-13.2556757897085,19.8386375318632,
12.));
#205008=CARTESIAN_POINT('Ctrl Pts',(-13.2609038446525,19.8586778231711,
0.));
#205009=CARTESIAN_POINT('Ctrl Pts',(-13.2609038446525,19.8586778231711,
12.));
#205010=CARTESIAN_POINT('Ctrl Pts',(-13.2661050556128,19.8788333760571,
0.));
#205011=CARTESIAN_POINT('Ctrl Pts',(-13.2661050556128,19.8788333760571,
12.));
#205012=CARTESIAN_POINT('Ctrl Pts',(-13.2712788215015,19.8991035111739,
0.));
#205013=CARTESIAN_POINT('Ctrl Pts',(-13.2712788215015,19.8991035111739,
12.));
#205014=CARTESIAN_POINT('Ctrl Pts',(-13.2764245494354,19.9194875559419,
0.));
#205015=CARTESIAN_POINT('Ctrl Pts',(-13.2764245494354,19.9194875559419,
12.));
#205016=CARTESIAN_POINT('Ctrl Pts',(-13.2815416545663,19.9399848444019,
0.));
#205017=CARTESIAN_POINT('Ctrl Pts',(-13.2815416545663,19.9399848444019,
12.));
#205018=CARTESIAN_POINT('Ctrl Pts',(-13.2866295599152,19.9605947170589,
0.));
#205019=CARTESIAN_POINT('Ctrl Pts',(-13.2866295599152,19.9605947170589,
12.));
#205020=CARTESIAN_POINT('Ctrl Pts',(-13.2916876962098,19.9813165207174,
0.));
#205021=CARTESIAN_POINT('Ctrl Pts',(-13.2916876962098,19.9813165207174,
12.));
#205022=CARTESIAN_POINT('Ctrl Pts',(-13.296715501731,20.0021496083742,0.));
#205023=CARTESIAN_POINT('Ctrl Pts',(-13.296715501731,20.0021496083742,12.));
#205024=CARTESIAN_POINT('Ctrl Pts',(-13.3017124221639,20.0230933391039,
0.));
#205025=CARTESIAN_POINT('Ctrl Pts',(-13.3017124221639,20.0230933391039,
12.));
#205026=CARTESIAN_POINT('Ctrl Pts',(-13.3066779104515,20.0441470779345,
0.));
#205027=CARTESIAN_POINT('Ctrl Pts',(-13.3066779104515,20.0441470779345,
12.));
#205028=CARTESIAN_POINT('Ctrl Pts',(-13.3116114266514,20.0653101957188,
0.));
#205029=CARTESIAN_POINT('Ctrl Pts',(-13.3116114266514,20.0653101957188,
12.));
#205030=CARTESIAN_POINT('Ctrl Pts',(-13.3165124377963,20.0865820689883,
0.));
#205031=CARTESIAN_POINT('Ctrl Pts',(-13.3165124377963,20.0865820689883,
12.));
#205032=CARTESIAN_POINT('Ctrl Pts',(-13.3213804177588,20.1079620798377,
0.));
#205033=CARTESIAN_POINT('Ctrl Pts',(-13.3213804177588,20.1079620798377,
12.));
#205034=CARTESIAN_POINT('Ctrl Pts',(-13.3262148471228,20.1294496158405,
0.));
#205035=CARTESIAN_POINT('Ctrl Pts',(-13.3262148471228,20.1294496158405,
12.));
#205036=CARTESIAN_POINT('Ctrl Pts',(-13.3310152130565,20.1510440699477,
0.));
#205037=CARTESIAN_POINT('Ctrl Pts',(-13.3310152130565,20.1510440699477,
12.));
#205038=CARTESIAN_POINT('Ctrl Pts',(-13.3357810091903,20.1727448403818,
0.));
#205039=CARTESIAN_POINT('Ctrl Pts',(-13.3357810091903,20.1727448403818,
12.));
#205040=CARTESIAN_POINT('Ctrl Pts',(-13.3405117354969,20.1945513305233,
0.));
#205041=CARTESIAN_POINT('Ctrl Pts',(-13.3405117354969,20.1945513305233,
12.));
#205042=CARTESIAN_POINT('Ctrl Pts',(-13.3452068981763,20.2164629487855,
0.));
#205043=CARTESIAN_POINT('Ctrl Pts',(-13.3452068981763,20.2164629487855,
12.));
#205044=CARTESIAN_POINT('Ctrl Pts',(-13.3498660095382,20.2384791085354,
0.));
#205045=CARTESIAN_POINT('Ctrl Pts',(-13.3498660095382,20.2384791085354,
12.));
#205046=CARTESIAN_POINT('Ctrl Pts',(-13.3544885878886,20.2605992280117,
0.));
#205047=CARTESIAN_POINT('Ctrl Pts',(-13.3544885878886,20.2605992280117,
12.));
#205048=CARTESIAN_POINT('Ctrl Pts',(-13.3590741574194,20.2828227302337,
0.));
#205049=CARTESIAN_POINT('Ctrl Pts',(-13.3590741574194,20.2828227302337,
12.));
#205050=CARTESIAN_POINT('Ctrl Pts',(-13.3636222481017,20.3051490429049,
0.));
#205051=CARTESIAN_POINT('Ctrl Pts',(-13.3636222481017,20.3051490429049,
12.));
#205052=CARTESIAN_POINT('Ctrl Pts',(-13.3681323955828,20.3275775983032,
0.));
#205053=CARTESIAN_POINT('Ctrl Pts',(-13.3681323955828,20.3275775983032,
12.));
#205054=CARTESIAN_POINT('Ctrl Pts',(-13.3726041410869,20.3501078331818,
0.));
#205055=CARTESIAN_POINT('Ctrl Pts',(-13.3726041410869,20.3501078331818,
12.));
#205056=CARTESIAN_POINT('Ctrl Pts',(-13.377037031319,20.3727391887187,0.));
#205057=CARTESIAN_POINT('Ctrl Pts',(-13.377037031319,20.3727391887187,12.));
#205058=CARTESIAN_POINT('Ctrl Pts',(-13.3814306183721,20.3954711104504,
0.));
#205059=CARTESIAN_POINT('Ctrl Pts',(-13.3814306183721,20.3954711104504,
12.));
#205060=CARTESIAN_POINT('Ctrl Pts',(-13.3857844596387,20.4183030482002,
0.));
#205061=CARTESIAN_POINT('Ctrl Pts',(-13.3857844596387,20.4183030482002,
12.));
#205062=CARTESIAN_POINT('Ctrl Pts',(-13.3900981177254,20.4412344560007,
0.));
#205063=CARTESIAN_POINT('Ctrl Pts',(-13.3900981177254,20.4412344560007,
12.));
#205064=CARTESIAN_POINT('Ctrl Pts',(-13.3943711603739,20.4642647920038,
0.));
#205065=CARTESIAN_POINT('Ctrl Pts',(-13.3943711603739,20.4642647920038,
12.));
#205066=CARTESIAN_POINT('Ctrl Pts',(-13.3986031603716,20.4873935184041,
0.));
#205067=CARTESIAN_POINT('Ctrl Pts',(-13.3986031603716,20.4873935184041,
12.));
#205068=CARTESIAN_POINT('Ctrl Pts',(-13.4027936954529,20.5106201013755,
0.));
#205069=CARTESIAN_POINT('Ctrl Pts',(-13.4027936954529,20.5106201013755,
12.));
#205070=CARTESIAN_POINT('Ctrl Pts',(-13.4069423482076,20.5339440109957,
0.));
#205071=CARTESIAN_POINT('Ctrl Pts',(-13.4069423482076,20.5339440109957,
12.));
#205072=CARTESIAN_POINT('Ctrl Pts',(-13.4110487059912,20.557364721164,0.));
#205073=CARTESIAN_POINT('Ctrl Pts',(-13.4110487059912,20.557364721164,12.));
#205074=CARTESIAN_POINT('Ctrl Pts',(-13.4151123608411,20.5808817095155,
0.));
#205075=CARTESIAN_POINT('Ctrl Pts',(-13.4151123608411,20.5808817095155,
12.));
#205076=CARTESIAN_POINT('Ctrl Pts',(-13.4191329093932,20.6044944573151,
0.));
#205077=CARTESIAN_POINT('Ctrl Pts',(-13.4191329093932,20.6044944573151,
12.));
#205078=CARTESIAN_POINT('Ctrl Pts',(-13.4231099528178,20.6282024494234,
0.));
#205079=CARTESIAN_POINT('Ctrl Pts',(-13.4231099528178,20.6282024494234,
12.));
#205080=CARTESIAN_POINT('Ctrl Pts',(-13.427043096765,20.6520051742867,0.));
#205081=CARTESIAN_POINT('Ctrl Pts',(-13.427043096765,20.6520051742867,12.));
#205082=CARTESIAN_POINT('Ctrl Pts',(-13.4309319513119,20.6759021239102,
0.));
#205083=CARTESIAN_POINT('Ctrl Pts',(-13.4309319513119,20.6759021239102,
12.));
#205084=CARTESIAN_POINT('Ctrl Pts',(-13.4347761309154,20.6998927938288,
0.));
#205085=CARTESIAN_POINT('Ctrl Pts',(-13.4347761309154,20.6998927938288,
12.));
#205086=CARTESIAN_POINT('Ctrl Pts',(-13.4385752543663,20.7239766830675,
0.));
#205087=CARTESIAN_POINT('Ctrl Pts',(-13.4385752543663,20.7239766830675,
12.));
#205088=CARTESIAN_POINT('Ctrl Pts',(-13.4423289447561,20.7481532941014,
0.));
#205089=CARTESIAN_POINT('Ctrl Pts',(-13.4423289447561,20.7481532941014,
12.));
#205090=CARTESIAN_POINT('Ctrl Pts',(-13.4460368293689,20.7724221327609,
0.));
#205091=CARTESIAN_POINT('Ctrl Pts',(-13.4460368293689,20.7724221327609,
12.));
#205092=CARTESIAN_POINT('Ctrl Pts',(-13.4496985395637,20.7967827081228,
0.));
#205093=CARTESIAN_POINT('Ctrl Pts',(-13.4496985395637,20.7967827081228,
12.));
#205094=CARTESIAN_POINT('Ctrl Pts',(-13.4533137106667,20.821234532398,0.));
#205095=CARTESIAN_POINT('Ctrl Pts',(-13.4533137106667,20.821234532398,12.));
#205096=CARTESIAN_POINT('Ctrl Pts',(-13.4568819818631,20.8457771208083,
0.));
#205097=CARTESIAN_POINT('Ctrl Pts',(-13.4568819818631,20.8457771208083,
12.));
#205098=CARTESIAN_POINT('Ctrl Pts',(-13.4604029960983,20.8704099914641,
0.));
#205099=CARTESIAN_POINT('Ctrl Pts',(-13.4604029960983,20.8704099914641,
12.));
#205100=CARTESIAN_POINT('Ctrl Pts',(-13.4638763999725,20.8951326652158,
0.));
#205101=CARTESIAN_POINT('Ctrl Pts',(-13.4638763999725,20.8951326652158,
12.));
#205102=CARTESIAN_POINT('Ctrl Pts',(-13.4673018437717,20.9199446657583,
0.));
#205103=CARTESIAN_POINT('Ctrl Pts',(-13.4673018437717,20.9199446657583,
12.));
#205104=CARTESIAN_POINT('Ctrl Pts',(-13.4706789815166,20.9448455197557,
0.));
#205105=CARTESIAN_POINT('Ctrl Pts',(-13.4706789815166,20.9448455197557,
12.));
#205106=CARTESIAN_POINT('Ctrl Pts',(-13.4740074710086,20.9698347569476,
0.));
#205107=CARTESIAN_POINT('Ctrl Pts',(-13.4740074710086,20.9698347569476,
12.));
#205108=CARTESIAN_POINT('Ctrl Pts',(-13.4772869738879,20.9949119102592,
0.));
#205109=CARTESIAN_POINT('Ctrl Pts',(-13.4772869738879,20.9949119102592,
12.));
#205110=CARTESIAN_POINT('Ctrl Pts',(-13.4805171556822,21.0200765158884,
0.));
#205111=CARTESIAN_POINT('Ctrl Pts',(-13.4805171556822,21.0200765158884,
12.));
#205112=CARTESIAN_POINT('Ctrl Pts',(-13.4836976858912,21.0453281134245,
0.));
#205113=CARTESIAN_POINT('Ctrl Pts',(-13.4836976858912,21.0453281134245,
12.));
#205114=CARTESIAN_POINT('Ctrl Pts',(-13.4868282377191,21.0706662455199,
0.));
#205115=CARTESIAN_POINT('Ctrl Pts',(-13.4868282377191,21.0706662455199,
12.));
#205116=CARTESIAN_POINT('Ctrl Pts',(-13.4899084877717,21.0960904575046,
0.));
#205117=CARTESIAN_POINT('Ctrl Pts',(-13.4899084877717,21.0960904575046,
12.));
#205118=CARTESIAN_POINT('Ctrl Pts',(-13.4929381157778,21.1216002970207,
0.));
#205119=CARTESIAN_POINT('Ctrl Pts',(-13.4929381157778,21.1216002970207,
12.));
#205120=CARTESIAN_POINT('Ctrl Pts',(-13.4959168042934,21.1471953136209,
0.));
#205121=CARTESIAN_POINT('Ctrl Pts',(-13.4959168042934,21.1471953136209,
12.));
#205122=CARTESIAN_POINT('Ctrl Pts',(-13.4988442384491,21.1728750584175,
0.));
#205123=CARTESIAN_POINT('Ctrl Pts',(-13.4988442384491,21.1728750584175,
12.));
#205124=CARTESIAN_POINT('Ctrl Pts',(-13.5017201056088,21.1986390835828,
0.));
#205125=CARTESIAN_POINT('Ctrl Pts',(-13.5017201056088,21.1986390835828,
12.));
#205126=CARTESIAN_POINT('Ctrl Pts',(-13.5045440957404,21.2244869429332,
0.));
#205127=CARTESIAN_POINT('Ctrl Pts',(-13.5045440957404,21.2244869429332,
12.));
#205128=CARTESIAN_POINT('Ctrl Pts',(-13.5073159019452,21.250418192743,0.));
#205129=CARTESIAN_POINT('Ctrl Pts',(-13.5073159019452,21.250418192743,12.));
#205130=CARTESIAN_POINT('Ctrl Pts',(-13.5100352209205,21.2764323924442,
0.));
#205131=CARTESIAN_POINT('Ctrl Pts',(-13.5100352209205,21.2764323924442,
12.));
#205132=CARTESIAN_POINT('Ctrl Pts',(-13.5127017534971,21.3025291054235,
0.));
#205133=CARTESIAN_POINT('Ctrl Pts',(-13.5127017534971,21.3025291054235,
12.));
#205134=CARTESIAN_POINT('Ctrl Pts',(-13.5153152050555,21.328707899634,0.));
#205135=CARTESIAN_POINT('Ctrl Pts',(-13.5153152050555,21.328707899634,12.));
#205136=CARTESIAN_POINT('Ctrl Pts',(-13.5178752862466,21.3549683486222,
0.));
#205137=CARTESIAN_POINT('Ctrl Pts',(-13.5178752862466,21.3549683486222,
12.));
#205138=CARTESIAN_POINT('Ctrl Pts',(-13.5203817122504,21.3813100304973,
0.));
#205139=CARTESIAN_POINT('Ctrl Pts',(-13.5203817122504,21.3813100304973,
12.));
#205140=CARTESIAN_POINT('Ctrl Pts',(-13.5228342013516,21.4077325259324,
0.));
#205141=CARTESIAN_POINT('Ctrl Pts',(-13.5228342013516,21.4077325259324,
12.));
#205142=CARTESIAN_POINT('Ctrl Pts',(-13.5252324737802,21.4342354165259,
0.));
#205143=CARTESIAN_POINT('Ctrl Pts',(-13.5252324737802,21.4342354165259,
12.));
#205144=CARTESIAN_POINT('Ctrl Pts',(-13.5275762503555,21.4608182828697,
0.));
#205145=CARTESIAN_POINT('Ctrl Pts',(-13.5275762503555,21.4608182828697,
12.));
#205146=CARTESIAN_POINT('Ctrl Pts',(-13.5298652514355,21.4874807030468,
0.));
#205147=CARTESIAN_POINT('Ctrl Pts',(-13.5298652514355,21.4874807030468,
12.));
#205148=CARTESIAN_POINT('Ctrl Pts',(-13.5320991952138,21.5142222501666,
0.));
#205149=CARTESIAN_POINT('Ctrl Pts',(-13.5320991952138,21.5142222501666,
12.));
#205150=CARTESIAN_POINT('Ctrl Pts',(-13.5342777983215,21.5410424932503,
0.));
#205151=CARTESIAN_POINT('Ctrl Pts',(-13.5342777983215,21.5410424932503,
12.));
#205152=CARTESIAN_POINT('Ctrl Pts',(-13.536400779028,21.5679410019001,0.));
#205153=CARTESIAN_POINT('Ctrl Pts',(-13.536400779028,21.5679410019001,12.));
#205154=CARTESIAN_POINT('Ctrl Pts',(-13.5384678597195,21.5949173499013,
0.));
#205155=CARTESIAN_POINT('Ctrl Pts',(-13.5384678597195,21.5949173499013,
12.));
#205156=CARTESIAN_POINT('Ctrl Pts',(-13.5404787697792,21.6219711193946,
0.));
#205157=CARTESIAN_POINT('Ctrl Pts',(-13.5404787697792,21.6219711193946,
12.));
#205158=CARTESIAN_POINT('Ctrl Pts',(-13.5424332480699,21.6491019044648,
0.));
#205159=CARTESIAN_POINT('Ctrl Pts',(-13.5424332480699,21.6491019044648,
12.));
#205160=CARTESIAN_POINT('Ctrl Pts',(-13.5443310461526,21.6763093157699,
0.));
#205161=CARTESIAN_POINT('Ctrl Pts',(-13.5443310461526,21.6763093157699,
12.));
#205162=CARTESIAN_POINT('Ctrl Pts',(-13.5461719295048,21.7035929822955,
0.));
#205163=CARTESIAN_POINT('Ctrl Pts',(-13.5461719295048,21.7035929822955,
12.));
#205164=CARTESIAN_POINT('Ctrl Pts',(-13.5479556704481,21.7309525412281,
0.));
#205165=CARTESIAN_POINT('Ctrl Pts',(-13.5479556704481,21.7309525412281,
12.));
#205166=CARTESIAN_POINT('Ctrl Pts',(-13.5496820422211,21.7583876294554,
0.));
#205167=CARTESIAN_POINT('Ctrl Pts',(-13.5496820422211,21.7583876294554,
12.));
#205168=CARTESIAN_POINT('Ctrl Pts',(-13.551350812725,21.7858978745865,0.));
#205169=CARTESIAN_POINT('Ctrl Pts',(-13.551350812725,21.7858978745865,12.));
#205170=CARTESIAN_POINT('Ctrl Pts',(-13.5529617381573,21.8134828857967,
0.));
#205171=CARTESIAN_POINT('Ctrl Pts',(-13.5529617381573,21.8134828857967,
12.));
#205172=CARTESIAN_POINT('Ctrl Pts',(-13.5545145573031,21.8411422456075,
0.));
#205173=CARTESIAN_POINT('Ctrl Pts',(-13.5545145573031,21.8411422456075,
12.));
#205174=CARTESIAN_POINT('Ctrl Pts',(-13.5560089839385,21.8688754989365,
0.));
#205175=CARTESIAN_POINT('Ctrl Pts',(-13.5560089839385,21.8688754989365,
12.));
#205176=CARTESIAN_POINT('Ctrl Pts',(-13.5574447178424,21.8966821688824,
0.));
#205177=CARTESIAN_POINT('Ctrl Pts',(-13.5574447178424,21.8966821688824,
12.));
#205178=CARTESIAN_POINT('Ctrl Pts',(-13.5588214586604,21.9245617765769,
0.));
#205179=CARTESIAN_POINT('Ctrl Pts',(-13.5588214586604,21.9245617765769,
12.));
#205180=CARTESIAN_POINT('Ctrl Pts',(-13.5601389185257,21.9525138592813,
0.));
#205181=CARTESIAN_POINT('Ctrl Pts',(-13.5601389185257,21.9525138592813,
12.));
#205182=CARTESIAN_POINT('Ctrl Pts',(-13.5613968357561,21.9805379899168,
0.));
#205183=CARTESIAN_POINT('Ctrl Pts',(-13.5613968357561,21.9805379899168,
12.));
#205184=CARTESIAN_POINT('Ctrl Pts',(-13.5625949868333,22.0086337943449,
0.));
#205185=CARTESIAN_POINT('Ctrl Pts',(-13.5625949868333,22.0086337943449,
12.));
#205186=CARTESIAN_POINT('Ctrl Pts',(-13.5637332022473,22.0368009736295,
0.));
#205187=CARTESIAN_POINT('Ctrl Pts',(-13.5637332022473,22.0368009736295,
12.));
#205188=CARTESIAN_POINT('Ctrl Pts',(-13.5648113689033,22.0650393089609,
0.));
#205189=CARTESIAN_POINT('Ctrl Pts',(-13.5648113689033,22.0650393089609,
12.));
#205190=CARTESIAN_POINT('Ctrl Pts',(-13.5658294169284,22.0933486464593,
0.));
#205191=CARTESIAN_POINT('Ctrl Pts',(-13.5658294169284,22.0933486464593,
12.));
#205192=CARTESIAN_POINT('Ctrl Pts',(-13.5667873105359,22.1217288871975,
0.));
#205193=CARTESIAN_POINT('Ctrl Pts',(-13.5667873105359,22.1217288871975,
12.));
#205194=CARTESIAN_POINT('Ctrl Pts',(-13.5675054919061,22.1444897575194,
0.));
#205195=CARTESIAN_POINT('Ctrl Pts',(-13.5675054919061,22.1444897575194,
12.));
#205196=CARTESIAN_POINT('Ctrl Pts',(-13.5680170531805,22.1615922805008,
0.));
#205197=CARTESIAN_POINT('Ctrl Pts',(-13.5680170531805,22.1615922805008,
12.));
#205198=CARTESIAN_POINT('Ctrl Pts',(-13.5683460612942,22.1730081264608,
0.));
#205199=CARTESIAN_POINT('Ctrl Pts',(-13.5683460612942,22.1730081264608,
12.));
#205200=CARTESIAN_POINT('Ctrl Pts',(-13.5685075571671,22.1787195904339,
0.));
#205201=CARTESIAN_POINT('Ctrl Pts',(-13.5685075571671,22.1787195904339,
12.));
#205202=CARTESIAN_POINT('',(-13.5685075571671,22.1787195904339,0.));
#205203=CARTESIAN_POINT('Ctrl Pts',(-12.7689476255363,18.5896416359912,
0.));
#205204=CARTESIAN_POINT('Ctrl Pts',(-12.7689524524483,18.5896460962964,
0.));
#205205=CARTESIAN_POINT('Ctrl Pts',(-12.768986426692,18.5896919669165,0.));
#205206=CARTESIAN_POINT('Ctrl Pts',(-12.769110348199,18.589871621843,0.));
#205207=CARTESIAN_POINT('Ctrl Pts',(-12.7694215127919,18.5903328777227,
0.));
#205208=CARTESIAN_POINT('Ctrl Pts',(-12.7700520897173,18.5912775137806,
0.));
#205209=CARTESIAN_POINT('Ctrl Pts',(-12.7709195951156,18.5925859134579,
0.));
#205210=CARTESIAN_POINT('Ctrl Pts',(-12.7720142287172,18.5942490615407,
0.));
#205211=CARTESIAN_POINT('Ctrl Pts',(-12.7733231262108,18.5962551167772,
0.));
#205212=CARTESIAN_POINT('Ctrl Pts',(-12.7748328937638,18.598591752595,0.));
#205213=CARTESIAN_POINT('Ctrl Pts',(-12.7765325225081,18.6012488486709,
0.));
#205214=CARTESIAN_POINT('Ctrl Pts',(-12.7784139605066,18.6042190183704,
0.));
#205215=CARTESIAN_POINT('Ctrl Pts',(-12.7804705387658,18.6074961535723,
0.));
#205216=CARTESIAN_POINT('Ctrl Pts',(-12.7826959526925,18.6110744826219,
0.));
#205217=CARTESIAN_POINT('Ctrl Pts',(-12.7850831657901,18.6149475565188,
0.));
#205218=CARTESIAN_POINT('Ctrl Pts',(-12.7876249657834,18.6191087624752,
0.));
#205219=CARTESIAN_POINT('Ctrl Pts',(-12.7903142925234,18.6235516265575,
0.));
#205220=CARTESIAN_POINT('Ctrl Pts',(-12.7931447451555,18.6282702819371,
0.));
#205221=CARTESIAN_POINT('Ctrl Pts',(-12.7961106222251,18.6332595057006,
0.));
#205222=CARTESIAN_POINT('Ctrl Pts',(-12.7992066625264,18.63851447924,0.));
#205223=CARTESIAN_POINT('Ctrl Pts',(-12.8024278770152,18.6440306327456,
0.));
#205224=CARTESIAN_POINT('Ctrl Pts',(-12.805769331162,18.6498034438986,0.));
#205225=CARTESIAN_POINT('Ctrl Pts',(-12.8092261933858,18.6558284825773,
0.));
#205226=CARTESIAN_POINT('Ctrl Pts',(-12.8127937909631,18.6621014624746,
0.));
#205227=CARTESIAN_POINT('Ctrl Pts',(-12.8164676687362,18.6686182952799,
0.));
#205228=CARTESIAN_POINT('Ctrl Pts',(-12.8202436318474,18.6753751301092,
0.));
#205229=CARTESIAN_POINT('Ctrl Pts',(-12.8241176980017,18.6823683094139,
0.));
#205230=CARTESIAN_POINT('Ctrl Pts',(-12.8280860635231,18.6895943376171,
0.));
#205231=CARTESIAN_POINT('Ctrl Pts',(-12.8321450599789,18.6970498410172,
0.));
#205232=CARTESIAN_POINT('Ctrl Pts',(-12.8362911280361,18.7047315436294,
0.));
#205233=CARTESIAN_POINT('Ctrl Pts',(-12.8405208263431,18.7126362754445,
0.));
#205234=CARTESIAN_POINT('Ctrl Pts',(-12.8448308329494,18.7207609737702,
0.));
#205235=CARTESIAN_POINT('Ctrl Pts',(-12.8492179511591,18.7291026886554,
0.));
#205236=CARTESIAN_POINT('Ctrl Pts',(-12.8536791086316,18.7376585820854,
0.));
#205237=CARTESIAN_POINT('Ctrl Pts',(-12.8582113455646,18.7464259171251,
0.));
#205238=CARTESIAN_POINT('Ctrl Pts',(-12.8628118054171,18.7554020493887,
0.));
#205239=CARTESIAN_POINT('Ctrl Pts',(-12.8674777239653,18.7645844169564,
0.));
#205240=CARTESIAN_POINT('Ctrl Pts',(-12.872206421181,18.7739705329022,0.));
#205241=CARTESIAN_POINT('Ctrl Pts',(-12.8769952998095,18.7835579840477,
0.));
#205242=CARTESIAN_POINT('Ctrl Pts',(-12.8818418427475,18.7933444285868,
0.));
#205243=CARTESIAN_POINT('Ctrl Pts',(-12.8867436109546,18.8033275941943,
0.));
#205244=CARTESIAN_POINT('Ctrl Pts',(-12.8916982409935,18.813505275782,0.));
#205245=CARTESIAN_POINT('Ctrl Pts',(-12.8967034410755,18.8238753319128,
0.));
#205246=CARTESIAN_POINT('Ctrl Pts',(-12.9017569871738,18.834435681259,0.));
#205247=CARTESIAN_POINT('Ctrl Pts',(-12.9068567191854,18.8451842990984,
0.));
#205248=CARTESIAN_POINT('Ctrl Pts',(-12.9120005369063,18.8561192136198,
0.));
#205249=CARTESIAN_POINT('Ctrl Pts',(-12.9171863977045,18.8672385038326,
0.));
#205250=CARTESIAN_POINT('Ctrl Pts',(-12.9224123144982,18.8785402977527,
0.));
#205251=CARTESIAN_POINT('Ctrl Pts',(-12.9276763536373,18.8900227704889,
0.));
#205252=CARTESIAN_POINT('Ctrl Pts',(-12.9329766328185,18.9016841423403,
0.));
#205253=CARTESIAN_POINT('Ctrl Pts',(-12.9383113190375,18.9135226769465,
0.));
#205254=CARTESIAN_POINT('Ctrl Pts',(-12.9436786266105,18.9255366795195,
0.));
#205255=CARTESIAN_POINT('Ctrl Pts',(-12.9490768151821,18.9377244950435,
0.));
#205256=CARTESIAN_POINT('Ctrl Pts',(-12.9545041877377,18.9500845064715,
0.));
#205257=CARTESIAN_POINT('Ctrl Pts',(-12.9599590886319,18.9626151329229,
0.));
#205258=CARTESIAN_POINT('Ctrl Pts',(-12.9654399021869,18.9753148284475,
0.));
#205259=CARTESIAN_POINT('Ctrl Pts',(-12.9709450512747,18.9881820807585,
0.));
#205260=CARTESIAN_POINT('Ctrl Pts',(-12.9764729959205,19.0012154099791,
0.));
#205261=CARTESIAN_POINT('Ctrl Pts',(-12.9820222318716,19.0144133673348,
0.));
#205262=CARTESIAN_POINT('Ctrl Pts',(-12.9875912893003,19.0277745339908,
0.));
#205263=CARTESIAN_POINT('Ctrl Pts',(-12.9931787316515,19.0412975200398,
0.));
#205264=CARTESIAN_POINT('Ctrl Pts',(-12.9987831544502,19.0549809634355,
0.));
#205265=CARTESIAN_POINT('Ctrl Pts',(-13.0044031841381,19.0688235289437,
0.));
#205266=CARTESIAN_POINT('Ctrl Pts',(-13.0100374768785,19.0828239070482,
0.));
#205267=CARTESIAN_POINT('Ctrl Pts',(-13.0156847176093,19.0969808131225,
0.));
#205268=CARTESIAN_POINT('Ctrl Pts',(-13.0213436191326,19.1112929866308,
0.));
#205269=CARTESIAN_POINT('Ctrl Pts',(-13.0270129211976,19.1257591903099,
0.));
#205270=CARTESIAN_POINT('Ctrl Pts',(-13.0326913895841,19.1403782093389,
0.));
#205271=CARTESIAN_POINT('Ctrl Pts',(-13.0383778152072,19.1551488505233,
0.));
#205272=CARTESIAN_POINT('Ctrl Pts',(-13.0440710133775,19.1700699416625,
0.));
#205273=CARTESIAN_POINT('Ctrl Pts',(-13.0497698230442,19.1851403308825,
0.));
#205274=CARTESIAN_POINT('Ctrl Pts',(-13.0554731060537,19.2003588859771,
0.));
#205275=CARTESIAN_POINT('Ctrl Pts',(-13.0611797463913,19.2157244937141,
0.));
#205276=CARTESIAN_POINT('Ctrl Pts',(-13.0668886494791,19.2312360592031,
0.));
#205277=CARTESIAN_POINT('Ctrl Pts',(-13.0725987415856,19.2468925053988,
0.));
#205278=CARTESIAN_POINT('Ctrl Pts',(-13.0783089692118,19.2626927725596,
0.));
#205279=CARTESIAN_POINT('Ctrl Pts',(-13.0840182984949,19.2786358177198,
0.));
#205280=CARTESIAN_POINT('Ctrl Pts',(-13.089725714597,19.2947206141246,0.));
#205281=CARTESIAN_POINT('Ctrl Pts',(-13.095430221148,19.3109461507358,0.));
#205282=CARTESIAN_POINT('Ctrl Pts',(-13.1011308397592,19.3273114318268,
0.));
#205283=CARTESIAN_POINT('Ctrl Pts',(-13.1068266095186,19.3438154765395,
0.));
#205284=CARTESIAN_POINT('Ctrl Pts',(-13.1125165865021,19.3604573184516,
0.));
#205285=CARTESIAN_POINT('Ctrl Pts',(-13.118199843271,19.3772360051093,0.));
#205286=CARTESIAN_POINT('Ctrl Pts',(-13.1238754684177,19.3941505976267,
0.));
#205287=CARTESIAN_POINT('Ctrl Pts',(-13.1295425661635,19.4112001703561,
0.));
#205288=CARTESIAN_POINT('Ctrl Pts',(-13.1352002559439,19.4283838105265,
0.));
#205289=CARTESIAN_POINT('Ctrl Pts',(-13.140847672006,19.4457006178875,0.));
#205290=CARTESIAN_POINT('Ctrl Pts',(-13.1464839629966,19.463149704325,0.));
#205291=CARTESIAN_POINT('Ctrl Pts',(-13.1521082915846,19.4807301935256,
0.));
#205292=CARTESIAN_POINT('Ctrl Pts',(-13.1577198341238,19.498441220707,0.));
#205293=CARTESIAN_POINT('Ctrl Pts',(-13.1633177803097,19.5162819323207,
0.));
#205294=CARTESIAN_POINT('Ctrl Pts',(-13.1689013328432,19.5342514857564,
0.));
#205295=CARTESIAN_POINT('Ctrl Pts',(-13.1744697070918,19.5523490490254,
0.));
#205296=CARTESIAN_POINT('Ctrl Pts',(-13.1800221307683,19.5705738004682,
0.));
#205297=CARTESIAN_POINT('Ctrl Pts',(-13.1855578436479,19.5889249285351,
0.));
#205298=CARTESIAN_POINT('Ctrl Pts',(-13.1910760972818,19.6074016315421,
0.));
#205299=CARTESIAN_POINT('Ctrl Pts',(-13.196576154715,19.6260031174244,0.));
#205300=CARTESIAN_POINT('Ctrl Pts',(-13.202057290206,19.6447286034764,0.));
#205301=CARTESIAN_POINT('Ctrl Pts',(-13.2075187889522,19.6635773160924,
0.));
#205302=CARTESIAN_POINT('Ctrl Pts',(-13.2129599468478,19.6825484905812,
0.));
#205303=CARTESIAN_POINT('Ctrl Pts',(-13.2183800702431,19.7016413709678,
0.));
#205304=CARTESIAN_POINT('Ctrl Pts',(-13.2237784757065,19.7208552097867,
0.));
#205305=CARTESIAN_POINT('Ctrl Pts',(-13.2291544897902,19.7401892678701,
0.));
#205306=CARTESIAN_POINT('Ctrl Pts',(-13.2345074487968,19.7596428141176,
0.));
#205307=CARTESIAN_POINT('Ctrl Pts',(-13.239836698568,19.7792151253297,0.));
#205308=CARTESIAN_POINT('Ctrl Pts',(-13.2451415942809,19.7989054860501,
0.));
#205309=CARTESIAN_POINT('Ctrl Pts',(-13.2504215002458,19.8187131883919,
0.));
#205310=CARTESIAN_POINT('Ctrl Pts',(-13.2556757897085,19.8386375318632,
0.));
#205311=CARTESIAN_POINT('Ctrl Pts',(-13.2609038446525,19.8586778231711,
0.));
#205312=CARTESIAN_POINT('Ctrl Pts',(-13.2661050556128,19.8788333760571,
0.));
#205313=CARTESIAN_POINT('Ctrl Pts',(-13.2712788215015,19.8991035111739,
0.));
#205314=CARTESIAN_POINT('Ctrl Pts',(-13.2764245494354,19.9194875559419,
0.));
#205315=CARTESIAN_POINT('Ctrl Pts',(-13.2815416545663,19.9399848444019,
0.));
#205316=CARTESIAN_POINT('Ctrl Pts',(-13.2866295599152,19.9605947170589,
0.));
#205317=CARTESIAN_POINT('Ctrl Pts',(-13.2916876962098,19.9813165207174,
0.));
#205318=CARTESIAN_POINT('Ctrl Pts',(-13.296715501731,20.0021496083742,0.));
#205319=CARTESIAN_POINT('Ctrl Pts',(-13.3017124221639,20.0230933391039,
0.));
#205320=CARTESIAN_POINT('Ctrl Pts',(-13.3066779104515,20.0441470779345,
0.));
#205321=CARTESIAN_POINT('Ctrl Pts',(-13.3116114266514,20.0653101957188,
0.));
#205322=CARTESIAN_POINT('Ctrl Pts',(-13.3165124377963,20.0865820689883,
0.));
#205323=CARTESIAN_POINT('Ctrl Pts',(-13.3213804177588,20.1079620798377,
0.));
#205324=CARTESIAN_POINT('Ctrl Pts',(-13.3262148471228,20.1294496158405,
0.));
#205325=CARTESIAN_POINT('Ctrl Pts',(-13.3310152130565,20.1510440699477,
0.));
#205326=CARTESIAN_POINT('Ctrl Pts',(-13.3357810091903,20.1727448403818,
0.));
#205327=CARTESIAN_POINT('Ctrl Pts',(-13.3405117354969,20.1945513305233,
0.));
#205328=CARTESIAN_POINT('Ctrl Pts',(-13.3452068981763,20.2164629487855,
0.));
#205329=CARTESIAN_POINT('Ctrl Pts',(-13.3498660095382,20.2384791085354,
0.));
#205330=CARTESIAN_POINT('Ctrl Pts',(-13.3544885878886,20.2605992280117,
0.));
#205331=CARTESIAN_POINT('Ctrl Pts',(-13.3590741574194,20.2828227302337,
0.));
#205332=CARTESIAN_POINT('Ctrl Pts',(-13.3636222481017,20.3051490429049,
0.));
#205333=CARTESIAN_POINT('Ctrl Pts',(-13.3681323955828,20.3275775983032,
0.));
#205334=CARTESIAN_POINT('Ctrl Pts',(-13.3726041410869,20.3501078331818,
0.));
#205335=CARTESIAN_POINT('Ctrl Pts',(-13.377037031319,20.3727391887187,0.));
#205336=CARTESIAN_POINT('Ctrl Pts',(-13.3814306183721,20.3954711104504,
0.));
#205337=CARTESIAN_POINT('Ctrl Pts',(-13.3857844596387,20.4183030482002,
0.));
#205338=CARTESIAN_POINT('Ctrl Pts',(-13.3900981177254,20.4412344560007,
0.));
#205339=CARTESIAN_POINT('Ctrl Pts',(-13.3943711603739,20.4642647920038,
0.));
#205340=CARTESIAN_POINT('Ctrl Pts',(-13.3986031603716,20.4873935184041,
0.));
#205341=CARTESIAN_POINT('Ctrl Pts',(-13.4027936954529,20.5106201013755,
0.));
#205342=CARTESIAN_POINT('Ctrl Pts',(-13.4069423482076,20.5339440109957,
0.));
#205343=CARTESIAN_POINT('Ctrl Pts',(-13.4110487059912,20.557364721164,0.));
#205344=CARTESIAN_POINT('Ctrl Pts',(-13.4151123608411,20.5808817095155,
0.));
#205345=CARTESIAN_POINT('Ctrl Pts',(-13.4191329093932,20.6044944573151,
0.));
#205346=CARTESIAN_POINT('Ctrl Pts',(-13.4231099528178,20.6282024494234,
0.));
#205347=CARTESIAN_POINT('Ctrl Pts',(-13.427043096765,20.6520051742867,0.));
#205348=CARTESIAN_POINT('Ctrl Pts',(-13.4309319513119,20.6759021239102,
0.));
#205349=CARTESIAN_POINT('Ctrl Pts',(-13.4347761309154,20.6998927938288,
0.));
#205350=CARTESIAN_POINT('Ctrl Pts',(-13.4385752543663,20.7239766830675,
0.));
#205351=CARTESIAN_POINT('Ctrl Pts',(-13.4423289447561,20.7481532941014,
0.));
#205352=CARTESIAN_POINT('Ctrl Pts',(-13.4460368293689,20.7724221327609,
0.));
#205353=CARTESIAN_POINT('Ctrl Pts',(-13.4496985395637,20.7967827081228,
0.));
#205354=CARTESIAN_POINT('Ctrl Pts',(-13.4533137106667,20.821234532398,0.));
#205355=CARTESIAN_POINT('Ctrl Pts',(-13.4568819818631,20.8457771208083,
0.));
#205356=CARTESIAN_POINT('Ctrl Pts',(-13.4604029960983,20.8704099914641,
0.));
#205357=CARTESIAN_POINT('Ctrl Pts',(-13.4638763999725,20.8951326652158,
0.));
#205358=CARTESIAN_POINT('Ctrl Pts',(-13.4673018437717,20.9199446657583,
0.));
#205359=CARTESIAN_POINT('Ctrl Pts',(-13.4706789815166,20.9448455197557,
0.));
#205360=CARTESIAN_POINT('Ctrl Pts',(-13.4740074710086,20.9698347569476,
0.));
#205361=CARTESIAN_POINT('Ctrl Pts',(-13.4772869738879,20.9949119102592,
0.));
#205362=CARTESIAN_POINT('Ctrl Pts',(-13.4805171556822,21.0200765158884,
0.));
#205363=CARTESIAN_POINT('Ctrl Pts',(-13.4836976858912,21.0453281134245,
0.));
#205364=CARTESIAN_POINT('Ctrl Pts',(-13.4868282377191,21.0706662455199,
0.));
#205365=CARTESIAN_POINT('Ctrl Pts',(-13.4899084877717,21.0960904575046,
0.));
#205366=CARTESIAN_POINT('Ctrl Pts',(-13.4929381157778,21.1216002970207,
0.));
#205367=CARTESIAN_POINT('Ctrl Pts',(-13.4959168042934,21.1471953136209,
0.));
#205368=CARTESIAN_POINT('Ctrl Pts',(-13.4988442384491,21.1728750584175,
0.));
#205369=CARTESIAN_POINT('Ctrl Pts',(-13.5017201056088,21.1986390835828,
0.));
#205370=CARTESIAN_POINT('Ctrl Pts',(-13.5045440957404,21.2244869429332,
0.));
#205371=CARTESIAN_POINT('Ctrl Pts',(-13.5073159019452,21.250418192743,0.));
#205372=CARTESIAN_POINT('Ctrl Pts',(-13.5100352209205,21.2764323924442,
0.));
#205373=CARTESIAN_POINT('Ctrl Pts',(-13.5127017534971,21.3025291054235,
0.));
#205374=CARTESIAN_POINT('Ctrl Pts',(-13.5153152050555,21.328707899634,0.));
#205375=CARTESIAN_POINT('Ctrl Pts',(-13.5178752862466,21.3549683486222,
0.));
#205376=CARTESIAN_POINT('Ctrl Pts',(-13.5203817122504,21.3813100304973,
0.));
#205377=CARTESIAN_POINT('Ctrl Pts',(-13.5228342013516,21.4077325259324,
0.));
#205378=CARTESIAN_POINT('Ctrl Pts',(-13.5252324737802,21.4342354165259,
0.));
#205379=CARTESIAN_POINT('Ctrl Pts',(-13.5275762503555,21.4608182828697,
0.));
#205380=CARTESIAN_POINT('Ctrl Pts',(-13.5298652514355,21.4874807030468,
0.));
#205381=CARTESIAN_POINT('Ctrl Pts',(-13.5320991952138,21.5142222501666,
0.));
#205382=CARTESIAN_POINT('Ctrl Pts',(-13.5342777983215,21.5410424932503,
0.));
#205383=CARTESIAN_POINT('Ctrl Pts',(-13.536400779028,21.5679410019001,0.));
#205384=CARTESIAN_POINT('Ctrl Pts',(-13.5384678597195,21.5949173499013,
0.));
#205385=CARTESIAN_POINT('Ctrl Pts',(-13.5404787697792,21.6219711193946,
0.));
#205386=CARTESIAN_POINT('Ctrl Pts',(-13.5424332480699,21.6491019044648,
0.));
#205387=CARTESIAN_POINT('Ctrl Pts',(-13.5443310461526,21.6763093157699,
0.));
#205388=CARTESIAN_POINT('Ctrl Pts',(-13.5461719295048,21.7035929822955,
0.));
#205389=CARTESIAN_POINT('Ctrl Pts',(-13.5479556704481,21.7309525412281,
0.));
#205390=CARTESIAN_POINT('Ctrl Pts',(-13.5496820422211,21.7583876294554,
0.));
#205391=CARTESIAN_POINT('Ctrl Pts',(-13.551350812725,21.7858978745865,0.));
#205392=CARTESIAN_POINT('Ctrl Pts',(-13.5529617381573,21.8134828857967,
0.));
#205393=CARTESIAN_POINT('Ctrl Pts',(-13.5545145573031,21.8411422456075,
0.));
#205394=CARTESIAN_POINT('Ctrl Pts',(-13.5560089839385,21.8688754989365,
0.));
#205395=CARTESIAN_POINT('Ctrl Pts',(-13.5574447178424,21.8966821688824,
0.));
#205396=CARTESIAN_POINT('Ctrl Pts',(-13.5588214586604,21.9245617765769,
0.));
#205397=CARTESIAN_POINT('Ctrl Pts',(-13.5601389185257,21.9525138592813,
0.));
#205398=CARTESIAN_POINT('Ctrl Pts',(-13.5613968357561,21.9805379899168,
0.));
#205399=CARTESIAN_POINT('Ctrl Pts',(-13.5625949868333,22.0086337943449,
0.));
#205400=CARTESIAN_POINT('Ctrl Pts',(-13.5637332022473,22.0368009736295,
0.));
#205401=CARTESIAN_POINT('Ctrl Pts',(-13.5648113689033,22.0650393089609,
0.));
#205402=CARTESIAN_POINT('Ctrl Pts',(-13.5658294169284,22.0933486464593,
0.));
#205403=CARTESIAN_POINT('Ctrl Pts',(-13.5667873105359,22.1217288871975,
0.));
#205404=CARTESIAN_POINT('Ctrl Pts',(-13.5675054919061,22.1444897575194,
0.));
#205405=CARTESIAN_POINT('Ctrl Pts',(-13.5680170531805,22.1615922805008,
0.));
#205406=CARTESIAN_POINT('Ctrl Pts',(-13.5683460612942,22.1730081264608,
0.));
#205407=CARTESIAN_POINT('Ctrl Pts',(-13.5685075571671,22.1787195904339,
0.));
#205408=CARTESIAN_POINT('',(-13.5685075571671,22.1787195904339,0.));
#205409=CARTESIAN_POINT('Origin',(-7.17139709155223,20.2687213152502,0.));
#205410=CARTESIAN_POINT('',(-7.52250298901264,21.2610617890679,0.));
#205411=CARTESIAN_POINT('',(-7.52250298901264,21.2610617890679,0.));
#205412=CARTESIAN_POINT('',(-3.58569854577611,10.1343606576251,0.));
#205413=CARTESIAN_POINT('Ctrl Pts',(-12.4230808101438,22.8400320311648,
0.));
#205414=CARTESIAN_POINT('Ctrl Pts',(-12.4230808101438,22.8400320311648,
12.));
#205415=CARTESIAN_POINT('Ctrl Pts',(-12.418215285186,22.8370364396459,0.));
#205416=CARTESIAN_POINT('Ctrl Pts',(-12.418215285186,22.8370364396459,12.));
#205417=CARTESIAN_POINT('Ctrl Pts',(-12.4084933766347,22.8310435872747,
0.));
#205418=CARTESIAN_POINT('Ctrl Pts',(-12.4084933766347,22.8310435872747,
12.));
#205419=CARTESIAN_POINT('Ctrl Pts',(-12.3939379378998,22.8220493007173,
0.));
#205420=CARTESIAN_POINT('Ctrl Pts',(-12.3939379378998,22.8220493007173,
12.));
#205421=CARTESIAN_POINT('Ctrl Pts',(-12.374585536673,22.81004690224,0.));
#205422=CARTESIAN_POINT('Ctrl Pts',(-12.374585536673,22.81004690224,12.));
#205423=CARTESIAN_POINT('Ctrl Pts',(-12.3504864740319,22.795027221673,0.));
#205424=CARTESIAN_POINT('Ctrl Pts',(-12.3504864740319,22.795027221673,12.));
#205425=CARTESIAN_POINT('Ctrl Pts',(-12.3264788926075,22.7799908974768,
0.));
#205426=CARTESIAN_POINT('Ctrl Pts',(-12.3264788926075,22.7799908974768,
12.));
#205427=CARTESIAN_POINT('Ctrl Pts',(-12.3025628601792,22.764938010105,0.));
#205428=CARTESIAN_POINT('Ctrl Pts',(-12.3025628601792,22.764938010105,12.));
#205429=CARTESIAN_POINT('Ctrl Pts',(-12.2787384750742,22.7498686970069,
0.));
#205430=CARTESIAN_POINT('Ctrl Pts',(-12.2787384750742,22.7498686970069,
12.));
#205431=CARTESIAN_POINT('Ctrl Pts',(-12.2550058702395,22.7347831655287,
0.));
#205432=CARTESIAN_POINT('Ctrl Pts',(-12.2550058702395,22.7347831655287,
12.));
#205433=CARTESIAN_POINT('Ctrl Pts',(-12.2313652198061,22.7196817119374,
0.));
#205434=CARTESIAN_POINT('Ctrl Pts',(-12.2313652198061,22.7196817119374,
12.));
#205435=CARTESIAN_POINT('Ctrl Pts',(-12.2078167360284,22.7045647168747,
0.));
#205436=CARTESIAN_POINT('Ctrl Pts',(-12.2078167360284,22.7045647168747,
12.));
#205437=CARTESIAN_POINT('Ctrl Pts',(-12.1843606579262,22.6894326205037,
0.));
#205438=CARTESIAN_POINT('Ctrl Pts',(-12.1843606579262,22.6894326205037,
12.));
#205439=CARTESIAN_POINT('Ctrl Pts',(-12.1609972423099,22.6742859034944,
0.));
#205440=CARTESIAN_POINT('Ctrl Pts',(-12.1609972423099,22.6742859034944,
12.));
#205441=CARTESIAN_POINT('Ctrl Pts',(-12.1377267537145,22.6591250653965,
0.));
#205442=CARTESIAN_POINT('Ctrl Pts',(-12.1377267537145,22.6591250653965,
12.));
#205443=CARTESIAN_POINT('Ctrl Pts',(-12.1145494550383,22.6439506046605,
0.));
#205444=CARTESIAN_POINT('Ctrl Pts',(-12.1145494550383,22.6439506046605,
12.));
#205445=CARTESIAN_POINT('Ctrl Pts',(-12.0914655972823,22.6287629967056,
0.));
#205446=CARTESIAN_POINT('Ctrl Pts',(-12.0914655972823,22.6287629967056,
12.));
#205447=CARTESIAN_POINT('Ctrl Pts',(-12.0684754113862,22.6135626764898,
0.));
#205448=CARTESIAN_POINT('Ctrl Pts',(-12.0684754113862,22.6135626764898,
12.));
#205449=CARTESIAN_POINT('Ctrl Pts',(-12.0455791139128,22.5983500505644,
0.));
#205450=CARTESIAN_POINT('Ctrl Pts',(-12.0455791139128,22.5983500505644,
12.));
#205451=CARTESIAN_POINT('Ctrl Pts',(-12.0227769113127,22.5831255061282,
0.));
#205452=CARTESIAN_POINT('Ctrl Pts',(-12.0227769113127,22.5831255061282,
12.));
#205453=CARTESIAN_POINT('Ctrl Pts',(-12.0000690046695,22.5678894211181,
0.));
#205454=CARTESIAN_POINT('Ctrl Pts',(-12.0000690046695,22.5678894211181,
12.));
#205455=CARTESIAN_POINT('Ctrl Pts',(-11.9774555943496,22.5526421741158,
0.));
#205456=CARTESIAN_POINT('Ctrl Pts',(-11.9774555943496,22.5526421741158,
12.));
#205457=CARTESIAN_POINT('Ctrl Pts',(-11.9549368843997,22.5373841537307,
0.));
#205458=CARTESIAN_POINT('Ctrl Pts',(-11.9549368843997,22.5373841537307,
12.));
#205459=CARTESIAN_POINT('Ctrl Pts',(-11.9325130877803,22.5221157697883,
0.));
#205460=CARTESIAN_POINT('Ctrl Pts',(-11.9325130877803,22.5221157697883,
12.));
#205461=CARTESIAN_POINT('Ctrl Pts',(-11.9101844254557,22.5068374513973,
0.));
#205462=CARTESIAN_POINT('Ctrl Pts',(-11.9101844254557,22.5068374513973,
12.));
#205463=CARTESIAN_POINT('Ctrl Pts',(-11.8879511239943,22.4915496418485,
0.));
#205464=CARTESIAN_POINT('Ctrl Pts',(-11.8879511239943,22.4915496418485,
12.));
#205465=CARTESIAN_POINT('Ctrl Pts',(-11.8658134137019,22.4762527946702,
0.));
#205466=CARTESIAN_POINT('Ctrl Pts',(-11.8658134137019,22.4762527946702,
12.));
#205467=CARTESIAN_POINT('Ctrl Pts',(-11.8437715264487,22.4609473690471,
0.));
#205468=CARTESIAN_POINT('Ctrl Pts',(-11.8437715264487,22.4609473690471,
12.));
#205469=CARTESIAN_POINT('Ctrl Pts',(-11.8218256937889,22.4456338258735,
0.));
#205470=CARTESIAN_POINT('Ctrl Pts',(-11.8218256937889,22.4456338258735,
12.));
#205471=CARTESIAN_POINT('Ctrl Pts',(-11.7999761445173,22.430312622646,0.));
#205472=CARTESIAN_POINT('Ctrl Pts',(-11.7999761445173,22.430312622646,12.));
#205473=CARTESIAN_POINT('Ctrl Pts',(-11.7782231042039,22.4149842125008,
0.));
#205474=CARTESIAN_POINT('Ctrl Pts',(-11.7782231042039,22.4149842125008,
12.));
#205475=CARTESIAN_POINT('Ctrl Pts',(-11.7565667964764,22.3996490469191,
0.));
#205476=CARTESIAN_POINT('Ctrl Pts',(-11.7565667964764,22.3996490469191,
12.));
#205477=CARTESIAN_POINT('Ctrl Pts',(-11.7350074437961,22.3843075773899,
0.));
#205478=CARTESIAN_POINT('Ctrl Pts',(-11.7350074437961,22.3843075773899,
12.));
#205479=CARTESIAN_POINT('Ctrl Pts',(-11.7135452684532,22.3689602575491,
0.));
#205480=CARTESIAN_POINT('Ctrl Pts',(-11.7135452684532,22.3689602575491,
12.));
#205481=CARTESIAN_POINT('Ctrl Pts',(-11.6921804934056,22.3536075450029,
0.));
#205482=CARTESIAN_POINT('Ctrl Pts',(-11.6921804934056,22.3536075450029,
12.));
#205483=CARTESIAN_POINT('Ctrl Pts',(-11.6709133432985,22.3382499035619,
0.));
#205484=CARTESIAN_POINT('Ctrl Pts',(-11.6709133432985,22.3382499035619,
12.));
#205485=CARTESIAN_POINT('Ctrl Pts',(-11.6497440449857,22.3228878043976,
0.));
#205486=CARTESIAN_POINT('Ctrl Pts',(-11.6497440449857,22.3228878043976,
12.));
#205487=CARTESIAN_POINT('Ctrl Pts',(-11.6286728270009,22.3075217249049,
0.));
#205488=CARTESIAN_POINT('Ctrl Pts',(-11.6286728270009,22.3075217249049,
12.));
#205489=CARTESIAN_POINT('Ctrl Pts',(-11.6076999192357,22.2921521480356,
0.));
#205490=CARTESIAN_POINT('Ctrl Pts',(-11.6076999192357,22.2921521480356,
12.));
#205491=CARTESIAN_POINT('Ctrl Pts',(-11.5868255525188,22.2767795614348,
0.));
#205492=CARTESIAN_POINT('Ctrl Pts',(-11.5868255525188,22.2767795614348,
12.));
#205493=CARTESIAN_POINT('Ctrl Pts',(-11.5660499582403,22.2614044566898,
0.));
#205494=CARTESIAN_POINT('Ctrl Pts',(-11.5660499582403,22.2614044566898,
12.));
#205495=CARTESIAN_POINT('Ctrl Pts',(-11.5453733679121,22.2460273284654,
0.));
#205496=CARTESIAN_POINT('Ctrl Pts',(-11.5453733679121,22.2460273284654,
12.));
#205497=CARTESIAN_POINT('Ctrl Pts',(-11.5247960128477,22.2306486738901,
0.));
#205498=CARTESIAN_POINT('Ctrl Pts',(-11.5247960128477,22.2306486738901,
12.));
#205499=CARTESIAN_POINT('Ctrl Pts',(-11.5043181244242,22.2152689931022,
0.));
#205500=CARTESIAN_POINT('Ctrl Pts',(-11.5043181244242,22.2152689931022,
12.));
#205501=CARTESIAN_POINT('Ctrl Pts',(-11.483939934259,22.1998887896436,0.));
#205502=CARTESIAN_POINT('Ctrl Pts',(-11.483939934259,22.1998887896436,12.));
#205503=CARTESIAN_POINT('Ctrl Pts',(-11.463661674411,22.184508570917,0.));
#205504=CARTESIAN_POINT('Ctrl Pts',(-11.463661674411,22.184508570917,12.));
#205505=CARTESIAN_POINT('Ctrl Pts',(-11.443483577557,22.1691288486096,0.));
#205506=CARTESIAN_POINT('Ctrl Pts',(-11.443483577557,22.1691288486096,12.));
#205507=CARTESIAN_POINT('Ctrl Pts',(-11.4234058771742,22.1537501391487,
0.));
#205508=CARTESIAN_POINT('Ctrl Pts',(-11.4234058771742,22.1537501391487,
12.));
#205509=CARTESIAN_POINT('Ctrl Pts',(-11.4034288076908,22.1383729640964,
0.));
#205510=CARTESIAN_POINT('Ctrl Pts',(-11.4034288076908,22.1383729640964,
12.));
#205511=CARTESIAN_POINT('Ctrl Pts',(-11.3835526044256,22.1229978500186,
0.));
#205512=CARTESIAN_POINT('Ctrl Pts',(-11.3835526044256,22.1229978500186,
12.));
#205513=CARTESIAN_POINT('Ctrl Pts',(-11.3637775035367,22.1076253283979,
0.));
#205514=CARTESIAN_POINT('Ctrl Pts',(-11.3637775035367,22.1076253283979,
12.));
#205515=CARTESIAN_POINT('Ctrl Pts',(-11.3441037419553,22.0922559355294,
0.));
#205516=CARTESIAN_POINT('Ctrl Pts',(-11.3441037419553,22.0922559355294,
12.));
#205517=CARTESIAN_POINT('Ctrl Pts',(-11.3245315573168,22.0768902124267,
0.));
#205518=CARTESIAN_POINT('Ctrl Pts',(-11.3245315573168,22.0768902124267,
12.));
#205519=CARTESIAN_POINT('Ctrl Pts',(-11.3050611878771,22.0615287047179,
0.));
#205520=CARTESIAN_POINT('Ctrl Pts',(-11.3050611878771,22.0615287047179,
12.));
#205521=CARTESIAN_POINT('Ctrl Pts',(-11.2856928724374,22.046171962566,0.));
#205522=CARTESIAN_POINT('Ctrl Pts',(-11.2856928724374,22.046171962566,12.));
#205523=CARTESIAN_POINT('Ctrl Pts',(-11.2664268504206,22.030820540835,0.));
#205524=CARTESIAN_POINT('Ctrl Pts',(-11.2664268504206,22.030820540835,12.));
#205525=CARTESIAN_POINT('Ctrl Pts',(-11.2472633619275,22.0154749992363,
0.));
#205526=CARTESIAN_POINT('Ctrl Pts',(-11.2472633619275,22.0154749992363,
12.));
#205527=CARTESIAN_POINT('Ctrl Pts',(-11.2282026477896,22.0001359024839,
0.));
#205528=CARTESIAN_POINT('Ctrl Pts',(-11.2282026477896,22.0001359024839,
12.));
#205529=CARTESIAN_POINT('Ctrl Pts',(-11.2092449496125,21.9848038204439,
0.));
#205530=CARTESIAN_POINT('Ctrl Pts',(-11.2092449496125,21.9848038204439,
12.));
#205531=CARTESIAN_POINT('Ctrl Pts',(-11.190390509811,21.9694793282914,0.));
#205532=CARTESIAN_POINT('Ctrl Pts',(-11.190390509811,21.9694793282914,12.));
#205533=CARTESIAN_POINT('Ctrl Pts',(-11.1716395716376,21.9541630066506,
0.));
#205534=CARTESIAN_POINT('Ctrl Pts',(-11.1716395716376,21.9541630066506,
12.));
#205535=CARTESIAN_POINT('Ctrl Pts',(-11.1529923792003,21.9388554416439,
0.));
#205536=CARTESIAN_POINT('Ctrl Pts',(-11.1529923792003,21.9388554416439,
12.));
#205537=CARTESIAN_POINT('Ctrl Pts',(-11.1344491774741,21.923557224952,0.));
#205538=CARTESIAN_POINT('Ctrl Pts',(-11.1344491774741,21.923557224952,12.));
#205539=CARTESIAN_POINT('Ctrl Pts',(-11.1160102123024,21.9082689538688,
0.));
#205540=CARTESIAN_POINT('Ctrl Pts',(-11.1160102123024,21.9082689538688,
12.));
#205541=CARTESIAN_POINT('Ctrl Pts',(-11.0976757303944,21.8929912313608,
0.));
#205542=CARTESIAN_POINT('Ctrl Pts',(-11.0976757303944,21.8929912313608,
12.));
#205543=CARTESIAN_POINT('Ctrl Pts',(-11.0794459793057,21.877724666119,0.));
#205544=CARTESIAN_POINT('Ctrl Pts',(-11.0794459793057,21.877724666119,12.));
#205545=CARTESIAN_POINT('Ctrl Pts',(-11.0613212074363,21.8624698726318,
0.));
#205546=CARTESIAN_POINT('Ctrl Pts',(-11.0613212074363,21.8624698726318,
12.));
#205547=CARTESIAN_POINT('Ctrl Pts',(-11.0433016640807,21.8472274713103,
0.));
#205548=CARTESIAN_POINT('Ctrl Pts',(-11.0433016640807,21.8472274713103,
12.));
#205549=CARTESIAN_POINT('Ctrl Pts',(-11.0253875994598,21.8319980886033,
0.));
#205550=CARTESIAN_POINT('Ctrl Pts',(-11.0253875994598,21.8319980886033,
12.));
#205551=CARTESIAN_POINT('Ctrl Pts',(-11.0075792647477,21.8167823571168,
0.));
#205552=CARTESIAN_POINT('Ctrl Pts',(-11.0075792647477,21.8167823571168,
12.));
#205553=CARTESIAN_POINT('Ctrl Pts',(-10.9898769120912,21.8015809157301,
0.));
#205554=CARTESIAN_POINT('Ctrl Pts',(-10.9898769120912,21.8015809157301,
12.));
#205555=CARTESIAN_POINT('Ctrl Pts',(-10.9722807946156,21.7863944097141,
0.));
#205556=CARTESIAN_POINT('Ctrl Pts',(-10.9722807946156,21.7863944097141,
12.));
#205557=CARTESIAN_POINT('Ctrl Pts',(-10.9547911664455,21.7712234908464,
0.));
#205558=CARTESIAN_POINT('Ctrl Pts',(-10.9547911664455,21.7712234908464,
12.));
#205559=CARTESIAN_POINT('Ctrl Pts',(-10.9374082827444,21.7560688175247,
0.));
#205560=CARTESIAN_POINT('Ctrl Pts',(-10.9374082827444,21.7560688175247,
12.));
#205561=CARTESIAN_POINT('Ctrl Pts',(-10.9201323997384,21.7409310548797,
0.));
#205562=CARTESIAN_POINT('Ctrl Pts',(-10.9201323997384,21.7409310548797,
12.));
#205563=CARTESIAN_POINT('Ctrl Pts',(-10.902963774734,21.7258108748873,0.));
#205564=CARTESIAN_POINT('Ctrl Pts',(-10.902963774734,21.7258108748873,12.));
#205565=CARTESIAN_POINT('Ctrl Pts',(-10.8859026661293,21.7107089564825,
0.));
#205566=CARTESIAN_POINT('Ctrl Pts',(-10.8859026661293,21.7107089564825,
12.));
#205567=CARTESIAN_POINT('Ctrl Pts',(-10.8689493334095,21.6956259856672,
0.));
#205568=CARTESIAN_POINT('Ctrl Pts',(-10.8689493334095,21.6956259856672,
12.));
#205569=CARTESIAN_POINT('Ctrl Pts',(-10.8521040371835,21.6805626556467,
0.));
#205570=CARTESIAN_POINT('Ctrl Pts',(-10.8521040371835,21.6805626556467,
12.));
#205571=CARTESIAN_POINT('Ctrl Pts',(-10.8353670392272,21.6655196669732,
0.));
#205572=CARTESIAN_POINT('Ctrl Pts',(-10.8353670392272,21.6655196669732,
12.));
#205573=CARTESIAN_POINT('Ctrl Pts',(-10.8187386025136,21.6504977276866,
0.));
#205574=CARTESIAN_POINT('Ctrl Pts',(-10.8187386025136,21.6504977276866,
12.));
#205575=CARTESIAN_POINT('Ctrl Pts',(-10.8022189912369,21.6354975534557,
0.));
#205576=CARTESIAN_POINT('Ctrl Pts',(-10.8022189912369,21.6354975534557,
12.));
#205577=CARTESIAN_POINT('Ctrl Pts',(-10.7858084708261,21.6205198677173,
0.));
#205578=CARTESIAN_POINT('Ctrl Pts',(-10.7858084708261,21.6205198677173,
12.));
#205579=CARTESIAN_POINT('Ctrl Pts',(-10.7695073079552,21.6055654018176,
0.));
#205580=CARTESIAN_POINT('Ctrl Pts',(-10.7695073079552,21.6055654018176,
12.));
#205581=CARTESIAN_POINT('Ctrl Pts',(-10.7533157705941,21.5906348951743,
0.));
#205582=CARTESIAN_POINT('Ctrl Pts',(-10.7533157705941,21.5906348951743,
12.));
#205583=CARTESIAN_POINT('Ctrl Pts',(-10.7372341280467,21.5757290954371,
0.));
#205584=CARTESIAN_POINT('Ctrl Pts',(-10.7372341280467,21.5757290954371,
12.));
#205585=CARTESIAN_POINT('Ctrl Pts',(-10.7212626509816,21.5608487586468,
0.));
#205586=CARTESIAN_POINT('Ctrl Pts',(-10.7212626509816,21.5608487586468,
12.));
#205587=CARTESIAN_POINT('Ctrl Pts',(-10.7054016114571,21.5459946493955,
0.));
#205588=CARTESIAN_POINT('Ctrl Pts',(-10.7054016114571,21.5459946493955,
12.));
#205589=CARTESIAN_POINT('Ctrl Pts',(-10.689651282929,21.5311675409807,0.));
#205590=CARTESIAN_POINT('Ctrl Pts',(-10.689651282929,21.5311675409807,12.));
#205591=CARTESIAN_POINT('Ctrl Pts',(-10.6740119402834,21.51636821558,0.));
#205592=CARTESIAN_POINT('Ctrl Pts',(-10.6740119402834,21.51636821558,12.));
#205593=CARTESIAN_POINT('Ctrl Pts',(-10.6584838598939,21.5015974644449,
0.));
#205594=CARTESIAN_POINT('Ctrl Pts',(-10.6584838598939,21.5015974644449,
12.));
#205595=CARTESIAN_POINT('Ctrl Pts',(-10.6430673196607,21.4868560880889,
0.));
#205596=CARTESIAN_POINT('Ctrl Pts',(-10.6430673196607,21.4868560880889,
12.));
#205597=CARTESIAN_POINT('Ctrl Pts',(-10.6277625990456,21.4721448964766,
0.));
#205598=CARTESIAN_POINT('Ctrl Pts',(-10.6277625990456,21.4721448964766,
12.));
#205599=CARTESIAN_POINT('Ctrl Pts',(-10.6125699790961,21.4574647092097,
0.));
#205600=CARTESIAN_POINT('Ctrl Pts',(-10.6125699790961,21.4574647092097,
12.));
#205601=CARTESIAN_POINT('Ctrl Pts',(-10.5974897424622,21.4428163557144,
0.));
#205602=CARTESIAN_POINT('Ctrl Pts',(-10.5974897424622,21.4428163557144,
12.));
#205603=CARTESIAN_POINT('Ctrl Pts',(-10.5825221734573,21.4282006754631,
0.));
#205604=CARTESIAN_POINT('Ctrl Pts',(-10.5825221734573,21.4282006754631,
12.));
#205605=CARTESIAN_POINT('Ctrl Pts',(-10.5676675581108,21.4136185181979,
0.));
#205606=CARTESIAN_POINT('Ctrl Pts',(-10.5676675581108,21.4136185181979,
12.));
#205607=CARTESIAN_POINT('Ctrl Pts',(-10.5529261842108,21.3990707441497,
0.));
#205608=CARTESIAN_POINT('Ctrl Pts',(-10.5529261842108,21.3990707441497,
12.));
#205609=CARTESIAN_POINT('Ctrl Pts',(-10.5382983413421,21.3845582242602,
0.));
#205610=CARTESIAN_POINT('Ctrl Pts',(-10.5382983413421,21.3845582242602,
12.));
#205611=CARTESIAN_POINT('Ctrl Pts',(-10.5237843209057,21.3700818403936,
0.));
#205612=CARTESIAN_POINT('Ctrl Pts',(-10.5237843209057,21.3700818403936,
12.));
#205613=CARTESIAN_POINT('Ctrl Pts',(-10.5093844161685,21.3556424855814,
0.));
#205614=CARTESIAN_POINT('Ctrl Pts',(-10.5093844161685,21.3556424855814,
12.));
#205615=CARTESIAN_POINT('Ctrl Pts',(-10.4950989223337,21.3412410642904,
0.));
#205616=CARTESIAN_POINT('Ctrl Pts',(-10.4950989223337,21.3412410642904,
12.));
#205617=CARTESIAN_POINT('Ctrl Pts',(-10.4809281365931,21.3268784926819,
0.));
#205618=CARTESIAN_POINT('Ctrl Pts',(-10.4809281365931,21.3268784926819,
12.));
#205619=CARTESIAN_POINT('Ctrl Pts',(-10.4668723581768,21.3125556988731,
0.));
#205620=CARTESIAN_POINT('Ctrl Pts',(-10.4668723581768,21.3125556988731,
12.));
#205621=CARTESIAN_POINT('Ctrl Pts',(-10.4529318883874,21.2982736231931,
0.));
#205622=CARTESIAN_POINT('Ctrl Pts',(-10.4529318883874,21.2982736231931,
12.));
#205623=CARTESIAN_POINT('Ctrl Pts',(-10.4391070306391,21.2840332184483,
0.));
#205624=CARTESIAN_POINT('Ctrl Pts',(-10.4391070306391,21.2840332184483,
12.));
#205625=CARTESIAN_POINT('Ctrl Pts',(-10.42539809054,21.2698354502403,0.));
#205626=CARTESIAN_POINT('Ctrl Pts',(-10.42539809054,21.2698354502403,12.));
#205627=CARTESIAN_POINT('Ctrl Pts',(-10.4118053759588,21.255681297275,0.));
#205628=CARTESIAN_POINT('Ctrl Pts',(-10.4118053759588,21.255681297275,12.));
#205629=CARTESIAN_POINT('Ctrl Pts',(-10.3983291970846,21.2415717516714,
0.));
#205630=CARTESIAN_POINT('Ctrl Pts',(-10.3983291970846,21.2415717516714,
12.));
#205631=CARTESIAN_POINT('Ctrl Pts',(-10.3849698664786,21.22750781927,0.));
#205632=CARTESIAN_POINT('Ctrl Pts',(-10.3849698664786,21.22750781927,12.));
#205633=CARTESIAN_POINT('Ctrl Pts',(-10.371727699113,21.2134905199345,0.));
#205634=CARTESIAN_POINT('Ctrl Pts',(-10.371727699113,21.2134905199345,12.));
#205635=CARTESIAN_POINT('Ctrl Pts',(-10.3586030124587,21.199520887919,0.));
#205636=CARTESIAN_POINT('Ctrl Pts',(-10.3586030124587,21.199520887919,12.));
#205637=CARTESIAN_POINT('Ctrl Pts',(-10.3455961265701,21.1855999722416,
0.));
#205638=CARTESIAN_POINT('Ctrl Pts',(-10.3455961265701,21.1855999722416,
12.));
#205639=CARTESIAN_POINT('Ctrl Pts',(-10.3327073641572,21.1717288370509,
0.));
#205640=CARTESIAN_POINT('Ctrl Pts',(-10.3327073641572,21.1717288370509,
12.));
#205641=CARTESIAN_POINT('Ctrl Pts',(-10.3199370506544,21.1579085619965,
0.));
#205642=CARTESIAN_POINT('Ctrl Pts',(-10.3199370506544,21.1579085619965,
12.));
#205643=CARTESIAN_POINT('Ctrl Pts',(-10.3072855142687,21.1441402425843,
0.));
#205644=CARTESIAN_POINT('Ctrl Pts',(-10.3072855142687,21.1441402425843,
12.));
#205645=CARTESIAN_POINT('Ctrl Pts',(-10.2947530860721,21.1304249906002,
0.));
#205646=CARTESIAN_POINT('Ctrl Pts',(-10.2947530860721,21.1304249906002,
12.));
#205647=CARTESIAN_POINT('Ctrl Pts',(-10.2823401001072,21.1167639345631,
0.));
#205648=CARTESIAN_POINT('Ctrl Pts',(-10.2823401001072,21.1167639345631,
12.));
#205649=CARTESIAN_POINT('Ctrl Pts',(-10.2700468934744,21.1031582201627,
0.));
#205650=CARTESIAN_POINT('Ctrl Pts',(-10.2700468934744,21.1031582201627,
12.));
#205651=CARTESIAN_POINT('Ctrl Pts',(-10.2578738064181,21.0896090107063,
0.));
#205652=CARTESIAN_POINT('Ctrl Pts',(-10.2578738064181,21.0896090107063,
12.));
#205653=CARTESIAN_POINT('Ctrl Pts',(-10.2458211823912,21.0761174875445,
0.));
#205654=CARTESIAN_POINT('Ctrl Pts',(-10.2458211823912,21.0761174875445,
12.));
#205655=CARTESIAN_POINT('Ctrl Pts',(-10.2338893681567,21.0626848505663,
0.));
#205656=CARTESIAN_POINT('Ctrl Pts',(-10.2338893681567,21.0626848505663,
12.));
#205657=CARTESIAN_POINT('Ctrl Pts',(-10.2220787139155,21.0493123187483,
0.));
#205658=CARTESIAN_POINT('Ctrl Pts',(-10.2220787139155,21.0493123187483,
12.));
#205659=CARTESIAN_POINT('Ctrl Pts',(-10.2103895734123,21.0360011306815,
0.));
#205660=CARTESIAN_POINT('Ctrl Pts',(-10.2103895734123,21.0360011306815,
12.));
#205661=CARTESIAN_POINT('Ctrl Pts',(-10.1988223040425,21.0227525451107,
0.));
#205662=CARTESIAN_POINT('Ctrl Pts',(-10.1988223040425,21.0227525451107,
12.));
#205663=CARTESIAN_POINT('Ctrl Pts',(-10.187377266936,21.0095678414486,0.));
#205664=CARTESIAN_POINT('Ctrl Pts',(-10.187377266936,21.0095678414486,12.));
#205665=CARTESIAN_POINT('Ctrl Pts',(-10.1760548270767,20.9964483203686,
0.));
#205666=CARTESIAN_POINT('Ctrl Pts',(-10.1760548270767,20.9964483203686,
12.));
#205667=CARTESIAN_POINT('Ctrl Pts',(-10.1648553534568,20.9833953044736,
0.));
#205668=CARTESIAN_POINT('Ctrl Pts',(-10.1648553534568,20.9833953044736,
12.));
#205669=CARTESIAN_POINT('Ctrl Pts',(-10.1537792192065,20.9704101389369,
0.));
#205670=CARTESIAN_POINT('Ctrl Pts',(-10.1537792192065,20.9704101389369,
12.));
#205671=CARTESIAN_POINT('Ctrl Pts',(-10.1428268017256,20.9574941921591,
0.));
#205672=CARTESIAN_POINT('Ctrl Pts',(-10.1428268017256,20.9574941921591,
12.));
#205673=CARTESIAN_POINT('Ctrl Pts',(-10.1319984827908,20.9446488563933,
0.));
#205674=CARTESIAN_POINT('Ctrl Pts',(-10.1319984827908,20.9446488563933,
12.));
#205675=CARTESIAN_POINT('Ctrl Pts',(-10.1212946487057,20.9318755484734,
0.));
#205676=CARTESIAN_POINT('Ctrl Pts',(-10.1212946487057,20.9318755484734,
12.));
#205677=CARTESIAN_POINT('Ctrl Pts',(-10.1107156904836,20.919175710627,0.));
#205678=CARTESIAN_POINT('Ctrl Pts',(-10.1107156904836,20.919175710627,12.));
#205679=CARTESIAN_POINT('Ctrl Pts',(-10.1002620040076,20.9065508112557,
0.));
#205680=CARTESIAN_POINT('Ctrl Pts',(-10.1002620040076,20.9065508112557,
12.));
#205681=CARTESIAN_POINT('Ctrl Pts',(-10.0899339901916,20.894002345737,0.));
#205682=CARTESIAN_POINT('Ctrl Pts',(-10.0899339901916,20.894002345737,12.));
#205683=CARTESIAN_POINT('Ctrl Pts',(-10.0797320551154,20.881531837184,0.));
#205684=CARTESIAN_POINT('Ctrl Pts',(-10.0797320551154,20.881531837184,12.));
#205685=CARTESIAN_POINT('Ctrl Pts',(-10.0696566102218,20.86914083737,0.));
#205686=CARTESIAN_POINT('Ctrl Pts',(-10.0696566102218,20.86914083737,12.));
#205687=CARTESIAN_POINT('Ctrl Pts',(-10.0597080725375,20.8568309277316,
0.));
#205688=CARTESIAN_POINT('Ctrl Pts',(-10.0597080725375,20.8568309277316,
12.));
#205689=CARTESIAN_POINT('Ctrl Pts',(-10.0498868648733,20.8446037203402,
0.));
#205690=CARTESIAN_POINT('Ctrl Pts',(-10.0498868648733,20.8446037203402,
12.));
#205691=CARTESIAN_POINT('Ctrl Pts',(-10.0401934160234,20.8324608588909,
0.));
#205692=CARTESIAN_POINT('Ctrl Pts',(-10.0401934160234,20.8324608588909,
12.));
#205693=CARTESIAN_POINT('Ctrl Pts',(-10.0306281609435,20.8204040196602,
0.));
#205694=CARTESIAN_POINT('Ctrl Pts',(-10.0306281609435,20.8204040196602,
12.));
#205695=CARTESIAN_POINT('Ctrl Pts',(-10.0211915410095,20.8084349126888,
0.));
#205696=CARTESIAN_POINT('Ctrl Pts',(-10.0211915410095,20.8084349126888,
12.));
#205697=CARTESIAN_POINT('Ctrl Pts',(-10.0118840042786,20.7965552829908,
0.));
#205698=CARTESIAN_POINT('Ctrl Pts',(-10.0118840042786,20.7965552829908,
12.));
#205699=CARTESIAN_POINT('Ctrl Pts',(-10.0027060057389,20.7847669117568,
0.));
#205700=CARTESIAN_POINT('Ctrl Pts',(-10.0027060057389,20.7847669117568,
12.));
#205701=CARTESIAN_POINT('Ctrl Pts',(-9.9936580075464,20.7730716175417,0.));
#205702=CARTESIAN_POINT('Ctrl Pts',(-9.9936580075464,20.7730716175417,12.));
#205703=CARTESIAN_POINT('Ctrl Pts',(-9.98474047926852,20.761471257499,0.));
#205704=CARTESIAN_POINT('Ctrl Pts',(-9.98474047926852,20.761471257499,12.));
#205705=CARTESIAN_POINT('Ctrl Pts',(-9.9759538982347,20.7499677289627,0.));
#205706=CARTESIAN_POINT('Ctrl Pts',(-9.9759538982347,20.7499677289627,12.));
#205707=CARTESIAN_POINT('Ctrl Pts',(-9.96729874986202,20.7385629709795,
0.));
#205708=CARTESIAN_POINT('Ctrl Pts',(-9.96729874986202,20.7385629709795,
12.));
#205709=CARTESIAN_POINT('Ctrl Pts',(-9.95877552798398,20.7272589658751,
0.));
#205710=CARTESIAN_POINT('Ctrl Pts',(-9.95877552798398,20.7272589658751,
12.));
#205711=CARTESIAN_POINT('Ctrl Pts',(-9.95038473514949,20.7160577407579,
0.));
#205712=CARTESIAN_POINT('Ctrl Pts',(-9.95038473514949,20.7160577407579,
12.));
#205713=CARTESIAN_POINT('Ctrl Pts',(-9.94212688298236,20.7049613692234,
0.));
#205714=CARTESIAN_POINT('Ctrl Pts',(-9.94212688298236,20.7049613692234,
12.));
#205715=CARTESIAN_POINT('Ctrl Pts',(-9.9340024925973,20.6939719732484,0.));
#205716=CARTESIAN_POINT('Ctrl Pts',(-9.9340024925973,20.6939719732484,12.));
#205717=CARTESIAN_POINT('Ctrl Pts',(-9.92601209498749,20.6830917250255,
0.));
#205718=CARTESIAN_POINT('Ctrl Pts',(-9.92601209498749,20.6830917250255,
12.));
#205719=CARTESIAN_POINT('Ctrl Pts',(-9.91815623141289,20.6723228488263,
0.));
#205720=CARTESIAN_POINT('Ctrl Pts',(-9.91815623141289,20.6723228488263,
12.));
#205721=CARTESIAN_POINT('Ctrl Pts',(-9.91043545377007,20.6616676228315,
0.));
#205722=CARTESIAN_POINT('Ctrl Pts',(-9.91043545377007,20.6616676228315,
12.));
#205723=CARTESIAN_POINT('Ctrl Pts',(-9.90285032516693,20.6511283817414,
0.));
#205724=CARTESIAN_POINT('Ctrl Pts',(-9.90285032516693,20.6511283817414,
12.));
#205725=CARTESIAN_POINT('Ctrl Pts',(-9.8954014204912,20.6407075193976,0.));
#205726=CARTESIAN_POINT('Ctrl Pts',(-9.8954014204912,20.6407075193976,12.));
#205727=CARTESIAN_POINT('Ctrl Pts',(-9.88808932697306,20.6304074914087,
0.));
#205728=CARTESIAN_POINT('Ctrl Pts',(-9.88808932697306,20.6304074914087,
12.));
#205729=CARTESIAN_POINT('Ctrl Pts',(-9.88091464472676,20.6202308177474,
0.));
#205730=CARTESIAN_POINT('Ctrl Pts',(-9.88091464472676,20.6202308177474,
12.));
#205731=CARTESIAN_POINT('Ctrl Pts',(-9.87387798732956,20.6101800854494,
0.));
#205732=CARTESIAN_POINT('Ctrl Pts',(-9.87387798732956,20.6101800854494,
12.));
#205733=CARTESIAN_POINT('Ctrl Pts',(-9.86697998242623,20.6002579513699,
0.));
#205734=CARTESIAN_POINT('Ctrl Pts',(-9.86697998242623,20.6002579513699,
12.));
#205735=CARTESIAN_POINT('Ctrl Pts',(-9.86022127232748,20.5904671449754,
0.));
#205736=CARTESIAN_POINT('Ctrl Pts',(-9.86022127232748,20.5904671449754,
12.));
#205737=CARTESIAN_POINT('Ctrl Pts',(-9.85360251456981,20.5808104710015,
0.));
#205738=CARTESIAN_POINT('Ctrl Pts',(-9.85360251456981,20.5808104710015,
12.));
#205739=CARTESIAN_POINT('Ctrl Pts',(-9.84712438256278,20.5712908125139,
0.));
#205740=CARTESIAN_POINT('Ctrl Pts',(-9.84712438256278,20.5712908125139,
12.));
#205741=CARTESIAN_POINT('Ctrl Pts',(-9.84078756677565,20.5619111362402,
0.));
#205742=CARTESIAN_POINT('Ctrl Pts',(-9.84078756677565,20.5619111362402,
12.));
#205743=CARTESIAN_POINT('Ctrl Pts',(-9.83459277585315,20.552674497646,0.));
#205744=CARTESIAN_POINT('Ctrl Pts',(-9.83459277585315,20.552674497646,12.));
#205745=CARTESIAN_POINT('Ctrl Pts',(-9.82854073773877,20.5435840460721,
0.));
#205746=CARTESIAN_POINT('Ctrl Pts',(-9.82854073773877,20.5435840460721,
12.));
#205747=CARTESIAN_POINT('Ctrl Pts',(-9.82263220080363,20.5346430299517,
0.));
#205748=CARTESIAN_POINT('Ctrl Pts',(-9.82263220080363,20.5346430299517,
12.));
#205749=CARTESIAN_POINT('Ctrl Pts',(-9.81686793455943,20.5258548000629,
0.));
#205750=CARTESIAN_POINT('Ctrl Pts',(-9.81686793455943,20.5258548000629,
12.));
#205751=CARTESIAN_POINT('Ctrl Pts',(-9.81124873025282,20.517222812284,0.));
#205752=CARTESIAN_POINT('Ctrl Pts',(-9.81124873025282,20.517222812284,12.));
#205753=CARTESIAN_POINT('Ctrl Pts',(-9.80577540161088,20.5087506310505,
0.));
#205754=CARTESIAN_POINT('Ctrl Pts',(-9.80577540161088,20.5087506310505,
12.));
#205755=CARTESIAN_POINT('Ctrl Pts',(-9.80044878520949,20.5004419312107,
0.));
#205756=CARTESIAN_POINT('Ctrl Pts',(-9.80044878520949,20.5004419312107,
12.));
#205757=CARTESIAN_POINT('Ctrl Pts',(-9.79526974288331,20.4923005087943,
0.));
#205758=CARTESIAN_POINT('Ctrl Pts',(-9.79526974288331,20.4923005087943,
12.));
#205759=CARTESIAN_POINT('Ctrl Pts',(-9.79023916498656,20.4843302955329,
0.));
#205760=CARTESIAN_POINT('Ctrl Pts',(-9.79023916498656,20.4843302955329,
12.));
#205761=CARTESIAN_POINT('Ctrl Pts',(-9.78535797314167,20.4765353711586,
0.));
#205762=CARTESIAN_POINT('Ctrl Pts',(-9.78535797314167,20.4765353711586,
12.));
#205763=CARTESIAN_POINT('Ctrl Pts',(-9.78062712373321,20.4689199790669,
0.));
#205764=CARTESIAN_POINT('Ctrl Pts',(-9.78062712373321,20.4689199790669,
12.));
#205765=CARTESIAN_POINT('Ctrl Pts',(-9.77604760815529,20.4614885274975,
0.));
#205766=CARTESIAN_POINT('Ctrl Pts',(-9.77604760815529,20.4614885274975,
12.));
#205767=CARTESIAN_POINT('Ctrl Pts',(-9.7716204510407,20.4542455817527,0.));
#205768=CARTESIAN_POINT('Ctrl Pts',(-9.7716204510407,20.4542455817527,12.));
#205769=CARTESIAN_POINT('Ctrl Pts',(-9.76734670980892,20.447195862298,0.));
#205770=CARTESIAN_POINT('Ctrl Pts',(-9.76734670980892,20.447195862298,12.));
#205771=CARTESIAN_POINT('Ctrl Pts',(-9.76322747195495,20.44034423294,0.));
#205772=CARTESIAN_POINT('Ctrl Pts',(-9.76322747195495,20.44034423294,12.));
#205773=CARTESIAN_POINT('Ctrl Pts',(-9.75926386289923,20.4336957355473,
0.));
#205774=CARTESIAN_POINT('Ctrl Pts',(-9.75926386289923,20.4336957355473,
12.));
#205775=CARTESIAN_POINT('Ctrl Pts',(-9.75545705902418,20.4272556476629,
0.));
#205776=CARTESIAN_POINT('Ctrl Pts',(-9.75545705902418,20.4272556476629,
12.));
#205777=CARTESIAN_POINT('Ctrl Pts',(-9.7518082978643,20.4210295275817,0.));
#205778=CARTESIAN_POINT('Ctrl Pts',(-9.7518082978643,20.4210295275817,12.));
#205779=CARTESIAN_POINT('Ctrl Pts',(-9.74831889242174,20.4150232777393,
0.));
#205780=CARTESIAN_POINT('Ctrl Pts',(-9.74831889242174,20.4150232777393,
12.));
#205781=CARTESIAN_POINT('Ctrl Pts',(-9.74499021838538,20.4092430879861,
0.));
#205782=CARTESIAN_POINT('Ctrl Pts',(-9.74499021838538,20.4092430879861,
12.));
#205783=CARTESIAN_POINT('Ctrl Pts',(-9.74182369656272,20.4036953576549,
0.));
#205784=CARTESIAN_POINT('Ctrl Pts',(-9.74182369656272,20.4036953576549,
12.));
#205785=CARTESIAN_POINT('Ctrl Pts',(-9.73882077613201,20.3983866213331,
0.));
#205786=CARTESIAN_POINT('Ctrl Pts',(-9.73882077613201,20.3983866213331,
12.));
#205787=CARTESIAN_POINT('Ctrl Pts',(-9.73598292014243,20.3933234845647,
0.));
#205788=CARTESIAN_POINT('Ctrl Pts',(-9.73598292014243,20.3933234845647,
12.));
#205789=CARTESIAN_POINT('Ctrl Pts',(-9.73331167102808,20.3885129129912,
0.));
#205790=CARTESIAN_POINT('Ctrl Pts',(-9.73331167102808,20.3885129129912,
12.));
#205791=CARTESIAN_POINT('Ctrl Pts',(-9.73080870123727,20.3839624556742,
0.));
#205792=CARTESIAN_POINT('Ctrl Pts',(-9.73080870123727,20.3839624556742,
12.));
#205793=CARTESIAN_POINT('Ctrl Pts',(-9.72847589116542,20.3796805893304,
0.));
#205794=CARTESIAN_POINT('Ctrl Pts',(-9.72847589116542,20.3796805893304,
12.));
#205795=CARTESIAN_POINT('Ctrl Pts',(-9.7263153173288,20.3756766651951,0.));
#205796=CARTESIAN_POINT('Ctrl Pts',(-9.7263153173288,20.3756766651951,12.));
#205797=CARTESIAN_POINT('Ctrl Pts',(-9.72432910043194,20.371960235676,0.));
#205798=CARTESIAN_POINT('Ctrl Pts',(-9.72432910043194,20.371960235676,12.));
#205799=CARTESIAN_POINT('Ctrl Pts',(-9.7225193072249,20.3685406190576,0.));
#205800=CARTESIAN_POINT('Ctrl Pts',(-9.7225193072249,20.3685406190576,12.));
#205801=CARTESIAN_POINT('Ctrl Pts',(-9.72088778381081,20.3654261611056,
0.));
#205802=CARTESIAN_POINT('Ctrl Pts',(-9.72088778381081,20.3654261611056,
12.));
#205803=CARTESIAN_POINT('Ctrl Pts',(-9.71943648548099,20.3626256913981,
0.));
#205804=CARTESIAN_POINT('Ctrl Pts',(-9.71943648548099,20.3626256913981,
12.));
#205805=CARTESIAN_POINT('Ctrl Pts',(-9.71816778328006,20.3601498764344,
0.));
#205806=CARTESIAN_POINT('Ctrl Pts',(-9.71816778328006,20.3601498764344,
12.));
#205807=CARTESIAN_POINT('Ctrl Pts',(-9.71708493723096,20.3580133103356,
0.));
#205808=CARTESIAN_POINT('Ctrl Pts',(-9.71708493723096,20.3580133103356,
12.));
#205809=CARTESIAN_POINT('Ctrl Pts',(-9.71619192554186,20.3562337557875,
0.));
#205810=CARTESIAN_POINT('Ctrl Pts',(-9.71619192554186,20.3562337557875,
12.));
#205811=CARTESIAN_POINT('Ctrl Pts',(-9.71549257088172,20.3548282742361,
0.));
#205812=CARTESIAN_POINT('Ctrl Pts',(-9.71549257088172,20.3548282742361,
12.));
#205813=CARTESIAN_POINT('Ctrl Pts',(-9.71498978052021,20.3538098605706,
0.));
#205814=CARTESIAN_POINT('Ctrl Pts',(-9.71498978052021,20.3538098605706,
12.));
#205815=CARTESIAN_POINT('Ctrl Pts',(-9.71474590350681,20.3533097561886,
0.));
#205816=CARTESIAN_POINT('Ctrl Pts',(-9.71474590350681,20.3533097561886,
12.));
#205817=CARTESIAN_POINT('Ctrl Pts',(-9.71465227853041,20.3531126095522,
0.));
#205818=CARTESIAN_POINT('Ctrl Pts',(-9.71465227853041,20.3531126095522,
12.));
#205819=CARTESIAN_POINT('Ctrl Pts',(-9.71462954053042,20.353060251684,0.));
#205820=CARTESIAN_POINT('Ctrl Pts',(-9.71462954053042,20.353060251684,12.));
#205821=CARTESIAN_POINT('Ctrl Pts',(-9.71462809124916,20.353053841303,0.));
#205822=CARTESIAN_POINT('Ctrl Pts',(-9.71462809124916,20.353053841303,12.));
#205823=CARTESIAN_POINT('',(-12.4230808101438,22.8400320311648,0.));
#205824=CARTESIAN_POINT('Ctrl Pts',(-12.4230808101438,22.8400320311648,
0.));
#205825=CARTESIAN_POINT('Ctrl Pts',(-12.418215285186,22.8370364396459,0.));
#205826=CARTESIAN_POINT('Ctrl Pts',(-12.4084933766347,22.8310435872747,
0.));
#205827=CARTESIAN_POINT('Ctrl Pts',(-12.3939379378998,22.8220493007173,
0.));
#205828=CARTESIAN_POINT('Ctrl Pts',(-12.374585536673,22.81004690224,0.));
#205829=CARTESIAN_POINT('Ctrl Pts',(-12.3504864740319,22.795027221673,0.));
#205830=CARTESIAN_POINT('Ctrl Pts',(-12.3264788926075,22.7799908974768,
0.));
#205831=CARTESIAN_POINT('Ctrl Pts',(-12.3025628601792,22.764938010105,0.));
#205832=CARTESIAN_POINT('Ctrl Pts',(-12.2787384750742,22.7498686970069,
0.));
#205833=CARTESIAN_POINT('Ctrl Pts',(-12.2550058702395,22.7347831655287,
0.));
#205834=CARTESIAN_POINT('Ctrl Pts',(-12.2313652198061,22.7196817119374,
0.));
#205835=CARTESIAN_POINT('Ctrl Pts',(-12.2078167360284,22.7045647168747,
0.));
#205836=CARTESIAN_POINT('Ctrl Pts',(-12.1843606579262,22.6894326205037,
0.));
#205837=CARTESIAN_POINT('Ctrl Pts',(-12.1609972423099,22.6742859034944,
0.));
#205838=CARTESIAN_POINT('Ctrl Pts',(-12.1377267537145,22.6591250653965,
0.));
#205839=CARTESIAN_POINT('Ctrl Pts',(-12.1145494550383,22.6439506046605,
0.));
#205840=CARTESIAN_POINT('Ctrl Pts',(-12.0914655972823,22.6287629967056,
0.));
#205841=CARTESIAN_POINT('Ctrl Pts',(-12.0684754113862,22.6135626764898,
0.));
#205842=CARTESIAN_POINT('Ctrl Pts',(-12.0455791139128,22.5983500505644,
0.));
#205843=CARTESIAN_POINT('Ctrl Pts',(-12.0227769113127,22.5831255061282,
0.));
#205844=CARTESIAN_POINT('Ctrl Pts',(-12.0000690046695,22.5678894211181,
0.));
#205845=CARTESIAN_POINT('Ctrl Pts',(-11.9774555943496,22.5526421741158,
0.));
#205846=CARTESIAN_POINT('Ctrl Pts',(-11.9549368843997,22.5373841537307,
0.));
#205847=CARTESIAN_POINT('Ctrl Pts',(-11.9325130877803,22.5221157697883,
0.));
#205848=CARTESIAN_POINT('Ctrl Pts',(-11.9101844254557,22.5068374513973,
0.));
#205849=CARTESIAN_POINT('Ctrl Pts',(-11.8879511239943,22.4915496418485,
0.));
#205850=CARTESIAN_POINT('Ctrl Pts',(-11.8658134137019,22.4762527946702,
0.));
#205851=CARTESIAN_POINT('Ctrl Pts',(-11.8437715264487,22.4609473690471,
0.));
#205852=CARTESIAN_POINT('Ctrl Pts',(-11.8218256937889,22.4456338258735,
0.));
#205853=CARTESIAN_POINT('Ctrl Pts',(-11.7999761445173,22.430312622646,0.));
#205854=CARTESIAN_POINT('Ctrl Pts',(-11.7782231042039,22.4149842125008,
0.));
#205855=CARTESIAN_POINT('Ctrl Pts',(-11.7565667964764,22.3996490469191,
0.));
#205856=CARTESIAN_POINT('Ctrl Pts',(-11.7350074437961,22.3843075773899,
0.));
#205857=CARTESIAN_POINT('Ctrl Pts',(-11.7135452684532,22.3689602575491,
0.));
#205858=CARTESIAN_POINT('Ctrl Pts',(-11.6921804934056,22.3536075450029,
0.));
#205859=CARTESIAN_POINT('Ctrl Pts',(-11.6709133432985,22.3382499035619,
0.));
#205860=CARTESIAN_POINT('Ctrl Pts',(-11.6497440449857,22.3228878043976,
0.));
#205861=CARTESIAN_POINT('Ctrl Pts',(-11.6286728270009,22.3075217249049,
0.));
#205862=CARTESIAN_POINT('Ctrl Pts',(-11.6076999192357,22.2921521480356,
0.));
#205863=CARTESIAN_POINT('Ctrl Pts',(-11.5868255525188,22.2767795614348,
0.));
#205864=CARTESIAN_POINT('Ctrl Pts',(-11.5660499582403,22.2614044566898,
0.));
#205865=CARTESIAN_POINT('Ctrl Pts',(-11.5453733679121,22.2460273284654,
0.));
#205866=CARTESIAN_POINT('Ctrl Pts',(-11.5247960128477,22.2306486738901,
0.));
#205867=CARTESIAN_POINT('Ctrl Pts',(-11.5043181244242,22.2152689931022,
0.));
#205868=CARTESIAN_POINT('Ctrl Pts',(-11.483939934259,22.1998887896436,0.));
#205869=CARTESIAN_POINT('Ctrl Pts',(-11.463661674411,22.184508570917,0.));
#205870=CARTESIAN_POINT('Ctrl Pts',(-11.443483577557,22.1691288486096,0.));
#205871=CARTESIAN_POINT('Ctrl Pts',(-11.4234058771742,22.1537501391487,
0.));
#205872=CARTESIAN_POINT('Ctrl Pts',(-11.4034288076908,22.1383729640964,
0.));
#205873=CARTESIAN_POINT('Ctrl Pts',(-11.3835526044256,22.1229978500186,
0.));
#205874=CARTESIAN_POINT('Ctrl Pts',(-11.3637775035367,22.1076253283979,
0.));
#205875=CARTESIAN_POINT('Ctrl Pts',(-11.3441037419553,22.0922559355294,
0.));
#205876=CARTESIAN_POINT('Ctrl Pts',(-11.3245315573168,22.0768902124267,
0.));
#205877=CARTESIAN_POINT('Ctrl Pts',(-11.3050611878771,22.0615287047179,
0.));
#205878=CARTESIAN_POINT('Ctrl Pts',(-11.2856928724374,22.046171962566,0.));
#205879=CARTESIAN_POINT('Ctrl Pts',(-11.2664268504206,22.030820540835,0.));
#205880=CARTESIAN_POINT('Ctrl Pts',(-11.2472633619275,22.0154749992363,
0.));
#205881=CARTESIAN_POINT('Ctrl Pts',(-11.2282026477896,22.0001359024839,
0.));
#205882=CARTESIAN_POINT('Ctrl Pts',(-11.2092449496125,21.9848038204439,
0.));
#205883=CARTESIAN_POINT('Ctrl Pts',(-11.190390509811,21.9694793282914,0.));
#205884=CARTESIAN_POINT('Ctrl Pts',(-11.1716395716376,21.9541630066506,
0.));
#205885=CARTESIAN_POINT('Ctrl Pts',(-11.1529923792003,21.9388554416439,
0.));
#205886=CARTESIAN_POINT('Ctrl Pts',(-11.1344491774741,21.923557224952,0.));
#205887=CARTESIAN_POINT('Ctrl Pts',(-11.1160102123024,21.9082689538688,
0.));
#205888=CARTESIAN_POINT('Ctrl Pts',(-11.0976757303944,21.8929912313608,
0.));
#205889=CARTESIAN_POINT('Ctrl Pts',(-11.0794459793057,21.877724666119,0.));
#205890=CARTESIAN_POINT('Ctrl Pts',(-11.0613212074363,21.8624698726318,
0.));
#205891=CARTESIAN_POINT('Ctrl Pts',(-11.0433016640807,21.8472274713103,
0.));
#205892=CARTESIAN_POINT('Ctrl Pts',(-11.0253875994598,21.8319980886033,
0.));
#205893=CARTESIAN_POINT('Ctrl Pts',(-11.0075792647477,21.8167823571168,
0.));
#205894=CARTESIAN_POINT('Ctrl Pts',(-10.9898769120912,21.8015809157301,
0.));
#205895=CARTESIAN_POINT('Ctrl Pts',(-10.9722807946156,21.7863944097141,
0.));
#205896=CARTESIAN_POINT('Ctrl Pts',(-10.9547911664455,21.7712234908464,
0.));
#205897=CARTESIAN_POINT('Ctrl Pts',(-10.9374082827444,21.7560688175247,
0.));
#205898=CARTESIAN_POINT('Ctrl Pts',(-10.9201323997384,21.7409310548797,
0.));
#205899=CARTESIAN_POINT('Ctrl Pts',(-10.902963774734,21.7258108748873,0.));
#205900=CARTESIAN_POINT('Ctrl Pts',(-10.8859026661293,21.7107089564825,
0.));
#205901=CARTESIAN_POINT('Ctrl Pts',(-10.8689493334095,21.6956259856672,
0.));
#205902=CARTESIAN_POINT('Ctrl Pts',(-10.8521040371835,21.6805626556467,
0.));
#205903=CARTESIAN_POINT('Ctrl Pts',(-10.8353670392272,21.6655196669732,
0.));
#205904=CARTESIAN_POINT('Ctrl Pts',(-10.8187386025136,21.6504977276866,
0.));
#205905=CARTESIAN_POINT('Ctrl Pts',(-10.8022189912369,21.6354975534557,
0.));
#205906=CARTESIAN_POINT('Ctrl Pts',(-10.7858084708261,21.6205198677173,
0.));
#205907=CARTESIAN_POINT('Ctrl Pts',(-10.7695073079552,21.6055654018176,
0.));
#205908=CARTESIAN_POINT('Ctrl Pts',(-10.7533157705941,21.5906348951743,
0.));
#205909=CARTESIAN_POINT('Ctrl Pts',(-10.7372341280467,21.5757290954371,
0.));
#205910=CARTESIAN_POINT('Ctrl Pts',(-10.7212626509816,21.5608487586468,
0.));
#205911=CARTESIAN_POINT('Ctrl Pts',(-10.7054016114571,21.5459946493955,
0.));
#205912=CARTESIAN_POINT('Ctrl Pts',(-10.689651282929,21.5311675409807,0.));
#205913=CARTESIAN_POINT('Ctrl Pts',(-10.6740119402834,21.51636821558,0.));
#205914=CARTESIAN_POINT('Ctrl Pts',(-10.6584838598939,21.5015974644449,
0.));
#205915=CARTESIAN_POINT('Ctrl Pts',(-10.6430673196607,21.4868560880889,
0.));
#205916=CARTESIAN_POINT('Ctrl Pts',(-10.6277625990456,21.4721448964766,
0.));
#205917=CARTESIAN_POINT('Ctrl Pts',(-10.6125699790961,21.4574647092097,
0.));
#205918=CARTESIAN_POINT('Ctrl Pts',(-10.5974897424622,21.4428163557144,
0.));
#205919=CARTESIAN_POINT('Ctrl Pts',(-10.5825221734573,21.4282006754631,
0.));
#205920=CARTESIAN_POINT('Ctrl Pts',(-10.5676675581108,21.4136185181979,
0.));
#205921=CARTESIAN_POINT('Ctrl Pts',(-10.5529261842108,21.3990707441497,
0.));
#205922=CARTESIAN_POINT('Ctrl Pts',(-10.5382983413421,21.3845582242602,
0.));
#205923=CARTESIAN_POINT('Ctrl Pts',(-10.5237843209057,21.3700818403936,
0.));
#205924=CARTESIAN_POINT('Ctrl Pts',(-10.5093844161685,21.3556424855814,
0.));
#205925=CARTESIAN_POINT('Ctrl Pts',(-10.4950989223337,21.3412410642904,
0.));
#205926=CARTESIAN_POINT('Ctrl Pts',(-10.4809281365931,21.3268784926819,
0.));
#205927=CARTESIAN_POINT('Ctrl Pts',(-10.4668723581768,21.3125556988731,
0.));
#205928=CARTESIAN_POINT('Ctrl Pts',(-10.4529318883874,21.2982736231931,
0.));
#205929=CARTESIAN_POINT('Ctrl Pts',(-10.4391070306391,21.2840332184483,
0.));
#205930=CARTESIAN_POINT('Ctrl Pts',(-10.42539809054,21.2698354502403,0.));
#205931=CARTESIAN_POINT('Ctrl Pts',(-10.4118053759588,21.255681297275,0.));
#205932=CARTESIAN_POINT('Ctrl Pts',(-10.3983291970846,21.2415717516714,
0.));
#205933=CARTESIAN_POINT('Ctrl Pts',(-10.3849698664786,21.22750781927,0.));
#205934=CARTESIAN_POINT('Ctrl Pts',(-10.371727699113,21.2134905199345,0.));
#205935=CARTESIAN_POINT('Ctrl Pts',(-10.3586030124587,21.199520887919,0.));
#205936=CARTESIAN_POINT('Ctrl Pts',(-10.3455961265701,21.1855999722416,
0.));
#205937=CARTESIAN_POINT('Ctrl Pts',(-10.3327073641572,21.1717288370509,
0.));
#205938=CARTESIAN_POINT('Ctrl Pts',(-10.3199370506544,21.1579085619965,
0.));
#205939=CARTESIAN_POINT('Ctrl Pts',(-10.3072855142687,21.1441402425843,
0.));
#205940=CARTESIAN_POINT('Ctrl Pts',(-10.2947530860721,21.1304249906002,
0.));
#205941=CARTESIAN_POINT('Ctrl Pts',(-10.2823401001072,21.1167639345631,
0.));
#205942=CARTESIAN_POINT('Ctrl Pts',(-10.2700468934744,21.1031582201627,
0.));
#205943=CARTESIAN_POINT('Ctrl Pts',(-10.2578738064181,21.0896090107063,
0.));
#205944=CARTESIAN_POINT('Ctrl Pts',(-10.2458211823912,21.0761174875445,
0.));
#205945=CARTESIAN_POINT('Ctrl Pts',(-10.2338893681567,21.0626848505663,
0.));
#205946=CARTESIAN_POINT('Ctrl Pts',(-10.2220787139155,21.0493123187483,
0.));
#205947=CARTESIAN_POINT('Ctrl Pts',(-10.2103895734123,21.0360011306815,
0.));
#205948=CARTESIAN_POINT('Ctrl Pts',(-10.1988223040425,21.0227525451107,
0.));
#205949=CARTESIAN_POINT('Ctrl Pts',(-10.187377266936,21.0095678414486,0.));
#205950=CARTESIAN_POINT('Ctrl Pts',(-10.1760548270767,20.9964483203686,
0.));
#205951=CARTESIAN_POINT('Ctrl Pts',(-10.1648553534568,20.9833953044736,
0.));
#205952=CARTESIAN_POINT('Ctrl Pts',(-10.1537792192065,20.9704101389369,
0.));
#205953=CARTESIAN_POINT('Ctrl Pts',(-10.1428268017256,20.9574941921591,
0.));
#205954=CARTESIAN_POINT('Ctrl Pts',(-10.1319984827908,20.9446488563933,
0.));
#205955=CARTESIAN_POINT('Ctrl Pts',(-10.1212946487057,20.9318755484734,
0.));
#205956=CARTESIAN_POINT('Ctrl Pts',(-10.1107156904836,20.919175710627,0.));
#205957=CARTESIAN_POINT('Ctrl Pts',(-10.1002620040076,20.9065508112557,
0.));
#205958=CARTESIAN_POINT('Ctrl Pts',(-10.0899339901916,20.894002345737,0.));
#205959=CARTESIAN_POINT('Ctrl Pts',(-10.0797320551154,20.881531837184,0.));
#205960=CARTESIAN_POINT('Ctrl Pts',(-10.0696566102218,20.86914083737,0.));
#205961=CARTESIAN_POINT('Ctrl Pts',(-10.0597080725375,20.8568309277316,
0.));
#205962=CARTESIAN_POINT('Ctrl Pts',(-10.0498868648733,20.8446037203402,
0.));
#205963=CARTESIAN_POINT('Ctrl Pts',(-10.0401934160234,20.8324608588909,
0.));
#205964=CARTESIAN_POINT('Ctrl Pts',(-10.0306281609435,20.8204040196602,
0.));
#205965=CARTESIAN_POINT('Ctrl Pts',(-10.0211915410095,20.8084349126888,
0.));
#205966=CARTESIAN_POINT('Ctrl Pts',(-10.0118840042786,20.7965552829908,
0.));
#205967=CARTESIAN_POINT('Ctrl Pts',(-10.0027060057389,20.7847669117568,
0.));
#205968=CARTESIAN_POINT('Ctrl Pts',(-9.9936580075464,20.7730716175417,0.));
#205969=CARTESIAN_POINT('Ctrl Pts',(-9.98474047926852,20.761471257499,0.));
#205970=CARTESIAN_POINT('Ctrl Pts',(-9.9759538982347,20.7499677289627,0.));
#205971=CARTESIAN_POINT('Ctrl Pts',(-9.96729874986202,20.7385629709795,
0.));
#205972=CARTESIAN_POINT('Ctrl Pts',(-9.95877552798398,20.7272589658751,
0.));
#205973=CARTESIAN_POINT('Ctrl Pts',(-9.95038473514949,20.7160577407579,
0.));
#205974=CARTESIAN_POINT('Ctrl Pts',(-9.94212688298236,20.7049613692234,
0.));
#205975=CARTESIAN_POINT('Ctrl Pts',(-9.9340024925973,20.6939719732484,0.));
#205976=CARTESIAN_POINT('Ctrl Pts',(-9.92601209498749,20.6830917250255,
0.));
#205977=CARTESIAN_POINT('Ctrl Pts',(-9.91815623141289,20.6723228488263,
0.));
#205978=CARTESIAN_POINT('Ctrl Pts',(-9.91043545377007,20.6616676228315,
0.));
#205979=CARTESIAN_POINT('Ctrl Pts',(-9.90285032516693,20.6511283817414,
0.));
#205980=CARTESIAN_POINT('Ctrl Pts',(-9.8954014204912,20.6407075193976,0.));
#205981=CARTESIAN_POINT('Ctrl Pts',(-9.88808932697306,20.6304074914087,
0.));
#205982=CARTESIAN_POINT('Ctrl Pts',(-9.88091464472676,20.6202308177474,
0.));
#205983=CARTESIAN_POINT('Ctrl Pts',(-9.87387798732956,20.6101800854494,
0.));
#205984=CARTESIAN_POINT('Ctrl Pts',(-9.86697998242623,20.6002579513699,
0.));
#205985=CARTESIAN_POINT('Ctrl Pts',(-9.86022127232748,20.5904671449754,
0.));
#205986=CARTESIAN_POINT('Ctrl Pts',(-9.85360251456981,20.5808104710015,
0.));
#205987=CARTESIAN_POINT('Ctrl Pts',(-9.84712438256278,20.5712908125139,
0.));
#205988=CARTESIAN_POINT('Ctrl Pts',(-9.84078756677565,20.5619111362402,
0.));
#205989=CARTESIAN_POINT('Ctrl Pts',(-9.83459277585315,20.552674497646,0.));
#205990=CARTESIAN_POINT('Ctrl Pts',(-9.82854073773877,20.5435840460721,
0.));
#205991=CARTESIAN_POINT('Ctrl Pts',(-9.82263220080363,20.5346430299517,
0.));
#205992=CARTESIAN_POINT('Ctrl Pts',(-9.81686793455943,20.5258548000629,
0.));
#205993=CARTESIAN_POINT('Ctrl Pts',(-9.81124873025282,20.517222812284,0.));
#205994=CARTESIAN_POINT('Ctrl Pts',(-9.80577540161088,20.5087506310505,
0.));
#205995=CARTESIAN_POINT('Ctrl Pts',(-9.80044878520949,20.5004419312107,
0.));
#205996=CARTESIAN_POINT('Ctrl Pts',(-9.79526974288331,20.4923005087943,
0.));
#205997=CARTESIAN_POINT('Ctrl Pts',(-9.79023916498656,20.4843302955329,
0.));
#205998=CARTESIAN_POINT('Ctrl Pts',(-9.78535797314167,20.4765353711586,
0.));
#205999=CARTESIAN_POINT('Ctrl Pts',(-9.78062712373321,20.4689199790669,
0.));
#206000=CARTESIAN_POINT('Ctrl Pts',(-9.77604760815529,20.4614885274975,
0.));
#206001=CARTESIAN_POINT('Ctrl Pts',(-9.7716204510407,20.4542455817527,0.));
#206002=CARTESIAN_POINT('Ctrl Pts',(-9.76734670980892,20.447195862298,0.));
#206003=CARTESIAN_POINT('Ctrl Pts',(-9.76322747195495,20.44034423294,0.));
#206004=CARTESIAN_POINT('Ctrl Pts',(-9.75926386289923,20.4336957355473,
0.));
#206005=CARTESIAN_POINT('Ctrl Pts',(-9.75545705902418,20.4272556476629,
0.));
#206006=CARTESIAN_POINT('Ctrl Pts',(-9.7518082978643,20.4210295275817,0.));
#206007=CARTESIAN_POINT('Ctrl Pts',(-9.74831889242174,20.4150232777393,
0.));
#206008=CARTESIAN_POINT('Ctrl Pts',(-9.74499021838538,20.4092430879861,
0.));
#206009=CARTESIAN_POINT('Ctrl Pts',(-9.74182369656272,20.4036953576549,
0.));
#206010=CARTESIAN_POINT('Ctrl Pts',(-9.73882077613201,20.3983866213331,
0.));
#206011=CARTESIAN_POINT('Ctrl Pts',(-9.73598292014243,20.3933234845647,
0.));
#206012=CARTESIAN_POINT('Ctrl Pts',(-9.73331167102808,20.3885129129912,
0.));
#206013=CARTESIAN_POINT('Ctrl Pts',(-9.73080870123727,20.3839624556742,
0.));
#206014=CARTESIAN_POINT('Ctrl Pts',(-9.72847589116542,20.3796805893304,
0.));
#206015=CARTESIAN_POINT('Ctrl Pts',(-9.7263153173288,20.3756766651951,0.));
#206016=CARTESIAN_POINT('Ctrl Pts',(-9.72432910043194,20.371960235676,0.));
#206017=CARTESIAN_POINT('Ctrl Pts',(-9.7225193072249,20.3685406190576,0.));
#206018=CARTESIAN_POINT('Ctrl Pts',(-9.72088778381081,20.3654261611056,
0.));
#206019=CARTESIAN_POINT('Ctrl Pts',(-9.71943648548099,20.3626256913981,
0.));
#206020=CARTESIAN_POINT('Ctrl Pts',(-9.71816778328006,20.3601498764344,
0.));
#206021=CARTESIAN_POINT('Ctrl Pts',(-9.71708493723096,20.3580133103356,
0.));
#206022=CARTESIAN_POINT('Ctrl Pts',(-9.71619192554186,20.3562337557875,
0.));
#206023=CARTESIAN_POINT('Ctrl Pts',(-9.71549257088172,20.3548282742361,
0.));
#206024=CARTESIAN_POINT('Ctrl Pts',(-9.71498978052021,20.3538098605706,
0.));
#206025=CARTESIAN_POINT('Ctrl Pts',(-9.71474590350681,20.3533097561886,
0.));
#206026=CARTESIAN_POINT('Ctrl Pts',(-9.71465227853041,20.3531126095522,
0.));
#206027=CARTESIAN_POINT('Ctrl Pts',(-9.71462954053042,20.353060251684,0.));
#206028=CARTESIAN_POINT('Ctrl Pts',(-9.71462809124916,20.353053841303,0.));
#206029=CARTESIAN_POINT('',(-12.4230808101438,22.8400320311648,0.));
#206030=CARTESIAN_POINT('Ctrl Pts',(-7.52250298901264,21.2610617890679,
0.));
#206031=CARTESIAN_POINT('Ctrl Pts',(-7.52250298901264,21.2610617890679,
12.));
#206032=CARTESIAN_POINT('Ctrl Pts',(-7.5225064970397,21.2610673466886,0.));
#206033=CARTESIAN_POINT('Ctrl Pts',(-7.5225064970397,21.2610673466886,12.));
#206034=CARTESIAN_POINT('Ctrl Pts',(-7.52252744144904,21.2611204474866,
0.));
#206035=CARTESIAN_POINT('Ctrl Pts',(-7.52252744144904,21.2611204474866,
12.));
#206036=CARTESIAN_POINT('Ctrl Pts',(-7.52260064231661,21.261326054066,0.));
#206037=CARTESIAN_POINT('Ctrl Pts',(-7.52260064231661,21.261326054066,12.));
#206038=CARTESIAN_POINT('Ctrl Pts',(-7.5227818224267,21.2618521283555,0.));
#206039=CARTESIAN_POINT('Ctrl Pts',(-7.5227818224267,21.2618521283555,12.));
#206040=CARTESIAN_POINT('Ctrl Pts',(-7.52314642316199,21.262927782038,0.));
#206041=CARTESIAN_POINT('Ctrl Pts',(-7.52314642316199,21.262927782038,12.));
#206042=CARTESIAN_POINT('Ctrl Pts',(-7.52364573027553,21.2644161259962,
0.));
#206043=CARTESIAN_POINT('Ctrl Pts',(-7.52364573027553,21.2644161259962,
12.));
#206044=CARTESIAN_POINT('Ctrl Pts',(-7.52427261074298,21.2663059157058,
0.));
#206045=CARTESIAN_POINT('Ctrl Pts',(-7.52427261074298,21.2663059157058,
12.));
#206046=CARTESIAN_POINT('Ctrl Pts',(-7.5250177033353,21.2685823838671,0.));
#206047=CARTESIAN_POINT('Ctrl Pts',(-7.5250177033353,21.2685823838671,12.));
#206048=CARTESIAN_POINT('Ctrl Pts',(-7.5258712609553,21.2712301573466,0.));
#206049=CARTESIAN_POINT('Ctrl Pts',(-7.5258712609553,21.2712301573466,12.));
#206050=CARTESIAN_POINT('Ctrl Pts',(-7.52682526918541,21.2742366113579,
0.));
#206051=CARTESIAN_POINT('Ctrl Pts',(-7.52682526918541,21.2742366113579,
12.));
#206052=CARTESIAN_POINT('Ctrl Pts',(-7.52787386225333,21.2775925269652,
0.));
#206053=CARTESIAN_POINT('Ctrl Pts',(-7.52787386225333,21.2775925269652,
12.));
#206054=CARTESIAN_POINT('Ctrl Pts',(-7.52901217930408,21.2812902781143,
0.));
#206055=CARTESIAN_POINT('Ctrl Pts',(-7.52901217930408,21.2812902781143,
12.));
#206056=CARTESIAN_POINT('Ctrl Pts',(-7.53023562438229,21.2853226580657,
0.));
#206057=CARTESIAN_POINT('Ctrl Pts',(-7.53023562438229,21.2853226580657,
12.));
#206058=CARTESIAN_POINT('Ctrl Pts',(-7.53153906987855,21.2896816163842,
0.));
#206059=CARTESIAN_POINT('Ctrl Pts',(-7.53153906987855,21.2896816163842,
12.));
#206060=CARTESIAN_POINT('Ctrl Pts',(-7.53291726078527,21.2943588989331,
0.));
#206061=CARTESIAN_POINT('Ctrl Pts',(-7.53291726078527,21.2943588989331,
12.));
#206062=CARTESIAN_POINT('Ctrl Pts',(-7.53436505309943,21.2993464250717,
0.));
#206063=CARTESIAN_POINT('Ctrl Pts',(-7.53436505309943,21.2993464250717,
12.));
#206064=CARTESIAN_POINT('Ctrl Pts',(-7.53587778251736,21.3046368712157,
0.));
#206065=CARTESIAN_POINT('Ctrl Pts',(-7.53587778251736,21.3046368712157,
12.));
#206066=CARTESIAN_POINT('Ctrl Pts',(-7.53745129364616,21.310223716773,0.));
#206067=CARTESIAN_POINT('Ctrl Pts',(-7.53745129364616,21.310223716773,12.));
#206068=CARTESIAN_POINT('Ctrl Pts',(-7.53908175169898,21.3161009456256,
0.));
#206069=CARTESIAN_POINT('Ctrl Pts',(-7.53908175169898,21.3161009456256,
12.));
#206070=CARTESIAN_POINT('Ctrl Pts',(-7.54076552038279,21.3222628524165,
0.));
#206071=CARTESIAN_POINT('Ctrl Pts',(-7.54076552038279,21.3222628524165,
12.));
#206072=CARTESIAN_POINT('Ctrl Pts',(-7.54249900377031,21.328703791771,0.));
#206073=CARTESIAN_POINT('Ctrl Pts',(-7.54249900377031,21.328703791771,12.));
#206074=CARTESIAN_POINT('Ctrl Pts',(-7.54427868151268,21.3354182340149,
0.));
#206075=CARTESIAN_POINT('Ctrl Pts',(-7.54427868151268,21.3354182340149,
12.));
#206076=CARTESIAN_POINT('Ctrl Pts',(-7.54610114948347,21.3424008295038,
0.));
#206077=CARTESIAN_POINT('Ctrl Pts',(-7.54610114948347,21.3424008295038,
12.));
#206078=CARTESIAN_POINT('Ctrl Pts',(-7.5479631624633,21.3496464761531,0.));
#206079=CARTESIAN_POINT('Ctrl Pts',(-7.5479631624633,21.3496464761531,12.));
#206080=CARTESIAN_POINT('Ctrl Pts',(-7.5498616652131,21.3571503685855,0.));
#206081=CARTESIAN_POINT('Ctrl Pts',(-7.5498616652131,21.3571503685855,12.));
#206082=CARTESIAN_POINT('Ctrl Pts',(-7.55179375777444,21.3649079431865,
0.));
#206083=CARTESIAN_POINT('Ctrl Pts',(-7.55179375777444,21.3649079431865,
12.));
#206084=CARTESIAN_POINT('Ctrl Pts',(-7.55375667080029,21.3729148390243,
0.));
#206085=CARTESIAN_POINT('Ctrl Pts',(-7.55375667080029,21.3729148390243,
12.));
#206086=CARTESIAN_POINT('Ctrl Pts',(-7.55574773403503,21.3811668478932,
0.));
#206087=CARTESIAN_POINT('Ctrl Pts',(-7.55574773403503,21.3811668478932,
12.));
#206088=CARTESIAN_POINT('Ctrl Pts',(-7.55776435731417,21.3896598842117,
0.));
#206089=CARTESIAN_POINT('Ctrl Pts',(-7.55776435731417,21.3896598842117,
12.));
#206090=CARTESIAN_POINT('Ctrl Pts',(-7.55980403700611,21.3983899952987,
0.));
#206091=CARTESIAN_POINT('Ctrl Pts',(-7.55980403700611,21.3983899952987,
12.));
#206092=CARTESIAN_POINT('Ctrl Pts',(-7.56186435703622,21.4073533630365,
0.));
#206093=CARTESIAN_POINT('Ctrl Pts',(-7.56186435703622,21.4073533630365,
12.));
#206094=CARTESIAN_POINT('Ctrl Pts',(-7.56394299313685,21.4165463106254,
0.));
#206095=CARTESIAN_POINT('Ctrl Pts',(-7.56394299313685,21.4165463106254,
12.));
#206096=CARTESIAN_POINT('Ctrl Pts',(-7.56603771218712,21.4259653015736,
0.));
#206097=CARTESIAN_POINT('Ctrl Pts',(-7.56603771218712,21.4259653015736,
12.));
#206098=CARTESIAN_POINT('Ctrl Pts',(-7.56814636360847,21.4356069261513,
0.));
#206099=CARTESIAN_POINT('Ctrl Pts',(-7.56814636360847,21.4356069261513,
12.));
#206100=CARTESIAN_POINT('Ctrl Pts',(-7.57026687261166,21.4454678907509,
0.));
#206101=CARTESIAN_POINT('Ctrl Pts',(-7.57026687261166,21.4454678907509,
12.));
#206102=CARTESIAN_POINT('Ctrl Pts',(-7.57239723223506,21.4555450053142,
0.));
#206103=CARTESIAN_POINT('Ctrl Pts',(-7.57239723223506,21.4555450053142,
12.));
#206104=CARTESIAN_POINT('Ctrl Pts',(-7.57453549743412,21.4658351740128,
0.));
#206105=CARTESIAN_POINT('Ctrl Pts',(-7.57453549743412,21.4658351740128,
12.));
#206106=CARTESIAN_POINT('Ctrl Pts',(-7.57667978402987,21.4763353936762,
0.));
#206107=CARTESIAN_POINT('Ctrl Pts',(-7.57667978402987,21.4763353936762,
12.));
#206108=CARTESIAN_POINT('Ctrl Pts',(-7.57882826679132,21.4870427508194,
0.));
#206109=CARTESIAN_POINT('Ctrl Pts',(-7.57882826679132,21.4870427508194,
12.));
#206110=CARTESIAN_POINT('Ctrl Pts',(-7.58097917790744,21.4979544192744,
0.));
#206111=CARTESIAN_POINT('Ctrl Pts',(-7.58097917790744,21.4979544192744,
12.));
#206112=CARTESIAN_POINT('Ctrl Pts',(-7.5831308051918,21.5090676573873,0.));
#206113=CARTESIAN_POINT('Ctrl Pts',(-7.5831308051918,21.5090676573873,12.));
#206114=CARTESIAN_POINT('Ctrl Pts',(-7.5852814891913,21.5203798035299,0.));
#206115=CARTESIAN_POINT('Ctrl Pts',(-7.5852814891913,21.5203798035299,12.));
#206116=CARTESIAN_POINT('Ctrl Pts',(-7.58742962034834,21.5318882716736,
0.));
#206117=CARTESIAN_POINT('Ctrl Pts',(-7.58742962034834,21.5318882716736,
12.));
#206118=CARTESIAN_POINT('Ctrl Pts',(-7.58957363620014,21.543590547011,0.));
#206119=CARTESIAN_POINT('Ctrl Pts',(-7.58957363620014,21.543590547011,12.));
#206120=CARTESIAN_POINT('Ctrl Pts',(-7.59171201844777,21.5554841813462,
0.));
#206121=CARTESIAN_POINT('Ctrl Pts',(-7.59171201844777,21.5554841813462,
12.));
#206122=CARTESIAN_POINT('Ctrl Pts',(-7.59384329124918,21.5675667904726,
0.));
#206123=CARTESIAN_POINT('Ctrl Pts',(-7.59384329124918,21.5675667904726,
12.));
#206124=CARTESIAN_POINT('Ctrl Pts',(-7.59596601973584,21.5798360518978,
0.));
#206125=CARTESIAN_POINT('Ctrl Pts',(-7.59596601973584,21.5798360518978,
12.));
#206126=CARTESIAN_POINT('Ctrl Pts',(-7.59807880846195,21.5922897024466,
0.));
#206127=CARTESIAN_POINT('Ctrl Pts',(-7.59807880846195,21.5922897024466,
12.));
#206128=CARTESIAN_POINT('Ctrl Pts',(-7.60018029988241,21.6049255358843,
0.));
#206129=CARTESIAN_POINT('Ctrl Pts',(-7.60018029988241,21.6049255358843,
12.));
#206130=CARTESIAN_POINT('Ctrl Pts',(-7.60226917285429,21.617741400599,0.));
#206131=CARTESIAN_POINT('Ctrl Pts',(-7.60226917285429,21.617741400599,12.));
#206132=CARTESIAN_POINT('Ctrl Pts',(-7.60434414118296,21.6307351973822,
0.));
#206133=CARTESIAN_POINT('Ctrl Pts',(-7.60434414118296,21.6307351973822,
12.));
#206134=CARTESIAN_POINT('Ctrl Pts',(-7.60640395216357,21.6439048771743,
0.));
#206135=CARTESIAN_POINT('Ctrl Pts',(-7.60640395216357,21.6439048771743,
12.));
#206136=CARTESIAN_POINT('Ctrl Pts',(-7.60844738512874,21.6572484388081,
0.));
#206137=CARTESIAN_POINT('Ctrl Pts',(-7.60844738512874,21.6572484388081,
12.));
#206138=CARTESIAN_POINT('Ctrl Pts',(-7.61047325000956,21.6707639267576,
0.));
#206139=CARTESIAN_POINT('Ctrl Pts',(-7.61047325000956,21.6707639267576,
12.));
#206140=CARTESIAN_POINT('Ctrl Pts',(-7.61248038630268,21.6844494295815,
0.));
#206141=CARTESIAN_POINT('Ctrl Pts',(-7.61248038630268,21.6844494295815,
12.));
#206142=CARTESIAN_POINT('Ctrl Pts',(-7.61446766202787,21.6983030783322,
0.));
#206143=CARTESIAN_POINT('Ctrl Pts',(-7.61446766202787,21.6983030783322,
12.));
#206144=CARTESIAN_POINT('Ctrl Pts',(-7.61643397270421,21.7123230449834,
0.));
#206145=CARTESIAN_POINT('Ctrl Pts',(-7.61643397270421,21.7123230449834,
12.));
#206146=CARTESIAN_POINT('Ctrl Pts',(-7.61837824030538,21.7265075407975,
0.));
#206147=CARTESIAN_POINT('Ctrl Pts',(-7.61837824030538,21.7265075407975,
12.));
#206148=CARTESIAN_POINT('Ctrl Pts',(-7.62029941230855,21.7408548148656,
0.));
#206149=CARTESIAN_POINT('Ctrl Pts',(-7.62029941230855,21.7408548148656,
12.));
#206150=CARTESIAN_POINT('Ctrl Pts',(-7.62219646084228,21.7553631528328,
0.));
#206151=CARTESIAN_POINT('Ctrl Pts',(-7.62219646084228,21.7553631528328,
12.));
#206152=CARTESIAN_POINT('Ctrl Pts',(-7.62406838181166,21.7700308755584,
0.));
#206153=CARTESIAN_POINT('Ctrl Pts',(-7.62406838181166,21.7700308755584,
12.));
#206154=CARTESIAN_POINT('Ctrl Pts',(-7.62591419404512,21.7848563378021,
0.));
#206155=CARTESIAN_POINT('Ctrl Pts',(-7.62591419404512,21.7848563378021,
12.));
#206156=CARTESIAN_POINT('Ctrl Pts',(-7.62773293842389,21.799837926858,0.));
#206157=CARTESIAN_POINT('Ctrl Pts',(-7.62773293842389,21.799837926858,12.));
#206158=CARTESIAN_POINT('Ctrl Pts',(-7.62952367718127,21.814974061509,0.));
#206159=CARTESIAN_POINT('Ctrl Pts',(-7.62952367718127,21.814974061509,12.));
#206160=CARTESIAN_POINT('Ctrl Pts',(-7.63128549323023,21.8302631910195,
0.));
#206161=CARTESIAN_POINT('Ctrl Pts',(-7.63128549323023,21.8302631910195,
12.));
#206162=CARTESIAN_POINT('Ctrl Pts',(-7.63301748948936,21.8457037941084,
0.));
#206163=CARTESIAN_POINT('Ctrl Pts',(-7.63301748948936,21.8457037941084,
12.));
#206164=CARTESIAN_POINT('Ctrl Pts',(-7.63471878821226,21.8612943779089,
0.));
#206165=CARTESIAN_POINT('Ctrl Pts',(-7.63471878821226,21.8612943779089,
12.));
#206166=CARTESIAN_POINT('Ctrl Pts',(-7.636388530334,21.8770334769496,0.));
#206167=CARTESIAN_POINT('Ctrl Pts',(-7.636388530334,21.8770334769496,12.));
#206168=CARTESIAN_POINT('Ctrl Pts',(-7.63802587492035,21.8929196523514,
0.));
#206169=CARTESIAN_POINT('Ctrl Pts',(-7.63802587492035,21.8929196523514,
12.));
#206170=CARTESIAN_POINT('Ctrl Pts',(-7.63962999860927,21.9089514909874,
0.));
#206171=CARTESIAN_POINT('Ctrl Pts',(-7.63962999860927,21.9089514909874,
12.));
#206172=CARTESIAN_POINT('Ctrl Pts',(-7.64120009506532,21.9251276046546,
0.));
#206173=CARTESIAN_POINT('Ctrl Pts',(-7.64120009506532,21.9251276046546,
12.));
#206174=CARTESIAN_POINT('Ctrl Pts',(-7.64273537442682,21.9414466292072,
0.));
#206175=CARTESIAN_POINT('Ctrl Pts',(-7.64273537442682,21.9414466292072,
12.));
#206176=CARTESIAN_POINT('Ctrl Pts',(-7.64423506279123,21.9579072237651,
0.));
#206177=CARTESIAN_POINT('Ctrl Pts',(-7.64423506279123,21.9579072237651,
12.));
#206178=CARTESIAN_POINT('Ctrl Pts',(-7.64569840177336,21.9745080700798,
0.));
#206179=CARTESIAN_POINT('Ctrl Pts',(-7.64569840177336,21.9745080700798,
12.));
#206180=CARTESIAN_POINT('Ctrl Pts',(-7.6471246480525,21.9912478718542,0.));
#206181=CARTESIAN_POINT('Ctrl Pts',(-7.6471246480525,21.9912478718542,12.));
#206182=CARTESIAN_POINT('Ctrl Pts',(-7.64851307293352,22.0081253540774,
0.));
#206183=CARTESIAN_POINT('Ctrl Pts',(-7.64851307293352,22.0081253540774,
12.));
#206184=CARTESIAN_POINT('Ctrl Pts',(-7.64986296190168,22.0251392623209,
0.));
#206185=CARTESIAN_POINT('Ctrl Pts',(-7.64986296190168,22.0251392623209,
12.));
#206186=CARTESIAN_POINT('Ctrl Pts',(-7.65117361421358,22.0422883621174,
0.));
#206187=CARTESIAN_POINT('Ctrl Pts',(-7.65117361421358,22.0422883621174,
12.));
#206188=CARTESIAN_POINT('Ctrl Pts',(-7.65244434253113,22.0595714384431,
0.));
#206189=CARTESIAN_POINT('Ctrl Pts',(-7.65244434253113,22.0595714384431,
12.));
#206190=CARTESIAN_POINT('Ctrl Pts',(-7.65367447254949,22.0769872951596,
0.));
#206191=CARTESIAN_POINT('Ctrl Pts',(-7.65367447254949,22.0769872951596,
12.));
#206192=CARTESIAN_POINT('Ctrl Pts',(-7.65486334263644,22.094534754469,0.));
#206193=CARTESIAN_POINT('Ctrl Pts',(-7.65486334263644,22.094534754469,12.));
#206194=CARTESIAN_POINT('Ctrl Pts',(-7.65601030346807,22.1122126563329,
0.));
#206195=CARTESIAN_POINT('Ctrl Pts',(-7.65601030346807,22.1122126563329,
12.));
#206196=CARTESIAN_POINT('Ctrl Pts',(-7.65711471769397,22.1300198579675,
0.));
#206197=CARTESIAN_POINT('Ctrl Pts',(-7.65711471769397,22.1300198579675,
12.));
#206198=CARTESIAN_POINT('Ctrl Pts',(-7.65817595963349,22.1479552334211,
0.));
#206199=CARTESIAN_POINT('Ctrl Pts',(-7.65817595963349,22.1479552334211,
12.));
#206200=CARTESIAN_POINT('Ctrl Pts',(-7.6591934149693,22.1660176731178,0.));
#206201=CARTESIAN_POINT('Ctrl Pts',(-7.6591934149693,22.1660176731178,12.));
#206202=CARTESIAN_POINT('Ctrl Pts',(-7.66016648045005,22.1842060834091,
0.));
#206203=CARTESIAN_POINT('Ctrl Pts',(-7.66016648045005,22.1842060834091,
12.));
#206204=CARTESIAN_POINT('Ctrl Pts',(-7.66109456359271,22.2025193860964,
0.));
#206205=CARTESIAN_POINT('Ctrl Pts',(-7.66109456359271,22.2025193860964,
12.));
#206206=CARTESIAN_POINT('Ctrl Pts',(-7.661977082404,22.2209565180085,0.));
#206207=CARTESIAN_POINT('Ctrl Pts',(-7.661977082404,22.2209565180085,12.));
#206208=CARTESIAN_POINT('Ctrl Pts',(-7.66281346512509,22.2395164306547,
0.));
#206209=CARTESIAN_POINT('Ctrl Pts',(-7.66281346512509,22.2395164306547,
12.));
#206210=CARTESIAN_POINT('Ctrl Pts',(-7.66360314997641,22.258198089848,0.));
#206211=CARTESIAN_POINT('Ctrl Pts',(-7.66360314997641,22.258198089848,12.));
#206212=CARTESIAN_POINT('Ctrl Pts',(-7.66434558490979,22.2770004753335,
0.));
#206213=CARTESIAN_POINT('Ctrl Pts',(-7.66434558490979,22.2770004753335,
12.));
#206214=CARTESIAN_POINT('Ctrl Pts',(-7.66504022736299,22.2959225803937,
0.));
#206215=CARTESIAN_POINT('Ctrl Pts',(-7.66504022736299,22.2959225803937,
12.));
#206216=CARTESIAN_POINT('Ctrl Pts',(-7.66568654402494,22.314963411484,0.));
#206217=CARTESIAN_POINT('Ctrl Pts',(-7.66568654402494,22.314963411484,12.));
#206218=CARTESIAN_POINT('Ctrl Pts',(-7.66628401061952,22.3341219879469,
0.));
#206219=CARTESIAN_POINT('Ctrl Pts',(-7.66628401061952,22.3341219879469,
12.));
#206220=CARTESIAN_POINT('Ctrl Pts',(-7.66683211169158,22.3533973417021,
0.));
#206221=CARTESIAN_POINT('Ctrl Pts',(-7.66683211169158,22.3533973417021,
12.));
#206222=CARTESIAN_POINT('Ctrl Pts',(-7.66733034039883,22.372788516936,0.));
#206223=CARTESIAN_POINT('Ctrl Pts',(-7.66733034039883,22.372788516936,12.));
#206224=CARTESIAN_POINT('Ctrl Pts',(-7.6677781983079,22.3922945697773,0.));
#206225=CARTESIAN_POINT('Ctrl Pts',(-7.6677781983079,22.3922945697773,12.));
#206226=CARTESIAN_POINT('Ctrl Pts',(-7.6681751951964,22.4119145679758,0.));
#206227=CARTESIAN_POINT('Ctrl Pts',(-7.6681751951964,22.4119145679758,12.));
#206228=CARTESIAN_POINT('Ctrl Pts',(-7.66852084886704,22.4316475906603,
0.));
#206229=CARTESIAN_POINT('Ctrl Pts',(-7.66852084886704,22.4316475906603,
12.));
#206230=CARTESIAN_POINT('Ctrl Pts',(-7.66881468496635,22.4514927280855,
0.));
#206231=CARTESIAN_POINT('Ctrl Pts',(-7.66881468496635,22.4514927280855,
12.));
#206232=CARTESIAN_POINT('Ctrl Pts',(-7.66905623680831,22.47144908137,0.));
#206233=CARTESIAN_POINT('Ctrl Pts',(-7.66905623680831,22.47144908137,12.));
#206234=CARTESIAN_POINT('Ctrl Pts',(-7.66924504520315,22.4915157622312,
0.));
#206235=CARTESIAN_POINT('Ctrl Pts',(-7.66924504520315,22.4915157622312,
12.));
#206236=CARTESIAN_POINT('Ctrl Pts',(-7.66938065829108,22.5116918927031,
0.));
#206237=CARTESIAN_POINT('Ctrl Pts',(-7.66938065829108,22.5116918927031,
12.));
#206238=CARTESIAN_POINT('Ctrl Pts',(-7.66946263138144,22.53197660492,0.));
#206239=CARTESIAN_POINT('Ctrl Pts',(-7.66946263138144,22.53197660492,12.));
#206240=CARTESIAN_POINT('Ctrl Pts',(-7.66949052679693,22.5523690409116,
0.));
#206241=CARTESIAN_POINT('Ctrl Pts',(-7.66949052679693,22.5523690409116,
12.));
#206242=CARTESIAN_POINT('Ctrl Pts',(-7.66946391372306,22.5728683523831,
0.));
#206243=CARTESIAN_POINT('Ctrl Pts',(-7.66946391372306,22.5728683523831,
12.));
#206244=CARTESIAN_POINT('Ctrl Pts',(-7.66938236806233,22.5934737004953,
0.));
#206245=CARTESIAN_POINT('Ctrl Pts',(-7.66938236806233,22.5934737004953,
12.));
#206246=CARTESIAN_POINT('Ctrl Pts',(-7.66924547229414,22.6141842556243,
0.));
#206247=CARTESIAN_POINT('Ctrl Pts',(-7.66924547229414,22.6141842556243,
12.));
#206248=CARTESIAN_POINT('Ctrl Pts',(-7.66905281533715,22.6349991971541,
0.));
#206249=CARTESIAN_POINT('Ctrl Pts',(-7.66905281533715,22.6349991971541,
12.));
#206250=CARTESIAN_POINT('Ctrl Pts',(-7.66880399241323,22.6559177133127,
0.));
#206251=CARTESIAN_POINT('Ctrl Pts',(-7.66880399241323,22.6559177133127,
12.));
#206252=CARTESIAN_POINT('Ctrl Pts',(-7.66849860491743,22.6769390009885,
0.));
#206253=CARTESIAN_POINT('Ctrl Pts',(-7.66849860491743,22.6769390009885,
12.));
#206254=CARTESIAN_POINT('Ctrl Pts',(-7.66813626029275,22.6980622655446,
0.));
#206255=CARTESIAN_POINT('Ctrl Pts',(-7.66813626029275,22.6980622655446,
12.));
#206256=CARTESIAN_POINT('Ctrl Pts',(-7.66771657191027,22.7192867206245,
0.));
#206257=CARTESIAN_POINT('Ctrl Pts',(-7.66771657191027,22.7192867206245,
12.));
#206258=CARTESIAN_POINT('Ctrl Pts',(-7.6672391589544,22.7406115879513,0.));
#206259=CARTESIAN_POINT('Ctrl Pts',(-7.6672391589544,22.7406115879513,12.));
#206260=CARTESIAN_POINT('Ctrl Pts',(-7.66670364630299,22.7620360971843,
0.));
#206261=CARTESIAN_POINT('Ctrl Pts',(-7.66670364630299,22.7620360971843,
12.));
#206262=CARTESIAN_POINT('Ctrl Pts',(-7.66610966441273,22.7835594857699,
0.));
#206263=CARTESIAN_POINT('Ctrl Pts',(-7.66610966441273,22.7835594857699,
12.));
#206264=CARTESIAN_POINT('Ctrl Pts',(-7.66545684920987,22.8051809987833,
0.));
#206265=CARTESIAN_POINT('Ctrl Pts',(-7.66545684920987,22.8051809987833,
12.));
#206266=CARTESIAN_POINT('Ctrl Pts',(-7.66474484198549,22.8268998887678,
0.));
#206267=CARTESIAN_POINT('Ctrl Pts',(-7.66474484198549,22.8268998887678,
12.));
#206268=CARTESIAN_POINT('Ctrl Pts',(-7.66397328929803,22.848715415557,0.));
#206269=CARTESIAN_POINT('Ctrl Pts',(-7.66397328929803,22.848715415557,12.));
#206270=CARTESIAN_POINT('Ctrl Pts',(-7.66314184287337,22.8706268461283,
0.));
#206271=CARTESIAN_POINT('Ctrl Pts',(-7.66314184287337,22.8706268461283,
12.));
#206272=CARTESIAN_POINT('Ctrl Pts',(-7.66225015950156,22.8926334544883,
0.));
#206273=CARTESIAN_POINT('Ctrl Pts',(-7.66225015950156,22.8926334544883,
12.));
#206274=CARTESIAN_POINT('Ctrl Pts',(-7.66129790094108,22.9147345215421,
0.));
#206275=CARTESIAN_POINT('Ctrl Pts',(-7.66129790094108,22.9147345215421,
12.));
#206276=CARTESIAN_POINT('Ctrl Pts',(-7.66028473382778,22.9369293349593,
0.));
#206277=CARTESIAN_POINT('Ctrl Pts',(-7.66028473382778,22.9369293349593,
12.));
#206278=CARTESIAN_POINT('Ctrl Pts',(-7.65921032958902,22.959217189033,0.));
#206279=CARTESIAN_POINT('Ctrl Pts',(-7.65921032958902,22.959217189033,12.));
#206280=CARTESIAN_POINT('Ctrl Pts',(-7.65807436436432,22.9815973845296,
0.));
#206281=CARTESIAN_POINT('Ctrl Pts',(-7.65807436436432,22.9815973845296,
12.));
#206282=CARTESIAN_POINT('Ctrl Pts',(-7.65687651891304,23.0040692285814,
0.));
#206283=CARTESIAN_POINT('Ctrl Pts',(-7.65687651891304,23.0040692285814,
12.));
#206284=CARTESIAN_POINT('Ctrl Pts',(-7.65561647852534,23.0266320345787,
0.));
#206285=CARTESIAN_POINT('Ctrl Pts',(-7.65561647852534,23.0266320345787,
12.));
#206286=CARTESIAN_POINT('Ctrl Pts',(-7.65429393293946,23.0492851220528,
0.));
#206287=CARTESIAN_POINT('Ctrl Pts',(-7.65429393293946,23.0492851220528,
12.));
#206288=CARTESIAN_POINT('Ctrl Pts',(-7.65290857626358,23.072027816555,0.));
#206289=CARTESIAN_POINT('Ctrl Pts',(-7.65290857626358,23.072027816555,12.));
#206290=CARTESIAN_POINT('Ctrl Pts',(-7.65146010690476,23.094859449525,0.));
#206291=CARTESIAN_POINT('Ctrl Pts',(-7.65146010690476,23.094859449525,12.));
#206292=CARTESIAN_POINT('Ctrl Pts',(-7.6499482274986,23.1177793581679,0.));
#206293=CARTESIAN_POINT('Ctrl Pts',(-7.6499482274986,23.1177793581679,12.));
#206294=CARTESIAN_POINT('Ctrl Pts',(-7.64837264482943,23.1407868853819,
0.));
#206295=CARTESIAN_POINT('Ctrl Pts',(-7.64837264482943,23.1407868853819,
12.));
#206296=CARTESIAN_POINT('Ctrl Pts',(-7.64673306975805,23.1638813796694,
0.));
#206297=CARTESIAN_POINT('Ctrl Pts',(-7.64673306975805,23.1638813796694,
12.));
#206298=CARTESIAN_POINT('Ctrl Pts',(-7.64502921715483,23.1870621950452,
0.));
#206299=CARTESIAN_POINT('Ctrl Pts',(-7.64502921715483,23.1870621950452,
12.));
#206300=CARTESIAN_POINT('Ctrl Pts',(-7.6432608058368,23.2103286909398,0.));
#206301=CARTESIAN_POINT('Ctrl Pts',(-7.6432608058368,23.2103286909398,12.));
#206302=CARTESIAN_POINT('Ctrl Pts',(-7.64142755851504,23.2336802320912,
0.));
#206303=CARTESIAN_POINT('Ctrl Pts',(-7.64142755851504,23.2336802320912,
12.));
#206304=CARTESIAN_POINT('Ctrl Pts',(-7.63952920172835,23.2571161884488,
0.));
#206305=CARTESIAN_POINT('Ctrl Pts',(-7.63952920172835,23.2571161884488,
12.));
#206306=CARTESIAN_POINT('Ctrl Pts',(-7.63756546576374,23.2806359350855,
0.));
#206307=CARTESIAN_POINT('Ctrl Pts',(-7.63756546576374,23.2806359350855,
12.));
#206308=CARTESIAN_POINT('Ctrl Pts',(-7.63553608458783,23.3042388521022,
0.));
#206309=CARTESIAN_POINT('Ctrl Pts',(-7.63553608458783,23.3042388521022,
12.));
#206310=CARTESIAN_POINT('Ctrl Pts',(-7.63344079578161,23.3279243245241,
0.));
#206311=CARTESIAN_POINT('Ctrl Pts',(-7.63344079578161,23.3279243245241,
12.));
#206312=CARTESIAN_POINT('Ctrl Pts',(-7.63127934048136,23.3516917421972,
0.));
#206313=CARTESIAN_POINT('Ctrl Pts',(-7.63127934048136,23.3516917421972,
12.));
#206314=CARTESIAN_POINT('Ctrl Pts',(-7.62905146332593,23.3755404996636,
0.));
#206315=CARTESIAN_POINT('Ctrl Pts',(-7.62905146332593,23.3755404996636,
12.));
#206316=CARTESIAN_POINT('Ctrl Pts',(-7.62675691240329,23.399469996112,0.));
#206317=CARTESIAN_POINT('Ctrl Pts',(-7.62675691240329,23.399469996112,12.));
#206318=CARTESIAN_POINT('Ctrl Pts',(-7.6243954392005,23.4234796353542,0.));
#206319=CARTESIAN_POINT('Ctrl Pts',(-7.6243954392005,23.4234796353542,12.));
#206320=CARTESIAN_POINT('Ctrl Pts',(-7.62196679855955,23.4475688257854,
0.));
#206321=CARTESIAN_POINT('Ctrl Pts',(-7.62196679855955,23.4475688257854,
12.));
#206322=CARTESIAN_POINT('Ctrl Pts',(-7.61947074863977,23.4717369803438,
0.));
#206323=CARTESIAN_POINT('Ctrl Pts',(-7.61947074863977,23.4717369803438,
12.));
#206324=CARTESIAN_POINT('Ctrl Pts',(-7.61690705088319,23.4959835164609,
0.));
#206325=CARTESIAN_POINT('Ctrl Pts',(-7.61690705088319,23.4959835164609,
12.));
#206326=CARTESIAN_POINT('Ctrl Pts',(-7.61427546999298,23.5203078560129,
0.));
#206327=CARTESIAN_POINT('Ctrl Pts',(-7.61427546999298,23.5203078560129,
12.));
#206328=CARTESIAN_POINT('Ctrl Pts',(-7.61157577385372,23.544709425203,0.));
#206329=CARTESIAN_POINT('Ctrl Pts',(-7.61157577385372,23.544709425203,12.));
#206330=CARTESIAN_POINT('Ctrl Pts',(-7.608807733446,23.5691876544244,0.));
#206331=CARTESIAN_POINT('Ctrl Pts',(-7.608807733446,23.5691876544244,12.));
#206332=CARTESIAN_POINT('Ctrl Pts',(-7.60597112277094,23.5937419781245,
0.));
#206333=CARTESIAN_POINT('Ctrl Pts',(-7.60597112277094,23.5937419781245,
12.));
#206334=CARTESIAN_POINT('Ctrl Pts',(-7.60306571877806,23.6183718346576,
0.));
#206335=CARTESIAN_POINT('Ctrl Pts',(-7.60306571877806,23.6183718346576,
12.));
#206336=CARTESIAN_POINT('Ctrl Pts',(-7.60009130130126,23.6430766661418,
0.));
#206337=CARTESIAN_POINT('Ctrl Pts',(-7.60009130130126,23.6430766661418,
12.));
#206338=CARTESIAN_POINT('Ctrl Pts',(-7.59704765299567,23.6678559182875,
0.));
#206339=CARTESIAN_POINT('Ctrl Pts',(-7.59704765299567,23.6678559182875,
12.));
#206340=CARTESIAN_POINT('Ctrl Pts',(-7.59393455934035,23.6927090405066,
0.));
#206341=CARTESIAN_POINT('Ctrl Pts',(-7.59393455934035,23.6927090405066,
12.));
#206342=CARTESIAN_POINT('Ctrl Pts',(-7.5907518086532,23.7176354860456,0.));
#206343=CARTESIAN_POINT('Ctrl Pts',(-7.5907518086532,23.7176354860456,12.));
#206344=CARTESIAN_POINT('Ctrl Pts',(-7.58749919210826,23.7426347121006,
0.));
#206345=CARTESIAN_POINT('Ctrl Pts',(-7.58749919210826,23.7426347121006,
12.));
#206346=CARTESIAN_POINT('Ctrl Pts',(-7.58417650376271,23.7677061799376,
0.));
#206347=CARTESIAN_POINT('Ctrl Pts',(-7.58417650376271,23.7677061799376,
12.));
#206348=CARTESIAN_POINT('Ctrl Pts',(-7.58078354058213,23.7928493549908,
0.));
#206349=CARTESIAN_POINT('Ctrl Pts',(-7.58078354058213,23.7928493549908,
12.));
#206350=CARTESIAN_POINT('Ctrl Pts',(-7.57732010249066,23.8180637069976,
0.));
#206351=CARTESIAN_POINT('Ctrl Pts',(-7.57732010249066,23.8180637069976,
12.));
#206352=CARTESIAN_POINT('Ctrl Pts',(-7.57378599219814,23.8433487096132,
0.));
#206353=CARTESIAN_POINT('Ctrl Pts',(-7.57378599219814,23.8433487096132,
12.));
#206354=CARTESIAN_POINT('Ctrl Pts',(-7.57018101500709,23.8687038399595,
0.));
#206355=CARTESIAN_POINT('Ctrl Pts',(-7.57018101500709,23.8687038399595,
12.));
#206356=CARTESIAN_POINT('Ctrl Pts',(-7.56650497863791,23.8941285782002,
0.));
#206357=CARTESIAN_POINT('Ctrl Pts',(-7.56650497863791,23.8941285782002,
12.));
#206358=CARTESIAN_POINT('Ctrl Pts',(-7.56275769304773,23.9196224070759,
0.));
#206359=CARTESIAN_POINT('Ctrl Pts',(-7.56275769304773,23.9196224070759,
12.));
#206360=CARTESIAN_POINT('Ctrl Pts',(-7.5589389702768,23.9451848115002,0.));
#206361=CARTESIAN_POINT('Ctrl Pts',(-7.5589389702768,23.9451848115002,12.));
#206362=CARTESIAN_POINT('Ctrl Pts',(-7.55504862424808,23.9708152779886,
0.));
#206363=CARTESIAN_POINT('Ctrl Pts',(-7.55504862424808,23.9708152779886,
12.));
#206364=CARTESIAN_POINT('Ctrl Pts',(-7.55108647097432,23.9965132953187,
0.));
#206365=CARTESIAN_POINT('Ctrl Pts',(-7.55108647097432,23.9965132953187,
12.));
#206366=CARTESIAN_POINT('Ctrl Pts',(-7.54705232885895,24.0222783554531,
0.));
#206367=CARTESIAN_POINT('Ctrl Pts',(-7.54705232885895,24.0222783554531,
12.));
#206368=CARTESIAN_POINT('Ctrl Pts',(-7.54294601896128,24.0481099543353,
0.));
#206369=CARTESIAN_POINT('Ctrl Pts',(-7.54294601896128,24.0481099543353,
12.));
#206370=CARTESIAN_POINT('Ctrl Pts',(-7.53876736531005,24.0740075927984,
0.));
#206371=CARTESIAN_POINT('Ctrl Pts',(-7.53876736531005,24.0740075927984,
12.));
#206372=CARTESIAN_POINT('Ctrl Pts',(-7.53451619514658,24.0999707772643,
0.));
#206373=CARTESIAN_POINT('Ctrl Pts',(-7.53451619514658,24.0999707772643,
12.));
#206374=CARTESIAN_POINT('Ctrl Pts',(-7.53019233935536,24.1259990209211,
0.));
#206375=CARTESIAN_POINT('Ctrl Pts',(-7.53019233935536,24.1259990209211,
12.));
#206376=CARTESIAN_POINT('Ctrl Pts',(-7.52579563201479,24.152091842537,0.));
#206377=CARTESIAN_POINT('Ctrl Pts',(-7.52579563201479,24.152091842537,12.));
#206378=CARTESIAN_POINT('Ctrl Pts',(-7.52132590953862,24.1782487641602,
0.));
#206379=CARTESIAN_POINT('Ctrl Pts',(-7.52132590953862,24.1782487641602,
12.));
#206380=CARTESIAN_POINT('Ctrl Pts',(-7.51678300997998,24.2044693092356,
0.));
#206381=CARTESIAN_POINT('Ctrl Pts',(-7.51678300997998,24.2044693092356,
12.));
#206382=CARTESIAN_POINT('Ctrl Pts',(-7.51216677222199,24.230753000389,0.));
#206383=CARTESIAN_POINT('Ctrl Pts',(-7.51216677222199,24.230753000389,12.));
#206384=CARTESIAN_POINT('Ctrl Pts',(-7.50747703535115,24.2570993577032,
0.));
#206385=CARTESIAN_POINT('Ctrl Pts',(-7.50747703535115,24.2570993577032,
12.));
#206386=CARTESIAN_POINT('Ctrl Pts',(-7.50271363765098,24.2835078958966,
0.));
#206387=CARTESIAN_POINT('Ctrl Pts',(-7.50271363765098,24.2835078958966,
12.));
#206388=CARTESIAN_POINT('Ctrl Pts',(-7.49787641695359,24.3099781253345,
0.));
#206389=CARTESIAN_POINT('Ctrl Pts',(-7.49787641695359,24.3099781253345,
12.));
#206390=CARTESIAN_POINT('Ctrl Pts',(-7.4929652125233,24.3365095573673,0.));
#206391=CARTESIAN_POINT('Ctrl Pts',(-7.4929652125233,24.3365095573673,12.));
#206392=CARTESIAN_POINT('Ctrl Pts',(-7.48797986651828,24.3631017084513,
0.));
#206393=CARTESIAN_POINT('Ctrl Pts',(-7.48797986651828,24.3631017084513,
12.));
#206394=CARTESIAN_POINT('Ctrl Pts',(-7.48292022569254,24.3897541049248,
0.));
#206395=CARTESIAN_POINT('Ctrl Pts',(-7.48292022569254,24.3897541049248,
12.));
#206396=CARTESIAN_POINT('Ctrl Pts',(-7.47778614286573,24.4164662871165,
0.));
#206397=CARTESIAN_POINT('Ctrl Pts',(-7.47778614286573,24.4164662871165,
12.));
#206398=CARTESIAN_POINT('Ctrl Pts',(-7.47257747883319,24.4432378146501,
0.));
#206399=CARTESIAN_POINT('Ctrl Pts',(-7.47257747883319,24.4432378146501,
12.));
#206400=CARTESIAN_POINT('Ctrl Pts',(-7.46729410308923,24.4700682684544,
0.));
#206401=CARTESIAN_POINT('Ctrl Pts',(-7.46729410308923,24.4700682684544,
12.));
#206402=CARTESIAN_POINT('Ctrl Pts',(-7.46193588961642,24.4969572391509,
0.));
#206403=CARTESIAN_POINT('Ctrl Pts',(-7.46193588961642,24.4969572391509,
12.));
#206404=CARTESIAN_POINT('Ctrl Pts',(-7.45650271336045,24.52390431731,0.));
#206405=CARTESIAN_POINT('Ctrl Pts',(-7.45650271336045,24.52390431731,12.));
#206406=CARTESIAN_POINT('Ctrl Pts',(-7.45099444651296,24.5509090831579,
0.));
#206407=CARTESIAN_POINT('Ctrl Pts',(-7.45099444651296,24.5509090831579,
12.));
#206408=CARTESIAN_POINT('Ctrl Pts',(-7.44541095473163,24.5779710960865,
0.));
#206409=CARTESIAN_POINT('Ctrl Pts',(-7.44541095473163,24.5779710960865,
12.));
#206410=CARTESIAN_POINT('Ctrl Pts',(-7.43975209375375,24.6050898852349,
0.));
#206411=CARTESIAN_POINT('Ctrl Pts',(-7.43975209375375,24.6050898852349,
12.));
#206412=CARTESIAN_POINT('Ctrl Pts',(-7.4340177048922,24.6322649369472,0.));
#206413=CARTESIAN_POINT('Ctrl Pts',(-7.4340177048922,24.6322649369472,12.));
#206414=CARTESIAN_POINT('Ctrl Pts',(-7.42820762158681,24.659495712869,0.));
#206415=CARTESIAN_POINT('Ctrl Pts',(-7.42820762158681,24.659495712869,12.));
#206416=CARTESIAN_POINT('Ctrl Pts',(-7.42232167765763,24.6867816727118,
0.));
#206417=CARTESIAN_POINT('Ctrl Pts',(-7.42232167765763,24.6867816727118,
12.));
#206418=CARTESIAN_POINT('Ctrl Pts',(-7.41635971481243,24.7141222949988,
0.));
#206419=CARTESIAN_POINT('Ctrl Pts',(-7.41635971481243,24.7141222949988,
12.));
#206420=CARTESIAN_POINT('Ctrl Pts',(-7.41032159082173,24.7415170994754,
0.));
#206421=CARTESIAN_POINT('Ctrl Pts',(-7.41032159082173,24.7415170994754,
12.));
#206422=CARTESIAN_POINT('Ctrl Pts',(-7.40420718661754,24.7689656669005,
0.));
#206423=CARTESIAN_POINT('Ctrl Pts',(-7.40420718661754,24.7689656669005,
12.));
#206424=CARTESIAN_POINT('Ctrl Pts',(-7.39801641583612,24.7964676646518,
0.));
#206425=CARTESIAN_POINT('Ctrl Pts',(-7.39801641583612,24.7964676646518,
12.));
#206426=CARTESIAN_POINT('Ctrl Pts',(-7.39174922586841,24.8240228521042,
0.));
#206427=CARTESIAN_POINT('Ctrl Pts',(-7.39174922586841,24.8240228521042,
12.));
#206428=CARTESIAN_POINT('Ctrl Pts',(-7.38540558904946,24.8516310625367,
0.));
#206429=CARTESIAN_POINT('Ctrl Pts',(-7.38540558904946,24.8516310625367,
12.));
#206430=CARTESIAN_POINT('Ctrl Pts',(-7.3789854964161,24.8792921911309,0.));
#206431=CARTESIAN_POINT('Ctrl Pts',(-7.3789854964161,24.8792921911309,12.));
#206432=CARTESIAN_POINT('Ctrl Pts',(-7.37378825962718,24.9014633826201,
0.));
#206433=CARTESIAN_POINT('Ctrl Pts',(-7.37378825962718,24.9014633826201,
12.));
#206434=CARTESIAN_POINT('Ctrl Pts',(-7.36985593120696,24.9181155530631,
0.));
#206435=CARTESIAN_POINT('Ctrl Pts',(-7.36985593120696,24.9181155530631,
12.));
#206436=CARTESIAN_POINT('Ctrl Pts',(-7.3672190902906,24.9292275670705,0.));
#206437=CARTESIAN_POINT('Ctrl Pts',(-7.3672190902906,24.9292275670705,12.));
#206438=CARTESIAN_POINT('Ctrl Pts',(-7.36589684767344,24.9347862158358,
0.));
#206439=CARTESIAN_POINT('Ctrl Pts',(-7.36589684767344,24.9347862158358,
12.));
#206440=CARTESIAN_POINT('',(-7.36589684767344,24.9347862158358,0.));
#206441=CARTESIAN_POINT('Ctrl Pts',(-7.52250298901264,21.2610617890679,
0.));
#206442=CARTESIAN_POINT('Ctrl Pts',(-7.5225064970397,21.2610673466886,0.));
#206443=CARTESIAN_POINT('Ctrl Pts',(-7.52252744144904,21.2611204474866,
0.));
#206444=CARTESIAN_POINT('Ctrl Pts',(-7.52260064231661,21.261326054066,0.));
#206445=CARTESIAN_POINT('Ctrl Pts',(-7.5227818224267,21.2618521283555,0.));
#206446=CARTESIAN_POINT('Ctrl Pts',(-7.52314642316199,21.262927782038,0.));
#206447=CARTESIAN_POINT('Ctrl Pts',(-7.52364573027553,21.2644161259962,
0.));
#206448=CARTESIAN_POINT('Ctrl Pts',(-7.52427261074298,21.2663059157058,
0.));
#206449=CARTESIAN_POINT('Ctrl Pts',(-7.5250177033353,21.2685823838671,0.));
#206450=CARTESIAN_POINT('Ctrl Pts',(-7.5258712609553,21.2712301573466,0.));
#206451=CARTESIAN_POINT('Ctrl Pts',(-7.52682526918541,21.2742366113579,
0.));
#206452=CARTESIAN_POINT('Ctrl Pts',(-7.52787386225333,21.2775925269652,
0.));
#206453=CARTESIAN_POINT('Ctrl Pts',(-7.52901217930408,21.2812902781143,
0.));
#206454=CARTESIAN_POINT('Ctrl Pts',(-7.53023562438229,21.2853226580657,
0.));
#206455=CARTESIAN_POINT('Ctrl Pts',(-7.53153906987855,21.2896816163842,
0.));
#206456=CARTESIAN_POINT('Ctrl Pts',(-7.53291726078527,21.2943588989331,
0.));
#206457=CARTESIAN_POINT('Ctrl Pts',(-7.53436505309943,21.2993464250717,
0.));
#206458=CARTESIAN_POINT('Ctrl Pts',(-7.53587778251736,21.3046368712157,
0.));
#206459=CARTESIAN_POINT('Ctrl Pts',(-7.53745129364616,21.310223716773,0.));
#206460=CARTESIAN_POINT('Ctrl Pts',(-7.53908175169898,21.3161009456256,
0.));
#206461=CARTESIAN_POINT('Ctrl Pts',(-7.54076552038279,21.3222628524165,
0.));
#206462=CARTESIAN_POINT('Ctrl Pts',(-7.54249900377031,21.328703791771,0.));
#206463=CARTESIAN_POINT('Ctrl Pts',(-7.54427868151268,21.3354182340149,
0.));
#206464=CARTESIAN_POINT('Ctrl Pts',(-7.54610114948347,21.3424008295038,
0.));
#206465=CARTESIAN_POINT('Ctrl Pts',(-7.5479631624633,21.3496464761531,0.));
#206466=CARTESIAN_POINT('Ctrl Pts',(-7.5498616652131,21.3571503685855,0.));
#206467=CARTESIAN_POINT('Ctrl Pts',(-7.55179375777444,21.3649079431865,
0.));
#206468=CARTESIAN_POINT('Ctrl Pts',(-7.55375667080029,21.3729148390243,
0.));
#206469=CARTESIAN_POINT('Ctrl Pts',(-7.55574773403503,21.3811668478932,
0.));
#206470=CARTESIAN_POINT('Ctrl Pts',(-7.55776435731417,21.3896598842117,
0.));
#206471=CARTESIAN_POINT('Ctrl Pts',(-7.55980403700611,21.3983899952987,
0.));
#206472=CARTESIAN_POINT('Ctrl Pts',(-7.56186435703622,21.4073533630365,
0.));
#206473=CARTESIAN_POINT('Ctrl Pts',(-7.56394299313685,21.4165463106254,
0.));
#206474=CARTESIAN_POINT('Ctrl Pts',(-7.56603771218712,21.4259653015736,
0.));
#206475=CARTESIAN_POINT('Ctrl Pts',(-7.56814636360847,21.4356069261513,
0.));
#206476=CARTESIAN_POINT('Ctrl Pts',(-7.57026687261166,21.4454678907509,
0.));
#206477=CARTESIAN_POINT('Ctrl Pts',(-7.57239723223506,21.4555450053142,
0.));
#206478=CARTESIAN_POINT('Ctrl Pts',(-7.57453549743412,21.4658351740128,
0.));
#206479=CARTESIAN_POINT('Ctrl Pts',(-7.57667978402987,21.4763353936762,
0.));
#206480=CARTESIAN_POINT('Ctrl Pts',(-7.57882826679132,21.4870427508194,
0.));
#206481=CARTESIAN_POINT('Ctrl Pts',(-7.58097917790744,21.4979544192744,
0.));
#206482=CARTESIAN_POINT('Ctrl Pts',(-7.5831308051918,21.5090676573873,0.));
#206483=CARTESIAN_POINT('Ctrl Pts',(-7.5852814891913,21.5203798035299,0.));
#206484=CARTESIAN_POINT('Ctrl Pts',(-7.58742962034834,21.5318882716736,
0.));
#206485=CARTESIAN_POINT('Ctrl Pts',(-7.58957363620014,21.543590547011,0.));
#206486=CARTESIAN_POINT('Ctrl Pts',(-7.59171201844777,21.5554841813462,
0.));
#206487=CARTESIAN_POINT('Ctrl Pts',(-7.59384329124918,21.5675667904726,
0.));
#206488=CARTESIAN_POINT('Ctrl Pts',(-7.59596601973584,21.5798360518978,
0.));
#206489=CARTESIAN_POINT('Ctrl Pts',(-7.59807880846195,21.5922897024466,
0.));
#206490=CARTESIAN_POINT('Ctrl Pts',(-7.60018029988241,21.6049255358843,
0.));
#206491=CARTESIAN_POINT('Ctrl Pts',(-7.60226917285429,21.617741400599,0.));
#206492=CARTESIAN_POINT('Ctrl Pts',(-7.60434414118296,21.6307351973822,
0.));
#206493=CARTESIAN_POINT('Ctrl Pts',(-7.60640395216357,21.6439048771743,
0.));
#206494=CARTESIAN_POINT('Ctrl Pts',(-7.60844738512874,21.6572484388081,
0.));
#206495=CARTESIAN_POINT('Ctrl Pts',(-7.61047325000956,21.6707639267576,
0.));
#206496=CARTESIAN_POINT('Ctrl Pts',(-7.61248038630268,21.6844494295815,
0.));
#206497=CARTESIAN_POINT('Ctrl Pts',(-7.61446766202787,21.6983030783322,
0.));
#206498=CARTESIAN_POINT('Ctrl Pts',(-7.61643397270421,21.7123230449834,
0.));
#206499=CARTESIAN_POINT('Ctrl Pts',(-7.61837824030538,21.7265075407975,
0.));
#206500=CARTESIAN_POINT('Ctrl Pts',(-7.62029941230855,21.7408548148656,
0.));
#206501=CARTESIAN_POINT('Ctrl Pts',(-7.62219646084228,21.7553631528328,
0.));
#206502=CARTESIAN_POINT('Ctrl Pts',(-7.62406838181166,21.7700308755584,
0.));
#206503=CARTESIAN_POINT('Ctrl Pts',(-7.62591419404512,21.7848563378021,
0.));
#206504=CARTESIAN_POINT('Ctrl Pts',(-7.62773293842389,21.799837926858,0.));
#206505=CARTESIAN_POINT('Ctrl Pts',(-7.62952367718127,21.814974061509,0.));
#206506=CARTESIAN_POINT('Ctrl Pts',(-7.63128549323023,21.8302631910195,
0.));
#206507=CARTESIAN_POINT('Ctrl Pts',(-7.63301748948936,21.8457037941084,
0.));
#206508=CARTESIAN_POINT('Ctrl Pts',(-7.63471878821226,21.8612943779089,
0.));
#206509=CARTESIAN_POINT('Ctrl Pts',(-7.636388530334,21.8770334769496,0.));
#206510=CARTESIAN_POINT('Ctrl Pts',(-7.63802587492035,21.8929196523514,
0.));
#206511=CARTESIAN_POINT('Ctrl Pts',(-7.63962999860927,21.9089514909874,
0.));
#206512=CARTESIAN_POINT('Ctrl Pts',(-7.64120009506532,21.9251276046546,
0.));
#206513=CARTESIAN_POINT('Ctrl Pts',(-7.64273537442682,21.9414466292072,
0.));
#206514=CARTESIAN_POINT('Ctrl Pts',(-7.64423506279123,21.9579072237651,
0.));
#206515=CARTESIAN_POINT('Ctrl Pts',(-7.64569840177336,21.9745080700798,
0.));
#206516=CARTESIAN_POINT('Ctrl Pts',(-7.6471246480525,21.9912478718542,0.));
#206517=CARTESIAN_POINT('Ctrl Pts',(-7.64851307293352,22.0081253540774,
0.));
#206518=CARTESIAN_POINT('Ctrl Pts',(-7.64986296190168,22.0251392623209,
0.));
#206519=CARTESIAN_POINT('Ctrl Pts',(-7.65117361421358,22.0422883621174,
0.));
#206520=CARTESIAN_POINT('Ctrl Pts',(-7.65244434253113,22.0595714384431,
0.));
#206521=CARTESIAN_POINT('Ctrl Pts',(-7.65367447254949,22.0769872951596,
0.));
#206522=CARTESIAN_POINT('Ctrl Pts',(-7.65486334263644,22.094534754469,0.));
#206523=CARTESIAN_POINT('Ctrl Pts',(-7.65601030346807,22.1122126563329,
0.));
#206524=CARTESIAN_POINT('Ctrl Pts',(-7.65711471769397,22.1300198579675,
0.));
#206525=CARTESIAN_POINT('Ctrl Pts',(-7.65817595963349,22.1479552334211,
0.));
#206526=CARTESIAN_POINT('Ctrl Pts',(-7.6591934149693,22.1660176731178,0.));
#206527=CARTESIAN_POINT('Ctrl Pts',(-7.66016648045005,22.1842060834091,
0.));
#206528=CARTESIAN_POINT('Ctrl Pts',(-7.66109456359271,22.2025193860964,
0.));
#206529=CARTESIAN_POINT('Ctrl Pts',(-7.661977082404,22.2209565180085,0.));
#206530=CARTESIAN_POINT('Ctrl Pts',(-7.66281346512509,22.2395164306547,
0.));
#206531=CARTESIAN_POINT('Ctrl Pts',(-7.66360314997641,22.258198089848,0.));
#206532=CARTESIAN_POINT('Ctrl Pts',(-7.66434558490979,22.2770004753335,
0.));
#206533=CARTESIAN_POINT('Ctrl Pts',(-7.66504022736299,22.2959225803937,
0.));
#206534=CARTESIAN_POINT('Ctrl Pts',(-7.66568654402494,22.314963411484,0.));
#206535=CARTESIAN_POINT('Ctrl Pts',(-7.66628401061952,22.3341219879469,
0.));
#206536=CARTESIAN_POINT('Ctrl Pts',(-7.66683211169158,22.3533973417021,
0.));
#206537=CARTESIAN_POINT('Ctrl Pts',(-7.66733034039883,22.372788516936,0.));
#206538=CARTESIAN_POINT('Ctrl Pts',(-7.6677781983079,22.3922945697773,0.));
#206539=CARTESIAN_POINT('Ctrl Pts',(-7.6681751951964,22.4119145679758,0.));
#206540=CARTESIAN_POINT('Ctrl Pts',(-7.66852084886704,22.4316475906603,
0.));
#206541=CARTESIAN_POINT('Ctrl Pts',(-7.66881468496635,22.4514927280855,
0.));
#206542=CARTESIAN_POINT('Ctrl Pts',(-7.66905623680831,22.47144908137,0.));
#206543=CARTESIAN_POINT('Ctrl Pts',(-7.66924504520315,22.4915157622312,
0.));
#206544=CARTESIAN_POINT('Ctrl Pts',(-7.66938065829108,22.5116918927031,
0.));
#206545=CARTESIAN_POINT('Ctrl Pts',(-7.66946263138144,22.53197660492,0.));
#206546=CARTESIAN_POINT('Ctrl Pts',(-7.66949052679693,22.5523690409116,
0.));
#206547=CARTESIAN_POINT('Ctrl Pts',(-7.66946391372306,22.5728683523831,
0.));
#206548=CARTESIAN_POINT('Ctrl Pts',(-7.66938236806233,22.5934737004953,
0.));
#206549=CARTESIAN_POINT('Ctrl Pts',(-7.66924547229414,22.6141842556243,
0.));
#206550=CARTESIAN_POINT('Ctrl Pts',(-7.66905281533715,22.6349991971541,
0.));
#206551=CARTESIAN_POINT('Ctrl Pts',(-7.66880399241323,22.6559177133127,
0.));
#206552=CARTESIAN_POINT('Ctrl Pts',(-7.66849860491743,22.6769390009885,
0.));
#206553=CARTESIAN_POINT('Ctrl Pts',(-7.66813626029275,22.6980622655446,
0.));
#206554=CARTESIAN_POINT('Ctrl Pts',(-7.66771657191027,22.7192867206245,
0.));
#206555=CARTESIAN_POINT('Ctrl Pts',(-7.6672391589544,22.7406115879513,0.));
#206556=CARTESIAN_POINT('Ctrl Pts',(-7.66670364630299,22.7620360971843,
0.));
#206557=CARTESIAN_POINT('Ctrl Pts',(-7.66610966441273,22.7835594857699,
0.));
#206558=CARTESIAN_POINT('Ctrl Pts',(-7.66545684920987,22.8051809987833,
0.));
#206559=CARTESIAN_POINT('Ctrl Pts',(-7.66474484198549,22.8268998887678,
0.));
#206560=CARTESIAN_POINT('Ctrl Pts',(-7.66397328929803,22.848715415557,0.));
#206561=CARTESIAN_POINT('Ctrl Pts',(-7.66314184287337,22.8706268461283,
0.));
#206562=CARTESIAN_POINT('Ctrl Pts',(-7.66225015950156,22.8926334544883,
0.));
#206563=CARTESIAN_POINT('Ctrl Pts',(-7.66129790094108,22.9147345215421,
0.));
#206564=CARTESIAN_POINT('Ctrl Pts',(-7.66028473382778,22.9369293349593,
0.));
#206565=CARTESIAN_POINT('Ctrl Pts',(-7.65921032958902,22.959217189033,0.));
#206566=CARTESIAN_POINT('Ctrl Pts',(-7.65807436436432,22.9815973845296,
0.));
#206567=CARTESIAN_POINT('Ctrl Pts',(-7.65687651891304,23.0040692285814,
0.));
#206568=CARTESIAN_POINT('Ctrl Pts',(-7.65561647852534,23.0266320345787,
0.));
#206569=CARTESIAN_POINT('Ctrl Pts',(-7.65429393293946,23.0492851220528,
0.));
#206570=CARTESIAN_POINT('Ctrl Pts',(-7.65290857626358,23.072027816555,0.));
#206571=CARTESIAN_POINT('Ctrl Pts',(-7.65146010690476,23.094859449525,0.));
#206572=CARTESIAN_POINT('Ctrl Pts',(-7.6499482274986,23.1177793581679,0.));
#206573=CARTESIAN_POINT('Ctrl Pts',(-7.64837264482943,23.1407868853819,
0.));
#206574=CARTESIAN_POINT('Ctrl Pts',(-7.64673306975805,23.1638813796694,
0.));
#206575=CARTESIAN_POINT('Ctrl Pts',(-7.64502921715483,23.1870621950452,
0.));
#206576=CARTESIAN_POINT('Ctrl Pts',(-7.6432608058368,23.2103286909398,0.));
#206577=CARTESIAN_POINT('Ctrl Pts',(-7.64142755851504,23.2336802320912,
0.));
#206578=CARTESIAN_POINT('Ctrl Pts',(-7.63952920172835,23.2571161884488,
0.));
#206579=CARTESIAN_POINT('Ctrl Pts',(-7.63756546576374,23.2806359350855,
0.));
#206580=CARTESIAN_POINT('Ctrl Pts',(-7.63553608458783,23.3042388521022,
0.));
#206581=CARTESIAN_POINT('Ctrl Pts',(-7.63344079578161,23.3279243245241,
0.));
#206582=CARTESIAN_POINT('Ctrl Pts',(-7.63127934048136,23.3516917421972,
0.));
#206583=CARTESIAN_POINT('Ctrl Pts',(-7.62905146332593,23.3755404996636,
0.));
#206584=CARTESIAN_POINT('Ctrl Pts',(-7.62675691240329,23.399469996112,0.));
#206585=CARTESIAN_POINT('Ctrl Pts',(-7.6243954392005,23.4234796353542,0.));
#206586=CARTESIAN_POINT('Ctrl Pts',(-7.62196679855955,23.4475688257854,
0.));
#206587=CARTESIAN_POINT('Ctrl Pts',(-7.61947074863977,23.4717369803438,
0.));
#206588=CARTESIAN_POINT('Ctrl Pts',(-7.61690705088319,23.4959835164609,
0.));
#206589=CARTESIAN_POINT('Ctrl Pts',(-7.61427546999298,23.5203078560129,
0.));
#206590=CARTESIAN_POINT('Ctrl Pts',(-7.61157577385372,23.544709425203,0.));
#206591=CARTESIAN_POINT('Ctrl Pts',(-7.608807733446,23.5691876544244,0.));
#206592=CARTESIAN_POINT('Ctrl Pts',(-7.60597112277094,23.5937419781245,
0.));
#206593=CARTESIAN_POINT('Ctrl Pts',(-7.60306571877806,23.6183718346576,
0.));
#206594=CARTESIAN_POINT('Ctrl Pts',(-7.60009130130126,23.6430766661418,
0.));
#206595=CARTESIAN_POINT('Ctrl Pts',(-7.59704765299567,23.6678559182875,
0.));
#206596=CARTESIAN_POINT('Ctrl Pts',(-7.59393455934035,23.6927090405066,
0.));
#206597=CARTESIAN_POINT('Ctrl Pts',(-7.5907518086532,23.7176354860456,0.));
#206598=CARTESIAN_POINT('Ctrl Pts',(-7.58749919210826,23.7426347121006,
0.));
#206599=CARTESIAN_POINT('Ctrl Pts',(-7.58417650376271,23.7677061799376,
0.));
#206600=CARTESIAN_POINT('Ctrl Pts',(-7.58078354058213,23.7928493549908,
0.));
#206601=CARTESIAN_POINT('Ctrl Pts',(-7.57732010249066,23.8180637069976,
0.));
#206602=CARTESIAN_POINT('Ctrl Pts',(-7.57378599219814,23.8433487096132,
0.));
#206603=CARTESIAN_POINT('Ctrl Pts',(-7.57018101500709,23.8687038399595,
0.));
#206604=CARTESIAN_POINT('Ctrl Pts',(-7.56650497863791,23.8941285782002,
0.));
#206605=CARTESIAN_POINT('Ctrl Pts',(-7.56275769304773,23.9196224070759,
0.));
#206606=CARTESIAN_POINT('Ctrl Pts',(-7.5589389702768,23.9451848115002,0.));
#206607=CARTESIAN_POINT('Ctrl Pts',(-7.55504862424808,23.9708152779886,
0.));
#206608=CARTESIAN_POINT('Ctrl Pts',(-7.55108647097432,23.9965132953187,
0.));
#206609=CARTESIAN_POINT('Ctrl Pts',(-7.54705232885895,24.0222783554531,
0.));
#206610=CARTESIAN_POINT('Ctrl Pts',(-7.54294601896128,24.0481099543353,
0.));
#206611=CARTESIAN_POINT('Ctrl Pts',(-7.53876736531005,24.0740075927984,
0.));
#206612=CARTESIAN_POINT('Ctrl Pts',(-7.53451619514658,24.0999707772643,
0.));
#206613=CARTESIAN_POINT('Ctrl Pts',(-7.53019233935536,24.1259990209211,
0.));
#206614=CARTESIAN_POINT('Ctrl Pts',(-7.52579563201479,24.152091842537,0.));
#206615=CARTESIAN_POINT('Ctrl Pts',(-7.52132590953862,24.1782487641602,
0.));
#206616=CARTESIAN_POINT('Ctrl Pts',(-7.51678300997998,24.2044693092356,
0.));
#206617=CARTESIAN_POINT('Ctrl Pts',(-7.51216677222199,24.230753000389,0.));
#206618=CARTESIAN_POINT('Ctrl Pts',(-7.50747703535115,24.2570993577032,
0.));
#206619=CARTESIAN_POINT('Ctrl Pts',(-7.50271363765098,24.2835078958966,
0.));
#206620=CARTESIAN_POINT('Ctrl Pts',(-7.49787641695359,24.3099781253345,
0.));
#206621=CARTESIAN_POINT('Ctrl Pts',(-7.4929652125233,24.3365095573673,0.));
#206622=CARTESIAN_POINT('Ctrl Pts',(-7.48797986651828,24.3631017084513,
0.));
#206623=CARTESIAN_POINT('Ctrl Pts',(-7.48292022569254,24.3897541049248,
0.));
#206624=CARTESIAN_POINT('Ctrl Pts',(-7.47778614286573,24.4164662871165,
0.));
#206625=CARTESIAN_POINT('Ctrl Pts',(-7.47257747883319,24.4432378146501,
0.));
#206626=CARTESIAN_POINT('Ctrl Pts',(-7.46729410308923,24.4700682684544,
0.));
#206627=CARTESIAN_POINT('Ctrl Pts',(-7.46193588961642,24.4969572391509,
0.));
#206628=CARTESIAN_POINT('Ctrl Pts',(-7.45650271336045,24.52390431731,0.));
#206629=CARTESIAN_POINT('Ctrl Pts',(-7.45099444651296,24.5509090831579,
0.));
#206630=CARTESIAN_POINT('Ctrl Pts',(-7.44541095473163,24.5779710960865,
0.));
#206631=CARTESIAN_POINT('Ctrl Pts',(-7.43975209375375,24.6050898852349,
0.));
#206632=CARTESIAN_POINT('Ctrl Pts',(-7.4340177048922,24.6322649369472,0.));
#206633=CARTESIAN_POINT('Ctrl Pts',(-7.42820762158681,24.659495712869,0.));
#206634=CARTESIAN_POINT('Ctrl Pts',(-7.42232167765763,24.6867816727118,
0.));
#206635=CARTESIAN_POINT('Ctrl Pts',(-7.41635971481243,24.7141222949988,
0.));
#206636=CARTESIAN_POINT('Ctrl Pts',(-7.41032159082173,24.7415170994754,
0.));
#206637=CARTESIAN_POINT('Ctrl Pts',(-7.40420718661754,24.7689656669005,
0.));
#206638=CARTESIAN_POINT('Ctrl Pts',(-7.39801641583612,24.7964676646518,
0.));
#206639=CARTESIAN_POINT('Ctrl Pts',(-7.39174922586841,24.8240228521042,
0.));
#206640=CARTESIAN_POINT('Ctrl Pts',(-7.38540558904946,24.8516310625367,
0.));
#206641=CARTESIAN_POINT('Ctrl Pts',(-7.3789854964161,24.8792921911309,0.));
#206642=CARTESIAN_POINT('Ctrl Pts',(-7.37378825962718,24.9014633826201,
0.));
#206643=CARTESIAN_POINT('Ctrl Pts',(-7.36985593120696,24.9181155530631,
0.));
#206644=CARTESIAN_POINT('Ctrl Pts',(-7.3672190902906,24.9292275670705,0.));
#206645=CARTESIAN_POINT('Ctrl Pts',(-7.36589684767344,24.9347862158358,
0.));
#206646=CARTESIAN_POINT('',(-7.36589684767344,24.9347862158358,0.));
#206647=CARTESIAN_POINT('Origin',(-1.68110656504246,21.4341755315424,0.));
#206648=CARTESIAN_POINT('',(-1.76341220531179,22.4835757167854,0.));
#206649=CARTESIAN_POINT('',(-1.76341220531179,22.4835757167854,0.));
#206650=CARTESIAN_POINT('',(-0.840553282521227,10.7170877657712,0.));
#206651=CARTESIAN_POINT('Ctrl Pts',(-6.08833931617698,25.2771067246846,
0.));
#206652=CARTESIAN_POINT('Ctrl Pts',(-6.08833931617698,25.2771067246846,
12.));
#206653=CARTESIAN_POINT('Ctrl Pts',(-6.08441489609824,25.2729539149479,
0.));
#206654=CARTESIAN_POINT('Ctrl Pts',(-6.08441489609824,25.2729539149479,
12.));
#206655=CARTESIAN_POINT('Ctrl Pts',(-6.07657531787578,25.2646490489816,
0.));
#206656=CARTESIAN_POINT('Ctrl Pts',(-6.07657531787578,25.2646490489816,
12.));
#206657=CARTESIAN_POINT('Ctrl Pts',(-6.06484373634697,25.2521940105523,
0.));
#206658=CARTESIAN_POINT('Ctrl Pts',(-6.06484373634697,25.2521940105523,
12.));
#206659=CARTESIAN_POINT('Ctrl Pts',(-6.04925720151412,25.2355918138798,
0.));
#206660=CARTESIAN_POINT('Ctrl Pts',(-6.04925720151412,25.2355918138798,
12.));
#206661=CARTESIAN_POINT('Ctrl Pts',(-6.02986667390187,25.2148466201368,
0.));
#206662=CARTESIAN_POINT('Ctrl Pts',(-6.02986667390187,25.2148466201368,
12.));
#206663=CARTESIAN_POINT('Ctrl Pts',(-6.0105688180476,25.1941090269638,0.));
#206664=CARTESIAN_POINT('Ctrl Pts',(-6.0105688180476,25.1941090269638,12.));
#206665=CARTESIAN_POINT('Ctrl Pts',(-5.99136367859838,25.1733791296154,
0.));
#206666=CARTESIAN_POINT('Ctrl Pts',(-5.99136367859838,25.1733791296154,
12.));
#206667=CARTESIAN_POINT('Ctrl Pts',(-5.97225131495636,25.1526570863065,
0.));
#206668=CARTESIAN_POINT('Ctrl Pts',(-5.97225131495636,25.1526570863065,
12.));
#206669=CARTESIAN_POINT('Ctrl Pts',(-5.95323180187348,25.1319431317273,
0.));
#206670=CARTESIAN_POINT('Ctrl Pts',(-5.95323180187348,25.1319431317273,
12.));
#206671=CARTESIAN_POINT('Ctrl Pts',(-5.93430523086776,25.1112375971182,
0.));
#206672=CARTESIAN_POINT('Ctrl Pts',(-5.93430523086776,25.1112375971182,
12.));
#206673=CARTESIAN_POINT('Ctrl Pts',(-5.91547170844382,25.0905409050863,
0.));
#206674=CARTESIAN_POINT('Ctrl Pts',(-5.91547170844382,25.0905409050863,
12.));
#206675=CARTESIAN_POINT('Ctrl Pts',(-5.89673135155459,25.0698535426593,
0.));
#206676=CARTESIAN_POINT('Ctrl Pts',(-5.89673135155459,25.0698535426593,
12.));
#206677=CARTESIAN_POINT('Ctrl Pts',(-5.87808428385329,25.0491760405965,
0.));
#206678=CARTESIAN_POINT('Ctrl Pts',(-5.87808428385329,25.0491760405965,
12.));
#206679=CARTESIAN_POINT('Ctrl Pts',(-5.8595306315681,25.0285089498922,0.));
#206680=CARTESIAN_POINT('Ctrl Pts',(-5.8595306315681,25.0285089498922,12.));
#206681=CARTESIAN_POINT('Ctrl Pts',(-5.84107051963073,25.0078528200558,
0.));
#206682=CARTESIAN_POINT('Ctrl Pts',(-5.84107051963073,25.0078528200558,
12.));
#206683=CARTESIAN_POINT('Ctrl Pts',(-5.82270406744214,24.9872081752709,
0.));
#206684=CARTESIAN_POINT('Ctrl Pts',(-5.82270406744214,24.9872081752709,
12.));
#206685=CARTESIAN_POINT('Ctrl Pts',(-5.80443138549747,24.9665754954462,
0.));
#206686=CARTESIAN_POINT('Ctrl Pts',(-5.80443138549747,24.9665754954462,
12.));
#206687=CARTESIAN_POINT('Ctrl Pts',(-5.78625257775703,24.9459552293308,
0.));
#206688=CARTESIAN_POINT('Ctrl Pts',(-5.78625257775703,24.9459552293308,
12.));
#206689=CARTESIAN_POINT('Ctrl Pts',(-5.76816774342236,24.9253478043632,
0.));
#206690=CARTESIAN_POINT('Ctrl Pts',(-5.76816774342236,24.9253478043632,
12.));
#206691=CARTESIAN_POINT('Ctrl Pts',(-5.75017697890813,24.9047536376467,
0.));
#206692=CARTESIAN_POINT('Ctrl Pts',(-5.75017697890813,24.9047536376467,
12.));
#206693=CARTESIAN_POINT('Ctrl Pts',(-5.73228037976927,24.8841731467219,
0.));
#206694=CARTESIAN_POINT('Ctrl Pts',(-5.73228037976927,24.8841731467219,
12.));
#206695=CARTESIAN_POINT('Ctrl Pts',(-5.71447804252019,24.8636067597677,
0.));
#206696=CARTESIAN_POINT('Ctrl Pts',(-5.71447804252019,24.8636067597677,
12.));
#206697=CARTESIAN_POINT('Ctrl Pts',(-5.69677006679429,24.8430549277634,
0.));
#206698=CARTESIAN_POINT('Ctrl Pts',(-5.69677006679429,24.8430549277634,
12.));
#206699=CARTESIAN_POINT('Ctrl Pts',(-5.67915655496524,24.822518122386,0.));
#206700=CARTESIAN_POINT('Ctrl Pts',(-5.67915655496524,24.822518122386,12.));
#206701=CARTESIAN_POINT('Ctrl Pts',(-5.66163761114903,24.8019968304618,
0.));
#206702=CARTESIAN_POINT('Ctrl Pts',(-5.66163761114903,24.8019968304618,
12.));
#206703=CARTESIAN_POINT('Ctrl Pts',(-5.64421334042248,24.7814915496728,
0.));
#206704=CARTESIAN_POINT('Ctrl Pts',(-5.64421334042248,24.7814915496728,
12.));
#206705=CARTESIAN_POINT('Ctrl Pts',(-5.62688384790919,24.76100278357,0.));
#206706=CARTESIAN_POINT('Ctrl Pts',(-5.62688384790919,24.76100278357,12.));
#206707=CARTESIAN_POINT('Ctrl Pts',(-5.60964923798495,24.7405310372736,
0.));
#206708=CARTESIAN_POINT('Ctrl Pts',(-5.60964923798495,24.7405310372736,
12.));
#206709=CARTESIAN_POINT('Ctrl Pts',(-5.59250961323995,24.7200768119079,
0.));
#206710=CARTESIAN_POINT('Ctrl Pts',(-5.59250961323995,24.7200768119079,
12.));
#206711=CARTESIAN_POINT('Ctrl Pts',(-5.57546507427767,24.6996406035507,
0.));
#206712=CARTESIAN_POINT('Ctrl Pts',(-5.57546507427767,24.6996406035507,
12.));
#206713=CARTESIAN_POINT('Ctrl Pts',(-5.55851572025389,24.6792229061785,
0.));
#206714=CARTESIAN_POINT('Ctrl Pts',(-5.55851572025389,24.6792229061785,
12.));
#206715=CARTESIAN_POINT('Ctrl Pts',(-5.54166164919593,24.6588242134733,
0.));
#206716=CARTESIAN_POINT('Ctrl Pts',(-5.54166164919593,24.6588242134733,
12.));
#206717=CARTESIAN_POINT('Ctrl Pts',(-5.52490295840996,24.6384450211466,
0.));
#206718=CARTESIAN_POINT('Ctrl Pts',(-5.52490295840996,24.6384450211466,
12.));
#206719=CARTESIAN_POINT('Ctrl Pts',(-5.50823974481959,24.618085828918,0.));
#206720=CARTESIAN_POINT('Ctrl Pts',(-5.50823974481959,24.618085828918,12.));
#206721=CARTESIAN_POINT('Ctrl Pts',(-5.49167210537235,24.5977471429365,
0.));
#206722=CARTESIAN_POINT('Ctrl Pts',(-5.49167210537235,24.5977471429365,
12.));
#206723=CARTESIAN_POINT('Ctrl Pts',(-5.47520013724403,24.5774294770329,
0.));
#206724=CARTESIAN_POINT('Ctrl Pts',(-5.47520013724403,24.5774294770329,
12.));
#206725=CARTESIAN_POINT('Ctrl Pts',(-5.45882393762244,24.5571333514841,
0.));
#206726=CARTESIAN_POINT('Ctrl Pts',(-5.45882393762244,24.5571333514841,
12.));
#206727=CARTESIAN_POINT('Ctrl Pts',(-5.44254360356865,24.5368592922861,
0.));
#206728=CARTESIAN_POINT('Ctrl Pts',(-5.44254360356865,24.5368592922861,
12.));
#206729=CARTESIAN_POINT('Ctrl Pts',(-5.42635923183411,24.5166078302107,
0.));
#206730=CARTESIAN_POINT('Ctrl Pts',(-5.42635923183411,24.5166078302107,
12.));
#206731=CARTESIAN_POINT('Ctrl Pts',(-5.41027091869242,24.4963794999831,
0.));
#206732=CARTESIAN_POINT('Ctrl Pts',(-5.41027091869242,24.4963794999831,
12.));
#206733=CARTESIAN_POINT('Ctrl Pts',(-5.3942787597383,24.4761748393322,0.));
#206734=CARTESIAN_POINT('Ctrl Pts',(-5.3942787597383,24.4761748393322,12.));
#206735=CARTESIAN_POINT('Ctrl Pts',(-5.37838284973706,24.4559943883159,
0.));
#206736=CARTESIAN_POINT('Ctrl Pts',(-5.37838284973706,24.4559943883159,
12.));
#206737=CARTESIAN_POINT('Ctrl Pts',(-5.36258328273639,24.4358386899152,
0.));
#206738=CARTESIAN_POINT('Ctrl Pts',(-5.36258328273639,24.4358386899152,
12.));
#206739=CARTESIAN_POINT('Ctrl Pts',(-5.34688015213546,24.4157082904615,
0.));
#206740=CARTESIAN_POINT('Ctrl Pts',(-5.34688015213546,24.4157082904615,
12.));
#206741=CARTESIAN_POINT('Ctrl Pts',(-5.33127355076037,24.3956037401293,
0.));
#206742=CARTESIAN_POINT('Ctrl Pts',(-5.33127355076037,24.3956037401293,
12.));
#206743=CARTESIAN_POINT('Ctrl Pts',(-5.31576357092524,24.3755255933917,
0.));
#206744=CARTESIAN_POINT('Ctrl Pts',(-5.31576357092524,24.3755255933917,
12.));
#206745=CARTESIAN_POINT('Ctrl Pts',(-5.30035030449059,24.3554744095075,
0.));
#206746=CARTESIAN_POINT('Ctrl Pts',(-5.30035030449059,24.3554744095075,
12.));
#206747=CARTESIAN_POINT('Ctrl Pts',(-5.28503384290644,24.3354507529415,
0.));
#206748=CARTESIAN_POINT('Ctrl Pts',(-5.28503384290644,24.3354507529415,
12.));
#206749=CARTESIAN_POINT('Ctrl Pts',(-5.26981427718796,24.3154551932222,
0.));
#206750=CARTESIAN_POINT('Ctrl Pts',(-5.26981427718796,24.3154551932222,
12.));
#206751=CARTESIAN_POINT('Ctrl Pts',(-5.25469169788856,24.2954883048448,
0.));
#206752=CARTESIAN_POINT('Ctrl Pts',(-5.25469169788856,24.2954883048448,
12.));
#206753=CARTESIAN_POINT('Ctrl Pts',(-5.23966619506289,24.2755506671526,
0.));
#206754=CARTESIAN_POINT('Ctrl Pts',(-5.23966619506289,24.2755506671526,
12.));
#206755=CARTESIAN_POINT('Ctrl Pts',(-5.22473785822441,24.2556428642294,
0.));
#206756=CARTESIAN_POINT('Ctrl Pts',(-5.22473785822441,24.2556428642294,
12.));
#206757=CARTESIAN_POINT('Ctrl Pts',(-5.20990677629173,24.2357654847765,
0.));
#206758=CARTESIAN_POINT('Ctrl Pts',(-5.20990677629173,24.2357654847765,
12.));
#206759=CARTESIAN_POINT('Ctrl Pts',(-5.19517303753643,24.215919122017,0.));
#206760=CARTESIAN_POINT('Ctrl Pts',(-5.19517303753643,24.215919122017,12.));
#206761=CARTESIAN_POINT('Ctrl Pts',(-5.18053672961392,24.1961043738754,
0.));
#206762=CARTESIAN_POINT('Ctrl Pts',(-5.18053672961392,24.1961043738754,
12.));
#206763=CARTESIAN_POINT('Ctrl Pts',(-5.16599793957979,24.1763218431343,
0.));
#206764=CARTESIAN_POINT('Ctrl Pts',(-5.16599793957979,24.1763218431343,
12.));
#206765=CARTESIAN_POINT('Ctrl Pts',(-5.15155675390075,24.156572137597,0.));
#206766=CARTESIAN_POINT('Ctrl Pts',(-5.15155675390075,24.156572137597,12.));
#206767=CARTESIAN_POINT('Ctrl Pts',(-5.13721325845745,24.1368558702443,
0.));
#206768=CARTESIAN_POINT('Ctrl Pts',(-5.13721325845745,24.1368558702443,
12.));
#206769=CARTESIAN_POINT('Ctrl Pts',(-5.12296753853859,24.117173659394,0.));
#206770=CARTESIAN_POINT('Ctrl Pts',(-5.12296753853859,24.117173659394,12.));
#206771=CARTESIAN_POINT('Ctrl Pts',(-5.10881967883132,24.0975261288446,
0.));
#206772=CARTESIAN_POINT('Ctrl Pts',(-5.10881967883132,24.0975261288446,
12.));
#206773=CARTESIAN_POINT('Ctrl Pts',(-5.09476976342625,24.0779139079266,
0.));
#206774=CARTESIAN_POINT('Ctrl Pts',(-5.09476976342625,24.0779139079266,
12.));
#206775=CARTESIAN_POINT('Ctrl Pts',(-5.08081787581276,24.0583376315638,
0.));
#206776=CARTESIAN_POINT('Ctrl Pts',(-5.08081787581276,24.0583376315638,
12.));
#206777=CARTESIAN_POINT('Ctrl Pts',(-5.06696409886641,24.0387979403268,
0.));
#206778=CARTESIAN_POINT('Ctrl Pts',(-5.06696409886641,24.0387979403268,
12.));
#206779=CARTESIAN_POINT('Ctrl Pts',(-5.05320851483065,24.0192954804896,
0.));
#206780=CARTESIAN_POINT('Ctrl Pts',(-5.05320851483065,24.0192954804896,
12.));
#206781=CARTESIAN_POINT('Ctrl Pts',(-5.03955120528521,23.9998309040746,
0.));
#206782=CARTESIAN_POINT('Ctrl Pts',(-5.03955120528521,23.9998309040746,
12.));
#206783=CARTESIAN_POINT('Ctrl Pts',(-5.02599225112454,23.9804048689227,
0.));
#206784=CARTESIAN_POINT('Ctrl Pts',(-5.02599225112454,23.9804048689227,
12.));
#206785=CARTESIAN_POINT('Ctrl Pts',(-5.01253173257453,23.9610180388271,
0.));
#206786=CARTESIAN_POINT('Ctrl Pts',(-5.01253173257453,23.9610180388271,
12.));
#206787=CARTESIAN_POINT('Ctrl Pts',(-4.99916972919307,23.9416710836529,
0.));
#206788=CARTESIAN_POINT('Ctrl Pts',(-4.99916972919307,23.9416710836529,
12.));
#206789=CARTESIAN_POINT('Ctrl Pts',(-4.98590631986533,23.9223646794592,
0.));
#206790=CARTESIAN_POINT('Ctrl Pts',(-4.98590631986533,23.9223646794592,
12.));
#206791=CARTESIAN_POINT('Ctrl Pts',(-4.97274158279227,23.9030995086163,
0.));
#206792=CARTESIAN_POINT('Ctrl Pts',(-4.97274158279227,23.9030995086163,
12.));
#206793=CARTESIAN_POINT('Ctrl Pts',(-4.95967559546561,23.8838762599218,
0.));
#206794=CARTESIAN_POINT('Ctrl Pts',(-4.95967559546561,23.8838762599218,
12.));
#206795=CARTESIAN_POINT('Ctrl Pts',(-4.9467084346586,23.8646956287168,0.));
#206796=CARTESIAN_POINT('Ctrl Pts',(-4.9467084346586,23.8646956287168,12.));
#206797=CARTESIAN_POINT('Ctrl Pts',(-4.93384017643432,23.8455583170057,
0.));
#206798=CARTESIAN_POINT('Ctrl Pts',(-4.93384017643432,23.8455583170057,
12.));
#206799=CARTESIAN_POINT('Ctrl Pts',(-4.92107089613969,23.8264650335717,
0.));
#206800=CARTESIAN_POINT('Ctrl Pts',(-4.92107089613969,23.8264650335717,
12.));
#206801=CARTESIAN_POINT('Ctrl Pts',(-4.90840066839344,23.8074164940896,
0.));
#206802=CARTESIAN_POINT('Ctrl Pts',(-4.90840066839344,23.8074164940896,
12.));
#206803=CARTESIAN_POINT('Ctrl Pts',(-4.89582956706775,23.7884134212384,
0.));
#206804=CARTESIAN_POINT('Ctrl Pts',(-4.89582956706775,23.7884134212384,
12.));
#206805=CARTESIAN_POINT('Ctrl Pts',(-4.88335766525573,23.7694565448049,
0.));
#206806=CARTESIAN_POINT('Ctrl Pts',(-4.88335766525573,23.7694565448049,
12.));
#206807=CARTESIAN_POINT('Ctrl Pts',(-4.87098503527152,23.7505466018245,
0.));
#206808=CARTESIAN_POINT('Ctrl Pts',(-4.87098503527152,23.7505466018245,
12.));
#206809=CARTESIAN_POINT('Ctrl Pts',(-4.85871174865499,23.7316843367313,
0.));
#206810=CARTESIAN_POINT('Ctrl Pts',(-4.85871174865499,23.7316843367313,
12.));
#206811=CARTESIAN_POINT('Ctrl Pts',(-4.84653787616425,23.7128705015017,
0.));
#206812=CARTESIAN_POINT('Ctrl Pts',(-4.84653787616425,23.7128705015017,
12.));
#206813=CARTESIAN_POINT('Ctrl Pts',(-4.83446348776266,23.6941058557971,
0.));
#206814=CARTESIAN_POINT('Ctrl Pts',(-4.83446348776266,23.6941058557971,
12.));
#206815=CARTESIAN_POINT('Ctrl Pts',(-4.82248865259562,23.675391167102,0.));
#206816=CARTESIAN_POINT('Ctrl Pts',(-4.82248865259562,23.675391167102,12.));
#206817=CARTESIAN_POINT('Ctrl Pts',(-4.81061343896432,23.6567272108628,
0.));
#206818=CARTESIAN_POINT('Ctrl Pts',(-4.81061343896432,23.6567272108628,
12.));
#206819=CARTESIAN_POINT('Ctrl Pts',(-4.7988379143322,23.6381147706579,0.));
#206820=CARTESIAN_POINT('Ctrl Pts',(-4.7988379143322,23.6381147706579,12.));
#206821=CARTESIAN_POINT('Ctrl Pts',(-4.78716214532098,23.6195546383624,
0.));
#206822=CARTESIAN_POINT('Ctrl Pts',(-4.78716214532098,23.6195546383624,
12.));
#206823=CARTESIAN_POINT('Ctrl Pts',(-4.77558619769872,23.6010476143099,
0.));
#206824=CARTESIAN_POINT('Ctrl Pts',(-4.77558619769872,23.6010476143099,
12.));
#206825=CARTESIAN_POINT('Ctrl Pts',(-4.76411013636251,23.5825945074535,
0.));
#206826=CARTESIAN_POINT('Ctrl Pts',(-4.76411013636251,23.5825945074535,
12.));
#206827=CARTESIAN_POINT('Ctrl Pts',(-4.75273402530617,23.5641961355168,
0.));
#206828=CARTESIAN_POINT('Ctrl Pts',(-4.75273402530617,23.5641961355168,
12.));
#206829=CARTESIAN_POINT('Ctrl Pts',(-4.74145792760698,23.545853325171,0.));
#206830=CARTESIAN_POINT('Ctrl Pts',(-4.74145792760698,23.545853325171,12.));
#206831=CARTESIAN_POINT('Ctrl Pts',(-4.7302819054303,23.5275669122372,0.));
#206832=CARTESIAN_POINT('Ctrl Pts',(-4.7302819054303,23.5275669122372,12.));
#206833=CARTESIAN_POINT('Ctrl Pts',(-4.71920602001902,23.509337741878,0.));
#206834=CARTESIAN_POINT('Ctrl Pts',(-4.71920602001902,23.509337741878,12.));
#206835=CARTESIAN_POINT('Ctrl Pts',(-4.70823033167819,23.491166668789,0.));
#206836=CARTESIAN_POINT('Ctrl Pts',(-4.70823033167819,23.491166668789,12.));
#206837=CARTESIAN_POINT('Ctrl Pts',(-4.69735489975024,23.4730545573853,
0.));
#206838=CARTESIAN_POINT('Ctrl Pts',(-4.69735489975024,23.4730545573853,
12.));
#206839=CARTESIAN_POINT('Ctrl Pts',(-4.68657978258303,23.455002281986,0.));
#206840=CARTESIAN_POINT('Ctrl Pts',(-4.68657978258303,23.455002281986,12.));
#206841=CARTESIAN_POINT('Ctrl Pts',(-4.67590503753058,23.4370107270451,
0.));
#206842=CARTESIAN_POINT('Ctrl Pts',(-4.67590503753058,23.4370107270451,
12.));
#206843=CARTESIAN_POINT('Ctrl Pts',(-4.6653307209467,23.4190807873803,0.));
#206844=CARTESIAN_POINT('Ctrl Pts',(-4.6653307209467,23.4190807873803,12.));
#206845=CARTESIAN_POINT('Ctrl Pts',(-4.65485688816924,23.4012133683959,
0.));
#206846=CARTESIAN_POINT('Ctrl Pts',(-4.65485688816924,23.4012133683959,
12.));
#206847=CARTESIAN_POINT('Ctrl Pts',(-4.6444835934993,23.3834093863068,0.));
#206848=CARTESIAN_POINT('Ctrl Pts',(-4.6444835934993,23.3834093863068,12.));
#206849=CARTESIAN_POINT('Ctrl Pts',(-4.63421089016541,23.3656697683489,
0.));
#206850=CARTESIAN_POINT('Ctrl Pts',(-4.63421089016541,23.3656697683489,
12.));
#206851=CARTESIAN_POINT('Ctrl Pts',(-4.62403883030805,23.3479954530272,
0.));
#206852=CARTESIAN_POINT('Ctrl Pts',(-4.62403883030805,23.3479954530272,
12.));
#206853=CARTESIAN_POINT('Ctrl Pts',(-4.6139674649783,23.3303873903938,0.));
#206854=CARTESIAN_POINT('Ctrl Pts',(-4.6139674649783,23.3303873903938,12.));
#206855=CARTESIAN_POINT('Ctrl Pts',(-4.60399684412163,23.3128465423115,
0.));
#206856=CARTESIAN_POINT('Ctrl Pts',(-4.60399684412163,23.3128465423115,
12.));
#206857=CARTESIAN_POINT('Ctrl Pts',(-4.5941270165575,23.2953738827191,0.));
#206858=CARTESIAN_POINT('Ctrl Pts',(-4.5941270165575,23.2953738827191,12.));
#206859=CARTESIAN_POINT('Ctrl Pts',(-4.5843580299469,23.2779703978876,0.));
#206860=CARTESIAN_POINT('Ctrl Pts',(-4.5843580299469,23.2779703978876,12.));
#206861=CARTESIAN_POINT('Ctrl Pts',(-4.57468993076097,23.2606370866866,
0.));
#206862=CARTESIAN_POINT('Ctrl Pts',(-4.57468993076097,23.2606370866866,
12.));
#206863=CARTESIAN_POINT('Ctrl Pts',(-4.56512276427839,23.2433749609131,
0.));
#206864=CARTESIAN_POINT('Ctrl Pts',(-4.56512276427839,23.2433749609131,
12.));
#206865=CARTESIAN_POINT('Ctrl Pts',(-4.55565657456975,23.2261850456064,
0.));
#206866=CARTESIAN_POINT('Ctrl Pts',(-4.55565657456975,23.2261850456064,
12.));
#206867=CARTESIAN_POINT('Ctrl Pts',(-4.54629140447544,23.2090683793629,
0.));
#206868=CARTESIAN_POINT('Ctrl Pts',(-4.54629140447544,23.2090683793629,
12.));
#206869=CARTESIAN_POINT('Ctrl Pts',(-4.53702729557566,23.1920260146465,
0.));
#206870=CARTESIAN_POINT('Ctrl Pts',(-4.53702729557566,23.1920260146465,
12.));
#206871=CARTESIAN_POINT('Ctrl Pts',(-4.52786428815015,23.1750590180908,
0.));
#206872=CARTESIAN_POINT('Ctrl Pts',(-4.52786428815015,23.1750590180908,
12.));
#206873=CARTESIAN_POINT('Ctrl Pts',(-4.51880242116748,23.1581684708761,
0.));
#206874=CARTESIAN_POINT('Ctrl Pts',(-4.51880242116748,23.1581684708761,
12.));
#206875=CARTESIAN_POINT('Ctrl Pts',(-4.5098417322706,23.1413554691123,0.));
#206876=CARTESIAN_POINT('Ctrl Pts',(-4.5098417322706,23.1413554691123,12.));
#206877=CARTESIAN_POINT('Ctrl Pts',(-4.50098225775171,23.1246211242115,
0.));
#206878=CARTESIAN_POINT('Ctrl Pts',(-4.50098225775171,23.1246211242115,
12.));
#206879=CARTESIAN_POINT('Ctrl Pts',(-4.49222403252216,23.1079665632636,
0.));
#206880=CARTESIAN_POINT('Ctrl Pts',(-4.49222403252216,23.1079665632636,
12.));
#206881=CARTESIAN_POINT('Ctrl Pts',(-4.48356709006788,23.0913929293922,
0.));
#206882=CARTESIAN_POINT('Ctrl Pts',(-4.48356709006788,23.0913929293922,
12.));
#206883=CARTESIAN_POINT('Ctrl Pts',(-4.47501146242856,23.0749013821881,
0.));
#206884=CARTESIAN_POINT('Ctrl Pts',(-4.47501146242856,23.0749013821881,
12.));
#206885=CARTESIAN_POINT('Ctrl Pts',(-4.4665571801823,23.0584930981732,0.));
#206886=CARTESIAN_POINT('Ctrl Pts',(-4.4665571801823,23.0584930981732,12.));
#206887=CARTESIAN_POINT('Ctrl Pts',(-4.45820427241683,23.0421692712467,
0.));
#206888=CARTESIAN_POINT('Ctrl Pts',(-4.45820427241683,23.0421692712467,
12.));
#206889=CARTESIAN_POINT('Ctrl Pts',(-4.44995276669686,23.0259311131392,
0.));
#206890=CARTESIAN_POINT('Ctrl Pts',(-4.44995276669686,23.0259311131392,
12.));
#206891=CARTESIAN_POINT('Ctrl Pts',(-4.44180268901643,23.0097798538395,
0.));
#206892=CARTESIAN_POINT('Ctrl Pts',(-4.44180268901643,23.0097798538395,
12.));
#206893=CARTESIAN_POINT('Ctrl Pts',(-4.43375406376879,22.9937167421006,
0.));
#206894=CARTESIAN_POINT('Ctrl Pts',(-4.43375406376879,22.9937167421006,
12.));
#206895=CARTESIAN_POINT('Ctrl Pts',(-4.42580691372751,22.977743046002,0.));
#206896=CARTESIAN_POINT('Ctrl Pts',(-4.42580691372751,22.977743046002,12.));
#206897=CARTESIAN_POINT('Ctrl Pts',(-4.41796126001302,22.9618600534866,
0.));
#206898=CARTESIAN_POINT('Ctrl Pts',(-4.41796126001302,22.9618600534866,
12.));
#206899=CARTESIAN_POINT('Ctrl Pts',(-4.41021712205553,22.9460690729093,
0.));
#206900=CARTESIAN_POINT('Ctrl Pts',(-4.41021712205553,22.9460690729093,
12.));
#206901=CARTESIAN_POINT('Ctrl Pts',(-4.40257451754323,22.930371433555,0.));
#206902=CARTESIAN_POINT('Ctrl Pts',(-4.40257451754323,22.930371433555,12.));
#206903=CARTESIAN_POINT('Ctrl Pts',(-4.39503346238473,22.9147684862426,
0.));
#206904=CARTESIAN_POINT('Ctrl Pts',(-4.39503346238473,22.9147684862426,
12.));
#206905=CARTESIAN_POINT('Ctrl Pts',(-4.38759397068406,22.8992616040108,
0.));
#206906=CARTESIAN_POINT('Ctrl Pts',(-4.38759397068406,22.8992616040108,
12.));
#206907=CARTESIAN_POINT('Ctrl Pts',(-4.38025605470093,22.8838521827701,
0.));
#206908=CARTESIAN_POINT('Ctrl Pts',(-4.38025605470093,22.8838521827701,
12.));
#206909=CARTESIAN_POINT('Ctrl Pts',(-4.37301972480746,22.8685416419725,
0.));
#206910=CARTESIAN_POINT('Ctrl Pts',(-4.37301972480746,22.8685416419725,
12.));
#206911=CARTESIAN_POINT('Ctrl Pts',(-4.36588498942997,22.8533314252422,
0.));
#206912=CARTESIAN_POINT('Ctrl Pts',(-4.36588498942997,22.8533314252422,
12.));
#206913=CARTESIAN_POINT('Ctrl Pts',(-4.35885185500546,22.8382230011184,
0.));
#206914=CARTESIAN_POINT('Ctrl Pts',(-4.35885185500546,22.8382230011184,
12.));
#206915=CARTESIAN_POINT('Ctrl Pts',(-4.35192032594791,22.8232178638876,
0.));
#206916=CARTESIAN_POINT('Ctrl Pts',(-4.35192032594791,22.8232178638876,
12.));
#206917=CARTESIAN_POINT('Ctrl Pts',(-4.34509040460062,22.8083175343791,
0.));
#206918=CARTESIAN_POINT('Ctrl Pts',(-4.34509040460062,22.8083175343791,
12.));
#206919=CARTESIAN_POINT('Ctrl Pts',(-4.33836209118446,22.7935235607806,
0.));
#206920=CARTESIAN_POINT('Ctrl Pts',(-4.33836209118446,22.7935235607806,
12.));
#206921=CARTESIAN_POINT('Ctrl Pts',(-4.3317353837319,22.7788375194076,0.));
#206922=CARTESIAN_POINT('Ctrl Pts',(-4.3317353837319,22.7788375194076,12.));
#206923=CARTESIAN_POINT('Ctrl Pts',(-4.32521027803754,22.7642610156475,
0.));
#206924=CARTESIAN_POINT('Ctrl Pts',(-4.32521027803754,22.7642610156475,
12.));
#206925=CARTESIAN_POINT('Ctrl Pts',(-4.31878676761235,22.7497956849848,
0.));
#206926=CARTESIAN_POINT('Ctrl Pts',(-4.31878676761235,22.7497956849848,
12.));
#206927=CARTESIAN_POINT('Ctrl Pts',(-4.31246484362549,22.7354431939926,
0.));
#206928=CARTESIAN_POINT('Ctrl Pts',(-4.31246484362549,22.7354431939926,
12.));
#206929=CARTESIAN_POINT('Ctrl Pts',(-4.30624449484069,22.7212052413386,
0.));
#206930=CARTESIAN_POINT('Ctrl Pts',(-4.30624449484069,22.7212052413386,
12.));
#206931=CARTESIAN_POINT('Ctrl Pts',(-4.3001257075406,22.7070835587564,0.));
#206932=CARTESIAN_POINT('Ctrl Pts',(-4.3001257075406,22.7070835587564,12.));
#206933=CARTESIAN_POINT('Ctrl Pts',(-4.29410846547056,22.6930799122548,
0.));
#206934=CARTESIAN_POINT('Ctrl Pts',(-4.29410846547056,22.6930799122548,
12.));
#206935=CARTESIAN_POINT('Ctrl Pts',(-4.28819274977763,22.6791961033538,
0.));
#206936=CARTESIAN_POINT('Ctrl Pts',(-4.28819274977763,22.6791961033538,
12.));
#206937=CARTESIAN_POINT('Ctrl Pts',(-4.28237853894059,22.6654339703109,
0.));
#206938=CARTESIAN_POINT('Ctrl Pts',(-4.28237853894059,22.6654339703109,
12.));
#206939=CARTESIAN_POINT('Ctrl Pts',(-4.2766658086912,22.6517953893303,0.));
#206940=CARTESIAN_POINT('Ctrl Pts',(-4.2766658086912,22.6517953893303,12.));
#206941=CARTESIAN_POINT('Ctrl Pts',(-4.27105453193004,22.6382822758172,
0.));
#206942=CARTESIAN_POINT('Ctrl Pts',(-4.27105453193004,22.6382822758172,
12.));
#206943=CARTESIAN_POINT('Ctrl Pts',(-4.26554467865576,22.6248965859977,
0.));
#206944=CARTESIAN_POINT('Ctrl Pts',(-4.26554467865576,22.6248965859977,
12.));
#206945=CARTESIAN_POINT('Ctrl Pts',(-4.26013621588305,22.6116403184821,
0.));
#206946=CARTESIAN_POINT('Ctrl Pts',(-4.26013621588305,22.6116403184821,
12.));
#206947=CARTESIAN_POINT('Ctrl Pts',(-4.25482910755481,22.5985155158636,
0.));
#206948=CARTESIAN_POINT('Ctrl Pts',(-4.25482910755481,22.5985155158636,
12.));
#206949=CARTESIAN_POINT('Ctrl Pts',(-4.24962331444177,22.5855242662477,
0.));
#206950=CARTESIAN_POINT('Ctrl Pts',(-4.24962331444177,22.5855242662477,
12.));
#206951=CARTESIAN_POINT('Ctrl Pts',(-4.24451879404851,22.572668704992,0.));
#206952=CARTESIAN_POINT('Ctrl Pts',(-4.24451879404851,22.572668704992,12.));
#206953=CARTESIAN_POINT('Ctrl Pts',(-4.23951550052523,22.5599510166429,
0.));
#206954=CARTESIAN_POINT('Ctrl Pts',(-4.23951550052523,22.5599510166429,
12.));
#206955=CARTESIAN_POINT('Ctrl Pts',(-4.23461338456712,22.5473734368086,
0.));
#206956=CARTESIAN_POINT('Ctrl Pts',(-4.23461338456712,22.5473734368086,
12.));
#206957=CARTESIAN_POINT('Ctrl Pts',(-4.22981239330733,22.5349382540588,
0.));
#206958=CARTESIAN_POINT('Ctrl Pts',(-4.22981239330733,22.5349382540588,
12.));
#206959=CARTESIAN_POINT('Ctrl Pts',(-4.22511247020041,22.5226478117886,
0.));
#206960=CARTESIAN_POINT('Ctrl Pts',(-4.22511247020041,22.5226478117886,
12.));
#206961=CARTESIAN_POINT('Ctrl Pts',(-4.22051355490196,22.5105045108881,
0.));
#206962=CARTESIAN_POINT('Ctrl Pts',(-4.22051355490196,22.5105045108881,
12.));
#206963=CARTESIAN_POINT('Ctrl Pts',(-4.21601558313906,22.4985108124228,
0.));
#206964=CARTESIAN_POINT('Ctrl Pts',(-4.21601558313906,22.4985108124228,
12.));
#206965=CARTESIAN_POINT('Ctrl Pts',(-4.21161848657428,22.4866692403147,
0.));
#206966=CARTESIAN_POINT('Ctrl Pts',(-4.21161848657428,22.4866692403147,
12.));
#206967=CARTESIAN_POINT('Ctrl Pts',(-4.20732219265649,22.4749823839917,
0.));
#206968=CARTESIAN_POINT('Ctrl Pts',(-4.20732219265649,22.4749823839917,
12.));
#206969=CARTESIAN_POINT('Ctrl Pts',(-4.20312662448174,22.4634529011437,
0.));
#206970=CARTESIAN_POINT('Ctrl Pts',(-4.20312662448174,22.4634529011437,
12.));
#206971=CARTESIAN_POINT('Ctrl Pts',(-4.19903170066358,22.4520835205422,
0.));
#206972=CARTESIAN_POINT('Ctrl Pts',(-4.19903170066358,22.4520835205422,
12.));
#206973=CARTESIAN_POINT('Ctrl Pts',(-4.1950373351886,22.4408770448917,0.));
#206974=CARTESIAN_POINT('Ctrl Pts',(-4.1950373351886,22.4408770448917,12.));
#206975=CARTESIAN_POINT('Ctrl Pts',(-4.19114343726932,22.4298363535416,
0.));
#206976=CARTESIAN_POINT('Ctrl Pts',(-4.19114343726932,22.4298363535416,
12.));
#206977=CARTESIAN_POINT('Ctrl Pts',(-4.18734991117707,22.4189644056109,
0.));
#206978=CARTESIAN_POINT('Ctrl Pts',(-4.18734991117707,22.4189644056109,
12.));
#206979=CARTESIAN_POINT('Ctrl Pts',(-4.18365665600839,22.4082642454448,
0.));
#206980=CARTESIAN_POINT('Ctrl Pts',(-4.18365665600839,22.4082642454448,
12.));
#206981=CARTESIAN_POINT('Ctrl Pts',(-4.18006356544879,22.3977390078074,
0.));
#206982=CARTESIAN_POINT('Ctrl Pts',(-4.18006356544879,22.3977390078074,
12.));
#206983=CARTESIAN_POINT('Ctrl Pts',(-4.17657052752834,22.3873919231339,
0.));
#206984=CARTESIAN_POINT('Ctrl Pts',(-4.17657052752834,22.3873919231339,
12.));
#206985=CARTESIAN_POINT('Ctrl Pts',(-4.17317742436162,22.3772263228624,
0.));
#206986=CARTESIAN_POINT('Ctrl Pts',(-4.17317742436162,22.3772263228624,
12.));
#206987=CARTESIAN_POINT('Ctrl Pts',(-4.1698841319947,22.3672456427605,0.));
#206988=CARTESIAN_POINT('Ctrl Pts',(-4.1698841319947,22.3672456427605,12.));
#206989=CARTESIAN_POINT('Ctrl Pts',(-4.16669052026602,22.3574534257397,
0.));
#206990=CARTESIAN_POINT('Ctrl Pts',(-4.16669052026602,22.3574534257397,
12.));
#206991=CARTESIAN_POINT('Ctrl Pts',(-4.1635964526318,22.3478533253886,0.));
#206992=CARTESIAN_POINT('Ctrl Pts',(-4.1635964526318,22.3478533253886,12.));
#206993=CARTESIAN_POINT('Ctrl Pts',(-4.16060178604154,22.3384491078599,
0.));
#206994=CARTESIAN_POINT('Ctrl Pts',(-4.16060178604154,22.3384491078599,
12.));
#206995=CARTESIAN_POINT('Ctrl Pts',(-4.15770637047882,22.3292446628957,
0.));
#206996=CARTESIAN_POINT('Ctrl Pts',(-4.15770637047882,22.3292446628957,
12.));
#206997=CARTESIAN_POINT('Ctrl Pts',(-4.15491004835278,22.3202440186979,
0.));
#206998=CARTESIAN_POINT('Ctrl Pts',(-4.15491004835278,22.3202440186979,
12.));
#206999=CARTESIAN_POINT('Ctrl Pts',(-4.15221265396992,22.3114513545186,
0.));
#207000=CARTESIAN_POINT('Ctrl Pts',(-4.15221265396992,22.3114513545186,
12.));
#207001=CARTESIAN_POINT('Ctrl Pts',(-4.14961401285526,22.3028710166935,
0.));
#207002=CARTESIAN_POINT('Ctrl Pts',(-4.14961401285526,22.3028710166935,
12.));
#207003=CARTESIAN_POINT('Ctrl Pts',(-4.14711394168559,22.2945075198468,
0.));
#207004=CARTESIAN_POINT('Ctrl Pts',(-4.14711394168559,22.2945075198468,
12.));
#207005=CARTESIAN_POINT('Ctrl Pts',(-4.14471224859295,22.2863655389166,
0.));
#207006=CARTESIAN_POINT('Ctrl Pts',(-4.14471224859295,22.2863655389166,
12.));
#207007=CARTESIAN_POINT('Ctrl Pts',(-4.14240873321982,22.2784499072026,
0.));
#207008=CARTESIAN_POINT('Ctrl Pts',(-4.14240873321982,22.2784499072026,
12.));
#207009=CARTESIAN_POINT('Ctrl Pts',(-4.14020318715988,22.2707656042456,
0.));
#207010=CARTESIAN_POINT('Ctrl Pts',(-4.14020318715988,22.2707656042456,
12.));
#207011=CARTESIAN_POINT('Ctrl Pts',(-4.13809539255419,22.263317791397,0.));
#207012=CARTESIAN_POINT('Ctrl Pts',(-4.13809539255419,22.263317791397,12.));
#207013=CARTESIAN_POINT('Ctrl Pts',(-4.13608511977226,22.2561118708422,
0.));
#207014=CARTESIAN_POINT('Ctrl Pts',(-4.13608511977226,22.2561118708422,
12.));
#207015=CARTESIAN_POINT('Ctrl Pts',(-4.13417212558808,22.2491535317789,
0.));
#207016=CARTESIAN_POINT('Ctrl Pts',(-4.13417212558808,22.2491535317789,
12.));
#207017=CARTESIAN_POINT('Ctrl Pts',(-4.1323561506016,22.2424488153523,0.));
#207018=CARTESIAN_POINT('Ctrl Pts',(-4.1323561506016,22.2424488153523,12.));
#207019=CARTESIAN_POINT('Ctrl Pts',(-4.13063692157499,22.2360040565534,
0.));
#207020=CARTESIAN_POINT('Ctrl Pts',(-4.13063692157499,22.2360040565534,
12.));
#207021=CARTESIAN_POINT('Ctrl Pts',(-4.12901415463379,22.2298258043947,
0.));
#207022=CARTESIAN_POINT('Ctrl Pts',(-4.12901415463379,22.2298258043947,
12.));
#207023=CARTESIAN_POINT('Ctrl Pts',(-4.12748755830099,22.2239207458781,
0.));
#207024=CARTESIAN_POINT('Ctrl Pts',(-4.12748755830099,22.2239207458781,
12.));
#207025=CARTESIAN_POINT('Ctrl Pts',(-4.126056836133,22.2182956401341,0.));
#207026=CARTESIAN_POINT('Ctrl Pts',(-4.126056836133,22.2182956401341,12.));
#207027=CARTESIAN_POINT('Ctrl Pts',(-4.12472167516602,22.2129576146671,
0.));
#207028=CARTESIAN_POINT('Ctrl Pts',(-4.12472167516602,22.2129576146671,
12.));
#207029=CARTESIAN_POINT('Ctrl Pts',(-4.12348173702025,22.2079143941719,
0.));
#207030=CARTESIAN_POINT('Ctrl Pts',(-4.12348173702025,22.2079143941719,
12.));
#207031=CARTESIAN_POINT('Ctrl Pts',(-4.12233664408237,22.2031746532106,
0.));
#207032=CARTESIAN_POINT('Ctrl Pts',(-4.12233664408237,22.2031746532106,
12.));
#207033=CARTESIAN_POINT('Ctrl Pts',(-4.12128598183533,22.1987479618246,
0.));
#207034=CARTESIAN_POINT('Ctrl Pts',(-4.12128598183533,22.1987479618246,
12.));
#207035=CARTESIAN_POINT('Ctrl Pts',(-4.12032932637738,22.1946440958098,
0.));
#207036=CARTESIAN_POINT('Ctrl Pts',(-4.12032932637738,22.1946440958098,
12.));
#207037=CARTESIAN_POINT('Ctrl Pts',(-4.11946626228623,22.1908725908525,
0.));
#207038=CARTESIAN_POINT('Ctrl Pts',(-4.11946626228623,22.1908725908525,
12.));
#207039=CARTESIAN_POINT('Ctrl Pts',(-4.11869641271752,22.1874419861496,
0.));
#207040=CARTESIAN_POINT('Ctrl Pts',(-4.11869641271752,22.1874419861496,
12.));
#207041=CARTESIAN_POINT('Ctrl Pts',(-4.11801938107464,22.1843613164855,
0.));
#207042=CARTESIAN_POINT('Ctrl Pts',(-4.11801938107464,22.1843613164855,
12.));
#207043=CARTESIAN_POINT('Ctrl Pts',(-4.11743469691765,22.1816414985788,
0.));
#207044=CARTESIAN_POINT('Ctrl Pts',(-4.11743469691765,22.1816414985788,
12.));
#207045=CARTESIAN_POINT('Ctrl Pts',(-4.11694173195041,22.179297473024,0.));
#207046=CARTESIAN_POINT('Ctrl Pts',(-4.11694173195041,22.179297473024,12.));
#207047=CARTESIAN_POINT('Ctrl Pts',(-4.11653973150558,22.177347426894,0.));
#207048=CARTESIAN_POINT('Ctrl Pts',(-4.11653973150558,22.177347426894,12.));
#207049=CARTESIAN_POINT('Ctrl Pts',(-4.11622797217066,22.1758088296598,
0.));
#207050=CARTESIAN_POINT('Ctrl Pts',(-4.11622797217066,22.1758088296598,
12.));
#207051=CARTESIAN_POINT('Ctrl Pts',(-4.11600589882767,22.1746949858773,
0.));
#207052=CARTESIAN_POINT('Ctrl Pts',(-4.11600589882767,22.1746949858773,
12.));
#207053=CARTESIAN_POINT('Ctrl Pts',(-4.11589976826061,22.174148802123,0.));
#207054=CARTESIAN_POINT('Ctrl Pts',(-4.11589976826061,22.174148802123,12.));
#207055=CARTESIAN_POINT('Ctrl Pts',(-4.1158603587821,22.1739341411684,0.));
#207056=CARTESIAN_POINT('Ctrl Pts',(-4.1158603587821,22.1739341411684,12.));
#207057=CARTESIAN_POINT('Ctrl Pts',(-4.11585194677412,22.1738776823239,
0.));
#207058=CARTESIAN_POINT('Ctrl Pts',(-4.11585194677412,22.1738776823239,
12.));
#207059=CARTESIAN_POINT('Ctrl Pts',(-4.11585220600461,22.1738711152697,
0.));
#207060=CARTESIAN_POINT('Ctrl Pts',(-4.11585220600461,22.1738711152697,
12.));
#207061=CARTESIAN_POINT('',(-6.08833931617698,25.2771067246846,0.));
#207062=CARTESIAN_POINT('Ctrl Pts',(-6.08833931617698,25.2771067246846,
0.));
#207063=CARTESIAN_POINT('Ctrl Pts',(-6.08441489609824,25.2729539149479,
0.));
#207064=CARTESIAN_POINT('Ctrl Pts',(-6.07657531787578,25.2646490489816,
0.));
#207065=CARTESIAN_POINT('Ctrl Pts',(-6.06484373634697,25.2521940105523,
0.));
#207066=CARTESIAN_POINT('Ctrl Pts',(-6.04925720151412,25.2355918138798,
0.));
#207067=CARTESIAN_POINT('Ctrl Pts',(-6.02986667390187,25.2148466201368,
0.));
#207068=CARTESIAN_POINT('Ctrl Pts',(-6.0105688180476,25.1941090269638,0.));
#207069=CARTESIAN_POINT('Ctrl Pts',(-5.99136367859838,25.1733791296154,
0.));
#207070=CARTESIAN_POINT('Ctrl Pts',(-5.97225131495636,25.1526570863065,
0.));
#207071=CARTESIAN_POINT('Ctrl Pts',(-5.95323180187348,25.1319431317273,
0.));
#207072=CARTESIAN_POINT('Ctrl Pts',(-5.93430523086776,25.1112375971182,
0.));
#207073=CARTESIAN_POINT('Ctrl Pts',(-5.91547170844382,25.0905409050863,
0.));
#207074=CARTESIAN_POINT('Ctrl Pts',(-5.89673135155459,25.0698535426593,
0.));
#207075=CARTESIAN_POINT('Ctrl Pts',(-5.87808428385329,25.0491760405965,
0.));
#207076=CARTESIAN_POINT('Ctrl Pts',(-5.8595306315681,25.0285089498922,0.));
#207077=CARTESIAN_POINT('Ctrl Pts',(-5.84107051963073,25.0078528200558,
0.));
#207078=CARTESIAN_POINT('Ctrl Pts',(-5.82270406744214,24.9872081752709,
0.));
#207079=CARTESIAN_POINT('Ctrl Pts',(-5.80443138549747,24.9665754954462,
0.));
#207080=CARTESIAN_POINT('Ctrl Pts',(-5.78625257775703,24.9459552293308,
0.));
#207081=CARTESIAN_POINT('Ctrl Pts',(-5.76816774342236,24.9253478043632,
0.));
#207082=CARTESIAN_POINT('Ctrl Pts',(-5.75017697890813,24.9047536376467,
0.));
#207083=CARTESIAN_POINT('Ctrl Pts',(-5.73228037976927,24.8841731467219,
0.));
#207084=CARTESIAN_POINT('Ctrl Pts',(-5.71447804252019,24.8636067597677,
0.));
#207085=CARTESIAN_POINT('Ctrl Pts',(-5.69677006679429,24.8430549277634,
0.));
#207086=CARTESIAN_POINT('Ctrl Pts',(-5.67915655496524,24.822518122386,0.));
#207087=CARTESIAN_POINT('Ctrl Pts',(-5.66163761114903,24.8019968304618,
0.));
#207088=CARTESIAN_POINT('Ctrl Pts',(-5.64421334042248,24.7814915496728,
0.));
#207089=CARTESIAN_POINT('Ctrl Pts',(-5.62688384790919,24.76100278357,0.));
#207090=CARTESIAN_POINT('Ctrl Pts',(-5.60964923798495,24.7405310372736,
0.));
#207091=CARTESIAN_POINT('Ctrl Pts',(-5.59250961323995,24.7200768119079,
0.));
#207092=CARTESIAN_POINT('Ctrl Pts',(-5.57546507427767,24.6996406035507,
0.));
#207093=CARTESIAN_POINT('Ctrl Pts',(-5.55851572025389,24.6792229061785,
0.));
#207094=CARTESIAN_POINT('Ctrl Pts',(-5.54166164919593,24.6588242134733,
0.));
#207095=CARTESIAN_POINT('Ctrl Pts',(-5.52490295840996,24.6384450211466,
0.));
#207096=CARTESIAN_POINT('Ctrl Pts',(-5.50823974481959,24.618085828918,0.));
#207097=CARTESIAN_POINT('Ctrl Pts',(-5.49167210537235,24.5977471429365,
0.));
#207098=CARTESIAN_POINT('Ctrl Pts',(-5.47520013724403,24.5774294770329,
0.));
#207099=CARTESIAN_POINT('Ctrl Pts',(-5.45882393762244,24.5571333514841,
0.));
#207100=CARTESIAN_POINT('Ctrl Pts',(-5.44254360356865,24.5368592922861,
0.));
#207101=CARTESIAN_POINT('Ctrl Pts',(-5.42635923183411,24.5166078302107,
0.));
#207102=CARTESIAN_POINT('Ctrl Pts',(-5.41027091869242,24.4963794999831,
0.));
#207103=CARTESIAN_POINT('Ctrl Pts',(-5.3942787597383,24.4761748393322,0.));
#207104=CARTESIAN_POINT('Ctrl Pts',(-5.37838284973706,24.4559943883159,
0.));
#207105=CARTESIAN_POINT('Ctrl Pts',(-5.36258328273639,24.4358386899152,
0.));
#207106=CARTESIAN_POINT('Ctrl Pts',(-5.34688015213546,24.4157082904615,
0.));
#207107=CARTESIAN_POINT('Ctrl Pts',(-5.33127355076037,24.3956037401293,
0.));
#207108=CARTESIAN_POINT('Ctrl Pts',(-5.31576357092524,24.3755255933917,
0.));
#207109=CARTESIAN_POINT('Ctrl Pts',(-5.30035030449059,24.3554744095075,
0.));
#207110=CARTESIAN_POINT('Ctrl Pts',(-5.28503384290644,24.3354507529415,
0.));
#207111=CARTESIAN_POINT('Ctrl Pts',(-5.26981427718796,24.3154551932222,
0.));
#207112=CARTESIAN_POINT('Ctrl Pts',(-5.25469169788856,24.2954883048448,
0.));
#207113=CARTESIAN_POINT('Ctrl Pts',(-5.23966619506289,24.2755506671526,
0.));
#207114=CARTESIAN_POINT('Ctrl Pts',(-5.22473785822441,24.2556428642294,
0.));
#207115=CARTESIAN_POINT('Ctrl Pts',(-5.20990677629173,24.2357654847765,
0.));
#207116=CARTESIAN_POINT('Ctrl Pts',(-5.19517303753643,24.215919122017,0.));
#207117=CARTESIAN_POINT('Ctrl Pts',(-5.18053672961392,24.1961043738754,
0.));
#207118=CARTESIAN_POINT('Ctrl Pts',(-5.16599793957979,24.1763218431343,
0.));
#207119=CARTESIAN_POINT('Ctrl Pts',(-5.15155675390075,24.156572137597,0.));
#207120=CARTESIAN_POINT('Ctrl Pts',(-5.13721325845745,24.1368558702443,
0.));
#207121=CARTESIAN_POINT('Ctrl Pts',(-5.12296753853859,24.117173659394,0.));
#207122=CARTESIAN_POINT('Ctrl Pts',(-5.10881967883132,24.0975261288446,
0.));
#207123=CARTESIAN_POINT('Ctrl Pts',(-5.09476976342625,24.0779139079266,
0.));
#207124=CARTESIAN_POINT('Ctrl Pts',(-5.08081787581276,24.0583376315638,
0.));
#207125=CARTESIAN_POINT('Ctrl Pts',(-5.06696409886641,24.0387979403268,
0.));
#207126=CARTESIAN_POINT('Ctrl Pts',(-5.05320851483065,24.0192954804896,
0.));
#207127=CARTESIAN_POINT('Ctrl Pts',(-5.03955120528521,23.9998309040746,
0.));
#207128=CARTESIAN_POINT('Ctrl Pts',(-5.02599225112454,23.9804048689227,
0.));
#207129=CARTESIAN_POINT('Ctrl Pts',(-5.01253173257453,23.9610180388271,
0.));
#207130=CARTESIAN_POINT('Ctrl Pts',(-4.99916972919307,23.9416710836529,
0.));
#207131=CARTESIAN_POINT('Ctrl Pts',(-4.98590631986533,23.9223646794592,
0.));
#207132=CARTESIAN_POINT('Ctrl Pts',(-4.97274158279227,23.9030995086163,
0.));
#207133=CARTESIAN_POINT('Ctrl Pts',(-4.95967559546561,23.8838762599218,
0.));
#207134=CARTESIAN_POINT('Ctrl Pts',(-4.9467084346586,23.8646956287168,0.));
#207135=CARTESIAN_POINT('Ctrl Pts',(-4.93384017643432,23.8455583170057,
0.));
#207136=CARTESIAN_POINT('Ctrl Pts',(-4.92107089613969,23.8264650335717,
0.));
#207137=CARTESIAN_POINT('Ctrl Pts',(-4.90840066839344,23.8074164940896,
0.));
#207138=CARTESIAN_POINT('Ctrl Pts',(-4.89582956706775,23.7884134212384,
0.));
#207139=CARTESIAN_POINT('Ctrl Pts',(-4.88335766525573,23.7694565448049,
0.));
#207140=CARTESIAN_POINT('Ctrl Pts',(-4.87098503527152,23.7505466018245,
0.));
#207141=CARTESIAN_POINT('Ctrl Pts',(-4.85871174865499,23.7316843367313,
0.));
#207142=CARTESIAN_POINT('Ctrl Pts',(-4.84653787616425,23.7128705015017,
0.));
#207143=CARTESIAN_POINT('Ctrl Pts',(-4.83446348776266,23.6941058557971,
0.));
#207144=CARTESIAN_POINT('Ctrl Pts',(-4.82248865259562,23.675391167102,0.));
#207145=CARTESIAN_POINT('Ctrl Pts',(-4.81061343896432,23.6567272108628,
0.));
#207146=CARTESIAN_POINT('Ctrl Pts',(-4.7988379143322,23.6381147706579,0.));
#207147=CARTESIAN_POINT('Ctrl Pts',(-4.78716214532098,23.6195546383624,
0.));
#207148=CARTESIAN_POINT('Ctrl Pts',(-4.77558619769872,23.6010476143099,
0.));
#207149=CARTESIAN_POINT('Ctrl Pts',(-4.76411013636251,23.5825945074535,
0.));
#207150=CARTESIAN_POINT('Ctrl Pts',(-4.75273402530617,23.5641961355168,
0.));
#207151=CARTESIAN_POINT('Ctrl Pts',(-4.74145792760698,23.545853325171,0.));
#207152=CARTESIAN_POINT('Ctrl Pts',(-4.7302819054303,23.5275669122372,0.));
#207153=CARTESIAN_POINT('Ctrl Pts',(-4.71920602001902,23.509337741878,0.));
#207154=CARTESIAN_POINT('Ctrl Pts',(-4.70823033167819,23.491166668789,0.));
#207155=CARTESIAN_POINT('Ctrl Pts',(-4.69735489975024,23.4730545573853,
0.));
#207156=CARTESIAN_POINT('Ctrl Pts',(-4.68657978258303,23.455002281986,0.));
#207157=CARTESIAN_POINT('Ctrl Pts',(-4.67590503753058,23.4370107270451,
0.));
#207158=CARTESIAN_POINT('Ctrl Pts',(-4.6653307209467,23.4190807873803,0.));
#207159=CARTESIAN_POINT('Ctrl Pts',(-4.65485688816924,23.4012133683959,
0.));
#207160=CARTESIAN_POINT('Ctrl Pts',(-4.6444835934993,23.3834093863068,0.));
#207161=CARTESIAN_POINT('Ctrl Pts',(-4.63421089016541,23.3656697683489,
0.));
#207162=CARTESIAN_POINT('Ctrl Pts',(-4.62403883030805,23.3479954530272,
0.));
#207163=CARTESIAN_POINT('Ctrl Pts',(-4.6139674649783,23.3303873903938,0.));
#207164=CARTESIAN_POINT('Ctrl Pts',(-4.60399684412163,23.3128465423115,
0.));
#207165=CARTESIAN_POINT('Ctrl Pts',(-4.5941270165575,23.2953738827191,0.));
#207166=CARTESIAN_POINT('Ctrl Pts',(-4.5843580299469,23.2779703978876,0.));
#207167=CARTESIAN_POINT('Ctrl Pts',(-4.57468993076097,23.2606370866866,
0.));
#207168=CARTESIAN_POINT('Ctrl Pts',(-4.56512276427839,23.2433749609131,
0.));
#207169=CARTESIAN_POINT('Ctrl Pts',(-4.55565657456975,23.2261850456064,
0.));
#207170=CARTESIAN_POINT('Ctrl Pts',(-4.54629140447544,23.2090683793629,
0.));
#207171=CARTESIAN_POINT('Ctrl Pts',(-4.53702729557566,23.1920260146465,
0.));
#207172=CARTESIAN_POINT('Ctrl Pts',(-4.52786428815015,23.1750590180908,
0.));
#207173=CARTESIAN_POINT('Ctrl Pts',(-4.51880242116748,23.1581684708761,
0.));
#207174=CARTESIAN_POINT('Ctrl Pts',(-4.5098417322706,23.1413554691123,0.));
#207175=CARTESIAN_POINT('Ctrl Pts',(-4.50098225775171,23.1246211242115,
0.));
#207176=CARTESIAN_POINT('Ctrl Pts',(-4.49222403252216,23.1079665632636,
0.));
#207177=CARTESIAN_POINT('Ctrl Pts',(-4.48356709006788,23.0913929293922,
0.));
#207178=CARTESIAN_POINT('Ctrl Pts',(-4.47501146242856,23.0749013821881,
0.));
#207179=CARTESIAN_POINT('Ctrl Pts',(-4.4665571801823,23.0584930981732,0.));
#207180=CARTESIAN_POINT('Ctrl Pts',(-4.45820427241683,23.0421692712467,
0.));
#207181=CARTESIAN_POINT('Ctrl Pts',(-4.44995276669686,23.0259311131392,
0.));
#207182=CARTESIAN_POINT('Ctrl Pts',(-4.44180268901643,23.0097798538395,
0.));
#207183=CARTESIAN_POINT('Ctrl Pts',(-4.43375406376879,22.9937167421006,
0.));
#207184=CARTESIAN_POINT('Ctrl Pts',(-4.42580691372751,22.977743046002,0.));
#207185=CARTESIAN_POINT('Ctrl Pts',(-4.41796126001302,22.9618600534866,
0.));
#207186=CARTESIAN_POINT('Ctrl Pts',(-4.41021712205553,22.9460690729093,
0.));
#207187=CARTESIAN_POINT('Ctrl Pts',(-4.40257451754323,22.930371433555,0.));
#207188=CARTESIAN_POINT('Ctrl Pts',(-4.39503346238473,22.9147684862426,
0.));
#207189=CARTESIAN_POINT('Ctrl Pts',(-4.38759397068406,22.8992616040108,
0.));
#207190=CARTESIAN_POINT('Ctrl Pts',(-4.38025605470093,22.8838521827701,
0.));
#207191=CARTESIAN_POINT('Ctrl Pts',(-4.37301972480746,22.8685416419725,
0.));
#207192=CARTESIAN_POINT('Ctrl Pts',(-4.36588498942997,22.8533314252422,
0.));
#207193=CARTESIAN_POINT('Ctrl Pts',(-4.35885185500546,22.8382230011184,
0.));
#207194=CARTESIAN_POINT('Ctrl Pts',(-4.35192032594791,22.8232178638876,
0.));
#207195=CARTESIAN_POINT('Ctrl Pts',(-4.34509040460062,22.8083175343791,
0.));
#207196=CARTESIAN_POINT('Ctrl Pts',(-4.33836209118446,22.7935235607806,
0.));
#207197=CARTESIAN_POINT('Ctrl Pts',(-4.3317353837319,22.7788375194076,0.));
#207198=CARTESIAN_POINT('Ctrl Pts',(-4.32521027803754,22.7642610156475,
0.));
#207199=CARTESIAN_POINT('Ctrl Pts',(-4.31878676761235,22.7497956849848,
0.));
#207200=CARTESIAN_POINT('Ctrl Pts',(-4.31246484362549,22.7354431939926,
0.));
#207201=CARTESIAN_POINT('Ctrl Pts',(-4.30624449484069,22.7212052413386,
0.));
#207202=CARTESIAN_POINT('Ctrl Pts',(-4.3001257075406,22.7070835587564,0.));
#207203=CARTESIAN_POINT('Ctrl Pts',(-4.29410846547056,22.6930799122548,
0.));
#207204=CARTESIAN_POINT('Ctrl Pts',(-4.28819274977763,22.6791961033538,
0.));
#207205=CARTESIAN_POINT('Ctrl Pts',(-4.28237853894059,22.6654339703109,
0.));
#207206=CARTESIAN_POINT('Ctrl Pts',(-4.2766658086912,22.6517953893303,0.));
#207207=CARTESIAN_POINT('Ctrl Pts',(-4.27105453193004,22.6382822758172,
0.));
#207208=CARTESIAN_POINT('Ctrl Pts',(-4.26554467865576,22.6248965859977,
0.));
#207209=CARTESIAN_POINT('Ctrl Pts',(-4.26013621588305,22.6116403184821,
0.));
#207210=CARTESIAN_POINT('Ctrl Pts',(-4.25482910755481,22.5985155158636,
0.));
#207211=CARTESIAN_POINT('Ctrl Pts',(-4.24962331444177,22.5855242662477,
0.));
#207212=CARTESIAN_POINT('Ctrl Pts',(-4.24451879404851,22.572668704992,0.));
#207213=CARTESIAN_POINT('Ctrl Pts',(-4.23951550052523,22.5599510166429,
0.));
#207214=CARTESIAN_POINT('Ctrl Pts',(-4.23461338456712,22.5473734368086,
0.));
#207215=CARTESIAN_POINT('Ctrl Pts',(-4.22981239330733,22.5349382540588,
0.));
#207216=CARTESIAN_POINT('Ctrl Pts',(-4.22511247020041,22.5226478117886,
0.));
#207217=CARTESIAN_POINT('Ctrl Pts',(-4.22051355490196,22.5105045108881,
0.));
#207218=CARTESIAN_POINT('Ctrl Pts',(-4.21601558313906,22.4985108124228,
0.));
#207219=CARTESIAN_POINT('Ctrl Pts',(-4.21161848657428,22.4866692403147,
0.));
#207220=CARTESIAN_POINT('Ctrl Pts',(-4.20732219265649,22.4749823839917,
0.));
#207221=CARTESIAN_POINT('Ctrl Pts',(-4.20312662448174,22.4634529011437,
0.));
#207222=CARTESIAN_POINT('Ctrl Pts',(-4.19903170066358,22.4520835205422,
0.));
#207223=CARTESIAN_POINT('Ctrl Pts',(-4.1950373351886,22.4408770448917,0.));
#207224=CARTESIAN_POINT('Ctrl Pts',(-4.19114343726932,22.4298363535416,
0.));
#207225=CARTESIAN_POINT('Ctrl Pts',(-4.18734991117707,22.4189644056109,
0.));
#207226=CARTESIAN_POINT('Ctrl Pts',(-4.18365665600839,22.4082642454448,
0.));
#207227=CARTESIAN_POINT('Ctrl Pts',(-4.18006356544879,22.3977390078074,
0.));
#207228=CARTESIAN_POINT('Ctrl Pts',(-4.17657052752834,22.3873919231339,
0.));
#207229=CARTESIAN_POINT('Ctrl Pts',(-4.17317742436162,22.3772263228624,
0.));
#207230=CARTESIAN_POINT('Ctrl Pts',(-4.1698841319947,22.3672456427605,0.));
#207231=CARTESIAN_POINT('Ctrl Pts',(-4.16669052026602,22.3574534257397,
0.));
#207232=CARTESIAN_POINT('Ctrl Pts',(-4.1635964526318,22.3478533253886,0.));
#207233=CARTESIAN_POINT('Ctrl Pts',(-4.16060178604154,22.3384491078599,
0.));
#207234=CARTESIAN_POINT('Ctrl Pts',(-4.15770637047882,22.3292446628957,
0.));
#207235=CARTESIAN_POINT('Ctrl Pts',(-4.15491004835278,22.3202440186979,
0.));
#207236=CARTESIAN_POINT('Ctrl Pts',(-4.15221265396992,22.3114513545186,
0.));
#207237=CARTESIAN_POINT('Ctrl Pts',(-4.14961401285526,22.3028710166935,
0.));
#207238=CARTESIAN_POINT('Ctrl Pts',(-4.14711394168559,22.2945075198468,
0.));
#207239=CARTESIAN_POINT('Ctrl Pts',(-4.14471224859295,22.2863655389166,
0.));
#207240=CARTESIAN_POINT('Ctrl Pts',(-4.14240873321982,22.2784499072026,
0.));
#207241=CARTESIAN_POINT('Ctrl Pts',(-4.14020318715988,22.2707656042456,
0.));
#207242=CARTESIAN_POINT('Ctrl Pts',(-4.13809539255419,22.263317791397,0.));
#207243=CARTESIAN_POINT('Ctrl Pts',(-4.13608511977226,22.2561118708422,
0.));
#207244=CARTESIAN_POINT('Ctrl Pts',(-4.13417212558808,22.2491535317789,
0.));
#207245=CARTESIAN_POINT('Ctrl Pts',(-4.1323561506016,22.2424488153523,0.));
#207246=CARTESIAN_POINT('Ctrl Pts',(-4.13063692157499,22.2360040565534,
0.));
#207247=CARTESIAN_POINT('Ctrl Pts',(-4.12901415463379,22.2298258043947,
0.));
#207248=CARTESIAN_POINT('Ctrl Pts',(-4.12748755830099,22.2239207458781,
0.));
#207249=CARTESIAN_POINT('Ctrl Pts',(-4.126056836133,22.2182956401341,0.));
#207250=CARTESIAN_POINT('Ctrl Pts',(-4.12472167516602,22.2129576146671,
0.));
#207251=CARTESIAN_POINT('Ctrl Pts',(-4.12348173702025,22.2079143941719,
0.));
#207252=CARTESIAN_POINT('Ctrl Pts',(-4.12233664408237,22.2031746532106,
0.));
#207253=CARTESIAN_POINT('Ctrl Pts',(-4.12128598183533,22.1987479618246,
0.));
#207254=CARTESIAN_POINT('Ctrl Pts',(-4.12032932637738,22.1946440958098,
0.));
#207255=CARTESIAN_POINT('Ctrl Pts',(-4.11946626228623,22.1908725908525,
0.));
#207256=CARTESIAN_POINT('Ctrl Pts',(-4.11869641271752,22.1874419861496,
0.));
#207257=CARTESIAN_POINT('Ctrl Pts',(-4.11801938107464,22.1843613164855,
0.));
#207258=CARTESIAN_POINT('Ctrl Pts',(-4.11743469691765,22.1816414985788,
0.));
#207259=CARTESIAN_POINT('Ctrl Pts',(-4.11694173195041,22.179297473024,0.));
#207260=CARTESIAN_POINT('Ctrl Pts',(-4.11653973150558,22.177347426894,0.));
#207261=CARTESIAN_POINT('Ctrl Pts',(-4.11622797217066,22.1758088296598,
0.));
#207262=CARTESIAN_POINT('Ctrl Pts',(-4.11600589882767,22.1746949858773,
0.));
#207263=CARTESIAN_POINT('Ctrl Pts',(-4.11589976826061,22.174148802123,0.));
#207264=CARTESIAN_POINT('Ctrl Pts',(-4.1158603587821,22.1739341411684,0.));
#207265=CARTESIAN_POINT('Ctrl Pts',(-4.11585194677412,22.1738776823239,
0.));
#207266=CARTESIAN_POINT('Ctrl Pts',(-4.11585220600461,22.1738711152697,
0.));
#207267=CARTESIAN_POINT('',(-6.08833931617698,25.2771067246846,0.));
#207268=CARTESIAN_POINT('Ctrl Pts',(-1.76341220531179,22.4835757167854,
0.));
#207269=CARTESIAN_POINT('Ctrl Pts',(-1.76341220531179,22.4835757167854,
12.));
#207270=CARTESIAN_POINT('Ctrl Pts',(-1.76341415538764,22.483581992979,0.));
#207271=CARTESIAN_POINT('Ctrl Pts',(-1.76341415538764,22.483581992979,12.));
#207272=CARTESIAN_POINT('Ctrl Pts',(-1.7634206426357,22.4836387052232,0.));
#207273=CARTESIAN_POINT('Ctrl Pts',(-1.7634206426357,22.4836387052232,12.));
#207274=CARTESIAN_POINT('Ctrl Pts',(-1.76343813434565,22.483856251707,0.));
#207275=CARTESIAN_POINT('Ctrl Pts',(-1.76343813434565,22.483856251707,12.));
#207276=CARTESIAN_POINT('Ctrl Pts',(-1.76347698284792,22.4844112933129,
0.));
#207277=CARTESIAN_POINT('Ctrl Pts',(-1.76347698284792,22.4844112933129,
12.));
#207278=CARTESIAN_POINT('Ctrl Pts',(-1.76355076045546,22.4855446605991,
0.));
#207279=CARTESIAN_POINT('Ctrl Pts',(-1.76355076045546,22.4855446605991,
12.));
#207280=CARTESIAN_POINT('Ctrl Pts',(-1.76364784232963,22.4871115206571,
0.));
#207281=CARTESIAN_POINT('Ctrl Pts',(-1.76364784232963,22.4871115206571,
12.));
#207282=CARTESIAN_POINT('Ctrl Pts',(-1.76376424879505,22.4890991659478,
0.));
#207283=CARTESIAN_POINT('Ctrl Pts',(-1.76376424879505,22.4890991659478,
12.));
#207284=CARTESIAN_POINT('Ctrl Pts',(-1.76389475965724,22.4914909094908,
0.));
#207285=CARTESIAN_POINT('Ctrl Pts',(-1.76389475965724,22.4914909094908,
12.));
#207286=CARTESIAN_POINT('Ctrl Pts',(-1.76403393880301,22.4942693792449,
0.));
#207287=CARTESIAN_POINT('Ctrl Pts',(-1.76403393880301,22.4942693792449,
12.));
#207288=CARTESIAN_POINT('Ctrl Pts',(-1.76417731243462,22.4974203063191,
0.));
#207289=CARTESIAN_POINT('Ctrl Pts',(-1.76417731243462,22.4974203063191,
12.));
#207290=CARTESIAN_POINT('Ctrl Pts',(-1.76432160068725,22.5009332677316,
0.));
#207291=CARTESIAN_POINT('Ctrl Pts',(-1.76432160068725,22.5009332677316,
12.));
#207292=CARTESIAN_POINT('Ctrl Pts',(-1.76446408210366,22.5047996391978,
0.));
#207293=CARTESIAN_POINT('Ctrl Pts',(-1.76446408210366,22.5047996391978,
12.));
#207294=CARTESIAN_POINT('Ctrl Pts',(-1.76460218257323,22.5090112700212,
0.));
#207295=CARTESIAN_POINT('Ctrl Pts',(-1.76460218257323,22.5090112700212,
12.));
#207296=CARTESIAN_POINT('Ctrl Pts',(-1.76473303281159,22.5135590569554,
0.));
#207297=CARTESIAN_POINT('Ctrl Pts',(-1.76473303281159,22.5135590569554,
12.));
#207298=CARTESIAN_POINT('Ctrl Pts',(-1.76485369319896,22.5184336670207,
0.));
#207299=CARTESIAN_POINT('Ctrl Pts',(-1.76485369319896,22.5184336670207,
12.));
#207300=CARTESIAN_POINT('Ctrl Pts',(-1.76496128643369,22.5236259635515,
0.));
#207301=CARTESIAN_POINT('Ctrl Pts',(-1.76496128643369,22.5236259635515,
12.));
#207302=CARTESIAN_POINT('Ctrl Pts',(-1.76505320262752,22.529127665298,0.));
#207303=CARTESIAN_POINT('Ctrl Pts',(-1.76505320262752,22.529127665298,12.));
#207304=CARTESIAN_POINT('Ctrl Pts',(-1.7651271156325,22.5349313983571,0.));
#207305=CARTESIAN_POINT('Ctrl Pts',(-1.7651271156325,22.5349313983571,12.));
#207306=CARTESIAN_POINT('Ctrl Pts',(-1.76518087841493,22.5410303590891,
0.));
#207307=CARTESIAN_POINT('Ctrl Pts',(-1.76518087841493,22.5410303590891,
12.));
#207308=CARTESIAN_POINT('Ctrl Pts',(-1.76521245524047,22.5474180954006,
0.));
#207309=CARTESIAN_POINT('Ctrl Pts',(-1.76521245524047,22.5474180954006,
12.));
#207310=CARTESIAN_POINT('Ctrl Pts',(-1.76521983384063,22.5540882235837,
0.));
#207311=CARTESIAN_POINT('Ctrl Pts',(-1.76521983384063,22.5540882235837,
12.));
#207312=CARTESIAN_POINT('Ctrl Pts',(-1.76520104500449,22.5610344912501,
0.));
#207313=CARTESIAN_POINT('Ctrl Pts',(-1.76520104500449,22.5610344912501,
12.));
#207314=CARTESIAN_POINT('Ctrl Pts',(-1.76515418518829,22.5682508499873,
0.));
#207315=CARTESIAN_POINT('Ctrl Pts',(-1.76515418518829,22.5682508499873,
12.));
#207316=CARTESIAN_POINT('Ctrl Pts',(-1.76507744026747,22.5757315316355,
0.));
#207317=CARTESIAN_POINT('Ctrl Pts',(-1.76507744026747,22.5757315316355,
12.));
#207318=CARTESIAN_POINT('Ctrl Pts',(-1.76496910283088,22.5834711038024,
0.));
#207319=CARTESIAN_POINT('Ctrl Pts',(-1.76496910283088,22.5834711038024,
12.));
#207320=CARTESIAN_POINT('Ctrl Pts',(-1.76482755288411,22.5914644078106,
0.));
#207321=CARTESIAN_POINT('Ctrl Pts',(-1.76482755288411,22.5914644078106,
12.));
#207322=CARTESIAN_POINT('Ctrl Pts',(-1.76465124413556,22.5997065145638,
0.));
#207323=CARTESIAN_POINT('Ctrl Pts',(-1.76465124413556,22.5997065145638,
12.));
#207324=CARTESIAN_POINT('Ctrl Pts',(-1.76443868648015,22.6081926681342,
0.));
#207325=CARTESIAN_POINT('Ctrl Pts',(-1.76443868648015,22.6081926681342,
12.));
#207326=CARTESIAN_POINT('Ctrl Pts',(-1.76418843543739,22.6169182517693,
0.));
#207327=CARTESIAN_POINT('Ctrl Pts',(-1.76418843543739,22.6169182517693,
12.));
#207328=CARTESIAN_POINT('Ctrl Pts',(-1.76389909571402,22.6258787994847,
0.));
#207329=CARTESIAN_POINT('Ctrl Pts',(-1.76389909571402,22.6258787994847,
12.));
#207330=CARTESIAN_POINT('Ctrl Pts',(-1.76356932176272,22.635069997936,0.));
#207331=CARTESIAN_POINT('Ctrl Pts',(-1.76356932176272,22.635069997936,12.));
#207332=CARTESIAN_POINT('Ctrl Pts',(-1.76319782013914,22.6444876940425,
0.));
#207333=CARTESIAN_POINT('Ctrl Pts',(-1.76319782013914,22.6444876940425,
12.));
#207334=CARTESIAN_POINT('Ctrl Pts',(-1.76278334912559,22.6541278938413,
0.));
#207335=CARTESIAN_POINT('Ctrl Pts',(-1.76278334912559,22.6541278938413,
12.));
#207336=CARTESIAN_POINT('Ctrl Pts',(-1.76232471392567,22.6639867471756,
0.));
#207337=CARTESIAN_POINT('Ctrl Pts',(-1.76232471392567,22.6639867471756,
12.));
#207338=CARTESIAN_POINT('Ctrl Pts',(-1.76182076289525,22.6740605356699,
0.));
#207339=CARTESIAN_POINT('Ctrl Pts',(-1.76182076289525,22.6740605356699,
12.));
#207340=CARTESIAN_POINT('Ctrl Pts',(-1.76127038310613,22.6843456585245,
0.));
#207341=CARTESIAN_POINT('Ctrl Pts',(-1.76127038310613,22.6843456585245,
12.));
#207342=CARTESIAN_POINT('Ctrl Pts',(-1.76067249704884,22.6948386219843,
0.));
#207343=CARTESIAN_POINT('Ctrl Pts',(-1.76067249704884,22.6948386219843,
12.));
#207344=CARTESIAN_POINT('Ctrl Pts',(-1.76002606202399,22.7055360375481,
0.));
#207345=CARTESIAN_POINT('Ctrl Pts',(-1.76002606202399,22.7055360375481,
12.));
#207346=CARTESIAN_POINT('Ctrl Pts',(-1.75933006905924,22.7164346186007,
0.));
#207347=CARTESIAN_POINT('Ctrl Pts',(-1.75933006905924,22.7164346186007,
12.));
#207348=CARTESIAN_POINT('Ctrl Pts',(-1.75858354204635,22.7275311777305,
0.));
#207349=CARTESIAN_POINT('Ctrl Pts',(-1.75858354204635,22.7275311777305,
12.));
#207350=CARTESIAN_POINT('Ctrl Pts',(-1.75778553673249,22.7388226235565,
0.));
#207351=CARTESIAN_POINT('Ctrl Pts',(-1.75778553673249,22.7388226235565,
12.));
#207352=CARTESIAN_POINT('Ctrl Pts',(-1.75693513908911,22.7503059556455,
0.));
#207353=CARTESIAN_POINT('Ctrl Pts',(-1.75693513908911,22.7503059556455,
12.));
#207354=CARTESIAN_POINT('Ctrl Pts',(-1.7560314637164,22.7619782595013,0.));
#207355=CARTESIAN_POINT('Ctrl Pts',(-1.7560314637164,22.7619782595013,12.));
#207356=CARTESIAN_POINT('Ctrl Pts',(-1.75507365227127,22.7738367016115,
0.));
#207357=CARTESIAN_POINT('Ctrl Pts',(-1.75507365227127,22.7738367016115,
12.));
#207358=CARTESIAN_POINT('Ctrl Pts',(-1.7540608718293,22.7858785242358,0.));
#207359=CARTESIAN_POINT('Ctrl Pts',(-1.7540608718293,22.7858785242358,12.));
#207360=CARTESIAN_POINT('Ctrl Pts',(-1.75299231391461,22.7981010424312,
0.));
#207361=CARTESIAN_POINT('Ctrl Pts',(-1.75299231391461,22.7981010424312,
12.));
#207362=CARTESIAN_POINT('Ctrl Pts',(-1.7518671936559,22.8105016414712,0.));
#207363=CARTESIAN_POINT('Ctrl Pts',(-1.7518671936559,22.8105016414712,12.));
#207364=CARTESIAN_POINT('Ctrl Pts',(-1.75068474890884,22.8230777741285,
0.));
#207365=CARTESIAN_POINT('Ctrl Pts',(-1.75068474890884,22.8230777741285,
12.));
#207366=CARTESIAN_POINT('Ctrl Pts',(-1.74944423940117,22.8358269579854,
0.));
#207367=CARTESIAN_POINT('Ctrl Pts',(-1.74944423940117,22.8358269579854,
12.));
#207368=CARTESIAN_POINT('Ctrl Pts',(-1.74814494588492,22.8487467728075,
0.));
#207369=CARTESIAN_POINT('Ctrl Pts',(-1.74814494588492,22.8487467728075,
12.));
#207370=CARTESIAN_POINT('Ctrl Pts',(-1.74678616930663,22.8618348580234,
0.));
#207371=CARTESIAN_POINT('Ctrl Pts',(-1.74678616930663,22.8618348580234,
12.));
#207372=CARTESIAN_POINT('Ctrl Pts',(-1.745367229982,22.8750889101696,0.));
#207373=CARTESIAN_POINT('Ctrl Pts',(-1.745367229982,22.8750889101696,12.));
#207374=CARTESIAN_POINT('Ctrl Pts',(-1.74388746677702,22.8885066803351,
0.));
#207375=CARTESIAN_POINT('Ctrl Pts',(-1.74388746677702,22.8885066803351,
12.));
#207376=CARTESIAN_POINT('Ctrl Pts',(-1.74234623630079,22.9020859716144,
0.));
#207377=CARTESIAN_POINT('Ctrl Pts',(-1.74234623630079,22.9020859716144,
12.));
#207378=CARTESIAN_POINT('Ctrl Pts',(-1.74074291231057,22.9158246373365,
0.));
#207379=CARTESIAN_POINT('Ctrl Pts',(-1.74074291231057,22.9158246373365,
12.));
#207380=CARTESIAN_POINT('Ctrl Pts',(-1.73907688511664,22.9297205792587,
0.));
#207381=CARTESIAN_POINT('Ctrl Pts',(-1.73907688511664,22.9297205792587,
12.));
#207382=CARTESIAN_POINT('Ctrl Pts',(-1.73734756100038,22.9437717457825,
0.));
#207383=CARTESIAN_POINT('Ctrl Pts',(-1.73734756100038,22.9437717457825,
12.));
#207384=CARTESIAN_POINT('Ctrl Pts',(-1.73555436162771,22.9579761301062,
0.));
#207385=CARTESIAN_POINT('Ctrl Pts',(-1.73555436162771,22.9579761301062,
12.));
#207386=CARTESIAN_POINT('Ctrl Pts',(-1.73369672350818,22.9723317685688,
0.));
#207387=CARTESIAN_POINT('Ctrl Pts',(-1.73369672350818,22.9723317685688,
12.));
#207388=CARTESIAN_POINT('Ctrl Pts',(-1.73177409750194,22.9868367391978,
0.));
#207389=CARTESIAN_POINT('Ctrl Pts',(-1.73177409750194,22.9868367391978,
12.));
#207390=CARTESIAN_POINT('Ctrl Pts',(-1.72978594832137,23.0014891601891,
0.));
#207391=CARTESIAN_POINT('Ctrl Pts',(-1.72978594832137,23.0014891601891,
12.));
#207392=CARTESIAN_POINT('Ctrl Pts',(-1.72773175404703,23.0162871884167,
0.));
#207393=CARTESIAN_POINT('Ctrl Pts',(-1.72773175404703,23.0162871884167,
12.));
#207394=CARTESIAN_POINT('Ctrl Pts',(-1.72561100564033,23.031229017888,0.));
#207395=CARTESIAN_POINT('Ctrl Pts',(-1.72561100564033,23.031229017888,12.));
#207396=CARTESIAN_POINT('Ctrl Pts',(-1.72342320653731,23.0463128785528,
0.));
#207397=CARTESIAN_POINT('Ctrl Pts',(-1.72342320653731,23.0463128785528,
12.));
#207398=CARTESIAN_POINT('Ctrl Pts',(-1.7211678722598,23.061537035156,0.));
#207399=CARTESIAN_POINT('Ctrl Pts',(-1.7211678722598,23.061537035156,12.));
#207400=CARTESIAN_POINT('Ctrl Pts',(-1.71884453003027,23.0768997860709,
0.));
#207401=CARTESIAN_POINT('Ctrl Pts',(-1.71884453003027,23.0768997860709,
12.));
#207402=CARTESIAN_POINT('Ctrl Pts',(-1.71645271839311,23.0923994621216,
0.));
#207403=CARTESIAN_POINT('Ctrl Pts',(-1.71645271839311,23.0923994621216,
12.));
#207404=CARTESIAN_POINT('Ctrl Pts',(-1.71399198684725,23.1080344254291,
0.));
#207405=CARTESIAN_POINT('Ctrl Pts',(-1.71399198684725,23.1080344254291,
12.));
#207406=CARTESIAN_POINT('Ctrl Pts',(-1.71146189552192,23.1238030684929,
0.));
#207407=CARTESIAN_POINT('Ctrl Pts',(-1.71146189552192,23.1238030684929,
12.));
#207408=CARTESIAN_POINT('Ctrl Pts',(-1.7088620148546,23.1397038132358,0.));
#207409=CARTESIAN_POINT('Ctrl Pts',(-1.7088620148546,23.1397038132358,12.));
#207410=CARTESIAN_POINT('Ctrl Pts',(-1.70619192527847,23.1557351100613,
0.));
#207411=CARTESIAN_POINT('Ctrl Pts',(-1.70619192527847,23.1557351100613,
12.));
#207412=CARTESIAN_POINT('Ctrl Pts',(-1.70345121691259,23.1718954368749,
0.));
#207413=CARTESIAN_POINT('Ctrl Pts',(-1.70345121691259,23.1718954368749,
12.));
#207414=CARTESIAN_POINT('Ctrl Pts',(-1.70063948926987,23.1881832981848,
0.));
#207415=CARTESIAN_POINT('Ctrl Pts',(-1.70063948926987,23.1881832981848,
12.));
#207416=CARTESIAN_POINT('Ctrl Pts',(-1.69775635099425,23.2045972243765,
0.));
#207417=CARTESIAN_POINT('Ctrl Pts',(-1.69775635099425,23.2045972243765,
12.));
#207418=CARTESIAN_POINT('Ctrl Pts',(-1.69480141959946,23.2211357709374,
0.));
#207419=CARTESIAN_POINT('Ctrl Pts',(-1.69480141959946,23.2211357709374,
12.));
#207420=CARTESIAN_POINT('Ctrl Pts',(-1.69177432121716,23.2377975177014,
0.));
#207421=CARTESIAN_POINT('Ctrl Pts',(-1.69177432121716,23.2377975177014,
12.));
#207422=CARTESIAN_POINT('Ctrl Pts',(-1.6886746903491,23.2545810680536,0.));
#207423=CARTESIAN_POINT('Ctrl Pts',(-1.6886746903491,23.2545810680536,12.));
#207424=CARTESIAN_POINT('Ctrl Pts',(-1.68550216963275,23.2714850482245,
0.));
#207425=CARTESIAN_POINT('Ctrl Pts',(-1.68550216963275,23.2714850482245,
12.));
#207426=CARTESIAN_POINT('Ctrl Pts',(-1.68225640962181,23.2885081066949,
0.));
#207427=CARTESIAN_POINT('Ctrl Pts',(-1.68225640962181,23.2885081066949,
12.));
#207428=CARTESIAN_POINT('Ctrl Pts',(-1.67893706857123,23.3056489135611,
0.));
#207429=CARTESIAN_POINT('Ctrl Pts',(-1.67893706857123,23.3056489135611,
12.));
#207430=CARTESIAN_POINT('Ctrl Pts',(-1.67554381222987,23.3229061599145,
0.));
#207431=CARTESIAN_POINT('Ctrl Pts',(-1.67554381222987,23.3229061599145,
12.));
#207432=CARTESIAN_POINT('Ctrl Pts',(-1.67207631363905,23.3402785571866,
0.));
#207433=CARTESIAN_POINT('Ctrl Pts',(-1.67207631363905,23.3402785571866,
12.));
#207434=CARTESIAN_POINT('Ctrl Pts',(-1.66853425293978,23.3577648365747,
0.));
#207435=CARTESIAN_POINT('Ctrl Pts',(-1.66853425293978,23.3577648365747,
12.));
#207436=CARTESIAN_POINT('Ctrl Pts',(-1.66491731718864,23.375363748555,0.));
#207437=CARTESIAN_POINT('Ctrl Pts',(-1.66491731718864,23.375363748555,12.));
#207438=CARTESIAN_POINT('Ctrl Pts',(-1.66122520018008,23.3930740623622,
0.));
#207439=CARTESIAN_POINT('Ctrl Pts',(-1.66122520018008,23.3930740623622,
12.));
#207440=CARTESIAN_POINT('Ctrl Pts',(-1.65745760227507,23.4108945654803,
0.));
#207441=CARTESIAN_POINT('Ctrl Pts',(-1.65745760227507,23.4108945654803,
12.));
#207442=CARTESIAN_POINT('Ctrl Pts',(-1.6536142302373,23.4288240631034,0.));
#207443=CARTESIAN_POINT('Ctrl Pts',(-1.6536142302373,23.4288240631034,12.));
#207444=CARTESIAN_POINT('Ctrl Pts',(-1.6496947970734,23.446861377656,0.));
#207445=CARTESIAN_POINT('Ctrl Pts',(-1.6496947970734,23.446861377656,12.));
#207446=CARTESIAN_POINT('Ctrl Pts',(-1.64569902187608,23.4650053483919,
0.));
#207447=CARTESIAN_POINT('Ctrl Pts',(-1.64569902187608,23.4650053483919,
12.));
#207448=CARTESIAN_POINT('Ctrl Pts',(-1.64162662967525,23.4832548309638,
0.));
#207449=CARTESIAN_POINT('Ctrl Pts',(-1.64162662967525,23.4832548309638,
12.));
#207450=CARTESIAN_POINT('Ctrl Pts',(-1.63747735129474,23.5016086970006,
0.));
#207451=CARTESIAN_POINT('Ctrl Pts',(-1.63747735129474,23.5016086970006,
12.));
#207452=CARTESIAN_POINT('Ctrl Pts',(-1.63325092321731,23.5200658336624,
0.));
#207453=CARTESIAN_POINT('Ctrl Pts',(-1.63325092321731,23.5200658336624,
12.));
#207454=CARTESIAN_POINT('Ctrl Pts',(-1.62894708745231,23.5386251432278,
0.));
#207455=CARTESIAN_POINT('Ctrl Pts',(-1.62894708745231,23.5386251432278,
12.));
#207456=CARTESIAN_POINT('Ctrl Pts',(-1.62456559140072,23.5572855427617,
0.));
#207457=CARTESIAN_POINT('Ctrl Pts',(-1.62456559140072,23.5572855427617,
12.));
#207458=CARTESIAN_POINT('Ctrl Pts',(-1.62010618772869,23.5760459637608,
0.));
#207459=CARTESIAN_POINT('Ctrl Pts',(-1.62010618772869,23.5760459637608,
12.));
#207460=CARTESIAN_POINT('Ctrl Pts',(-1.61556863424697,23.5949053517996,
0.));
#207461=CARTESIAN_POINT('Ctrl Pts',(-1.61556863424697,23.5949053517996,
12.));
#207462=CARTESIAN_POINT('Ctrl Pts',(-1.61095269379773,23.6138626661644,
0.));
#207463=CARTESIAN_POINT('Ctrl Pts',(-1.61095269379773,23.6138626661644,
12.));
#207464=CARTESIAN_POINT('Ctrl Pts',(-1.60625813414666,23.6329168794916,
0.));
#207465=CARTESIAN_POINT('Ctrl Pts',(-1.60625813414666,23.6329168794916,
12.));
#207466=CARTESIAN_POINT('Ctrl Pts',(-1.60148472786588,23.6520669774863,
0.));
#207467=CARTESIAN_POINT('Ctrl Pts',(-1.60148472786588,23.6520669774863,
12.));
#207468=CARTESIAN_POINT('Ctrl Pts',(-1.59663225222458,23.6713119586302,
0.));
#207469=CARTESIAN_POINT('Ctrl Pts',(-1.59663225222458,23.6713119586302,
12.));
#207470=CARTESIAN_POINT('Ctrl Pts',(-1.59170048908632,23.6906508338833,
0.));
#207471=CARTESIAN_POINT('Ctrl Pts',(-1.59170048908632,23.6906508338833,
12.));
#207472=CARTESIAN_POINT('Ctrl Pts',(-1.58668922481222,23.7100826263835,
0.));
#207473=CARTESIAN_POINT('Ctrl Pts',(-1.58668922481222,23.7100826263835,
12.));
#207474=CARTESIAN_POINT('Ctrl Pts',(-1.58159825017362,23.7296063711308,
0.));
#207475=CARTESIAN_POINT('Ctrl Pts',(-1.58159825017362,23.7296063711308,
12.));
#207476=CARTESIAN_POINT('Ctrl Pts',(-1.57642736025251,23.7492211147369,
0.));
#207477=CARTESIAN_POINT('Ctrl Pts',(-1.57642736025251,23.7492211147369,
12.));
#207478=CARTESIAN_POINT('Ctrl Pts',(-1.57117635434412,23.7689259151869,
0.));
#207479=CARTESIAN_POINT('Ctrl Pts',(-1.57117635434412,23.7689259151869,
12.));
#207480=CARTESIAN_POINT('Ctrl Pts',(-1.56584503586844,23.788719841588,0.));
#207481=CARTESIAN_POINT('Ctrl Pts',(-1.56584503586844,23.788719841588,12.));
#207482=CARTESIAN_POINT('Ctrl Pts',(-1.56043321228631,23.8086019739192,
0.));
#207483=CARTESIAN_POINT('Ctrl Pts',(-1.56043321228631,23.8086019739192,
12.));
#207484=CARTESIAN_POINT('Ctrl Pts',(-1.55494069502628,23.8285714027631,
0.));
#207485=CARTESIAN_POINT('Ctrl Pts',(-1.55494069502628,23.8285714027631,
12.));
#207486=CARTESIAN_POINT('Ctrl Pts',(-1.5493672994053,23.8486272290698,0.));
#207487=CARTESIAN_POINT('Ctrl Pts',(-1.5493672994053,23.8486272290698,12.));
#207488=CARTESIAN_POINT('Ctrl Pts',(-1.54371284453978,23.8687685639635,
0.));
#207489=CARTESIAN_POINT('Ctrl Pts',(-1.54371284453978,23.8687685639635,
12.));
#207490=CARTESIAN_POINT('Ctrl Pts',(-1.53797715326748,23.8889945285313,
0.));
#207491=CARTESIAN_POINT('Ctrl Pts',(-1.53797715326748,23.8889945285313,
12.));
#207492=CARTESIAN_POINT('Ctrl Pts',(-1.53216005207462,23.9093042536119,
0.));
#207493=CARTESIAN_POINT('Ctrl Pts',(-1.53216005207462,23.9093042536119,
12.));
#207494=CARTESIAN_POINT('Ctrl Pts',(-1.5262613710304,23.9296968795761,0.));
#207495=CARTESIAN_POINT('Ctrl Pts',(-1.5262613710304,23.9296968795761,12.));
#207496=CARTESIAN_POINT('Ctrl Pts',(-1.52028094372806,23.9501715561038,
0.));
#207497=CARTESIAN_POINT('Ctrl Pts',(-1.52028094372806,23.9501715561038,
12.));
#207498=CARTESIAN_POINT('Ctrl Pts',(-1.51421860720628,23.9707274420145,
0.));
#207499=CARTESIAN_POINT('Ctrl Pts',(-1.51421860720628,23.9707274420145,
12.));
#207500=CARTESIAN_POINT('Ctrl Pts',(-1.50807420187703,23.991363705093,0.));
#207501=CARTESIAN_POINT('Ctrl Pts',(-1.50807420187703,23.991363705093,12.));
#207502=CARTESIAN_POINT('Ctrl Pts',(-1.50184757146099,24.0120795219086,
0.));
#207503=CARTESIAN_POINT('Ctrl Pts',(-1.50184757146099,24.0120795219086,
12.));
#207504=CARTESIAN_POINT('Ctrl Pts',(-1.49553856292798,24.0328740776331,
0.));
#207505=CARTESIAN_POINT('Ctrl Pts',(-1.49553856292798,24.0328740776331,
12.));
#207506=CARTESIAN_POINT('Ctrl Pts',(-1.48914702644883,24.053746565843,0.));
#207507=CARTESIAN_POINT('Ctrl Pts',(-1.48914702644883,24.053746565843,12.));
#207508=CARTESIAN_POINT('Ctrl Pts',(-1.4826728153368,24.074696188353,0.));
#207509=CARTESIAN_POINT('Ctrl Pts',(-1.4826728153368,24.074696188353,12.));
#207510=CARTESIAN_POINT('Ctrl Pts',(-1.47611578597741,24.0957221550782,
0.));
#207511=CARTESIAN_POINT('Ctrl Pts',(-1.47611578597741,24.0957221550782,
12.));
#207512=CARTESIAN_POINT('Ctrl Pts',(-1.46947579776992,24.1168236838827,
0.));
#207513=CARTESIAN_POINT('Ctrl Pts',(-1.46947579776992,24.1168236838827,
12.));
#207514=CARTESIAN_POINT('Ctrl Pts',(-1.46275271307398,24.1380000004272,
0.));
#207515=CARTESIAN_POINT('Ctrl Pts',(-1.46275271307398,24.1380000004272,
12.));
#207516=CARTESIAN_POINT('Ctrl Pts',(-1.45594639716314,24.1592503380105,
0.));
#207517=CARTESIAN_POINT('Ctrl Pts',(-1.45594639716314,24.1592503380105,
12.));
#207518=CARTESIAN_POINT('Ctrl Pts',(-1.44905671818721,24.1805739374033,
0.));
#207519=CARTESIAN_POINT('Ctrl Pts',(-1.44905671818721,24.1805739374033,
12.));
#207520=CARTESIAN_POINT('Ctrl Pts',(-1.44208354711074,24.2019700467214,
0.));
#207521=CARTESIAN_POINT('Ctrl Pts',(-1.44208354711074,24.2019700467214,
12.));
#207522=CARTESIAN_POINT('Ctrl Pts',(-1.43502675765502,24.2234379212978,
0.));
#207523=CARTESIAN_POINT('Ctrl Pts',(-1.43502675765502,24.2234379212978,
12.));
#207524=CARTESIAN_POINT('Ctrl Pts',(-1.42788622624851,24.2449768235485,
0.));
#207525=CARTESIAN_POINT('Ctrl Pts',(-1.42788622624851,24.2449768235485,
12.));
#207526=CARTESIAN_POINT('Ctrl Pts',(-1.42066183198252,24.2665860228357,
0.));
#207527=CARTESIAN_POINT('Ctrl Pts',(-1.42066183198252,24.2665860228357,
12.));
#207528=CARTESIAN_POINT('Ctrl Pts',(-1.41335345657685,24.2882647953214,
0.));
#207529=CARTESIAN_POINT('Ctrl Pts',(-1.41335345657685,24.2882647953214,
12.));
#207530=CARTESIAN_POINT('Ctrl Pts',(-1.40596098434341,24.3100124238316,
0.));
#207531=CARTESIAN_POINT('Ctrl Pts',(-1.40596098434341,24.3100124238316,
12.));
#207532=CARTESIAN_POINT('Ctrl Pts',(-1.3984843021281,24.3318281977647,0.));
#207533=CARTESIAN_POINT('Ctrl Pts',(-1.3984843021281,24.3318281977647,12.));
#207534=CARTESIAN_POINT('Ctrl Pts',(-1.3909232992639,24.3537114129877,0.));
#207535=CARTESIAN_POINT('Ctrl Pts',(-1.3909232992639,24.3537114129877,12.));
#207536=CARTESIAN_POINT('Ctrl Pts',(-1.38327786752998,24.37566137173,0.));
#207537=CARTESIAN_POINT('Ctrl Pts',(-1.38327786752998,24.37566137173,12.));
#207538=CARTESIAN_POINT('Ctrl Pts',(-1.37554790111608,24.3976773824731,
0.));
#207539=CARTESIAN_POINT('Ctrl Pts',(-1.37554790111608,24.3976773824731,
12.));
#207540=CARTESIAN_POINT('Ctrl Pts',(-1.36773329659954,24.4197587598337,
0.));
#207541=CARTESIAN_POINT('Ctrl Pts',(-1.36773329659954,24.4197587598337,
12.));
#207542=CARTESIAN_POINT('Ctrl Pts',(-1.35983395290624,24.4419048244524,
0.));
#207543=CARTESIAN_POINT('Ctrl Pts',(-1.35983395290624,24.4419048244524,
12.));
#207544=CARTESIAN_POINT('Ctrl Pts',(-1.35184977125645,24.4641149028894,
0.));
#207545=CARTESIAN_POINT('Ctrl Pts',(-1.35184977125645,24.4641149028894,
12.));
#207546=CARTESIAN_POINT('Ctrl Pts',(-1.34378065512335,24.4863883275135,
0.));
#207547=CARTESIAN_POINT('Ctrl Pts',(-1.34378065512335,24.4863883275135,
12.));
#207548=CARTESIAN_POINT('Ctrl Pts',(-1.33562651019684,24.5087244363856,
0.));
#207549=CARTESIAN_POINT('Ctrl Pts',(-1.33562651019684,24.5087244363856,
12.));
#207550=CARTESIAN_POINT('Ctrl Pts',(-1.32738724435326,24.5311225731434,
0.));
#207551=CARTESIAN_POINT('Ctrl Pts',(-1.32738724435326,24.5311225731434,
12.));
#207552=CARTESIAN_POINT('Ctrl Pts',(-1.31906276763669,24.5535820868671,
0.));
#207553=CARTESIAN_POINT('Ctrl Pts',(-1.31906276763669,24.5535820868671,
12.));
#207554=CARTESIAN_POINT('Ctrl Pts',(-1.31065299222023,24.576102332018,0.));
#207555=CARTESIAN_POINT('Ctrl Pts',(-1.31065299222023,24.576102332018,12.));
#207556=CARTESIAN_POINT('Ctrl Pts',(-1.30215783236364,24.5986826684025,
0.));
#207557=CARTESIAN_POINT('Ctrl Pts',(-1.30215783236364,24.5986826684025,
12.));
#207558=CARTESIAN_POINT('Ctrl Pts',(-1.29357720438108,24.6213224611228,
0.));
#207559=CARTESIAN_POINT('Ctrl Pts',(-1.29357720438108,24.6213224611228,
12.));
#207560=CARTESIAN_POINT('Ctrl Pts',(-1.28491102661514,24.6440210805278,
0.));
#207561=CARTESIAN_POINT('Ctrl Pts',(-1.28491102661514,24.6440210805278,
12.));
#207562=CARTESIAN_POINT('Ctrl Pts',(-1.2761592194164,24.666777902156,0.));
#207563=CARTESIAN_POINT('Ctrl Pts',(-1.2761592194164,24.666777902156,12.));
#207564=CARTESIAN_POINT('Ctrl Pts',(-1.26732170513497,24.6895923066837,
0.));
#207565=CARTESIAN_POINT('Ctrl Pts',(-1.26732170513497,24.6895923066837,
12.));
#207566=CARTESIAN_POINT('Ctrl Pts',(-1.25839840807415,24.7124636797895,
0.));
#207567=CARTESIAN_POINT('Ctrl Pts',(-1.25839840807415,24.7124636797895,
12.));
#207568=CARTESIAN_POINT('Ctrl Pts',(-1.24938925444324,24.7353914120012,
0.));
#207569=CARTESIAN_POINT('Ctrl Pts',(-1.24938925444324,24.7353914120012,
12.));
#207570=CARTESIAN_POINT('Ctrl Pts',(-1.24029417231988,24.7583748985439,
0.));
#207571=CARTESIAN_POINT('Ctrl Pts',(-1.24029417231988,24.7583748985439,
12.));
#207572=CARTESIAN_POINT('Ctrl Pts',(-1.23111309161843,24.78141353918,0.));
#207573=CARTESIAN_POINT('Ctrl Pts',(-1.23111309161843,24.78141353918,12.));
#207574=CARTESIAN_POINT('Ctrl Pts',(-1.22184594406526,24.8045067380536,
0.));
#207575=CARTESIAN_POINT('Ctrl Pts',(-1.22184594406526,24.8045067380536,
12.));
#207576=CARTESIAN_POINT('Ctrl Pts',(-1.21249266318205,24.8276539035092,
0.));
#207577=CARTESIAN_POINT('Ctrl Pts',(-1.21249266318205,24.8276539035092,
12.));
#207578=CARTESIAN_POINT('Ctrl Pts',(-1.20305318426015,24.8508544481973,
0.));
#207579=CARTESIAN_POINT('Ctrl Pts',(-1.20305318426015,24.8508544481973,
12.));
#207580=CARTESIAN_POINT('Ctrl Pts',(-1.19352744434059,24.8741077892074,
0.));
#207581=CARTESIAN_POINT('Ctrl Pts',(-1.19352744434059,24.8741077892074,
12.));
#207582=CARTESIAN_POINT('Ctrl Pts',(-1.18391538220098,24.8974133481829,
0.));
#207583=CARTESIAN_POINT('Ctrl Pts',(-1.18391538220098,24.8974133481829,
12.));
#207584=CARTESIAN_POINT('Ctrl Pts',(-1.17421693835039,24.9207705514449,
0.));
#207585=CARTESIAN_POINT('Ctrl Pts',(-1.17421693835039,24.9207705514449,
12.));
#207586=CARTESIAN_POINT('Ctrl Pts',(-1.16443205502852,24.9441788300932,
0.));
#207587=CARTESIAN_POINT('Ctrl Pts',(-1.16443205502852,24.9441788300932,
12.));
#207588=CARTESIAN_POINT('Ctrl Pts',(-1.15456067621894,24.9676376201501,
0.));
#207589=CARTESIAN_POINT('Ctrl Pts',(-1.15456067621894,24.9676376201501,
12.));
#207590=CARTESIAN_POINT('Ctrl Pts',(-1.14460274758206,24.9911463621431,
0.));
#207591=CARTESIAN_POINT('Ctrl Pts',(-1.14460274758206,24.9911463621431,
12.));
#207592=CARTESIAN_POINT('Ctrl Pts',(-1.13455821638536,25.0147045006193,
0.));
#207593=CARTESIAN_POINT('Ctrl Pts',(-1.13455821638536,25.0147045006193,
12.));
#207594=CARTESIAN_POINT('Ctrl Pts',(-1.12442703144455,25.0383114836898,
0.));
#207595=CARTESIAN_POINT('Ctrl Pts',(-1.12442703144455,25.0383114836898,
12.));
#207596=CARTESIAN_POINT('Ctrl Pts',(-1.1142091430689,25.0619667625336,0.));
#207597=CARTESIAN_POINT('Ctrl Pts',(-1.1142091430689,25.0619667625336,12.));
#207598=CARTESIAN_POINT('Ctrl Pts',(-1.1039045030174,25.085669790968,0.));
#207599=CARTESIAN_POINT('Ctrl Pts',(-1.1039045030174,25.085669790968,12.));
#207600=CARTESIAN_POINT('Ctrl Pts',(-1.09351306445299,25.1094200248448,
0.));
#207601=CARTESIAN_POINT('Ctrl Pts',(-1.09351306445299,25.1094200248448,
12.));
#207602=CARTESIAN_POINT('Ctrl Pts',(-1.08303478197174,25.1332169227415,
0.));
#207603=CARTESIAN_POINT('Ctrl Pts',(-1.08303478197174,25.1332169227415,
12.));
#207604=CARTESIAN_POINT('Ctrl Pts',(-1.0724696116546,25.1570599469311,0.));
#207605=CARTESIAN_POINT('Ctrl Pts',(-1.0724696116546,25.1570599469311,12.));
#207606=CARTESIAN_POINT('Ctrl Pts',(-1.06181751111754,25.1809485642191,
0.));
#207607=CARTESIAN_POINT('Ctrl Pts',(-1.06181751111754,25.1809485642191,
12.));
#207608=CARTESIAN_POINT('Ctrl Pts',(-1.05107843957926,25.2048822469027,
0.));
#207609=CARTESIAN_POINT('Ctrl Pts',(-1.05107843957926,25.2048822469027,
12.));
#207610=CARTESIAN_POINT('Ctrl Pts',(-1.04025235791515,25.2288604735087,
0.));
#207611=CARTESIAN_POINT('Ctrl Pts',(-1.04025235791515,25.2288604735087,
12.));
#207612=CARTESIAN_POINT('Ctrl Pts',(-1.0293392287683,25.2528827300427,0.));
#207613=CARTESIAN_POINT('Ctrl Pts',(-1.0293392287683,25.2528827300427,12.));
#207614=CARTESIAN_POINT('Ctrl Pts',(-1.01833901642272,25.2769485087268,
0.));
#207615=CARTESIAN_POINT('Ctrl Pts',(-1.01833901642272,25.2769485087268,
12.));
#207616=CARTESIAN_POINT('Ctrl Pts',(-1.00725168656934,25.3010573055557,
0.));
#207617=CARTESIAN_POINT('Ctrl Pts',(-1.00725168656934,25.3010573055557,
12.));
#207618=CARTESIAN_POINT('Ctrl Pts',(-0.99607720612092,25.3252086182976,
0.));
#207619=CARTESIAN_POINT('Ctrl Pts',(-0.99607720612092,25.3252086182976,
12.));
#207620=CARTESIAN_POINT('Ctrl Pts',(-0.984815543004092,25.3494019441444,
0.));
#207621=CARTESIAN_POINT('Ctrl Pts',(-0.984815543004092,25.3494019441444,
12.));
#207622=CARTESIAN_POINT('Ctrl Pts',(-0.973466666000049,25.3736367778842,
0.));
#207623=CARTESIAN_POINT('Ctrl Pts',(-0.973466666000049,25.3736367778842,
12.));
#207624=CARTESIAN_POINT('Ctrl Pts',(-0.962030544502803,25.3979126089155,
0.));
#207625=CARTESIAN_POINT('Ctrl Pts',(-0.962030544502803,25.3979126089155,
12.));
#207626=CARTESIAN_POINT('Ctrl Pts',(-0.95050714859697,25.4222289223155,
0.));
#207627=CARTESIAN_POINT('Ctrl Pts',(-0.95050714859697,25.4222289223155,
12.));
#207628=CARTESIAN_POINT('Ctrl Pts',(-0.938896449495633,25.4465852044835,
0.));
#207629=CARTESIAN_POINT('Ctrl Pts',(-0.938896449495633,25.4465852044835,
12.));
#207630=CARTESIAN_POINT('Ctrl Pts',(-0.927198419885605,25.4709809474996,
0.));
#207631=CARTESIAN_POINT('Ctrl Pts',(-0.927198419885605,25.4709809474996,
12.));
#207632=CARTESIAN_POINT('Ctrl Pts',(-0.915413034335334,25.4954156541787,
0.));
#207633=CARTESIAN_POINT('Ctrl Pts',(-0.915413034335334,25.4954156541787,
12.));
#207634=CARTESIAN_POINT('Ctrl Pts',(-0.903540269651155,25.5198888424195,
0.));
#207635=CARTESIAN_POINT('Ctrl Pts',(-0.903540269651155,25.5198888424195,
12.));
#207636=CARTESIAN_POINT('Ctrl Pts',(-0.891580105349468,25.5444000508223,
0.));
#207637=CARTESIAN_POINT('Ctrl Pts',(-0.891580105349468,25.5444000508223,
12.));
#207638=CARTESIAN_POINT('Ctrl Pts',(-0.879532523835092,25.568948840818,
0.));
#207639=CARTESIAN_POINT('Ctrl Pts',(-0.879532523835092,25.568948840818,
12.));
#207640=CARTESIAN_POINT('Ctrl Pts',(-0.86739750933947,25.5935347843616,
0.));
#207641=CARTESIAN_POINT('Ctrl Pts',(-0.86739750933947,25.5935347843616,
12.));
#207642=CARTESIAN_POINT('Ctrl Pts',(-0.855175047037615,25.618157453608,
0.));
#207643=CARTESIAN_POINT('Ctrl Pts',(-0.855175047037615,25.618157453608,
12.));
#207644=CARTESIAN_POINT('Ctrl Pts',(-0.842865122121547,25.6428164100078,
0.));
#207645=CARTESIAN_POINT('Ctrl Pts',(-0.842865122121547,25.6428164100078,
12.));
#207646=CARTESIAN_POINT('Ctrl Pts',(-0.830467718864369,25.6675111931957,
0.));
#207647=CARTESIAN_POINT('Ctrl Pts',(-0.830467718864369,25.6675111931957,
12.));
#207648=CARTESIAN_POINT('Ctrl Pts',(-0.81798281978672,25.6922413110172,
0.));
#207649=CARTESIAN_POINT('Ctrl Pts',(-0.81798281978672,25.6922413110172,
12.));
#207650=CARTESIAN_POINT('Ctrl Pts',(-0.805410404552596,25.7170062262474,
0.));
#207651=CARTESIAN_POINT('Ctrl Pts',(-0.805410404552596,25.7170062262474,
12.));
#207652=CARTESIAN_POINT('Ctrl Pts',(-0.792750451613536,25.7418053757671,
0.));
#207653=CARTESIAN_POINT('Ctrl Pts',(-0.792750451613536,25.7418053757671,
12.));
#207654=CARTESIAN_POINT('Ctrl Pts',(-0.780002940289027,25.7666381946871,
0.));
#207655=CARTESIAN_POINT('Ctrl Pts',(-0.780002940289027,25.7666381946871,
12.));
#207656=CARTESIAN_POINT('Ctrl Pts',(-0.767167852648641,25.7915041383304,
0.));
#207657=CARTESIAN_POINT('Ctrl Pts',(-0.767167852648641,25.7915041383304,
12.));
#207658=CARTESIAN_POINT('Ctrl Pts',(-0.75424517560829,25.816402705995,0.));
#207659=CARTESIAN_POINT('Ctrl Pts',(-0.75424517560829,25.816402705995,12.));
#207660=CARTESIAN_POINT('Ctrl Pts',(-0.741234902664698,25.841333461908,
0.));
#207661=CARTESIAN_POINT('Ctrl Pts',(-0.741234902664698,25.841333461908,
12.));
#207662=CARTESIAN_POINT('Ctrl Pts',(-0.728137036485879,25.8662960624285,
0.));
#207663=CARTESIAN_POINT('Ctrl Pts',(-0.728137036485879,25.8662960624285,
12.));
#207664=CARTESIAN_POINT('Ctrl Pts',(-0.714951588533753,25.8912902615141,
0.));
#207665=CARTESIAN_POINT('Ctrl Pts',(-0.714951588533753,25.8912902615141,
12.));
#207666=CARTESIAN_POINT('Ctrl Pts',(-0.701678575236603,25.9163158909645,
0.));
#207667=CARTESIAN_POINT('Ctrl Pts',(-0.701678575236603,25.9163158909645,
12.));
#207668=CARTESIAN_POINT('Ctrl Pts',(-0.688318015065679,25.941372847213,
0.));
#207669=CARTESIAN_POINT('Ctrl Pts',(-0.688318015065679,25.941372847213,
12.));
#207670=CARTESIAN_POINT('Ctrl Pts',(-0.677559543215903,25.9614434298092,
0.));
#207671=CARTESIAN_POINT('Ctrl Pts',(-0.677559543215903,25.9614434298092,
12.));
#207672=CARTESIAN_POINT('Ctrl Pts',(-0.669451306784418,25.9765104298171,
0.));
#207673=CARTESIAN_POINT('Ctrl Pts',(-0.669451306784418,25.9765104298171,
12.));
#207674=CARTESIAN_POINT('Ctrl Pts',(-0.664028313188914,25.9865613464809,
0.));
#207675=CARTESIAN_POINT('Ctrl Pts',(-0.664028313188914,25.9865613464809,
12.));
#207676=CARTESIAN_POINT('Ctrl Pts',(-0.661312440730891,25.991588367311,
0.));
#207677=CARTESIAN_POINT('Ctrl Pts',(-0.661312440730891,25.991588367311,
12.));
#207678=CARTESIAN_POINT('',(-0.661312440730891,25.991588367311,0.));
#207679=CARTESIAN_POINT('Ctrl Pts',(-1.76341220531179,22.4835757167854,
0.));
#207680=CARTESIAN_POINT('Ctrl Pts',(-1.76341415538764,22.483581992979,0.));
#207681=CARTESIAN_POINT('Ctrl Pts',(-1.7634206426357,22.4836387052232,0.));
#207682=CARTESIAN_POINT('Ctrl Pts',(-1.76343813434565,22.483856251707,0.));
#207683=CARTESIAN_POINT('Ctrl Pts',(-1.76347698284792,22.4844112933129,
0.));
#207684=CARTESIAN_POINT('Ctrl Pts',(-1.76355076045546,22.4855446605991,
0.));
#207685=CARTESIAN_POINT('Ctrl Pts',(-1.76364784232963,22.4871115206571,
0.));
#207686=CARTESIAN_POINT('Ctrl Pts',(-1.76376424879505,22.4890991659478,
0.));
#207687=CARTESIAN_POINT('Ctrl Pts',(-1.76389475965724,22.4914909094908,
0.));
#207688=CARTESIAN_POINT('Ctrl Pts',(-1.76403393880301,22.4942693792449,
0.));
#207689=CARTESIAN_POINT('Ctrl Pts',(-1.76417731243462,22.4974203063191,
0.));
#207690=CARTESIAN_POINT('Ctrl Pts',(-1.76432160068725,22.5009332677316,
0.));
#207691=CARTESIAN_POINT('Ctrl Pts',(-1.76446408210366,22.5047996391978,
0.));
#207692=CARTESIAN_POINT('Ctrl Pts',(-1.76460218257323,22.5090112700212,
0.));
#207693=CARTESIAN_POINT('Ctrl Pts',(-1.76473303281159,22.5135590569554,
0.));
#207694=CARTESIAN_POINT('Ctrl Pts',(-1.76485369319896,22.5184336670207,
0.));
#207695=CARTESIAN_POINT('Ctrl Pts',(-1.76496128643369,22.5236259635515,
0.));
#207696=CARTESIAN_POINT('Ctrl Pts',(-1.76505320262752,22.529127665298,0.));
#207697=CARTESIAN_POINT('Ctrl Pts',(-1.7651271156325,22.5349313983571,0.));
#207698=CARTESIAN_POINT('Ctrl Pts',(-1.76518087841493,22.5410303590891,
0.));
#207699=CARTESIAN_POINT('Ctrl Pts',(-1.76521245524047,22.5474180954006,
0.));
#207700=CARTESIAN_POINT('Ctrl Pts',(-1.76521983384063,22.5540882235837,
0.));
#207701=CARTESIAN_POINT('Ctrl Pts',(-1.76520104500449,22.5610344912501,
0.));
#207702=CARTESIAN_POINT('Ctrl Pts',(-1.76515418518829,22.5682508499873,
0.));
#207703=CARTESIAN_POINT('Ctrl Pts',(-1.76507744026747,22.5757315316355,
0.));
#207704=CARTESIAN_POINT('Ctrl Pts',(-1.76496910283088,22.5834711038024,
0.));
#207705=CARTESIAN_POINT('Ctrl Pts',(-1.76482755288411,22.5914644078106,
0.));
#207706=CARTESIAN_POINT('Ctrl Pts',(-1.76465124413556,22.5997065145638,
0.));
#207707=CARTESIAN_POINT('Ctrl Pts',(-1.76443868648015,22.6081926681342,
0.));
#207708=CARTESIAN_POINT('Ctrl Pts',(-1.76418843543739,22.6169182517693,
0.));
#207709=CARTESIAN_POINT('Ctrl Pts',(-1.76389909571402,22.6258787994847,
0.));
#207710=CARTESIAN_POINT('Ctrl Pts',(-1.76356932176272,22.635069997936,0.));
#207711=CARTESIAN_POINT('Ctrl Pts',(-1.76319782013914,22.6444876940425,
0.));
#207712=CARTESIAN_POINT('Ctrl Pts',(-1.76278334912559,22.6541278938413,
0.));
#207713=CARTESIAN_POINT('Ctrl Pts',(-1.76232471392567,22.6639867471756,
0.));
#207714=CARTESIAN_POINT('Ctrl Pts',(-1.76182076289525,22.6740605356699,
0.));
#207715=CARTESIAN_POINT('Ctrl Pts',(-1.76127038310613,22.6843456585245,
0.));
#207716=CARTESIAN_POINT('Ctrl Pts',(-1.76067249704884,22.6948386219843,
0.));
#207717=CARTESIAN_POINT('Ctrl Pts',(-1.76002606202399,22.7055360375481,
0.));
#207718=CARTESIAN_POINT('Ctrl Pts',(-1.75933006905924,22.7164346186007,
0.));
#207719=CARTESIAN_POINT('Ctrl Pts',(-1.75858354204635,22.7275311777305,
0.));
#207720=CARTESIAN_POINT('Ctrl Pts',(-1.75778553673249,22.7388226235565,
0.));
#207721=CARTESIAN_POINT('Ctrl Pts',(-1.75693513908911,22.7503059556455,
0.));
#207722=CARTESIAN_POINT('Ctrl Pts',(-1.7560314637164,22.7619782595013,0.));
#207723=CARTESIAN_POINT('Ctrl Pts',(-1.75507365227127,22.7738367016115,
0.));
#207724=CARTESIAN_POINT('Ctrl Pts',(-1.7540608718293,22.7858785242358,0.));
#207725=CARTESIAN_POINT('Ctrl Pts',(-1.75299231391461,22.7981010424312,
0.));
#207726=CARTESIAN_POINT('Ctrl Pts',(-1.7518671936559,22.8105016414712,0.));
#207727=CARTESIAN_POINT('Ctrl Pts',(-1.75068474890884,22.8230777741285,
0.));
#207728=CARTESIAN_POINT('Ctrl Pts',(-1.74944423940117,22.8358269579854,
0.));
#207729=CARTESIAN_POINT('Ctrl Pts',(-1.74814494588492,22.8487467728075,
0.));
#207730=CARTESIAN_POINT('Ctrl Pts',(-1.74678616930663,22.8618348580234,
0.));
#207731=CARTESIAN_POINT('Ctrl Pts',(-1.745367229982,22.8750889101696,0.));
#207732=CARTESIAN_POINT('Ctrl Pts',(-1.74388746677702,22.8885066803351,
0.));
#207733=CARTESIAN_POINT('Ctrl Pts',(-1.74234623630079,22.9020859716144,
0.));
#207734=CARTESIAN_POINT('Ctrl Pts',(-1.74074291231057,22.9158246373365,
0.));
#207735=CARTESIAN_POINT('Ctrl Pts',(-1.73907688511664,22.9297205792587,
0.));
#207736=CARTESIAN_POINT('Ctrl Pts',(-1.73734756100038,22.9437717457825,
0.));
#207737=CARTESIAN_POINT('Ctrl Pts',(-1.73555436162771,22.9579761301062,
0.));
#207738=CARTESIAN_POINT('Ctrl Pts',(-1.73369672350818,22.9723317685688,
0.));
#207739=CARTESIAN_POINT('Ctrl Pts',(-1.73177409750194,22.9868367391978,
0.));
#207740=CARTESIAN_POINT('Ctrl Pts',(-1.72978594832137,23.0014891601891,
0.));
#207741=CARTESIAN_POINT('Ctrl Pts',(-1.72773175404703,23.0162871884167,
0.));
#207742=CARTESIAN_POINT('Ctrl Pts',(-1.72561100564033,23.031229017888,0.));
#207743=CARTESIAN_POINT('Ctrl Pts',(-1.72342320653731,23.0463128785528,
0.));
#207744=CARTESIAN_POINT('Ctrl Pts',(-1.7211678722598,23.061537035156,0.));
#207745=CARTESIAN_POINT('Ctrl Pts',(-1.71884453003027,23.0768997860709,
0.));
#207746=CARTESIAN_POINT('Ctrl Pts',(-1.71645271839311,23.0923994621216,
0.));
#207747=CARTESIAN_POINT('Ctrl Pts',(-1.71399198684725,23.1080344254291,
0.));
#207748=CARTESIAN_POINT('Ctrl Pts',(-1.71146189552192,23.1238030684929,
0.));
#207749=CARTESIAN_POINT('Ctrl Pts',(-1.7088620148546,23.1397038132358,0.));
#207750=CARTESIAN_POINT('Ctrl Pts',(-1.70619192527847,23.1557351100613,
0.));
#207751=CARTESIAN_POINT('Ctrl Pts',(-1.70345121691259,23.1718954368749,
0.));
#207752=CARTESIAN_POINT('Ctrl Pts',(-1.70063948926987,23.1881832981848,
0.));
#207753=CARTESIAN_POINT('Ctrl Pts',(-1.69775635099425,23.2045972243765,
0.));
#207754=CARTESIAN_POINT('Ctrl Pts',(-1.69480141959946,23.2211357709374,
0.));
#207755=CARTESIAN_POINT('Ctrl Pts',(-1.69177432121716,23.2377975177014,
0.));
#207756=CARTESIAN_POINT('Ctrl Pts',(-1.6886746903491,23.2545810680536,0.));
#207757=CARTESIAN_POINT('Ctrl Pts',(-1.68550216963275,23.2714850482245,
0.));
#207758=CARTESIAN_POINT('Ctrl Pts',(-1.68225640962181,23.2885081066949,
0.));
#207759=CARTESIAN_POINT('Ctrl Pts',(-1.67893706857123,23.3056489135611,
0.));
#207760=CARTESIAN_POINT('Ctrl Pts',(-1.67554381222987,23.3229061599145,
0.));
#207761=CARTESIAN_POINT('Ctrl Pts',(-1.67207631363905,23.3402785571866,
0.));
#207762=CARTESIAN_POINT('Ctrl Pts',(-1.66853425293978,23.3577648365747,
0.));
#207763=CARTESIAN_POINT('Ctrl Pts',(-1.66491731718864,23.375363748555,0.));
#207764=CARTESIAN_POINT('Ctrl Pts',(-1.66122520018008,23.3930740623622,
0.));
#207765=CARTESIAN_POINT('Ctrl Pts',(-1.65745760227507,23.4108945654803,
0.));
#207766=CARTESIAN_POINT('Ctrl Pts',(-1.6536142302373,23.4288240631034,0.));
#207767=CARTESIAN_POINT('Ctrl Pts',(-1.6496947970734,23.446861377656,0.));
#207768=CARTESIAN_POINT('Ctrl Pts',(-1.64569902187608,23.4650053483919,
0.));
#207769=CARTESIAN_POINT('Ctrl Pts',(-1.64162662967525,23.4832548309638,
0.));
#207770=CARTESIAN_POINT('Ctrl Pts',(-1.63747735129474,23.5016086970006,
0.));
#207771=CARTESIAN_POINT('Ctrl Pts',(-1.63325092321731,23.5200658336624,
0.));
#207772=CARTESIAN_POINT('Ctrl Pts',(-1.62894708745231,23.5386251432278,
0.));
#207773=CARTESIAN_POINT('Ctrl Pts',(-1.62456559140072,23.5572855427617,
0.));
#207774=CARTESIAN_POINT('Ctrl Pts',(-1.62010618772869,23.5760459637608,
0.));
#207775=CARTESIAN_POINT('Ctrl Pts',(-1.61556863424697,23.5949053517996,
0.));
#207776=CARTESIAN_POINT('Ctrl Pts',(-1.61095269379773,23.6138626661644,
0.));
#207777=CARTESIAN_POINT('Ctrl Pts',(-1.60625813414666,23.6329168794916,
0.));
#207778=CARTESIAN_POINT('Ctrl Pts',(-1.60148472786588,23.6520669774863,
0.));
#207779=CARTESIAN_POINT('Ctrl Pts',(-1.59663225222458,23.6713119586302,
0.));
#207780=CARTESIAN_POINT('Ctrl Pts',(-1.59170048908632,23.6906508338833,
0.));
#207781=CARTESIAN_POINT('Ctrl Pts',(-1.58668922481222,23.7100826263835,
0.));
#207782=CARTESIAN_POINT('Ctrl Pts',(-1.58159825017362,23.7296063711308,
0.));
#207783=CARTESIAN_POINT('Ctrl Pts',(-1.57642736025251,23.7492211147369,
0.));
#207784=CARTESIAN_POINT('Ctrl Pts',(-1.57117635434412,23.7689259151869,
0.));
#207785=CARTESIAN_POINT('Ctrl Pts',(-1.56584503586844,23.788719841588,0.));
#207786=CARTESIAN_POINT('Ctrl Pts',(-1.56043321228631,23.8086019739192,
0.));
#207787=CARTESIAN_POINT('Ctrl Pts',(-1.55494069502628,23.8285714027631,
0.));
#207788=CARTESIAN_POINT('Ctrl Pts',(-1.5493672994053,23.8486272290698,0.));
#207789=CARTESIAN_POINT('Ctrl Pts',(-1.54371284453978,23.8687685639635,
0.));
#207790=CARTESIAN_POINT('Ctrl Pts',(-1.53797715326748,23.8889945285313,
0.));
#207791=CARTESIAN_POINT('Ctrl Pts',(-1.53216005207462,23.9093042536119,
0.));
#207792=CARTESIAN_POINT('Ctrl Pts',(-1.5262613710304,23.9296968795761,0.));
#207793=CARTESIAN_POINT('Ctrl Pts',(-1.52028094372806,23.9501715561038,
0.));
#207794=CARTESIAN_POINT('Ctrl Pts',(-1.51421860720628,23.9707274420145,
0.));
#207795=CARTESIAN_POINT('Ctrl Pts',(-1.50807420187703,23.991363705093,0.));
#207796=CARTESIAN_POINT('Ctrl Pts',(-1.50184757146099,24.0120795219086,
0.));
#207797=CARTESIAN_POINT('Ctrl Pts',(-1.49553856292798,24.0328740776331,
0.));
#207798=CARTESIAN_POINT('Ctrl Pts',(-1.48914702644883,24.053746565843,0.));
#207799=CARTESIAN_POINT('Ctrl Pts',(-1.4826728153368,24.074696188353,0.));
#207800=CARTESIAN_POINT('Ctrl Pts',(-1.47611578597741,24.0957221550782,
0.));
#207801=CARTESIAN_POINT('Ctrl Pts',(-1.46947579776992,24.1168236838827,
0.));
#207802=CARTESIAN_POINT('Ctrl Pts',(-1.46275271307398,24.1380000004272,
0.));
#207803=CARTESIAN_POINT('Ctrl Pts',(-1.45594639716314,24.1592503380105,
0.));
#207804=CARTESIAN_POINT('Ctrl Pts',(-1.44905671818721,24.1805739374033,
0.));
#207805=CARTESIAN_POINT('Ctrl Pts',(-1.44208354711074,24.2019700467214,
0.));
#207806=CARTESIAN_POINT('Ctrl Pts',(-1.43502675765502,24.2234379212978,
0.));
#207807=CARTESIAN_POINT('Ctrl Pts',(-1.42788622624851,24.2449768235485,
0.));
#207808=CARTESIAN_POINT('Ctrl Pts',(-1.42066183198252,24.2665860228357,
0.));
#207809=CARTESIAN_POINT('Ctrl Pts',(-1.41335345657685,24.2882647953214,
0.));
#207810=CARTESIAN_POINT('Ctrl Pts',(-1.40596098434341,24.3100124238316,
0.));
#207811=CARTESIAN_POINT('Ctrl Pts',(-1.3984843021281,24.3318281977647,0.));
#207812=CARTESIAN_POINT('Ctrl Pts',(-1.3909232992639,24.3537114129877,0.));
#207813=CARTESIAN_POINT('Ctrl Pts',(-1.38327786752998,24.37566137173,0.));
#207814=CARTESIAN_POINT('Ctrl Pts',(-1.37554790111608,24.3976773824731,
0.));
#207815=CARTESIAN_POINT('Ctrl Pts',(-1.36773329659954,24.4197587598337,
0.));
#207816=CARTESIAN_POINT('Ctrl Pts',(-1.35983395290624,24.4419048244524,
0.));
#207817=CARTESIAN_POINT('Ctrl Pts',(-1.35184977125645,24.4641149028894,
0.));
#207818=CARTESIAN_POINT('Ctrl Pts',(-1.34378065512335,24.4863883275135,
0.));
#207819=CARTESIAN_POINT('Ctrl Pts',(-1.33562651019684,24.5087244363856,
0.));
#207820=CARTESIAN_POINT('Ctrl Pts',(-1.32738724435326,24.5311225731434,
0.));
#207821=CARTESIAN_POINT('Ctrl Pts',(-1.31906276763669,24.5535820868671,
0.));
#207822=CARTESIAN_POINT('Ctrl Pts',(-1.31065299222023,24.576102332018,0.));
#207823=CARTESIAN_POINT('Ctrl Pts',(-1.30215783236364,24.5986826684025,
0.));
#207824=CARTESIAN_POINT('Ctrl Pts',(-1.29357720438108,24.6213224611228,
0.));
#207825=CARTESIAN_POINT('Ctrl Pts',(-1.28491102661514,24.6440210805278,
0.));
#207826=CARTESIAN_POINT('Ctrl Pts',(-1.2761592194164,24.666777902156,0.));
#207827=CARTESIAN_POINT('Ctrl Pts',(-1.26732170513497,24.6895923066837,
0.));
#207828=CARTESIAN_POINT('Ctrl Pts',(-1.25839840807415,24.7124636797895,
0.));
#207829=CARTESIAN_POINT('Ctrl Pts',(-1.24938925444324,24.7353914120012,
0.));
#207830=CARTESIAN_POINT('Ctrl Pts',(-1.24029417231988,24.7583748985439,
0.));
#207831=CARTESIAN_POINT('Ctrl Pts',(-1.23111309161843,24.78141353918,0.));
#207832=CARTESIAN_POINT('Ctrl Pts',(-1.22184594406526,24.8045067380536,
0.));
#207833=CARTESIAN_POINT('Ctrl Pts',(-1.21249266318205,24.8276539035092,
0.));
#207834=CARTESIAN_POINT('Ctrl Pts',(-1.20305318426015,24.8508544481973,
0.));
#207835=CARTESIAN_POINT('Ctrl Pts',(-1.19352744434059,24.8741077892074,
0.));
#207836=CARTESIAN_POINT('Ctrl Pts',(-1.18391538220098,24.8974133481829,
0.));
#207837=CARTESIAN_POINT('Ctrl Pts',(-1.17421693835039,24.9207705514449,
0.));
#207838=CARTESIAN_POINT('Ctrl Pts',(-1.16443205502852,24.9441788300932,
0.));
#207839=CARTESIAN_POINT('Ctrl Pts',(-1.15456067621894,24.9676376201501,
0.));
#207840=CARTESIAN_POINT('Ctrl Pts',(-1.14460274758206,24.9911463621431,
0.));
#207841=CARTESIAN_POINT('Ctrl Pts',(-1.13455821638536,25.0147045006193,
0.));
#207842=CARTESIAN_POINT('Ctrl Pts',(-1.12442703144455,25.0383114836898,
0.));
#207843=CARTESIAN_POINT('Ctrl Pts',(-1.1142091430689,25.0619667625336,0.));
#207844=CARTESIAN_POINT('Ctrl Pts',(-1.1039045030174,25.085669790968,0.));
#207845=CARTESIAN_POINT('Ctrl Pts',(-1.09351306445299,25.1094200248448,
0.));
#207846=CARTESIAN_POINT('Ctrl Pts',(-1.08303478197174,25.1332169227415,
0.));
#207847=CARTESIAN_POINT('Ctrl Pts',(-1.0724696116546,25.1570599469311,0.));
#207848=CARTESIAN_POINT('Ctrl Pts',(-1.06181751111754,25.1809485642191,
0.));
#207849=CARTESIAN_POINT('Ctrl Pts',(-1.05107843957926,25.2048822469027,
0.));
#207850=CARTESIAN_POINT('Ctrl Pts',(-1.04025235791515,25.2288604735087,
0.));
#207851=CARTESIAN_POINT('Ctrl Pts',(-1.0293392287683,25.2528827300427,0.));
#207852=CARTESIAN_POINT('Ctrl Pts',(-1.01833901642272,25.2769485087268,
0.));
#207853=CARTESIAN_POINT('Ctrl Pts',(-1.00725168656934,25.3010573055557,
0.));
#207854=CARTESIAN_POINT('Ctrl Pts',(-0.99607720612092,25.3252086182976,
0.));
#207855=CARTESIAN_POINT('Ctrl Pts',(-0.984815543004092,25.3494019441444,
0.));
#207856=CARTESIAN_POINT('Ctrl Pts',(-0.973466666000049,25.3736367778842,
0.));
#207857=CARTESIAN_POINT('Ctrl Pts',(-0.962030544502803,25.3979126089155,
0.));
#207858=CARTESIAN_POINT('Ctrl Pts',(-0.95050714859697,25.4222289223155,
0.));
#207859=CARTESIAN_POINT('Ctrl Pts',(-0.938896449495633,25.4465852044835,
0.));
#207860=CARTESIAN_POINT('Ctrl Pts',(-0.927198419885605,25.4709809474996,
0.));
#207861=CARTESIAN_POINT('Ctrl Pts',(-0.915413034335334,25.4954156541787,
0.));
#207862=CARTESIAN_POINT('Ctrl Pts',(-0.903540269651155,25.5198888424195,
0.));
#207863=CARTESIAN_POINT('Ctrl Pts',(-0.891580105349468,25.5444000508223,
0.));
#207864=CARTESIAN_POINT('Ctrl Pts',(-0.879532523835092,25.568948840818,
0.));
#207865=CARTESIAN_POINT('Ctrl Pts',(-0.86739750933947,25.5935347843616,
0.));
#207866=CARTESIAN_POINT('Ctrl Pts',(-0.855175047037615,25.618157453608,
0.));
#207867=CARTESIAN_POINT('Ctrl Pts',(-0.842865122121547,25.6428164100078,
0.));
#207868=CARTESIAN_POINT('Ctrl Pts',(-0.830467718864369,25.6675111931957,
0.));
#207869=CARTESIAN_POINT('Ctrl Pts',(-0.81798281978672,25.6922413110172,
0.));
#207870=CARTESIAN_POINT('Ctrl Pts',(-0.805410404552596,25.7170062262474,
0.));
#207871=CARTESIAN_POINT('Ctrl Pts',(-0.792750451613536,25.7418053757671,
0.));
#207872=CARTESIAN_POINT('Ctrl Pts',(-0.780002940289027,25.7666381946871,
0.));
#207873=CARTESIAN_POINT('Ctrl Pts',(-0.767167852648641,25.7915041383304,
0.));
#207874=CARTESIAN_POINT('Ctrl Pts',(-0.75424517560829,25.816402705995,0.));
#207875=CARTESIAN_POINT('Ctrl Pts',(-0.741234902664698,25.841333461908,
0.));
#207876=CARTESIAN_POINT('Ctrl Pts',(-0.728137036485879,25.8662960624285,
0.));
#207877=CARTESIAN_POINT('Ctrl Pts',(-0.714951588533753,25.8912902615141,
0.));
#207878=CARTESIAN_POINT('Ctrl Pts',(-0.701678575236603,25.9163158909645,
0.));
#207879=CARTESIAN_POINT('Ctrl Pts',(-0.688318015065679,25.941372847213,
0.));
#207880=CARTESIAN_POINT('Ctrl Pts',(-0.677559543215903,25.9614434298092,
0.));
#207881=CARTESIAN_POINT('Ctrl Pts',(-0.669451306784418,25.9765104298171,
0.));
#207882=CARTESIAN_POINT('Ctrl Pts',(-0.664028313188914,25.9865613464809,
0.));
#207883=CARTESIAN_POINT('Ctrl Pts',(-0.661312440730891,25.991588367311,
0.));
#207884=CARTESIAN_POINT('',(-0.661312440730891,25.991588367311,0.));
#207885=CARTESIAN_POINT('Origin',(3.92374859571501,21.1389261070099,0.));
#207886=CARTESIAN_POINT('',(4.11585220600461,22.1738711152697,0.));
#207887=CARTESIAN_POINT('',(4.11585220600461,22.1738711152697,0.));
#207888=CARTESIAN_POINT('',(1.96187429785751,10.5694630535049,0.));
#207889=CARTESIAN_POINT('Ctrl Pts',(0.661312440730901,25.991588367311,0.));
#207890=CARTESIAN_POINT('Ctrl Pts',(0.661312440730901,25.991588367311,12.));
#207891=CARTESIAN_POINT('Ctrl Pts',(0.664028313187627,25.9865613464773,
0.));
#207892=CARTESIAN_POINT('Ctrl Pts',(0.664028313187627,25.9865613464773,
12.));
#207893=CARTESIAN_POINT('Ctrl Pts',(0.669451306780825,25.9765104298071,
0.));
#207894=CARTESIAN_POINT('Ctrl Pts',(0.669451306780825,25.9765104298071,
12.));
#207895=CARTESIAN_POINT('Ctrl Pts',(0.677559543209725,25.9614434297919,
0.));
#207896=CARTESIAN_POINT('Ctrl Pts',(0.677559543209725,25.9614434297919,
12.));
#207897=CARTESIAN_POINT('Ctrl Pts',(0.688318015057729,25.9413728471909,
0.));
#207898=CARTESIAN_POINT('Ctrl Pts',(0.688318015057729,25.9413728471909,
12.));
#207899=CARTESIAN_POINT('Ctrl Pts',(0.701678575228756,25.9163158909426,
0.));
#207900=CARTESIAN_POINT('Ctrl Pts',(0.701678575228756,25.9163158909426,
12.));
#207901=CARTESIAN_POINT('Ctrl Pts',(0.714951588527638,25.891290261497,0.));
#207902=CARTESIAN_POINT('Ctrl Pts',(0.714951588527638,25.891290261497,12.));
#207903=CARTESIAN_POINT('Ctrl Pts',(0.728137036482335,25.8662960624185,
0.));
#207904=CARTESIAN_POINT('Ctrl Pts',(0.728137036482335,25.8662960624185,
12.));
#207905=CARTESIAN_POINT('Ctrl Pts',(0.741234902663807,25.8413334619055,
0.));
#207906=CARTESIAN_POINT('Ctrl Pts',(0.741234902663807,25.8413334619055,
12.));
#207907=CARTESIAN_POINT('Ctrl Pts',(0.754245175609524,25.8164027059984,
0.));
#207908=CARTESIAN_POINT('Ctrl Pts',(0.754245175609524,25.8164027059984,
12.));
#207909=CARTESIAN_POINT('Ctrl Pts',(0.767167852651168,25.7915041383376,
0.));
#207910=CARTESIAN_POINT('Ctrl Pts',(0.767167852651168,25.7915041383376,
12.));
#207911=CARTESIAN_POINT('Ctrl Pts',(0.780002940291965,25.7666381946955,
0.));
#207912=CARTESIAN_POINT('Ctrl Pts',(0.780002940291965,25.7666381946955,
12.));
#207913=CARTESIAN_POINT('Ctrl Pts',(0.792750451616127,25.7418053757746,
0.));
#207914=CARTESIAN_POINT('Ctrl Pts',(0.792750451616127,25.7418053757746,
12.));
#207915=CARTESIAN_POINT('Ctrl Pts',(0.805410404554352,25.7170062262525,
0.));
#207916=CARTESIAN_POINT('Ctrl Pts',(0.805410404554352,25.7170062262525,
12.));
#207917=CARTESIAN_POINT('Ctrl Pts',(0.817982819787464,25.6922413110194,
0.));
#207918=CARTESIAN_POINT('Ctrl Pts',(0.817982819787464,25.6922413110194,
12.));
#207919=CARTESIAN_POINT('Ctrl Pts',(0.830467718864205,25.6675111931952,
0.));
#207920=CARTESIAN_POINT('Ctrl Pts',(0.830467718864205,25.6675111931952,
12.));
#207921=CARTESIAN_POINT('Ctrl Pts',(0.842865122120758,25.6428164100055,
0.));
#207922=CARTESIAN_POINT('Ctrl Pts',(0.842865122120758,25.6428164100055,
12.));
#207923=CARTESIAN_POINT('Ctrl Pts',(0.855175047036549,25.6181574536049,
0.));
#207924=CARTESIAN_POINT('Ctrl Pts',(0.855175047036549,25.6181574536049,
12.));
#207925=CARTESIAN_POINT('Ctrl Pts',(0.867397509338431,25.5935347843585,
0.));
#207926=CARTESIAN_POINT('Ctrl Pts',(0.867397509338431,25.5935347843585,
12.));
#207927=CARTESIAN_POINT('Ctrl Pts',(0.879532523834294,25.5689488408156,
0.));
#207928=CARTESIAN_POINT('Ctrl Pts',(0.879532523834294,25.5689488408156,
12.));
#207929=CARTESIAN_POINT('Ctrl Pts',(0.89158010534904,25.5444000508211,0.));
#207930=CARTESIAN_POINT('Ctrl Pts',(0.89158010534904,25.5444000508211,12.));
#207931=CARTESIAN_POINT('Ctrl Pts',(0.903540269651106,25.5198888424194,
0.));
#207932=CARTESIAN_POINT('Ctrl Pts',(0.903540269651106,25.5198888424194,
12.));
#207933=CARTESIAN_POINT('Ctrl Pts',(0.915413034335613,25.4954156541795,
0.));
#207934=CARTESIAN_POINT('Ctrl Pts',(0.915413034335613,25.4954156541795,
12.));
#207935=CARTESIAN_POINT('Ctrl Pts',(0.927198419886094,25.4709809475009,
0.));
#207936=CARTESIAN_POINT('Ctrl Pts',(0.927198419886094,25.4709809475009,
12.));
#207937=CARTESIAN_POINT('Ctrl Pts',(0.938896449496192,25.4465852044849,
0.));
#207938=CARTESIAN_POINT('Ctrl Pts',(0.938896449496192,25.4465852044849,
12.));
#207939=CARTESIAN_POINT('Ctrl Pts',(0.950507148597468,25.4222289223167,
0.));
#207940=CARTESIAN_POINT('Ctrl Pts',(0.950507148597468,25.4222289223167,
12.));
#207941=CARTESIAN_POINT('Ctrl Pts',(0.962030544503142,25.3979126089163,
0.));
#207942=CARTESIAN_POINT('Ctrl Pts',(0.962030544503142,25.3979126089163,
12.));
#207943=CARTESIAN_POINT('Ctrl Pts',(0.973466666000163,25.3736367778845,
0.));
#207944=CARTESIAN_POINT('Ctrl Pts',(0.973466666000163,25.3736367778845,
12.));
#207945=CARTESIAN_POINT('Ctrl Pts',(0.984815543003973,25.3494019441441,
0.));
#207946=CARTESIAN_POINT('Ctrl Pts',(0.984815543003973,25.3494019441441,
12.));
#207947=CARTESIAN_POINT('Ctrl Pts',(0.996077206120624,25.3252086182968,
0.));
#207948=CARTESIAN_POINT('Ctrl Pts',(0.996077206120624,25.3252086182968,
12.));
#207949=CARTESIAN_POINT('Ctrl Pts',(1.00725168656896,25.3010573055547,0.));
#207950=CARTESIAN_POINT('Ctrl Pts',(1.00725168656896,25.3010573055547,12.));
#207951=CARTESIAN_POINT('Ctrl Pts',(1.01833901642237,25.276948508726,0.));
#207952=CARTESIAN_POINT('Ctrl Pts',(1.01833901642237,25.276948508726,12.));
#207953=CARTESIAN_POINT('Ctrl Pts',(1.02933922876806,25.2528827300422,0.));
#207954=CARTESIAN_POINT('Ctrl Pts',(1.02933922876806,25.2528827300422,12.));
#207955=CARTESIAN_POINT('Ctrl Pts',(1.04025235791507,25.2288604735086,0.));
#207956=CARTESIAN_POINT('Ctrl Pts',(1.04025235791507,25.2288604735086,12.));
#207957=CARTESIAN_POINT('Ctrl Pts',(1.05107843957931,25.2048822469028,0.));
#207958=CARTESIAN_POINT('Ctrl Pts',(1.05107843957931,25.2048822469028,12.));
#207959=CARTESIAN_POINT('Ctrl Pts',(1.06181751111768,25.1809485642192,0.));
#207960=CARTESIAN_POINT('Ctrl Pts',(1.06181751111768,25.1809485642192,12.));
#207961=CARTESIAN_POINT('Ctrl Pts',(1.07246961165475,25.157059946931,0.));
#207962=CARTESIAN_POINT('Ctrl Pts',(1.07246961165475,25.157059946931,12.));
#207963=CARTESIAN_POINT('Ctrl Pts',(1.08303478197187,25.1332169227413,0.));
#207964=CARTESIAN_POINT('Ctrl Pts',(1.08303478197187,25.1332169227413,12.));
#207965=CARTESIAN_POINT('Ctrl Pts',(1.09351306445308,25.1094200248446,0.));
#207966=CARTESIAN_POINT('Ctrl Pts',(1.09351306445308,25.1094200248446,12.));
#207967=CARTESIAN_POINT('Ctrl Pts',(1.10390450301745,25.0856697909679,0.));
#207968=CARTESIAN_POINT('Ctrl Pts',(1.10390450301745,25.0856697909679,12.));
#207969=CARTESIAN_POINT('Ctrl Pts',(1.11420914306889,25.0619667625336,0.));
#207970=CARTESIAN_POINT('Ctrl Pts',(1.11420914306889,25.0619667625336,12.));
#207971=CARTESIAN_POINT('Ctrl Pts',(1.12442703144451,25.0383114836899,0.));
#207972=CARTESIAN_POINT('Ctrl Pts',(1.12442703144451,25.0383114836899,12.));
#207973=CARTESIAN_POINT('Ctrl Pts',(1.1345582163853,25.0147045006196,0.));
#207974=CARTESIAN_POINT('Ctrl Pts',(1.1345582163853,25.0147045006196,12.));
#207975=CARTESIAN_POINT('Ctrl Pts',(1.144602747582,24.9911463621433,0.));
#207976=CARTESIAN_POINT('Ctrl Pts',(1.144602747582,24.9911463621433,12.));
#207977=CARTESIAN_POINT('Ctrl Pts',(1.15456067621889,24.9676376201502,0.));
#207978=CARTESIAN_POINT('Ctrl Pts',(1.15456067621889,24.9676376201502,12.));
#207979=CARTESIAN_POINT('Ctrl Pts',(1.16443205502849,24.9441788300932,0.));
#207980=CARTESIAN_POINT('Ctrl Pts',(1.16443205502849,24.9441788300932,12.));
#207981=CARTESIAN_POINT('Ctrl Pts',(1.17421693835041,24.9207705514449,0.));
#207982=CARTESIAN_POINT('Ctrl Pts',(1.17421693835041,24.9207705514449,12.));
#207983=CARTESIAN_POINT('Ctrl Pts',(1.18391538220103,24.8974133481829,0.));
#207984=CARTESIAN_POINT('Ctrl Pts',(1.18391538220103,24.8974133481829,12.));
#207985=CARTESIAN_POINT('Ctrl Pts',(1.19352744434064,24.8741077892075,0.));
#207986=CARTESIAN_POINT('Ctrl Pts',(1.19352744434064,24.8741077892075,12.));
#207987=CARTESIAN_POINT('Ctrl Pts',(1.2030531842602,24.8508544481974,0.));
#207988=CARTESIAN_POINT('Ctrl Pts',(1.2030531842602,24.8508544481974,12.));
#207989=CARTESIAN_POINT('Ctrl Pts',(1.21249266318208,24.8276539035092,0.));
#207990=CARTESIAN_POINT('Ctrl Pts',(1.21249266318208,24.8276539035092,12.));
#207991=CARTESIAN_POINT('Ctrl Pts',(1.22184594406528,24.8045067380536,0.));
#207992=CARTESIAN_POINT('Ctrl Pts',(1.22184594406528,24.8045067380536,12.));
#207993=CARTESIAN_POINT('Ctrl Pts',(1.23111309161843,24.7814135391799,0.));
#207994=CARTESIAN_POINT('Ctrl Pts',(1.23111309161843,24.7814135391799,12.));
#207995=CARTESIAN_POINT('Ctrl Pts',(1.24029417231989,24.7583748985438,0.));
#207996=CARTESIAN_POINT('Ctrl Pts',(1.24029417231989,24.7583748985438,12.));
#207997=CARTESIAN_POINT('Ctrl Pts',(1.24938925444325,24.7353914120011,0.));
#207998=CARTESIAN_POINT('Ctrl Pts',(1.24938925444325,24.7353914120011,12.));
#207999=CARTESIAN_POINT('Ctrl Pts',(1.25839840807418,24.7124636797894,0.));
#208000=CARTESIAN_POINT('Ctrl Pts',(1.25839840807418,24.7124636797894,12.));
#208001=CARTESIAN_POINT('Ctrl Pts',(1.267321705135,24.6895923066836,0.));
#208002=CARTESIAN_POINT('Ctrl Pts',(1.267321705135,24.6895923066836,12.));
#208003=CARTESIAN_POINT('Ctrl Pts',(1.27615921941642,24.666777902156,0.));
#208004=CARTESIAN_POINT('Ctrl Pts',(1.27615921941642,24.666777902156,12.));
#208005=CARTESIAN_POINT('Ctrl Pts',(1.28491102661514,24.6440210805278,0.));
#208006=CARTESIAN_POINT('Ctrl Pts',(1.28491102661514,24.6440210805278,12.));
#208007=CARTESIAN_POINT('Ctrl Pts',(1.29357720438107,24.6213224611229,0.));
#208008=CARTESIAN_POINT('Ctrl Pts',(1.29357720438107,24.6213224611229,12.));
#208009=CARTESIAN_POINT('Ctrl Pts',(1.30215783236362,24.5986826684027,0.));
#208010=CARTESIAN_POINT('Ctrl Pts',(1.30215783236362,24.5986826684027,12.));
#208011=CARTESIAN_POINT('Ctrl Pts',(1.31065299222021,24.5761023320183,0.));
#208012=CARTESIAN_POINT('Ctrl Pts',(1.31065299222021,24.5761023320183,12.));
#208013=CARTESIAN_POINT('Ctrl Pts',(1.31906276763668,24.5535820868674,0.));
#208014=CARTESIAN_POINT('Ctrl Pts',(1.31906276763668,24.5535820868674,12.));
#208015=CARTESIAN_POINT('Ctrl Pts',(1.32738724435326,24.5311225731435,0.));
#208016=CARTESIAN_POINT('Ctrl Pts',(1.32738724435326,24.5311225731435,12.));
#208017=CARTESIAN_POINT('Ctrl Pts',(1.33562651019686,24.5087244363856,0.));
#208018=CARTESIAN_POINT('Ctrl Pts',(1.33562651019686,24.5087244363856,12.));
#208019=CARTESIAN_POINT('Ctrl Pts',(1.34378065512337,24.4863883275134,0.));
#208020=CARTESIAN_POINT('Ctrl Pts',(1.34378065512337,24.4863883275134,12.));
#208021=CARTESIAN_POINT('Ctrl Pts',(1.35184977125648,24.4641149028892,0.));
#208022=CARTESIAN_POINT('Ctrl Pts',(1.35184977125648,24.4641149028892,12.));
#208023=CARTESIAN_POINT('Ctrl Pts',(1.35983395290627,24.4419048244523,0.));
#208024=CARTESIAN_POINT('Ctrl Pts',(1.35983395290627,24.4419048244523,12.));
#208025=CARTESIAN_POINT('Ctrl Pts',(1.36773329659956,24.4197587598337,0.));
#208026=CARTESIAN_POINT('Ctrl Pts',(1.36773329659956,24.4197587598337,12.));
#208027=CARTESIAN_POINT('Ctrl Pts',(1.37554790111609,24.3976773824732,0.));
#208028=CARTESIAN_POINT('Ctrl Pts',(1.37554790111609,24.3976773824732,12.));
#208029=CARTESIAN_POINT('Ctrl Pts',(1.38327786752998,24.3756613717299,0.));
#208030=CARTESIAN_POINT('Ctrl Pts',(1.38327786752998,24.3756613717299,12.));
#208031=CARTESIAN_POINT('Ctrl Pts',(1.39092329926388,24.3537114129875,0.));
#208032=CARTESIAN_POINT('Ctrl Pts',(1.39092329926388,24.3537114129875,12.));
#208033=CARTESIAN_POINT('Ctrl Pts',(1.39848430212807,24.3318281977643,0.));
#208034=CARTESIAN_POINT('Ctrl Pts',(1.39848430212807,24.3318281977643,12.));
#208035=CARTESIAN_POINT('Ctrl Pts',(1.40596098434337,24.3100124238311,0.));
#208036=CARTESIAN_POINT('Ctrl Pts',(1.40596098434337,24.3100124238311,12.));
#208037=CARTESIAN_POINT('Ctrl Pts',(1.41335345657682,24.288264795321,0.));
#208038=CARTESIAN_POINT('Ctrl Pts',(1.41335345657682,24.288264795321,12.));
#208039=CARTESIAN_POINT('Ctrl Pts',(1.42066183198252,24.2665860228356,0.));
#208040=CARTESIAN_POINT('Ctrl Pts',(1.42066183198252,24.2665860228356,12.));
#208041=CARTESIAN_POINT('Ctrl Pts',(1.42788622624854,24.2449768235488,0.));
#208042=CARTESIAN_POINT('Ctrl Pts',(1.42788622624854,24.2449768235488,12.));
#208043=CARTESIAN_POINT('Ctrl Pts',(1.43502675765508,24.2234379212984,0.));
#208044=CARTESIAN_POINT('Ctrl Pts',(1.43502675765508,24.2234379212984,12.));
#208045=CARTESIAN_POINT('Ctrl Pts',(1.44208354711082,24.201970046722,0.));
#208046=CARTESIAN_POINT('Ctrl Pts',(1.44208354711082,24.201970046722,12.));
#208047=CARTESIAN_POINT('Ctrl Pts',(1.44905671818727,24.1805739374038,0.));
#208048=CARTESIAN_POINT('Ctrl Pts',(1.44905671818727,24.1805739374038,12.));
#208049=CARTESIAN_POINT('Ctrl Pts',(1.45594639716317,24.1592503380107,0.));
#208050=CARTESIAN_POINT('Ctrl Pts',(1.45594639716317,24.1592503380107,12.));
#208051=CARTESIAN_POINT('Ctrl Pts',(1.46275271307397,24.1380000004272,0.));
#208052=CARTESIAN_POINT('Ctrl Pts',(1.46275271307397,24.1380000004272,12.));
#208053=CARTESIAN_POINT('Ctrl Pts',(1.46947579776991,24.1168236838824,0.));
#208054=CARTESIAN_POINT('Ctrl Pts',(1.46947579776991,24.1168236838824,12.));
#208055=CARTESIAN_POINT('Ctrl Pts',(1.47611578597742,24.0957221550778,0.));
#208056=CARTESIAN_POINT('Ctrl Pts',(1.47611578597742,24.0957221550778,12.));
#208057=CARTESIAN_POINT('Ctrl Pts',(1.48267281533683,24.0746961883528,0.));
#208058=CARTESIAN_POINT('Ctrl Pts',(1.48267281533683,24.0746961883528,12.));
#208059=CARTESIAN_POINT('Ctrl Pts',(1.48914702644887,24.0537465658429,0.));
#208060=CARTESIAN_POINT('Ctrl Pts',(1.48914702644887,24.0537465658429,12.));
#208061=CARTESIAN_POINT('Ctrl Pts',(1.49553856292801,24.0328740776331,0.));
#208062=CARTESIAN_POINT('Ctrl Pts',(1.49553856292801,24.0328740776331,12.));
#208063=CARTESIAN_POINT('Ctrl Pts',(1.50184757146098,24.0120795219086,0.));
#208064=CARTESIAN_POINT('Ctrl Pts',(1.50184757146098,24.0120795219086,12.));
#208065=CARTESIAN_POINT('Ctrl Pts',(1.50807420187694,23.9913637050927,0.));
#208066=CARTESIAN_POINT('Ctrl Pts',(1.50807420187694,23.9913637050927,12.));
#208067=CARTESIAN_POINT('Ctrl Pts',(1.51421860720614,23.970727442014,0.));
#208068=CARTESIAN_POINT('Ctrl Pts',(1.51421860720614,23.970727442014,12.));
#208069=CARTESIAN_POINT('Ctrl Pts',(1.52028094372792,23.9501715561033,0.));
#208070=CARTESIAN_POINT('Ctrl Pts',(1.52028094372792,23.9501715561033,12.));
#208071=CARTESIAN_POINT('Ctrl Pts',(1.52626137103032,23.9296968795757,0.));
#208072=CARTESIAN_POINT('Ctrl Pts',(1.52626137103032,23.9296968795757,12.));
#208073=CARTESIAN_POINT('Ctrl Pts',(1.53216005207463,23.9093042536119,0.));
#208074=CARTESIAN_POINT('Ctrl Pts',(1.53216005207463,23.9093042536119,12.));
#208075=CARTESIAN_POINT('Ctrl Pts',(1.53797715326758,23.8889945285318,0.));
#208076=CARTESIAN_POINT('Ctrl Pts',(1.53797715326758,23.8889945285318,12.));
#208077=CARTESIAN_POINT('Ctrl Pts',(1.5437128445399,23.8687685639642,0.));
#208078=CARTESIAN_POINT('Ctrl Pts',(1.5437128445399,23.8687685639642,12.));
#208079=CARTESIAN_POINT('Ctrl Pts',(1.54936729940541,23.8486272290705,0.));
#208080=CARTESIAN_POINT('Ctrl Pts',(1.54936729940541,23.8486272290705,12.));
#208081=CARTESIAN_POINT('Ctrl Pts',(1.55494069502635,23.8285714027636,0.));
#208082=CARTESIAN_POINT('Ctrl Pts',(1.55494069502635,23.8285714027636,12.));
#208083=CARTESIAN_POINT('Ctrl Pts',(1.56043321228633,23.8086019739194,0.));
#208084=CARTESIAN_POINT('Ctrl Pts',(1.56043321228633,23.8086019739194,12.));
#208085=CARTESIAN_POINT('Ctrl Pts',(1.56584503586843,23.7887198415878,0.));
#208086=CARTESIAN_POINT('Ctrl Pts',(1.56584503586843,23.7887198415878,12.));
#208087=CARTESIAN_POINT('Ctrl Pts',(1.57117635434408,23.7689259151862,0.));
#208088=CARTESIAN_POINT('Ctrl Pts',(1.57117635434408,23.7689259151862,12.));
#208089=CARTESIAN_POINT('Ctrl Pts',(1.57642736025246,23.749221114736,0.));
#208090=CARTESIAN_POINT('Ctrl Pts',(1.57642736025246,23.749221114736,12.));
#208091=CARTESIAN_POINT('Ctrl Pts',(1.58159825017358,23.72960637113,0.));
#208092=CARTESIAN_POINT('Ctrl Pts',(1.58159825017358,23.72960637113,12.));
#208093=CARTESIAN_POINT('Ctrl Pts',(1.58668922481221,23.710082626383,0.));
#208094=CARTESIAN_POINT('Ctrl Pts',(1.58668922481221,23.710082626383,12.));
#208095=CARTESIAN_POINT('Ctrl Pts',(1.59170048908633,23.6906508338833,0.));
#208096=CARTESIAN_POINT('Ctrl Pts',(1.59170048908633,23.6906508338833,12.));
#208097=CARTESIAN_POINT('Ctrl Pts',(1.59663225222463,23.671311958631,0.));
#208098=CARTESIAN_POINT('Ctrl Pts',(1.59663225222463,23.671311958631,12.));
#208099=CARTESIAN_POINT('Ctrl Pts',(1.60148472786595,23.6520669774876,0.));
#208100=CARTESIAN_POINT('Ctrl Pts',(1.60148472786595,23.6520669774876,12.));
#208101=CARTESIAN_POINT('Ctrl Pts',(1.60625813414672,23.6329168794929,0.));
#208102=CARTESIAN_POINT('Ctrl Pts',(1.60625813414672,23.6329168794929,12.));
#208103=CARTESIAN_POINT('Ctrl Pts',(1.61095269379778,23.6138626661653,0.));
#208104=CARTESIAN_POINT('Ctrl Pts',(1.61095269379778,23.6138626661653,12.));
#208105=CARTESIAN_POINT('Ctrl Pts',(1.61556863424698,23.5949053517997,0.));
#208106=CARTESIAN_POINT('Ctrl Pts',(1.61556863424698,23.5949053517997,12.));
#208107=CARTESIAN_POINT('Ctrl Pts',(1.62010618772866,23.57604596376,0.));
#208108=CARTESIAN_POINT('Ctrl Pts',(1.62010618772866,23.57604596376,12.));
#208109=CARTESIAN_POINT('Ctrl Pts',(1.62456559140064,23.5572855427601,0.));
#208110=CARTESIAN_POINT('Ctrl Pts',(1.62456559140064,23.5572855427601,12.));
#208111=CARTESIAN_POINT('Ctrl Pts',(1.62894708745223,23.538625143226,0.));
#208112=CARTESIAN_POINT('Ctrl Pts',(1.62894708745223,23.538625143226,12.));
#208113=CARTESIAN_POINT('Ctrl Pts',(1.63325092321725,23.5200658336612,0.));
#208114=CARTESIAN_POINT('Ctrl Pts',(1.63325092321725,23.5200658336612,12.));
#208115=CARTESIAN_POINT('Ctrl Pts',(1.63747735129474,23.5016086970003,0.));
#208116=CARTESIAN_POINT('Ctrl Pts',(1.63747735129474,23.5016086970003,12.));
#208117=CARTESIAN_POINT('Ctrl Pts',(1.64162662967528,23.4832548309645,0.));
#208118=CARTESIAN_POINT('Ctrl Pts',(1.64162662967528,23.4832548309645,12.));
#208119=CARTESIAN_POINT('Ctrl Pts',(1.64569902187611,23.4650053483932,0.));
#208120=CARTESIAN_POINT('Ctrl Pts',(1.64569902187611,23.4650053483932,12.));
#208121=CARTESIAN_POINT('Ctrl Pts',(1.6496947970734,23.4468613776574,0.));
#208122=CARTESIAN_POINT('Ctrl Pts',(1.6496947970734,23.4468613776574,12.));
#208123=CARTESIAN_POINT('Ctrl Pts',(1.65361423023728,23.4288240631043,0.));
#208124=CARTESIAN_POINT('Ctrl Pts',(1.65361423023728,23.4288240631043,12.));
#208125=CARTESIAN_POINT('Ctrl Pts',(1.65745760227505,23.4108945654805,0.));
#208126=CARTESIAN_POINT('Ctrl Pts',(1.65745760227505,23.4108945654805,12.));
#208127=CARTESIAN_POINT('Ctrl Pts',(1.66122520018011,23.3930740623619,0.));
#208128=CARTESIAN_POINT('Ctrl Pts',(1.66122520018011,23.3930740623619,12.));
#208129=CARTESIAN_POINT('Ctrl Pts',(1.66491731718876,23.3753637485545,0.));
#208130=CARTESIAN_POINT('Ctrl Pts',(1.66491731718876,23.3753637485545,12.));
#208131=CARTESIAN_POINT('Ctrl Pts',(1.66853425293995,23.3577648365744,0.));
#208132=CARTESIAN_POINT('Ctrl Pts',(1.66853425293995,23.3577648365744,12.));
#208133=CARTESIAN_POINT('Ctrl Pts',(1.67207631363921,23.3402785571865,0.));
#208134=CARTESIAN_POINT('Ctrl Pts',(1.67207631363921,23.3402785571865,12.));
#208135=CARTESIAN_POINT('Ctrl Pts',(1.67554381222994,23.3229061599145,0.));
#208136=CARTESIAN_POINT('Ctrl Pts',(1.67554381222994,23.3229061599145,12.));
#208137=CARTESIAN_POINT('Ctrl Pts',(1.67893706857117,23.3056489135611,0.));
#208138=CARTESIAN_POINT('Ctrl Pts',(1.67893706857117,23.3056489135611,12.));
#208139=CARTESIAN_POINT('Ctrl Pts',(1.68225640962168,23.2885081066951,0.));
#208140=CARTESIAN_POINT('Ctrl Pts',(1.68225640962168,23.2885081066951,12.));
#208141=CARTESIAN_POINT('Ctrl Pts',(1.68550216963258,23.2714850482246,0.));
#208142=CARTESIAN_POINT('Ctrl Pts',(1.68550216963258,23.2714850482246,12.));
#208143=CARTESIAN_POINT('Ctrl Pts',(1.68867469034896,23.2545810680537,0.));
#208144=CARTESIAN_POINT('Ctrl Pts',(1.68867469034896,23.2545810680537,12.));
#208145=CARTESIAN_POINT('Ctrl Pts',(1.69177432121711,23.2377975177013,0.));
#208146=CARTESIAN_POINT('Ctrl Pts',(1.69177432121711,23.2377975177013,12.));
#208147=CARTESIAN_POINT('Ctrl Pts',(1.69480141959953,23.2211357709374,0.));
#208148=CARTESIAN_POINT('Ctrl Pts',(1.69480141959953,23.2211357709374,12.));
#208149=CARTESIAN_POINT('Ctrl Pts',(1.69775635099443,23.2045972243767,0.));
#208150=CARTESIAN_POINT('Ctrl Pts',(1.69775635099443,23.2045972243767,12.));
#208151=CARTESIAN_POINT('Ctrl Pts',(1.7006394892701,23.1881832981851,0.));
#208152=CARTESIAN_POINT('Ctrl Pts',(1.7006394892701,23.1881832981851,12.));
#208153=CARTESIAN_POINT('Ctrl Pts',(1.70345121691276,23.1718954368751,0.));
#208154=CARTESIAN_POINT('Ctrl Pts',(1.70345121691276,23.1718954368751,12.));
#208155=CARTESIAN_POINT('Ctrl Pts',(1.70619192527852,23.1557351100614,0.));
#208156=CARTESIAN_POINT('Ctrl Pts',(1.70619192527852,23.1557351100614,12.));
#208157=CARTESIAN_POINT('Ctrl Pts',(1.70886201485452,23.1397038132356,0.));
#208158=CARTESIAN_POINT('Ctrl Pts',(1.70886201485452,23.1397038132356,12.));
#208159=CARTESIAN_POINT('Ctrl Pts',(1.71146189552174,23.1238030684925,0.));
#208160=CARTESIAN_POINT('Ctrl Pts',(1.71146189552174,23.1238030684925,12.));
#208161=CARTESIAN_POINT('Ctrl Pts',(1.71399198684704,23.1080344254286,0.));
#208162=CARTESIAN_POINT('Ctrl Pts',(1.71399198684704,23.1080344254286,12.));
#208163=CARTESIAN_POINT('Ctrl Pts',(1.71645271839296,23.0923994621213,0.));
#208164=CARTESIAN_POINT('Ctrl Pts',(1.71645271839296,23.0923994621213,12.));
#208165=CARTESIAN_POINT('Ctrl Pts',(1.71884453003027,23.0768997860709,0.));
#208166=CARTESIAN_POINT('Ctrl Pts',(1.71884453003027,23.0768997860709,12.));
#208167=CARTESIAN_POINT('Ctrl Pts',(1.72116787225991,23.0615370351562,0.));
#208168=CARTESIAN_POINT('Ctrl Pts',(1.72116787225991,23.0615370351562,12.));
#208169=CARTESIAN_POINT('Ctrl Pts',(1.72342320653746,23.0463128785531,0.));
#208170=CARTESIAN_POINT('Ctrl Pts',(1.72342320653746,23.0463128785531,12.));
#208171=CARTESIAN_POINT('Ctrl Pts',(1.72561100564045,23.0312290178883,0.));
#208172=CARTESIAN_POINT('Ctrl Pts',(1.72561100564045,23.0312290178883,12.));
#208173=CARTESIAN_POINT('Ctrl Pts',(1.72773175404708,23.0162871884168,0.));
#208174=CARTESIAN_POINT('Ctrl Pts',(1.72773175404708,23.0162871884168,12.));
#208175=CARTESIAN_POINT('Ctrl Pts',(1.72978594832136,23.001489160189,0.));
#208176=CARTESIAN_POINT('Ctrl Pts',(1.72978594832136,23.001489160189,12.));
#208177=CARTESIAN_POINT('Ctrl Pts',(1.7317740975019,22.9868367391978,0.));
#208178=CARTESIAN_POINT('Ctrl Pts',(1.7317740975019,22.9868367391978,12.));
#208179=CARTESIAN_POINT('Ctrl Pts',(1.73369672350814,22.9723317685688,0.));
#208180=CARTESIAN_POINT('Ctrl Pts',(1.73369672350814,22.9723317685688,12.));
#208181=CARTESIAN_POINT('Ctrl Pts',(1.73555436162769,22.9579761301063,0.));
#208182=CARTESIAN_POINT('Ctrl Pts',(1.73555436162769,22.9579761301063,12.));
#208183=CARTESIAN_POINT('Ctrl Pts',(1.73734756100039,22.9437717457826,0.));
#208184=CARTESIAN_POINT('Ctrl Pts',(1.73734756100039,22.9437717457826,12.));
#208185=CARTESIAN_POINT('Ctrl Pts',(1.73907688511666,22.9297205792586,0.));
#208186=CARTESIAN_POINT('Ctrl Pts',(1.73907688511666,22.9297205792586,12.));
#208187=CARTESIAN_POINT('Ctrl Pts',(1.74074291231058,22.9158246373363,0.));
#208188=CARTESIAN_POINT('Ctrl Pts',(1.74074291231058,22.9158246373363,12.));
#208189=CARTESIAN_POINT('Ctrl Pts',(1.7423462363008,22.9020859716141,0.));
#208190=CARTESIAN_POINT('Ctrl Pts',(1.7423462363008,22.9020859716141,12.));
#208191=CARTESIAN_POINT('Ctrl Pts',(1.74388746677702,22.888506680335,0.));
#208192=CARTESIAN_POINT('Ctrl Pts',(1.74388746677702,22.888506680335,12.));
#208193=CARTESIAN_POINT('Ctrl Pts',(1.74536722998201,22.8750889101696,0.));
#208194=CARTESIAN_POINT('Ctrl Pts',(1.74536722998201,22.8750889101696,12.));
#208195=CARTESIAN_POINT('Ctrl Pts',(1.74678616930664,22.8618348580235,0.));
#208196=CARTESIAN_POINT('Ctrl Pts',(1.74678616930664,22.8618348580235,12.));
#208197=CARTESIAN_POINT('Ctrl Pts',(1.74814494588492,22.8487467728076,0.));
#208198=CARTESIAN_POINT('Ctrl Pts',(1.74814494588492,22.8487467728076,12.));
#208199=CARTESIAN_POINT('Ctrl Pts',(1.74944423940115,22.8358269579853,0.));
#208200=CARTESIAN_POINT('Ctrl Pts',(1.74944423940115,22.8358269579853,12.));
#208201=CARTESIAN_POINT('Ctrl Pts',(1.75068474890883,22.8230777741284,0.));
#208202=CARTESIAN_POINT('Ctrl Pts',(1.75068474890883,22.8230777741284,12.));
#208203=CARTESIAN_POINT('Ctrl Pts',(1.75186719365592,22.8105016414713,0.));
#208204=CARTESIAN_POINT('Ctrl Pts',(1.75186719365592,22.8105016414713,12.));
#208205=CARTESIAN_POINT('Ctrl Pts',(1.75299231391466,22.7981010424314,0.));
#208206=CARTESIAN_POINT('Ctrl Pts',(1.75299231391466,22.7981010424314,12.));
#208207=CARTESIAN_POINT('Ctrl Pts',(1.75406087182936,22.7858785242361,0.));
#208208=CARTESIAN_POINT('Ctrl Pts',(1.75406087182936,22.7858785242361,12.));
#208209=CARTESIAN_POINT('Ctrl Pts',(1.75507365227131,22.7738367016118,0.));
#208210=CARTESIAN_POINT('Ctrl Pts',(1.75507365227131,22.7738367016118,12.));
#208211=CARTESIAN_POINT('Ctrl Pts',(1.75603146371641,22.7619782595013,0.));
#208212=CARTESIAN_POINT('Ctrl Pts',(1.75603146371641,22.7619782595013,12.));
#208213=CARTESIAN_POINT('Ctrl Pts',(1.75693513908907,22.750305955645,0.));
#208214=CARTESIAN_POINT('Ctrl Pts',(1.75693513908907,22.750305955645,12.));
#208215=CARTESIAN_POINT('Ctrl Pts',(1.75778553673244,22.7388226235559,0.));
#208216=CARTESIAN_POINT('Ctrl Pts',(1.75778553673244,22.7388226235559,12.));
#208217=CARTESIAN_POINT('Ctrl Pts',(1.75858354204633,22.72753117773,0.));
#208218=CARTESIAN_POINT('Ctrl Pts',(1.75858354204633,22.72753117773,12.));
#208219=CARTESIAN_POINT('Ctrl Pts',(1.75933006905925,22.7164346186006,0.));
#208220=CARTESIAN_POINT('Ctrl Pts',(1.75933006905925,22.7164346186006,12.));
#208221=CARTESIAN_POINT('Ctrl Pts',(1.76002606202401,22.7055360375485,0.));
#208222=CARTESIAN_POINT('Ctrl Pts',(1.76002606202401,22.7055360375485,12.));
#208223=CARTESIAN_POINT('Ctrl Pts',(1.76067249704886,22.6948386219851,0.));
#208224=CARTESIAN_POINT('Ctrl Pts',(1.76067249704886,22.6948386219851,12.));
#208225=CARTESIAN_POINT('Ctrl Pts',(1.76127038310614,22.684345658525,0.));
#208226=CARTESIAN_POINT('Ctrl Pts',(1.76127038310614,22.684345658525,12.));
#208227=CARTESIAN_POINT('Ctrl Pts',(1.76182076289525,22.67406053567,0.));
#208228=CARTESIAN_POINT('Ctrl Pts',(1.76182076289525,22.67406053567,12.));
#208229=CARTESIAN_POINT('Ctrl Pts',(1.76232471392568,22.6639867471753,0.));
#208230=CARTESIAN_POINT('Ctrl Pts',(1.76232471392568,22.6639867471753,12.));
#208231=CARTESIAN_POINT('Ctrl Pts',(1.76278334912561,22.6541278938409,0.));
#208232=CARTESIAN_POINT('Ctrl Pts',(1.76278334912561,22.6541278938409,12.));
#208233=CARTESIAN_POINT('Ctrl Pts',(1.76319782013916,22.6444876940423,0.));
#208234=CARTESIAN_POINT('Ctrl Pts',(1.76319782013916,22.6444876940423,12.));
#208235=CARTESIAN_POINT('Ctrl Pts',(1.76356932176273,22.6350699979359,0.));
#208236=CARTESIAN_POINT('Ctrl Pts',(1.76356932176273,22.6350699979359,12.));
#208237=CARTESIAN_POINT('Ctrl Pts',(1.76389909571403,22.6258787994848,0.));
#208238=CARTESIAN_POINT('Ctrl Pts',(1.76389909571403,22.6258787994848,12.));
#208239=CARTESIAN_POINT('Ctrl Pts',(1.76418843543739,22.6169182517694,0.));
#208240=CARTESIAN_POINT('Ctrl Pts',(1.76418843543739,22.6169182517694,12.));
#208241=CARTESIAN_POINT('Ctrl Pts',(1.76443868648015,22.6081926681343,0.));
#208242=CARTESIAN_POINT('Ctrl Pts',(1.76443868648015,22.6081926681343,12.));
#208243=CARTESIAN_POINT('Ctrl Pts',(1.76465124413557,22.5997065145638,0.));
#208244=CARTESIAN_POINT('Ctrl Pts',(1.76465124413557,22.5997065145638,12.));
#208245=CARTESIAN_POINT('Ctrl Pts',(1.76482755288411,22.5914644078106,0.));
#208246=CARTESIAN_POINT('Ctrl Pts',(1.76482755288411,22.5914644078106,12.));
#208247=CARTESIAN_POINT('Ctrl Pts',(1.76496910283088,22.5834711038022,0.));
#208248=CARTESIAN_POINT('Ctrl Pts',(1.76496910283088,22.5834711038022,12.));
#208249=CARTESIAN_POINT('Ctrl Pts',(1.76507744026746,22.5757315316353,0.));
#208250=CARTESIAN_POINT('Ctrl Pts',(1.76507744026746,22.5757315316353,12.));
#208251=CARTESIAN_POINT('Ctrl Pts',(1.76515418518831,22.5682508499873,0.));
#208252=CARTESIAN_POINT('Ctrl Pts',(1.76515418518831,22.5682508499873,12.));
#208253=CARTESIAN_POINT('Ctrl Pts',(1.7652010450045,22.5610344912501,0.));
#208254=CARTESIAN_POINT('Ctrl Pts',(1.7652010450045,22.5610344912501,12.));
#208255=CARTESIAN_POINT('Ctrl Pts',(1.76521983384062,22.5540882235837,0.));
#208256=CARTESIAN_POINT('Ctrl Pts',(1.76521983384062,22.5540882235837,12.));
#208257=CARTESIAN_POINT('Ctrl Pts',(1.76521245524047,22.5474180954006,0.));
#208258=CARTESIAN_POINT('Ctrl Pts',(1.76521245524047,22.5474180954006,12.));
#208259=CARTESIAN_POINT('Ctrl Pts',(1.76518087841493,22.5410303590892,0.));
#208260=CARTESIAN_POINT('Ctrl Pts',(1.76518087841493,22.5410303590892,12.));
#208261=CARTESIAN_POINT('Ctrl Pts',(1.76512711563254,22.5349313983571,0.));
#208262=CARTESIAN_POINT('Ctrl Pts',(1.76512711563254,22.5349313983571,12.));
#208263=CARTESIAN_POINT('Ctrl Pts',(1.76505320262759,22.529127665298,0.));
#208264=CARTESIAN_POINT('Ctrl Pts',(1.76505320262759,22.529127665298,12.));
#208265=CARTESIAN_POINT('Ctrl Pts',(1.76496128643375,22.5236259635515,0.));
#208266=CARTESIAN_POINT('Ctrl Pts',(1.76496128643375,22.5236259635515,12.));
#208267=CARTESIAN_POINT('Ctrl Pts',(1.76485369319895,22.5184336670207,0.));
#208268=CARTESIAN_POINT('Ctrl Pts',(1.76485369319895,22.5184336670207,12.));
#208269=CARTESIAN_POINT('Ctrl Pts',(1.76473303281149,22.5135590569554,0.));
#208270=CARTESIAN_POINT('Ctrl Pts',(1.76473303281149,22.5135590569554,12.));
#208271=CARTESIAN_POINT('Ctrl Pts',(1.76460218257313,22.5090112700212,0.));
#208272=CARTESIAN_POINT('Ctrl Pts',(1.76460218257313,22.5090112700212,12.));
#208273=CARTESIAN_POINT('Ctrl Pts',(1.76446408210364,22.5047996391978,0.));
#208274=CARTESIAN_POINT('Ctrl Pts',(1.76446408210364,22.5047996391978,12.));
#208275=CARTESIAN_POINT('Ctrl Pts',(1.76432160068737,22.5009332677316,0.));
#208276=CARTESIAN_POINT('Ctrl Pts',(1.76432160068737,22.5009332677316,12.));
#208277=CARTESIAN_POINT('Ctrl Pts',(1.76417731243483,22.4974203063191,0.));
#208278=CARTESIAN_POINT('Ctrl Pts',(1.76417731243483,22.4974203063191,12.));
#208279=CARTESIAN_POINT('Ctrl Pts',(1.76403393880316,22.4942693792449,0.));
#208280=CARTESIAN_POINT('Ctrl Pts',(1.76403393880316,22.4942693792449,12.));
#208281=CARTESIAN_POINT('Ctrl Pts',(1.76389475965714,22.4914909094908,0.));
#208282=CARTESIAN_POINT('Ctrl Pts',(1.76389475965714,22.4914909094908,12.));
#208283=CARTESIAN_POINT('Ctrl Pts',(1.76376424879468,22.4890991659479,0.));
#208284=CARTESIAN_POINT('Ctrl Pts',(1.76376424879468,22.4890991659479,12.));
#208285=CARTESIAN_POINT('Ctrl Pts',(1.76364784232925,22.4871115206572,0.));
#208286=CARTESIAN_POINT('Ctrl Pts',(1.76364784232925,22.4871115206572,12.));
#208287=CARTESIAN_POINT('Ctrl Pts',(1.76355076045549,22.4855446605991,0.));
#208288=CARTESIAN_POINT('Ctrl Pts',(1.76355076045549,22.4855446605991,12.));
#208289=CARTESIAN_POINT('Ctrl Pts',(1.76347698284861,22.4844112933125,0.));
#208290=CARTESIAN_POINT('Ctrl Pts',(1.76347698284861,22.4844112933125,12.));
#208291=CARTESIAN_POINT('Ctrl Pts',(1.76343813434659,22.4838562517064,0.));
#208292=CARTESIAN_POINT('Ctrl Pts',(1.76343813434659,22.4838562517064,12.));
#208293=CARTESIAN_POINT('Ctrl Pts',(1.76342064263637,22.4836387052228,0.));
#208294=CARTESIAN_POINT('Ctrl Pts',(1.76342064263637,22.4836387052228,12.));
#208295=CARTESIAN_POINT('Ctrl Pts',(1.7634141553879,22.4835819929788,0.));
#208296=CARTESIAN_POINT('Ctrl Pts',(1.7634141553879,22.4835819929788,12.));
#208297=CARTESIAN_POINT('Ctrl Pts',(1.7634122053118,22.4835757167854,0.));
#208298=CARTESIAN_POINT('Ctrl Pts',(1.7634122053118,22.4835757167854,12.));
#208299=CARTESIAN_POINT('',(0.661312440730901,25.991588367311,0.));
#208300=CARTESIAN_POINT('Ctrl Pts',(0.661312440730901,25.991588367311,0.));
#208301=CARTESIAN_POINT('Ctrl Pts',(0.664028313187627,25.9865613464773,
0.));
#208302=CARTESIAN_POINT('Ctrl Pts',(0.669451306780825,25.9765104298071,
0.));
#208303=CARTESIAN_POINT('Ctrl Pts',(0.677559543209725,25.9614434297919,
0.));
#208304=CARTESIAN_POINT('Ctrl Pts',(0.688318015057729,25.9413728471909,
0.));
#208305=CARTESIAN_POINT('Ctrl Pts',(0.701678575228756,25.9163158909426,
0.));
#208306=CARTESIAN_POINT('Ctrl Pts',(0.714951588527638,25.891290261497,0.));
#208307=CARTESIAN_POINT('Ctrl Pts',(0.728137036482335,25.8662960624185,
0.));
#208308=CARTESIAN_POINT('Ctrl Pts',(0.741234902663807,25.8413334619055,
0.));
#208309=CARTESIAN_POINT('Ctrl Pts',(0.754245175609524,25.8164027059984,
0.));
#208310=CARTESIAN_POINT('Ctrl Pts',(0.767167852651168,25.7915041383376,
0.));
#208311=CARTESIAN_POINT('Ctrl Pts',(0.780002940291965,25.7666381946955,
0.));
#208312=CARTESIAN_POINT('Ctrl Pts',(0.792750451616127,25.7418053757746,
0.));
#208313=CARTESIAN_POINT('Ctrl Pts',(0.805410404554352,25.7170062262525,
0.));
#208314=CARTESIAN_POINT('Ctrl Pts',(0.817982819787464,25.6922413110194,
0.));
#208315=CARTESIAN_POINT('Ctrl Pts',(0.830467718864205,25.6675111931952,
0.));
#208316=CARTESIAN_POINT('Ctrl Pts',(0.842865122120758,25.6428164100055,
0.));
#208317=CARTESIAN_POINT('Ctrl Pts',(0.855175047036549,25.6181574536049,
0.));
#208318=CARTESIAN_POINT('Ctrl Pts',(0.867397509338431,25.5935347843585,
0.));
#208319=CARTESIAN_POINT('Ctrl Pts',(0.879532523834294,25.5689488408156,
0.));
#208320=CARTESIAN_POINT('Ctrl Pts',(0.89158010534904,25.5444000508211,0.));
#208321=CARTESIAN_POINT('Ctrl Pts',(0.903540269651106,25.5198888424194,
0.));
#208322=CARTESIAN_POINT('Ctrl Pts',(0.915413034335613,25.4954156541795,
0.));
#208323=CARTESIAN_POINT('Ctrl Pts',(0.927198419886094,25.4709809475009,
0.));
#208324=CARTESIAN_POINT('Ctrl Pts',(0.938896449496192,25.4465852044849,
0.));
#208325=CARTESIAN_POINT('Ctrl Pts',(0.950507148597468,25.4222289223167,
0.));
#208326=CARTESIAN_POINT('Ctrl Pts',(0.962030544503142,25.3979126089163,
0.));
#208327=CARTESIAN_POINT('Ctrl Pts',(0.973466666000163,25.3736367778845,
0.));
#208328=CARTESIAN_POINT('Ctrl Pts',(0.984815543003973,25.3494019441441,
0.));
#208329=CARTESIAN_POINT('Ctrl Pts',(0.996077206120624,25.3252086182968,
0.));
#208330=CARTESIAN_POINT('Ctrl Pts',(1.00725168656896,25.3010573055547,0.));
#208331=CARTESIAN_POINT('Ctrl Pts',(1.01833901642237,25.276948508726,0.));
#208332=CARTESIAN_POINT('Ctrl Pts',(1.02933922876806,25.2528827300422,0.));
#208333=CARTESIAN_POINT('Ctrl Pts',(1.04025235791507,25.2288604735086,0.));
#208334=CARTESIAN_POINT('Ctrl Pts',(1.05107843957931,25.2048822469028,0.));
#208335=CARTESIAN_POINT('Ctrl Pts',(1.06181751111768,25.1809485642192,0.));
#208336=CARTESIAN_POINT('Ctrl Pts',(1.07246961165475,25.157059946931,0.));
#208337=CARTESIAN_POINT('Ctrl Pts',(1.08303478197187,25.1332169227413,0.));
#208338=CARTESIAN_POINT('Ctrl Pts',(1.09351306445308,25.1094200248446,0.));
#208339=CARTESIAN_POINT('Ctrl Pts',(1.10390450301745,25.0856697909679,0.));
#208340=CARTESIAN_POINT('Ctrl Pts',(1.11420914306889,25.0619667625336,0.));
#208341=CARTESIAN_POINT('Ctrl Pts',(1.12442703144451,25.0383114836899,0.));
#208342=CARTESIAN_POINT('Ctrl Pts',(1.1345582163853,25.0147045006196,0.));
#208343=CARTESIAN_POINT('Ctrl Pts',(1.144602747582,24.9911463621433,0.));
#208344=CARTESIAN_POINT('Ctrl Pts',(1.15456067621889,24.9676376201502,0.));
#208345=CARTESIAN_POINT('Ctrl Pts',(1.16443205502849,24.9441788300932,0.));
#208346=CARTESIAN_POINT('Ctrl Pts',(1.17421693835041,24.9207705514449,0.));
#208347=CARTESIAN_POINT('Ctrl Pts',(1.18391538220103,24.8974133481829,0.));
#208348=CARTESIAN_POINT('Ctrl Pts',(1.19352744434064,24.8741077892075,0.));
#208349=CARTESIAN_POINT('Ctrl Pts',(1.2030531842602,24.8508544481974,0.));
#208350=CARTESIAN_POINT('Ctrl Pts',(1.21249266318208,24.8276539035092,0.));
#208351=CARTESIAN_POINT('Ctrl Pts',(1.22184594406528,24.8045067380536,0.));
#208352=CARTESIAN_POINT('Ctrl Pts',(1.23111309161843,24.7814135391799,0.));
#208353=CARTESIAN_POINT('Ctrl Pts',(1.24029417231989,24.7583748985438,0.));
#208354=CARTESIAN_POINT('Ctrl Pts',(1.24938925444325,24.7353914120011,0.));
#208355=CARTESIAN_POINT('Ctrl Pts',(1.25839840807418,24.7124636797894,0.));
#208356=CARTESIAN_POINT('Ctrl Pts',(1.267321705135,24.6895923066836,0.));
#208357=CARTESIAN_POINT('Ctrl Pts',(1.27615921941642,24.666777902156,0.));
#208358=CARTESIAN_POINT('Ctrl Pts',(1.28491102661514,24.6440210805278,0.));
#208359=CARTESIAN_POINT('Ctrl Pts',(1.29357720438107,24.6213224611229,0.));
#208360=CARTESIAN_POINT('Ctrl Pts',(1.30215783236362,24.5986826684027,0.));
#208361=CARTESIAN_POINT('Ctrl Pts',(1.31065299222021,24.5761023320183,0.));
#208362=CARTESIAN_POINT('Ctrl Pts',(1.31906276763668,24.5535820868674,0.));
#208363=CARTESIAN_POINT('Ctrl Pts',(1.32738724435326,24.5311225731435,0.));
#208364=CARTESIAN_POINT('Ctrl Pts',(1.33562651019686,24.5087244363856,0.));
#208365=CARTESIAN_POINT('Ctrl Pts',(1.34378065512337,24.4863883275134,0.));
#208366=CARTESIAN_POINT('Ctrl Pts',(1.35184977125648,24.4641149028892,0.));
#208367=CARTESIAN_POINT('Ctrl Pts',(1.35983395290627,24.4419048244523,0.));
#208368=CARTESIAN_POINT('Ctrl Pts',(1.36773329659956,24.4197587598337,0.));
#208369=CARTESIAN_POINT('Ctrl Pts',(1.37554790111609,24.3976773824732,0.));
#208370=CARTESIAN_POINT('Ctrl Pts',(1.38327786752998,24.3756613717299,0.));
#208371=CARTESIAN_POINT('Ctrl Pts',(1.39092329926388,24.3537114129875,0.));
#208372=CARTESIAN_POINT('Ctrl Pts',(1.39848430212807,24.3318281977643,0.));
#208373=CARTESIAN_POINT('Ctrl Pts',(1.40596098434337,24.3100124238311,0.));
#208374=CARTESIAN_POINT('Ctrl Pts',(1.41335345657682,24.288264795321,0.));
#208375=CARTESIAN_POINT('Ctrl Pts',(1.42066183198252,24.2665860228356,0.));
#208376=CARTESIAN_POINT('Ctrl Pts',(1.42788622624854,24.2449768235488,0.));
#208377=CARTESIAN_POINT('Ctrl Pts',(1.43502675765508,24.2234379212984,0.));
#208378=CARTESIAN_POINT('Ctrl Pts',(1.44208354711082,24.201970046722,0.));
#208379=CARTESIAN_POINT('Ctrl Pts',(1.44905671818727,24.1805739374038,0.));
#208380=CARTESIAN_POINT('Ctrl Pts',(1.45594639716317,24.1592503380107,0.));
#208381=CARTESIAN_POINT('Ctrl Pts',(1.46275271307397,24.1380000004272,0.));
#208382=CARTESIAN_POINT('Ctrl Pts',(1.46947579776991,24.1168236838824,0.));
#208383=CARTESIAN_POINT('Ctrl Pts',(1.47611578597742,24.0957221550778,0.));
#208384=CARTESIAN_POINT('Ctrl Pts',(1.48267281533683,24.0746961883528,0.));
#208385=CARTESIAN_POINT('Ctrl Pts',(1.48914702644887,24.0537465658429,0.));
#208386=CARTESIAN_POINT('Ctrl Pts',(1.49553856292801,24.0328740776331,0.));
#208387=CARTESIAN_POINT('Ctrl Pts',(1.50184757146098,24.0120795219086,0.));
#208388=CARTESIAN_POINT('Ctrl Pts',(1.50807420187694,23.9913637050927,0.));
#208389=CARTESIAN_POINT('Ctrl Pts',(1.51421860720614,23.970727442014,0.));
#208390=CARTESIAN_POINT('Ctrl Pts',(1.52028094372792,23.9501715561033,0.));
#208391=CARTESIAN_POINT('Ctrl Pts',(1.52626137103032,23.9296968795757,0.));
#208392=CARTESIAN_POINT('Ctrl Pts',(1.53216005207463,23.9093042536119,0.));
#208393=CARTESIAN_POINT('Ctrl Pts',(1.53797715326758,23.8889945285318,0.));
#208394=CARTESIAN_POINT('Ctrl Pts',(1.5437128445399,23.8687685639642,0.));
#208395=CARTESIAN_POINT('Ctrl Pts',(1.54936729940541,23.8486272290705,0.));
#208396=CARTESIAN_POINT('Ctrl Pts',(1.55494069502635,23.8285714027636,0.));
#208397=CARTESIAN_POINT('Ctrl Pts',(1.56043321228633,23.8086019739194,0.));
#208398=CARTESIAN_POINT('Ctrl Pts',(1.56584503586843,23.7887198415878,0.));
#208399=CARTESIAN_POINT('Ctrl Pts',(1.57117635434408,23.7689259151862,0.));
#208400=CARTESIAN_POINT('Ctrl Pts',(1.57642736025246,23.749221114736,0.));
#208401=CARTESIAN_POINT('Ctrl Pts',(1.58159825017358,23.72960637113,0.));
#208402=CARTESIAN_POINT('Ctrl Pts',(1.58668922481221,23.710082626383,0.));
#208403=CARTESIAN_POINT('Ctrl Pts',(1.59170048908633,23.6906508338833,0.));
#208404=CARTESIAN_POINT('Ctrl Pts',(1.59663225222463,23.671311958631,0.));
#208405=CARTESIAN_POINT('Ctrl Pts',(1.60148472786595,23.6520669774876,0.));
#208406=CARTESIAN_POINT('Ctrl Pts',(1.60625813414672,23.6329168794929,0.));
#208407=CARTESIAN_POINT('Ctrl Pts',(1.61095269379778,23.6138626661653,0.));
#208408=CARTESIAN_POINT('Ctrl Pts',(1.61556863424698,23.5949053517997,0.));
#208409=CARTESIAN_POINT('Ctrl Pts',(1.62010618772866,23.57604596376,0.));
#208410=CARTESIAN_POINT('Ctrl Pts',(1.62456559140064,23.5572855427601,0.));
#208411=CARTESIAN_POINT('Ctrl Pts',(1.62894708745223,23.538625143226,0.));
#208412=CARTESIAN_POINT('Ctrl Pts',(1.63325092321725,23.5200658336612,0.));
#208413=CARTESIAN_POINT('Ctrl Pts',(1.63747735129474,23.5016086970003,0.));
#208414=CARTESIAN_POINT('Ctrl Pts',(1.64162662967528,23.4832548309645,0.));
#208415=CARTESIAN_POINT('Ctrl Pts',(1.64569902187611,23.4650053483932,0.));
#208416=CARTESIAN_POINT('Ctrl Pts',(1.6496947970734,23.4468613776574,0.));
#208417=CARTESIAN_POINT('Ctrl Pts',(1.65361423023728,23.4288240631043,0.));
#208418=CARTESIAN_POINT('Ctrl Pts',(1.65745760227505,23.4108945654805,0.));
#208419=CARTESIAN_POINT('Ctrl Pts',(1.66122520018011,23.3930740623619,0.));
#208420=CARTESIAN_POINT('Ctrl Pts',(1.66491731718876,23.3753637485545,0.));
#208421=CARTESIAN_POINT('Ctrl Pts',(1.66853425293995,23.3577648365744,0.));
#208422=CARTESIAN_POINT('Ctrl Pts',(1.67207631363921,23.3402785571865,0.));
#208423=CARTESIAN_POINT('Ctrl Pts',(1.67554381222994,23.3229061599145,0.));
#208424=CARTESIAN_POINT('Ctrl Pts',(1.67893706857117,23.3056489135611,0.));
#208425=CARTESIAN_POINT('Ctrl Pts',(1.68225640962168,23.2885081066951,0.));
#208426=CARTESIAN_POINT('Ctrl Pts',(1.68550216963258,23.2714850482246,0.));
#208427=CARTESIAN_POINT('Ctrl Pts',(1.68867469034896,23.2545810680537,0.));
#208428=CARTESIAN_POINT('Ctrl Pts',(1.69177432121711,23.2377975177013,0.));
#208429=CARTESIAN_POINT('Ctrl Pts',(1.69480141959953,23.2211357709374,0.));
#208430=CARTESIAN_POINT('Ctrl Pts',(1.69775635099443,23.2045972243767,0.));
#208431=CARTESIAN_POINT('Ctrl Pts',(1.7006394892701,23.1881832981851,0.));
#208432=CARTESIAN_POINT('Ctrl Pts',(1.70345121691276,23.1718954368751,0.));
#208433=CARTESIAN_POINT('Ctrl Pts',(1.70619192527852,23.1557351100614,0.));
#208434=CARTESIAN_POINT('Ctrl Pts',(1.70886201485452,23.1397038132356,0.));
#208435=CARTESIAN_POINT('Ctrl Pts',(1.71146189552174,23.1238030684925,0.));
#208436=CARTESIAN_POINT('Ctrl Pts',(1.71399198684704,23.1080344254286,0.));
#208437=CARTESIAN_POINT('Ctrl Pts',(1.71645271839296,23.0923994621213,0.));
#208438=CARTESIAN_POINT('Ctrl Pts',(1.71884453003027,23.0768997860709,0.));
#208439=CARTESIAN_POINT('Ctrl Pts',(1.72116787225991,23.0615370351562,0.));
#208440=CARTESIAN_POINT('Ctrl Pts',(1.72342320653746,23.0463128785531,0.));
#208441=CARTESIAN_POINT('Ctrl Pts',(1.72561100564045,23.0312290178883,0.));
#208442=CARTESIAN_POINT('Ctrl Pts',(1.72773175404708,23.0162871884168,0.));
#208443=CARTESIAN_POINT('Ctrl Pts',(1.72978594832136,23.001489160189,0.));
#208444=CARTESIAN_POINT('Ctrl Pts',(1.7317740975019,22.9868367391978,0.));
#208445=CARTESIAN_POINT('Ctrl Pts',(1.73369672350814,22.9723317685688,0.));
#208446=CARTESIAN_POINT('Ctrl Pts',(1.73555436162769,22.9579761301063,0.));
#208447=CARTESIAN_POINT('Ctrl Pts',(1.73734756100039,22.9437717457826,0.));
#208448=CARTESIAN_POINT('Ctrl Pts',(1.73907688511666,22.9297205792586,0.));
#208449=CARTESIAN_POINT('Ctrl Pts',(1.74074291231058,22.9158246373363,0.));
#208450=CARTESIAN_POINT('Ctrl Pts',(1.7423462363008,22.9020859716141,0.));
#208451=CARTESIAN_POINT('Ctrl Pts',(1.74388746677702,22.888506680335,0.));
#208452=CARTESIAN_POINT('Ctrl Pts',(1.74536722998201,22.8750889101696,0.));
#208453=CARTESIAN_POINT('Ctrl Pts',(1.74678616930664,22.8618348580235,0.));
#208454=CARTESIAN_POINT('Ctrl Pts',(1.74814494588492,22.8487467728076,0.));
#208455=CARTESIAN_POINT('Ctrl Pts',(1.74944423940115,22.8358269579853,0.));
#208456=CARTESIAN_POINT('Ctrl Pts',(1.75068474890883,22.8230777741284,0.));
#208457=CARTESIAN_POINT('Ctrl Pts',(1.75186719365592,22.8105016414713,0.));
#208458=CARTESIAN_POINT('Ctrl Pts',(1.75299231391466,22.7981010424314,0.));
#208459=CARTESIAN_POINT('Ctrl Pts',(1.75406087182936,22.7858785242361,0.));
#208460=CARTESIAN_POINT('Ctrl Pts',(1.75507365227131,22.7738367016118,0.));
#208461=CARTESIAN_POINT('Ctrl Pts',(1.75603146371641,22.7619782595013,0.));
#208462=CARTESIAN_POINT('Ctrl Pts',(1.75693513908907,22.750305955645,0.));
#208463=CARTESIAN_POINT('Ctrl Pts',(1.75778553673244,22.7388226235559,0.));
#208464=CARTESIAN_POINT('Ctrl Pts',(1.75858354204633,22.72753117773,0.));
#208465=CARTESIAN_POINT('Ctrl Pts',(1.75933006905925,22.7164346186006,0.));
#208466=CARTESIAN_POINT('Ctrl Pts',(1.76002606202401,22.7055360375485,0.));
#208467=CARTESIAN_POINT('Ctrl Pts',(1.76067249704886,22.6948386219851,0.));
#208468=CARTESIAN_POINT('Ctrl Pts',(1.76127038310614,22.684345658525,0.));
#208469=CARTESIAN_POINT('Ctrl Pts',(1.76182076289525,22.67406053567,0.));
#208470=CARTESIAN_POINT('Ctrl Pts',(1.76232471392568,22.6639867471753,0.));
#208471=CARTESIAN_POINT('Ctrl Pts',(1.76278334912561,22.6541278938409,0.));
#208472=CARTESIAN_POINT('Ctrl Pts',(1.76319782013916,22.6444876940423,0.));
#208473=CARTESIAN_POINT('Ctrl Pts',(1.76356932176273,22.6350699979359,0.));
#208474=CARTESIAN_POINT('Ctrl Pts',(1.76389909571403,22.6258787994848,0.));
#208475=CARTESIAN_POINT('Ctrl Pts',(1.76418843543739,22.6169182517694,0.));
#208476=CARTESIAN_POINT('Ctrl Pts',(1.76443868648015,22.6081926681343,0.));
#208477=CARTESIAN_POINT('Ctrl Pts',(1.76465124413557,22.5997065145638,0.));
#208478=CARTESIAN_POINT('Ctrl Pts',(1.76482755288411,22.5914644078106,0.));
#208479=CARTESIAN_POINT('Ctrl Pts',(1.76496910283088,22.5834711038022,0.));
#208480=CARTESIAN_POINT('Ctrl Pts',(1.76507744026746,22.5757315316353,0.));
#208481=CARTESIAN_POINT('Ctrl Pts',(1.76515418518831,22.5682508499873,0.));
#208482=CARTESIAN_POINT('Ctrl Pts',(1.7652010450045,22.5610344912501,0.));
#208483=CARTESIAN_POINT('Ctrl Pts',(1.76521983384062,22.5540882235837,0.));
#208484=CARTESIAN_POINT('Ctrl Pts',(1.76521245524047,22.5474180954006,0.));
#208485=CARTESIAN_POINT('Ctrl Pts',(1.76518087841493,22.5410303590892,0.));
#208486=CARTESIAN_POINT('Ctrl Pts',(1.76512711563254,22.5349313983571,0.));
#208487=CARTESIAN_POINT('Ctrl Pts',(1.76505320262759,22.529127665298,0.));
#208488=CARTESIAN_POINT('Ctrl Pts',(1.76496128643375,22.5236259635515,0.));
#208489=CARTESIAN_POINT('Ctrl Pts',(1.76485369319895,22.5184336670207,0.));
#208490=CARTESIAN_POINT('Ctrl Pts',(1.76473303281149,22.5135590569554,0.));
#208491=CARTESIAN_POINT('Ctrl Pts',(1.76460218257313,22.5090112700212,0.));
#208492=CARTESIAN_POINT('Ctrl Pts',(1.76446408210364,22.5047996391978,0.));
#208493=CARTESIAN_POINT('Ctrl Pts',(1.76432160068737,22.5009332677316,0.));
#208494=CARTESIAN_POINT('Ctrl Pts',(1.76417731243483,22.4974203063191,0.));
#208495=CARTESIAN_POINT('Ctrl Pts',(1.76403393880316,22.4942693792449,0.));
#208496=CARTESIAN_POINT('Ctrl Pts',(1.76389475965714,22.4914909094908,0.));
#208497=CARTESIAN_POINT('Ctrl Pts',(1.76376424879468,22.4890991659479,0.));
#208498=CARTESIAN_POINT('Ctrl Pts',(1.76364784232925,22.4871115206572,0.));
#208499=CARTESIAN_POINT('Ctrl Pts',(1.76355076045549,22.4855446605991,0.));
#208500=CARTESIAN_POINT('Ctrl Pts',(1.76347698284861,22.4844112933125,0.));
#208501=CARTESIAN_POINT('Ctrl Pts',(1.76343813434659,22.4838562517064,0.));
#208502=CARTESIAN_POINT('Ctrl Pts',(1.76342064263637,22.4836387052228,0.));
#208503=CARTESIAN_POINT('Ctrl Pts',(1.7634141553879,22.4835819929788,0.));
#208504=CARTESIAN_POINT('Ctrl Pts',(1.7634122053118,22.4835757167854,0.));
#208505=CARTESIAN_POINT('',(0.661312440730901,25.991588367311,0.));
#208506=CARTESIAN_POINT('Ctrl Pts',(4.11585220600461,22.1738711152697,0.));
#208507=CARTESIAN_POINT('Ctrl Pts',(4.11585220600461,22.1738711152697,12.));
#208508=CARTESIAN_POINT('Ctrl Pts',(4.11585194677442,22.173877682324,0.));
#208509=CARTESIAN_POINT('Ctrl Pts',(4.11585194677442,22.173877682324,12.));
#208510=CARTESIAN_POINT('Ctrl Pts',(4.11586035878287,22.1739341411687,0.));
#208511=CARTESIAN_POINT('Ctrl Pts',(4.11586035878287,22.1739341411687,12.));
#208512=CARTESIAN_POINT('Ctrl Pts',(4.11589976826166,22.1741488021234,0.));
#208513=CARTESIAN_POINT('Ctrl Pts',(4.11589976826166,22.1741488021234,12.));
#208514=CARTESIAN_POINT('Ctrl Pts',(4.11600589882845,22.1746949858775,0.));
#208515=CARTESIAN_POINT('Ctrl Pts',(4.11600589882845,22.1746949858775,12.));
#208516=CARTESIAN_POINT('Ctrl Pts',(4.11622797217068,22.1758088296598,0.));
#208517=CARTESIAN_POINT('Ctrl Pts',(4.11622797217068,22.1758088296598,12.));
#208518=CARTESIAN_POINT('Ctrl Pts',(4.11653973150518,22.177347426894,0.));
#208519=CARTESIAN_POINT('Ctrl Pts',(4.11653973150518,22.177347426894,12.));
#208520=CARTESIAN_POINT('Ctrl Pts',(4.11694173195003,22.179297473024,0.));
#208521=CARTESIAN_POINT('Ctrl Pts',(4.11694173195003,22.179297473024,12.));
#208522=CARTESIAN_POINT('Ctrl Pts',(4.11743469691756,22.1816414985788,0.));
#208523=CARTESIAN_POINT('Ctrl Pts',(4.11743469691756,22.1816414985788,12.));
#208524=CARTESIAN_POINT('Ctrl Pts',(4.11801938107479,22.1843613164855,0.));
#208525=CARTESIAN_POINT('Ctrl Pts',(4.11801938107479,22.1843613164855,12.));
#208526=CARTESIAN_POINT('Ctrl Pts',(4.11869641271773,22.1874419861496,0.));
#208527=CARTESIAN_POINT('Ctrl Pts',(4.11869641271773,22.1874419861496,12.));
#208528=CARTESIAN_POINT('Ctrl Pts',(4.11946626228636,22.1908725908525,0.));
#208529=CARTESIAN_POINT('Ctrl Pts',(4.11946626228636,22.1908725908525,12.));
#208530=CARTESIAN_POINT('Ctrl Pts',(4.12032932637736,22.1946440958098,0.));
#208531=CARTESIAN_POINT('Ctrl Pts',(4.12032932637736,22.1946440958098,12.));
#208532=CARTESIAN_POINT('Ctrl Pts',(4.12128598183522,22.1987479618246,0.));
#208533=CARTESIAN_POINT('Ctrl Pts',(4.12128598183522,22.1987479618246,12.));
#208534=CARTESIAN_POINT('Ctrl Pts',(4.12233664408227,22.2031746532106,0.));
#208535=CARTESIAN_POINT('Ctrl Pts',(4.12233664408227,22.2031746532106,12.));
#208536=CARTESIAN_POINT('Ctrl Pts',(4.12348173702023,22.2079143941719,0.));
#208537=CARTESIAN_POINT('Ctrl Pts',(4.12348173702023,22.2079143941719,12.));
#208538=CARTESIAN_POINT('Ctrl Pts',(4.12472167516607,22.2129576146671,0.));
#208539=CARTESIAN_POINT('Ctrl Pts',(4.12472167516607,22.2129576146671,12.));
#208540=CARTESIAN_POINT('Ctrl Pts',(4.12605683613307,22.2182956401341,0.));
#208541=CARTESIAN_POINT('Ctrl Pts',(4.12605683613307,22.2182956401341,12.));
#208542=CARTESIAN_POINT('Ctrl Pts',(4.12748755830104,22.2239207458781,0.));
#208543=CARTESIAN_POINT('Ctrl Pts',(4.12748755830104,22.2239207458781,12.));
#208544=CARTESIAN_POINT('Ctrl Pts',(4.12901415463379,22.2298258043947,0.));
#208545=CARTESIAN_POINT('Ctrl Pts',(4.12901415463379,22.2298258043947,12.));
#208546=CARTESIAN_POINT('Ctrl Pts',(4.13063692157498,22.2360040565533,0.));
#208547=CARTESIAN_POINT('Ctrl Pts',(4.13063692157498,22.2360040565533,12.));
#208548=CARTESIAN_POINT('Ctrl Pts',(4.1323561506016,22.2424488153523,0.));
#208549=CARTESIAN_POINT('Ctrl Pts',(4.1323561506016,22.2424488153523,12.));
#208550=CARTESIAN_POINT('Ctrl Pts',(4.1341721255881,22.249153531779,0.));
#208551=CARTESIAN_POINT('Ctrl Pts',(4.1341721255881,22.249153531779,12.));
#208552=CARTESIAN_POINT('Ctrl Pts',(4.13608511977225,22.2561118708421,0.));
#208553=CARTESIAN_POINT('Ctrl Pts',(4.13608511977225,22.2561118708421,12.));
#208554=CARTESIAN_POINT('Ctrl Pts',(4.13809539255421,22.2633177913972,0.));
#208555=CARTESIAN_POINT('Ctrl Pts',(4.13809539255421,22.2633177913972,12.));
#208556=CARTESIAN_POINT('Ctrl Pts',(4.14020318715991,22.2707656042457,0.));
#208557=CARTESIAN_POINT('Ctrl Pts',(4.14020318715991,22.2707656042457,12.));
#208558=CARTESIAN_POINT('Ctrl Pts',(4.14240873321984,22.2784499072027,0.));
#208559=CARTESIAN_POINT('Ctrl Pts',(4.14240873321984,22.2784499072027,12.));
#208560=CARTESIAN_POINT('Ctrl Pts',(4.14471224859295,22.2863655389166,0.));
#208561=CARTESIAN_POINT('Ctrl Pts',(4.14471224859295,22.2863655389166,12.));
#208562=CARTESIAN_POINT('Ctrl Pts',(4.14711394168556,22.2945075198467,0.));
#208563=CARTESIAN_POINT('Ctrl Pts',(4.14711394168556,22.2945075198467,12.));
#208564=CARTESIAN_POINT('Ctrl Pts',(4.14961401285522,22.3028710166933,0.));
#208565=CARTESIAN_POINT('Ctrl Pts',(4.14961401285522,22.3028710166933,12.));
#208566=CARTESIAN_POINT('Ctrl Pts',(4.1522126539699,22.3114513545185,0.));
#208567=CARTESIAN_POINT('Ctrl Pts',(4.1522126539699,22.3114513545185,12.));
#208568=CARTESIAN_POINT('Ctrl Pts',(4.15491004835281,22.3202440186979,0.));
#208569=CARTESIAN_POINT('Ctrl Pts',(4.15491004835281,22.3202440186979,12.));
#208570=CARTESIAN_POINT('Ctrl Pts',(4.15770637047889,22.3292446628959,0.));
#208571=CARTESIAN_POINT('Ctrl Pts',(4.15770637047889,22.3292446628959,12.));
#208572=CARTESIAN_POINT('Ctrl Pts',(4.16060178604164,22.3384491078602,0.));
#208573=CARTESIAN_POINT('Ctrl Pts',(4.16060178604164,22.3384491078602,12.));
#208574=CARTESIAN_POINT('Ctrl Pts',(4.16359645263187,22.3478533253889,0.));
#208575=CARTESIAN_POINT('Ctrl Pts',(4.16359645263187,22.3478533253889,12.));
#208576=CARTESIAN_POINT('Ctrl Pts',(4.166690520266,22.3574534257396,0.));
#208577=CARTESIAN_POINT('Ctrl Pts',(4.166690520266,22.3574534257396,12.));
#208578=CARTESIAN_POINT('Ctrl Pts',(4.16988413199457,22.36724564276,0.));
#208579=CARTESIAN_POINT('Ctrl Pts',(4.16988413199457,22.36724564276,12.));
#208580=CARTESIAN_POINT('Ctrl Pts',(4.17317742436145,22.3772263228617,0.));
#208581=CARTESIAN_POINT('Ctrl Pts',(4.17317742436145,22.3772263228617,12.));
#208582=CARTESIAN_POINT('Ctrl Pts',(4.17657052752825,22.3873919231334,0.));
#208583=CARTESIAN_POINT('Ctrl Pts',(4.17657052752825,22.3873919231334,12.));
#208584=CARTESIAN_POINT('Ctrl Pts',(4.18006356544882,22.3977390078075,0.));
#208585=CARTESIAN_POINT('Ctrl Pts',(4.18006356544882,22.3977390078075,12.));
#208586=CARTESIAN_POINT('Ctrl Pts',(4.1836566560085,22.4082642454453,0.));
#208587=CARTESIAN_POINT('Ctrl Pts',(4.1836566560085,22.4082642454453,12.));
#208588=CARTESIAN_POINT('Ctrl Pts',(4.1873499111772,22.4189644056115,0.));
#208589=CARTESIAN_POINT('Ctrl Pts',(4.1873499111772,22.4189644056115,12.));
#208590=CARTESIAN_POINT('Ctrl Pts',(4.19114343726941,22.4298363535421,0.));
#208591=CARTESIAN_POINT('Ctrl Pts',(4.19114343726941,22.4298363535421,12.));
#208592=CARTESIAN_POINT('Ctrl Pts',(4.1950373351886,22.4408770448917,0.));
#208593=CARTESIAN_POINT('Ctrl Pts',(4.1950373351886,22.4408770448917,12.));
#208594=CARTESIAN_POINT('Ctrl Pts',(4.19903170066354,22.4520835205419,0.));
#208595=CARTESIAN_POINT('Ctrl Pts',(4.19903170066354,22.4520835205419,12.));
#208596=CARTESIAN_POINT('Ctrl Pts',(4.2031266244817,22.4634529011433,0.));
#208597=CARTESIAN_POINT('Ctrl Pts',(4.2031266244817,22.4634529011433,12.));
#208598=CARTESIAN_POINT('Ctrl Pts',(4.20732219265648,22.4749823839915,0.));
#208599=CARTESIAN_POINT('Ctrl Pts',(4.20732219265648,22.4749823839915,12.));
#208600=CARTESIAN_POINT('Ctrl Pts',(4.21161848657428,22.4866692403147,0.));
#208601=CARTESIAN_POINT('Ctrl Pts',(4.21161848657428,22.4866692403147,12.));
#208602=CARTESIAN_POINT('Ctrl Pts',(4.21601558313908,22.4985108124229,0.));
#208603=CARTESIAN_POINT('Ctrl Pts',(4.21601558313908,22.4985108124229,12.));
#208604=CARTESIAN_POINT('Ctrl Pts',(4.22051355490196,22.5105045108882,0.));
#208605=CARTESIAN_POINT('Ctrl Pts',(4.22051355490196,22.5105045108882,12.));
#208606=CARTESIAN_POINT('Ctrl Pts',(4.2251124702004,22.5226478117885,0.));
#208607=CARTESIAN_POINT('Ctrl Pts',(4.2251124702004,22.5226478117885,12.));
#208608=CARTESIAN_POINT('Ctrl Pts',(4.22981239330731,22.5349382540587,0.));
#208609=CARTESIAN_POINT('Ctrl Pts',(4.22981239330731,22.5349382540587,12.));
#208610=CARTESIAN_POINT('Ctrl Pts',(4.23461338456713,22.5473734368086,0.));
#208611=CARTESIAN_POINT('Ctrl Pts',(4.23461338456713,22.5473734368086,12.));
#208612=CARTESIAN_POINT('Ctrl Pts',(4.23951550052526,22.559951016643,0.));
#208613=CARTESIAN_POINT('Ctrl Pts',(4.23951550052526,22.559951016643,12.));
#208614=CARTESIAN_POINT('Ctrl Pts',(4.24451879404858,22.5726687049922,0.));
#208615=CARTESIAN_POINT('Ctrl Pts',(4.24451879404858,22.5726687049922,12.));
#208616=CARTESIAN_POINT('Ctrl Pts',(4.24962331444184,22.5855242662479,0.));
#208617=CARTESIAN_POINT('Ctrl Pts',(4.24962331444184,22.5855242662479,12.));
#208618=CARTESIAN_POINT('Ctrl Pts',(4.25482910755485,22.5985155158637,0.));
#208619=CARTESIAN_POINT('Ctrl Pts',(4.25482910755485,22.5985155158637,12.));
#208620=CARTESIAN_POINT('Ctrl Pts',(4.26013621588303,22.611640318482,0.));
#208621=CARTESIAN_POINT('Ctrl Pts',(4.26013621588303,22.611640318482,12.));
#208622=CARTESIAN_POINT('Ctrl Pts',(4.26554467865571,22.6248965859975,0.));
#208623=CARTESIAN_POINT('Ctrl Pts',(4.26554467865571,22.6248965859975,12.));
#208624=CARTESIAN_POINT('Ctrl Pts',(4.27105453192999,22.6382822758171,0.));
#208625=CARTESIAN_POINT('Ctrl Pts',(4.27105453192999,22.6382822758171,12.));
#208626=CARTESIAN_POINT('Ctrl Pts',(4.27666580869117,22.6517953893303,0.));
#208627=CARTESIAN_POINT('Ctrl Pts',(4.27666580869117,22.6517953893303,12.));
#208628=CARTESIAN_POINT('Ctrl Pts',(4.28237853894059,22.665433970311,0.));
#208629=CARTESIAN_POINT('Ctrl Pts',(4.28237853894059,22.665433970311,12.));
#208630=CARTESIAN_POINT('Ctrl Pts',(4.28819274977766,22.6791961033537,0.));
#208631=CARTESIAN_POINT('Ctrl Pts',(4.28819274977766,22.6791961033537,12.));
#208632=CARTESIAN_POINT('Ctrl Pts',(4.29410846547061,22.6930799122545,0.));
#208633=CARTESIAN_POINT('Ctrl Pts',(4.29410846547061,22.6930799122545,12.));
#208634=CARTESIAN_POINT('Ctrl Pts',(4.30012570754066,22.707083558756,0.));
#208635=CARTESIAN_POINT('Ctrl Pts',(4.30012570754066,22.707083558756,12.));
#208636=CARTESIAN_POINT('Ctrl Pts',(4.30624449484074,22.7212052413384,0.));
#208637=CARTESIAN_POINT('Ctrl Pts',(4.30624449484074,22.7212052413384,12.));
#208638=CARTESIAN_POINT('Ctrl Pts',(4.3124648436255,22.7354431939927,0.));
#208639=CARTESIAN_POINT('Ctrl Pts',(4.3124648436255,22.7354431939927,12.));
#208640=CARTESIAN_POINT('Ctrl Pts',(4.3187867676123,22.7497956849852,0.));
#208641=CARTESIAN_POINT('Ctrl Pts',(4.3187867676123,22.7497956849852,12.));
#208642=CARTESIAN_POINT('Ctrl Pts',(4.32521027803747,22.764261015648,0.));
#208643=CARTESIAN_POINT('Ctrl Pts',(4.32521027803747,22.764261015648,12.));
#208644=CARTESIAN_POINT('Ctrl Pts',(4.33173538373182,22.7788375194081,0.));
#208645=CARTESIAN_POINT('Ctrl Pts',(4.33173538373182,22.7788375194081,12.));
#208646=CARTESIAN_POINT('Ctrl Pts',(4.33836209118442,22.7935235607807,0.));
#208647=CARTESIAN_POINT('Ctrl Pts',(4.33836209118442,22.7935235607807,12.));
#208648=CARTESIAN_POINT('Ctrl Pts',(4.34509040460065,22.808317534379,0.));
#208649=CARTESIAN_POINT('Ctrl Pts',(4.34509040460065,22.808317534379,12.));
#208650=CARTESIAN_POINT('Ctrl Pts',(4.35192032594801,22.8232178638873,0.));
#208651=CARTESIAN_POINT('Ctrl Pts',(4.35192032594801,22.8232178638873,12.));
#208652=CARTESIAN_POINT('Ctrl Pts',(4.35885185500559,22.838223001118,0.));
#208653=CARTESIAN_POINT('Ctrl Pts',(4.35885185500559,22.838223001118,12.));
#208654=CARTESIAN_POINT('Ctrl Pts',(4.36588498943009,22.8533314252419,0.));
#208655=CARTESIAN_POINT('Ctrl Pts',(4.36588498943009,22.8533314252419,12.));
#208656=CARTESIAN_POINT('Ctrl Pts',(4.37301972480752,22.8685416419725,0.));
#208657=CARTESIAN_POINT('Ctrl Pts',(4.37301972480752,22.8685416419725,12.));
#208658=CARTESIAN_POINT('Ctrl Pts',(4.38025605470089,22.8838521827702,0.));
#208659=CARTESIAN_POINT('Ctrl Pts',(4.38025605470089,22.8838521827702,12.));
#208660=CARTESIAN_POINT('Ctrl Pts',(4.38759397068391,22.8992616040108,0.));
#208661=CARTESIAN_POINT('Ctrl Pts',(4.38759397068391,22.8992616040108,12.));
#208662=CARTESIAN_POINT('Ctrl Pts',(4.39503346238454,22.9147684862425,0.));
#208663=CARTESIAN_POINT('Ctrl Pts',(4.39503346238454,22.9147684862425,12.));
#208664=CARTESIAN_POINT('Ctrl Pts',(4.40257451754307,22.9303714335549,0.));
#208665=CARTESIAN_POINT('Ctrl Pts',(4.40257451754307,22.9303714335549,12.));
#208666=CARTESIAN_POINT('Ctrl Pts',(4.41021712205547,22.9460690729093,0.));
#208667=CARTESIAN_POINT('Ctrl Pts',(4.41021712205547,22.9460690729093,12.));
#208668=CARTESIAN_POINT('Ctrl Pts',(4.41796126001309,22.9618600534866,0.));
#208669=CARTESIAN_POINT('Ctrl Pts',(4.41796126001309,22.9618600534866,12.));
#208670=CARTESIAN_POINT('Ctrl Pts',(4.42580691372771,22.9777430460021,0.));
#208671=CARTESIAN_POINT('Ctrl Pts',(4.42580691372771,22.9777430460021,12.));
#208672=CARTESIAN_POINT('Ctrl Pts',(4.43375406376904,22.9937167421009,0.));
#208673=CARTESIAN_POINT('Ctrl Pts',(4.43375406376904,22.9937167421009,12.));
#208674=CARTESIAN_POINT('Ctrl Pts',(4.44180268901666,23.0097798538399,0.));
#208675=CARTESIAN_POINT('Ctrl Pts',(4.44180268901666,23.0097798538399,12.));
#208676=CARTESIAN_POINT('Ctrl Pts',(4.44995276669698,23.0259311131395,0.));
#208677=CARTESIAN_POINT('Ctrl Pts',(4.44995276669698,23.0259311131395,12.));
#208678=CARTESIAN_POINT('Ctrl Pts',(4.45820427241676,23.0421692712466,0.));
#208679=CARTESIAN_POINT('Ctrl Pts',(4.45820427241676,23.0421692712466,12.));
#208680=CARTESIAN_POINT('Ctrl Pts',(4.46655718018205,23.0584930981723,0.));
#208681=CARTESIAN_POINT('Ctrl Pts',(4.46655718018205,23.0584930981723,12.));
#208682=CARTESIAN_POINT('Ctrl Pts',(4.47501146242821,23.0749013821868,0.));
#208683=CARTESIAN_POINT('Ctrl Pts',(4.47501146242821,23.0749013821868,12.));
#208684=CARTESIAN_POINT('Ctrl Pts',(4.48356709006756,23.0913929293909,0.));
#208685=CARTESIAN_POINT('Ctrl Pts',(4.48356709006756,23.0913929293909,12.));
#208686=CARTESIAN_POINT('Ctrl Pts',(4.49222403252201,23.1079665632629,0.));
#208687=CARTESIAN_POINT('Ctrl Pts',(4.49222403252201,23.1079665632629,12.));
#208688=CARTESIAN_POINT('Ctrl Pts',(4.50098225775178,23.1246211242117,0.));
#208689=CARTESIAN_POINT('Ctrl Pts',(4.50098225775178,23.1246211242117,12.));
#208690=CARTESIAN_POINT('Ctrl Pts',(4.50984173227087,23.1413554691136,0.));
#208691=CARTESIAN_POINT('Ctrl Pts',(4.50984173227087,23.1413554691136,12.));
#208692=CARTESIAN_POINT('Ctrl Pts',(4.51880242116785,23.1581684708778,0.));
#208693=CARTESIAN_POINT('Ctrl Pts',(4.51880242116785,23.1581684708778,12.));
#208694=CARTESIAN_POINT('Ctrl Pts',(4.52786428815047,23.1750590180923,0.));
#208695=CARTESIAN_POINT('Ctrl Pts',(4.52786428815047,23.1750590180923,12.));
#208696=CARTESIAN_POINT('Ctrl Pts',(4.53702729557585,23.1920260146474,0.));
#208697=CARTESIAN_POINT('Ctrl Pts',(4.53702729557585,23.1920260146474,12.));
#208698=CARTESIAN_POINT('Ctrl Pts',(4.54629140447542,23.2090683793627,0.));
#208699=CARTESIAN_POINT('Ctrl Pts',(4.54629140447542,23.2090683793627,12.));
#208700=CARTESIAN_POINT('Ctrl Pts',(4.55565657456956,23.2261850456055,0.));
#208701=CARTESIAN_POINT('Ctrl Pts',(4.55565657456956,23.2261850456055,12.));
#208702=CARTESIAN_POINT('Ctrl Pts',(4.5651227642781,23.2433749609117,0.));
#208703=CARTESIAN_POINT('Ctrl Pts',(4.5651227642781,23.2433749609117,12.));
#208704=CARTESIAN_POINT('Ctrl Pts',(4.5746899307607,23.2606370866853,0.));
#208705=CARTESIAN_POINT('Ctrl Pts',(4.5746899307607,23.2606370866853,12.));
#208706=CARTESIAN_POINT('Ctrl Pts',(4.58435802994674,23.2779703978868,0.));
#208707=CARTESIAN_POINT('Ctrl Pts',(4.58435802994674,23.2779703978868,12.));
#208708=CARTESIAN_POINT('Ctrl Pts',(4.59412701655749,23.295373882719,0.));
#208709=CARTESIAN_POINT('Ctrl Pts',(4.59412701655749,23.295373882719,12.));
#208710=CARTESIAN_POINT('Ctrl Pts',(4.60399684412174,23.3128465423119,0.));
#208711=CARTESIAN_POINT('Ctrl Pts',(4.60399684412174,23.3128465423119,12.));
#208712=CARTESIAN_POINT('Ctrl Pts',(4.61396746497848,23.3303873903947,0.));
#208713=CARTESIAN_POINT('Ctrl Pts',(4.61396746497848,23.3303873903947,12.));
#208714=CARTESIAN_POINT('Ctrl Pts',(4.62403883030823,23.3479954530281,0.));
#208715=CARTESIAN_POINT('Ctrl Pts',(4.62403883030823,23.3479954530281,12.));
#208716=CARTESIAN_POINT('Ctrl Pts',(4.63421089016554,23.3656697683496,0.));
#208717=CARTESIAN_POINT('Ctrl Pts',(4.63421089016554,23.3656697683496,12.));
#208718=CARTESIAN_POINT('Ctrl Pts',(4.64448359349935,23.383409386307,0.));
#208719=CARTESIAN_POINT('Ctrl Pts',(4.64448359349935,23.383409386307,12.));
#208720=CARTESIAN_POINT('Ctrl Pts',(4.65485688816921,23.4012133683957,0.));
#208721=CARTESIAN_POINT('Ctrl Pts',(4.65485688816921,23.4012133683957,12.));
#208722=CARTESIAN_POINT('Ctrl Pts',(4.66533072094663,23.4190807873798,0.));
#208723=CARTESIAN_POINT('Ctrl Pts',(4.66533072094663,23.4190807873798,12.));
#208724=CARTESIAN_POINT('Ctrl Pts',(4.6759050375305,23.4370107270444,0.));
#208725=CARTESIAN_POINT('Ctrl Pts',(4.6759050375305,23.4370107270444,12.));
#208726=CARTESIAN_POINT('Ctrl Pts',(4.68657978258297,23.4550022819853,0.));
#208727=CARTESIAN_POINT('Ctrl Pts',(4.68657978258297,23.4550022819853,12.));
#208728=CARTESIAN_POINT('Ctrl Pts',(4.69735489975023,23.4730545573849,0.));
#208729=CARTESIAN_POINT('Ctrl Pts',(4.69735489975023,23.4730545573849,12.));
#208730=CARTESIAN_POINT('Ctrl Pts',(4.7082303316782,23.491166668789,0.));
#208731=CARTESIAN_POINT('Ctrl Pts',(4.7082303316782,23.491166668789,12.));
#208732=CARTESIAN_POINT('Ctrl Pts',(4.71920602001904,23.5093377418784,0.));
#208733=CARTESIAN_POINT('Ctrl Pts',(4.71920602001904,23.5093377418784,12.));
#208734=CARTESIAN_POINT('Ctrl Pts',(4.73028190543031,23.5275669122378,0.));
#208735=CARTESIAN_POINT('Ctrl Pts',(4.73028190543031,23.5275669122378,12.));
#208736=CARTESIAN_POINT('Ctrl Pts',(4.74145792760698,23.5458533251715,0.));
#208737=CARTESIAN_POINT('Ctrl Pts',(4.74145792760698,23.5458533251715,12.));
#208738=CARTESIAN_POINT('Ctrl Pts',(4.75273402530615,23.564196135517,0.));
#208739=CARTESIAN_POINT('Ctrl Pts',(4.75273402530615,23.564196135517,12.));
#208740=CARTESIAN_POINT('Ctrl Pts',(4.7641101363625,23.5825945074535,0.));
#208741=CARTESIAN_POINT('Ctrl Pts',(4.7641101363625,23.5825945074535,12.));
#208742=CARTESIAN_POINT('Ctrl Pts',(4.77558619769875,23.6010476143099,0.));
#208743=CARTESIAN_POINT('Ctrl Pts',(4.77558619769875,23.6010476143099,12.));
#208744=CARTESIAN_POINT('Ctrl Pts',(4.78716214532104,23.6195546383625,0.));
#208745=CARTESIAN_POINT('Ctrl Pts',(4.78716214532104,23.6195546383625,12.));
#208746=CARTESIAN_POINT('Ctrl Pts',(4.79883791433229,23.6381147706581,0.));
#208747=CARTESIAN_POINT('Ctrl Pts',(4.79883791433229,23.6381147706581,12.));
#208748=CARTESIAN_POINT('Ctrl Pts',(4.81061343896442,23.6567272108631,0.));
#208749=CARTESIAN_POINT('Ctrl Pts',(4.81061343896442,23.6567272108631,12.));
#208750=CARTESIAN_POINT('Ctrl Pts',(4.82248865259569,23.6753911671023,0.));
#208751=CARTESIAN_POINT('Ctrl Pts',(4.82248865259569,23.6753911671023,12.));
#208752=CARTESIAN_POINT('Ctrl Pts',(4.83446348776267,23.6941058557971,0.));
#208753=CARTESIAN_POINT('Ctrl Pts',(4.83446348776267,23.6941058557971,12.));
#208754=CARTESIAN_POINT('Ctrl Pts',(4.84653787616422,23.7128705015014,0.));
#208755=CARTESIAN_POINT('Ctrl Pts',(4.84653787616422,23.7128705015014,12.));
#208756=CARTESIAN_POINT('Ctrl Pts',(4.85871174865491,23.7316843367308,0.));
#208757=CARTESIAN_POINT('Ctrl Pts',(4.85871174865491,23.7316843367308,12.));
#208758=CARTESIAN_POINT('Ctrl Pts',(4.87098503527142,23.7505466018239,0.));
#208759=CARTESIAN_POINT('Ctrl Pts',(4.87098503527142,23.7505466018239,12.));
#208760=CARTESIAN_POINT('Ctrl Pts',(4.88335766525565,23.7694565448044,0.));
#208761=CARTESIAN_POINT('Ctrl Pts',(4.88335766525565,23.7694565448044,12.));
#208762=CARTESIAN_POINT('Ctrl Pts',(4.89582956706771,23.7884134212381,0.));
#208763=CARTESIAN_POINT('Ctrl Pts',(4.89582956706771,23.7884134212381,12.));
#208764=CARTESIAN_POINT('Ctrl Pts',(4.90840066839346,23.8074164940897,0.));
#208765=CARTESIAN_POINT('Ctrl Pts',(4.90840066839346,23.8074164940897,12.));
#208766=CARTESIAN_POINT('Ctrl Pts',(4.92107089613976,23.8264650335721,0.));
#208767=CARTESIAN_POINT('Ctrl Pts',(4.92107089613976,23.8264650335721,12.));
#208768=CARTESIAN_POINT('Ctrl Pts',(4.93384017643441,23.8455583170062,0.));
#208769=CARTESIAN_POINT('Ctrl Pts',(4.93384017643441,23.8455583170062,12.));
#208770=CARTESIAN_POINT('Ctrl Pts',(4.94670843465868,23.8646956287172,0.));
#208771=CARTESIAN_POINT('Ctrl Pts',(4.94670843465868,23.8646956287172,12.));
#208772=CARTESIAN_POINT('Ctrl Pts',(4.95967559546565,23.883876259922,0.));
#208773=CARTESIAN_POINT('Ctrl Pts',(4.95967559546565,23.883876259922,12.));
#208774=CARTESIAN_POINT('Ctrl Pts',(4.97274158279228,23.9030995086164,0.));
#208775=CARTESIAN_POINT('Ctrl Pts',(4.97274158279228,23.9030995086164,12.));
#208776=CARTESIAN_POINT('Ctrl Pts',(4.98590631986532,23.9223646794591,0.));
#208777=CARTESIAN_POINT('Ctrl Pts',(4.98590631986532,23.9223646794591,12.));
#208778=CARTESIAN_POINT('Ctrl Pts',(4.99916972919309,23.9416710836529,0.));
#208779=CARTESIAN_POINT('Ctrl Pts',(4.99916972919309,23.9416710836529,12.));
#208780=CARTESIAN_POINT('Ctrl Pts',(5.01253173257458,23.9610180388271,0.));
#208781=CARTESIAN_POINT('Ctrl Pts',(5.01253173257458,23.9610180388271,12.));
#208782=CARTESIAN_POINT('Ctrl Pts',(5.02599225112461,23.9804048689228,0.));
#208783=CARTESIAN_POINT('Ctrl Pts',(5.02599225112461,23.9804048689228,12.));
#208784=CARTESIAN_POINT('Ctrl Pts',(5.03955120528527,23.9998309040747,0.));
#208785=CARTESIAN_POINT('Ctrl Pts',(5.03955120528527,23.9998309040747,12.));
#208786=CARTESIAN_POINT('Ctrl Pts',(5.05320851483068,24.0192954804896,0.));
#208787=CARTESIAN_POINT('Ctrl Pts',(5.05320851483068,24.0192954804896,12.));
#208788=CARTESIAN_POINT('Ctrl Pts',(5.06696409886639,24.0387979403268,0.));
#208789=CARTESIAN_POINT('Ctrl Pts',(5.06696409886639,24.0387979403268,12.));
#208790=CARTESIAN_POINT('Ctrl Pts',(5.0808178758127,24.0583376315636,0.));
#208791=CARTESIAN_POINT('Ctrl Pts',(5.0808178758127,24.0583376315636,12.));
#208792=CARTESIAN_POINT('Ctrl Pts',(5.09476976342616,24.0779139079264,0.));
#208793=CARTESIAN_POINT('Ctrl Pts',(5.09476976342616,24.0779139079264,12.));
#208794=CARTESIAN_POINT('Ctrl Pts',(5.10881967883124,24.0975261288444,0.));
#208795=CARTESIAN_POINT('Ctrl Pts',(5.10881967883124,24.0975261288444,12.));
#208796=CARTESIAN_POINT('Ctrl Pts',(5.12296753853857,24.117173659394,0.));
#208797=CARTESIAN_POINT('Ctrl Pts',(5.12296753853857,24.117173659394,12.));
#208798=CARTESIAN_POINT('Ctrl Pts',(5.13721325845745,24.1368558702443,0.));
#208799=CARTESIAN_POINT('Ctrl Pts',(5.13721325845745,24.1368558702443,12.));
#208800=CARTESIAN_POINT('Ctrl Pts',(5.15155675390079,24.1565721375971,0.));
#208801=CARTESIAN_POINT('Ctrl Pts',(5.15155675390079,24.1565721375971,12.));
#208802=CARTESIAN_POINT('Ctrl Pts',(5.16599793957985,24.1763218431344,0.));
#208803=CARTESIAN_POINT('Ctrl Pts',(5.16599793957985,24.1763218431344,12.));
#208804=CARTESIAN_POINT('Ctrl Pts',(5.18053672961398,24.1961043738756,0.));
#208805=CARTESIAN_POINT('Ctrl Pts',(5.18053672961398,24.1961043738756,12.));
#208806=CARTESIAN_POINT('Ctrl Pts',(5.19517303753647,24.2159191220171,0.));
#208807=CARTESIAN_POINT('Ctrl Pts',(5.19517303753647,24.2159191220171,12.));
#208808=CARTESIAN_POINT('Ctrl Pts',(5.20990677629176,24.2357654847766,0.));
#208809=CARTESIAN_POINT('Ctrl Pts',(5.20990677629176,24.2357654847766,12.));
#208810=CARTESIAN_POINT('Ctrl Pts',(5.22473785822442,24.2556428642294,0.));
#208811=CARTESIAN_POINT('Ctrl Pts',(5.22473785822442,24.2556428642294,12.));
#208812=CARTESIAN_POINT('Ctrl Pts',(5.23966619506289,24.2755506671525,0.));
#208813=CARTESIAN_POINT('Ctrl Pts',(5.23966619506289,24.2755506671525,12.));
#208814=CARTESIAN_POINT('Ctrl Pts',(5.25469169788856,24.2954883048447,0.));
#208815=CARTESIAN_POINT('Ctrl Pts',(5.25469169788856,24.2954883048447,12.));
#208816=CARTESIAN_POINT('Ctrl Pts',(5.26981427718798,24.3154551932221,0.));
#208817=CARTESIAN_POINT('Ctrl Pts',(5.26981427718798,24.3154551932221,12.));
#208818=CARTESIAN_POINT('Ctrl Pts',(5.28503384290648,24.3354507529414,0.));
#208819=CARTESIAN_POINT('Ctrl Pts',(5.28503384290648,24.3354507529414,12.));
#208820=CARTESIAN_POINT('Ctrl Pts',(5.30035030449063,24.3554744095075,0.));
#208821=CARTESIAN_POINT('Ctrl Pts',(5.30035030449063,24.3554744095075,12.));
#208822=CARTESIAN_POINT('Ctrl Pts',(5.31576357092526,24.3755255933917,0.));
#208823=CARTESIAN_POINT('Ctrl Pts',(5.31576357092526,24.3755255933917,12.));
#208824=CARTESIAN_POINT('Ctrl Pts',(5.33127355076033,24.3956037401293,0.));
#208825=CARTESIAN_POINT('Ctrl Pts',(5.33127355076033,24.3956037401293,12.));
#208826=CARTESIAN_POINT('Ctrl Pts',(5.34688015213537,24.4157082904614,0.));
#208827=CARTESIAN_POINT('Ctrl Pts',(5.34688015213537,24.4157082904614,12.));
#208828=CARTESIAN_POINT('Ctrl Pts',(5.36258328273627,24.435838689915,0.));
#208829=CARTESIAN_POINT('Ctrl Pts',(5.36258328273627,24.435838689915,12.));
#208830=CARTESIAN_POINT('Ctrl Pts',(5.37838284973695,24.4559943883157,0.));
#208831=CARTESIAN_POINT('Ctrl Pts',(5.37838284973695,24.4559943883157,12.));
#208832=CARTESIAN_POINT('Ctrl Pts',(5.39427875973824,24.4761748393321,0.));
#208833=CARTESIAN_POINT('Ctrl Pts',(5.39427875973824,24.4761748393321,12.));
#208834=CARTESIAN_POINT('Ctrl Pts',(5.41027091869241,24.4963794999831,0.));
#208835=CARTESIAN_POINT('Ctrl Pts',(5.41027091869241,24.4963794999831,12.));
#208836=CARTESIAN_POINT('Ctrl Pts',(5.42635923183419,24.5166078302108,0.));
#208837=CARTESIAN_POINT('Ctrl Pts',(5.42635923183419,24.5166078302108,12.));
#208838=CARTESIAN_POINT('Ctrl Pts',(5.4425436035688,24.5368592922863,0.));
#208839=CARTESIAN_POINT('Ctrl Pts',(5.4425436035688,24.5368592922863,12.));
#208840=CARTESIAN_POINT('Ctrl Pts',(5.45882393762261,24.5571333514842,0.));
#208841=CARTESIAN_POINT('Ctrl Pts',(5.45882393762261,24.5571333514842,12.));
#208842=CARTESIAN_POINT('Ctrl Pts',(5.47520013724419,24.5774294770329,0.));
#208843=CARTESIAN_POINT('Ctrl Pts',(5.47520013724419,24.5774294770329,12.));
#208844=CARTESIAN_POINT('Ctrl Pts',(5.49167210537246,24.5977471429364,0.));
#208845=CARTESIAN_POINT('Ctrl Pts',(5.49167210537246,24.5977471429364,12.));
#208846=CARTESIAN_POINT('Ctrl Pts',(5.50823974481962,24.6180858289179,0.));
#208847=CARTESIAN_POINT('Ctrl Pts',(5.50823974481962,24.6180858289179,12.));
#208848=CARTESIAN_POINT('Ctrl Pts',(5.52490295840991,24.6384450211467,0.));
#208849=CARTESIAN_POINT('Ctrl Pts',(5.52490295840991,24.6384450211467,12.));
#208850=CARTESIAN_POINT('Ctrl Pts',(5.54166164919583,24.6588242134738,0.));
#208851=CARTESIAN_POINT('Ctrl Pts',(5.54166164919583,24.6588242134738,12.));
#208852=CARTESIAN_POINT('Ctrl Pts',(5.55851572025376,24.6792229061794,0.));
#208853=CARTESIAN_POINT('Ctrl Pts',(5.55851572025376,24.6792229061794,12.));
#208854=CARTESIAN_POINT('Ctrl Pts',(5.57546507427754,24.6996406035517,0.));
#208855=CARTESIAN_POINT('Ctrl Pts',(5.57546507427754,24.6996406035517,12.));
#208856=CARTESIAN_POINT('Ctrl Pts',(5.59250961323987,24.7200768119088,0.));
#208857=CARTESIAN_POINT('Ctrl Pts',(5.59250961323987,24.7200768119088,12.));
#208858=CARTESIAN_POINT('Ctrl Pts',(5.60964923798491,24.7405310372739,0.));
#208859=CARTESIAN_POINT('Ctrl Pts',(5.60964923798491,24.7405310372739,12.));
#208860=CARTESIAN_POINT('Ctrl Pts',(5.62688384790923,24.7610027835697,0.));
#208861=CARTESIAN_POINT('Ctrl Pts',(5.62688384790923,24.7610027835697,12.));
#208862=CARTESIAN_POINT('Ctrl Pts',(5.6442133404226,24.781491549672,0.));
#208863=CARTESIAN_POINT('Ctrl Pts',(5.6442133404226,24.781491549672,12.));
#208864=CARTESIAN_POINT('Ctrl Pts',(5.66163761114921,24.8019968304605,0.));
#208865=CARTESIAN_POINT('Ctrl Pts',(5.66163761114921,24.8019968304605,12.));
#208866=CARTESIAN_POINT('Ctrl Pts',(5.67915655496542,24.8225181223845,0.));
#208867=CARTESIAN_POINT('Ctrl Pts',(5.67915655496542,24.8225181223845,12.));
#208868=CARTESIAN_POINT('Ctrl Pts',(5.69677006679444,24.8430549277621,0.));
#208869=CARTESIAN_POINT('Ctrl Pts',(5.69677006679444,24.8430549277621,12.));
#208870=CARTESIAN_POINT('Ctrl Pts',(5.71447804252027,24.8636067597669,0.));
#208871=CARTESIAN_POINT('Ctrl Pts',(5.71447804252027,24.8636067597669,12.));
#208872=CARTESIAN_POINT('Ctrl Pts',(5.73228037976926,24.884173146722,0.));
#208873=CARTESIAN_POINT('Ctrl Pts',(5.73228037976926,24.884173146722,12.));
#208874=CARTESIAN_POINT('Ctrl Pts',(5.75017697890804,24.904753637648,0.));
#208875=CARTESIAN_POINT('Ctrl Pts',(5.75017697890804,24.904753637648,12.));
#208876=CARTESIAN_POINT('Ctrl Pts',(5.76816774342219,24.9253478043656,0.));
#208877=CARTESIAN_POINT('Ctrl Pts',(5.76816774342219,24.9253478043656,12.));
#208878=CARTESIAN_POINT('Ctrl Pts',(5.78625257775681,24.945955229334,0.));
#208879=CARTESIAN_POINT('Ctrl Pts',(5.78625257775681,24.945955229334,12.));
#208880=CARTESIAN_POINT('Ctrl Pts',(5.80443138549726,24.9665754954496,0.));
#208881=CARTESIAN_POINT('Ctrl Pts',(5.80443138549726,24.9665754954496,12.));
#208882=CARTESIAN_POINT('Ctrl Pts',(5.82270406744198,24.9872081752734,0.));
#208883=CARTESIAN_POINT('Ctrl Pts',(5.82270406744198,24.9872081752734,12.));
#208884=CARTESIAN_POINT('Ctrl Pts',(5.84107051963071,25.0078528200564,0.));
#208885=CARTESIAN_POINT('Ctrl Pts',(5.84107051963071,25.0078528200564,12.));
#208886=CARTESIAN_POINT('Ctrl Pts',(5.85953063156826,25.0285089498899,0.));
#208887=CARTESIAN_POINT('Ctrl Pts',(5.85953063156826,25.0285089498899,12.));
#208888=CARTESIAN_POINT('Ctrl Pts',(5.87808428385365,25.0491760405911,0.));
#208889=CARTESIAN_POINT('Ctrl Pts',(5.87808428385365,25.0491760405911,12.));
#208890=CARTESIAN_POINT('Ctrl Pts',(5.89673135155514,25.0698535426514,0.));
#208891=CARTESIAN_POINT('Ctrl Pts',(5.89673135155514,25.0698535426514,12.));
#208892=CARTESIAN_POINT('Ctrl Pts',(5.91547170844447,25.0905409050773,0.));
#208893=CARTESIAN_POINT('Ctrl Pts',(5.91547170844447,25.0905409050773,12.));
#208894=CARTESIAN_POINT('Ctrl Pts',(5.93430523086834,25.1112375971106,0.));
#208895=CARTESIAN_POINT('Ctrl Pts',(5.93430523086834,25.1112375971106,12.));
#208896=CARTESIAN_POINT('Ctrl Pts',(5.95323180187378,25.1319431317237,0.));
#208897=CARTESIAN_POINT('Ctrl Pts',(5.95323180187378,25.1319431317237,12.));
#208898=CARTESIAN_POINT('Ctrl Pts',(5.97225131495616,25.1526570863092,0.));
#208899=CARTESIAN_POINT('Ctrl Pts',(5.97225131495616,25.1526570863092,12.));
#208900=CARTESIAN_POINT('Ctrl Pts',(5.99136367859754,25.1733791296259,0.));
#208901=CARTESIAN_POINT('Ctrl Pts',(5.99136367859754,25.1733791296259,12.));
#208902=CARTESIAN_POINT('Ctrl Pts',(6.01056881804612,25.1941090269819,0.));
#208903=CARTESIAN_POINT('Ctrl Pts',(6.01056881804612,25.1941090269819,12.));
#208904=CARTESIAN_POINT('Ctrl Pts',(6.02986667389996,25.21484662016,0.));
#208905=CARTESIAN_POINT('Ctrl Pts',(6.02986667389996,25.21484662016,12.));
#208906=CARTESIAN_POINT('Ctrl Pts',(6.04925720151218,25.2355918139032,0.));
#208907=CARTESIAN_POINT('Ctrl Pts',(6.04925720151218,25.2355918139032,12.));
#208908=CARTESIAN_POINT('Ctrl Pts',(6.06484373634546,25.2521940105705,0.));
#208909=CARTESIAN_POINT('Ctrl Pts',(6.06484373634546,25.2521940105705,12.));
#208910=CARTESIAN_POINT('Ctrl Pts',(6.0765753178749,25.2646490489923,0.));
#208911=CARTESIAN_POINT('Ctrl Pts',(6.0765753178749,25.2646490489923,12.));
#208912=CARTESIAN_POINT('Ctrl Pts',(6.08441489609793,25.2729539149517,0.));
#208913=CARTESIAN_POINT('Ctrl Pts',(6.08441489609793,25.2729539149517,12.));
#208914=CARTESIAN_POINT('Ctrl Pts',(6.08833931617699,25.2771067246846,0.));
#208915=CARTESIAN_POINT('Ctrl Pts',(6.08833931617699,25.2771067246846,12.));
#208916=CARTESIAN_POINT('',(6.08833931617699,25.2771067246846,0.));
#208917=CARTESIAN_POINT('Ctrl Pts',(4.11585220600461,22.1738711152697,0.));
#208918=CARTESIAN_POINT('Ctrl Pts',(4.11585194677442,22.173877682324,0.));
#208919=CARTESIAN_POINT('Ctrl Pts',(4.11586035878287,22.1739341411687,0.));
#208920=CARTESIAN_POINT('Ctrl Pts',(4.11589976826166,22.1741488021234,0.));
#208921=CARTESIAN_POINT('Ctrl Pts',(4.11600589882845,22.1746949858775,0.));
#208922=CARTESIAN_POINT('Ctrl Pts',(4.11622797217068,22.1758088296598,0.));
#208923=CARTESIAN_POINT('Ctrl Pts',(4.11653973150518,22.177347426894,0.));
#208924=CARTESIAN_POINT('Ctrl Pts',(4.11694173195003,22.179297473024,0.));
#208925=CARTESIAN_POINT('Ctrl Pts',(4.11743469691756,22.1816414985788,0.));
#208926=CARTESIAN_POINT('Ctrl Pts',(4.11801938107479,22.1843613164855,0.));
#208927=CARTESIAN_POINT('Ctrl Pts',(4.11869641271773,22.1874419861496,0.));
#208928=CARTESIAN_POINT('Ctrl Pts',(4.11946626228636,22.1908725908525,0.));
#208929=CARTESIAN_POINT('Ctrl Pts',(4.12032932637736,22.1946440958098,0.));
#208930=CARTESIAN_POINT('Ctrl Pts',(4.12128598183522,22.1987479618246,0.));
#208931=CARTESIAN_POINT('Ctrl Pts',(4.12233664408227,22.2031746532106,0.));
#208932=CARTESIAN_POINT('Ctrl Pts',(4.12348173702023,22.2079143941719,0.));
#208933=CARTESIAN_POINT('Ctrl Pts',(4.12472167516607,22.2129576146671,0.));
#208934=CARTESIAN_POINT('Ctrl Pts',(4.12605683613307,22.2182956401341,0.));
#208935=CARTESIAN_POINT('Ctrl Pts',(4.12748755830104,22.2239207458781,0.));
#208936=CARTESIAN_POINT('Ctrl Pts',(4.12901415463379,22.2298258043947,0.));
#208937=CARTESIAN_POINT('Ctrl Pts',(4.13063692157498,22.2360040565533,0.));
#208938=CARTESIAN_POINT('Ctrl Pts',(4.1323561506016,22.2424488153523,0.));
#208939=CARTESIAN_POINT('Ctrl Pts',(4.1341721255881,22.249153531779,0.));
#208940=CARTESIAN_POINT('Ctrl Pts',(4.13608511977225,22.2561118708421,0.));
#208941=CARTESIAN_POINT('Ctrl Pts',(4.13809539255421,22.2633177913972,0.));
#208942=CARTESIAN_POINT('Ctrl Pts',(4.14020318715991,22.2707656042457,0.));
#208943=CARTESIAN_POINT('Ctrl Pts',(4.14240873321984,22.2784499072027,0.));
#208944=CARTESIAN_POINT('Ctrl Pts',(4.14471224859295,22.2863655389166,0.));
#208945=CARTESIAN_POINT('Ctrl Pts',(4.14711394168556,22.2945075198467,0.));
#208946=CARTESIAN_POINT('Ctrl Pts',(4.14961401285522,22.3028710166933,0.));
#208947=CARTESIAN_POINT('Ctrl Pts',(4.1522126539699,22.3114513545185,0.));
#208948=CARTESIAN_POINT('Ctrl Pts',(4.15491004835281,22.3202440186979,0.));
#208949=CARTESIAN_POINT('Ctrl Pts',(4.15770637047889,22.3292446628959,0.));
#208950=CARTESIAN_POINT('Ctrl Pts',(4.16060178604164,22.3384491078602,0.));
#208951=CARTESIAN_POINT('Ctrl Pts',(4.16359645263187,22.3478533253889,0.));
#208952=CARTESIAN_POINT('Ctrl Pts',(4.166690520266,22.3574534257396,0.));
#208953=CARTESIAN_POINT('Ctrl Pts',(4.16988413199457,22.36724564276,0.));
#208954=CARTESIAN_POINT('Ctrl Pts',(4.17317742436145,22.3772263228617,0.));
#208955=CARTESIAN_POINT('Ctrl Pts',(4.17657052752825,22.3873919231334,0.));
#208956=CARTESIAN_POINT('Ctrl Pts',(4.18006356544882,22.3977390078075,0.));
#208957=CARTESIAN_POINT('Ctrl Pts',(4.1836566560085,22.4082642454453,0.));
#208958=CARTESIAN_POINT('Ctrl Pts',(4.1873499111772,22.4189644056115,0.));
#208959=CARTESIAN_POINT('Ctrl Pts',(4.19114343726941,22.4298363535421,0.));
#208960=CARTESIAN_POINT('Ctrl Pts',(4.1950373351886,22.4408770448917,0.));
#208961=CARTESIAN_POINT('Ctrl Pts',(4.19903170066354,22.4520835205419,0.));
#208962=CARTESIAN_POINT('Ctrl Pts',(4.2031266244817,22.4634529011433,0.));
#208963=CARTESIAN_POINT('Ctrl Pts',(4.20732219265648,22.4749823839915,0.));
#208964=CARTESIAN_POINT('Ctrl Pts',(4.21161848657428,22.4866692403147,0.));
#208965=CARTESIAN_POINT('Ctrl Pts',(4.21601558313908,22.4985108124229,0.));
#208966=CARTESIAN_POINT('Ctrl Pts',(4.22051355490196,22.5105045108882,0.));
#208967=CARTESIAN_POINT('Ctrl Pts',(4.2251124702004,22.5226478117885,0.));
#208968=CARTESIAN_POINT('Ctrl Pts',(4.22981239330731,22.5349382540587,0.));
#208969=CARTESIAN_POINT('Ctrl Pts',(4.23461338456713,22.5473734368086,0.));
#208970=CARTESIAN_POINT('Ctrl Pts',(4.23951550052526,22.559951016643,0.));
#208971=CARTESIAN_POINT('Ctrl Pts',(4.24451879404858,22.5726687049922,0.));
#208972=CARTESIAN_POINT('Ctrl Pts',(4.24962331444184,22.5855242662479,0.));
#208973=CARTESIAN_POINT('Ctrl Pts',(4.25482910755485,22.5985155158637,0.));
#208974=CARTESIAN_POINT('Ctrl Pts',(4.26013621588303,22.611640318482,0.));
#208975=CARTESIAN_POINT('Ctrl Pts',(4.26554467865571,22.6248965859975,0.));
#208976=CARTESIAN_POINT('Ctrl Pts',(4.27105453192999,22.6382822758171,0.));
#208977=CARTESIAN_POINT('Ctrl Pts',(4.27666580869117,22.6517953893303,0.));
#208978=CARTESIAN_POINT('Ctrl Pts',(4.28237853894059,22.665433970311,0.));
#208979=CARTESIAN_POINT('Ctrl Pts',(4.28819274977766,22.6791961033537,0.));
#208980=CARTESIAN_POINT('Ctrl Pts',(4.29410846547061,22.6930799122545,0.));
#208981=CARTESIAN_POINT('Ctrl Pts',(4.30012570754066,22.707083558756,0.));
#208982=CARTESIAN_POINT('Ctrl Pts',(4.30624449484074,22.7212052413384,0.));
#208983=CARTESIAN_POINT('Ctrl Pts',(4.3124648436255,22.7354431939927,0.));
#208984=CARTESIAN_POINT('Ctrl Pts',(4.3187867676123,22.7497956849852,0.));
#208985=CARTESIAN_POINT('Ctrl Pts',(4.32521027803747,22.764261015648,0.));
#208986=CARTESIAN_POINT('Ctrl Pts',(4.33173538373182,22.7788375194081,0.));
#208987=CARTESIAN_POINT('Ctrl Pts',(4.33836209118442,22.7935235607807,0.));
#208988=CARTESIAN_POINT('Ctrl Pts',(4.34509040460065,22.808317534379,0.));
#208989=CARTESIAN_POINT('Ctrl Pts',(4.35192032594801,22.8232178638873,0.));
#208990=CARTESIAN_POINT('Ctrl Pts',(4.35885185500559,22.838223001118,0.));
#208991=CARTESIAN_POINT('Ctrl Pts',(4.36588498943009,22.8533314252419,0.));
#208992=CARTESIAN_POINT('Ctrl Pts',(4.37301972480752,22.8685416419725,0.));
#208993=CARTESIAN_POINT('Ctrl Pts',(4.38025605470089,22.8838521827702,0.));
#208994=CARTESIAN_POINT('Ctrl Pts',(4.38759397068391,22.8992616040108,0.));
#208995=CARTESIAN_POINT('Ctrl Pts',(4.39503346238454,22.9147684862425,0.));
#208996=CARTESIAN_POINT('Ctrl Pts',(4.40257451754307,22.9303714335549,0.));
#208997=CARTESIAN_POINT('Ctrl Pts',(4.41021712205547,22.9460690729093,0.));
#208998=CARTESIAN_POINT('Ctrl Pts',(4.41796126001309,22.9618600534866,0.));
#208999=CARTESIAN_POINT('Ctrl Pts',(4.42580691372771,22.9777430460021,0.));
#209000=CARTESIAN_POINT('Ctrl Pts',(4.43375406376904,22.9937167421009,0.));
#209001=CARTESIAN_POINT('Ctrl Pts',(4.44180268901666,23.0097798538399,0.));
#209002=CARTESIAN_POINT('Ctrl Pts',(4.44995276669698,23.0259311131395,0.));
#209003=CARTESIAN_POINT('Ctrl Pts',(4.45820427241676,23.0421692712466,0.));
#209004=CARTESIAN_POINT('Ctrl Pts',(4.46655718018205,23.0584930981723,0.));
#209005=CARTESIAN_POINT('Ctrl Pts',(4.47501146242821,23.0749013821868,0.));
#209006=CARTESIAN_POINT('Ctrl Pts',(4.48356709006756,23.0913929293909,0.));
#209007=CARTESIAN_POINT('Ctrl Pts',(4.49222403252201,23.1079665632629,0.));
#209008=CARTESIAN_POINT('Ctrl Pts',(4.50098225775178,23.1246211242117,0.));
#209009=CARTESIAN_POINT('Ctrl Pts',(4.50984173227087,23.1413554691136,0.));
#209010=CARTESIAN_POINT('Ctrl Pts',(4.51880242116785,23.1581684708778,0.));
#209011=CARTESIAN_POINT('Ctrl Pts',(4.52786428815047,23.1750590180923,0.));
#209012=CARTESIAN_POINT('Ctrl Pts',(4.53702729557585,23.1920260146474,0.));
#209013=CARTESIAN_POINT('Ctrl Pts',(4.54629140447542,23.2090683793627,0.));
#209014=CARTESIAN_POINT('Ctrl Pts',(4.55565657456956,23.2261850456055,0.));
#209015=CARTESIAN_POINT('Ctrl Pts',(4.5651227642781,23.2433749609117,0.));
#209016=CARTESIAN_POINT('Ctrl Pts',(4.5746899307607,23.2606370866853,0.));
#209017=CARTESIAN_POINT('Ctrl Pts',(4.58435802994674,23.2779703978868,0.));
#209018=CARTESIAN_POINT('Ctrl Pts',(4.59412701655749,23.295373882719,0.));
#209019=CARTESIAN_POINT('Ctrl Pts',(4.60399684412174,23.3128465423119,0.));
#209020=CARTESIAN_POINT('Ctrl Pts',(4.61396746497848,23.3303873903947,0.));
#209021=CARTESIAN_POINT('Ctrl Pts',(4.62403883030823,23.3479954530281,0.));
#209022=CARTESIAN_POINT('Ctrl Pts',(4.63421089016554,23.3656697683496,0.));
#209023=CARTESIAN_POINT('Ctrl Pts',(4.64448359349935,23.383409386307,0.));
#209024=CARTESIAN_POINT('Ctrl Pts',(4.65485688816921,23.4012133683957,0.));
#209025=CARTESIAN_POINT('Ctrl Pts',(4.66533072094663,23.4190807873798,0.));
#209026=CARTESIAN_POINT('Ctrl Pts',(4.6759050375305,23.4370107270444,0.));
#209027=CARTESIAN_POINT('Ctrl Pts',(4.68657978258297,23.4550022819853,0.));
#209028=CARTESIAN_POINT('Ctrl Pts',(4.69735489975023,23.4730545573849,0.));
#209029=CARTESIAN_POINT('Ctrl Pts',(4.7082303316782,23.491166668789,0.));
#209030=CARTESIAN_POINT('Ctrl Pts',(4.71920602001904,23.5093377418784,0.));
#209031=CARTESIAN_POINT('Ctrl Pts',(4.73028190543031,23.5275669122378,0.));
#209032=CARTESIAN_POINT('Ctrl Pts',(4.74145792760698,23.5458533251715,0.));
#209033=CARTESIAN_POINT('Ctrl Pts',(4.75273402530615,23.564196135517,0.));
#209034=CARTESIAN_POINT('Ctrl Pts',(4.7641101363625,23.5825945074535,0.));
#209035=CARTESIAN_POINT('Ctrl Pts',(4.77558619769875,23.6010476143099,0.));
#209036=CARTESIAN_POINT('Ctrl Pts',(4.78716214532104,23.6195546383625,0.));
#209037=CARTESIAN_POINT('Ctrl Pts',(4.79883791433229,23.6381147706581,0.));
#209038=CARTESIAN_POINT('Ctrl Pts',(4.81061343896442,23.6567272108631,0.));
#209039=CARTESIAN_POINT('Ctrl Pts',(4.82248865259569,23.6753911671023,0.));
#209040=CARTESIAN_POINT('Ctrl Pts',(4.83446348776267,23.6941058557971,0.));
#209041=CARTESIAN_POINT('Ctrl Pts',(4.84653787616422,23.7128705015014,0.));
#209042=CARTESIAN_POINT('Ctrl Pts',(4.85871174865491,23.7316843367308,0.));
#209043=CARTESIAN_POINT('Ctrl Pts',(4.87098503527142,23.7505466018239,0.));
#209044=CARTESIAN_POINT('Ctrl Pts',(4.88335766525565,23.7694565448044,0.));
#209045=CARTESIAN_POINT('Ctrl Pts',(4.89582956706771,23.7884134212381,0.));
#209046=CARTESIAN_POINT('Ctrl Pts',(4.90840066839346,23.8074164940897,0.));
#209047=CARTESIAN_POINT('Ctrl Pts',(4.92107089613976,23.8264650335721,0.));
#209048=CARTESIAN_POINT('Ctrl Pts',(4.93384017643441,23.8455583170062,0.));
#209049=CARTESIAN_POINT('Ctrl Pts',(4.94670843465868,23.8646956287172,0.));
#209050=CARTESIAN_POINT('Ctrl Pts',(4.95967559546565,23.883876259922,0.));
#209051=CARTESIAN_POINT('Ctrl Pts',(4.97274158279228,23.9030995086164,0.));
#209052=CARTESIAN_POINT('Ctrl Pts',(4.98590631986532,23.9223646794591,0.));
#209053=CARTESIAN_POINT('Ctrl Pts',(4.99916972919309,23.9416710836529,0.));
#209054=CARTESIAN_POINT('Ctrl Pts',(5.01253173257458,23.9610180388271,0.));
#209055=CARTESIAN_POINT('Ctrl Pts',(5.02599225112461,23.9804048689228,0.));
#209056=CARTESIAN_POINT('Ctrl Pts',(5.03955120528527,23.9998309040747,0.));
#209057=CARTESIAN_POINT('Ctrl Pts',(5.05320851483068,24.0192954804896,0.));
#209058=CARTESIAN_POINT('Ctrl Pts',(5.06696409886639,24.0387979403268,0.));
#209059=CARTESIAN_POINT('Ctrl Pts',(5.0808178758127,24.0583376315636,0.));
#209060=CARTESIAN_POINT('Ctrl Pts',(5.09476976342616,24.0779139079264,0.));
#209061=CARTESIAN_POINT('Ctrl Pts',(5.10881967883124,24.0975261288444,0.));
#209062=CARTESIAN_POINT('Ctrl Pts',(5.12296753853857,24.117173659394,0.));
#209063=CARTESIAN_POINT('Ctrl Pts',(5.13721325845745,24.1368558702443,0.));
#209064=CARTESIAN_POINT('Ctrl Pts',(5.15155675390079,24.1565721375971,0.));
#209065=CARTESIAN_POINT('Ctrl Pts',(5.16599793957985,24.1763218431344,0.));
#209066=CARTESIAN_POINT('Ctrl Pts',(5.18053672961398,24.1961043738756,0.));
#209067=CARTESIAN_POINT('Ctrl Pts',(5.19517303753647,24.2159191220171,0.));
#209068=CARTESIAN_POINT('Ctrl Pts',(5.20990677629176,24.2357654847766,0.));
#209069=CARTESIAN_POINT('Ctrl Pts',(5.22473785822442,24.2556428642294,0.));
#209070=CARTESIAN_POINT('Ctrl Pts',(5.23966619506289,24.2755506671525,0.));
#209071=CARTESIAN_POINT('Ctrl Pts',(5.25469169788856,24.2954883048447,0.));
#209072=CARTESIAN_POINT('Ctrl Pts',(5.26981427718798,24.3154551932221,0.));
#209073=CARTESIAN_POINT('Ctrl Pts',(5.28503384290648,24.3354507529414,0.));
#209074=CARTESIAN_POINT('Ctrl Pts',(5.30035030449063,24.3554744095075,0.));
#209075=CARTESIAN_POINT('Ctrl Pts',(5.31576357092526,24.3755255933917,0.));
#209076=CARTESIAN_POINT('Ctrl Pts',(5.33127355076033,24.3956037401293,0.));
#209077=CARTESIAN_POINT('Ctrl Pts',(5.34688015213537,24.4157082904614,0.));
#209078=CARTESIAN_POINT('Ctrl Pts',(5.36258328273627,24.435838689915,0.));
#209079=CARTESIAN_POINT('Ctrl Pts',(5.37838284973695,24.4559943883157,0.));
#209080=CARTESIAN_POINT('Ctrl Pts',(5.39427875973824,24.4761748393321,0.));
#209081=CARTESIAN_POINT('Ctrl Pts',(5.41027091869241,24.4963794999831,0.));
#209082=CARTESIAN_POINT('Ctrl Pts',(5.42635923183419,24.5166078302108,0.));
#209083=CARTESIAN_POINT('Ctrl Pts',(5.4425436035688,24.5368592922863,0.));
#209084=CARTESIAN_POINT('Ctrl Pts',(5.45882393762261,24.5571333514842,0.));
#209085=CARTESIAN_POINT('Ctrl Pts',(5.47520013724419,24.5774294770329,0.));
#209086=CARTESIAN_POINT('Ctrl Pts',(5.49167210537246,24.5977471429364,0.));
#209087=CARTESIAN_POINT('Ctrl Pts',(5.50823974481962,24.6180858289179,0.));
#209088=CARTESIAN_POINT('Ctrl Pts',(5.52490295840991,24.6384450211467,0.));
#209089=CARTESIAN_POINT('Ctrl Pts',(5.54166164919583,24.6588242134738,0.));
#209090=CARTESIAN_POINT('Ctrl Pts',(5.55851572025376,24.6792229061794,0.));
#209091=CARTESIAN_POINT('Ctrl Pts',(5.57546507427754,24.6996406035517,0.));
#209092=CARTESIAN_POINT('Ctrl Pts',(5.59250961323987,24.7200768119088,0.));
#209093=CARTESIAN_POINT('Ctrl Pts',(5.60964923798491,24.7405310372739,0.));
#209094=CARTESIAN_POINT('Ctrl Pts',(5.62688384790923,24.7610027835697,0.));
#209095=CARTESIAN_POINT('Ctrl Pts',(5.6442133404226,24.781491549672,0.));
#209096=CARTESIAN_POINT('Ctrl Pts',(5.66163761114921,24.8019968304605,0.));
#209097=CARTESIAN_POINT('Ctrl Pts',(5.67915655496542,24.8225181223845,0.));
#209098=CARTESIAN_POINT('Ctrl Pts',(5.69677006679444,24.8430549277621,0.));
#209099=CARTESIAN_POINT('Ctrl Pts',(5.71447804252027,24.8636067597669,0.));
#209100=CARTESIAN_POINT('Ctrl Pts',(5.73228037976926,24.884173146722,0.));
#209101=CARTESIAN_POINT('Ctrl Pts',(5.75017697890804,24.904753637648,0.));
#209102=CARTESIAN_POINT('Ctrl Pts',(5.76816774342219,24.9253478043656,0.));
#209103=CARTESIAN_POINT('Ctrl Pts',(5.78625257775681,24.945955229334,0.));
#209104=CARTESIAN_POINT('Ctrl Pts',(5.80443138549726,24.9665754954496,0.));
#209105=CARTESIAN_POINT('Ctrl Pts',(5.82270406744198,24.9872081752734,0.));
#209106=CARTESIAN_POINT('Ctrl Pts',(5.84107051963071,25.0078528200564,0.));
#209107=CARTESIAN_POINT('Ctrl Pts',(5.85953063156826,25.0285089498899,0.));
#209108=CARTESIAN_POINT('Ctrl Pts',(5.87808428385365,25.0491760405911,0.));
#209109=CARTESIAN_POINT('Ctrl Pts',(5.89673135155514,25.0698535426514,0.));
#209110=CARTESIAN_POINT('Ctrl Pts',(5.91547170844447,25.0905409050773,0.));
#209111=CARTESIAN_POINT('Ctrl Pts',(5.93430523086834,25.1112375971106,0.));
#209112=CARTESIAN_POINT('Ctrl Pts',(5.95323180187378,25.1319431317237,0.));
#209113=CARTESIAN_POINT('Ctrl Pts',(5.97225131495616,25.1526570863092,0.));
#209114=CARTESIAN_POINT('Ctrl Pts',(5.99136367859754,25.1733791296259,0.));
#209115=CARTESIAN_POINT('Ctrl Pts',(6.01056881804612,25.1941090269819,0.));
#209116=CARTESIAN_POINT('Ctrl Pts',(6.02986667389996,25.21484662016,0.));
#209117=CARTESIAN_POINT('Ctrl Pts',(6.04925720151218,25.2355918139032,0.));
#209118=CARTESIAN_POINT('Ctrl Pts',(6.06484373634546,25.2521940105705,0.));
#209119=CARTESIAN_POINT('Ctrl Pts',(6.0765753178749,25.2646490489923,0.));
#209120=CARTESIAN_POINT('Ctrl Pts',(6.08441489609793,25.2729539149517,0.));
#209121=CARTESIAN_POINT('Ctrl Pts',(6.08833931617699,25.2771067246846,0.));
#209122=CARTESIAN_POINT('',(6.08833931617699,25.2771067246846,0.));
#209123=CARTESIAN_POINT('Origin',(9.26120677397564,19.4030938020118,0.));
#209124=CARTESIAN_POINT('',(9.71462809124917,20.353053841303,0.));
#209125=CARTESIAN_POINT('',(9.71462809124917,20.353053841303,0.));
#209126=CARTESIAN_POINT('',(4.63060338698782,9.70154690100589,0.));
#209127=CARTESIAN_POINT('Ctrl Pts',(7.36589684767344,24.9347862158358,0.));
#209128=CARTESIAN_POINT('Ctrl Pts',(7.36589684767344,24.9347862158358,12.));
#209129=CARTESIAN_POINT('Ctrl Pts',(7.36721909028842,24.9292275670674,0.));
#209130=CARTESIAN_POINT('Ctrl Pts',(7.36721909028842,24.9292275670674,12.));
#209131=CARTESIAN_POINT('Ctrl Pts',(7.3698559312009,24.9181155530543,0.));
#209132=CARTESIAN_POINT('Ctrl Pts',(7.3698559312009,24.9181155530543,12.));
#209133=CARTESIAN_POINT('Ctrl Pts',(7.37378825961676,24.901463382605,0.));
#209134=CARTESIAN_POINT('Ctrl Pts',(7.37378825961676,24.901463382605,12.));
#209135=CARTESIAN_POINT('Ctrl Pts',(7.37898549640269,24.8792921911115,0.));
#209136=CARTESIAN_POINT('Ctrl Pts',(7.37898549640269,24.8792921911115,12.));
#209137=CARTESIAN_POINT('Ctrl Pts',(7.3854055890362,24.8516310625176,0.));
#209138=CARTESIAN_POINT('Ctrl Pts',(7.3854055890362,24.8516310625176,12.));
#209139=CARTESIAN_POINT('Ctrl Pts',(7.39174922585808,24.8240228520893,0.));
#209140=CARTESIAN_POINT('Ctrl Pts',(7.39174922585808,24.8240228520893,12.));
#209141=CARTESIAN_POINT('Ctrl Pts',(7.39801641583012,24.7964676646431,0.));
#209142=CARTESIAN_POINT('Ctrl Pts',(7.39801641583012,24.7964676646431,12.));
#209143=CARTESIAN_POINT('Ctrl Pts',(7.40420718661602,24.7689656668983,0.));
#209144=CARTESIAN_POINT('Ctrl Pts',(7.40420718661602,24.7689656668983,12.));
#209145=CARTESIAN_POINT('Ctrl Pts',(7.41032159082381,24.7415170994784,0.));
#209146=CARTESIAN_POINT('Ctrl Pts',(7.41032159082381,24.7415170994784,12.));
#209147=CARTESIAN_POINT('Ctrl Pts',(7.41635971481674,24.7141222950051,0.));
#209148=CARTESIAN_POINT('Ctrl Pts',(7.41635971481674,24.7141222950051,12.));
#209149=CARTESIAN_POINT('Ctrl Pts',(7.42232167766265,24.6867816727192,0.));
#209150=CARTESIAN_POINT('Ctrl Pts',(7.42232167766265,24.6867816727192,12.));
#209151=CARTESIAN_POINT('Ctrl Pts',(7.42820762159125,24.6594957128756,0.));
#209152=CARTESIAN_POINT('Ctrl Pts',(7.42820762159125,24.6594957128756,12.));
#209153=CARTESIAN_POINT('Ctrl Pts',(7.43401770489523,24.6322649369517,0.));
#209154=CARTESIAN_POINT('Ctrl Pts',(7.43401770489523,24.6322649369517,12.));
#209155=CARTESIAN_POINT('Ctrl Pts',(7.43975209375503,24.6050898852368,0.));
#209156=CARTESIAN_POINT('Ctrl Pts',(7.43975209375503,24.6050898852368,12.));
#209157=CARTESIAN_POINT('Ctrl Pts',(7.44541095473134,24.577971096086,0.));
#209158=CARTESIAN_POINT('Ctrl Pts',(7.44541095473134,24.577971096086,12.));
#209159=CARTESIAN_POINT('Ctrl Pts',(7.4509944465116,24.5509090831559,0.));
#209160=CARTESIAN_POINT('Ctrl Pts',(7.4509944465116,24.5509090831559,12.));
#209161=CARTESIAN_POINT('Ctrl Pts',(7.45650271335861,24.5239043173072,0.));
#209162=CARTESIAN_POINT('Ctrl Pts',(7.45650271335861,24.5239043173072,12.));
#209163=CARTESIAN_POINT('Ctrl Pts',(7.46193588961463,24.4969572391483,0.));
#209164=CARTESIAN_POINT('Ctrl Pts',(7.46193588961463,24.4969572391483,12.));
#209165=CARTESIAN_POINT('Ctrl Pts',(7.46729410308786,24.4700682684524,0.));
#209166=CARTESIAN_POINT('Ctrl Pts',(7.46729410308786,24.4700682684524,12.));
#209167=CARTESIAN_POINT('Ctrl Pts',(7.47257747883246,24.443237814649,0.));
#209168=CARTESIAN_POINT('Ctrl Pts',(7.47257747883246,24.443237814649,12.));
#209169=CARTESIAN_POINT('Ctrl Pts',(7.47778614286564,24.4164662871163,0.));
#209170=CARTESIAN_POINT('Ctrl Pts',(7.47778614286564,24.4164662871163,12.));
#209171=CARTESIAN_POINT('Ctrl Pts',(7.482920225693,24.3897541049254,0.));
#209172=CARTESIAN_POINT('Ctrl Pts',(7.482920225693,24.3897541049254,12.));
#209173=CARTESIAN_POINT('Ctrl Pts',(7.48797986651908,24.3631017084524,0.));
#209174=CARTESIAN_POINT('Ctrl Pts',(7.48797986651908,24.3631017084524,12.));
#209175=CARTESIAN_POINT('Ctrl Pts',(7.4929652125242,24.3365095573685,0.));
#209176=CARTESIAN_POINT('Ctrl Pts',(7.4929652125242,24.3365095573685,12.));
#209177=CARTESIAN_POINT('Ctrl Pts',(7.49787641695438,24.3099781253355,0.));
#209178=CARTESIAN_POINT('Ctrl Pts',(7.49787641695438,24.3099781253355,12.));
#209179=CARTESIAN_POINT('Ctrl Pts',(7.50271363765151,24.2835078958973,0.));
#209180=CARTESIAN_POINT('Ctrl Pts',(7.50271363765151,24.2835078958973,12.));
#209181=CARTESIAN_POINT('Ctrl Pts',(7.50747703535133,24.2570993577034,0.));
#209182=CARTESIAN_POINT('Ctrl Pts',(7.50747703535133,24.2570993577034,12.));
#209183=CARTESIAN_POINT('Ctrl Pts',(7.5121667722218,24.2307530003887,0.));
#209184=CARTESIAN_POINT('Ctrl Pts',(7.5121667722218,24.2307530003887,12.));
#209185=CARTESIAN_POINT('Ctrl Pts',(7.51678300997949,24.2044693092349,0.));
#209186=CARTESIAN_POINT('Ctrl Pts',(7.51678300997949,24.2044693092349,12.));
#209187=CARTESIAN_POINT('Ctrl Pts',(7.52132590953801,24.1782487641594,0.));
#209188=CARTESIAN_POINT('Ctrl Pts',(7.52132590953801,24.1782487641594,12.));
#209189=CARTESIAN_POINT('Ctrl Pts',(7.52579563201423,24.1520918425364,0.));
#209190=CARTESIAN_POINT('Ctrl Pts',(7.52579563201423,24.1520918425364,12.));
#209191=CARTESIAN_POINT('Ctrl Pts',(7.53019233935501,24.1259990209207,0.));
#209192=CARTESIAN_POINT('Ctrl Pts',(7.53019233935501,24.1259990209207,12.));
#209193=CARTESIAN_POINT('Ctrl Pts',(7.53451619514649,24.0999707772642,0.));
#209194=CARTESIAN_POINT('Ctrl Pts',(7.53451619514649,24.0999707772642,12.));
#209195=CARTESIAN_POINT('Ctrl Pts',(7.53876736531013,24.0740075927985,0.));
#209196=CARTESIAN_POINT('Ctrl Pts',(7.53876736531013,24.0740075927985,12.));
#209197=CARTESIAN_POINT('Ctrl Pts',(7.54294601896144,24.0481099543353,0.));
#209198=CARTESIAN_POINT('Ctrl Pts',(7.54294601896144,24.0481099543353,12.));
#209199=CARTESIAN_POINT('Ctrl Pts',(7.5470523288591,24.022278355453,0.));
#209200=CARTESIAN_POINT('Ctrl Pts',(7.5470523288591,24.022278355453,12.));
#209201=CARTESIAN_POINT('Ctrl Pts',(7.5510864709744,23.9965132953185,0.));
#209202=CARTESIAN_POINT('Ctrl Pts',(7.5510864709744,23.9965132953185,12.));
#209203=CARTESIAN_POINT('Ctrl Pts',(7.55504862424811,23.9708152779884,0.));
#209204=CARTESIAN_POINT('Ctrl Pts',(7.55504862424811,23.9708152779884,12.));
#209205=CARTESIAN_POINT('Ctrl Pts',(7.55893897027682,23.9451848115,0.));
#209206=CARTESIAN_POINT('Ctrl Pts',(7.55893897027682,23.9451848115,12.));
#209207=CARTESIAN_POINT('Ctrl Pts',(7.56275769304773,23.9196224070759,0.));
#209208=CARTESIAN_POINT('Ctrl Pts',(7.56275769304773,23.9196224070759,12.));
#209209=CARTESIAN_POINT('Ctrl Pts',(7.56650497863791,23.8941285782003,0.));
#209210=CARTESIAN_POINT('Ctrl Pts',(7.56650497863791,23.8941285782003,12.));
#209211=CARTESIAN_POINT('Ctrl Pts',(7.5701810150071,23.8687038399598,0.));
#209212=CARTESIAN_POINT('Ctrl Pts',(7.5701810150071,23.8687038399598,12.));
#209213=CARTESIAN_POINT('Ctrl Pts',(7.57378599219816,23.8433487096134,0.));
#209214=CARTESIAN_POINT('Ctrl Pts',(7.57378599219816,23.8433487096134,12.));
#209215=CARTESIAN_POINT('Ctrl Pts',(7.57732010249065,23.8180637069977,0.));
#209216=CARTESIAN_POINT('Ctrl Pts',(7.57732010249065,23.8180637069977,12.));
#209217=CARTESIAN_POINT('Ctrl Pts',(7.58078354058211,23.7928493549908,0.));
#209218=CARTESIAN_POINT('Ctrl Pts',(7.58078354058211,23.7928493549908,12.));
#209219=CARTESIAN_POINT('Ctrl Pts',(7.58417650376271,23.7677061799376,0.));
#209220=CARTESIAN_POINT('Ctrl Pts',(7.58417650376271,23.7677061799376,12.));
#209221=CARTESIAN_POINT('Ctrl Pts',(7.58749919210831,23.7426347121006,0.));
#209222=CARTESIAN_POINT('Ctrl Pts',(7.58749919210831,23.7426347121006,12.));
#209223=CARTESIAN_POINT('Ctrl Pts',(7.59075180865326,23.7176354860457,0.));
#209224=CARTESIAN_POINT('Ctrl Pts',(7.59075180865326,23.7176354860457,12.));
#209225=CARTESIAN_POINT('Ctrl Pts',(7.59393455934041,23.6927090405067,0.));
#209226=CARTESIAN_POINT('Ctrl Pts',(7.59393455934041,23.6927090405067,12.));
#209227=CARTESIAN_POINT('Ctrl Pts',(7.59704765299572,23.6678559182876,0.));
#209228=CARTESIAN_POINT('Ctrl Pts',(7.59704765299572,23.6678559182876,12.));
#209229=CARTESIAN_POINT('Ctrl Pts',(7.60009130130129,23.6430766661419,0.));
#209230=CARTESIAN_POINT('Ctrl Pts',(7.60009130130129,23.6430766661419,12.));
#209231=CARTESIAN_POINT('Ctrl Pts',(7.60306571877806,23.6183718346576,0.));
#209232=CARTESIAN_POINT('Ctrl Pts',(7.60306571877806,23.6183718346576,12.));
#209233=CARTESIAN_POINT('Ctrl Pts',(7.60597112277094,23.5937419781244,0.));
#209234=CARTESIAN_POINT('Ctrl Pts',(7.60597112277094,23.5937419781244,12.));
#209235=CARTESIAN_POINT('Ctrl Pts',(7.60880773344599,23.5691876544243,0.));
#209236=CARTESIAN_POINT('Ctrl Pts',(7.60880773344599,23.5691876544243,12.));
#209237=CARTESIAN_POINT('Ctrl Pts',(7.61157577385371,23.5447094252029,0.));
#209238=CARTESIAN_POINT('Ctrl Pts',(7.61157577385371,23.5447094252029,12.));
#209239=CARTESIAN_POINT('Ctrl Pts',(7.61427546999298,23.5203078560128,0.));
#209240=CARTESIAN_POINT('Ctrl Pts',(7.61427546999298,23.5203078560128,12.));
#209241=CARTESIAN_POINT('Ctrl Pts',(7.61690705088318,23.4959835164608,0.));
#209242=CARTESIAN_POINT('Ctrl Pts',(7.61690705088318,23.4959835164608,12.));
#209243=CARTESIAN_POINT('Ctrl Pts',(7.61947074863977,23.4717369803438,0.));
#209244=CARTESIAN_POINT('Ctrl Pts',(7.61947074863977,23.4717369803438,12.));
#209245=CARTESIAN_POINT('Ctrl Pts',(7.62196679855957,23.4475688257855,0.));
#209246=CARTESIAN_POINT('Ctrl Pts',(7.62196679855957,23.4475688257855,12.));
#209247=CARTESIAN_POINT('Ctrl Pts',(7.62439543920053,23.4234796353544,0.));
#209248=CARTESIAN_POINT('Ctrl Pts',(7.62439543920053,23.4234796353544,12.));
#209249=CARTESIAN_POINT('Ctrl Pts',(7.62675691240334,23.3994699961122,0.));
#209250=CARTESIAN_POINT('Ctrl Pts',(7.62675691240334,23.3994699961122,12.));
#209251=CARTESIAN_POINT('Ctrl Pts',(7.62905146332597,23.3755404996638,0.));
#209252=CARTESIAN_POINT('Ctrl Pts',(7.62905146332597,23.3755404996638,12.));
#209253=CARTESIAN_POINT('Ctrl Pts',(7.63127934048138,23.3516917421973,0.));
#209254=CARTESIAN_POINT('Ctrl Pts',(7.63127934048138,23.3516917421973,12.));
#209255=CARTESIAN_POINT('Ctrl Pts',(7.63344079578162,23.3279243245241,0.));
#209256=CARTESIAN_POINT('Ctrl Pts',(7.63344079578162,23.3279243245241,12.));
#209257=CARTESIAN_POINT('Ctrl Pts',(7.63553608458783,23.3042388521021,0.));
#209258=CARTESIAN_POINT('Ctrl Pts',(7.63553608458783,23.3042388521021,12.));
#209259=CARTESIAN_POINT('Ctrl Pts',(7.63756546576374,23.2806359350853,0.));
#209260=CARTESIAN_POINT('Ctrl Pts',(7.63756546576374,23.2806359350853,12.));
#209261=CARTESIAN_POINT('Ctrl Pts',(7.63952920172837,23.2571161884487,0.));
#209262=CARTESIAN_POINT('Ctrl Pts',(7.63952920172837,23.2571161884487,12.));
#209263=CARTESIAN_POINT('Ctrl Pts',(7.64142755851507,23.2336802320912,0.));
#209264=CARTESIAN_POINT('Ctrl Pts',(7.64142755851507,23.2336802320912,12.));
#209265=CARTESIAN_POINT('Ctrl Pts',(7.64326080583683,23.2103286909399,0.));
#209266=CARTESIAN_POINT('Ctrl Pts',(7.64326080583683,23.2103286909399,12.));
#209267=CARTESIAN_POINT('Ctrl Pts',(7.64502921715482,23.1870621950452,0.));
#209268=CARTESIAN_POINT('Ctrl Pts',(7.64502921715482,23.1870621950452,12.));
#209269=CARTESIAN_POINT('Ctrl Pts',(7.64673306975796,23.1638813796691,0.));
#209270=CARTESIAN_POINT('Ctrl Pts',(7.64673306975796,23.1638813796691,12.));
#209271=CARTESIAN_POINT('Ctrl Pts',(7.64837264482929,23.1407868853815,0.));
#209272=CARTESIAN_POINT('Ctrl Pts',(7.64837264482929,23.1407868853815,12.));
#209273=CARTESIAN_POINT('Ctrl Pts',(7.64994822749844,23.1177793581674,0.));
#209274=CARTESIAN_POINT('Ctrl Pts',(7.64994822749844,23.1177793581674,12.));
#209275=CARTESIAN_POINT('Ctrl Pts',(7.65146010690464,23.0948594495246,0.));
#209276=CARTESIAN_POINT('Ctrl Pts',(7.65146010690464,23.0948594495246,12.));
#209277=CARTESIAN_POINT('Ctrl Pts',(7.65290857626356,23.072027816555,0.));
#209278=CARTESIAN_POINT('Ctrl Pts',(7.65290857626356,23.072027816555,12.));
#209279=CARTESIAN_POINT('Ctrl Pts',(7.65429393293955,23.049285122053,0.));
#209280=CARTESIAN_POINT('Ctrl Pts',(7.65429393293955,23.049285122053,12.));
#209281=CARTESIAN_POINT('Ctrl Pts',(7.65561647852554,23.0266320345792,0.));
#209282=CARTESIAN_POINT('Ctrl Pts',(7.65561647852554,23.0266320345792,12.));
#209283=CARTESIAN_POINT('Ctrl Pts',(7.6568765189133,23.004069228582,0.));
#209284=CARTESIAN_POINT('Ctrl Pts',(7.6568765189133,23.004069228582,12.));
#209285=CARTESIAN_POINT('Ctrl Pts',(7.65807436436452,22.9815973845301,0.));
#209286=CARTESIAN_POINT('Ctrl Pts',(7.65807436436452,22.9815973845301,12.));
#209287=CARTESIAN_POINT('Ctrl Pts',(7.65921032958911,22.9592171890332,0.));
#209288=CARTESIAN_POINT('Ctrl Pts',(7.65921032958911,22.9592171890332,12.));
#209289=CARTESIAN_POINT('Ctrl Pts',(7.66028473382776,22.9369293349592,0.));
#209290=CARTESIAN_POINT('Ctrl Pts',(7.66028473382776,22.9369293349592,12.));
#209291=CARTESIAN_POINT('Ctrl Pts',(7.66129790094099,22.9147345215418,0.));
#209292=CARTESIAN_POINT('Ctrl Pts',(7.66129790094099,22.9147345215418,12.));
#209293=CARTESIAN_POINT('Ctrl Pts',(7.66225015950147,22.8926334544879,0.));
#209294=CARTESIAN_POINT('Ctrl Pts',(7.66225015950147,22.8926334544879,12.));
#209295=CARTESIAN_POINT('Ctrl Pts',(7.66314184287333,22.870626846128,0.));
#209296=CARTESIAN_POINT('Ctrl Pts',(7.66314184287333,22.870626846128,12.));
#209297=CARTESIAN_POINT('Ctrl Pts',(7.66397328929805,22.8487154155569,0.));
#209298=CARTESIAN_POINT('Ctrl Pts',(7.66397328929805,22.8487154155569,12.));
#209299=CARTESIAN_POINT('Ctrl Pts',(7.66474484198552,22.8268998887679,0.));
#209300=CARTESIAN_POINT('Ctrl Pts',(7.66474484198552,22.8268998887679,12.));
#209301=CARTESIAN_POINT('Ctrl Pts',(7.66545684920987,22.8051809987834,0.));
#209302=CARTESIAN_POINT('Ctrl Pts',(7.66545684920987,22.8051809987834,12.));
#209303=CARTESIAN_POINT('Ctrl Pts',(7.66610966441259,22.7835594857697,0.));
#209304=CARTESIAN_POINT('Ctrl Pts',(7.66610966441259,22.7835594857697,12.));
#209305=CARTESIAN_POINT('Ctrl Pts',(7.66670364630273,22.7620360971839,0.));
#209306=CARTESIAN_POINT('Ctrl Pts',(7.66670364630273,22.7620360971839,12.));
#209307=CARTESIAN_POINT('Ctrl Pts',(7.66723915895412,22.7406115879508,0.));
#209308=CARTESIAN_POINT('Ctrl Pts',(7.66723915895412,22.7406115879508,12.));
#209309=CARTESIAN_POINT('Ctrl Pts',(7.6677165719101,22.7192867206242,0.));
#209310=CARTESIAN_POINT('Ctrl Pts',(7.6677165719101,22.7192867206242,12.));
#209311=CARTESIAN_POINT('Ctrl Pts',(7.66813626029276,22.6980622655446,0.));
#209312=CARTESIAN_POINT('Ctrl Pts',(7.66813626029276,22.6980622655446,12.));
#209313=CARTESIAN_POINT('Ctrl Pts',(7.66849860491762,22.6769390009889,0.));
#209314=CARTESIAN_POINT('Ctrl Pts',(7.66849860491762,22.6769390009889,12.));
#209315=CARTESIAN_POINT('Ctrl Pts',(7.66880399241353,22.6559177133133,0.));
#209316=CARTESIAN_POINT('Ctrl Pts',(7.66880399241353,22.6559177133133,12.));
#209317=CARTESIAN_POINT('Ctrl Pts',(7.66905281533744,22.6349991971548,0.));
#209318=CARTESIAN_POINT('Ctrl Pts',(7.66905281533744,22.6349991971548,12.));
#209319=CARTESIAN_POINT('Ctrl Pts',(7.66924547229434,22.6141842556248,0.));
#209320=CARTESIAN_POINT('Ctrl Pts',(7.66924547229434,22.6141842556248,12.));
#209321=CARTESIAN_POINT('Ctrl Pts',(7.6693823680624,22.5934737004955,0.));
#209322=CARTESIAN_POINT('Ctrl Pts',(7.6693823680624,22.5934737004955,12.));
#209323=CARTESIAN_POINT('Ctrl Pts',(7.66946391372299,22.5728683523829,0.));
#209324=CARTESIAN_POINT('Ctrl Pts',(7.66946391372299,22.5728683523829,12.));
#209325=CARTESIAN_POINT('Ctrl Pts',(7.66949052679671,22.5523690409109,0.));
#209326=CARTESIAN_POINT('Ctrl Pts',(7.66949052679671,22.5523690409109,12.));
#209327=CARTESIAN_POINT('Ctrl Pts',(7.66946263138115,22.5319766049191,0.));
#209328=CARTESIAN_POINT('Ctrl Pts',(7.66946263138115,22.5319766049191,12.));
#209329=CARTESIAN_POINT('Ctrl Pts',(7.66938065829082,22.5116918927023,0.));
#209330=CARTESIAN_POINT('Ctrl Pts',(7.66938065829082,22.5116918927023,12.));
#209331=CARTESIAN_POINT('Ctrl Pts',(7.66924504520301,22.4915157622308,0.));
#209332=CARTESIAN_POINT('Ctrl Pts',(7.66924504520301,22.4915157622308,12.));
#209333=CARTESIAN_POINT('Ctrl Pts',(7.66905623680835,22.47144908137,0.));
#209334=CARTESIAN_POINT('Ctrl Pts',(7.66905623680835,22.47144908137,12.));
#209335=CARTESIAN_POINT('Ctrl Pts',(7.66881468496659,22.4514927280863,0.));
#209336=CARTESIAN_POINT('Ctrl Pts',(7.66881468496659,22.4514927280863,12.));
#209337=CARTESIAN_POINT('Ctrl Pts',(7.66852084886745,22.4316475906616,0.));
#209338=CARTESIAN_POINT('Ctrl Pts',(7.66852084886745,22.4316475906616,12.));
#209339=CARTESIAN_POINT('Ctrl Pts',(7.66817519519681,22.411914567977,0.));
#209340=CARTESIAN_POINT('Ctrl Pts',(7.66817519519681,22.411914567977,12.));
#209341=CARTESIAN_POINT('Ctrl Pts',(7.66777819830819,22.3922945697782,0.));
#209342=CARTESIAN_POINT('Ctrl Pts',(7.66777819830819,22.3922945697782,12.));
#209343=CARTESIAN_POINT('Ctrl Pts',(7.66733034039887,22.3727885169361,0.));
#209344=CARTESIAN_POINT('Ctrl Pts',(7.66733034039887,22.3727885169361,12.));
#209345=CARTESIAN_POINT('Ctrl Pts',(7.66683211169133,22.3533973417013,0.));
#209346=CARTESIAN_POINT('Ctrl Pts',(7.66683211169133,22.3533973417013,12.));
#209347=CARTESIAN_POINT('Ctrl Pts',(7.66628401061905,22.3341219879454,0.));
#209348=CARTESIAN_POINT('Ctrl Pts',(7.66628401061905,22.3341219879454,12.));
#209349=CARTESIAN_POINT('Ctrl Pts',(7.66568654402441,22.3149634114823,0.));
#209350=CARTESIAN_POINT('Ctrl Pts',(7.66568654402441,22.3149634114823,12.));
#209351=CARTESIAN_POINT('Ctrl Pts',(7.66504022736262,22.2959225803925,0.));
#209352=CARTESIAN_POINT('Ctrl Pts',(7.66504022736262,22.2959225803925,12.));
#209353=CARTESIAN_POINT('Ctrl Pts',(7.66434558490972,22.2770004753332,0.));
#209354=CARTESIAN_POINT('Ctrl Pts',(7.66434558490972,22.2770004753332,12.));
#209355=CARTESIAN_POINT('Ctrl Pts',(7.66360314997661,22.2581980898487,0.));
#209356=CARTESIAN_POINT('Ctrl Pts',(7.66360314997661,22.2581980898487,12.));
#209357=CARTESIAN_POINT('Ctrl Pts',(7.66281346512545,22.239516430656,0.));
#209358=CARTESIAN_POINT('Ctrl Pts',(7.66281346512545,22.239516430656,12.));
#209359=CARTESIAN_POINT('Ctrl Pts',(7.66197708240435,22.2209565180098,0.));
#209360=CARTESIAN_POINT('Ctrl Pts',(7.66197708240435,22.2209565180098,12.));
#209361=CARTESIAN_POINT('Ctrl Pts',(7.66109456359292,22.2025193860972,0.));
#209362=CARTESIAN_POINT('Ctrl Pts',(7.66109456359292,22.2025193860972,12.));
#209363=CARTESIAN_POINT('Ctrl Pts',(7.66016648045007,22.1842060834093,0.));
#209364=CARTESIAN_POINT('Ctrl Pts',(7.66016648045007,22.1842060834093,12.));
#209365=CARTESIAN_POINT('Ctrl Pts',(7.65919341496925,22.1660176731174,0.));
#209366=CARTESIAN_POINT('Ctrl Pts',(7.65919341496925,22.1660176731174,12.));
#209367=CARTESIAN_POINT('Ctrl Pts',(7.6581759596335,22.1479552334206,0.));
#209368=CARTESIAN_POINT('Ctrl Pts',(7.6581759596335,22.1479552334206,12.));
#209369=CARTESIAN_POINT('Ctrl Pts',(7.65711471769406,22.1300198579671,0.));
#209370=CARTESIAN_POINT('Ctrl Pts',(7.65711471769406,22.1300198579671,12.));
#209371=CARTESIAN_POINT('Ctrl Pts',(7.65601030346818,22.1122126563327,0.));
#209372=CARTESIAN_POINT('Ctrl Pts',(7.65601030346818,22.1122126563327,12.));
#209373=CARTESIAN_POINT('Ctrl Pts',(7.6548633426365,22.094534754469,0.));
#209374=CARTESIAN_POINT('Ctrl Pts',(7.6548633426365,22.094534754469,12.));
#209375=CARTESIAN_POINT('Ctrl Pts',(7.65367447254944,22.0769872951596,0.));
#209376=CARTESIAN_POINT('Ctrl Pts',(7.65367447254944,22.0769872951596,12.));
#209377=CARTESIAN_POINT('Ctrl Pts',(7.65244434253103,22.0595714384432,0.));
#209378=CARTESIAN_POINT('Ctrl Pts',(7.65244434253103,22.0595714384432,12.));
#209379=CARTESIAN_POINT('Ctrl Pts',(7.65117361421346,22.0422883621176,0.));
#209380=CARTESIAN_POINT('Ctrl Pts',(7.65117361421346,22.0422883621176,12.));
#209381=CARTESIAN_POINT('Ctrl Pts',(7.64986296190156,22.025139262321,0.));
#209382=CARTESIAN_POINT('Ctrl Pts',(7.64986296190156,22.025139262321,12.));
#209383=CARTESIAN_POINT('Ctrl Pts',(7.64851307293345,22.0081253540774,0.));
#209384=CARTESIAN_POINT('Ctrl Pts',(7.64851307293345,22.0081253540774,12.));
#209385=CARTESIAN_POINT('Ctrl Pts',(7.64712464805257,21.9912478718542,0.));
#209386=CARTESIAN_POINT('Ctrl Pts',(7.64712464805257,21.9912478718542,12.));
#209387=CARTESIAN_POINT('Ctrl Pts',(7.64569840177359,21.97450807008,0.));
#209388=CARTESIAN_POINT('Ctrl Pts',(7.64569840177359,21.97450807008,12.));
#209389=CARTESIAN_POINT('Ctrl Pts',(7.64423506279153,21.9579072237653,0.));
#209390=CARTESIAN_POINT('Ctrl Pts',(7.64423506279153,21.9579072237653,12.));
#209391=CARTESIAN_POINT('Ctrl Pts',(7.64273537442706,21.9414466292074,0.));
#209392=CARTESIAN_POINT('Ctrl Pts',(7.64273537442706,21.9414466292074,12.));
#209393=CARTESIAN_POINT('Ctrl Pts',(7.64120009506539,21.9251276046546,0.));
#209394=CARTESIAN_POINT('Ctrl Pts',(7.64120009506539,21.9251276046546,12.));
#209395=CARTESIAN_POINT('Ctrl Pts',(7.63962999860916,21.9089514909873,0.));
#209396=CARTESIAN_POINT('Ctrl Pts',(7.63962999860916,21.9089514909873,12.));
#209397=CARTESIAN_POINT('Ctrl Pts',(7.63802587492007,21.8929196523511,0.));
#209398=CARTESIAN_POINT('Ctrl Pts',(7.63802587492007,21.8929196523511,12.));
#209399=CARTESIAN_POINT('Ctrl Pts',(7.63638853033367,21.8770334769492,0.));
#209400=CARTESIAN_POINT('Ctrl Pts',(7.63638853033367,21.8770334769492,12.));
#209401=CARTESIAN_POINT('Ctrl Pts',(7.63471878821203,21.8612943779086,0.));
#209402=CARTESIAN_POINT('Ctrl Pts',(7.63471878821203,21.8612943779086,12.));
#209403=CARTESIAN_POINT('Ctrl Pts',(7.63301748948936,21.8457037941084,0.));
#209404=CARTESIAN_POINT('Ctrl Pts',(7.63301748948936,21.8457037941084,12.));
#209405=CARTESIAN_POINT('Ctrl Pts',(7.6312854932304,21.8302631910197,0.));
#209406=CARTESIAN_POINT('Ctrl Pts',(7.6312854932304,21.8302631910197,12.));
#209407=CARTESIAN_POINT('Ctrl Pts',(7.62952367718151,21.8149740615093,0.));
#209408=CARTESIAN_POINT('Ctrl Pts',(7.62952367718151,21.8149740615093,12.));
#209409=CARTESIAN_POINT('Ctrl Pts',(7.62773293842409,21.7998379268583,0.));
#209410=CARTESIAN_POINT('Ctrl Pts',(7.62773293842409,21.7998379268583,12.));
#209411=CARTESIAN_POINT('Ctrl Pts',(7.6259141940452,21.7848563378022,0.));
#209412=CARTESIAN_POINT('Ctrl Pts',(7.6259141940452,21.7848563378022,12.));
#209413=CARTESIAN_POINT('Ctrl Pts',(7.62406838181164,21.7700308755584,0.));
#209414=CARTESIAN_POINT('Ctrl Pts',(7.62406838181164,21.7700308755584,12.));
#209415=CARTESIAN_POINT('Ctrl Pts',(7.62219646084225,21.7553631528329,0.));
#209416=CARTESIAN_POINT('Ctrl Pts',(7.62219646084225,21.7553631528329,12.));
#209417=CARTESIAN_POINT('Ctrl Pts',(7.62029941230854,21.7408548148657,0.));
#209418=CARTESIAN_POINT('Ctrl Pts',(7.62029941230854,21.7408548148657,12.));
#209419=CARTESIAN_POINT('Ctrl Pts',(7.61837824030541,21.7265075407977,0.));
#209420=CARTESIAN_POINT('Ctrl Pts',(7.61837824030541,21.7265075407977,12.));
#209421=CARTESIAN_POINT('Ctrl Pts',(7.61643397270424,21.7123230449835,0.));
#209422=CARTESIAN_POINT('Ctrl Pts',(7.61643397270424,21.7123230449835,12.));
#209423=CARTESIAN_POINT('Ctrl Pts',(7.61446766202786,21.6983030783321,0.));
#209424=CARTESIAN_POINT('Ctrl Pts',(7.61446766202786,21.6983030783321,12.));
#209425=CARTESIAN_POINT('Ctrl Pts',(7.61248038630264,21.6844494295813,0.));
#209426=CARTESIAN_POINT('Ctrl Pts',(7.61248038630264,21.6844494295813,12.));
#209427=CARTESIAN_POINT('Ctrl Pts',(7.61047325000949,21.6707639267573,0.));
#209428=CARTESIAN_POINT('Ctrl Pts',(7.61047325000949,21.6707639267573,12.));
#209429=CARTESIAN_POINT('Ctrl Pts',(7.60844738512871,21.6572484388079,0.));
#209430=CARTESIAN_POINT('Ctrl Pts',(7.60844738512871,21.6572484388079,12.));
#209431=CARTESIAN_POINT('Ctrl Pts',(7.60640395216358,21.6439048771743,0.));
#209432=CARTESIAN_POINT('Ctrl Pts',(7.60640395216358,21.6439048771743,12.));
#209433=CARTESIAN_POINT('Ctrl Pts',(7.60434414118299,21.6307351973823,0.));
#209434=CARTESIAN_POINT('Ctrl Pts',(7.60434414118299,21.6307351973823,12.));
#209435=CARTESIAN_POINT('Ctrl Pts',(7.60226917285431,21.6177414005991,0.));
#209436=CARTESIAN_POINT('Ctrl Pts',(7.60226917285431,21.6177414005991,12.));
#209437=CARTESIAN_POINT('Ctrl Pts',(7.60018029988238,21.6049255358843,0.));
#209438=CARTESIAN_POINT('Ctrl Pts',(7.60018029988238,21.6049255358843,12.));
#209439=CARTESIAN_POINT('Ctrl Pts',(7.59807880846192,21.5922897024466,0.));
#209440=CARTESIAN_POINT('Ctrl Pts',(7.59807880846192,21.5922897024466,12.));
#209441=CARTESIAN_POINT('Ctrl Pts',(7.59596601973588,21.5798360518978,0.));
#209442=CARTESIAN_POINT('Ctrl Pts',(7.59596601973588,21.5798360518978,12.));
#209443=CARTESIAN_POINT('Ctrl Pts',(7.59384329124929,21.5675667904728,0.));
#209444=CARTESIAN_POINT('Ctrl Pts',(7.59384329124929,21.5675667904728,12.));
#209445=CARTESIAN_POINT('Ctrl Pts',(7.59171201844792,21.5554841813466,0.));
#209446=CARTESIAN_POINT('Ctrl Pts',(7.59171201844792,21.5554841813466,12.));
#209447=CARTESIAN_POINT('Ctrl Pts',(7.58957363620026,21.5435905470113,0.));
#209448=CARTESIAN_POINT('Ctrl Pts',(7.58957363620026,21.5435905470113,12.));
#209449=CARTESIAN_POINT('Ctrl Pts',(7.58742962034834,21.5318882716736,0.));
#209450=CARTESIAN_POINT('Ctrl Pts',(7.58742962034834,21.5318882716736,12.));
#209451=CARTESIAN_POINT('Ctrl Pts',(7.58528148919113,21.5203798035294,0.));
#209452=CARTESIAN_POINT('Ctrl Pts',(7.58528148919113,21.5203798035294,12.));
#209453=CARTESIAN_POINT('Ctrl Pts',(7.58313080519158,21.5090676573866,0.));
#209454=CARTESIAN_POINT('Ctrl Pts',(7.58313080519158,21.5090676573866,12.));
#209455=CARTESIAN_POINT('Ctrl Pts',(7.58097917790729,21.497954419274,0.));
#209456=CARTESIAN_POINT('Ctrl Pts',(7.58097917790729,21.497954419274,12.));
#209457=CARTESIAN_POINT('Ctrl Pts',(7.57882826679131,21.4870427508193,0.));
#209458=CARTESIAN_POINT('Ctrl Pts',(7.57882826679131,21.4870427508193,12.));
#209459=CARTESIAN_POINT('Ctrl Pts',(7.57667978403001,21.4763353936766,0.));
#209460=CARTESIAN_POINT('Ctrl Pts',(7.57667978403001,21.4763353936766,12.));
#209461=CARTESIAN_POINT('Ctrl Pts',(7.57453549743434,21.4658351740135,0.));
#209462=CARTESIAN_POINT('Ctrl Pts',(7.57453549743434,21.4658351740135,12.));
#209463=CARTESIAN_POINT('Ctrl Pts',(7.57239723223521,21.4555450053147,0.));
#209464=CARTESIAN_POINT('Ctrl Pts',(7.57239723223521,21.4555450053147,12.));
#209465=CARTESIAN_POINT('Ctrl Pts',(7.57026687261169,21.445467890751,0.));
#209466=CARTESIAN_POINT('Ctrl Pts',(7.57026687261169,21.445467890751,12.));
#209467=CARTESIAN_POINT('Ctrl Pts',(7.56814636360841,21.435606926151,0.));
#209468=CARTESIAN_POINT('Ctrl Pts',(7.56814636360841,21.435606926151,12.));
#209469=CARTESIAN_POINT('Ctrl Pts',(7.56603771218706,21.4259653015732,0.));
#209470=CARTESIAN_POINT('Ctrl Pts',(7.56603771218706,21.4259653015732,12.));
#209471=CARTESIAN_POINT('Ctrl Pts',(7.56394299313682,21.4165463106252,0.));
#209472=CARTESIAN_POINT('Ctrl Pts',(7.56394299313682,21.4165463106252,12.));
#209473=CARTESIAN_POINT('Ctrl Pts',(7.56186435703622,21.4073533630364,0.));
#209474=CARTESIAN_POINT('Ctrl Pts',(7.56186435703622,21.4073533630364,12.));
#209475=CARTESIAN_POINT('Ctrl Pts',(7.55980403700614,21.3983899952988,0.));
#209476=CARTESIAN_POINT('Ctrl Pts',(7.55980403700614,21.3983899952988,12.));
#209477=CARTESIAN_POINT('Ctrl Pts',(7.55776435731421,21.3896598842119,0.));
#209478=CARTESIAN_POINT('Ctrl Pts',(7.55776435731421,21.3896598842119,12.));
#209479=CARTESIAN_POINT('Ctrl Pts',(7.55574773403507,21.3811668478933,0.));
#209480=CARTESIAN_POINT('Ctrl Pts',(7.55574773403507,21.3811668478933,12.));
#209481=CARTESIAN_POINT('Ctrl Pts',(7.55375667080031,21.3729148390244,0.));
#209482=CARTESIAN_POINT('Ctrl Pts',(7.55375667080031,21.3729148390244,12.));
#209483=CARTESIAN_POINT('Ctrl Pts',(7.55179375777441,21.3649079431864,0.));
#209484=CARTESIAN_POINT('Ctrl Pts',(7.55179375777441,21.3649079431864,12.));
#209485=CARTESIAN_POINT('Ctrl Pts',(7.54986166521306,21.3571503685853,0.));
#209486=CARTESIAN_POINT('Ctrl Pts',(7.54986166521306,21.3571503685853,12.));
#209487=CARTESIAN_POINT('Ctrl Pts',(7.54796316246326,21.349646476153,0.));
#209488=CARTESIAN_POINT('Ctrl Pts',(7.54796316246326,21.349646476153,12.));
#209489=CARTESIAN_POINT('Ctrl Pts',(7.5461011494835,21.3424008295038,0.));
#209490=CARTESIAN_POINT('Ctrl Pts',(7.5461011494835,21.3424008295038,12.));
#209491=CARTESIAN_POINT('Ctrl Pts',(7.54427868151268,21.3354182340149,0.));
#209492=CARTESIAN_POINT('Ctrl Pts',(7.54427868151268,21.3354182340149,12.));
#209493=CARTESIAN_POINT('Ctrl Pts',(7.54249900377031,21.328703791771,0.));
#209494=CARTESIAN_POINT('Ctrl Pts',(7.54249900377031,21.328703791771,12.));
#209495=CARTESIAN_POINT('Ctrl Pts',(7.54076552038279,21.3222628524165,0.));
#209496=CARTESIAN_POINT('Ctrl Pts',(7.54076552038279,21.3222628524165,12.));
#209497=CARTESIAN_POINT('Ctrl Pts',(7.53908175169898,21.3161009456256,0.));
#209498=CARTESIAN_POINT('Ctrl Pts',(7.53908175169898,21.3161009456256,12.));
#209499=CARTESIAN_POINT('Ctrl Pts',(7.53745129364619,21.3102237167729,0.));
#209500=CARTESIAN_POINT('Ctrl Pts',(7.53745129364619,21.3102237167729,12.));
#209501=CARTESIAN_POINT('Ctrl Pts',(7.53587778251743,21.3046368712157,0.));
#209502=CARTESIAN_POINT('Ctrl Pts',(7.53587778251743,21.3046368712157,12.));
#209503=CARTESIAN_POINT('Ctrl Pts',(7.53436505309948,21.2993464250717,0.));
#209504=CARTESIAN_POINT('Ctrl Pts',(7.53436505309948,21.2993464250717,12.));
#209505=CARTESIAN_POINT('Ctrl Pts',(7.53291726078526,21.2943588989331,0.));
#209506=CARTESIAN_POINT('Ctrl Pts',(7.53291726078526,21.2943588989331,12.));
#209507=CARTESIAN_POINT('Ctrl Pts',(7.53153906987846,21.2896816163843,0.));
#209508=CARTESIAN_POINT('Ctrl Pts',(7.53153906987846,21.2896816163843,12.));
#209509=CARTESIAN_POINT('Ctrl Pts',(7.5302356243822,21.2853226580658,0.));
#209510=CARTESIAN_POINT('Ctrl Pts',(7.5302356243822,21.2853226580658,12.));
#209511=CARTESIAN_POINT('Ctrl Pts',(7.52901217930407,21.2812902781143,0.));
#209512=CARTESIAN_POINT('Ctrl Pts',(7.52901217930407,21.2812902781143,12.));
#209513=CARTESIAN_POINT('Ctrl Pts',(7.52787386225343,21.2775925269652,0.));
#209514=CARTESIAN_POINT('Ctrl Pts',(7.52787386225343,21.2775925269652,12.));
#209515=CARTESIAN_POINT('Ctrl Pts',(7.5268252691856,21.2742366113578,0.));
#209516=CARTESIAN_POINT('Ctrl Pts',(7.5268252691856,21.2742366113578,12.));
#209517=CARTESIAN_POINT('Ctrl Pts',(7.52587126095544,21.2712301573465,0.));
#209518=CARTESIAN_POINT('Ctrl Pts',(7.52587126095544,21.2712301573465,12.));
#209519=CARTESIAN_POINT('Ctrl Pts',(7.52501770333521,21.2685823838672,0.));
#209520=CARTESIAN_POINT('Ctrl Pts',(7.52501770333521,21.2685823838672,12.));
#209521=CARTESIAN_POINT('Ctrl Pts',(7.52427261074263,21.266305915706,0.));
#209522=CARTESIAN_POINT('Ctrl Pts',(7.52427261074263,21.266305915706,12.));
#209523=CARTESIAN_POINT('Ctrl Pts',(7.52364573027521,21.2644161259965,0.));
#209524=CARTESIAN_POINT('Ctrl Pts',(7.52364573027521,21.2644161259965,12.));
#209525=CARTESIAN_POINT('Ctrl Pts',(7.52314642316202,21.262927782038,0.));
#209526=CARTESIAN_POINT('Ctrl Pts',(7.52314642316202,21.262927782038,12.));
#209527=CARTESIAN_POINT('Ctrl Pts',(7.52278182242727,21.261852128355,0.));
#209528=CARTESIAN_POINT('Ctrl Pts',(7.52278182242727,21.261852128355,12.));
#209529=CARTESIAN_POINT('Ctrl Pts',(7.52260064231736,21.2613260540651,0.));
#209530=CARTESIAN_POINT('Ctrl Pts',(7.52260064231736,21.2613260540651,12.));
#209531=CARTESIAN_POINT('Ctrl Pts',(7.52252744144957,21.261120447486,0.));
#209532=CARTESIAN_POINT('Ctrl Pts',(7.52252744144957,21.261120447486,12.));
#209533=CARTESIAN_POINT('Ctrl Pts',(7.52250649703991,21.2610673466883,0.));
#209534=CARTESIAN_POINT('Ctrl Pts',(7.52250649703991,21.2610673466883,12.));
#209535=CARTESIAN_POINT('Ctrl Pts',(7.52250298901265,21.2610617890679,0.));
#209536=CARTESIAN_POINT('Ctrl Pts',(7.52250298901265,21.2610617890679,12.));
#209537=CARTESIAN_POINT('',(7.36589684767344,24.9347862158358,0.));
#209538=CARTESIAN_POINT('Ctrl Pts',(7.36589684767344,24.9347862158358,0.));
#209539=CARTESIAN_POINT('Ctrl Pts',(7.36721909028842,24.9292275670674,0.));
#209540=CARTESIAN_POINT('Ctrl Pts',(7.3698559312009,24.9181155530543,0.));
#209541=CARTESIAN_POINT('Ctrl Pts',(7.37378825961676,24.901463382605,0.));
#209542=CARTESIAN_POINT('Ctrl Pts',(7.37898549640269,24.8792921911115,0.));
#209543=CARTESIAN_POINT('Ctrl Pts',(7.3854055890362,24.8516310625176,0.));
#209544=CARTESIAN_POINT('Ctrl Pts',(7.39174922585808,24.8240228520893,0.));
#209545=CARTESIAN_POINT('Ctrl Pts',(7.39801641583012,24.7964676646431,0.));
#209546=CARTESIAN_POINT('Ctrl Pts',(7.40420718661602,24.7689656668983,0.));
#209547=CARTESIAN_POINT('Ctrl Pts',(7.41032159082381,24.7415170994784,0.));
#209548=CARTESIAN_POINT('Ctrl Pts',(7.41635971481674,24.7141222950051,0.));
#209549=CARTESIAN_POINT('Ctrl Pts',(7.42232167766265,24.6867816727192,0.));
#209550=CARTESIAN_POINT('Ctrl Pts',(7.42820762159125,24.6594957128756,0.));
#209551=CARTESIAN_POINT('Ctrl Pts',(7.43401770489523,24.6322649369517,0.));
#209552=CARTESIAN_POINT('Ctrl Pts',(7.43975209375503,24.6050898852368,0.));
#209553=CARTESIAN_POINT('Ctrl Pts',(7.44541095473134,24.577971096086,0.));
#209554=CARTESIAN_POINT('Ctrl Pts',(7.4509944465116,24.5509090831559,0.));
#209555=CARTESIAN_POINT('Ctrl Pts',(7.45650271335861,24.5239043173072,0.));
#209556=CARTESIAN_POINT('Ctrl Pts',(7.46193588961463,24.4969572391483,0.));
#209557=CARTESIAN_POINT('Ctrl Pts',(7.46729410308786,24.4700682684524,0.));
#209558=CARTESIAN_POINT('Ctrl Pts',(7.47257747883246,24.443237814649,0.));
#209559=CARTESIAN_POINT('Ctrl Pts',(7.47778614286564,24.4164662871163,0.));
#209560=CARTESIAN_POINT('Ctrl Pts',(7.482920225693,24.3897541049254,0.));
#209561=CARTESIAN_POINT('Ctrl Pts',(7.48797986651908,24.3631017084524,0.));
#209562=CARTESIAN_POINT('Ctrl Pts',(7.4929652125242,24.3365095573685,0.));
#209563=CARTESIAN_POINT('Ctrl Pts',(7.49787641695438,24.3099781253355,0.));
#209564=CARTESIAN_POINT('Ctrl Pts',(7.50271363765151,24.2835078958973,0.));
#209565=CARTESIAN_POINT('Ctrl Pts',(7.50747703535133,24.2570993577034,0.));
#209566=CARTESIAN_POINT('Ctrl Pts',(7.5121667722218,24.2307530003887,0.));
#209567=CARTESIAN_POINT('Ctrl Pts',(7.51678300997949,24.2044693092349,0.));
#209568=CARTESIAN_POINT('Ctrl Pts',(7.52132590953801,24.1782487641594,0.));
#209569=CARTESIAN_POINT('Ctrl Pts',(7.52579563201423,24.1520918425364,0.));
#209570=CARTESIAN_POINT('Ctrl Pts',(7.53019233935501,24.1259990209207,0.));
#209571=CARTESIAN_POINT('Ctrl Pts',(7.53451619514649,24.0999707772642,0.));
#209572=CARTESIAN_POINT('Ctrl Pts',(7.53876736531013,24.0740075927985,0.));
#209573=CARTESIAN_POINT('Ctrl Pts',(7.54294601896144,24.0481099543353,0.));
#209574=CARTESIAN_POINT('Ctrl Pts',(7.5470523288591,24.022278355453,0.));
#209575=CARTESIAN_POINT('Ctrl Pts',(7.5510864709744,23.9965132953185,0.));
#209576=CARTESIAN_POINT('Ctrl Pts',(7.55504862424811,23.9708152779884,0.));
#209577=CARTESIAN_POINT('Ctrl Pts',(7.55893897027682,23.9451848115,0.));
#209578=CARTESIAN_POINT('Ctrl Pts',(7.56275769304773,23.9196224070759,0.));
#209579=CARTESIAN_POINT('Ctrl Pts',(7.56650497863791,23.8941285782003,0.));
#209580=CARTESIAN_POINT('Ctrl Pts',(7.5701810150071,23.8687038399598,0.));
#209581=CARTESIAN_POINT('Ctrl Pts',(7.57378599219816,23.8433487096134,0.));
#209582=CARTESIAN_POINT('Ctrl Pts',(7.57732010249065,23.8180637069977,0.));
#209583=CARTESIAN_POINT('Ctrl Pts',(7.58078354058211,23.7928493549908,0.));
#209584=CARTESIAN_POINT('Ctrl Pts',(7.58417650376271,23.7677061799376,0.));
#209585=CARTESIAN_POINT('Ctrl Pts',(7.58749919210831,23.7426347121006,0.));
#209586=CARTESIAN_POINT('Ctrl Pts',(7.59075180865326,23.7176354860457,0.));
#209587=CARTESIAN_POINT('Ctrl Pts',(7.59393455934041,23.6927090405067,0.));
#209588=CARTESIAN_POINT('Ctrl Pts',(7.59704765299572,23.6678559182876,0.));
#209589=CARTESIAN_POINT('Ctrl Pts',(7.60009130130129,23.6430766661419,0.));
#209590=CARTESIAN_POINT('Ctrl Pts',(7.60306571877806,23.6183718346576,0.));
#209591=CARTESIAN_POINT('Ctrl Pts',(7.60597112277094,23.5937419781244,0.));
#209592=CARTESIAN_POINT('Ctrl Pts',(7.60880773344599,23.5691876544243,0.));
#209593=CARTESIAN_POINT('Ctrl Pts',(7.61157577385371,23.5447094252029,0.));
#209594=CARTESIAN_POINT('Ctrl Pts',(7.61427546999298,23.5203078560128,0.));
#209595=CARTESIAN_POINT('Ctrl Pts',(7.61690705088318,23.4959835164608,0.));
#209596=CARTESIAN_POINT('Ctrl Pts',(7.61947074863977,23.4717369803438,0.));
#209597=CARTESIAN_POINT('Ctrl Pts',(7.62196679855957,23.4475688257855,0.));
#209598=CARTESIAN_POINT('Ctrl Pts',(7.62439543920053,23.4234796353544,0.));
#209599=CARTESIAN_POINT('Ctrl Pts',(7.62675691240334,23.3994699961122,0.));
#209600=CARTESIAN_POINT('Ctrl Pts',(7.62905146332597,23.3755404996638,0.));
#209601=CARTESIAN_POINT('Ctrl Pts',(7.63127934048138,23.3516917421973,0.));
#209602=CARTESIAN_POINT('Ctrl Pts',(7.63344079578162,23.3279243245241,0.));
#209603=CARTESIAN_POINT('Ctrl Pts',(7.63553608458783,23.3042388521021,0.));
#209604=CARTESIAN_POINT('Ctrl Pts',(7.63756546576374,23.2806359350853,0.));
#209605=CARTESIAN_POINT('Ctrl Pts',(7.63952920172837,23.2571161884487,0.));
#209606=CARTESIAN_POINT('Ctrl Pts',(7.64142755851507,23.2336802320912,0.));
#209607=CARTESIAN_POINT('Ctrl Pts',(7.64326080583683,23.2103286909399,0.));
#209608=CARTESIAN_POINT('Ctrl Pts',(7.64502921715482,23.1870621950452,0.));
#209609=CARTESIAN_POINT('Ctrl Pts',(7.64673306975796,23.1638813796691,0.));
#209610=CARTESIAN_POINT('Ctrl Pts',(7.64837264482929,23.1407868853815,0.));
#209611=CARTESIAN_POINT('Ctrl Pts',(7.64994822749844,23.1177793581674,0.));
#209612=CARTESIAN_POINT('Ctrl Pts',(7.65146010690464,23.0948594495246,0.));
#209613=CARTESIAN_POINT('Ctrl Pts',(7.65290857626356,23.072027816555,0.));
#209614=CARTESIAN_POINT('Ctrl Pts',(7.65429393293955,23.049285122053,0.));
#209615=CARTESIAN_POINT('Ctrl Pts',(7.65561647852554,23.0266320345792,0.));
#209616=CARTESIAN_POINT('Ctrl Pts',(7.6568765189133,23.004069228582,0.));
#209617=CARTESIAN_POINT('Ctrl Pts',(7.65807436436452,22.9815973845301,0.));
#209618=CARTESIAN_POINT('Ctrl Pts',(7.65921032958911,22.9592171890332,0.));
#209619=CARTESIAN_POINT('Ctrl Pts',(7.66028473382776,22.9369293349592,0.));
#209620=CARTESIAN_POINT('Ctrl Pts',(7.66129790094099,22.9147345215418,0.));
#209621=CARTESIAN_POINT('Ctrl Pts',(7.66225015950147,22.8926334544879,0.));
#209622=CARTESIAN_POINT('Ctrl Pts',(7.66314184287333,22.870626846128,0.));
#209623=CARTESIAN_POINT('Ctrl Pts',(7.66397328929805,22.8487154155569,0.));
#209624=CARTESIAN_POINT('Ctrl Pts',(7.66474484198552,22.8268998887679,0.));
#209625=CARTESIAN_POINT('Ctrl Pts',(7.66545684920987,22.8051809987834,0.));
#209626=CARTESIAN_POINT('Ctrl Pts',(7.66610966441259,22.7835594857697,0.));
#209627=CARTESIAN_POINT('Ctrl Pts',(7.66670364630273,22.7620360971839,0.));
#209628=CARTESIAN_POINT('Ctrl Pts',(7.66723915895412,22.7406115879508,0.));
#209629=CARTESIAN_POINT('Ctrl Pts',(7.6677165719101,22.7192867206242,0.));
#209630=CARTESIAN_POINT('Ctrl Pts',(7.66813626029276,22.6980622655446,0.));
#209631=CARTESIAN_POINT('Ctrl Pts',(7.66849860491762,22.6769390009889,0.));
#209632=CARTESIAN_POINT('Ctrl Pts',(7.66880399241353,22.6559177133133,0.));
#209633=CARTESIAN_POINT('Ctrl Pts',(7.66905281533744,22.6349991971548,0.));
#209634=CARTESIAN_POINT('Ctrl Pts',(7.66924547229434,22.6141842556248,0.));
#209635=CARTESIAN_POINT('Ctrl Pts',(7.6693823680624,22.5934737004955,0.));
#209636=CARTESIAN_POINT('Ctrl Pts',(7.66946391372299,22.5728683523829,0.));
#209637=CARTESIAN_POINT('Ctrl Pts',(7.66949052679671,22.5523690409109,0.));
#209638=CARTESIAN_POINT('Ctrl Pts',(7.66946263138115,22.5319766049191,0.));
#209639=CARTESIAN_POINT('Ctrl Pts',(7.66938065829082,22.5116918927023,0.));
#209640=CARTESIAN_POINT('Ctrl Pts',(7.66924504520301,22.4915157622308,0.));
#209641=CARTESIAN_POINT('Ctrl Pts',(7.66905623680835,22.47144908137,0.));
#209642=CARTESIAN_POINT('Ctrl Pts',(7.66881468496659,22.4514927280863,0.));
#209643=CARTESIAN_POINT('Ctrl Pts',(7.66852084886745,22.4316475906616,0.));
#209644=CARTESIAN_POINT('Ctrl Pts',(7.66817519519681,22.411914567977,0.));
#209645=CARTESIAN_POINT('Ctrl Pts',(7.66777819830819,22.3922945697782,0.));
#209646=CARTESIAN_POINT('Ctrl Pts',(7.66733034039887,22.3727885169361,0.));
#209647=CARTESIAN_POINT('Ctrl Pts',(7.66683211169133,22.3533973417013,0.));
#209648=CARTESIAN_POINT('Ctrl Pts',(7.66628401061905,22.3341219879454,0.));
#209649=CARTESIAN_POINT('Ctrl Pts',(7.66568654402441,22.3149634114823,0.));
#209650=CARTESIAN_POINT('Ctrl Pts',(7.66504022736262,22.2959225803925,0.));
#209651=CARTESIAN_POINT('Ctrl Pts',(7.66434558490972,22.2770004753332,0.));
#209652=CARTESIAN_POINT('Ctrl Pts',(7.66360314997661,22.2581980898487,0.));
#209653=CARTESIAN_POINT('Ctrl Pts',(7.66281346512545,22.239516430656,0.));
#209654=CARTESIAN_POINT('Ctrl Pts',(7.66197708240435,22.2209565180098,0.));
#209655=CARTESIAN_POINT('Ctrl Pts',(7.66109456359292,22.2025193860972,0.));
#209656=CARTESIAN_POINT('Ctrl Pts',(7.66016648045007,22.1842060834093,0.));
#209657=CARTESIAN_POINT('Ctrl Pts',(7.65919341496925,22.1660176731174,0.));
#209658=CARTESIAN_POINT('Ctrl Pts',(7.6581759596335,22.1479552334206,0.));
#209659=CARTESIAN_POINT('Ctrl Pts',(7.65711471769406,22.1300198579671,0.));
#209660=CARTESIAN_POINT('Ctrl Pts',(7.65601030346818,22.1122126563327,0.));
#209661=CARTESIAN_POINT('Ctrl Pts',(7.6548633426365,22.094534754469,0.));
#209662=CARTESIAN_POINT('Ctrl Pts',(7.65367447254944,22.0769872951596,0.));
#209663=CARTESIAN_POINT('Ctrl Pts',(7.65244434253103,22.0595714384432,0.));
#209664=CARTESIAN_POINT('Ctrl Pts',(7.65117361421346,22.0422883621176,0.));
#209665=CARTESIAN_POINT('Ctrl Pts',(7.64986296190156,22.025139262321,0.));
#209666=CARTESIAN_POINT('Ctrl Pts',(7.64851307293345,22.0081253540774,0.));
#209667=CARTESIAN_POINT('Ctrl Pts',(7.64712464805257,21.9912478718542,0.));
#209668=CARTESIAN_POINT('Ctrl Pts',(7.64569840177359,21.97450807008,0.));
#209669=CARTESIAN_POINT('Ctrl Pts',(7.64423506279153,21.9579072237653,0.));
#209670=CARTESIAN_POINT('Ctrl Pts',(7.64273537442706,21.9414466292074,0.));
#209671=CARTESIAN_POINT('Ctrl Pts',(7.64120009506539,21.9251276046546,0.));
#209672=CARTESIAN_POINT('Ctrl Pts',(7.63962999860916,21.9089514909873,0.));
#209673=CARTESIAN_POINT('Ctrl Pts',(7.63802587492007,21.8929196523511,0.));
#209674=CARTESIAN_POINT('Ctrl Pts',(7.63638853033367,21.8770334769492,0.));
#209675=CARTESIAN_POINT('Ctrl Pts',(7.63471878821203,21.8612943779086,0.));
#209676=CARTESIAN_POINT('Ctrl Pts',(7.63301748948936,21.8457037941084,0.));
#209677=CARTESIAN_POINT('Ctrl Pts',(7.6312854932304,21.8302631910197,0.));
#209678=CARTESIAN_POINT('Ctrl Pts',(7.62952367718151,21.8149740615093,0.));
#209679=CARTESIAN_POINT('Ctrl Pts',(7.62773293842409,21.7998379268583,0.));
#209680=CARTESIAN_POINT('Ctrl Pts',(7.6259141940452,21.7848563378022,0.));
#209681=CARTESIAN_POINT('Ctrl Pts',(7.62406838181164,21.7700308755584,0.));
#209682=CARTESIAN_POINT('Ctrl Pts',(7.62219646084225,21.7553631528329,0.));
#209683=CARTESIAN_POINT('Ctrl Pts',(7.62029941230854,21.7408548148657,0.));
#209684=CARTESIAN_POINT('Ctrl Pts',(7.61837824030541,21.7265075407977,0.));
#209685=CARTESIAN_POINT('Ctrl Pts',(7.61643397270424,21.7123230449835,0.));
#209686=CARTESIAN_POINT('Ctrl Pts',(7.61446766202786,21.6983030783321,0.));
#209687=CARTESIAN_POINT('Ctrl Pts',(7.61248038630264,21.6844494295813,0.));
#209688=CARTESIAN_POINT('Ctrl Pts',(7.61047325000949,21.6707639267573,0.));
#209689=CARTESIAN_POINT('Ctrl Pts',(7.60844738512871,21.6572484388079,0.));
#209690=CARTESIAN_POINT('Ctrl Pts',(7.60640395216358,21.6439048771743,0.));
#209691=CARTESIAN_POINT('Ctrl Pts',(7.60434414118299,21.6307351973823,0.));
#209692=CARTESIAN_POINT('Ctrl Pts',(7.60226917285431,21.6177414005991,0.));
#209693=CARTESIAN_POINT('Ctrl Pts',(7.60018029988238,21.6049255358843,0.));
#209694=CARTESIAN_POINT('Ctrl Pts',(7.59807880846192,21.5922897024466,0.));
#209695=CARTESIAN_POINT('Ctrl Pts',(7.59596601973588,21.5798360518978,0.));
#209696=CARTESIAN_POINT('Ctrl Pts',(7.59384329124929,21.5675667904728,0.));
#209697=CARTESIAN_POINT('Ctrl Pts',(7.59171201844792,21.5554841813466,0.));
#209698=CARTESIAN_POINT('Ctrl Pts',(7.58957363620026,21.5435905470113,0.));
#209699=CARTESIAN_POINT('Ctrl Pts',(7.58742962034834,21.5318882716736,0.));
#209700=CARTESIAN_POINT('Ctrl Pts',(7.58528148919113,21.5203798035294,0.));
#209701=CARTESIAN_POINT('Ctrl Pts',(7.58313080519158,21.5090676573866,0.));
#209702=CARTESIAN_POINT('Ctrl Pts',(7.58097917790729,21.497954419274,0.));
#209703=CARTESIAN_POINT('Ctrl Pts',(7.57882826679131,21.4870427508193,0.));
#209704=CARTESIAN_POINT('Ctrl Pts',(7.57667978403001,21.4763353936766,0.));
#209705=CARTESIAN_POINT('Ctrl Pts',(7.57453549743434,21.4658351740135,0.));
#209706=CARTESIAN_POINT('Ctrl Pts',(7.57239723223521,21.4555450053147,0.));
#209707=CARTESIAN_POINT('Ctrl Pts',(7.57026687261169,21.445467890751,0.));
#209708=CARTESIAN_POINT('Ctrl Pts',(7.56814636360841,21.435606926151,0.));
#209709=CARTESIAN_POINT('Ctrl Pts',(7.56603771218706,21.4259653015732,0.));
#209710=CARTESIAN_POINT('Ctrl Pts',(7.56394299313682,21.4165463106252,0.));
#209711=CARTESIAN_POINT('Ctrl Pts',(7.56186435703622,21.4073533630364,0.));
#209712=CARTESIAN_POINT('Ctrl Pts',(7.55980403700614,21.3983899952988,0.));
#209713=CARTESIAN_POINT('Ctrl Pts',(7.55776435731421,21.3896598842119,0.));
#209714=CARTESIAN_POINT('Ctrl Pts',(7.55574773403507,21.3811668478933,0.));
#209715=CARTESIAN_POINT('Ctrl Pts',(7.55375667080031,21.3729148390244,0.));
#209716=CARTESIAN_POINT('Ctrl Pts',(7.55179375777441,21.3649079431864,0.));
#209717=CARTESIAN_POINT('Ctrl Pts',(7.54986166521306,21.3571503685853,0.));
#209718=CARTESIAN_POINT('Ctrl Pts',(7.54796316246326,21.349646476153,0.));
#209719=CARTESIAN_POINT('Ctrl Pts',(7.5461011494835,21.3424008295038,0.));
#209720=CARTESIAN_POINT('Ctrl Pts',(7.54427868151268,21.3354182340149,0.));
#209721=CARTESIAN_POINT('Ctrl Pts',(7.54249900377031,21.328703791771,0.));
#209722=CARTESIAN_POINT('Ctrl Pts',(7.54076552038279,21.3222628524165,0.));
#209723=CARTESIAN_POINT('Ctrl Pts',(7.53908175169898,21.3161009456256,0.));
#209724=CARTESIAN_POINT('Ctrl Pts',(7.53745129364619,21.3102237167729,0.));
#209725=CARTESIAN_POINT('Ctrl Pts',(7.53587778251743,21.3046368712157,0.));
#209726=CARTESIAN_POINT('Ctrl Pts',(7.53436505309948,21.2993464250717,0.));
#209727=CARTESIAN_POINT('Ctrl Pts',(7.53291726078526,21.2943588989331,0.));
#209728=CARTESIAN_POINT('Ctrl Pts',(7.53153906987846,21.2896816163843,0.));
#209729=CARTESIAN_POINT('Ctrl Pts',(7.5302356243822,21.2853226580658,0.));
#209730=CARTESIAN_POINT('Ctrl Pts',(7.52901217930407,21.2812902781143,0.));
#209731=CARTESIAN_POINT('Ctrl Pts',(7.52787386225343,21.2775925269652,0.));
#209732=CARTESIAN_POINT('Ctrl Pts',(7.5268252691856,21.2742366113578,0.));
#209733=CARTESIAN_POINT('Ctrl Pts',(7.52587126095544,21.2712301573465,0.));
#209734=CARTESIAN_POINT('Ctrl Pts',(7.52501770333521,21.2685823838672,0.));
#209735=CARTESIAN_POINT('Ctrl Pts',(7.52427261074263,21.266305915706,0.));
#209736=CARTESIAN_POINT('Ctrl Pts',(7.52364573027521,21.2644161259965,0.));
#209737=CARTESIAN_POINT('Ctrl Pts',(7.52314642316202,21.262927782038,0.));
#209738=CARTESIAN_POINT('Ctrl Pts',(7.52278182242727,21.261852128355,0.));
#209739=CARTESIAN_POINT('Ctrl Pts',(7.52260064231736,21.2613260540651,0.));
#209740=CARTESIAN_POINT('Ctrl Pts',(7.52252744144957,21.261120447486,0.));
#209741=CARTESIAN_POINT('Ctrl Pts',(7.52250649703991,21.2610673466883,0.));
#209742=CARTESIAN_POINT('Ctrl Pts',(7.52250298901265,21.2610617890679,0.));
#209743=CARTESIAN_POINT('',(7.36589684767344,24.9347862158358,0.));
#209744=CARTESIAN_POINT('Ctrl Pts',(9.71462809124917,20.353053841303,0.));
#209745=CARTESIAN_POINT('Ctrl Pts',(9.71462809124917,20.353053841303,12.));
#209746=CARTESIAN_POINT('Ctrl Pts',(9.71462954053074,20.353060251684,0.));
#209747=CARTESIAN_POINT('Ctrl Pts',(9.71462954053074,20.353060251684,12.));
#209748=CARTESIAN_POINT('Ctrl Pts',(9.71465227853122,20.3531126095522,0.));
#209749=CARTESIAN_POINT('Ctrl Pts',(9.71465227853122,20.3531126095522,12.));
#209750=CARTESIAN_POINT('Ctrl Pts',(9.71474590350791,20.3533097561886,0.));
#209751=CARTESIAN_POINT('Ctrl Pts',(9.71474590350791,20.3533097561886,12.));
#209752=CARTESIAN_POINT('Ctrl Pts',(9.714989780521,20.3538098605706,0.));
#209753=CARTESIAN_POINT('Ctrl Pts',(9.714989780521,20.3538098605706,12.));
#209754=CARTESIAN_POINT('Ctrl Pts',(9.71549257088174,20.3548282742361,0.));
#209755=CARTESIAN_POINT('Ctrl Pts',(9.71549257088174,20.3548282742361,12.));
#209756=CARTESIAN_POINT('Ctrl Pts',(9.71619192554146,20.3562337557875,0.));
#209757=CARTESIAN_POINT('Ctrl Pts',(9.71619192554146,20.3562337557875,12.));
#209758=CARTESIAN_POINT('Ctrl Pts',(9.71708493723061,20.3580133103357,0.));
#209759=CARTESIAN_POINT('Ctrl Pts',(9.71708493723061,20.3580133103357,12.));
#209760=CARTESIAN_POINT('Ctrl Pts',(9.71816778327998,20.3601498764344,0.));
#209761=CARTESIAN_POINT('Ctrl Pts',(9.71816778327998,20.3601498764344,12.));
#209762=CARTESIAN_POINT('Ctrl Pts',(9.71943648548114,20.362625691398,0.));
#209763=CARTESIAN_POINT('Ctrl Pts',(9.71943648548114,20.362625691398,12.));
#209764=CARTESIAN_POINT('Ctrl Pts',(9.72088778381101,20.3654261611055,0.));
#209765=CARTESIAN_POINT('Ctrl Pts',(9.72088778381101,20.3654261611055,12.));
#209766=CARTESIAN_POINT('Ctrl Pts',(9.72251930722503,20.3685406190576,0.));
#209767=CARTESIAN_POINT('Ctrl Pts',(9.72251930722503,20.3685406190576,12.));
#209768=CARTESIAN_POINT('Ctrl Pts',(9.72432910043192,20.371960235676,0.));
#209769=CARTESIAN_POINT('Ctrl Pts',(9.72432910043192,20.371960235676,12.));
#209770=CARTESIAN_POINT('Ctrl Pts',(9.7263153173287,20.3756766651952,0.));
#209771=CARTESIAN_POINT('Ctrl Pts',(9.7263153173287,20.3756766651952,12.));
#209772=CARTESIAN_POINT('Ctrl Pts',(9.72847589116532,20.3796805893304,0.));
#209773=CARTESIAN_POINT('Ctrl Pts',(9.72847589116532,20.3796805893304,12.));
#209774=CARTESIAN_POINT('Ctrl Pts',(9.73080870123726,20.3839624556742,0.));
#209775=CARTESIAN_POINT('Ctrl Pts',(9.73080870123726,20.3839624556742,12.));
#209776=CARTESIAN_POINT('Ctrl Pts',(9.73331167102812,20.3885129129912,0.));
#209777=CARTESIAN_POINT('Ctrl Pts',(9.73331167102812,20.3885129129912,12.));
#209778=CARTESIAN_POINT('Ctrl Pts',(9.73598292014249,20.3933234845646,0.));
#209779=CARTESIAN_POINT('Ctrl Pts',(9.73598292014249,20.3933234845646,12.));
#209780=CARTESIAN_POINT('Ctrl Pts',(9.73882077613206,20.3983866213331,0.));
#209781=CARTESIAN_POINT('Ctrl Pts',(9.73882077613206,20.3983866213331,12.));
#209782=CARTESIAN_POINT('Ctrl Pts',(9.74182369656272,20.4036953576549,0.));
#209783=CARTESIAN_POINT('Ctrl Pts',(9.74182369656272,20.4036953576549,12.));
#209784=CARTESIAN_POINT('Ctrl Pts',(9.74499021838536,20.4092430879861,0.));
#209785=CARTESIAN_POINT('Ctrl Pts',(9.74499021838536,20.4092430879861,12.));
#209786=CARTESIAN_POINT('Ctrl Pts',(9.74831889242174,20.4150232777393,0.));
#209787=CARTESIAN_POINT('Ctrl Pts',(9.74831889242174,20.4150232777393,12.));
#209788=CARTESIAN_POINT('Ctrl Pts',(9.75180829786433,20.4210295275818,0.));
#209789=CARTESIAN_POINT('Ctrl Pts',(9.75180829786433,20.4210295275818,12.));
#209790=CARTESIAN_POINT('Ctrl Pts',(9.75545705902416,20.4272556476629,0.));
#209791=CARTESIAN_POINT('Ctrl Pts',(9.75545705902416,20.4272556476629,12.));
#209792=CARTESIAN_POINT('Ctrl Pts',(9.75926386289929,20.4336957355474,0.));
#209793=CARTESIAN_POINT('Ctrl Pts',(9.75926386289929,20.4336957355474,12.));
#209794=CARTESIAN_POINT('Ctrl Pts',(9.76322747195502,20.4403442329401,0.));
#209795=CARTESIAN_POINT('Ctrl Pts',(9.76322747195502,20.4403442329401,12.));
#209796=CARTESIAN_POINT('Ctrl Pts',(9.76734670980896,20.447195862298,0.));
#209797=CARTESIAN_POINT('Ctrl Pts',(9.76734670980896,20.447195862298,12.));
#209798=CARTESIAN_POINT('Ctrl Pts',(9.77162045104069,20.4542455817527,0.));
#209799=CARTESIAN_POINT('Ctrl Pts',(9.77162045104069,20.4542455817527,12.));
#209800=CARTESIAN_POINT('Ctrl Pts',(9.77604760815522,20.4614885274973,0.));
#209801=CARTESIAN_POINT('Ctrl Pts',(9.77604760815522,20.4614885274973,12.));
#209802=CARTESIAN_POINT('Ctrl Pts',(9.78062712373313,20.4689199790668,0.));
#209803=CARTESIAN_POINT('Ctrl Pts',(9.78062712373313,20.4689199790668,12.));
#209804=CARTESIAN_POINT('Ctrl Pts',(9.78535797314162,20.4765353711585,0.));
#209805=CARTESIAN_POINT('Ctrl Pts',(9.78535797314162,20.4765353711585,12.));
#209806=CARTESIAN_POINT('Ctrl Pts',(9.79023916498659,20.4843302955329,0.));
#209807=CARTESIAN_POINT('Ctrl Pts',(9.79023916498659,20.4843302955329,12.));
#209808=CARTESIAN_POINT('Ctrl Pts',(9.79526974288343,20.4923005087945,0.));
#209809=CARTESIAN_POINT('Ctrl Pts',(9.79526974288343,20.4923005087945,12.));
#209810=CARTESIAN_POINT('Ctrl Pts',(9.80044878520967,20.500441931211,0.));
#209811=CARTESIAN_POINT('Ctrl Pts',(9.80044878520967,20.500441931211,12.));
#209812=CARTESIAN_POINT('Ctrl Pts',(9.80577540161102,20.5087506310507,0.));
#209813=CARTESIAN_POINT('Ctrl Pts',(9.80577540161102,20.5087506310507,12.));
#209814=CARTESIAN_POINT('Ctrl Pts',(9.81124873025278,20.5172228122839,0.));
#209815=CARTESIAN_POINT('Ctrl Pts',(9.81124873025278,20.5172228122839,12.));
#209816=CARTESIAN_POINT('Ctrl Pts',(9.81686793455918,20.5258548000625,0.));
#209817=CARTESIAN_POINT('Ctrl Pts',(9.81686793455918,20.5258548000625,12.));
#209818=CARTESIAN_POINT('Ctrl Pts',(9.82263220080327,20.534643029951,0.));
#209819=CARTESIAN_POINT('Ctrl Pts',(9.82263220080327,20.534643029951,12.));
#209820=CARTESIAN_POINT('Ctrl Pts',(9.82854073773857,20.5435840460717,0.));
#209821=CARTESIAN_POINT('Ctrl Pts',(9.82854073773857,20.5435840460717,12.));
#209822=CARTESIAN_POINT('Ctrl Pts',(9.8345927758532,20.5526744976461,0.));
#209823=CARTESIAN_POINT('Ctrl Pts',(9.8345927758532,20.5526744976461,12.));
#209824=CARTESIAN_POINT('Ctrl Pts',(9.84078756677589,20.5619111362406,0.));
#209825=CARTESIAN_POINT('Ctrl Pts',(9.84078756677589,20.5619111362406,12.));
#209826=CARTESIAN_POINT('Ctrl Pts',(9.84712438256308,20.5712908125145,0.));
#209827=CARTESIAN_POINT('Ctrl Pts',(9.84712438256308,20.5712908125145,12.));
#209828=CARTESIAN_POINT('Ctrl Pts',(9.85360251457004,20.580810471002,0.));
#209829=CARTESIAN_POINT('Ctrl Pts',(9.85360251457004,20.580810471002,12.));
#209830=CARTESIAN_POINT('Ctrl Pts',(9.86022127232749,20.5904671449755,0.));
#209831=CARTESIAN_POINT('Ctrl Pts',(9.86022127232749,20.5904671449755,12.));
#209832=CARTESIAN_POINT('Ctrl Pts',(9.86697998242612,20.6002579513696,0.));
#209833=CARTESIAN_POINT('Ctrl Pts',(9.86697998242612,20.6002579513696,12.));
#209834=CARTESIAN_POINT('Ctrl Pts',(9.87387798732943,20.6101800854491,0.));
#209835=CARTESIAN_POINT('Ctrl Pts',(9.87387798732943,20.6101800854491,12.));
#209836=CARTESIAN_POINT('Ctrl Pts',(9.88091464472669,20.6202308177472,0.));
#209837=CARTESIAN_POINT('Ctrl Pts',(9.88091464472669,20.6202308177472,12.));
#209838=CARTESIAN_POINT('Ctrl Pts',(9.88808932697304,20.6304074914086,0.));
#209839=CARTESIAN_POINT('Ctrl Pts',(9.88808932697304,20.6304074914086,12.));
#209840=CARTESIAN_POINT('Ctrl Pts',(9.89540142049123,20.6407075193977,0.));
#209841=CARTESIAN_POINT('Ctrl Pts',(9.89540142049123,20.6407075193977,12.));
#209842=CARTESIAN_POINT('Ctrl Pts',(9.90285032516695,20.6511283817415,0.));
#209843=CARTESIAN_POINT('Ctrl Pts',(9.90285032516695,20.6511283817415,12.));
#209844=CARTESIAN_POINT('Ctrl Pts',(9.91043545377004,20.6616676228315,0.));
#209845=CARTESIAN_POINT('Ctrl Pts',(9.91043545377004,20.6616676228315,12.));
#209846=CARTESIAN_POINT('Ctrl Pts',(9.91815623141284,20.6723228488262,0.));
#209847=CARTESIAN_POINT('Ctrl Pts',(9.91815623141284,20.6723228488262,12.));
#209848=CARTESIAN_POINT('Ctrl Pts',(9.9260120949875,20.6830917250255,0.));
#209849=CARTESIAN_POINT('Ctrl Pts',(9.9260120949875,20.6830917250255,12.));
#209850=CARTESIAN_POINT('Ctrl Pts',(9.93400249259736,20.6939719732485,0.));
#209851=CARTESIAN_POINT('Ctrl Pts',(9.93400249259736,20.6939719732485,12.));
#209852=CARTESIAN_POINT('Ctrl Pts',(9.9421268829825,20.7049613692237,0.));
#209853=CARTESIAN_POINT('Ctrl Pts',(9.9421268829825,20.7049613692237,12.));
#209854=CARTESIAN_POINT('Ctrl Pts',(9.95038473514962,20.7160577407581,0.));
#209855=CARTESIAN_POINT('Ctrl Pts',(9.95038473514962,20.7160577407581,12.));
#209856=CARTESIAN_POINT('Ctrl Pts',(9.95877552798403,20.7272589658752,0.));
#209857=CARTESIAN_POINT('Ctrl Pts',(9.95877552798403,20.7272589658752,12.));
#209858=CARTESIAN_POINT('Ctrl Pts',(9.96729874986198,20.7385629709795,0.));
#209859=CARTESIAN_POINT('Ctrl Pts',(9.96729874986198,20.7385629709795,12.));
#209860=CARTESIAN_POINT('Ctrl Pts',(9.97595389823461,20.7499677289626,0.));
#209861=CARTESIAN_POINT('Ctrl Pts',(9.97595389823461,20.7499677289626,12.));
#209862=CARTESIAN_POINT('Ctrl Pts',(9.98474047926846,20.7614712574989,0.));
#209863=CARTESIAN_POINT('Ctrl Pts',(9.98474047926846,20.7614712574989,12.));
#209864=CARTESIAN_POINT('Ctrl Pts',(9.99365800754637,20.7730716175417,0.));
#209865=CARTESIAN_POINT('Ctrl Pts',(9.99365800754637,20.7730716175417,12.));
#209866=CARTESIAN_POINT('Ctrl Pts',(10.0027060057389,20.7847669117568,0.));
#209867=CARTESIAN_POINT('Ctrl Pts',(10.0027060057389,20.7847669117568,12.));
#209868=CARTESIAN_POINT('Ctrl Pts',(10.0118840042786,20.7965552829907,0.));
#209869=CARTESIAN_POINT('Ctrl Pts',(10.0118840042786,20.7965552829907,12.));
#209870=CARTESIAN_POINT('Ctrl Pts',(10.0211915410095,20.8084349126885,0.));
#209871=CARTESIAN_POINT('Ctrl Pts',(10.0211915410095,20.8084349126885,12.));
#209872=CARTESIAN_POINT('Ctrl Pts',(10.0306281609435,20.8204040196599,0.));
#209873=CARTESIAN_POINT('Ctrl Pts',(10.0306281609435,20.8204040196599,12.));
#209874=CARTESIAN_POINT('Ctrl Pts',(10.0401934160234,20.8324608588906,0.));
#209875=CARTESIAN_POINT('Ctrl Pts',(10.0401934160234,20.8324608588906,12.));
#209876=CARTESIAN_POINT('Ctrl Pts',(10.0498868648733,20.8446037203402,0.));
#209877=CARTESIAN_POINT('Ctrl Pts',(10.0498868648733,20.8446037203402,12.));
#209878=CARTESIAN_POINT('Ctrl Pts',(10.0597080725375,20.856830927732,0.));
#209879=CARTESIAN_POINT('Ctrl Pts',(10.0597080725375,20.856830927732,12.));
#209880=CARTESIAN_POINT('Ctrl Pts',(10.0696566102219,20.8691408373705,0.));
#209881=CARTESIAN_POINT('Ctrl Pts',(10.0696566102219,20.8691408373705,12.));
#209882=CARTESIAN_POINT('Ctrl Pts',(10.0797320551154,20.8815318371844,0.));
#209883=CARTESIAN_POINT('Ctrl Pts',(10.0797320551154,20.8815318371844,12.));
#209884=CARTESIAN_POINT('Ctrl Pts',(10.0899339901916,20.8940023457371,0.));
#209885=CARTESIAN_POINT('Ctrl Pts',(10.0899339901916,20.8940023457371,12.));
#209886=CARTESIAN_POINT('Ctrl Pts',(10.1002620040076,20.9065508112556,0.));
#209887=CARTESIAN_POINT('Ctrl Pts',(10.1002620040076,20.9065508112556,12.));
#209888=CARTESIAN_POINT('Ctrl Pts',(10.1107156904836,20.9191757106266,0.));
#209889=CARTESIAN_POINT('Ctrl Pts',(10.1107156904836,20.9191757106266,12.));
#209890=CARTESIAN_POINT('Ctrl Pts',(10.1212946487057,20.931875548473,0.));
#209891=CARTESIAN_POINT('Ctrl Pts',(10.1212946487057,20.931875548473,12.));
#209892=CARTESIAN_POINT('Ctrl Pts',(10.1319984827909,20.944648856393,0.));
#209893=CARTESIAN_POINT('Ctrl Pts',(10.1319984827909,20.944648856393,12.));
#209894=CARTESIAN_POINT('Ctrl Pts',(10.1428268017257,20.9574941921591,0.));
#209895=CARTESIAN_POINT('Ctrl Pts',(10.1428268017257,20.9574941921591,12.));
#209896=CARTESIAN_POINT('Ctrl Pts',(10.1537792192065,20.970410138937,0.));
#209897=CARTESIAN_POINT('Ctrl Pts',(10.1537792192065,20.970410138937,12.));
#209898=CARTESIAN_POINT('Ctrl Pts',(10.1648553534567,20.9833953044737,0.));
#209899=CARTESIAN_POINT('Ctrl Pts',(10.1648553534567,20.9833953044737,12.));
#209900=CARTESIAN_POINT('Ctrl Pts',(10.1760548270765,20.9964483203685,0.));
#209901=CARTESIAN_POINT('Ctrl Pts',(10.1760548270765,20.9964483203685,12.));
#209902=CARTESIAN_POINT('Ctrl Pts',(10.1873772669358,21.0095678414486,0.));
#209903=CARTESIAN_POINT('Ctrl Pts',(10.1873772669358,21.0095678414486,12.));
#209904=CARTESIAN_POINT('Ctrl Pts',(10.1988223040425,21.0227525451107,0.));
#209905=CARTESIAN_POINT('Ctrl Pts',(10.1988223040425,21.0227525451107,12.));
#209906=CARTESIAN_POINT('Ctrl Pts',(10.2103895734123,21.0360011306814,0.));
#209907=CARTESIAN_POINT('Ctrl Pts',(10.2103895734123,21.0360011306814,12.));
#209908=CARTESIAN_POINT('Ctrl Pts',(10.2220787139157,21.0493123187484,0.));
#209909=CARTESIAN_POINT('Ctrl Pts',(10.2220787139157,21.0493123187484,12.));
#209910=CARTESIAN_POINT('Ctrl Pts',(10.233889368157,21.0626848505665,0.));
#209911=CARTESIAN_POINT('Ctrl Pts',(10.233889368157,21.0626848505665,12.));
#209912=CARTESIAN_POINT('Ctrl Pts',(10.2458211823915,21.0761174875448,0.));
#209913=CARTESIAN_POINT('Ctrl Pts',(10.2458211823915,21.0761174875448,12.));
#209914=CARTESIAN_POINT('Ctrl Pts',(10.2578738064183,21.0896090107066,0.));
#209915=CARTESIAN_POINT('Ctrl Pts',(10.2578738064183,21.0896090107066,12.));
#209916=CARTESIAN_POINT('Ctrl Pts',(10.2700468934743,21.1031582201625,0.));
#209917=CARTESIAN_POINT('Ctrl Pts',(10.2700468934743,21.1031582201625,12.));
#209918=CARTESIAN_POINT('Ctrl Pts',(10.2823401001067,21.1167639345623,0.));
#209919=CARTESIAN_POINT('Ctrl Pts',(10.2823401001067,21.1167639345623,12.));
#209920=CARTESIAN_POINT('Ctrl Pts',(10.2947530860714,21.130424990599,0.));
#209921=CARTESIAN_POINT('Ctrl Pts',(10.2947530860714,21.130424990599,12.));
#209922=CARTESIAN_POINT('Ctrl Pts',(10.307285514268,21.1441402425831,0.));
#209923=CARTESIAN_POINT('Ctrl Pts',(10.307285514268,21.1441402425831,12.));
#209924=CARTESIAN_POINT('Ctrl Pts',(10.3199370506541,21.1579085619959,0.));
#209925=CARTESIAN_POINT('Ctrl Pts',(10.3199370506541,21.1579085619959,12.));
#209926=CARTESIAN_POINT('Ctrl Pts',(10.3327073641574,21.1717288370512,0.));
#209927=CARTESIAN_POINT('Ctrl Pts',(10.3327073641574,21.1717288370512,12.));
#209928=CARTESIAN_POINT('Ctrl Pts',(10.3455961265706,21.1855999722427,0.));
#209929=CARTESIAN_POINT('Ctrl Pts',(10.3455961265706,21.1855999722427,12.));
#209930=CARTESIAN_POINT('Ctrl Pts',(10.3586030124595,21.1995208879205,0.));
#209931=CARTESIAN_POINT('Ctrl Pts',(10.3586030124595,21.1995208879205,12.));
#209932=CARTESIAN_POINT('Ctrl Pts',(10.3717276991137,21.2134905199359,0.));
#209933=CARTESIAN_POINT('Ctrl Pts',(10.3717276991137,21.2134905199359,12.));
#209934=CARTESIAN_POINT('Ctrl Pts',(10.384969866479,21.2275078192708,0.));
#209935=CARTESIAN_POINT('Ctrl Pts',(10.384969866479,21.2275078192708,12.));
#209936=CARTESIAN_POINT('Ctrl Pts',(10.3983291970846,21.2415717516713,0.));
#209937=CARTESIAN_POINT('Ctrl Pts',(10.3983291970846,21.2415717516713,12.));
#209938=CARTESIAN_POINT('Ctrl Pts',(10.4118053759584,21.2556812972741,0.));
#209939=CARTESIAN_POINT('Ctrl Pts',(10.4118053759584,21.2556812972741,12.));
#209940=CARTESIAN_POINT('Ctrl Pts',(10.4253980905394,21.2698354502391,0.));
#209941=CARTESIAN_POINT('Ctrl Pts',(10.4253980905394,21.2698354502391,12.));
#209942=CARTESIAN_POINT('Ctrl Pts',(10.4391070306385,21.2840332184471,0.));
#209943=CARTESIAN_POINT('Ctrl Pts',(10.4391070306385,21.2840332184471,12.));
#209944=CARTESIAN_POINT('Ctrl Pts',(10.452931888387,21.2982736231924,0.));
#209945=CARTESIAN_POINT('Ctrl Pts',(10.452931888387,21.2982736231924,12.));
#209946=CARTESIAN_POINT('Ctrl Pts',(10.4668723581768,21.312555698873,0.));
#209947=CARTESIAN_POINT('Ctrl Pts',(10.4668723581768,21.312555698873,12.));
#209948=CARTESIAN_POINT('Ctrl Pts',(10.4809281365933,21.3268784926823,0.));
#209949=CARTESIAN_POINT('Ctrl Pts',(10.4809281365933,21.3268784926823,12.));
#209950=CARTESIAN_POINT('Ctrl Pts',(10.4950989223341,21.3412410642912,0.));
#209951=CARTESIAN_POINT('Ctrl Pts',(10.4950989223341,21.3412410642912,12.));
#209952=CARTESIAN_POINT('Ctrl Pts',(10.5093844161689,21.3556424855822,0.));
#209953=CARTESIAN_POINT('Ctrl Pts',(10.5093844161689,21.3556424855822,12.));
#209954=CARTESIAN_POINT('Ctrl Pts',(10.523784320906,21.3700818403942,0.));
#209955=CARTESIAN_POINT('Ctrl Pts',(10.523784320906,21.3700818403942,12.));
#209956=CARTESIAN_POINT('Ctrl Pts',(10.5382983413422,21.3845582242604,0.));
#209957=CARTESIAN_POINT('Ctrl Pts',(10.5382983413422,21.3845582242604,12.));
#209958=CARTESIAN_POINT('Ctrl Pts',(10.5529261842107,21.3990707441495,0.));
#209959=CARTESIAN_POINT('Ctrl Pts',(10.5529261842107,21.3990707441495,12.));
#209960=CARTESIAN_POINT('Ctrl Pts',(10.5676675581106,21.4136185181974,0.));
#209961=CARTESIAN_POINT('Ctrl Pts',(10.5676675581106,21.4136185181974,12.));
#209962=CARTESIAN_POINT('Ctrl Pts',(10.582522173457,21.4282006754624,0.));
#209963=CARTESIAN_POINT('Ctrl Pts',(10.582522173457,21.4282006754624,12.));
#209964=CARTESIAN_POINT('Ctrl Pts',(10.597489742462,21.4428163557137,0.));
#209965=CARTESIAN_POINT('Ctrl Pts',(10.597489742462,21.4428163557137,12.));
#209966=CARTESIAN_POINT('Ctrl Pts',(10.612569979096,21.4574647092093,0.));
#209967=CARTESIAN_POINT('Ctrl Pts',(10.612569979096,21.4574647092093,12.));
#209968=CARTESIAN_POINT('Ctrl Pts',(10.6277625990456,21.4721448964766,0.));
#209969=CARTESIAN_POINT('Ctrl Pts',(10.6277625990456,21.4721448964766,12.));
#209970=CARTESIAN_POINT('Ctrl Pts',(10.6430673196609,21.4868560880893,0.));
#209971=CARTESIAN_POINT('Ctrl Pts',(10.6430673196609,21.4868560880893,12.));
#209972=CARTESIAN_POINT('Ctrl Pts',(10.658483859894,21.5015974644454,0.));
#209973=CARTESIAN_POINT('Ctrl Pts',(10.658483859894,21.5015974644454,12.));
#209974=CARTESIAN_POINT('Ctrl Pts',(10.6740119402835,21.5163682155805,0.));
#209975=CARTESIAN_POINT('Ctrl Pts',(10.6740119402835,21.5163682155805,12.));
#209976=CARTESIAN_POINT('Ctrl Pts',(10.689651282929,21.531167540981,0.));
#209977=CARTESIAN_POINT('Ctrl Pts',(10.689651282929,21.531167540981,12.));
#209978=CARTESIAN_POINT('Ctrl Pts',(10.7054016114571,21.5459946493955,0.));
#209979=CARTESIAN_POINT('Ctrl Pts',(10.7054016114571,21.5459946493955,12.));
#209980=CARTESIAN_POINT('Ctrl Pts',(10.7212626509816,21.5608487586467,0.));
#209981=CARTESIAN_POINT('Ctrl Pts',(10.7212626509816,21.5608487586467,12.));
#209982=CARTESIAN_POINT('Ctrl Pts',(10.7372341280468,21.5757290954372,0.));
#209983=CARTESIAN_POINT('Ctrl Pts',(10.7372341280468,21.5757290954372,12.));
#209984=CARTESIAN_POINT('Ctrl Pts',(10.7533157705943,21.5906348951745,0.));
#209985=CARTESIAN_POINT('Ctrl Pts',(10.7533157705943,21.5906348951745,12.));
#209986=CARTESIAN_POINT('Ctrl Pts',(10.7695073079554,21.6055654018179,0.));
#209987=CARTESIAN_POINT('Ctrl Pts',(10.7695073079554,21.6055654018179,12.));
#209988=CARTESIAN_POINT('Ctrl Pts',(10.7858084708262,21.6205198677176,0.));
#209989=CARTESIAN_POINT('Ctrl Pts',(10.7858084708262,21.6205198677176,12.));
#209990=CARTESIAN_POINT('Ctrl Pts',(10.8022189912369,21.6354975534558,0.));
#209991=CARTESIAN_POINT('Ctrl Pts',(10.8022189912369,21.6354975534558,12.));
#209992=CARTESIAN_POINT('Ctrl Pts',(10.8187386025135,21.6504977276864,0.));
#209993=CARTESIAN_POINT('Ctrl Pts',(10.8187386025135,21.6504977276864,12.));
#209994=CARTESIAN_POINT('Ctrl Pts',(10.835367039227,21.6655196669727,0.));
#209995=CARTESIAN_POINT('Ctrl Pts',(10.835367039227,21.6655196669727,12.));
#209996=CARTESIAN_POINT('Ctrl Pts',(10.8521040371832,21.6805626556461,0.));
#209997=CARTESIAN_POINT('Ctrl Pts',(10.8521040371832,21.6805626556461,12.));
#209998=CARTESIAN_POINT('Ctrl Pts',(10.8689493334093,21.6956259856667,0.));
#209999=CARTESIAN_POINT('Ctrl Pts',(10.8689493334093,21.6956259856667,12.));
#210000=CARTESIAN_POINT('Ctrl Pts',(10.8859026661292,21.7107089564822,0.));
#210001=CARTESIAN_POINT('Ctrl Pts',(10.8859026661292,21.7107089564822,12.));
#210002=CARTESIAN_POINT('Ctrl Pts',(10.9029637747341,21.7258108748874,0.));
#210003=CARTESIAN_POINT('Ctrl Pts',(10.9029637747341,21.7258108748874,12.));
#210004=CARTESIAN_POINT('Ctrl Pts',(10.9201323997386,21.74093105488,0.));
#210005=CARTESIAN_POINT('Ctrl Pts',(10.9201323997386,21.74093105488,12.));
#210006=CARTESIAN_POINT('Ctrl Pts',(10.9374082827446,21.7560688175252,0.));
#210007=CARTESIAN_POINT('Ctrl Pts',(10.9374082827446,21.7560688175252,12.));
#210008=CARTESIAN_POINT('Ctrl Pts',(10.9547911664457,21.7712234908468,0.));
#210009=CARTESIAN_POINT('Ctrl Pts',(10.9547911664457,21.7712234908468,12.));
#210010=CARTESIAN_POINT('Ctrl Pts',(10.9722807946157,21.7863944097143,0.));
#210011=CARTESIAN_POINT('Ctrl Pts',(10.9722807946157,21.7863944097143,12.));
#210012=CARTESIAN_POINT('Ctrl Pts',(10.9898769120913,21.8015809157302,0.));
#210013=CARTESIAN_POINT('Ctrl Pts',(10.9898769120913,21.8015809157302,12.));
#210014=CARTESIAN_POINT('Ctrl Pts',(11.0075792647477,21.8167823571168,0.));
#210015=CARTESIAN_POINT('Ctrl Pts',(11.0075792647477,21.8167823571168,12.));
#210016=CARTESIAN_POINT('Ctrl Pts',(11.0253875994598,21.8319980886033,0.));
#210017=CARTESIAN_POINT('Ctrl Pts',(11.0253875994598,21.8319980886033,12.));
#210018=CARTESIAN_POINT('Ctrl Pts',(11.0433016640808,21.8472274713103,0.));
#210019=CARTESIAN_POINT('Ctrl Pts',(11.0433016640808,21.8472274713103,12.));
#210020=CARTESIAN_POINT('Ctrl Pts',(11.0613212074364,21.8624698726319,0.));
#210021=CARTESIAN_POINT('Ctrl Pts',(11.0613212074364,21.8624698726319,12.));
#210022=CARTESIAN_POINT('Ctrl Pts',(11.0794459793058,21.8777246661191,0.));
#210023=CARTESIAN_POINT('Ctrl Pts',(11.0794459793058,21.8777246661191,12.));
#210024=CARTESIAN_POINT('Ctrl Pts',(11.0976757303944,21.8929912313608,0.));
#210025=CARTESIAN_POINT('Ctrl Pts',(11.0976757303944,21.8929912313608,12.));
#210026=CARTESIAN_POINT('Ctrl Pts',(11.1160102123024,21.9082689538687,0.));
#210027=CARTESIAN_POINT('Ctrl Pts',(11.1160102123024,21.9082689538687,12.));
#210028=CARTESIAN_POINT('Ctrl Pts',(11.134449177474,21.9235572249518,0.));
#210029=CARTESIAN_POINT('Ctrl Pts',(11.134449177474,21.9235572249518,12.));
#210030=CARTESIAN_POINT('Ctrl Pts',(11.1529923792002,21.9388554416437,0.));
#210031=CARTESIAN_POINT('Ctrl Pts',(11.1529923792002,21.9388554416437,12.));
#210032=CARTESIAN_POINT('Ctrl Pts',(11.1716395716375,21.9541630066504,0.));
#210033=CARTESIAN_POINT('Ctrl Pts',(11.1716395716375,21.9541630066504,12.));
#210034=CARTESIAN_POINT('Ctrl Pts',(11.1903905098109,21.9694793282913,0.));
#210035=CARTESIAN_POINT('Ctrl Pts',(11.1903905098109,21.9694793282913,12.));
#210036=CARTESIAN_POINT('Ctrl Pts',(11.2092449496125,21.9848038204439,0.));
#210037=CARTESIAN_POINT('Ctrl Pts',(11.2092449496125,21.9848038204439,12.));
#210038=CARTESIAN_POINT('Ctrl Pts',(11.2282026477897,22.000135902484,0.));
#210039=CARTESIAN_POINT('Ctrl Pts',(11.2282026477897,22.000135902484,12.));
#210040=CARTESIAN_POINT('Ctrl Pts',(11.2472633619276,22.0154749992364,0.));
#210041=CARTESIAN_POINT('Ctrl Pts',(11.2472633619276,22.0154749992364,12.));
#210042=CARTESIAN_POINT('Ctrl Pts',(11.2664268504207,22.0308205408351,0.));
#210043=CARTESIAN_POINT('Ctrl Pts',(11.2664268504207,22.0308205408351,12.));
#210044=CARTESIAN_POINT('Ctrl Pts',(11.2856928724374,22.0461719625661,0.));
#210045=CARTESIAN_POINT('Ctrl Pts',(11.2856928724374,22.0461719625661,12.));
#210046=CARTESIAN_POINT('Ctrl Pts',(11.3050611878771,22.0615287047179,0.));
#210047=CARTESIAN_POINT('Ctrl Pts',(11.3050611878771,22.0615287047179,12.));
#210048=CARTESIAN_POINT('Ctrl Pts',(11.3245315573168,22.0768902124267,0.));
#210049=CARTESIAN_POINT('Ctrl Pts',(11.3245315573168,22.0768902124267,12.));
#210050=CARTESIAN_POINT('Ctrl Pts',(11.3441037419553,22.0922559355293,0.));
#210051=CARTESIAN_POINT('Ctrl Pts',(11.3441037419553,22.0922559355293,12.));
#210052=CARTESIAN_POINT('Ctrl Pts',(11.3637775035367,22.1076253283978,0.));
#210053=CARTESIAN_POINT('Ctrl Pts',(11.3637775035367,22.1076253283978,12.));
#210054=CARTESIAN_POINT('Ctrl Pts',(11.3835526044256,22.1229978500185,0.));
#210055=CARTESIAN_POINT('Ctrl Pts',(11.3835526044256,22.1229978500185,12.));
#210056=CARTESIAN_POINT('Ctrl Pts',(11.4034288076908,22.1383729640963,0.));
#210057=CARTESIAN_POINT('Ctrl Pts',(11.4034288076908,22.1383729640963,12.));
#210058=CARTESIAN_POINT('Ctrl Pts',(11.4234058771742,22.1537501391486,0.));
#210059=CARTESIAN_POINT('Ctrl Pts',(11.4234058771742,22.1537501391486,12.));
#210060=CARTESIAN_POINT('Ctrl Pts',(11.443483577557,22.1691288486096,0.));
#210061=CARTESIAN_POINT('Ctrl Pts',(11.443483577557,22.1691288486096,12.));
#210062=CARTESIAN_POINT('Ctrl Pts',(11.463661674411,22.184508570917,0.));
#210063=CARTESIAN_POINT('Ctrl Pts',(11.463661674411,22.184508570917,12.));
#210064=CARTESIAN_POINT('Ctrl Pts',(11.4839399342589,22.1998887896435,0.));
#210065=CARTESIAN_POINT('Ctrl Pts',(11.4839399342589,22.1998887896435,12.));
#210066=CARTESIAN_POINT('Ctrl Pts',(11.504318124424,22.215268993102,0.));
#210067=CARTESIAN_POINT('Ctrl Pts',(11.504318124424,22.215268993102,12.));
#210068=CARTESIAN_POINT('Ctrl Pts',(11.5247960128476,22.2306486738899,0.));
#210069=CARTESIAN_POINT('Ctrl Pts',(11.5247960128476,22.2306486738899,12.));
#210070=CARTESIAN_POINT('Ctrl Pts',(11.545373367912,22.2460273284653,0.));
#210071=CARTESIAN_POINT('Ctrl Pts',(11.545373367912,22.2460273284653,12.));
#210072=CARTESIAN_POINT('Ctrl Pts',(11.5660499582403,22.2614044566898,0.));
#210073=CARTESIAN_POINT('Ctrl Pts',(11.5660499582403,22.2614044566898,12.));
#210074=CARTESIAN_POINT('Ctrl Pts',(11.5868255525189,22.2767795614349,0.));
#210075=CARTESIAN_POINT('Ctrl Pts',(11.5868255525189,22.2767795614349,12.));
#210076=CARTESIAN_POINT('Ctrl Pts',(11.6076999192359,22.2921521480358,0.));
#210077=CARTESIAN_POINT('Ctrl Pts',(11.6076999192359,22.2921521480358,12.));
#210078=CARTESIAN_POINT('Ctrl Pts',(11.6286728270011,22.3075217249049,0.));
#210079=CARTESIAN_POINT('Ctrl Pts',(11.6286728270011,22.3075217249049,12.));
#210080=CARTESIAN_POINT('Ctrl Pts',(11.6497440449858,22.3228878043976,0.));
#210081=CARTESIAN_POINT('Ctrl Pts',(11.6497440449858,22.3228878043976,12.));
#210082=CARTESIAN_POINT('Ctrl Pts',(11.6709133432986,22.3382499035618,0.));
#210083=CARTESIAN_POINT('Ctrl Pts',(11.6709133432986,22.3382499035618,12.));
#210084=CARTESIAN_POINT('Ctrl Pts',(11.6921804934056,22.3536075450028,0.));
#210085=CARTESIAN_POINT('Ctrl Pts',(11.6921804934056,22.3536075450028,12.));
#210086=CARTESIAN_POINT('Ctrl Pts',(11.7135452684532,22.3689602575492,0.));
#210087=CARTESIAN_POINT('Ctrl Pts',(11.7135452684532,22.3689602575492,12.));
#210088=CARTESIAN_POINT('Ctrl Pts',(11.7350074437961,22.3843075773905,0.));
#210089=CARTESIAN_POINT('Ctrl Pts',(11.7350074437961,22.3843075773905,12.));
#210090=CARTESIAN_POINT('Ctrl Pts',(11.7565667964765,22.39964904692,0.));
#210091=CARTESIAN_POINT('Ctrl Pts',(11.7565667964765,22.39964904692,12.));
#210092=CARTESIAN_POINT('Ctrl Pts',(11.7782231042041,22.4149842125018,0.));
#210093=CARTESIAN_POINT('Ctrl Pts',(11.7782231042041,22.4149842125018,12.));
#210094=CARTESIAN_POINT('Ctrl Pts',(11.7999761445175,22.4303126226468,0.));
#210095=CARTESIAN_POINT('Ctrl Pts',(11.7999761445175,22.4303126226468,12.));
#210096=CARTESIAN_POINT('Ctrl Pts',(11.8218256937889,22.4456338258738,0.));
#210097=CARTESIAN_POINT('Ctrl Pts',(11.8218256937889,22.4456338258738,12.));
#210098=CARTESIAN_POINT('Ctrl Pts',(11.8437715264487,22.4609473690469,0.));
#210099=CARTESIAN_POINT('Ctrl Pts',(11.8437715264487,22.4609473690469,12.));
#210100=CARTESIAN_POINT('Ctrl Pts',(11.8658134137018,22.4762527946694,0.));
#210101=CARTESIAN_POINT('Ctrl Pts',(11.8658134137018,22.4762527946694,12.));
#210102=CARTESIAN_POINT('Ctrl Pts',(11.8879511239941,22.4915496418472,0.));
#210103=CARTESIAN_POINT('Ctrl Pts',(11.8879511239941,22.4915496418472,12.));
#210104=CARTESIAN_POINT('Ctrl Pts',(11.9101844254555,22.5068374513958,0.));
#210105=CARTESIAN_POINT('Ctrl Pts',(11.9101844254555,22.5068374513958,12.));
#210106=CARTESIAN_POINT('Ctrl Pts',(11.9325130877801,22.5221157697869,0.));
#210107=CARTESIAN_POINT('Ctrl Pts',(11.9325130877801,22.5221157697869,12.));
#210108=CARTESIAN_POINT('Ctrl Pts',(11.9549368843996,22.5373841537299,0.));
#210109=CARTESIAN_POINT('Ctrl Pts',(11.9549368843996,22.5373841537299,12.));
#210110=CARTESIAN_POINT('Ctrl Pts',(11.9774555943496,22.5526421741159,0.));
#210111=CARTESIAN_POINT('Ctrl Pts',(11.9774555943496,22.5526421741159,12.));
#210112=CARTESIAN_POINT('Ctrl Pts',(12.0000690046697,22.5678894211194,0.));
#210113=CARTESIAN_POINT('Ctrl Pts',(12.0000690046697,22.5678894211194,12.));
#210114=CARTESIAN_POINT('Ctrl Pts',(12.0227769113132,22.5831255061306,0.));
#210115=CARTESIAN_POINT('Ctrl Pts',(12.0227769113132,22.5831255061306,12.));
#210116=CARTESIAN_POINT('Ctrl Pts',(12.0455791139135,22.5983500505675,0.));
#210117=CARTESIAN_POINT('Ctrl Pts',(12.0455791139135,22.5983500505675,12.));
#210118=CARTESIAN_POINT('Ctrl Pts',(12.0684754113869,22.613562676493,0.));
#210119=CARTESIAN_POINT('Ctrl Pts',(12.0684754113869,22.613562676493,12.));
#210120=CARTESIAN_POINT('Ctrl Pts',(12.0914655972828,22.628762996708,0.));
#210121=CARTESIAN_POINT('Ctrl Pts',(12.0914655972828,22.628762996708,12.));
#210122=CARTESIAN_POINT('Ctrl Pts',(12.1145494550384,22.6439506046611,0.));
#210123=CARTESIAN_POINT('Ctrl Pts',(12.1145494550384,22.6439506046611,12.));
#210124=CARTESIAN_POINT('Ctrl Pts',(12.1377267537141,22.6591250653942,0.));
#210125=CARTESIAN_POINT('Ctrl Pts',(12.1377267537141,22.6591250653942,12.));
#210126=CARTESIAN_POINT('Ctrl Pts',(12.1609972423088,22.6742859034891,0.));
#210127=CARTESIAN_POINT('Ctrl Pts',(12.1609972423088,22.6742859034891,12.));
#210128=CARTESIAN_POINT('Ctrl Pts',(12.1843606579246,22.6894326204959,0.));
#210129=CARTESIAN_POINT('Ctrl Pts',(12.1843606579246,22.6894326204959,12.));
#210130=CARTESIAN_POINT('Ctrl Pts',(12.2078167360267,22.7045647168659,0.));
#210131=CARTESIAN_POINT('Ctrl Pts',(12.2078167360267,22.7045647168659,12.));
#210132=CARTESIAN_POINT('Ctrl Pts',(12.2313652198047,22.7196817119299,0.));
#210133=CARTESIAN_POINT('Ctrl Pts',(12.2313652198047,22.7196817119299,12.));
#210134=CARTESIAN_POINT('Ctrl Pts',(12.2550058702389,22.7347831655251,0.));
#210135=CARTESIAN_POINT('Ctrl Pts',(12.2550058702389,22.7347831655251,12.));
#210136=CARTESIAN_POINT('Ctrl Pts',(12.2787384750747,22.7498686970096,0.));
#210137=CARTESIAN_POINT('Ctrl Pts',(12.2787384750747,22.7498686970096,12.));
#210138=CARTESIAN_POINT('Ctrl Pts',(12.3025628601811,22.7649380101154,0.));
#210139=CARTESIAN_POINT('Ctrl Pts',(12.3025628601811,22.7649380101154,12.));
#210140=CARTESIAN_POINT('Ctrl Pts',(12.3264788926108,22.7799908974947,0.));
#210141=CARTESIAN_POINT('Ctrl Pts',(12.3264788926108,22.7799908974947,12.));
#210142=CARTESIAN_POINT('Ctrl Pts',(12.3504864740361,22.7950272216959,0.));
#210143=CARTESIAN_POINT('Ctrl Pts',(12.3504864740361,22.7950272216959,12.));
#210144=CARTESIAN_POINT('Ctrl Pts',(12.3745855366772,22.8100469022632,0.));
#210145=CARTESIAN_POINT('Ctrl Pts',(12.3745855366772,22.8100469022632,12.));
#210146=CARTESIAN_POINT('Ctrl Pts',(12.393937937903,22.8220493007353,0.));
#210147=CARTESIAN_POINT('Ctrl Pts',(12.393937937903,22.8220493007353,12.));
#210148=CARTESIAN_POINT('Ctrl Pts',(12.4084933766366,22.8310435872852,0.));
#210149=CARTESIAN_POINT('Ctrl Pts',(12.4084933766366,22.8310435872852,12.));
#210150=CARTESIAN_POINT('Ctrl Pts',(12.4182152851867,22.8370364396497,0.));
#210151=CARTESIAN_POINT('Ctrl Pts',(12.4182152851867,22.8370364396497,12.));
#210152=CARTESIAN_POINT('Ctrl Pts',(12.4230808101438,22.8400320311648,0.));
#210153=CARTESIAN_POINT('Ctrl Pts',(12.4230808101438,22.8400320311648,12.));
#210154=CARTESIAN_POINT('',(12.4230808101438,22.8400320311648,0.));
#210155=CARTESIAN_POINT('Ctrl Pts',(9.71462809124917,20.353053841303,0.));
#210156=CARTESIAN_POINT('Ctrl Pts',(9.71462954053074,20.353060251684,0.));
#210157=CARTESIAN_POINT('Ctrl Pts',(9.71465227853122,20.3531126095522,0.));
#210158=CARTESIAN_POINT('Ctrl Pts',(9.71474590350791,20.3533097561886,0.));
#210159=CARTESIAN_POINT('Ctrl Pts',(9.714989780521,20.3538098605706,0.));
#210160=CARTESIAN_POINT('Ctrl Pts',(9.71549257088174,20.3548282742361,0.));
#210161=CARTESIAN_POINT('Ctrl Pts',(9.71619192554146,20.3562337557875,0.));
#210162=CARTESIAN_POINT('Ctrl Pts',(9.71708493723061,20.3580133103357,0.));
#210163=CARTESIAN_POINT('Ctrl Pts',(9.71816778327998,20.3601498764344,0.));
#210164=CARTESIAN_POINT('Ctrl Pts',(9.71943648548114,20.362625691398,0.));
#210165=CARTESIAN_POINT('Ctrl Pts',(9.72088778381101,20.3654261611055,0.));
#210166=CARTESIAN_POINT('Ctrl Pts',(9.72251930722503,20.3685406190576,0.));
#210167=CARTESIAN_POINT('Ctrl Pts',(9.72432910043192,20.371960235676,0.));
#210168=CARTESIAN_POINT('Ctrl Pts',(9.7263153173287,20.3756766651952,0.));
#210169=CARTESIAN_POINT('Ctrl Pts',(9.72847589116532,20.3796805893304,0.));
#210170=CARTESIAN_POINT('Ctrl Pts',(9.73080870123726,20.3839624556742,0.));
#210171=CARTESIAN_POINT('Ctrl Pts',(9.73331167102812,20.3885129129912,0.));
#210172=CARTESIAN_POINT('Ctrl Pts',(9.73598292014249,20.3933234845646,0.));
#210173=CARTESIAN_POINT('Ctrl Pts',(9.73882077613206,20.3983866213331,0.));
#210174=CARTESIAN_POINT('Ctrl Pts',(9.74182369656272,20.4036953576549,0.));
#210175=CARTESIAN_POINT('Ctrl Pts',(9.74499021838536,20.4092430879861,0.));
#210176=CARTESIAN_POINT('Ctrl Pts',(9.74831889242174,20.4150232777393,0.));
#210177=CARTESIAN_POINT('Ctrl Pts',(9.75180829786433,20.4210295275818,0.));
#210178=CARTESIAN_POINT('Ctrl Pts',(9.75545705902416,20.4272556476629,0.));
#210179=CARTESIAN_POINT('Ctrl Pts',(9.75926386289929,20.4336957355474,0.));
#210180=CARTESIAN_POINT('Ctrl Pts',(9.76322747195502,20.4403442329401,0.));
#210181=CARTESIAN_POINT('Ctrl Pts',(9.76734670980896,20.447195862298,0.));
#210182=CARTESIAN_POINT('Ctrl Pts',(9.77162045104069,20.4542455817527,0.));
#210183=CARTESIAN_POINT('Ctrl Pts',(9.77604760815522,20.4614885274973,0.));
#210184=CARTESIAN_POINT('Ctrl Pts',(9.78062712373313,20.4689199790668,0.));
#210185=CARTESIAN_POINT('Ctrl Pts',(9.78535797314162,20.4765353711585,0.));
#210186=CARTESIAN_POINT('Ctrl Pts',(9.79023916498659,20.4843302955329,0.));
#210187=CARTESIAN_POINT('Ctrl Pts',(9.79526974288343,20.4923005087945,0.));
#210188=CARTESIAN_POINT('Ctrl Pts',(9.80044878520967,20.500441931211,0.));
#210189=CARTESIAN_POINT('Ctrl Pts',(9.80577540161102,20.5087506310507,0.));
#210190=CARTESIAN_POINT('Ctrl Pts',(9.81124873025278,20.5172228122839,0.));
#210191=CARTESIAN_POINT('Ctrl Pts',(9.81686793455918,20.5258548000625,0.));
#210192=CARTESIAN_POINT('Ctrl Pts',(9.82263220080327,20.534643029951,0.));
#210193=CARTESIAN_POINT('Ctrl Pts',(9.82854073773857,20.5435840460717,0.));
#210194=CARTESIAN_POINT('Ctrl Pts',(9.8345927758532,20.5526744976461,0.));
#210195=CARTESIAN_POINT('Ctrl Pts',(9.84078756677589,20.5619111362406,0.));
#210196=CARTESIAN_POINT('Ctrl Pts',(9.84712438256308,20.5712908125145,0.));
#210197=CARTESIAN_POINT('Ctrl Pts',(9.85360251457004,20.580810471002,0.));
#210198=CARTESIAN_POINT('Ctrl Pts',(9.86022127232749,20.5904671449755,0.));
#210199=CARTESIAN_POINT('Ctrl Pts',(9.86697998242612,20.6002579513696,0.));
#210200=CARTESIAN_POINT('Ctrl Pts',(9.87387798732943,20.6101800854491,0.));
#210201=CARTESIAN_POINT('Ctrl Pts',(9.88091464472669,20.6202308177472,0.));
#210202=CARTESIAN_POINT('Ctrl Pts',(9.88808932697304,20.6304074914086,0.));
#210203=CARTESIAN_POINT('Ctrl Pts',(9.89540142049123,20.6407075193977,0.));
#210204=CARTESIAN_POINT('Ctrl Pts',(9.90285032516695,20.6511283817415,0.));
#210205=CARTESIAN_POINT('Ctrl Pts',(9.91043545377004,20.6616676228315,0.));
#210206=CARTESIAN_POINT('Ctrl Pts',(9.91815623141284,20.6723228488262,0.));
#210207=CARTESIAN_POINT('Ctrl Pts',(9.9260120949875,20.6830917250255,0.));
#210208=CARTESIAN_POINT('Ctrl Pts',(9.93400249259736,20.6939719732485,0.));
#210209=CARTESIAN_POINT('Ctrl Pts',(9.9421268829825,20.7049613692237,0.));
#210210=CARTESIAN_POINT('Ctrl Pts',(9.95038473514962,20.7160577407581,0.));
#210211=CARTESIAN_POINT('Ctrl Pts',(9.95877552798403,20.7272589658752,0.));
#210212=CARTESIAN_POINT('Ctrl Pts',(9.96729874986198,20.7385629709795,0.));
#210213=CARTESIAN_POINT('Ctrl Pts',(9.97595389823461,20.7499677289626,0.));
#210214=CARTESIAN_POINT('Ctrl Pts',(9.98474047926846,20.7614712574989,0.));
#210215=CARTESIAN_POINT('Ctrl Pts',(9.99365800754637,20.7730716175417,0.));
#210216=CARTESIAN_POINT('Ctrl Pts',(10.0027060057389,20.7847669117568,0.));
#210217=CARTESIAN_POINT('Ctrl Pts',(10.0118840042786,20.7965552829907,0.));
#210218=CARTESIAN_POINT('Ctrl Pts',(10.0211915410095,20.8084349126885,0.));
#210219=CARTESIAN_POINT('Ctrl Pts',(10.0306281609435,20.8204040196599,0.));
#210220=CARTESIAN_POINT('Ctrl Pts',(10.0401934160234,20.8324608588906,0.));
#210221=CARTESIAN_POINT('Ctrl Pts',(10.0498868648733,20.8446037203402,0.));
#210222=CARTESIAN_POINT('Ctrl Pts',(10.0597080725375,20.856830927732,0.));
#210223=CARTESIAN_POINT('Ctrl Pts',(10.0696566102219,20.8691408373705,0.));
#210224=CARTESIAN_POINT('Ctrl Pts',(10.0797320551154,20.8815318371844,0.));
#210225=CARTESIAN_POINT('Ctrl Pts',(10.0899339901916,20.8940023457371,0.));
#210226=CARTESIAN_POINT('Ctrl Pts',(10.1002620040076,20.9065508112556,0.));
#210227=CARTESIAN_POINT('Ctrl Pts',(10.1107156904836,20.9191757106266,0.));
#210228=CARTESIAN_POINT('Ctrl Pts',(10.1212946487057,20.931875548473,0.));
#210229=CARTESIAN_POINT('Ctrl Pts',(10.1319984827909,20.944648856393,0.));
#210230=CARTESIAN_POINT('Ctrl Pts',(10.1428268017257,20.9574941921591,0.));
#210231=CARTESIAN_POINT('Ctrl Pts',(10.1537792192065,20.970410138937,0.));
#210232=CARTESIAN_POINT('Ctrl Pts',(10.1648553534567,20.9833953044737,0.));
#210233=CARTESIAN_POINT('Ctrl Pts',(10.1760548270765,20.9964483203685,0.));
#210234=CARTESIAN_POINT('Ctrl Pts',(10.1873772669358,21.0095678414486,0.));
#210235=CARTESIAN_POINT('Ctrl Pts',(10.1988223040425,21.0227525451107,0.));
#210236=CARTESIAN_POINT('Ctrl Pts',(10.2103895734123,21.0360011306814,0.));
#210237=CARTESIAN_POINT('Ctrl Pts',(10.2220787139157,21.0493123187484,0.));
#210238=CARTESIAN_POINT('Ctrl Pts',(10.233889368157,21.0626848505665,0.));
#210239=CARTESIAN_POINT('Ctrl Pts',(10.2458211823915,21.0761174875448,0.));
#210240=CARTESIAN_POINT('Ctrl Pts',(10.2578738064183,21.0896090107066,0.));
#210241=CARTESIAN_POINT('Ctrl Pts',(10.2700468934743,21.1031582201625,0.));
#210242=CARTESIAN_POINT('Ctrl Pts',(10.2823401001067,21.1167639345623,0.));
#210243=CARTESIAN_POINT('Ctrl Pts',(10.2947530860714,21.130424990599,0.));
#210244=CARTESIAN_POINT('Ctrl Pts',(10.307285514268,21.1441402425831,0.));
#210245=CARTESIAN_POINT('Ctrl Pts',(10.3199370506541,21.1579085619959,0.));
#210246=CARTESIAN_POINT('Ctrl Pts',(10.3327073641574,21.1717288370512,0.));
#210247=CARTESIAN_POINT('Ctrl Pts',(10.3455961265706,21.1855999722427,0.));
#210248=CARTESIAN_POINT('Ctrl Pts',(10.3586030124595,21.1995208879205,0.));
#210249=CARTESIAN_POINT('Ctrl Pts',(10.3717276991137,21.2134905199359,0.));
#210250=CARTESIAN_POINT('Ctrl Pts',(10.384969866479,21.2275078192708,0.));
#210251=CARTESIAN_POINT('Ctrl Pts',(10.3983291970846,21.2415717516713,0.));
#210252=CARTESIAN_POINT('Ctrl Pts',(10.4118053759584,21.2556812972741,0.));
#210253=CARTESIAN_POINT('Ctrl Pts',(10.4253980905394,21.2698354502391,0.));
#210254=CARTESIAN_POINT('Ctrl Pts',(10.4391070306385,21.2840332184471,0.));
#210255=CARTESIAN_POINT('Ctrl Pts',(10.452931888387,21.2982736231924,0.));
#210256=CARTESIAN_POINT('Ctrl Pts',(10.4668723581768,21.312555698873,0.));
#210257=CARTESIAN_POINT('Ctrl Pts',(10.4809281365933,21.3268784926823,0.));
#210258=CARTESIAN_POINT('Ctrl Pts',(10.4950989223341,21.3412410642912,0.));
#210259=CARTESIAN_POINT('Ctrl Pts',(10.5093844161689,21.3556424855822,0.));
#210260=CARTESIAN_POINT('Ctrl Pts',(10.523784320906,21.3700818403942,0.));
#210261=CARTESIAN_POINT('Ctrl Pts',(10.5382983413422,21.3845582242604,0.));
#210262=CARTESIAN_POINT('Ctrl Pts',(10.5529261842107,21.3990707441495,0.));
#210263=CARTESIAN_POINT('Ctrl Pts',(10.5676675581106,21.4136185181974,0.));
#210264=CARTESIAN_POINT('Ctrl Pts',(10.582522173457,21.4282006754624,0.));
#210265=CARTESIAN_POINT('Ctrl Pts',(10.597489742462,21.4428163557137,0.));
#210266=CARTESIAN_POINT('Ctrl Pts',(10.612569979096,21.4574647092093,0.));
#210267=CARTESIAN_POINT('Ctrl Pts',(10.6277625990456,21.4721448964766,0.));
#210268=CARTESIAN_POINT('Ctrl Pts',(10.6430673196609,21.4868560880893,0.));
#210269=CARTESIAN_POINT('Ctrl Pts',(10.658483859894,21.5015974644454,0.));
#210270=CARTESIAN_POINT('Ctrl Pts',(10.6740119402835,21.5163682155805,0.));
#210271=CARTESIAN_POINT('Ctrl Pts',(10.689651282929,21.531167540981,0.));
#210272=CARTESIAN_POINT('Ctrl Pts',(10.7054016114571,21.5459946493955,0.));
#210273=CARTESIAN_POINT('Ctrl Pts',(10.7212626509816,21.5608487586467,0.));
#210274=CARTESIAN_POINT('Ctrl Pts',(10.7372341280468,21.5757290954372,0.));
#210275=CARTESIAN_POINT('Ctrl Pts',(10.7533157705943,21.5906348951745,0.));
#210276=CARTESIAN_POINT('Ctrl Pts',(10.7695073079554,21.6055654018179,0.));
#210277=CARTESIAN_POINT('Ctrl Pts',(10.7858084708262,21.6205198677176,0.));
#210278=CARTESIAN_POINT('Ctrl Pts',(10.8022189912369,21.6354975534558,0.));
#210279=CARTESIAN_POINT('Ctrl Pts',(10.8187386025135,21.6504977276864,0.));
#210280=CARTESIAN_POINT('Ctrl Pts',(10.835367039227,21.6655196669727,0.));
#210281=CARTESIAN_POINT('Ctrl Pts',(10.8521040371832,21.6805626556461,0.));
#210282=CARTESIAN_POINT('Ctrl Pts',(10.8689493334093,21.6956259856667,0.));
#210283=CARTESIAN_POINT('Ctrl Pts',(10.8859026661292,21.7107089564822,0.));
#210284=CARTESIAN_POINT('Ctrl Pts',(10.9029637747341,21.7258108748874,0.));
#210285=CARTESIAN_POINT('Ctrl Pts',(10.9201323997386,21.74093105488,0.));
#210286=CARTESIAN_POINT('Ctrl Pts',(10.9374082827446,21.7560688175252,0.));
#210287=CARTESIAN_POINT('Ctrl Pts',(10.9547911664457,21.7712234908468,0.));
#210288=CARTESIAN_POINT('Ctrl Pts',(10.9722807946157,21.7863944097143,0.));
#210289=CARTESIAN_POINT('Ctrl Pts',(10.9898769120913,21.8015809157302,0.));
#210290=CARTESIAN_POINT('Ctrl Pts',(11.0075792647477,21.8167823571168,0.));
#210291=CARTESIAN_POINT('Ctrl Pts',(11.0253875994598,21.8319980886033,0.));
#210292=CARTESIAN_POINT('Ctrl Pts',(11.0433016640808,21.8472274713103,0.));
#210293=CARTESIAN_POINT('Ctrl Pts',(11.0613212074364,21.8624698726319,0.));
#210294=CARTESIAN_POINT('Ctrl Pts',(11.0794459793058,21.8777246661191,0.));
#210295=CARTESIAN_POINT('Ctrl Pts',(11.0976757303944,21.8929912313608,0.));
#210296=CARTESIAN_POINT('Ctrl Pts',(11.1160102123024,21.9082689538687,0.));
#210297=CARTESIAN_POINT('Ctrl Pts',(11.134449177474,21.9235572249518,0.));
#210298=CARTESIAN_POINT('Ctrl Pts',(11.1529923792002,21.9388554416437,0.));
#210299=CARTESIAN_POINT('Ctrl Pts',(11.1716395716375,21.9541630066504,0.));
#210300=CARTESIAN_POINT('Ctrl Pts',(11.1903905098109,21.9694793282913,0.));
#210301=CARTESIAN_POINT('Ctrl Pts',(11.2092449496125,21.9848038204439,0.));
#210302=CARTESIAN_POINT('Ctrl Pts',(11.2282026477897,22.000135902484,0.));
#210303=CARTESIAN_POINT('Ctrl Pts',(11.2472633619276,22.0154749992364,0.));
#210304=CARTESIAN_POINT('Ctrl Pts',(11.2664268504207,22.0308205408351,0.));
#210305=CARTESIAN_POINT('Ctrl Pts',(11.2856928724374,22.0461719625661,0.));
#210306=CARTESIAN_POINT('Ctrl Pts',(11.3050611878771,22.0615287047179,0.));
#210307=CARTESIAN_POINT('Ctrl Pts',(11.3245315573168,22.0768902124267,0.));
#210308=CARTESIAN_POINT('Ctrl Pts',(11.3441037419553,22.0922559355293,0.));
#210309=CARTESIAN_POINT('Ctrl Pts',(11.3637775035367,22.1076253283978,0.));
#210310=CARTESIAN_POINT('Ctrl Pts',(11.3835526044256,22.1229978500185,0.));
#210311=CARTESIAN_POINT('Ctrl Pts',(11.4034288076908,22.1383729640963,0.));
#210312=CARTESIAN_POINT('Ctrl Pts',(11.4234058771742,22.1537501391486,0.));
#210313=CARTESIAN_POINT('Ctrl Pts',(11.443483577557,22.1691288486096,0.));
#210314=CARTESIAN_POINT('Ctrl Pts',(11.463661674411,22.184508570917,0.));
#210315=CARTESIAN_POINT('Ctrl Pts',(11.4839399342589,22.1998887896435,0.));
#210316=CARTESIAN_POINT('Ctrl Pts',(11.504318124424,22.215268993102,0.));
#210317=CARTESIAN_POINT('Ctrl Pts',(11.5247960128476,22.2306486738899,0.));
#210318=CARTESIAN_POINT('Ctrl Pts',(11.545373367912,22.2460273284653,0.));
#210319=CARTESIAN_POINT('Ctrl Pts',(11.5660499582403,22.2614044566898,0.));
#210320=CARTESIAN_POINT('Ctrl Pts',(11.5868255525189,22.2767795614349,0.));
#210321=CARTESIAN_POINT('Ctrl Pts',(11.6076999192359,22.2921521480358,0.));
#210322=CARTESIAN_POINT('Ctrl Pts',(11.6286728270011,22.3075217249049,0.));
#210323=CARTESIAN_POINT('Ctrl Pts',(11.6497440449858,22.3228878043976,0.));
#210324=CARTESIAN_POINT('Ctrl Pts',(11.6709133432986,22.3382499035618,0.));
#210325=CARTESIAN_POINT('Ctrl Pts',(11.6921804934056,22.3536075450028,0.));
#210326=CARTESIAN_POINT('Ctrl Pts',(11.7135452684532,22.3689602575492,0.));
#210327=CARTESIAN_POINT('Ctrl Pts',(11.7350074437961,22.3843075773905,0.));
#210328=CARTESIAN_POINT('Ctrl Pts',(11.7565667964765,22.39964904692,0.));
#210329=CARTESIAN_POINT('Ctrl Pts',(11.7782231042041,22.4149842125018,0.));
#210330=CARTESIAN_POINT('Ctrl Pts',(11.7999761445175,22.4303126226468,0.));
#210331=CARTESIAN_POINT('Ctrl Pts',(11.8218256937889,22.4456338258738,0.));
#210332=CARTESIAN_POINT('Ctrl Pts',(11.8437715264487,22.4609473690469,0.));
#210333=CARTESIAN_POINT('Ctrl Pts',(11.8658134137018,22.4762527946694,0.));
#210334=CARTESIAN_POINT('Ctrl Pts',(11.8879511239941,22.4915496418472,0.));
#210335=CARTESIAN_POINT('Ctrl Pts',(11.9101844254555,22.5068374513958,0.));
#210336=CARTESIAN_POINT('Ctrl Pts',(11.9325130877801,22.5221157697869,0.));
#210337=CARTESIAN_POINT('Ctrl Pts',(11.9549368843996,22.5373841537299,0.));
#210338=CARTESIAN_POINT('Ctrl Pts',(11.9774555943496,22.5526421741159,0.));
#210339=CARTESIAN_POINT('Ctrl Pts',(12.0000690046697,22.5678894211194,0.));
#210340=CARTESIAN_POINT('Ctrl Pts',(12.0227769113132,22.5831255061306,0.));
#210341=CARTESIAN_POINT('Ctrl Pts',(12.0455791139135,22.5983500505675,0.));
#210342=CARTESIAN_POINT('Ctrl Pts',(12.0684754113869,22.613562676493,0.));
#210343=CARTESIAN_POINT('Ctrl Pts',(12.0914655972828,22.628762996708,0.));
#210344=CARTESIAN_POINT('Ctrl Pts',(12.1145494550384,22.6439506046611,0.));
#210345=CARTESIAN_POINT('Ctrl Pts',(12.1377267537141,22.6591250653942,0.));
#210346=CARTESIAN_POINT('Ctrl Pts',(12.1609972423088,22.6742859034891,0.));
#210347=CARTESIAN_POINT('Ctrl Pts',(12.1843606579246,22.6894326204959,0.));
#210348=CARTESIAN_POINT('Ctrl Pts',(12.2078167360267,22.7045647168659,0.));
#210349=CARTESIAN_POINT('Ctrl Pts',(12.2313652198047,22.7196817119299,0.));
#210350=CARTESIAN_POINT('Ctrl Pts',(12.2550058702389,22.7347831655251,0.));
#210351=CARTESIAN_POINT('Ctrl Pts',(12.2787384750747,22.7498686970096,0.));
#210352=CARTESIAN_POINT('Ctrl Pts',(12.3025628601811,22.7649380101154,0.));
#210353=CARTESIAN_POINT('Ctrl Pts',(12.3264788926108,22.7799908974947,0.));
#210354=CARTESIAN_POINT('Ctrl Pts',(12.3504864740361,22.7950272216959,0.));
#210355=CARTESIAN_POINT('Ctrl Pts',(12.3745855366772,22.8100469022632,0.));
#210356=CARTESIAN_POINT('Ctrl Pts',(12.393937937903,22.8220493007353,0.));
#210357=CARTESIAN_POINT('Ctrl Pts',(12.4084933766366,22.8310435872852,0.));
#210358=CARTESIAN_POINT('Ctrl Pts',(12.4182152851867,22.8370364396497,0.));
#210359=CARTESIAN_POINT('Ctrl Pts',(12.4230808101438,22.8400320311648,0.));
#210360=CARTESIAN_POINT('',(12.4230808101438,22.8400320311648,0.));
#210361=CARTESIAN_POINT('Origin',(13.9675290154577,16.3449727195352,0.));
#210362=CARTESIAN_POINT('',(14.6513681262571,17.1452095830633,0.));
#210363=CARTESIAN_POINT('',(14.6513681262571,17.1452095830633,0.));
#210364=CARTESIAN_POINT('',(6.98376450772883,8.17248635976757,0.));
#210365=CARTESIAN_POINT('Ctrl Pts',(13.5685075571671,22.1787195904339,0.));
#210366=CARTESIAN_POINT('Ctrl Pts',(13.5685075571671,22.1787195904339,12.));
#210367=CARTESIAN_POINT('Ctrl Pts',(13.5683460612913,22.1730081264583,0.));
#210368=CARTESIAN_POINT('Ctrl Pts',(13.5683460612913,22.1730081264583,12.));
#210369=CARTESIAN_POINT('Ctrl Pts',(13.5680170531724,22.1615922804939,0.));
#210370=CARTESIAN_POINT('Ctrl Pts',(13.5680170531724,22.1615922804939,12.));
#210371=CARTESIAN_POINT('Ctrl Pts',(13.5675054918922,22.1444897575076,0.));
#210372=CARTESIAN_POINT('Ctrl Pts',(13.5675054918922,22.1444897575076,12.));
#210373=CARTESIAN_POINT('Ctrl Pts',(13.5667873105179,22.1217288871823,0.));
#210374=CARTESIAN_POINT('Ctrl Pts',(13.5667873105179,22.1217288871823,12.));
#210375=CARTESIAN_POINT('Ctrl Pts',(13.5658294169106,22.0933486464442,0.));
#210376=CARTESIAN_POINT('Ctrl Pts',(13.5658294169106,22.0933486464442,12.));
#210377=CARTESIAN_POINT('Ctrl Pts',(13.5648113688894,22.0650393089492,0.));
#210378=CARTESIAN_POINT('Ctrl Pts',(13.5648113688894,22.0650393089492,12.));
#210379=CARTESIAN_POINT('Ctrl Pts',(13.5637332022393,22.0368009736227,0.));
#210380=CARTESIAN_POINT('Ctrl Pts',(13.5637332022393,22.0368009736227,12.));
#210381=CARTESIAN_POINT('Ctrl Pts',(13.5625949868313,22.0086337943431,0.));
#210382=CARTESIAN_POINT('Ctrl Pts',(13.5625949868313,22.0086337943431,12.));
#210383=CARTESIAN_POINT('Ctrl Pts',(13.5613968357589,21.9805379899192,0.));
#210384=CARTESIAN_POINT('Ctrl Pts',(13.5613968357589,21.9805379899192,12.));
#210385=CARTESIAN_POINT('Ctrl Pts',(13.5601389185315,21.9525138592862,0.));
#210386=CARTESIAN_POINT('Ctrl Pts',(13.5601389185315,21.9525138592862,12.));
#210387=CARTESIAN_POINT('Ctrl Pts',(13.5588214586672,21.9245617765827,0.));
#210388=CARTESIAN_POINT('Ctrl Pts',(13.5588214586672,21.9245617765827,12.));
#210389=CARTESIAN_POINT('Ctrl Pts',(13.5574447178484,21.8966821688876,0.));
#210390=CARTESIAN_POINT('Ctrl Pts',(13.5574447178484,21.8966821688876,12.));
#210391=CARTESIAN_POINT('Ctrl Pts',(13.5560089839426,21.8688754989401,0.));
#210392=CARTESIAN_POINT('Ctrl Pts',(13.5560089839426,21.8688754989401,12.));
#210393=CARTESIAN_POINT('Ctrl Pts',(13.5545145573048,21.841142245609,0.));
#210394=CARTESIAN_POINT('Ctrl Pts',(13.5545145573048,21.841142245609,12.));
#210395=CARTESIAN_POINT('Ctrl Pts',(13.5529617381569,21.8134828857963,0.));
#210396=CARTESIAN_POINT('Ctrl Pts',(13.5529617381569,21.8134828857963,12.));
#210397=CARTESIAN_POINT('Ctrl Pts',(13.5513508127232,21.7858978745848,0.));
#210398=CARTESIAN_POINT('Ctrl Pts',(13.5513508127232,21.7858978745848,12.));
#210399=CARTESIAN_POINT('Ctrl Pts',(13.5496820422186,21.7583876294532,0.));
#210400=CARTESIAN_POINT('Ctrl Pts',(13.5496820422186,21.7583876294532,12.));
#210401=CARTESIAN_POINT('Ctrl Pts',(13.5479556704457,21.730952541226,0.));
#210402=CARTESIAN_POINT('Ctrl Pts',(13.5479556704457,21.730952541226,12.));
#210403=CARTESIAN_POINT('Ctrl Pts',(13.546171929503,21.7035929822939,0.));
#210404=CARTESIAN_POINT('Ctrl Pts',(13.546171929503,21.7035929822939,12.));
#210405=CARTESIAN_POINT('Ctrl Pts',(13.5443310461516,21.676309315769,0.));
#210406=CARTESIAN_POINT('Ctrl Pts',(13.5443310461516,21.676309315769,12.));
#210407=CARTESIAN_POINT('Ctrl Pts',(13.5424332480698,21.6491019044647,0.));
#210408=CARTESIAN_POINT('Ctrl Pts',(13.5424332480698,21.6491019044647,12.));
#210409=CARTESIAN_POINT('Ctrl Pts',(13.5404787697798,21.6219711193951,0.));
#210410=CARTESIAN_POINT('Ctrl Pts',(13.5404787697798,21.6219711193951,12.));
#210411=CARTESIAN_POINT('Ctrl Pts',(13.5384678597206,21.5949173499022,0.));
#210412=CARTESIAN_POINT('Ctrl Pts',(13.5384678597206,21.5949173499022,12.));
#210413=CARTESIAN_POINT('Ctrl Pts',(13.5364007790292,21.5679410019011,0.));
#210414=CARTESIAN_POINT('Ctrl Pts',(13.5364007790292,21.5679410019011,12.));
#210415=CARTESIAN_POINT('Ctrl Pts',(13.5342777983225,21.5410424932511,0.));
#210416=CARTESIAN_POINT('Ctrl Pts',(13.5342777983225,21.5410424932511,12.));
#210417=CARTESIAN_POINT('Ctrl Pts',(13.5320991952145,21.5142222501671,0.));
#210418=CARTESIAN_POINT('Ctrl Pts',(13.5320991952145,21.5142222501671,12.));
#210419=CARTESIAN_POINT('Ctrl Pts',(13.5298652514357,21.487480703047,0.));
#210420=CARTESIAN_POINT('Ctrl Pts',(13.5298652514357,21.487480703047,12.));
#210421=CARTESIAN_POINT('Ctrl Pts',(13.5275762503553,21.4608182828695,0.));
#210422=CARTESIAN_POINT('Ctrl Pts',(13.5275762503553,21.4608182828695,12.));
#210423=CARTESIAN_POINT('Ctrl Pts',(13.5252324737795,21.4342354165254,0.));
#210424=CARTESIAN_POINT('Ctrl Pts',(13.5252324737795,21.4342354165254,12.));
#210425=CARTESIAN_POINT('Ctrl Pts',(13.5228342013508,21.4077325259318,0.));
#210426=CARTESIAN_POINT('Ctrl Pts',(13.5228342013508,21.4077325259318,12.));
#210427=CARTESIAN_POINT('Ctrl Pts',(13.5203817122496,21.3813100304967,0.));
#210428=CARTESIAN_POINT('Ctrl Pts',(13.5203817122496,21.3813100304967,12.));
#210429=CARTESIAN_POINT('Ctrl Pts',(13.5178752862461,21.3549683486219,0.));
#210430=CARTESIAN_POINT('Ctrl Pts',(13.5178752862461,21.3549683486219,12.));
#210431=CARTESIAN_POINT('Ctrl Pts',(13.5153152050554,21.328707899634,0.));
#210432=CARTESIAN_POINT('Ctrl Pts',(13.5153152050554,21.328707899634,12.));
#210433=CARTESIAN_POINT('Ctrl Pts',(13.5127017534972,21.3025291054236,0.));
#210434=CARTESIAN_POINT('Ctrl Pts',(13.5127017534972,21.3025291054236,12.));
#210435=CARTESIAN_POINT('Ctrl Pts',(13.5100352209207,21.2764323924442,0.));
#210436=CARTESIAN_POINT('Ctrl Pts',(13.5100352209207,21.2764323924442,12.));
#210437=CARTESIAN_POINT('Ctrl Pts',(13.5073159019454,21.2504181927429,0.));
#210438=CARTESIAN_POINT('Ctrl Pts',(13.5073159019454,21.2504181927429,12.));
#210439=CARTESIAN_POINT('Ctrl Pts',(13.5045440957404,21.224486942933,0.));
#210440=CARTESIAN_POINT('Ctrl Pts',(13.5045440957404,21.224486942933,12.));
#210441=CARTESIAN_POINT('Ctrl Pts',(13.5017201056088,21.1986390835825,0.));
#210442=CARTESIAN_POINT('Ctrl Pts',(13.5017201056088,21.1986390835825,12.));
#210443=CARTESIAN_POINT('Ctrl Pts',(13.4988442384491,21.1728750584173,0.));
#210444=CARTESIAN_POINT('Ctrl Pts',(13.4988442384491,21.1728750584173,12.));
#210445=CARTESIAN_POINT('Ctrl Pts',(13.4959168042934,21.1471953136209,0.));
#210446=CARTESIAN_POINT('Ctrl Pts',(13.4959168042934,21.1471953136209,12.));
#210447=CARTESIAN_POINT('Ctrl Pts',(13.4929381157778,21.1216002970209,0.));
#210448=CARTESIAN_POINT('Ctrl Pts',(13.4929381157778,21.1216002970209,12.));
#210449=CARTESIAN_POINT('Ctrl Pts',(13.4899084877718,21.0960904575048,0.));
#210450=CARTESIAN_POINT('Ctrl Pts',(13.4899084877718,21.0960904575048,12.));
#210451=CARTESIAN_POINT('Ctrl Pts',(13.4868282377191,21.0706662455202,0.));
#210452=CARTESIAN_POINT('Ctrl Pts',(13.4868282377191,21.0706662455202,12.));
#210453=CARTESIAN_POINT('Ctrl Pts',(13.4836976858912,21.0453281134247,0.));
#210454=CARTESIAN_POINT('Ctrl Pts',(13.4836976858912,21.0453281134247,12.));
#210455=CARTESIAN_POINT('Ctrl Pts',(13.4805171556822,21.0200765158885,0.));
#210456=CARTESIAN_POINT('Ctrl Pts',(13.4805171556822,21.0200765158885,12.));
#210457=CARTESIAN_POINT('Ctrl Pts',(13.4772869738879,20.9949119102592,0.));
#210458=CARTESIAN_POINT('Ctrl Pts',(13.4772869738879,20.9949119102592,12.));
#210459=CARTESIAN_POINT('Ctrl Pts',(13.4740074710087,20.9698347569476,0.));
#210460=CARTESIAN_POINT('Ctrl Pts',(13.4740074710087,20.9698347569476,12.));
#210461=CARTESIAN_POINT('Ctrl Pts',(13.4706789815166,20.9448455197557,0.));
#210462=CARTESIAN_POINT('Ctrl Pts',(13.4706789815166,20.9448455197557,12.));
#210463=CARTESIAN_POINT('Ctrl Pts',(13.4673018437718,20.9199446657584,0.));
#210464=CARTESIAN_POINT('Ctrl Pts',(13.4673018437718,20.9199446657584,12.));
#210465=CARTESIAN_POINT('Ctrl Pts',(13.4638763999725,20.8951326652158,0.));
#210466=CARTESIAN_POINT('Ctrl Pts',(13.4638763999725,20.8951326652158,12.));
#210467=CARTESIAN_POINT('Ctrl Pts',(13.4604029960983,20.8704099914641,0.));
#210468=CARTESIAN_POINT('Ctrl Pts',(13.4604029960983,20.8704099914641,12.));
#210469=CARTESIAN_POINT('Ctrl Pts',(13.4568819818631,20.8457771208082,0.));
#210470=CARTESIAN_POINT('Ctrl Pts',(13.4568819818631,20.8457771208082,12.));
#210471=CARTESIAN_POINT('Ctrl Pts',(13.4533137106667,20.821234532398,0.));
#210472=CARTESIAN_POINT('Ctrl Pts',(13.4533137106667,20.821234532398,12.));
#210473=CARTESIAN_POINT('Ctrl Pts',(13.4496985395637,20.7967827081227,0.));
#210474=CARTESIAN_POINT('Ctrl Pts',(13.4496985395637,20.7967827081227,12.));
#210475=CARTESIAN_POINT('Ctrl Pts',(13.4460368293688,20.7724221327608,0.));
#210476=CARTESIAN_POINT('Ctrl Pts',(13.4460368293688,20.7724221327608,12.));
#210477=CARTESIAN_POINT('Ctrl Pts',(13.4423289447561,20.7481532941013,0.));
#210478=CARTESIAN_POINT('Ctrl Pts',(13.4423289447561,20.7481532941013,12.));
#210479=CARTESIAN_POINT('Ctrl Pts',(13.4385752543663,20.7239766830675,0.));
#210480=CARTESIAN_POINT('Ctrl Pts',(13.4385752543663,20.7239766830675,12.));
#210481=CARTESIAN_POINT('Ctrl Pts',(13.4347761309154,20.6998927938288,0.));
#210482=CARTESIAN_POINT('Ctrl Pts',(13.4347761309154,20.6998927938288,12.));
#210483=CARTESIAN_POINT('Ctrl Pts',(13.4309319513119,20.6759021239103,0.));
#210484=CARTESIAN_POINT('Ctrl Pts',(13.4309319513119,20.6759021239103,12.));
#210485=CARTESIAN_POINT('Ctrl Pts',(13.4270430967651,20.6520051742869,0.));
#210486=CARTESIAN_POINT('Ctrl Pts',(13.4270430967651,20.6520051742869,12.));
#210487=CARTESIAN_POINT('Ctrl Pts',(13.4231099528179,20.6282024494237,0.));
#210488=CARTESIAN_POINT('Ctrl Pts',(13.4231099528179,20.6282024494237,12.));
#210489=CARTESIAN_POINT('Ctrl Pts',(13.4191329093932,20.6044944573153,0.));
#210490=CARTESIAN_POINT('Ctrl Pts',(13.4191329093932,20.6044944573153,12.));
#210491=CARTESIAN_POINT('Ctrl Pts',(13.4151123608411,20.5808817095155,0.));
#210492=CARTESIAN_POINT('Ctrl Pts',(13.4151123608411,20.5808817095155,12.));
#210493=CARTESIAN_POINT('Ctrl Pts',(13.4110487059912,20.5573647211639,0.));
#210494=CARTESIAN_POINT('Ctrl Pts',(13.4110487059912,20.5573647211639,12.));
#210495=CARTESIAN_POINT('Ctrl Pts',(13.4069423482076,20.5339440109956,0.));
#210496=CARTESIAN_POINT('Ctrl Pts',(13.4069423482076,20.5339440109956,12.));
#210497=CARTESIAN_POINT('Ctrl Pts',(13.4027936954529,20.5106201013753,0.));
#210498=CARTESIAN_POINT('Ctrl Pts',(13.4027936954529,20.5106201013753,12.));
#210499=CARTESIAN_POINT('Ctrl Pts',(13.3986031603716,20.487393518404,0.));
#210500=CARTESIAN_POINT('Ctrl Pts',(13.3986031603716,20.487393518404,12.));
#210501=CARTESIAN_POINT('Ctrl Pts',(13.3943711603739,20.4642647920038,0.));
#210502=CARTESIAN_POINT('Ctrl Pts',(13.3943711603739,20.4642647920038,12.));
#210503=CARTESIAN_POINT('Ctrl Pts',(13.3900981177255,20.4412344560008,0.));
#210504=CARTESIAN_POINT('Ctrl Pts',(13.3900981177255,20.4412344560008,12.));
#210505=CARTESIAN_POINT('Ctrl Pts',(13.3857844596387,20.4183030482002,0.));
#210506=CARTESIAN_POINT('Ctrl Pts',(13.3857844596387,20.4183030482002,12.));
#210507=CARTESIAN_POINT('Ctrl Pts',(13.3814306183719,20.3954711104502,0.));
#210508=CARTESIAN_POINT('Ctrl Pts',(13.3814306183719,20.3954711104502,12.));
#210509=CARTESIAN_POINT('Ctrl Pts',(13.3770370313188,20.3727391887184,0.));
#210510=CARTESIAN_POINT('Ctrl Pts',(13.3770370313188,20.3727391887184,12.));
#210511=CARTESIAN_POINT('Ctrl Pts',(13.3726041410867,20.3501078331814,0.));
#210512=CARTESIAN_POINT('Ctrl Pts',(13.3726041410867,20.3501078331814,12.));
#210513=CARTESIAN_POINT('Ctrl Pts',(13.3681323955826,20.3275775983029,0.));
#210514=CARTESIAN_POINT('Ctrl Pts',(13.3681323955826,20.3275775983029,12.));
#210515=CARTESIAN_POINT('Ctrl Pts',(13.3636222481016,20.3051490429048,0.));
#210516=CARTESIAN_POINT('Ctrl Pts',(13.3636222481016,20.3051490429048,12.));
#210517=CARTESIAN_POINT('Ctrl Pts',(13.3590741574195,20.2828227302339,0.));
#210518=CARTESIAN_POINT('Ctrl Pts',(13.3590741574195,20.2828227302339,12.));
#210519=CARTESIAN_POINT('Ctrl Pts',(13.3544885878889,20.2605992280122,0.));
#210520=CARTESIAN_POINT('Ctrl Pts',(13.3544885878889,20.2605992280122,12.));
#210521=CARTESIAN_POINT('Ctrl Pts',(13.3498660095386,20.2384791085359,0.));
#210522=CARTESIAN_POINT('Ctrl Pts',(13.3498660095386,20.2384791085359,12.));
#210523=CARTESIAN_POINT('Ctrl Pts',(13.3452068981766,20.216462948786,0.));
#210524=CARTESIAN_POINT('Ctrl Pts',(13.3452068981766,20.216462948786,12.));
#210525=CARTESIAN_POINT('Ctrl Pts',(13.3405117354971,20.1945513305235,0.));
#210526=CARTESIAN_POINT('Ctrl Pts',(13.3405117354971,20.1945513305235,12.));
#210527=CARTESIAN_POINT('Ctrl Pts',(13.3357810091903,20.1727448403817,0.));
#210528=CARTESIAN_POINT('Ctrl Pts',(13.3357810091903,20.1727448403817,12.));
#210529=CARTESIAN_POINT('Ctrl Pts',(13.3310152130564,20.1510440699474,0.));
#210530=CARTESIAN_POINT('Ctrl Pts',(13.3310152130564,20.1510440699474,12.));
#210531=CARTESIAN_POINT('Ctrl Pts',(13.3262148471226,20.1294496158402,0.));
#210532=CARTESIAN_POINT('Ctrl Pts',(13.3262148471226,20.1294496158402,12.));
#210533=CARTESIAN_POINT('Ctrl Pts',(13.3213804177587,20.1079620798375,0.));
#210534=CARTESIAN_POINT('Ctrl Pts',(13.3213804177587,20.1079620798375,12.));
#210535=CARTESIAN_POINT('Ctrl Pts',(13.3165124377962,20.0865820689883,0.));
#210536=CARTESIAN_POINT('Ctrl Pts',(13.3165124377962,20.0865820689883,12.));
#210537=CARTESIAN_POINT('Ctrl Pts',(13.3116114266515,20.0653101957188,0.));
#210538=CARTESIAN_POINT('Ctrl Pts',(13.3116114266515,20.0653101957188,12.));
#210539=CARTESIAN_POINT('Ctrl Pts',(13.3066779104515,20.0441470779345,0.));
#210540=CARTESIAN_POINT('Ctrl Pts',(13.3066779104515,20.0441470779345,12.));
#210541=CARTESIAN_POINT('Ctrl Pts',(13.3017124221637,20.0230933391038,0.));
#210542=CARTESIAN_POINT('Ctrl Pts',(13.3017124221637,20.0230933391038,12.));
#210543=CARTESIAN_POINT('Ctrl Pts',(13.2967155017306,20.0021496083738,0.));
#210544=CARTESIAN_POINT('Ctrl Pts',(13.2967155017306,20.0021496083738,12.));
#210545=CARTESIAN_POINT('Ctrl Pts',(13.2916876962094,19.981316520717,0.));
#210546=CARTESIAN_POINT('Ctrl Pts',(13.2916876962094,19.981316520717,12.));
#210547=CARTESIAN_POINT('Ctrl Pts',(13.286629559915,19.9605947170586,0.));
#210548=CARTESIAN_POINT('Ctrl Pts',(13.286629559915,19.9605947170586,12.));
#210549=CARTESIAN_POINT('Ctrl Pts',(13.2815416545663,19.9399848444019,0.));
#210550=CARTESIAN_POINT('Ctrl Pts',(13.2815416545663,19.9399848444019,12.));
#210551=CARTESIAN_POINT('Ctrl Pts',(13.2764245494357,19.9194875559422,0.));
#210552=CARTESIAN_POINT('Ctrl Pts',(13.2764245494357,19.9194875559422,12.));
#210553=CARTESIAN_POINT('Ctrl Pts',(13.271278821502,19.8991035111745,0.));
#210554=CARTESIAN_POINT('Ctrl Pts',(13.271278821502,19.8991035111745,12.));
#210555=CARTESIAN_POINT('Ctrl Pts',(13.2661050556132,19.8788333760577,0.));
#210556=CARTESIAN_POINT('Ctrl Pts',(13.2661050556132,19.8788333760577,12.));
#210557=CARTESIAN_POINT('Ctrl Pts',(13.2609038446529,19.8586778231715,0.));
#210558=CARTESIAN_POINT('Ctrl Pts',(13.2609038446529,19.8586778231715,12.));
#210559=CARTESIAN_POINT('Ctrl Pts',(13.2556757897086,19.8386375318634,0.));
#210560=CARTESIAN_POINT('Ctrl Pts',(13.2556757897086,19.8386375318634,12.));
#210561=CARTESIAN_POINT('Ctrl Pts',(13.2504215002457,19.8187131883917,0.));
#210562=CARTESIAN_POINT('Ctrl Pts',(13.2504215002457,19.8187131883917,12.));
#210563=CARTESIAN_POINT('Ctrl Pts',(13.2451415942805,19.7989054860495,0.));
#210564=CARTESIAN_POINT('Ctrl Pts',(13.2451415942805,19.7989054860495,12.));
#210565=CARTESIAN_POINT('Ctrl Pts',(13.2398366985675,19.7792151253289,0.));
#210566=CARTESIAN_POINT('Ctrl Pts',(13.2398366985675,19.7792151253289,12.));
#210567=CARTESIAN_POINT('Ctrl Pts',(13.2345074487963,19.7596428141168,0.));
#210568=CARTESIAN_POINT('Ctrl Pts',(13.2345074487963,19.7596428141168,12.));
#210569=CARTESIAN_POINT('Ctrl Pts',(13.2291544897899,19.7401892678697,0.));
#210570=CARTESIAN_POINT('Ctrl Pts',(13.2291544897899,19.7401892678697,12.));
#210571=CARTESIAN_POINT('Ctrl Pts',(13.2237784757065,19.7208552097868,0.));
#210572=CARTESIAN_POINT('Ctrl Pts',(13.2237784757065,19.7208552097868,12.));
#210573=CARTESIAN_POINT('Ctrl Pts',(13.2183800702436,19.7016413709685,0.));
#210574=CARTESIAN_POINT('Ctrl Pts',(13.2183800702436,19.7016413709685,12.));
#210575=CARTESIAN_POINT('Ctrl Pts',(13.2129599468485,19.6825484905823,0.));
#210576=CARTESIAN_POINT('Ctrl Pts',(13.2129599468485,19.6825484905823,12.));
#210577=CARTESIAN_POINT('Ctrl Pts',(13.2075187889529,19.6635773160936,0.));
#210578=CARTESIAN_POINT('Ctrl Pts',(13.2075187889529,19.6635773160936,12.));
#210579=CARTESIAN_POINT('Ctrl Pts',(13.2020572902065,19.6447286034772,0.));
#210580=CARTESIAN_POINT('Ctrl Pts',(13.2020572902065,19.6447286034772,12.));
#210581=CARTESIAN_POINT('Ctrl Pts',(13.1965761547151,19.6260031174244,0.));
#210582=CARTESIAN_POINT('Ctrl Pts',(13.1965761547151,19.6260031174244,12.));
#210583=CARTESIAN_POINT('Ctrl Pts',(13.1910760972814,19.6074016315414,0.));
#210584=CARTESIAN_POINT('Ctrl Pts',(13.1910760972814,19.6074016315414,12.));
#210585=CARTESIAN_POINT('Ctrl Pts',(13.1855578436471,19.5889249285338,0.));
#210586=CARTESIAN_POINT('Ctrl Pts',(13.1855578436471,19.5889249285338,12.));
#210587=CARTESIAN_POINT('Ctrl Pts',(13.1800221307673,19.5705738004667,0.));
#210588=CARTESIAN_POINT('Ctrl Pts',(13.1800221307673,19.5705738004667,12.));
#210589=CARTESIAN_POINT('Ctrl Pts',(13.1744697070911,19.5523490490244,0.));
#210590=CARTESIAN_POINT('Ctrl Pts',(13.1744697070911,19.5523490490244,12.));
#210591=CARTESIAN_POINT('Ctrl Pts',(13.168901332843,19.5342514857562,0.));
#210592=CARTESIAN_POINT('Ctrl Pts',(13.168901332843,19.5342514857562,12.));
#210593=CARTESIAN_POINT('Ctrl Pts',(13.1633177803101,19.5162819323213,0.));
#210594=CARTESIAN_POINT('Ctrl Pts',(13.1633177803101,19.5162819323213,12.));
#210595=CARTESIAN_POINT('Ctrl Pts',(13.1577198341245,19.4984412207082,0.));
#210596=CARTESIAN_POINT('Ctrl Pts',(13.1577198341245,19.4984412207082,12.));
#210597=CARTESIAN_POINT('Ctrl Pts',(13.1521082915853,19.4807301935268,0.));
#210598=CARTESIAN_POINT('Ctrl Pts',(13.1521082915853,19.4807301935268,12.));
#210599=CARTESIAN_POINT('Ctrl Pts',(13.1464839629971,19.4631497043258,0.));
#210600=CARTESIAN_POINT('Ctrl Pts',(13.1464839629971,19.4631497043258,12.));
#210601=CARTESIAN_POINT('Ctrl Pts',(13.1408476720061,19.4457006178876,0.));
#210602=CARTESIAN_POINT('Ctrl Pts',(13.1408476720061,19.4457006178876,12.));
#210603=CARTESIAN_POINT('Ctrl Pts',(13.1352002559438,19.4283838105262,0.));
#210604=CARTESIAN_POINT('Ctrl Pts',(13.1352002559438,19.4283838105262,12.));
#210605=CARTESIAN_POINT('Ctrl Pts',(13.1295425661634,19.4112001703557,0.));
#210606=CARTESIAN_POINT('Ctrl Pts',(13.1295425661634,19.4112001703557,12.));
#210607=CARTESIAN_POINT('Ctrl Pts',(13.1238754684177,19.3941505976263,0.));
#210608=CARTESIAN_POINT('Ctrl Pts',(13.1238754684177,19.3941505976263,12.));
#210609=CARTESIAN_POINT('Ctrl Pts',(13.118199843271,19.3772360051091,0.));
#210610=CARTESIAN_POINT('Ctrl Pts',(13.118199843271,19.3772360051091,12.));
#210611=CARTESIAN_POINT('Ctrl Pts',(13.1125165865022,19.3604573184515,0.));
#210612=CARTESIAN_POINT('Ctrl Pts',(13.1125165865022,19.3604573184515,12.));
#210613=CARTESIAN_POINT('Ctrl Pts',(13.1068266095186,19.3438154765395,0.));
#210614=CARTESIAN_POINT('Ctrl Pts',(13.1068266095186,19.3438154765395,12.));
#210615=CARTESIAN_POINT('Ctrl Pts',(13.1011308397591,19.3273114318269,0.));
#210616=CARTESIAN_POINT('Ctrl Pts',(13.1011308397591,19.3273114318269,12.));
#210617=CARTESIAN_POINT('Ctrl Pts',(13.0954302211479,19.310946150736,0.));
#210618=CARTESIAN_POINT('Ctrl Pts',(13.0954302211479,19.310946150736,12.));
#210619=CARTESIAN_POINT('Ctrl Pts',(13.0897257145968,19.2947206141247,0.));
#210620=CARTESIAN_POINT('Ctrl Pts',(13.0897257145968,19.2947206141247,12.));
#210621=CARTESIAN_POINT('Ctrl Pts',(13.0840182984949,19.2786358177198,0.));
#210622=CARTESIAN_POINT('Ctrl Pts',(13.0840182984949,19.2786358177198,12.));
#210623=CARTESIAN_POINT('Ctrl Pts',(13.0783089692118,19.2626927725596,0.));
#210624=CARTESIAN_POINT('Ctrl Pts',(13.0783089692118,19.2626927725596,12.));
#210625=CARTESIAN_POINT('Ctrl Pts',(13.0725987415859,19.2468925053989,0.));
#210626=CARTESIAN_POINT('Ctrl Pts',(13.0725987415859,19.2468925053989,12.));
#210627=CARTESIAN_POINT('Ctrl Pts',(13.0668886494795,19.2312360592033,0.));
#210628=CARTESIAN_POINT('Ctrl Pts',(13.0668886494795,19.2312360592033,12.));
#210629=CARTESIAN_POINT('Ctrl Pts',(13.0611797463915,19.2157244937142,0.));
#210630=CARTESIAN_POINT('Ctrl Pts',(13.0611797463915,19.2157244937142,12.));
#210631=CARTESIAN_POINT('Ctrl Pts',(13.0554731060538,19.2003588859772,0.));
#210632=CARTESIAN_POINT('Ctrl Pts',(13.0554731060538,19.2003588859772,12.));
#210633=CARTESIAN_POINT('Ctrl Pts',(13.0497698230441,19.1851403308825,0.));
#210634=CARTESIAN_POINT('Ctrl Pts',(13.0497698230441,19.1851403308825,12.));
#210635=CARTESIAN_POINT('Ctrl Pts',(13.0440710133772,19.1700699416622,0.));
#210636=CARTESIAN_POINT('Ctrl Pts',(13.0440710133772,19.1700699416622,12.));
#210637=CARTESIAN_POINT('Ctrl Pts',(13.0383778152068,19.155148850523,0.));
#210638=CARTESIAN_POINT('Ctrl Pts',(13.0383778152068,19.155148850523,12.));
#210639=CARTESIAN_POINT('Ctrl Pts',(13.0326913895838,19.1403782093386,0.));
#210640=CARTESIAN_POINT('Ctrl Pts',(13.0326913895838,19.1403782093386,12.));
#210641=CARTESIAN_POINT('Ctrl Pts',(13.0270129211976,19.1257591903099,0.));
#210642=CARTESIAN_POINT('Ctrl Pts',(13.0270129211976,19.1257591903099,12.));
#210643=CARTESIAN_POINT('Ctrl Pts',(13.0213436191328,19.111292986631,0.));
#210644=CARTESIAN_POINT('Ctrl Pts',(13.0213436191328,19.111292986631,12.));
#210645=CARTESIAN_POINT('Ctrl Pts',(13.0156847176096,19.0969808131228,0.));
#210646=CARTESIAN_POINT('Ctrl Pts',(13.0156847176096,19.0969808131228,12.));
#210647=CARTESIAN_POINT('Ctrl Pts',(13.0100374768788,19.0828239070484,0.));
#210648=CARTESIAN_POINT('Ctrl Pts',(13.0100374768788,19.0828239070484,12.));
#210649=CARTESIAN_POINT('Ctrl Pts',(13.0044031841382,19.0688235289437,0.));
#210650=CARTESIAN_POINT('Ctrl Pts',(13.0044031841382,19.0688235289437,12.));
#210651=CARTESIAN_POINT('Ctrl Pts',(12.9987831544502,19.0549809634354,0.));
#210652=CARTESIAN_POINT('Ctrl Pts',(12.9987831544502,19.0549809634354,12.));
#210653=CARTESIAN_POINT('Ctrl Pts',(12.9931787316514,19.0412975200398,0.));
#210654=CARTESIAN_POINT('Ctrl Pts',(12.9931787316514,19.0412975200398,12.));
#210655=CARTESIAN_POINT('Ctrl Pts',(12.9875912893003,19.0277745339909,0.));
#210656=CARTESIAN_POINT('Ctrl Pts',(12.9875912893003,19.0277745339909,12.));
#210657=CARTESIAN_POINT('Ctrl Pts',(12.9820222318716,19.014413367335,0.));
#210658=CARTESIAN_POINT('Ctrl Pts',(12.9820222318716,19.014413367335,12.));
#210659=CARTESIAN_POINT('Ctrl Pts',(12.9764729959206,19.0012154099792,0.));
#210660=CARTESIAN_POINT('Ctrl Pts',(12.9764729959206,19.0012154099792,12.));
#210661=CARTESIAN_POINT('Ctrl Pts',(12.9709450512747,18.9881820807585,0.));
#210662=CARTESIAN_POINT('Ctrl Pts',(12.9709450512747,18.9881820807585,12.));
#210663=CARTESIAN_POINT('Ctrl Pts',(12.9654399021868,18.9753148284473,0.));
#210664=CARTESIAN_POINT('Ctrl Pts',(12.9654399021868,18.9753148284473,12.));
#210665=CARTESIAN_POINT('Ctrl Pts',(12.9599590886317,18.9626151329226,0.));
#210666=CARTESIAN_POINT('Ctrl Pts',(12.9599590886317,18.9626151329226,12.));
#210667=CARTESIAN_POINT('Ctrl Pts',(12.9545041877377,18.9500845064714,0.));
#210668=CARTESIAN_POINT('Ctrl Pts',(12.9545041877377,18.9500845064714,12.));
#210669=CARTESIAN_POINT('Ctrl Pts',(12.9490768151821,18.9377244950435,0.));
#210670=CARTESIAN_POINT('Ctrl Pts',(12.9490768151821,18.9377244950435,12.));
#210671=CARTESIAN_POINT('Ctrl Pts',(12.9436786266106,18.9255366795196,0.));
#210672=CARTESIAN_POINT('Ctrl Pts',(12.9436786266106,18.9255366795196,12.));
#210673=CARTESIAN_POINT('Ctrl Pts',(12.9383113190375,18.9135226769466,0.));
#210674=CARTESIAN_POINT('Ctrl Pts',(12.9383113190375,18.9135226769466,12.));
#210675=CARTESIAN_POINT('Ctrl Pts',(12.9329766328184,18.9016841423402,0.));
#210676=CARTESIAN_POINT('Ctrl Pts',(12.9329766328184,18.9016841423402,12.));
#210677=CARTESIAN_POINT('Ctrl Pts',(12.9276763536372,18.8900227704888,0.));
#210678=CARTESIAN_POINT('Ctrl Pts',(12.9276763536372,18.8900227704888,12.));
#210679=CARTESIAN_POINT('Ctrl Pts',(12.9224123144982,18.8785402977528,0.));
#210680=CARTESIAN_POINT('Ctrl Pts',(12.9224123144982,18.8785402977528,12.));
#210681=CARTESIAN_POINT('Ctrl Pts',(12.9171863977047,18.8672385038328,0.));
#210682=CARTESIAN_POINT('Ctrl Pts',(12.9171863977047,18.8672385038328,12.));
#210683=CARTESIAN_POINT('Ctrl Pts',(12.9120005369066,18.8561192136201,0.));
#210684=CARTESIAN_POINT('Ctrl Pts',(12.9120005369066,18.8561192136201,12.));
#210685=CARTESIAN_POINT('Ctrl Pts',(12.9068567191856,18.8451842990986,0.));
#210686=CARTESIAN_POINT('Ctrl Pts',(12.9068567191856,18.8451842990986,12.));
#210687=CARTESIAN_POINT('Ctrl Pts',(12.9017569871738,18.834435681259,0.));
#210688=CARTESIAN_POINT('Ctrl Pts',(12.9017569871738,18.834435681259,12.));
#210689=CARTESIAN_POINT('Ctrl Pts',(12.8967034410752,18.8238753319124,0.));
#210690=CARTESIAN_POINT('Ctrl Pts',(12.8967034410752,18.8238753319124,12.));
#210691=CARTESIAN_POINT('Ctrl Pts',(12.8916982409931,18.8135052757815,0.));
#210692=CARTESIAN_POINT('Ctrl Pts',(12.8916982409931,18.8135052757815,12.));
#210693=CARTESIAN_POINT('Ctrl Pts',(12.8867436109543,18.8033275941939,0.));
#210694=CARTESIAN_POINT('Ctrl Pts',(12.8867436109543,18.8033275941939,12.));
#210695=CARTESIAN_POINT('Ctrl Pts',(12.8818418427474,18.7933444285867,0.));
#210696=CARTESIAN_POINT('Ctrl Pts',(12.8818418427474,18.7933444285867,12.));
#210697=CARTESIAN_POINT('Ctrl Pts',(12.8769952998097,18.7835579840481,0.));
#210698=CARTESIAN_POINT('Ctrl Pts',(12.8769952998097,18.7835579840481,12.));
#210699=CARTESIAN_POINT('Ctrl Pts',(12.8722064211814,18.7739705329029,0.));
#210700=CARTESIAN_POINT('Ctrl Pts',(12.8722064211814,18.7739705329029,12.));
#210701=CARTESIAN_POINT('Ctrl Pts',(12.8674777239656,18.7645844169568,0.));
#210702=CARTESIAN_POINT('Ctrl Pts',(12.8674777239656,18.7645844169568,12.));
#210703=CARTESIAN_POINT('Ctrl Pts',(12.8628118054172,18.7554020493888,0.));
#210704=CARTESIAN_POINT('Ctrl Pts',(12.8628118054172,18.7554020493888,12.));
#210705=CARTESIAN_POINT('Ctrl Pts',(12.8582113455644,18.7464259171248,0.));
#210706=CARTESIAN_POINT('Ctrl Pts',(12.8582113455644,18.7464259171248,12.));
#210707=CARTESIAN_POINT('Ctrl Pts',(12.8536791086315,18.7376585820851,0.));
#210708=CARTESIAN_POINT('Ctrl Pts',(12.8536791086315,18.7376585820851,12.));
#210709=CARTESIAN_POINT('Ctrl Pts',(12.849217951159,18.7291026886552,0.));
#210710=CARTESIAN_POINT('Ctrl Pts',(12.849217951159,18.7291026886552,12.));
#210711=CARTESIAN_POINT('Ctrl Pts',(12.8448308329494,18.7207609737701,0.));
#210712=CARTESIAN_POINT('Ctrl Pts',(12.8448308329494,18.7207609737701,12.));
#210713=CARTESIAN_POINT('Ctrl Pts',(12.8405208263432,18.7126362754446,0.));
#210714=CARTESIAN_POINT('Ctrl Pts',(12.8405208263432,18.7126362754446,12.));
#210715=CARTESIAN_POINT('Ctrl Pts',(12.8362911280362,18.7047315436296,0.));
#210716=CARTESIAN_POINT('Ctrl Pts',(12.8362911280362,18.7047315436296,12.));
#210717=CARTESIAN_POINT('Ctrl Pts',(12.832145059979,18.6970498410173,0.));
#210718=CARTESIAN_POINT('Ctrl Pts',(12.832145059979,18.6970498410173,12.));
#210719=CARTESIAN_POINT('Ctrl Pts',(12.8280860635231,18.6895943376172,0.));
#210720=CARTESIAN_POINT('Ctrl Pts',(12.8280860635231,18.6895943376172,12.));
#210721=CARTESIAN_POINT('Ctrl Pts',(12.8241176980016,18.6823683094139,0.));
#210722=CARTESIAN_POINT('Ctrl Pts',(12.8241176980016,18.6823683094139,12.));
#210723=CARTESIAN_POINT('Ctrl Pts',(12.8202436318473,18.6753751301091,0.));
#210724=CARTESIAN_POINT('Ctrl Pts',(12.8202436318473,18.6753751301091,12.));
#210725=CARTESIAN_POINT('Ctrl Pts',(12.8164676687361,18.6686182952798,0.));
#210726=CARTESIAN_POINT('Ctrl Pts',(12.8164676687361,18.6686182952798,12.));
#210727=CARTESIAN_POINT('Ctrl Pts',(12.8127937909632,18.6621014624746,0.));
#210728=CARTESIAN_POINT('Ctrl Pts',(12.8127937909632,18.6621014624746,12.));
#210729=CARTESIAN_POINT('Ctrl Pts',(12.8092261933858,18.6558284825772,0.));
#210730=CARTESIAN_POINT('Ctrl Pts',(12.8092261933858,18.6558284825772,12.));
#210731=CARTESIAN_POINT('Ctrl Pts',(12.805769331162,18.6498034438986,0.));
#210732=CARTESIAN_POINT('Ctrl Pts',(12.805769331162,18.6498034438986,12.));
#210733=CARTESIAN_POINT('Ctrl Pts',(12.8024278770153,18.6440306327457,0.));
#210734=CARTESIAN_POINT('Ctrl Pts',(12.8024278770153,18.6440306327457,12.));
#210735=CARTESIAN_POINT('Ctrl Pts',(12.7992066625264,18.63851447924,0.));
#210736=CARTESIAN_POINT('Ctrl Pts',(12.7992066625264,18.63851447924,12.));
#210737=CARTESIAN_POINT('Ctrl Pts',(12.7961106222251,18.6332595057005,0.));
#210738=CARTESIAN_POINT('Ctrl Pts',(12.7961106222251,18.6332595057005,12.));
#210739=CARTESIAN_POINT('Ctrl Pts',(12.7931447451556,18.6282702819371,0.));
#210740=CARTESIAN_POINT('Ctrl Pts',(12.7931447451556,18.6282702819371,12.));
#210741=CARTESIAN_POINT('Ctrl Pts',(12.7903142925234,18.6235516265575,0.));
#210742=CARTESIAN_POINT('Ctrl Pts',(12.7903142925234,18.6235516265575,12.));
#210743=CARTESIAN_POINT('Ctrl Pts',(12.7876249657834,18.6191087624752,0.));
#210744=CARTESIAN_POINT('Ctrl Pts',(12.7876249657834,18.6191087624752,12.));
#210745=CARTESIAN_POINT('Ctrl Pts',(12.78508316579,18.6149475565189,0.));
#210746=CARTESIAN_POINT('Ctrl Pts',(12.78508316579,18.6149475565189,12.));
#210747=CARTESIAN_POINT('Ctrl Pts',(12.7826959526924,18.611074482622,0.));
#210748=CARTESIAN_POINT('Ctrl Pts',(12.7826959526924,18.611074482622,12.));
#210749=CARTESIAN_POINT('Ctrl Pts',(12.7804705387658,18.6074961535723,0.));
#210750=CARTESIAN_POINT('Ctrl Pts',(12.7804705387658,18.6074961535723,12.));
#210751=CARTESIAN_POINT('Ctrl Pts',(12.7784139605067,18.6042190183703,0.));
#210752=CARTESIAN_POINT('Ctrl Pts',(12.7784139605067,18.6042190183703,12.));
#210753=CARTESIAN_POINT('Ctrl Pts',(12.7765325225082,18.6012488486708,0.));
#210754=CARTESIAN_POINT('Ctrl Pts',(12.7765325225082,18.6012488486708,12.));
#210755=CARTESIAN_POINT('Ctrl Pts',(12.7748328937639,18.5985917525949,0.));
#210756=CARTESIAN_POINT('Ctrl Pts',(12.7748328937639,18.5985917525949,12.));
#210757=CARTESIAN_POINT('Ctrl Pts',(12.7733231262107,18.5962551167772,0.));
#210758=CARTESIAN_POINT('Ctrl Pts',(12.7733231262107,18.5962551167772,12.));
#210759=CARTESIAN_POINT('Ctrl Pts',(12.7720142287169,18.5942490615409,0.));
#210760=CARTESIAN_POINT('Ctrl Pts',(12.7720142287169,18.5942490615409,12.));
#210761=CARTESIAN_POINT('Ctrl Pts',(12.7709195951153,18.5925859134582,0.));
#210762=CARTESIAN_POINT('Ctrl Pts',(12.7709195951153,18.5925859134582,12.));
#210763=CARTESIAN_POINT('Ctrl Pts',(12.7700520897174,18.5912775137806,0.));
#210764=CARTESIAN_POINT('Ctrl Pts',(12.7700520897174,18.5912775137806,12.));
#210765=CARTESIAN_POINT('Ctrl Pts',(12.7694215127923,18.590332877722,0.));
#210766=CARTESIAN_POINT('Ctrl Pts',(12.7694215127923,18.590332877722,12.));
#210767=CARTESIAN_POINT('Ctrl Pts',(12.7691103481996,18.589871621842,0.));
#210768=CARTESIAN_POINT('Ctrl Pts',(12.7691103481996,18.589871621842,12.));
#210769=CARTESIAN_POINT('Ctrl Pts',(12.7689864266924,18.5896919669158,0.));
#210770=CARTESIAN_POINT('Ctrl Pts',(12.7689864266924,18.5896919669158,12.));
#210771=CARTESIAN_POINT('Ctrl Pts',(12.7689524524484,18.5896460962961,0.));
#210772=CARTESIAN_POINT('Ctrl Pts',(12.7689524524484,18.5896460962961,12.));
#210773=CARTESIAN_POINT('Ctrl Pts',(12.7689476255363,18.5896416359912,0.));
#210774=CARTESIAN_POINT('Ctrl Pts',(12.7689476255363,18.5896416359912,12.));
#210775=CARTESIAN_POINT('',(13.5685075571671,22.1787195904339,0.));
#210776=CARTESIAN_POINT('Ctrl Pts',(13.5685075571671,22.1787195904339,0.));
#210777=CARTESIAN_POINT('Ctrl Pts',(13.5683460612913,22.1730081264583,0.));
#210778=CARTESIAN_POINT('Ctrl Pts',(13.5680170531724,22.1615922804939,0.));
#210779=CARTESIAN_POINT('Ctrl Pts',(13.5675054918922,22.1444897575076,0.));
#210780=CARTESIAN_POINT('Ctrl Pts',(13.5667873105179,22.1217288871823,0.));
#210781=CARTESIAN_POINT('Ctrl Pts',(13.5658294169106,22.0933486464442,0.));
#210782=CARTESIAN_POINT('Ctrl Pts',(13.5648113688894,22.0650393089492,0.));
#210783=CARTESIAN_POINT('Ctrl Pts',(13.5637332022393,22.0368009736227,0.));
#210784=CARTESIAN_POINT('Ctrl Pts',(13.5625949868313,22.0086337943431,0.));
#210785=CARTESIAN_POINT('Ctrl Pts',(13.5613968357589,21.9805379899192,0.));
#210786=CARTESIAN_POINT('Ctrl Pts',(13.5601389185315,21.9525138592862,0.));
#210787=CARTESIAN_POINT('Ctrl Pts',(13.5588214586672,21.9245617765827,0.));
#210788=CARTESIAN_POINT('Ctrl Pts',(13.5574447178484,21.8966821688876,0.));
#210789=CARTESIAN_POINT('Ctrl Pts',(13.5560089839426,21.8688754989401,0.));
#210790=CARTESIAN_POINT('Ctrl Pts',(13.5545145573048,21.841142245609,0.));
#210791=CARTESIAN_POINT('Ctrl Pts',(13.5529617381569,21.8134828857963,0.));
#210792=CARTESIAN_POINT('Ctrl Pts',(13.5513508127232,21.7858978745848,0.));
#210793=CARTESIAN_POINT('Ctrl Pts',(13.5496820422186,21.7583876294532,0.));
#210794=CARTESIAN_POINT('Ctrl Pts',(13.5479556704457,21.730952541226,0.));
#210795=CARTESIAN_POINT('Ctrl Pts',(13.546171929503,21.7035929822939,0.));
#210796=CARTESIAN_POINT('Ctrl Pts',(13.5443310461516,21.676309315769,0.));
#210797=CARTESIAN_POINT('Ctrl Pts',(13.5424332480698,21.6491019044647,0.));
#210798=CARTESIAN_POINT('Ctrl Pts',(13.5404787697798,21.6219711193951,0.));
#210799=CARTESIAN_POINT('Ctrl Pts',(13.5384678597206,21.5949173499022,0.));
#210800=CARTESIAN_POINT('Ctrl Pts',(13.5364007790292,21.5679410019011,0.));
#210801=CARTESIAN_POINT('Ctrl Pts',(13.5342777983225,21.5410424932511,0.));
#210802=CARTESIAN_POINT('Ctrl Pts',(13.5320991952145,21.5142222501671,0.));
#210803=CARTESIAN_POINT('Ctrl Pts',(13.5298652514357,21.487480703047,0.));
#210804=CARTESIAN_POINT('Ctrl Pts',(13.5275762503553,21.4608182828695,0.));
#210805=CARTESIAN_POINT('Ctrl Pts',(13.5252324737795,21.4342354165254,0.));
#210806=CARTESIAN_POINT('Ctrl Pts',(13.5228342013508,21.4077325259318,0.));
#210807=CARTESIAN_POINT('Ctrl Pts',(13.5203817122496,21.3813100304967,0.));
#210808=CARTESIAN_POINT('Ctrl Pts',(13.5178752862461,21.3549683486219,0.));
#210809=CARTESIAN_POINT('Ctrl Pts',(13.5153152050554,21.328707899634,0.));
#210810=CARTESIAN_POINT('Ctrl Pts',(13.5127017534972,21.3025291054236,0.));
#210811=CARTESIAN_POINT('Ctrl Pts',(13.5100352209207,21.2764323924442,0.));
#210812=CARTESIAN_POINT('Ctrl Pts',(13.5073159019454,21.2504181927429,0.));
#210813=CARTESIAN_POINT('Ctrl Pts',(13.5045440957404,21.224486942933,0.));
#210814=CARTESIAN_POINT('Ctrl Pts',(13.5017201056088,21.1986390835825,0.));
#210815=CARTESIAN_POINT('Ctrl Pts',(13.4988442384491,21.1728750584173,0.));
#210816=CARTESIAN_POINT('Ctrl Pts',(13.4959168042934,21.1471953136209,0.));
#210817=CARTESIAN_POINT('Ctrl Pts',(13.4929381157778,21.1216002970209,0.));
#210818=CARTESIAN_POINT('Ctrl Pts',(13.4899084877718,21.0960904575048,0.));
#210819=CARTESIAN_POINT('Ctrl Pts',(13.4868282377191,21.0706662455202,0.));
#210820=CARTESIAN_POINT('Ctrl Pts',(13.4836976858912,21.0453281134247,0.));
#210821=CARTESIAN_POINT('Ctrl Pts',(13.4805171556822,21.0200765158885,0.));
#210822=CARTESIAN_POINT('Ctrl Pts',(13.4772869738879,20.9949119102592,0.));
#210823=CARTESIAN_POINT('Ctrl Pts',(13.4740074710087,20.9698347569476,0.));
#210824=CARTESIAN_POINT('Ctrl Pts',(13.4706789815166,20.9448455197557,0.));
#210825=CARTESIAN_POINT('Ctrl Pts',(13.4673018437718,20.9199446657584,0.));
#210826=CARTESIAN_POINT('Ctrl Pts',(13.4638763999725,20.8951326652158,0.));
#210827=CARTESIAN_POINT('Ctrl Pts',(13.4604029960983,20.8704099914641,0.));
#210828=CARTESIAN_POINT('Ctrl Pts',(13.4568819818631,20.8457771208082,0.));
#210829=CARTESIAN_POINT('Ctrl Pts',(13.4533137106667,20.821234532398,0.));
#210830=CARTESIAN_POINT('Ctrl Pts',(13.4496985395637,20.7967827081227,0.));
#210831=CARTESIAN_POINT('Ctrl Pts',(13.4460368293688,20.7724221327608,0.));
#210832=CARTESIAN_POINT('Ctrl Pts',(13.4423289447561,20.7481532941013,0.));
#210833=CARTESIAN_POINT('Ctrl Pts',(13.4385752543663,20.7239766830675,0.));
#210834=CARTESIAN_POINT('Ctrl Pts',(13.4347761309154,20.6998927938288,0.));
#210835=CARTESIAN_POINT('Ctrl Pts',(13.4309319513119,20.6759021239103,0.));
#210836=CARTESIAN_POINT('Ctrl Pts',(13.4270430967651,20.6520051742869,0.));
#210837=CARTESIAN_POINT('Ctrl Pts',(13.4231099528179,20.6282024494237,0.));
#210838=CARTESIAN_POINT('Ctrl Pts',(13.4191329093932,20.6044944573153,0.));
#210839=CARTESIAN_POINT('Ctrl Pts',(13.4151123608411,20.5808817095155,0.));
#210840=CARTESIAN_POINT('Ctrl Pts',(13.4110487059912,20.5573647211639,0.));
#210841=CARTESIAN_POINT('Ctrl Pts',(13.4069423482076,20.5339440109956,0.));
#210842=CARTESIAN_POINT('Ctrl Pts',(13.4027936954529,20.5106201013753,0.));
#210843=CARTESIAN_POINT('Ctrl Pts',(13.3986031603716,20.487393518404,0.));
#210844=CARTESIAN_POINT('Ctrl Pts',(13.3943711603739,20.4642647920038,0.));
#210845=CARTESIAN_POINT('Ctrl Pts',(13.3900981177255,20.4412344560008,0.));
#210846=CARTESIAN_POINT('Ctrl Pts',(13.3857844596387,20.4183030482002,0.));
#210847=CARTESIAN_POINT('Ctrl Pts',(13.3814306183719,20.3954711104502,0.));
#210848=CARTESIAN_POINT('Ctrl Pts',(13.3770370313188,20.3727391887184,0.));
#210849=CARTESIAN_POINT('Ctrl Pts',(13.3726041410867,20.3501078331814,0.));
#210850=CARTESIAN_POINT('Ctrl Pts',(13.3681323955826,20.3275775983029,0.));
#210851=CARTESIAN_POINT('Ctrl Pts',(13.3636222481016,20.3051490429048,0.));
#210852=CARTESIAN_POINT('Ctrl Pts',(13.3590741574195,20.2828227302339,0.));
#210853=CARTESIAN_POINT('Ctrl Pts',(13.3544885878889,20.2605992280122,0.));
#210854=CARTESIAN_POINT('Ctrl Pts',(13.3498660095386,20.2384791085359,0.));
#210855=CARTESIAN_POINT('Ctrl Pts',(13.3452068981766,20.216462948786,0.));
#210856=CARTESIAN_POINT('Ctrl Pts',(13.3405117354971,20.1945513305235,0.));
#210857=CARTESIAN_POINT('Ctrl Pts',(13.3357810091903,20.1727448403817,0.));
#210858=CARTESIAN_POINT('Ctrl Pts',(13.3310152130564,20.1510440699474,0.));
#210859=CARTESIAN_POINT('Ctrl Pts',(13.3262148471226,20.1294496158402,0.));
#210860=CARTESIAN_POINT('Ctrl Pts',(13.3213804177587,20.1079620798375,0.));
#210861=CARTESIAN_POINT('Ctrl Pts',(13.3165124377962,20.0865820689883,0.));
#210862=CARTESIAN_POINT('Ctrl Pts',(13.3116114266515,20.0653101957188,0.));
#210863=CARTESIAN_POINT('Ctrl Pts',(13.3066779104515,20.0441470779345,0.));
#210864=CARTESIAN_POINT('Ctrl Pts',(13.3017124221637,20.0230933391038,0.));
#210865=CARTESIAN_POINT('Ctrl Pts',(13.2967155017306,20.0021496083738,0.));
#210866=CARTESIAN_POINT('Ctrl Pts',(13.2916876962094,19.981316520717,0.));
#210867=CARTESIAN_POINT('Ctrl Pts',(13.286629559915,19.9605947170586,0.));
#210868=CARTESIAN_POINT('Ctrl Pts',(13.2815416545663,19.9399848444019,0.));
#210869=CARTESIAN_POINT('Ctrl Pts',(13.2764245494357,19.9194875559422,0.));
#210870=CARTESIAN_POINT('Ctrl Pts',(13.271278821502,19.8991035111745,0.));
#210871=CARTESIAN_POINT('Ctrl Pts',(13.2661050556132,19.8788333760577,0.));
#210872=CARTESIAN_POINT('Ctrl Pts',(13.2609038446529,19.8586778231715,0.));
#210873=CARTESIAN_POINT('Ctrl Pts',(13.2556757897086,19.8386375318634,0.));
#210874=CARTESIAN_POINT('Ctrl Pts',(13.2504215002457,19.8187131883917,0.));
#210875=CARTESIAN_POINT('Ctrl Pts',(13.2451415942805,19.7989054860495,0.));
#210876=CARTESIAN_POINT('Ctrl Pts',(13.2398366985675,19.7792151253289,0.));
#210877=CARTESIAN_POINT('Ctrl Pts',(13.2345074487963,19.7596428141168,0.));
#210878=CARTESIAN_POINT('Ctrl Pts',(13.2291544897899,19.7401892678697,0.));
#210879=CARTESIAN_POINT('Ctrl Pts',(13.2237784757065,19.7208552097868,0.));
#210880=CARTESIAN_POINT('Ctrl Pts',(13.2183800702436,19.7016413709685,0.));
#210881=CARTESIAN_POINT('Ctrl Pts',(13.2129599468485,19.6825484905823,0.));
#210882=CARTESIAN_POINT('Ctrl Pts',(13.2075187889529,19.6635773160936,0.));
#210883=CARTESIAN_POINT('Ctrl Pts',(13.2020572902065,19.6447286034772,0.));
#210884=CARTESIAN_POINT('Ctrl Pts',(13.1965761547151,19.6260031174244,0.));
#210885=CARTESIAN_POINT('Ctrl Pts',(13.1910760972814,19.6074016315414,0.));
#210886=CARTESIAN_POINT('Ctrl Pts',(13.1855578436471,19.5889249285338,0.));
#210887=CARTESIAN_POINT('Ctrl Pts',(13.1800221307673,19.5705738004667,0.));
#210888=CARTESIAN_POINT('Ctrl Pts',(13.1744697070911,19.5523490490244,0.));
#210889=CARTESIAN_POINT('Ctrl Pts',(13.168901332843,19.5342514857562,0.));
#210890=CARTESIAN_POINT('Ctrl Pts',(13.1633177803101,19.5162819323213,0.));
#210891=CARTESIAN_POINT('Ctrl Pts',(13.1577198341245,19.4984412207082,0.));
#210892=CARTESIAN_POINT('Ctrl Pts',(13.1521082915853,19.4807301935268,0.));
#210893=CARTESIAN_POINT('Ctrl Pts',(13.1464839629971,19.4631497043258,0.));
#210894=CARTESIAN_POINT('Ctrl Pts',(13.1408476720061,19.4457006178876,0.));
#210895=CARTESIAN_POINT('Ctrl Pts',(13.1352002559438,19.4283838105262,0.));
#210896=CARTESIAN_POINT('Ctrl Pts',(13.1295425661634,19.4112001703557,0.));
#210897=CARTESIAN_POINT('Ctrl Pts',(13.1238754684177,19.3941505976263,0.));
#210898=CARTESIAN_POINT('Ctrl Pts',(13.118199843271,19.3772360051091,0.));
#210899=CARTESIAN_POINT('Ctrl Pts',(13.1125165865022,19.3604573184515,0.));
#210900=CARTESIAN_POINT('Ctrl Pts',(13.1068266095186,19.3438154765395,0.));
#210901=CARTESIAN_POINT('Ctrl Pts',(13.1011308397591,19.3273114318269,0.));
#210902=CARTESIAN_POINT('Ctrl Pts',(13.0954302211479,19.310946150736,0.));
#210903=CARTESIAN_POINT('Ctrl Pts',(13.0897257145968,19.2947206141247,0.));
#210904=CARTESIAN_POINT('Ctrl Pts',(13.0840182984949,19.2786358177198,0.));
#210905=CARTESIAN_POINT('Ctrl Pts',(13.0783089692118,19.2626927725596,0.));
#210906=CARTESIAN_POINT('Ctrl Pts',(13.0725987415859,19.2468925053989,0.));
#210907=CARTESIAN_POINT('Ctrl Pts',(13.0668886494795,19.2312360592033,0.));
#210908=CARTESIAN_POINT('Ctrl Pts',(13.0611797463915,19.2157244937142,0.));
#210909=CARTESIAN_POINT('Ctrl Pts',(13.0554731060538,19.2003588859772,0.));
#210910=CARTESIAN_POINT('Ctrl Pts',(13.0497698230441,19.1851403308825,0.));
#210911=CARTESIAN_POINT('Ctrl Pts',(13.0440710133772,19.1700699416622,0.));
#210912=CARTESIAN_POINT('Ctrl Pts',(13.0383778152068,19.155148850523,0.));
#210913=CARTESIAN_POINT('Ctrl Pts',(13.0326913895838,19.1403782093386,0.));
#210914=CARTESIAN_POINT('Ctrl Pts',(13.0270129211976,19.1257591903099,0.));
#210915=CARTESIAN_POINT('Ctrl Pts',(13.0213436191328,19.111292986631,0.));
#210916=CARTESIAN_POINT('Ctrl Pts',(13.0156847176096,19.0969808131228,0.));
#210917=CARTESIAN_POINT('Ctrl Pts',(13.0100374768788,19.0828239070484,0.));
#210918=CARTESIAN_POINT('Ctrl Pts',(13.0044031841382,19.0688235289437,0.));
#210919=CARTESIAN_POINT('Ctrl Pts',(12.9987831544502,19.0549809634354,0.));
#210920=CARTESIAN_POINT('Ctrl Pts',(12.9931787316514,19.0412975200398,0.));
#210921=CARTESIAN_POINT('Ctrl Pts',(12.9875912893003,19.0277745339909,0.));
#210922=CARTESIAN_POINT('Ctrl Pts',(12.9820222318716,19.014413367335,0.));
#210923=CARTESIAN_POINT('Ctrl Pts',(12.9764729959206,19.0012154099792,0.));
#210924=CARTESIAN_POINT('Ctrl Pts',(12.9709450512747,18.9881820807585,0.));
#210925=CARTESIAN_POINT('Ctrl Pts',(12.9654399021868,18.9753148284473,0.));
#210926=CARTESIAN_POINT('Ctrl Pts',(12.9599590886317,18.9626151329226,0.));
#210927=CARTESIAN_POINT('Ctrl Pts',(12.9545041877377,18.9500845064714,0.));
#210928=CARTESIAN_POINT('Ctrl Pts',(12.9490768151821,18.9377244950435,0.));
#210929=CARTESIAN_POINT('Ctrl Pts',(12.9436786266106,18.9255366795196,0.));
#210930=CARTESIAN_POINT('Ctrl Pts',(12.9383113190375,18.9135226769466,0.));
#210931=CARTESIAN_POINT('Ctrl Pts',(12.9329766328184,18.9016841423402,0.));
#210932=CARTESIAN_POINT('Ctrl Pts',(12.9276763536372,18.8900227704888,0.));
#210933=CARTESIAN_POINT('Ctrl Pts',(12.9224123144982,18.8785402977528,0.));
#210934=CARTESIAN_POINT('Ctrl Pts',(12.9171863977047,18.8672385038328,0.));
#210935=CARTESIAN_POINT('Ctrl Pts',(12.9120005369066,18.8561192136201,0.));
#210936=CARTESIAN_POINT('Ctrl Pts',(12.9068567191856,18.8451842990986,0.));
#210937=CARTESIAN_POINT('Ctrl Pts',(12.9017569871738,18.834435681259,0.));
#210938=CARTESIAN_POINT('Ctrl Pts',(12.8967034410752,18.8238753319124,0.));
#210939=CARTESIAN_POINT('Ctrl Pts',(12.8916982409931,18.8135052757815,0.));
#210940=CARTESIAN_POINT('Ctrl Pts',(12.8867436109543,18.8033275941939,0.));
#210941=CARTESIAN_POINT('Ctrl Pts',(12.8818418427474,18.7933444285867,0.));
#210942=CARTESIAN_POINT('Ctrl Pts',(12.8769952998097,18.7835579840481,0.));
#210943=CARTESIAN_POINT('Ctrl Pts',(12.8722064211814,18.7739705329029,0.));
#210944=CARTESIAN_POINT('Ctrl Pts',(12.8674777239656,18.7645844169568,0.));
#210945=CARTESIAN_POINT('Ctrl Pts',(12.8628118054172,18.7554020493888,0.));
#210946=CARTESIAN_POINT('Ctrl Pts',(12.8582113455644,18.7464259171248,0.));
#210947=CARTESIAN_POINT('Ctrl Pts',(12.8536791086315,18.7376585820851,0.));
#210948=CARTESIAN_POINT('Ctrl Pts',(12.849217951159,18.7291026886552,0.));
#210949=CARTESIAN_POINT('Ctrl Pts',(12.8448308329494,18.7207609737701,0.));
#210950=CARTESIAN_POINT('Ctrl Pts',(12.8405208263432,18.7126362754446,0.));
#210951=CARTESIAN_POINT('Ctrl Pts',(12.8362911280362,18.7047315436296,0.));
#210952=CARTESIAN_POINT('Ctrl Pts',(12.832145059979,18.6970498410173,0.));
#210953=CARTESIAN_POINT('Ctrl Pts',(12.8280860635231,18.6895943376172,0.));
#210954=CARTESIAN_POINT('Ctrl Pts',(12.8241176980016,18.6823683094139,0.));
#210955=CARTESIAN_POINT('Ctrl Pts',(12.8202436318473,18.6753751301091,0.));
#210956=CARTESIAN_POINT('Ctrl Pts',(12.8164676687361,18.6686182952798,0.));
#210957=CARTESIAN_POINT('Ctrl Pts',(12.8127937909632,18.6621014624746,0.));
#210958=CARTESIAN_POINT('Ctrl Pts',(12.8092261933858,18.6558284825772,0.));
#210959=CARTESIAN_POINT('Ctrl Pts',(12.805769331162,18.6498034438986,0.));
#210960=CARTESIAN_POINT('Ctrl Pts',(12.8024278770153,18.6440306327457,0.));
#210961=CARTESIAN_POINT('Ctrl Pts',(12.7992066625264,18.63851447924,0.));
#210962=CARTESIAN_POINT('Ctrl Pts',(12.7961106222251,18.6332595057005,0.));
#210963=CARTESIAN_POINT('Ctrl Pts',(12.7931447451556,18.6282702819371,0.));
#210964=CARTESIAN_POINT('Ctrl Pts',(12.7903142925234,18.6235516265575,0.));
#210965=CARTESIAN_POINT('Ctrl Pts',(12.7876249657834,18.6191087624752,0.));
#210966=CARTESIAN_POINT('Ctrl Pts',(12.78508316579,18.6149475565189,0.));
#210967=CARTESIAN_POINT('Ctrl Pts',(12.7826959526924,18.611074482622,0.));
#210968=CARTESIAN_POINT('Ctrl Pts',(12.7804705387658,18.6074961535723,0.));
#210969=CARTESIAN_POINT('Ctrl Pts',(12.7784139605067,18.6042190183703,0.));
#210970=CARTESIAN_POINT('Ctrl Pts',(12.7765325225082,18.6012488486708,0.));
#210971=CARTESIAN_POINT('Ctrl Pts',(12.7748328937639,18.5985917525949,0.));
#210972=CARTESIAN_POINT('Ctrl Pts',(12.7733231262107,18.5962551167772,0.));
#210973=CARTESIAN_POINT('Ctrl Pts',(12.7720142287169,18.5942490615409,0.));
#210974=CARTESIAN_POINT('Ctrl Pts',(12.7709195951153,18.5925859134582,0.));
#210975=CARTESIAN_POINT('Ctrl Pts',(12.7700520897174,18.5912775137806,0.));
#210976=CARTESIAN_POINT('Ctrl Pts',(12.7694215127923,18.590332877722,0.));
#210977=CARTESIAN_POINT('Ctrl Pts',(12.7691103481996,18.589871621842,0.));
#210978=CARTESIAN_POINT('Ctrl Pts',(12.7689864266924,18.5896919669158,0.));
#210979=CARTESIAN_POINT('Ctrl Pts',(12.7689524524484,18.5896460962961,0.));
#210980=CARTESIAN_POINT('Ctrl Pts',(12.7689476255363,18.5896416359912,0.));
#210981=CARTESIAN_POINT('',(13.5685075571671,22.1787195904339,0.));
#210982=CARTESIAN_POINT('Ctrl Pts',(14.6513681262571,17.1452095830633,0.));
#210983=CARTESIAN_POINT('Ctrl Pts',(14.6513681262571,17.1452095830633,12.));
#210984=CARTESIAN_POINT('Ctrl Pts',(14.6513711852843,17.1452153999142,0.));
#210985=CARTESIAN_POINT('Ctrl Pts',(14.6513711852843,17.1452153999142,12.));
#210986=CARTESIAN_POINT('Ctrl Pts',(14.6514066997196,17.1452600887037,0.));
#210987=CARTESIAN_POINT('Ctrl Pts',(14.6514066997196,17.1452600887037,12.));
#210988=CARTESIAN_POINT('Ctrl Pts',(14.6515481598068,17.1454262858043,0.));
#210989=CARTESIAN_POINT('Ctrl Pts',(14.6515481598068,17.1454262858043,12.));
#210990=CARTESIAN_POINT('Ctrl Pts',(14.6519131634508,17.1458462295271,0.));
#210991=CARTESIAN_POINT('Ctrl Pts',(14.6519131634508,17.1458462295271,12.));
#210992=CARTESIAN_POINT('Ctrl Pts',(14.6526624064978,17.1466998098673,0.));
#210993=CARTESIAN_POINT('Ctrl Pts',(14.6526624064978,17.1466998098673,12.));
#210994=CARTESIAN_POINT('Ctrl Pts',(14.6537016966184,17.147876394491,0.));
#210995=CARTESIAN_POINT('Ctrl Pts',(14.6537016966184,17.147876394491,12.));
#210996=CARTESIAN_POINT('Ctrl Pts',(14.655024862281,17.1493641837558,0.));
#210997=CARTESIAN_POINT('Ctrl Pts',(14.655024862281,17.1493641837558,12.));
#210998=CARTESIAN_POINT('Ctrl Pts',(14.6566237952435,17.1511476869496,0.));
#210999=CARTESIAN_POINT('Ctrl Pts',(14.6566237952435,17.1511476869496,12.));
#211000=CARTESIAN_POINT('Ctrl Pts',(14.6584900555302,17.1532107762718,0.));
#211001=CARTESIAN_POINT('Ctrl Pts',(14.6584900555302,17.1532107762718,12.));
#211002=CARTESIAN_POINT('Ctrl Pts',(14.6606167169642,17.1555401986401,0.));
#211003=CARTESIAN_POINT('Ctrl Pts',(14.6606167169642,17.1555401986401,12.));
#211004=CARTESIAN_POINT('Ctrl Pts',(14.6629987285992,17.1581262646789,0.));
#211005=CARTESIAN_POINT('Ctrl Pts',(14.6629987285992,17.1581262646789,12.));
#211006=CARTESIAN_POINT('Ctrl Pts',(14.6656319165057,17.1609609517369,0.));
#211007=CARTESIAN_POINT('Ctrl Pts',(14.6656319165057,17.1609609517369,12.));
#211008=CARTESIAN_POINT('Ctrl Pts',(14.6685123374423,17.1640366762305,0.));
#211009=CARTESIAN_POINT('Ctrl Pts',(14.6685123374423,17.1640366762305,12.));
#211010=CARTESIAN_POINT('Ctrl Pts',(14.671635583332,17.167344972302,0.));
#211011=CARTESIAN_POINT('Ctrl Pts',(14.671635583332,17.167344972302,12.));
#211012=CARTESIAN_POINT('Ctrl Pts',(14.6749971333867,17.1708771619129,0.));
#211013=CARTESIAN_POINT('Ctrl Pts',(14.6749971333867,17.1708771619129,12.));
#211014=CARTESIAN_POINT('Ctrl Pts',(14.6785925615677,17.1746247499057,0.));
#211015=CARTESIAN_POINT('Ctrl Pts',(14.6785925615677,17.1746247499057,12.));
#211016=CARTESIAN_POINT('Ctrl Pts',(14.6824178576167,17.1785800350826,0.));
#211017=CARTESIAN_POINT('Ctrl Pts',(14.6824178576167,17.1785800350826,12.));
#211018=CARTESIAN_POINT('Ctrl Pts',(14.686469452232,17.182736158472,0.));
#211019=CARTESIAN_POINT('Ctrl Pts',(14.686469452232,17.182736158472,12.));
#211020=CARTESIAN_POINT('Ctrl Pts',(14.6907440526958,17.1870867909918,0.));
#211021=CARTESIAN_POINT('Ctrl Pts',(14.6907440526958,17.1870867909918,12.));
#211022=CARTESIAN_POINT('Ctrl Pts',(14.6952385361705,17.1916259308415,0.));
#211023=CARTESIAN_POINT('Ctrl Pts',(14.6952385361705,17.1916259308415,12.));
#211024=CARTESIAN_POINT('Ctrl Pts',(14.699949811582,17.1963476411694,0.));
#211025=CARTESIAN_POINT('Ctrl Pts',(14.699949811582,17.1963476411694,12.));
#211026=CARTESIAN_POINT('Ctrl Pts',(14.7048748502663,17.2012461084268,0.));
#211027=CARTESIAN_POINT('Ctrl Pts',(14.7048748502663,17.2012461084268,12.));
#211028=CARTESIAN_POINT('Ctrl Pts',(14.7100107213586,17.2063157097315,0.));
#211029=CARTESIAN_POINT('Ctrl Pts',(14.7100107213586,17.2063157097315,12.));
#211030=CARTESIAN_POINT('Ctrl Pts',(14.7153546289339,17.2115510835989,0.));
#211031=CARTESIAN_POINT('Ctrl Pts',(14.7153546289339,17.2115510835989,12.));
#211032=CARTESIAN_POINT('Ctrl Pts',(14.7209039390327,17.2169471814256,0.));
#211033=CARTESIAN_POINT('Ctrl Pts',(14.7209039390327,17.2169471814256,12.));
#211034=CARTESIAN_POINT('Ctrl Pts',(14.7266561494282,17.2224992099667,0.));
#211035=CARTESIAN_POINT('Ctrl Pts',(14.7266561494282,17.2224992099667,12.));
#211036=CARTESIAN_POINT('Ctrl Pts',(14.7326088681163,17.2282025904314,0.));
#211037=CARTESIAN_POINT('Ctrl Pts',(14.7326088681163,17.2282025904314,12.));
#211038=CARTESIAN_POINT('Ctrl Pts',(14.7387597858116,17.2340529062076,0.));
#211039=CARTESIAN_POINT('Ctrl Pts',(14.7387597858116,17.2340529062076,12.));
#211040=CARTESIAN_POINT('Ctrl Pts',(14.7451066593792,17.2400458713565,0.));
#211041=CARTESIAN_POINT('Ctrl Pts',(14.7451066593792,17.2400458713565,12.));
#211042=CARTESIAN_POINT('Ctrl Pts',(14.7516473175124,17.2461773413288,0.));
#211043=CARTESIAN_POINT('Ctrl Pts',(14.7516473175124,17.2461773413288,12.));
#211044=CARTESIAN_POINT('Ctrl Pts',(14.7583796616617,17.2524433146837,0.));
#211045=CARTESIAN_POINT('Ctrl Pts',(14.7583796616617,17.2524433146837,12.));
#211046=CARTESIAN_POINT('Ctrl Pts',(14.7653016697591,17.2588399401465,0.));
#211047=CARTESIAN_POINT('Ctrl Pts',(14.7653016697591,17.2588399401465,12.));
#211048=CARTESIAN_POINT('Ctrl Pts',(14.7724113956731,17.2653635155319,0.));
#211049=CARTESIAN_POINT('Ctrl Pts',(14.7724113956731,17.2653635155319,12.));
#211050=CARTESIAN_POINT('Ctrl Pts',(14.7797069617804,17.2720104735194,0.));
#211051=CARTESIAN_POINT('Ctrl Pts',(14.7797069617804,17.2720104735194,12.));
#211052=CARTESIAN_POINT('Ctrl Pts',(14.787186553128,17.2787773704849,0.));
#211053=CARTESIAN_POINT('Ctrl Pts',(14.787186553128,17.2787773704849,12.));
#211054=CARTESIAN_POINT('Ctrl Pts',(14.7948484105249,17.2856608733196,0.));
#211055=CARTESIAN_POINT('Ctrl Pts',(14.7948484105249,17.2856608733196,12.));
#211056=CARTESIAN_POINT('Ctrl Pts',(14.8026908254276,17.2926577496513,0.));
#211057=CARTESIAN_POINT('Ctrl Pts',(14.8026908254276,17.2926577496513,12.));
#211058=CARTESIAN_POINT('Ctrl Pts',(14.8107121391035,17.299764866148,0.));
#211059=CARTESIAN_POINT('Ctrl Pts',(14.8107121391035,17.299764866148,12.));
#211060=CARTESIAN_POINT('Ctrl Pts',(14.8189107410162,17.3069791853706,0.));
#211061=CARTESIAN_POINT('Ctrl Pts',(14.8189107410162,17.3069791853706,12.));
#211062=CARTESIAN_POINT('Ctrl Pts',(14.8272850675379,17.3142977632659,0.));
#211063=CARTESIAN_POINT('Ctrl Pts',(14.8272850675379,17.3142977632659,12.));
#211064=CARTESIAN_POINT('Ctrl Pts',(14.8358336004197,17.3217177462101,0.));
#211065=CARTESIAN_POINT('Ctrl Pts',(14.8358336004197,17.3217177462101,12.));
#211066=CARTESIAN_POINT('Ctrl Pts',(14.8445548643508,17.3292363662605,0.));
#211067=CARTESIAN_POINT('Ctrl Pts',(14.8445548643508,17.3292363662605,12.));
#211068=CARTESIAN_POINT('Ctrl Pts',(14.8534474245433,17.336850936485,0.));
#211069=CARTESIAN_POINT('Ctrl Pts',(14.8534474245433,17.336850936485,12.));
#211070=CARTESIAN_POINT('Ctrl Pts',(14.8625098843417,17.3445588463475,0.));
#211071=CARTESIAN_POINT('Ctrl Pts',(14.8625098843417,17.3445588463475,12.));
#211072=CARTESIAN_POINT('Ctrl Pts',(14.8717408826955,17.3523575568645,0.));
#211073=CARTESIAN_POINT('Ctrl Pts',(14.8717408826955,17.3523575568645,12.));
#211074=CARTESIAN_POINT('Ctrl Pts',(14.8811390927423,17.3602445978161,0.));
#211075=CARTESIAN_POINT('Ctrl Pts',(14.8811390927423,17.3602445978161,12.));
#211076=CARTESIAN_POINT('Ctrl Pts',(14.8907032205788,17.3682175653235,0.));
#211077=CARTESIAN_POINT('Ctrl Pts',(14.8907032205788,17.3682175653235,12.));
#211078=CARTESIAN_POINT('Ctrl Pts',(14.900432003961,17.3762741193076,0.));
#211079=CARTESIAN_POINT('Ctrl Pts',(14.900432003961,17.3762741193076,12.));
#211080=CARTESIAN_POINT('Ctrl Pts',(14.9103242110057,17.3844119809824,0.));
#211081=CARTESIAN_POINT('Ctrl Pts',(14.9103242110057,17.3844119809824,12.));
#211082=CARTESIAN_POINT('Ctrl Pts',(14.9203786389342,17.3926289303986,0.));
#211083=CARTESIAN_POINT('Ctrl Pts',(14.9203786389342,17.3926289303986,12.));
#211084=CARTESIAN_POINT('Ctrl Pts',(14.9305941128757,17.4009228040749,0.));
#211085=CARTESIAN_POINT('Ctrl Pts',(14.9305941128757,17.4009228040749,12.));
#211086=CARTESIAN_POINT('Ctrl Pts',(14.940969484645,17.4092914926071,0.));
#211087=CARTESIAN_POINT('Ctrl Pts',(14.940969484645,17.4092914926071,12.));
#211088=CARTESIAN_POINT('Ctrl Pts',(14.9515036315143,17.4177329382828,0.));
#211089=CARTESIAN_POINT('Ctrl Pts',(14.9515036315143,17.4177329382828,12.));
#211090=CARTESIAN_POINT('Ctrl Pts',(14.9621954549827,17.426245132709,0.));
#211091=CARTESIAN_POINT('Ctrl Pts',(14.9621954549827,17.426245132709,12.));
#211092=CARTESIAN_POINT('Ctrl Pts',(14.9730438799452,17.4348261151396,0.));
#211093=CARTESIAN_POINT('Ctrl Pts',(14.9730438799452,17.4348261151396,12.));
#211094=CARTESIAN_POINT('Ctrl Pts',(14.9840478538358,17.4434739707773,0.));
#211095=CARTESIAN_POINT('Ctrl Pts',(14.9840478538358,17.4434739707773,12.));
#211096=CARTESIAN_POINT('Ctrl Pts',(14.9952063457778,17.4521868291004,0.));
#211097=CARTESIAN_POINT('Ctrl Pts',(14.9952063457778,17.4521868291004,12.));
#211098=CARTESIAN_POINT('Ctrl Pts',(15.0065183456921,17.4609628621418,0.));
#211099=CARTESIAN_POINT('Ctrl Pts',(15.0065183456921,17.4609628621418,12.));
#211100=CARTESIAN_POINT('Ctrl Pts',(15.0179828635086,17.4698002829357,0.));
#211101=CARTESIAN_POINT('Ctrl Pts',(15.0179828635086,17.4698002829357,12.));
#211102=CARTESIAN_POINT('Ctrl Pts',(15.029598928488,17.4786973441417,0.));
#211103=CARTESIAN_POINT('Ctrl Pts',(15.029598928488,17.4786973441417,12.));
#211104=CARTESIAN_POINT('Ctrl Pts',(15.0413655884993,17.4876523366178,0.));
#211105=CARTESIAN_POINT('Ctrl Pts',(15.0413655884993,17.4876523366178,12.));
#211106=CARTESIAN_POINT('Ctrl Pts',(15.0532819093085,17.4966635880245,0.));
#211107=CARTESIAN_POINT('Ctrl Pts',(15.0532819093085,17.4966635880245,12.));
#211108=CARTESIAN_POINT('Ctrl Pts',(15.0653469738306,17.5057294613874,0.));
#211109=CARTESIAN_POINT('Ctrl Pts',(15.0653469738306,17.5057294613874,12.));
#211110=CARTESIAN_POINT('Ctrl Pts',(15.0775598815748,17.5148483539684,0.));
#211111=CARTESIAN_POINT('Ctrl Pts',(15.0775598815748,17.5148483539684,12.));
#211112=CARTESIAN_POINT('Ctrl Pts',(15.0899197481082,17.5240186961788,0.));
#211113=CARTESIAN_POINT('Ctrl Pts',(15.0899197481082,17.5240186961788,12.));
#211114=CARTESIAN_POINT('Ctrl Pts',(15.1024257045033,17.5332389504829,0.));
#211115=CARTESIAN_POINT('Ctrl Pts',(15.1024257045033,17.5332389504829,12.));
#211116=CARTESIAN_POINT('Ctrl Pts',(15.1150768967729,17.5425076102966,0.));
#211117=CARTESIAN_POINT('Ctrl Pts',(15.1150768967729,17.5425076102966,12.));
#211118=CARTESIAN_POINT('Ctrl Pts',(15.127872485314,17.5518231989122,0.));
#211119=CARTESIAN_POINT('Ctrl Pts',(15.127872485314,17.5518231989122,12.));
#211120=CARTESIAN_POINT('Ctrl Pts',(15.1408116444877,17.5611842686196,0.));
#211121=CARTESIAN_POINT('Ctrl Pts',(15.1408116444877,17.5611842686196,12.));
#211122=CARTESIAN_POINT('Ctrl Pts',(15.1538935621714,17.570589399803,0.));
#211123=CARTESIAN_POINT('Ctrl Pts',(15.1538935621714,17.570589399803,12.));
#211124=CARTESIAN_POINT('Ctrl Pts',(15.1671174393136,17.5800372000539,0.));
#211125=CARTESIAN_POINT('Ctrl Pts',(15.1671174393136,17.5800372000539,12.));
#211126=CARTESIAN_POINT('Ctrl Pts',(15.1804824894605,17.5895263032592,0.));
#211127=CARTESIAN_POINT('Ctrl Pts',(15.1804824894605,17.5895263032592,12.));
#211128=CARTESIAN_POINT('Ctrl Pts',(15.1939879383268,17.5990553687595,0.));
#211129=CARTESIAN_POINT('Ctrl Pts',(15.1939879383268,17.5990553687595,12.));
#211130=CARTESIAN_POINT('Ctrl Pts',(15.2076330234686,17.6086230806497,0.));
#211131=CARTESIAN_POINT('Ctrl Pts',(15.2076330234686,17.6086230806497,12.));
#211132=CARTESIAN_POINT('Ctrl Pts',(15.22141699392,17.6182281470467,0.));
#211133=CARTESIAN_POINT('Ctrl Pts',(15.22141699392,17.6182281470467,12.));
#211134=CARTESIAN_POINT('Ctrl Pts',(15.2353391098367,17.6278692993765,0.));
#211135=CARTESIAN_POINT('Ctrl Pts',(15.2353391098367,17.6278692993765,12.));
#211136=CARTESIAN_POINT('Ctrl Pts',(15.2493986421091,17.637545291637,0.));
#211137=CARTESIAN_POINT('Ctrl Pts',(15.2493986421091,17.637545291637,12.));
#211138=CARTESIAN_POINT('Ctrl Pts',(15.263594872029,17.6472548997329,0.));
#211139=CARTESIAN_POINT('Ctrl Pts',(15.263594872029,17.6472548997329,12.));
#211140=CARTESIAN_POINT('Ctrl Pts',(15.2779270910238,17.6569969209,0.));
#211141=CARTESIAN_POINT('Ctrl Pts',(15.2779270910238,17.6569969209,12.));
#211142=CARTESIAN_POINT('Ctrl Pts',(15.2923946003598,17.6667701731041,0.));
#211143=CARTESIAN_POINT('Ctrl Pts',(15.2923946003598,17.6667701731041,12.));
#211144=CARTESIAN_POINT('Ctrl Pts',(15.3069967108501,17.6765734944559,0.));
#211145=CARTESIAN_POINT('Ctrl Pts',(15.3069967108501,17.6765734944559,12.));
#211146=CARTESIAN_POINT('Ctrl Pts',(15.3217327425341,17.6864057426052,0.));
#211147=CARTESIAN_POINT('Ctrl Pts',(15.3217327425341,17.6864057426052,12.));
#211148=CARTESIAN_POINT('Ctrl Pts',(15.3366020244069,17.6962657941984,0.));
#211149=CARTESIAN_POINT('Ctrl Pts',(15.3366020244069,17.6962657941984,12.));
#211150=CARTESIAN_POINT('Ctrl Pts',(15.3516038942064,17.7061525444044,0.));
#211151=CARTESIAN_POINT('Ctrl Pts',(15.3516038942064,17.7061525444044,12.));
#211152=CARTESIAN_POINT('Ctrl Pts',(15.3667376981702,17.7160649064208,0.));
#211153=CARTESIAN_POINT('Ctrl Pts',(15.3667376981702,17.7160649064208,12.));
#211154=CARTESIAN_POINT('Ctrl Pts',(15.3820027907965,17.7260018109923,0.));
#211155=CARTESIAN_POINT('Ctrl Pts',(15.3820027907965,17.7260018109923,12.));
#211156=CARTESIAN_POINT('Ctrl Pts',(15.3973985345796,17.7359622059143,0.));
#211157=CARTESIAN_POINT('Ctrl Pts',(15.3973985345796,17.7359622059143,12.));
#211158=CARTESIAN_POINT('Ctrl Pts',(15.4129242997828,17.7459450555803,0.));
#211159=CARTESIAN_POINT('Ctrl Pts',(15.4129242997828,17.7459450555803,12.));
#211160=CARTESIAN_POINT('Ctrl Pts',(15.4285794642658,17.7559493405871,0.));
#211161=CARTESIAN_POINT('Ctrl Pts',(15.4285794642658,17.7559493405871,12.));
#211162=CARTESIAN_POINT('Ctrl Pts',(15.4443634132865,17.765974057326,0.));
#211163=CARTESIAN_POINT('Ctrl Pts',(15.4443634132865,17.765974057326,12.));
#211164=CARTESIAN_POINT('Ctrl Pts',(15.4602755393019,17.7760182175817,0.));
#211165=CARTESIAN_POINT('Ctrl Pts',(15.4602755393019,17.7760182175817,12.));
#211166=CARTESIAN_POINT('Ctrl Pts',(15.4763152417506,17.7860808481229,0.));
#211167=CARTESIAN_POINT('Ctrl Pts',(15.4763152417506,17.7860808481229,12.));
#211168=CARTESIAN_POINT('Ctrl Pts',(15.4924819268529,17.7961609903161,0.));
#211169=CARTESIAN_POINT('Ctrl Pts',(15.4924819268529,17.7961609903161,12.));
#211170=CARTESIAN_POINT('Ctrl Pts',(15.5087750074728,17.8062576997964,0.));
#211171=CARTESIAN_POINT('Ctrl Pts',(15.5087750074728,17.8062576997964,12.));
#211172=CARTESIAN_POINT('Ctrl Pts',(15.5251939029558,17.8163700461263,0.));
#211173=CARTESIAN_POINT('Ctrl Pts',(15.5251939029558,17.8163700461263,12.));
#211174=CARTESIAN_POINT('Ctrl Pts',(15.5417380389639,17.8264971124606,0.));
#211175=CARTESIAN_POINT('Ctrl Pts',(15.5417380389639,17.8264971124606,12.));
#211176=CARTESIAN_POINT('Ctrl Pts',(15.5584068472976,17.8366379952078,0.));
#211177=CARTESIAN_POINT('Ctrl Pts',(15.5584068472976,17.8366379952078,12.));
#211178=CARTESIAN_POINT('Ctrl Pts',(15.5751997657153,17.8467918036977,0.));
#211179=CARTESIAN_POINT('Ctrl Pts',(15.5751997657153,17.8467918036977,12.));
#211180=CARTESIAN_POINT('Ctrl Pts',(15.5921162378183,17.8569576598996,0.));
#211181=CARTESIAN_POINT('Ctrl Pts',(15.5921162378183,17.8569576598996,12.));
#211182=CARTESIAN_POINT('Ctrl Pts',(15.6091557129205,17.8671346981388,0.));
#211183=CARTESIAN_POINT('Ctrl Pts',(15.6091557129205,17.8671346981388,12.));
#211184=CARTESIAN_POINT('Ctrl Pts',(15.6263176459107,17.8773220648125,0.));
#211185=CARTESIAN_POINT('Ctrl Pts',(15.6263176459107,17.8773220648125,12.));
#211186=CARTESIAN_POINT('Ctrl Pts',(15.6436014971088,17.8875189181095,0.));
#211187=CARTESIAN_POINT('Ctrl Pts',(15.6436014971088,17.8875189181095,12.));
#211188=CARTESIAN_POINT('Ctrl Pts',(15.6610067321036,17.8977244277247,0.));
#211189=CARTESIAN_POINT('Ctrl Pts',(15.6610067321036,17.8977244277247,12.));
#211190=CARTESIAN_POINT('Ctrl Pts',(15.6785328216467,17.9079377746118,0.));
#211191=CARTESIAN_POINT('Ctrl Pts',(15.6785328216467,17.9079377746118,12.));
#211192=CARTESIAN_POINT('Ctrl Pts',(15.6961792415526,17.918158150746,0.));
#211193=CARTESIAN_POINT('Ctrl Pts',(15.6961792415526,17.918158150746,12.));
#211194=CARTESIAN_POINT('Ctrl Pts',(15.713945472584,17.9283847588837,0.));
#211195=CARTESIAN_POINT('Ctrl Pts',(15.713945472584,17.9283847588837,12.));
#211196=CARTESIAN_POINT('Ctrl Pts',(15.7318310003334,17.9386168123261,0.));
#211197=CARTESIAN_POINT('Ctrl Pts',(15.7318310003334,17.9386168123261,12.));
#211198=CARTESIAN_POINT('Ctrl Pts',(15.7498353150856,17.9488535346776,0.));
#211199=CARTESIAN_POINT('Ctrl Pts',(15.7498353150856,17.9488535346776,12.));
#211200=CARTESIAN_POINT('Ctrl Pts',(15.7679579117072,17.9590941596236,0.));
#211201=CARTESIAN_POINT('Ctrl Pts',(15.7679579117072,17.9590941596236,12.));
#211202=CARTESIAN_POINT('Ctrl Pts',(15.786198289572,17.9693379307297,0.));
#211203=CARTESIAN_POINT('Ctrl Pts',(15.786198289572,17.9693379307297,12.));
#211204=CARTESIAN_POINT('Ctrl Pts',(15.8045559524674,17.9795841012383,0.));
#211205=CARTESIAN_POINT('Ctrl Pts',(15.8045559524674,17.9795841012383,12.));
#211206=CARTESIAN_POINT('Ctrl Pts',(15.8230304084963,17.9898319338664,0.));
#211207=CARTESIAN_POINT('Ctrl Pts',(15.8230304084963,17.9898319338664,12.));
#211208=CARTESIAN_POINT('Ctrl Pts',(15.8416211699681,18.0000807006055,0.));
#211209=CARTESIAN_POINT('Ctrl Pts',(15.8416211699681,18.0000807006055,12.));
#211210=CARTESIAN_POINT('Ctrl Pts',(15.8603277532834,18.010329682521,0.));
#211211=CARTESIAN_POINT('Ctrl Pts',(15.8603277532834,18.010329682521,12.));
#211212=CARTESIAN_POINT('Ctrl Pts',(15.8791496788685,18.0205781695773,0.));
#211213=CARTESIAN_POINT('Ctrl Pts',(15.8791496788685,18.0205781695773,12.));
#211214=CARTESIAN_POINT('Ctrl Pts',(15.8980864711043,18.0308254604638,0.));
#211215=CARTESIAN_POINT('Ctrl Pts',(15.8980864711043,18.0308254604638,12.));
#211216=CARTESIAN_POINT('Ctrl Pts',(15.9171376582436,18.0410708624208,0.));
#211217=CARTESIAN_POINT('Ctrl Pts',(15.9171376582436,18.0410708624208,12.));
#211218=CARTESIAN_POINT('Ctrl Pts',(15.9363027723244,18.0513136910691,0.));
#211219=CARTESIAN_POINT('Ctrl Pts',(15.9363027723244,18.0513136910691,12.));
#211220=CARTESIAN_POINT('Ctrl Pts',(15.9555813490645,18.061553270236,0.));
#211221=CARTESIAN_POINT('Ctrl Pts',(15.9555813490645,18.061553270236,12.));
#211222=CARTESIAN_POINT('Ctrl Pts',(15.9749729277848,18.071788931796,0.));
#211223=CARTESIAN_POINT('Ctrl Pts',(15.9749729277848,18.071788931796,12.));
#211224=CARTESIAN_POINT('Ctrl Pts',(15.9944770513616,18.0820200155239,0.));
#211225=CARTESIAN_POINT('Ctrl Pts',(15.9944770513616,18.0820200155239,12.));
#211226=CARTESIAN_POINT('Ctrl Pts',(16.0140932661612,18.0922458689464,0.));
#211227=CARTESIAN_POINT('Ctrl Pts',(16.0140932661612,18.0922458689464,12.));
#211228=CARTESIAN_POINT('Ctrl Pts',(16.0338211219693,18.1024658471966,0.));
#211229=CARTESIAN_POINT('Ctrl Pts',(16.0338211219693,18.1024658471966,12.));
#211230=CARTESIAN_POINT('Ctrl Pts',(16.0536601719124,18.1126793128688,0.));
#211231=CARTESIAN_POINT('Ctrl Pts',(16.0536601719124,18.1126793128688,12.));
#211232=CARTESIAN_POINT('Ctrl Pts',(16.0736099723664,18.1228856358746,0.));
#211233=CARTESIAN_POINT('Ctrl Pts',(16.0736099723664,18.1228856358746,12.));
#211234=CARTESIAN_POINT('Ctrl Pts',(16.0936700829108,18.1330841933099,0.));
#211235=CARTESIAN_POINT('Ctrl Pts',(16.0936700829108,18.1330841933099,12.));
#211236=CARTESIAN_POINT('Ctrl Pts',(16.113840066279,18.1432743693231,0.));
#211237=CARTESIAN_POINT('Ctrl Pts',(16.113840066279,18.1432743693231,12.));
#211238=CARTESIAN_POINT('Ctrl Pts',(16.1341194882987,18.1534555549851,0.));
#211239=CARTESIAN_POINT('Ctrl Pts',(16.1341194882987,18.1534555549851,12.));
#211240=CARTESIAN_POINT('Ctrl Pts',(16.1545079178261,18.1636271481616,0.));
#211241=CARTESIAN_POINT('Ctrl Pts',(16.1545079178261,18.1636271481616,12.));
#211242=CARTESIAN_POINT('Ctrl Pts',(16.1750049266673,18.1737885533852,0.));
#211243=CARTESIAN_POINT('Ctrl Pts',(16.1750049266673,18.1737885533852,12.));
#211244=CARTESIAN_POINT('Ctrl Pts',(16.1956100895076,18.1839391817335,0.));
#211245=CARTESIAN_POINT('Ctrl Pts',(16.1956100895076,18.1839391817335,12.));
#211246=CARTESIAN_POINT('Ctrl Pts',(16.2163229838878,18.1940784507232,0.));
#211247=CARTESIAN_POINT('Ctrl Pts',(16.2163229838878,18.1940784507232,12.));
#211248=CARTESIAN_POINT('Ctrl Pts',(16.237143190164,18.2042057842037,0.));
#211249=CARTESIAN_POINT('Ctrl Pts',(16.237143190164,18.2042057842037,12.));
#211250=CARTESIAN_POINT('Ctrl Pts',(16.2580702914615,18.214320612253,0.));
#211251=CARTESIAN_POINT('Ctrl Pts',(16.2580702914615,18.214320612253,12.));
#211252=CARTESIAN_POINT('Ctrl Pts',(16.2791038736223,18.2244223710745,0.));
#211253=CARTESIAN_POINT('Ctrl Pts',(16.2791038736223,18.2244223710745,12.));
#211254=CARTESIAN_POINT('Ctrl Pts',(16.3002435251378,18.2345105028981,0.));
#211255=CARTESIAN_POINT('Ctrl Pts',(16.3002435251378,18.2345105028981,12.));
#211256=CARTESIAN_POINT('Ctrl Pts',(16.3214888370988,18.2445844558742,0.));
#211257=CARTESIAN_POINT('Ctrl Pts',(16.3214888370988,18.2445844558742,12.));
#211258=CARTESIAN_POINT('Ctrl Pts',(16.342839403159,18.2546436839609,0.));
#211259=CARTESIAN_POINT('Ctrl Pts',(16.342839403159,18.2546436839609,12.));
#211260=CARTESIAN_POINT('Ctrl Pts',(16.3642948194869,18.2646876468169,0.));
#211261=CARTESIAN_POINT('Ctrl Pts',(16.3642948194869,18.2646876468169,12.));
#211262=CARTESIAN_POINT('Ctrl Pts',(16.385854684708,18.2747158096934,0.));
#211263=CARTESIAN_POINT('Ctrl Pts',(16.385854684708,18.2747158096934,12.));
#211264=CARTESIAN_POINT('Ctrl Pts',(16.4075185998454,18.2847276433308,0.));
#211265=CARTESIAN_POINT('Ctrl Pts',(16.4075185998454,18.2847276433308,12.));
#211266=CARTESIAN_POINT('Ctrl Pts',(16.4292861682377,18.2947226238509,0.));
#211267=CARTESIAN_POINT('Ctrl Pts',(16.4292861682377,18.2947226238509,12.));
#211268=CARTESIAN_POINT('Ctrl Pts',(16.4511569955231,18.3047002326858,0.));
#211269=CARTESIAN_POINT('Ctrl Pts',(16.4511569955231,18.3047002326858,12.));
#211270=CARTESIAN_POINT('Ctrl Pts',(16.4731306896439,18.3146599565229,0.));
#211271=CARTESIAN_POINT('Ctrl Pts',(16.4731306896439,18.3146599565229,12.));
#211272=CARTESIAN_POINT('Ctrl Pts',(16.4952068608344,18.3246012872468,0.));
#211273=CARTESIAN_POINT('Ctrl Pts',(16.4952068608344,18.3246012872468,12.));
#211274=CARTESIAN_POINT('Ctrl Pts',(16.5173851216045,18.3345237218864,0.));
#211275=CARTESIAN_POINT('Ctrl Pts',(16.5173851216045,18.3345237218864,12.));
#211276=CARTESIAN_POINT('Ctrl Pts',(16.5396650867139,18.3444267625601,0.));
#211277=CARTESIAN_POINT('Ctrl Pts',(16.5396650867139,18.3444267625601,12.));
#211278=CARTESIAN_POINT('Ctrl Pts',(16.5620463731414,18.3543099164331,0.));
#211279=CARTESIAN_POINT('Ctrl Pts',(16.5620463731414,18.3543099164331,12.));
#211280=CARTESIAN_POINT('Ctrl Pts',(16.5845286000218,18.364172695589,0.));
#211281=CARTESIAN_POINT('Ctrl Pts',(16.5845286000218,18.364172695589,12.));
#211282=CARTESIAN_POINT('Ctrl Pts',(16.6071113885711,18.3740146168879,0.));
#211283=CARTESIAN_POINT('Ctrl Pts',(16.6071113885711,18.3740146168879,12.));
#211284=CARTESIAN_POINT('Ctrl Pts',(16.6297943620056,18.3838352018327,0.));
#211285=CARTESIAN_POINT('Ctrl Pts',(16.6297943620056,18.3838352018327,12.));
#211286=CARTESIAN_POINT('Ctrl Pts',(16.6525771454513,18.3936339764332,0.));
#211287=CARTESIAN_POINT('Ctrl Pts',(16.6525771454513,18.3936339764332,12.));
#211288=CARTESIAN_POINT('Ctrl Pts',(16.6754593658513,18.4034104710789,0.));
#211289=CARTESIAN_POINT('Ctrl Pts',(16.6754593658513,18.4034104710789,12.));
#211290=CARTESIAN_POINT('Ctrl Pts',(16.698440651849,18.413164220399,0.));
#211291=CARTESIAN_POINT('Ctrl Pts',(16.698440651849,18.413164220399,12.));
#211292=CARTESIAN_POINT('Ctrl Pts',(16.7215206338818,18.4228947633186,0.));
#211293=CARTESIAN_POINT('Ctrl Pts',(16.7215206338818,18.4228947633186,12.));
#211294=CARTESIAN_POINT('Ctrl Pts',(16.7446989442882,18.4326016431392,0.));
#211295=CARTESIAN_POINT('Ctrl Pts',(16.7446989442882,18.4326016431392,12.));
#211296=CARTESIAN_POINT('Ctrl Pts',(16.7679752173992,18.4422844076099,0.));
#211297=CARTESIAN_POINT('Ctrl Pts',(16.7679752173992,18.4422844076099,12.));
#211298=CARTESIAN_POINT('Ctrl Pts',(16.791349089629,18.4519426090124,0.));
#211299=CARTESIAN_POINT('Ctrl Pts',(16.791349089629,18.4519426090124,12.));
#211300=CARTESIAN_POINT('Ctrl Pts',(16.8148201995472,18.4615758042305,0.));
#211301=CARTESIAN_POINT('Ctrl Pts',(16.8148201995472,18.4615758042305,12.));
#211302=CARTESIAN_POINT('Ctrl Pts',(16.8383881879707,18.4711835548622,0.));
#211303=CARTESIAN_POINT('Ctrl Pts',(16.8383881879707,18.4711835548622,12.));
#211304=CARTESIAN_POINT('Ctrl Pts',(16.8620526977169,18.4807654268769,0.));
#211305=CARTESIAN_POINT('Ctrl Pts',(16.8620526977169,18.4807654268769,12.));
#211306=CARTESIAN_POINT('Ctrl Pts',(16.8858133733086,18.4903209902226,0.));
#211307=CARTESIAN_POINT('Ctrl Pts',(16.8858133733086,18.4903209902226,12.));
#211308=CARTESIAN_POINT('Ctrl Pts',(16.9096698606942,18.4998498184619,0.));
#211309=CARTESIAN_POINT('Ctrl Pts',(16.9096698606942,18.4998498184619,12.));
#211310=CARTESIAN_POINT('Ctrl Pts',(16.9336218069353,18.5093514883835,0.));
#211311=CARTESIAN_POINT('Ctrl Pts',(16.9336218069353,18.5093514883835,12.));
#211312=CARTESIAN_POINT('Ctrl Pts',(16.957668859934,18.518825579666,0.));
#211313=CARTESIAN_POINT('Ctrl Pts',(16.957668859934,18.518825579666,12.));
#211314=CARTESIAN_POINT('Ctrl Pts',(16.9818106680382,18.5282716744198,0.));
#211315=CARTESIAN_POINT('Ctrl Pts',(16.9818106680382,18.5282716744198,12.));
#211316=CARTESIAN_POINT('Ctrl Pts',(17.0060468805099,18.5376893576961,0.));
#211317=CARTESIAN_POINT('Ctrl Pts',(17.0060468805099,18.5376893576961,12.));
#211318=CARTESIAN_POINT('Ctrl Pts',(17.030377148174,18.5470782182089,0.));
#211319=CARTESIAN_POINT('Ctrl Pts',(17.030377148174,18.5470782182089,12.));
#211320=CARTESIAN_POINT('Ctrl Pts',(17.0548011239751,18.5564378489628,0.));
#211321=CARTESIAN_POINT('Ctrl Pts',(17.0548011239751,18.5564378489628,12.));
#211322=CARTESIAN_POINT('Ctrl Pts',(17.0793184636079,18.5657678479788,0.));
#211323=CARTESIAN_POINT('Ctrl Pts',(17.0793184636079,18.5657678479788,12.));
#211324=CARTESIAN_POINT('Ctrl Pts',(17.1039288260001,18.5750678188543,0.));
#211325=CARTESIAN_POINT('Ctrl Pts',(17.1039288260001,18.5750678188543,12.));
#211326=CARTESIAN_POINT('Ctrl Pts',(17.1286318741185,18.5843373717253,0.));
#211327=CARTESIAN_POINT('Ctrl Pts',(17.1286318741185,18.5843373717253,12.));
#211328=CARTESIAN_POINT('Ctrl Pts',(17.1534272741646,18.5935761222833,0.));
#211329=CARTESIAN_POINT('Ctrl Pts',(17.1534272741646,18.5935761222833,12.));
#211330=CARTESIAN_POINT('Ctrl Pts',(17.1783146940131,18.6027836898826,0.));
#211331=CARTESIAN_POINT('Ctrl Pts',(17.1783146940131,18.6027836898826,12.));
#211332=CARTESIAN_POINT('Ctrl Pts',(17.2032938019288,18.6119596959957,0.));
#211333=CARTESIAN_POINT('Ctrl Pts',(17.2032938019288,18.6119596959957,12.));
#211334=CARTESIAN_POINT('Ctrl Pts',(17.2283642650519,18.6211037624041,0.));
#211335=CARTESIAN_POINT('Ctrl Pts',(17.2283642650519,18.6211037624041,12.));
#211336=CARTESIAN_POINT('Ctrl Pts',(17.2535257482186,18.630215509794,0.));
#211337=CARTESIAN_POINT('Ctrl Pts',(17.2535257482186,18.630215509794,12.));
#211338=CARTESIAN_POINT('Ctrl Pts',(17.278777912021,18.639294555474,0.));
#211339=CARTESIAN_POINT('Ctrl Pts',(17.278777912021,18.639294555474,12.));
#211340=CARTESIAN_POINT('Ctrl Pts',(17.3041204135069,18.6483405141853,0.));
#211341=CARTESIAN_POINT('Ctrl Pts',(17.3041204135069,18.6483405141853,12.));
#211342=CARTESIAN_POINT('Ctrl Pts',(17.3295529098612,18.6573530024019,0.));
#211343=CARTESIAN_POINT('Ctrl Pts',(17.3295529098612,18.6573530024019,12.));
#211344=CARTESIAN_POINT('Ctrl Pts',(17.3550750612438,18.6663316416569,0.));
#211345=CARTESIAN_POINT('Ctrl Pts',(17.3550750612438,18.6663316416569,12.));
#211346=CARTESIAN_POINT('Ctrl Pts',(17.3806865340744,18.6752760624045,0.));
#211347=CARTESIAN_POINT('Ctrl Pts',(17.3806865340744,18.6752760624045,12.));
#211348=CARTESIAN_POINT('Ctrl Pts',(17.4063870038563,18.6841859073472,0.));
#211349=CARTESIAN_POINT('Ctrl Pts',(17.4063870038563,18.6841859073472,12.));
#211350=CARTESIAN_POINT('Ctrl Pts',(17.4321761588148,18.6930608357421,0.));
#211351=CARTESIAN_POINT('Ctrl Pts',(17.4321761588148,18.6930608357421,12.));
#211352=CARTESIAN_POINT('Ctrl Pts',(17.4580537012764,18.7019005250322,0.));
#211353=CARTESIAN_POINT('Ctrl Pts',(17.4580537012764,18.7019005250322,12.));
#211354=CARTESIAN_POINT('Ctrl Pts',(17.4840193397176,18.7107046613941,0.));
#211355=CARTESIAN_POINT('Ctrl Pts',(17.4840193397176,18.7107046613941,12.));
#211356=CARTESIAN_POINT('Ctrl Pts',(17.5100727820891,18.7194729318128,0.));
#211357=CARTESIAN_POINT('Ctrl Pts',(17.5100727820891,18.7194729318128,12.));
#211358=CARTESIAN_POINT('Ctrl Pts',(17.5362137287604,18.728205015716,0.));
#211359=CARTESIAN_POINT('Ctrl Pts',(17.5362137287604,18.728205015716,12.));
#211360=CARTESIAN_POINT('Ctrl Pts',(17.5624418653248,18.7369005764558,0.));
#211361=CARTESIAN_POINT('Ctrl Pts',(17.5624418653248,18.7369005764558,12.));
#211362=CARTESIAN_POINT('Ctrl Pts',(17.5887568561361,18.7455592536667,0.));
#211363=CARTESIAN_POINT('Ctrl Pts',(17.5887568561361,18.7455592536667,12.));
#211364=CARTESIAN_POINT('Ctrl Pts',(17.6151583356988,18.7541806530935,0.));
#211365=CARTESIAN_POINT('Ctrl Pts',(17.6151583356988,18.7541806530935,12.));
#211366=CARTESIAN_POINT('Ctrl Pts',(17.6416459210646,18.7627643613139,0.));
#211367=CARTESIAN_POINT('Ctrl Pts',(17.6416459210646,18.7627643613139,12.));
#211368=CARTESIAN_POINT('Ctrl Pts',(17.6682192274197,18.7713099642673,0.));
#211369=CARTESIAN_POINT('Ctrl Pts',(17.6682192274197,18.7713099642673,12.));
#211370=CARTESIAN_POINT('Ctrl Pts',(17.6948778822981,18.7798170641305,0.));
#211371=CARTESIAN_POINT('Ctrl Pts',(17.6948778822981,18.7798170641305,12.));
#211372=CARTESIAN_POINT('Ctrl Pts',(17.7216215409019,18.7882852976016,0.));
#211373=CARTESIAN_POINT('Ctrl Pts',(17.7216215409019,18.7882852976016,12.));
#211374=CARTESIAN_POINT('Ctrl Pts',(17.7484498996916,18.7967143519444,0.));
#211375=CARTESIAN_POINT('Ctrl Pts',(17.7484498996916,18.7967143519444,12.));
#211376=CARTESIAN_POINT('Ctrl Pts',(17.7753627137898,18.8051039860543,0.));
#211377=CARTESIAN_POINT('Ctrl Pts',(17.7753627137898,18.8051039860543,12.));
#211378=CARTESIAN_POINT('Ctrl Pts',(17.8023598011135,18.8134540340581,0.));
#211379=CARTESIAN_POINT('Ctrl Pts',(17.8023598011135,18.8134540340581,12.));
#211380=CARTESIAN_POINT('Ctrl Pts',(17.8294410311105,18.8217643886368,0.));
#211381=CARTESIAN_POINT('Ctrl Pts',(17.8294410311105,18.8217643886368,12.));
#211382=CARTESIAN_POINT('Ctrl Pts',(17.8566063174871,18.8300349896187,0.));
#211383=CARTESIAN_POINT('Ctrl Pts',(17.8566063174871,18.8300349896187,12.));
#211384=CARTESIAN_POINT('Ctrl Pts',(17.8784057509434,18.8366196462746,0.));
#211385=CARTESIAN_POINT('Ctrl Pts',(17.8784057509434,18.8366196462746,12.));
#211386=CARTESIAN_POINT('Ctrl Pts',(17.8947931177853,18.8415402351882,0.));
#211387=CARTESIAN_POINT('Ctrl Pts',(17.8947931177853,18.8415402351882,12.));
#211388=CARTESIAN_POINT('Ctrl Pts',(17.9057348246611,18.8448126709726,0.));
#211389=CARTESIAN_POINT('Ctrl Pts',(17.9057348246611,18.8448126709726,12.));
#211390=CARTESIAN_POINT('Ctrl Pts',(17.9112098770111,18.8464468996588,0.));
#211391=CARTESIAN_POINT('Ctrl Pts',(17.9112098770111,18.8464468996588,12.));
#211392=CARTESIAN_POINT('',(17.9112098770111,18.8464468996588,0.));
#211393=CARTESIAN_POINT('Ctrl Pts',(14.6513681262571,17.1452095830633,0.));
#211394=CARTESIAN_POINT('Ctrl Pts',(14.6513711852843,17.1452153999142,0.));
#211395=CARTESIAN_POINT('Ctrl Pts',(14.6514066997196,17.1452600887037,0.));
#211396=CARTESIAN_POINT('Ctrl Pts',(14.6515481598068,17.1454262858043,0.));
#211397=CARTESIAN_POINT('Ctrl Pts',(14.6519131634508,17.1458462295271,0.));
#211398=CARTESIAN_POINT('Ctrl Pts',(14.6526624064978,17.1466998098673,0.));
#211399=CARTESIAN_POINT('Ctrl Pts',(14.6537016966184,17.147876394491,0.));
#211400=CARTESIAN_POINT('Ctrl Pts',(14.655024862281,17.1493641837558,0.));
#211401=CARTESIAN_POINT('Ctrl Pts',(14.6566237952435,17.1511476869496,0.));
#211402=CARTESIAN_POINT('Ctrl Pts',(14.6584900555302,17.1532107762718,0.));
#211403=CARTESIAN_POINT('Ctrl Pts',(14.6606167169642,17.1555401986401,0.));
#211404=CARTESIAN_POINT('Ctrl Pts',(14.6629987285992,17.1581262646789,0.));
#211405=CARTESIAN_POINT('Ctrl Pts',(14.6656319165057,17.1609609517369,0.));
#211406=CARTESIAN_POINT('Ctrl Pts',(14.6685123374423,17.1640366762305,0.));
#211407=CARTESIAN_POINT('Ctrl Pts',(14.671635583332,17.167344972302,0.));
#211408=CARTESIAN_POINT('Ctrl Pts',(14.6749971333867,17.1708771619129,0.));
#211409=CARTESIAN_POINT('Ctrl Pts',(14.6785925615677,17.1746247499057,0.));
#211410=CARTESIAN_POINT('Ctrl Pts',(14.6824178576167,17.1785800350826,0.));
#211411=CARTESIAN_POINT('Ctrl Pts',(14.686469452232,17.182736158472,0.));
#211412=CARTESIAN_POINT('Ctrl Pts',(14.6907440526958,17.1870867909918,0.));
#211413=CARTESIAN_POINT('Ctrl Pts',(14.6952385361705,17.1916259308415,0.));
#211414=CARTESIAN_POINT('Ctrl Pts',(14.699949811582,17.1963476411694,0.));
#211415=CARTESIAN_POINT('Ctrl Pts',(14.7048748502663,17.2012461084268,0.));
#211416=CARTESIAN_POINT('Ctrl Pts',(14.7100107213586,17.2063157097315,0.));
#211417=CARTESIAN_POINT('Ctrl Pts',(14.7153546289339,17.2115510835989,0.));
#211418=CARTESIAN_POINT('Ctrl Pts',(14.7209039390327,17.2169471814256,0.));
#211419=CARTESIAN_POINT('Ctrl Pts',(14.7266561494282,17.2224992099667,0.));
#211420=CARTESIAN_POINT('Ctrl Pts',(14.7326088681163,17.2282025904314,0.));
#211421=CARTESIAN_POINT('Ctrl Pts',(14.7387597858116,17.2340529062076,0.));
#211422=CARTESIAN_POINT('Ctrl Pts',(14.7451066593792,17.2400458713565,0.));
#211423=CARTESIAN_POINT('Ctrl Pts',(14.7516473175124,17.2461773413288,0.));
#211424=CARTESIAN_POINT('Ctrl Pts',(14.7583796616617,17.2524433146837,0.));
#211425=CARTESIAN_POINT('Ctrl Pts',(14.7653016697591,17.2588399401465,0.));
#211426=CARTESIAN_POINT('Ctrl Pts',(14.7724113956731,17.2653635155319,0.));
#211427=CARTESIAN_POINT('Ctrl Pts',(14.7797069617804,17.2720104735194,0.));
#211428=CARTESIAN_POINT('Ctrl Pts',(14.787186553128,17.2787773704849,0.));
#211429=CARTESIAN_POINT('Ctrl Pts',(14.7948484105249,17.2856608733196,0.));
#211430=CARTESIAN_POINT('Ctrl Pts',(14.8026908254276,17.2926577496513,0.));
#211431=CARTESIAN_POINT('Ctrl Pts',(14.8107121391035,17.299764866148,0.));
#211432=CARTESIAN_POINT('Ctrl Pts',(14.8189107410162,17.3069791853706,0.));
#211433=CARTESIAN_POINT('Ctrl Pts',(14.8272850675379,17.3142977632659,0.));
#211434=CARTESIAN_POINT('Ctrl Pts',(14.8358336004197,17.3217177462101,0.));
#211435=CARTESIAN_POINT('Ctrl Pts',(14.8445548643508,17.3292363662605,0.));
#211436=CARTESIAN_POINT('Ctrl Pts',(14.8534474245433,17.336850936485,0.));
#211437=CARTESIAN_POINT('Ctrl Pts',(14.8625098843417,17.3445588463475,0.));
#211438=CARTESIAN_POINT('Ctrl Pts',(14.8717408826955,17.3523575568645,0.));
#211439=CARTESIAN_POINT('Ctrl Pts',(14.8811390927423,17.3602445978161,0.));
#211440=CARTESIAN_POINT('Ctrl Pts',(14.8907032205788,17.3682175653235,0.));
#211441=CARTESIAN_POINT('Ctrl Pts',(14.900432003961,17.3762741193076,0.));
#211442=CARTESIAN_POINT('Ctrl Pts',(14.9103242110057,17.3844119809824,0.));
#211443=CARTESIAN_POINT('Ctrl Pts',(14.9203786389342,17.3926289303986,0.));
#211444=CARTESIAN_POINT('Ctrl Pts',(14.9305941128757,17.4009228040749,0.));
#211445=CARTESIAN_POINT('Ctrl Pts',(14.940969484645,17.4092914926071,0.));
#211446=CARTESIAN_POINT('Ctrl Pts',(14.9515036315143,17.4177329382828,0.));
#211447=CARTESIAN_POINT('Ctrl Pts',(14.9621954549827,17.426245132709,0.));
#211448=CARTESIAN_POINT('Ctrl Pts',(14.9730438799452,17.4348261151396,0.));
#211449=CARTESIAN_POINT('Ctrl Pts',(14.9840478538358,17.4434739707773,0.));
#211450=CARTESIAN_POINT('Ctrl Pts',(14.9952063457778,17.4521868291004,0.));
#211451=CARTESIAN_POINT('Ctrl Pts',(15.0065183456921,17.4609628621418,0.));
#211452=CARTESIAN_POINT('Ctrl Pts',(15.0179828635086,17.4698002829357,0.));
#211453=CARTESIAN_POINT('Ctrl Pts',(15.029598928488,17.4786973441417,0.));
#211454=CARTESIAN_POINT('Ctrl Pts',(15.0413655884993,17.4876523366178,0.));
#211455=CARTESIAN_POINT('Ctrl Pts',(15.0532819093085,17.4966635880245,0.));
#211456=CARTESIAN_POINT('Ctrl Pts',(15.0653469738306,17.5057294613874,0.));
#211457=CARTESIAN_POINT('Ctrl Pts',(15.0775598815748,17.5148483539684,0.));
#211458=CARTESIAN_POINT('Ctrl Pts',(15.0899197481082,17.5240186961788,0.));
#211459=CARTESIAN_POINT('Ctrl Pts',(15.1024257045033,17.5332389504829,0.));
#211460=CARTESIAN_POINT('Ctrl Pts',(15.1150768967729,17.5425076102966,0.));
#211461=CARTESIAN_POINT('Ctrl Pts',(15.127872485314,17.5518231989122,0.));
#211462=CARTESIAN_POINT('Ctrl Pts',(15.1408116444877,17.5611842686196,0.));
#211463=CARTESIAN_POINT('Ctrl Pts',(15.1538935621714,17.570589399803,0.));
#211464=CARTESIAN_POINT('Ctrl Pts',(15.1671174393136,17.5800372000539,0.));
#211465=CARTESIAN_POINT('Ctrl Pts',(15.1804824894605,17.5895263032592,0.));
#211466=CARTESIAN_POINT('Ctrl Pts',(15.1939879383268,17.5990553687595,0.));
#211467=CARTESIAN_POINT('Ctrl Pts',(15.2076330234686,17.6086230806497,0.));
#211468=CARTESIAN_POINT('Ctrl Pts',(15.22141699392,17.6182281470467,0.));
#211469=CARTESIAN_POINT('Ctrl Pts',(15.2353391098367,17.6278692993765,0.));
#211470=CARTESIAN_POINT('Ctrl Pts',(15.2493986421091,17.637545291637,0.));
#211471=CARTESIAN_POINT('Ctrl Pts',(15.263594872029,17.6472548997329,0.));
#211472=CARTESIAN_POINT('Ctrl Pts',(15.2779270910238,17.6569969209,0.));
#211473=CARTESIAN_POINT('Ctrl Pts',(15.2923946003598,17.6667701731041,0.));
#211474=CARTESIAN_POINT('Ctrl Pts',(15.3069967108501,17.6765734944559,0.));
#211475=CARTESIAN_POINT('Ctrl Pts',(15.3217327425341,17.6864057426052,0.));
#211476=CARTESIAN_POINT('Ctrl Pts',(15.3366020244069,17.6962657941984,0.));
#211477=CARTESIAN_POINT('Ctrl Pts',(15.3516038942064,17.7061525444044,0.));
#211478=CARTESIAN_POINT('Ctrl Pts',(15.3667376981702,17.7160649064208,0.));
#211479=CARTESIAN_POINT('Ctrl Pts',(15.3820027907965,17.7260018109923,0.));
#211480=CARTESIAN_POINT('Ctrl Pts',(15.3973985345796,17.7359622059143,0.));
#211481=CARTESIAN_POINT('Ctrl Pts',(15.4129242997828,17.7459450555803,0.));
#211482=CARTESIAN_POINT('Ctrl Pts',(15.4285794642658,17.7559493405871,0.));
#211483=CARTESIAN_POINT('Ctrl Pts',(15.4443634132865,17.765974057326,0.));
#211484=CARTESIAN_POINT('Ctrl Pts',(15.4602755393019,17.7760182175817,0.));
#211485=CARTESIAN_POINT('Ctrl Pts',(15.4763152417506,17.7860808481229,0.));
#211486=CARTESIAN_POINT('Ctrl Pts',(15.4924819268529,17.7961609903161,0.));
#211487=CARTESIAN_POINT('Ctrl Pts',(15.5087750074728,17.8062576997964,0.));
#211488=CARTESIAN_POINT('Ctrl Pts',(15.5251939029558,17.8163700461263,0.));
#211489=CARTESIAN_POINT('Ctrl Pts',(15.5417380389639,17.8264971124606,0.));
#211490=CARTESIAN_POINT('Ctrl Pts',(15.5584068472976,17.8366379952078,0.));
#211491=CARTESIAN_POINT('Ctrl Pts',(15.5751997657153,17.8467918036977,0.));
#211492=CARTESIAN_POINT('Ctrl Pts',(15.5921162378183,17.8569576598996,0.));
#211493=CARTESIAN_POINT('Ctrl Pts',(15.6091557129205,17.8671346981388,0.));
#211494=CARTESIAN_POINT('Ctrl Pts',(15.6263176459107,17.8773220648125,0.));
#211495=CARTESIAN_POINT('Ctrl Pts',(15.6436014971088,17.8875189181095,0.));
#211496=CARTESIAN_POINT('Ctrl Pts',(15.6610067321036,17.8977244277247,0.));
#211497=CARTESIAN_POINT('Ctrl Pts',(15.6785328216467,17.9079377746118,0.));
#211498=CARTESIAN_POINT('Ctrl Pts',(15.6961792415526,17.918158150746,0.));
#211499=CARTESIAN_POINT('Ctrl Pts',(15.713945472584,17.9283847588837,0.));
#211500=CARTESIAN_POINT('Ctrl Pts',(15.7318310003334,17.9386168123261,0.));
#211501=CARTESIAN_POINT('Ctrl Pts',(15.7498353150856,17.9488535346776,0.));
#211502=CARTESIAN_POINT('Ctrl Pts',(15.7679579117072,17.9590941596236,0.));
#211503=CARTESIAN_POINT('Ctrl Pts',(15.786198289572,17.9693379307297,0.));
#211504=CARTESIAN_POINT('Ctrl Pts',(15.8045559524674,17.9795841012383,0.));
#211505=CARTESIAN_POINT('Ctrl Pts',(15.8230304084963,17.9898319338664,0.));
#211506=CARTESIAN_POINT('Ctrl Pts',(15.8416211699681,18.0000807006055,0.));
#211507=CARTESIAN_POINT('Ctrl Pts',(15.8603277532834,18.010329682521,0.));
#211508=CARTESIAN_POINT('Ctrl Pts',(15.8791496788685,18.0205781695773,0.));
#211509=CARTESIAN_POINT('Ctrl Pts',(15.8980864711043,18.0308254604638,0.));
#211510=CARTESIAN_POINT('Ctrl Pts',(15.9171376582436,18.0410708624208,0.));
#211511=CARTESIAN_POINT('Ctrl Pts',(15.9363027723244,18.0513136910691,0.));
#211512=CARTESIAN_POINT('Ctrl Pts',(15.9555813490645,18.061553270236,0.));
#211513=CARTESIAN_POINT('Ctrl Pts',(15.9749729277848,18.071788931796,0.));
#211514=CARTESIAN_POINT('Ctrl Pts',(15.9944770513616,18.0820200155239,0.));
#211515=CARTESIAN_POINT('Ctrl Pts',(16.0140932661612,18.0922458689464,0.));
#211516=CARTESIAN_POINT('Ctrl Pts',(16.0338211219693,18.1024658471966,0.));
#211517=CARTESIAN_POINT('Ctrl Pts',(16.0536601719124,18.1126793128688,0.));
#211518=CARTESIAN_POINT('Ctrl Pts',(16.0736099723664,18.1228856358746,0.));
#211519=CARTESIAN_POINT('Ctrl Pts',(16.0936700829108,18.1330841933099,0.));
#211520=CARTESIAN_POINT('Ctrl Pts',(16.113840066279,18.1432743693231,0.));
#211521=CARTESIAN_POINT('Ctrl Pts',(16.1341194882987,18.1534555549851,0.));
#211522=CARTESIAN_POINT('Ctrl Pts',(16.1545079178261,18.1636271481616,0.));
#211523=CARTESIAN_POINT('Ctrl Pts',(16.1750049266673,18.1737885533852,0.));
#211524=CARTESIAN_POINT('Ctrl Pts',(16.1956100895076,18.1839391817335,0.));
#211525=CARTESIAN_POINT('Ctrl Pts',(16.2163229838878,18.1940784507232,0.));
#211526=CARTESIAN_POINT('Ctrl Pts',(16.237143190164,18.2042057842037,0.));
#211527=CARTESIAN_POINT('Ctrl Pts',(16.2580702914615,18.214320612253,0.));
#211528=CARTESIAN_POINT('Ctrl Pts',(16.2791038736223,18.2244223710745,0.));
#211529=CARTESIAN_POINT('Ctrl Pts',(16.3002435251378,18.2345105028981,0.));
#211530=CARTESIAN_POINT('Ctrl Pts',(16.3214888370988,18.2445844558742,0.));
#211531=CARTESIAN_POINT('Ctrl Pts',(16.342839403159,18.2546436839609,0.));
#211532=CARTESIAN_POINT('Ctrl Pts',(16.3642948194869,18.2646876468169,0.));
#211533=CARTESIAN_POINT('Ctrl Pts',(16.385854684708,18.2747158096934,0.));
#211534=CARTESIAN_POINT('Ctrl Pts',(16.4075185998454,18.2847276433308,0.));
#211535=CARTESIAN_POINT('Ctrl Pts',(16.4292861682377,18.2947226238509,0.));
#211536=CARTESIAN_POINT('Ctrl Pts',(16.4511569955231,18.3047002326858,0.));
#211537=CARTESIAN_POINT('Ctrl Pts',(16.4731306896439,18.3146599565229,0.));
#211538=CARTESIAN_POINT('Ctrl Pts',(16.4952068608344,18.3246012872468,0.));
#211539=CARTESIAN_POINT('Ctrl Pts',(16.5173851216045,18.3345237218864,0.));
#211540=CARTESIAN_POINT('Ctrl Pts',(16.5396650867139,18.3444267625601,0.));
#211541=CARTESIAN_POINT('Ctrl Pts',(16.5620463731414,18.3543099164331,0.));
#211542=CARTESIAN_POINT('Ctrl Pts',(16.5845286000218,18.364172695589,0.));
#211543=CARTESIAN_POINT('Ctrl Pts',(16.6071113885711,18.3740146168879,0.));
#211544=CARTESIAN_POINT('Ctrl Pts',(16.6297943620056,18.3838352018327,0.));
#211545=CARTESIAN_POINT('Ctrl Pts',(16.6525771454513,18.3936339764332,0.));
#211546=CARTESIAN_POINT('Ctrl Pts',(16.6754593658513,18.4034104710789,0.));
#211547=CARTESIAN_POINT('Ctrl Pts',(16.698440651849,18.413164220399,0.));
#211548=CARTESIAN_POINT('Ctrl Pts',(16.7215206338818,18.4228947633186,0.));
#211549=CARTESIAN_POINT('Ctrl Pts',(16.7446989442882,18.4326016431392,0.));
#211550=CARTESIAN_POINT('Ctrl Pts',(16.7679752173992,18.4422844076099,0.));
#211551=CARTESIAN_POINT('Ctrl Pts',(16.791349089629,18.4519426090124,0.));
#211552=CARTESIAN_POINT('Ctrl Pts',(16.8148201995472,18.4615758042305,0.));
#211553=CARTESIAN_POINT('Ctrl Pts',(16.8383881879707,18.4711835548622,0.));
#211554=CARTESIAN_POINT('Ctrl Pts',(16.8620526977169,18.4807654268769,0.));
#211555=CARTESIAN_POINT('Ctrl Pts',(16.8858133733086,18.4903209902226,0.));
#211556=CARTESIAN_POINT('Ctrl Pts',(16.9096698606942,18.4998498184619,0.));
#211557=CARTESIAN_POINT('Ctrl Pts',(16.9336218069353,18.5093514883835,0.));
#211558=CARTESIAN_POINT('Ctrl Pts',(16.957668859934,18.518825579666,0.));
#211559=CARTESIAN_POINT('Ctrl Pts',(16.9818106680382,18.5282716744198,0.));
#211560=CARTESIAN_POINT('Ctrl Pts',(17.0060468805099,18.5376893576961,0.));
#211561=CARTESIAN_POINT('Ctrl Pts',(17.030377148174,18.5470782182089,0.));
#211562=CARTESIAN_POINT('Ctrl Pts',(17.0548011239751,18.5564378489628,0.));
#211563=CARTESIAN_POINT('Ctrl Pts',(17.0793184636079,18.5657678479788,0.));
#211564=CARTESIAN_POINT('Ctrl Pts',(17.1039288260001,18.5750678188543,0.));
#211565=CARTESIAN_POINT('Ctrl Pts',(17.1286318741185,18.5843373717253,0.));
#211566=CARTESIAN_POINT('Ctrl Pts',(17.1534272741646,18.5935761222833,0.));
#211567=CARTESIAN_POINT('Ctrl Pts',(17.1783146940131,18.6027836898826,0.));
#211568=CARTESIAN_POINT('Ctrl Pts',(17.2032938019288,18.6119596959957,0.));
#211569=CARTESIAN_POINT('Ctrl Pts',(17.2283642650519,18.6211037624041,0.));
#211570=CARTESIAN_POINT('Ctrl Pts',(17.2535257482186,18.630215509794,0.));
#211571=CARTESIAN_POINT('Ctrl Pts',(17.278777912021,18.639294555474,0.));
#211572=CARTESIAN_POINT('Ctrl Pts',(17.3041204135069,18.6483405141853,0.));
#211573=CARTESIAN_POINT('Ctrl Pts',(17.3295529098612,18.6573530024019,0.));
#211574=CARTESIAN_POINT('Ctrl Pts',(17.3550750612438,18.6663316416569,0.));
#211575=CARTESIAN_POINT('Ctrl Pts',(17.3806865340744,18.6752760624045,0.));
#211576=CARTESIAN_POINT('Ctrl Pts',(17.4063870038563,18.6841859073472,0.));
#211577=CARTESIAN_POINT('Ctrl Pts',(17.4321761588148,18.6930608357421,0.));
#211578=CARTESIAN_POINT('Ctrl Pts',(17.4580537012764,18.7019005250322,0.));
#211579=CARTESIAN_POINT('Ctrl Pts',(17.4840193397176,18.7107046613941,0.));
#211580=CARTESIAN_POINT('Ctrl Pts',(17.5100727820891,18.7194729318128,0.));
#211581=CARTESIAN_POINT('Ctrl Pts',(17.5362137287604,18.728205015716,0.));
#211582=CARTESIAN_POINT('Ctrl Pts',(17.5624418653248,18.7369005764558,0.));
#211583=CARTESIAN_POINT('Ctrl Pts',(17.5887568561361,18.7455592536667,0.));
#211584=CARTESIAN_POINT('Ctrl Pts',(17.6151583356988,18.7541806530935,0.));
#211585=CARTESIAN_POINT('Ctrl Pts',(17.6416459210646,18.7627643613139,0.));
#211586=CARTESIAN_POINT('Ctrl Pts',(17.6682192274197,18.7713099642673,0.));
#211587=CARTESIAN_POINT('Ctrl Pts',(17.6948778822981,18.7798170641305,0.));
#211588=CARTESIAN_POINT('Ctrl Pts',(17.7216215409019,18.7882852976016,0.));
#211589=CARTESIAN_POINT('Ctrl Pts',(17.7484498996916,18.7967143519444,0.));
#211590=CARTESIAN_POINT('Ctrl Pts',(17.7753627137898,18.8051039860543,0.));
#211591=CARTESIAN_POINT('Ctrl Pts',(17.8023598011135,18.8134540340581,0.));
#211592=CARTESIAN_POINT('Ctrl Pts',(17.8294410311105,18.8217643886368,0.));
#211593=CARTESIAN_POINT('Ctrl Pts',(17.8566063174871,18.8300349896187,0.));
#211594=CARTESIAN_POINT('Ctrl Pts',(17.8784057509434,18.8366196462746,0.));
#211595=CARTESIAN_POINT('Ctrl Pts',(17.8947931177853,18.8415402351882,0.));
#211596=CARTESIAN_POINT('Ctrl Pts',(17.9057348246611,18.8448126709726,0.));
#211597=CARTESIAN_POINT('Ctrl Pts',(17.9112098770111,18.8464468996588,0.));
#211598=CARTESIAN_POINT('',(17.9112098770111,18.8464468996588,0.));
#211599=CARTESIAN_POINT('Origin',(17.7219872369693,12.1729687575668,0.));
#211600=CARTESIAN_POINT('',(18.5896416359912,12.7689476255363,0.));
#211601=CARTESIAN_POINT('',(18.5896416359912,12.7689476255363,0.));
#211602=CARTESIAN_POINT('',(8.86099361848466,6.08648437878338,0.));
#211603=CARTESIAN_POINT('Ctrl Pts',(18.8464468996588,17.9112098770111,0.));
#211604=CARTESIAN_POINT('Ctrl Pts',(18.8464468996588,17.9112098770111,12.));
#211605=CARTESIAN_POINT('Ctrl Pts',(18.8448126709691,17.9057348246595,0.));
#211606=CARTESIAN_POINT('Ctrl Pts',(18.8448126709691,17.9057348246595,12.));
#211607=CARTESIAN_POINT('Ctrl Pts',(18.8415402351786,17.8947931177807,0.));
#211608=CARTESIAN_POINT('Ctrl Pts',(18.8415402351786,17.8947931177807,12.));
#211609=CARTESIAN_POINT('Ctrl Pts',(18.8366196462581,17.8784057509356,0.));
#211610=CARTESIAN_POINT('Ctrl Pts',(18.8366196462581,17.8784057509356,12.));
#211611=CARTESIAN_POINT('Ctrl Pts',(18.8300349895974,17.8566063174771,0.));
#211612=CARTESIAN_POINT('Ctrl Pts',(18.8300349895974,17.8566063174771,12.));
#211613=CARTESIAN_POINT('Ctrl Pts',(18.8217643886157,17.8294410311006,0.));
#211614=CARTESIAN_POINT('Ctrl Pts',(18.8217643886157,17.8294410311006,12.));
#211615=CARTESIAN_POINT('Ctrl Pts',(18.8134540340417,17.8023598011057,0.));
#211616=CARTESIAN_POINT('Ctrl Pts',(18.8134540340417,17.8023598011057,12.));
#211617=CARTESIAN_POINT('Ctrl Pts',(18.8051039860448,17.7753627137853,0.));
#211618=CARTESIAN_POINT('Ctrl Pts',(18.8051039860448,17.7753627137853,12.));
#211619=CARTESIAN_POINT('Ctrl Pts',(18.7967143519419,17.7484498996905,0.));
#211620=CARTESIAN_POINT('Ctrl Pts',(18.7967143519419,17.7484498996905,12.));
#211621=CARTESIAN_POINT('Ctrl Pts',(18.7882852976049,17.7216215409035,0.));
#211622=CARTESIAN_POINT('Ctrl Pts',(18.7882852976049,17.7216215409035,12.));
#211623=CARTESIAN_POINT('Ctrl Pts',(18.7798170641374,17.6948778823014,0.));
#211624=CARTESIAN_POINT('Ctrl Pts',(18.7798170641374,17.6948778823014,12.));
#211625=CARTESIAN_POINT('Ctrl Pts',(18.7713099642754,17.6682192274236,0.));
#211626=CARTESIAN_POINT('Ctrl Pts',(18.7713099642754,17.6682192274236,12.));
#211627=CARTESIAN_POINT('Ctrl Pts',(18.762764361321,17.6416459210681,0.));
#211628=CARTESIAN_POINT('Ctrl Pts',(18.762764361321,17.6416459210681,12.));
#211629=CARTESIAN_POINT('Ctrl Pts',(18.7541806530984,17.6151583357012,0.));
#211630=CARTESIAN_POINT('Ctrl Pts',(18.7541806530984,17.6151583357012,12.));
#211631=CARTESIAN_POINT('Ctrl Pts',(18.7455592536687,17.5887568561371,0.));
#211632=CARTESIAN_POINT('Ctrl Pts',(18.7455592536687,17.5887568561371,12.));
#211633=CARTESIAN_POINT('Ctrl Pts',(18.7369005764553,17.5624418653245,0.));
#211634=CARTESIAN_POINT('Ctrl Pts',(18.7369005764553,17.5624418653245,12.));
#211635=CARTESIAN_POINT('Ctrl Pts',(18.7282050157138,17.5362137287593,0.));
#211636=CARTESIAN_POINT('Ctrl Pts',(18.7282050157138,17.5362137287593,12.));
#211637=CARTESIAN_POINT('Ctrl Pts',(18.7194729318098,17.5100727820876,0.));
#211638=CARTESIAN_POINT('Ctrl Pts',(18.7194729318098,17.5100727820876,12.));
#211639=CARTESIAN_POINT('Ctrl Pts',(18.7107046613912,17.4840193397162,0.));
#211640=CARTESIAN_POINT('Ctrl Pts',(18.7107046613912,17.4840193397162,12.));
#211641=CARTESIAN_POINT('Ctrl Pts',(18.70190052503,17.4580537012753,0.));
#211642=CARTESIAN_POINT('Ctrl Pts',(18.70190052503,17.4580537012753,12.));
#211643=CARTESIAN_POINT('Ctrl Pts',(18.6930608357409,17.4321761588142,0.));
#211644=CARTESIAN_POINT('Ctrl Pts',(18.6930608357409,17.4321761588142,12.));
#211645=CARTESIAN_POINT('Ctrl Pts',(18.6841859073471,17.4063870038562,0.));
#211646=CARTESIAN_POINT('Ctrl Pts',(18.6841859073471,17.4063870038562,12.));
#211647=CARTESIAN_POINT('Ctrl Pts',(18.6752760624052,17.3806865340747,0.));
#211648=CARTESIAN_POINT('Ctrl Pts',(18.6752760624052,17.3806865340747,12.));
#211649=CARTESIAN_POINT('Ctrl Pts',(18.6663316416582,17.3550750612443,0.));
#211650=CARTESIAN_POINT('Ctrl Pts',(18.6663316416582,17.3550750612443,12.));
#211651=CARTESIAN_POINT('Ctrl Pts',(18.6573530024033,17.3295529098618,0.));
#211652=CARTESIAN_POINT('Ctrl Pts',(18.6573530024033,17.3295529098618,12.));
#211653=CARTESIAN_POINT('Ctrl Pts',(18.6483405141865,17.3041204135074,0.));
#211654=CARTESIAN_POINT('Ctrl Pts',(18.6483405141865,17.3041204135074,12.));
#211655=CARTESIAN_POINT('Ctrl Pts',(18.6392945554748,17.2787779120213,0.));
#211656=CARTESIAN_POINT('Ctrl Pts',(18.6392945554748,17.2787779120213,12.));
#211657=CARTESIAN_POINT('Ctrl Pts',(18.6302155097943,17.2535257482187,0.));
#211658=CARTESIAN_POINT('Ctrl Pts',(18.6302155097943,17.2535257482187,12.));
#211659=CARTESIAN_POINT('Ctrl Pts',(18.6211037624038,17.2283642650518,0.));
#211660=CARTESIAN_POINT('Ctrl Pts',(18.6211037624038,17.2283642650518,12.));
#211661=CARTESIAN_POINT('Ctrl Pts',(18.6119596959949,17.2032938019284,0.));
#211662=CARTESIAN_POINT('Ctrl Pts',(18.6119596959949,17.2032938019284,12.));
#211663=CARTESIAN_POINT('Ctrl Pts',(18.6027836898817,17.1783146940127,0.));
#211664=CARTESIAN_POINT('Ctrl Pts',(18.6027836898817,17.1783146940127,12.));
#211665=CARTESIAN_POINT('Ctrl Pts',(18.5935761222825,17.1534272741643,0.));
#211666=CARTESIAN_POINT('Ctrl Pts',(18.5935761222825,17.1534272741643,12.));
#211667=CARTESIAN_POINT('Ctrl Pts',(18.5843373717247,17.1286318741183,0.));
#211668=CARTESIAN_POINT('Ctrl Pts',(18.5843373717247,17.1286318741183,12.));
#211669=CARTESIAN_POINT('Ctrl Pts',(18.5750678188542,17.1039288260001,0.));
#211670=CARTESIAN_POINT('Ctrl Pts',(18.5750678188542,17.1039288260001,12.));
#211671=CARTESIAN_POINT('Ctrl Pts',(18.5657678479789,17.0793184636079,0.));
#211672=CARTESIAN_POINT('Ctrl Pts',(18.5657678479789,17.0793184636079,12.));
#211673=CARTESIAN_POINT('Ctrl Pts',(18.556437848963,17.0548011239751,0.));
#211674=CARTESIAN_POINT('Ctrl Pts',(18.556437848963,17.0548011239751,12.));
#211675=CARTESIAN_POINT('Ctrl Pts',(18.547078218209,17.0303771481738,0.));
#211676=CARTESIAN_POINT('Ctrl Pts',(18.547078218209,17.0303771481738,12.));
#211677=CARTESIAN_POINT('Ctrl Pts',(18.5376893576961,17.0060468805097,0.));
#211678=CARTESIAN_POINT('Ctrl Pts',(18.5376893576961,17.0060468805097,12.));
#211679=CARTESIAN_POINT('Ctrl Pts',(18.5282716744197,16.981810668038,0.));
#211680=CARTESIAN_POINT('Ctrl Pts',(18.5282716744197,16.981810668038,12.));
#211681=CARTESIAN_POINT('Ctrl Pts',(18.5188255796659,16.9576688599339,0.));
#211682=CARTESIAN_POINT('Ctrl Pts',(18.5188255796659,16.9576688599339,12.));
#211683=CARTESIAN_POINT('Ctrl Pts',(18.5093514883835,16.9336218069353,0.));
#211684=CARTESIAN_POINT('Ctrl Pts',(18.5093514883835,16.9336218069353,12.));
#211685=CARTESIAN_POINT('Ctrl Pts',(18.499849818462,16.9096698606943,0.));
#211686=CARTESIAN_POINT('Ctrl Pts',(18.499849818462,16.9096698606943,12.));
#211687=CARTESIAN_POINT('Ctrl Pts',(18.4903209902227,16.8858133733088,0.));
#211688=CARTESIAN_POINT('Ctrl Pts',(18.4903209902227,16.8858133733088,12.));
#211689=CARTESIAN_POINT('Ctrl Pts',(18.4807654268771,16.8620526977171,0.));
#211690=CARTESIAN_POINT('Ctrl Pts',(18.4807654268771,16.8620526977171,12.));
#211691=CARTESIAN_POINT('Ctrl Pts',(18.4711835548623,16.8383881879709,0.));
#211692=CARTESIAN_POINT('Ctrl Pts',(18.4711835548623,16.8383881879709,12.));
#211693=CARTESIAN_POINT('Ctrl Pts',(18.4615758042305,16.8148201995472,0.));
#211694=CARTESIAN_POINT('Ctrl Pts',(18.4615758042305,16.8148201995472,12.));
#211695=CARTESIAN_POINT('Ctrl Pts',(18.4519426090123,16.791349089629,0.));
#211696=CARTESIAN_POINT('Ctrl Pts',(18.4519426090123,16.791349089629,12.));
#211697=CARTESIAN_POINT('Ctrl Pts',(18.44228440761,16.7679752173992,0.));
#211698=CARTESIAN_POINT('Ctrl Pts',(18.44228440761,16.7679752173992,12.));
#211699=CARTESIAN_POINT('Ctrl Pts',(18.4326016431392,16.7446989442882,0.));
#211700=CARTESIAN_POINT('Ctrl Pts',(18.4326016431392,16.7446989442882,12.));
#211701=CARTESIAN_POINT('Ctrl Pts',(18.4228947633187,16.7215206338818,0.));
#211702=CARTESIAN_POINT('Ctrl Pts',(18.4228947633187,16.7215206338818,12.));
#211703=CARTESIAN_POINT('Ctrl Pts',(18.413164220399,16.6984406518491,0.));
#211704=CARTESIAN_POINT('Ctrl Pts',(18.413164220399,16.6984406518491,12.));
#211705=CARTESIAN_POINT('Ctrl Pts',(18.403410471079,16.6754593658513,0.));
#211706=CARTESIAN_POINT('Ctrl Pts',(18.403410471079,16.6754593658513,12.));
#211707=CARTESIAN_POINT('Ctrl Pts',(18.3936339764332,16.6525771454513,0.));
#211708=CARTESIAN_POINT('Ctrl Pts',(18.3936339764332,16.6525771454513,12.));
#211709=CARTESIAN_POINT('Ctrl Pts',(18.3838352018327,16.6297943620056,0.));
#211710=CARTESIAN_POINT('Ctrl Pts',(18.3838352018327,16.6297943620056,12.));
#211711=CARTESIAN_POINT('Ctrl Pts',(18.3740146168879,16.607111388571,0.));
#211712=CARTESIAN_POINT('Ctrl Pts',(18.3740146168879,16.607111388571,12.));
#211713=CARTESIAN_POINT('Ctrl Pts',(18.3641726955889,16.5845286000217,0.));
#211714=CARTESIAN_POINT('Ctrl Pts',(18.3641726955889,16.5845286000217,12.));
#211715=CARTESIAN_POINT('Ctrl Pts',(18.354309916433,16.5620463731413,0.));
#211716=CARTESIAN_POINT('Ctrl Pts',(18.354309916433,16.5620463731413,12.));
#211717=CARTESIAN_POINT('Ctrl Pts',(18.34442676256,16.5396650867139,0.));
#211718=CARTESIAN_POINT('Ctrl Pts',(18.34442676256,16.5396650867139,12.));
#211719=CARTESIAN_POINT('Ctrl Pts',(18.3345237218864,16.5173851216045,0.));
#211720=CARTESIAN_POINT('Ctrl Pts',(18.3345237218864,16.5173851216045,12.));
#211721=CARTESIAN_POINT('Ctrl Pts',(18.3246012872469,16.4952068608345,0.));
#211722=CARTESIAN_POINT('Ctrl Pts',(18.3246012872469,16.4952068608345,12.));
#211723=CARTESIAN_POINT('Ctrl Pts',(18.3146599565231,16.4731306896441,0.));
#211724=CARTESIAN_POINT('Ctrl Pts',(18.3146599565231,16.4731306896441,12.));
#211725=CARTESIAN_POINT('Ctrl Pts',(18.304700232686,16.4511569955233,0.));
#211726=CARTESIAN_POINT('Ctrl Pts',(18.304700232686,16.4511569955233,12.));
#211727=CARTESIAN_POINT('Ctrl Pts',(18.294722623851,16.4292861682379,0.));
#211728=CARTESIAN_POINT('Ctrl Pts',(18.294722623851,16.4292861682379,12.));
#211729=CARTESIAN_POINT('Ctrl Pts',(18.2847276433309,16.4075185998455,0.));
#211730=CARTESIAN_POINT('Ctrl Pts',(18.2847276433309,16.4075185998455,12.));
#211731=CARTESIAN_POINT('Ctrl Pts',(18.2747158096934,16.385854684708,0.));
#211732=CARTESIAN_POINT('Ctrl Pts',(18.2747158096934,16.385854684708,12.));
#211733=CARTESIAN_POINT('Ctrl Pts',(18.2646876468169,16.3642948194868,0.));
#211734=CARTESIAN_POINT('Ctrl Pts',(18.2646876468169,16.3642948194868,12.));
#211735=CARTESIAN_POINT('Ctrl Pts',(18.2546436839608,16.3428394031589,0.));
#211736=CARTESIAN_POINT('Ctrl Pts',(18.2546436839608,16.3428394031589,12.));
#211737=CARTESIAN_POINT('Ctrl Pts',(18.2445844558742,16.3214888370987,0.));
#211738=CARTESIAN_POINT('Ctrl Pts',(18.2445844558742,16.3214888370987,12.));
#211739=CARTESIAN_POINT('Ctrl Pts',(18.2345105028982,16.3002435251378,0.));
#211740=CARTESIAN_POINT('Ctrl Pts',(18.2345105028982,16.3002435251378,12.));
#211741=CARTESIAN_POINT('Ctrl Pts',(18.2244223710745,16.2791038736223,0.));
#211742=CARTESIAN_POINT('Ctrl Pts',(18.2244223710745,16.2791038736223,12.));
#211743=CARTESIAN_POINT('Ctrl Pts',(18.2143206122529,16.2580702914615,0.));
#211744=CARTESIAN_POINT('Ctrl Pts',(18.2143206122529,16.2580702914615,12.));
#211745=CARTESIAN_POINT('Ctrl Pts',(18.2042057842035,16.2371431901638,0.));
#211746=CARTESIAN_POINT('Ctrl Pts',(18.2042057842035,16.2371431901638,12.));
#211747=CARTESIAN_POINT('Ctrl Pts',(18.1940784507229,16.2163229838875,0.));
#211748=CARTESIAN_POINT('Ctrl Pts',(18.1940784507229,16.2163229838875,12.));
#211749=CARTESIAN_POINT('Ctrl Pts',(18.1839391817331,16.1956100895073,0.));
#211750=CARTESIAN_POINT('Ctrl Pts',(18.1839391817331,16.1956100895073,12.));
#211751=CARTESIAN_POINT('Ctrl Pts',(18.1737885533849,16.1750049266671,0.));
#211752=CARTESIAN_POINT('Ctrl Pts',(18.1737885533849,16.1750049266671,12.));
#211753=CARTESIAN_POINT('Ctrl Pts',(18.1636271481615,16.154507917826,0.));
#211754=CARTESIAN_POINT('Ctrl Pts',(18.1636271481615,16.154507917826,12.));
#211755=CARTESIAN_POINT('Ctrl Pts',(18.1534555549852,16.1341194882988,0.));
#211756=CARTESIAN_POINT('Ctrl Pts',(18.1534555549852,16.1341194882988,12.));
#211757=CARTESIAN_POINT('Ctrl Pts',(18.1432743693235,16.1138400662794,0.));
#211758=CARTESIAN_POINT('Ctrl Pts',(18.1432743693235,16.1138400662794,12.));
#211759=CARTESIAN_POINT('Ctrl Pts',(18.1330841933105,16.0936700829112,0.));
#211760=CARTESIAN_POINT('Ctrl Pts',(18.1330841933105,16.0936700829112,12.));
#211761=CARTESIAN_POINT('Ctrl Pts',(18.1228856358751,16.0736099723668,0.));
#211762=CARTESIAN_POINT('Ctrl Pts',(18.1228856358751,16.0736099723668,12.));
#211763=CARTESIAN_POINT('Ctrl Pts',(18.112679312869,16.0536601719126,0.));
#211764=CARTESIAN_POINT('Ctrl Pts',(18.112679312869,16.0536601719126,12.));
#211765=CARTESIAN_POINT('Ctrl Pts',(18.1024658471966,16.0338211219693,0.));
#211766=CARTESIAN_POINT('Ctrl Pts',(18.1024658471966,16.0338211219693,12.));
#211767=CARTESIAN_POINT('Ctrl Pts',(18.0922458689462,16.014093266161,0.));
#211768=CARTESIAN_POINT('Ctrl Pts',(18.0922458689462,16.014093266161,12.));
#211769=CARTESIAN_POINT('Ctrl Pts',(18.0820200155236,15.9944770513613,0.));
#211770=CARTESIAN_POINT('Ctrl Pts',(18.0820200155236,15.9944770513613,12.));
#211771=CARTESIAN_POINT('Ctrl Pts',(18.0717889317958,15.9749729277846,0.));
#211772=CARTESIAN_POINT('Ctrl Pts',(18.0717889317958,15.9749729277846,12.));
#211773=CARTESIAN_POINT('Ctrl Pts',(18.061553270236,15.9555813490644,0.));
#211774=CARTESIAN_POINT('Ctrl Pts',(18.061553270236,15.9555813490644,12.));
#211775=CARTESIAN_POINT('Ctrl Pts',(18.0513136910691,15.9363027723244,0.));
#211776=CARTESIAN_POINT('Ctrl Pts',(18.0513136910691,15.9363027723244,12.));
#211777=CARTESIAN_POINT('Ctrl Pts',(18.0410708624208,15.9171376582436,0.));
#211778=CARTESIAN_POINT('Ctrl Pts',(18.0410708624208,15.9171376582436,12.));
#211779=CARTESIAN_POINT('Ctrl Pts',(18.0308254604636,15.8980864711042,0.));
#211780=CARTESIAN_POINT('Ctrl Pts',(18.0308254604636,15.8980864711042,12.));
#211781=CARTESIAN_POINT('Ctrl Pts',(18.0205781695769,15.8791496788683,0.));
#211782=CARTESIAN_POINT('Ctrl Pts',(18.0205781695769,15.8791496788683,12.));
#211783=CARTESIAN_POINT('Ctrl Pts',(18.0103296825205,15.8603277532831,0.));
#211784=CARTESIAN_POINT('Ctrl Pts',(18.0103296825205,15.8603277532831,12.));
#211785=CARTESIAN_POINT('Ctrl Pts',(18.0000807006052,15.8416211699679,0.));
#211786=CARTESIAN_POINT('Ctrl Pts',(18.0000807006052,15.8416211699679,12.));
#211787=CARTESIAN_POINT('Ctrl Pts',(17.9898319338664,15.8230304084962,0.));
#211788=CARTESIAN_POINT('Ctrl Pts',(17.9898319338664,15.8230304084962,12.));
#211789=CARTESIAN_POINT('Ctrl Pts',(17.9795841012386,15.8045559524677,0.));
#211790=CARTESIAN_POINT('Ctrl Pts',(17.9795841012386,15.8045559524677,12.));
#211791=CARTESIAN_POINT('Ctrl Pts',(17.9693379307303,15.7861982895724,0.));
#211792=CARTESIAN_POINT('Ctrl Pts',(17.9693379307303,15.7861982895724,12.));
#211793=CARTESIAN_POINT('Ctrl Pts',(17.9590941596242,15.7679579117077,0.));
#211794=CARTESIAN_POINT('Ctrl Pts',(17.9590941596242,15.7679579117077,12.));
#211795=CARTESIAN_POINT('Ctrl Pts',(17.9488535346781,15.749835315086,0.));
#211796=CARTESIAN_POINT('Ctrl Pts',(17.9488535346781,15.749835315086,12.));
#211797=CARTESIAN_POINT('Ctrl Pts',(17.9386168123262,15.7318310003335,0.));
#211798=CARTESIAN_POINT('Ctrl Pts',(17.9386168123262,15.7318310003335,12.));
#211799=CARTESIAN_POINT('Ctrl Pts',(17.9283847588836,15.7139454725839,0.));
#211800=CARTESIAN_POINT('Ctrl Pts',(17.9283847588836,15.7139454725839,12.));
#211801=CARTESIAN_POINT('Ctrl Pts',(17.9181581507455,15.6961792415522,0.));
#211802=CARTESIAN_POINT('Ctrl Pts',(17.9181581507455,15.6961792415522,12.));
#211803=CARTESIAN_POINT('Ctrl Pts',(17.9079377746111,15.6785328216461,0.));
#211804=CARTESIAN_POINT('Ctrl Pts',(17.9079377746111,15.6785328216461,12.));
#211805=CARTESIAN_POINT('Ctrl Pts',(17.897724427724,15.661006732103,0.));
#211806=CARTESIAN_POINT('Ctrl Pts',(17.897724427724,15.661006732103,12.));
#211807=CARTESIAN_POINT('Ctrl Pts',(17.8875189181091,15.6436014971085,0.));
#211808=CARTESIAN_POINT('Ctrl Pts',(17.8875189181091,15.6436014971085,12.));
#211809=CARTESIAN_POINT('Ctrl Pts',(17.8773220648125,15.6263176459108,0.));
#211810=CARTESIAN_POINT('Ctrl Pts',(17.8773220648125,15.6263176459108,12.));
#211811=CARTESIAN_POINT('Ctrl Pts',(17.8671346981394,15.609155712921,0.));
#211812=CARTESIAN_POINT('Ctrl Pts',(17.8671346981394,15.609155712921,12.));
#211813=CARTESIAN_POINT('Ctrl Pts',(17.8569576599006,15.5921162378192,0.));
#211814=CARTESIAN_POINT('Ctrl Pts',(17.8569576599006,15.5921162378192,12.));
#211815=CARTESIAN_POINT('Ctrl Pts',(17.8467918036987,15.5751997657163,0.));
#211816=CARTESIAN_POINT('Ctrl Pts',(17.8467918036987,15.5751997657163,12.));
#211817=CARTESIAN_POINT('Ctrl Pts',(17.8366379952085,15.5584068472982,0.));
#211818=CARTESIAN_POINT('Ctrl Pts',(17.8366379952085,15.5584068472982,12.));
#211819=CARTESIAN_POINT('Ctrl Pts',(17.8264971124606,15.541738038964,0.));
#211820=CARTESIAN_POINT('Ctrl Pts',(17.8264971124606,15.541738038964,12.));
#211821=CARTESIAN_POINT('Ctrl Pts',(17.8163700461256,15.5251939029552,0.));
#211822=CARTESIAN_POINT('Ctrl Pts',(17.8163700461256,15.5251939029552,12.));
#211823=CARTESIAN_POINT('Ctrl Pts',(17.8062576997952,15.5087750074718,0.));
#211824=CARTESIAN_POINT('Ctrl Pts',(17.8062576997952,15.5087750074718,12.));
#211825=CARTESIAN_POINT('Ctrl Pts',(17.7961609903148,15.4924819268517,0.));
#211826=CARTESIAN_POINT('Ctrl Pts',(17.7961609903148,15.4924819268517,12.));
#211827=CARTESIAN_POINT('Ctrl Pts',(17.7860808481219,15.4763152417497,0.));
#211828=CARTESIAN_POINT('Ctrl Pts',(17.7860808481219,15.4763152417497,12.));
#211829=CARTESIAN_POINT('Ctrl Pts',(17.7760182175815,15.4602755393018,0.));
#211830=CARTESIAN_POINT('Ctrl Pts',(17.7760182175815,15.4602755393018,12.));
#211831=CARTESIAN_POINT('Ctrl Pts',(17.7659740573265,15.4443634132869,0.));
#211832=CARTESIAN_POINT('Ctrl Pts',(17.7659740573265,15.4443634132869,12.));
#211833=CARTESIAN_POINT('Ctrl Pts',(17.7559493405881,15.4285794642668,0.));
#211834=CARTESIAN_POINT('Ctrl Pts',(17.7559493405881,15.4285794642668,12.));
#211835=CARTESIAN_POINT('Ctrl Pts',(17.7459450555812,15.4129242997837,0.));
#211836=CARTESIAN_POINT('Ctrl Pts',(17.7459450555812,15.4129242997837,12.));
#211837=CARTESIAN_POINT('Ctrl Pts',(17.7359622059149,15.3973985345802,0.));
#211838=CARTESIAN_POINT('Ctrl Pts',(17.7359622059149,15.3973985345802,12.));
#211839=CARTESIAN_POINT('Ctrl Pts',(17.7260018109924,15.3820027907967,0.));
#211840=CARTESIAN_POINT('Ctrl Pts',(17.7260018109924,15.3820027907967,12.));
#211841=CARTESIAN_POINT('Ctrl Pts',(17.7160649064206,15.3667376981699,0.));
#211842=CARTESIAN_POINT('Ctrl Pts',(17.7160649064206,15.3667376981699,12.));
#211843=CARTESIAN_POINT('Ctrl Pts',(17.7061525444042,15.351603894206,0.));
#211844=CARTESIAN_POINT('Ctrl Pts',(17.7061525444042,15.351603894206,12.));
#211845=CARTESIAN_POINT('Ctrl Pts',(17.6962657941983,15.3366020244066,0.));
#211846=CARTESIAN_POINT('Ctrl Pts',(17.6962657941983,15.3366020244066,12.));
#211847=CARTESIAN_POINT('Ctrl Pts',(17.6864057426052,15.3217327425338,0.));
#211848=CARTESIAN_POINT('Ctrl Pts',(17.6864057426052,15.3217327425338,12.));
#211849=CARTESIAN_POINT('Ctrl Pts',(17.676573494456,15.3069967108501,0.));
#211850=CARTESIAN_POINT('Ctrl Pts',(17.676573494456,15.3069967108501,12.));
#211851=CARTESIAN_POINT('Ctrl Pts',(17.6667701731041,15.2923946003598,0.));
#211852=CARTESIAN_POINT('Ctrl Pts',(17.6667701731041,15.2923946003598,12.));
#211853=CARTESIAN_POINT('Ctrl Pts',(17.6569969209,15.2779270910239,0.));
#211854=CARTESIAN_POINT('Ctrl Pts',(17.6569969209,15.2779270910239,12.));
#211855=CARTESIAN_POINT('Ctrl Pts',(17.6472548997328,15.2635948720292,0.));
#211856=CARTESIAN_POINT('Ctrl Pts',(17.6472548997328,15.2635948720292,12.));
#211857=CARTESIAN_POINT('Ctrl Pts',(17.6375452916369,15.2493986421092,0.));
#211858=CARTESIAN_POINT('Ctrl Pts',(17.6375452916369,15.2493986421092,12.));
#211859=CARTESIAN_POINT('Ctrl Pts',(17.6278692993764,15.2353391098367,0.));
#211860=CARTESIAN_POINT('Ctrl Pts',(17.6278692993764,15.2353391098367,12.));
#211861=CARTESIAN_POINT('Ctrl Pts',(17.6182281470468,15.22141699392,0.));
#211862=CARTESIAN_POINT('Ctrl Pts',(17.6182281470468,15.22141699392,12.));
#211863=CARTESIAN_POINT('Ctrl Pts',(17.60862308065,15.2076330234686,0.));
#211864=CARTESIAN_POINT('Ctrl Pts',(17.60862308065,15.2076330234686,12.));
#211865=CARTESIAN_POINT('Ctrl Pts',(17.5990553687599,15.1939879383268,0.));
#211866=CARTESIAN_POINT('Ctrl Pts',(17.5990553687599,15.1939879383268,12.));
#211867=CARTESIAN_POINT('Ctrl Pts',(17.5895263032595,15.1804824894605,0.));
#211868=CARTESIAN_POINT('Ctrl Pts',(17.5895263032595,15.1804824894605,12.));
#211869=CARTESIAN_POINT('Ctrl Pts',(17.580037200054,15.1671174393137,0.));
#211870=CARTESIAN_POINT('Ctrl Pts',(17.580037200054,15.1671174393137,12.));
#211871=CARTESIAN_POINT('Ctrl Pts',(17.5705893998029,15.1538935621714,0.));
#211872=CARTESIAN_POINT('Ctrl Pts',(17.5705893998029,15.1538935621714,12.));
#211873=CARTESIAN_POINT('Ctrl Pts',(17.5611842686192,15.1408116444876,0.));
#211874=CARTESIAN_POINT('Ctrl Pts',(17.5611842686192,15.1408116444876,12.));
#211875=CARTESIAN_POINT('Ctrl Pts',(17.5518231989117,15.1278724853138,0.));
#211876=CARTESIAN_POINT('Ctrl Pts',(17.5518231989117,15.1278724853138,12.));
#211877=CARTESIAN_POINT('Ctrl Pts',(17.5425076102963,15.1150768967728,0.));
#211878=CARTESIAN_POINT('Ctrl Pts',(17.5425076102963,15.1150768967728,12.));
#211879=CARTESIAN_POINT('Ctrl Pts',(17.5332389504829,15.1024257045033,0.));
#211880=CARTESIAN_POINT('Ctrl Pts',(17.5332389504829,15.1024257045033,12.));
#211881=CARTESIAN_POINT('Ctrl Pts',(17.524018696179,15.0899197481082,0.));
#211882=CARTESIAN_POINT('Ctrl Pts',(17.524018696179,15.0899197481082,12.));
#211883=CARTESIAN_POINT('Ctrl Pts',(17.5148483539687,15.0775598815749,0.));
#211884=CARTESIAN_POINT('Ctrl Pts',(17.5148483539687,15.0775598815749,12.));
#211885=CARTESIAN_POINT('Ctrl Pts',(17.5057294613877,15.0653469738307,0.));
#211886=CARTESIAN_POINT('Ctrl Pts',(17.5057294613877,15.0653469738307,12.));
#211887=CARTESIAN_POINT('Ctrl Pts',(17.4966635880246,15.0532819093085,0.));
#211888=CARTESIAN_POINT('Ctrl Pts',(17.4966635880246,15.0532819093085,12.));
#211889=CARTESIAN_POINT('Ctrl Pts',(17.4876523366178,15.0413655884993,0.));
#211890=CARTESIAN_POINT('Ctrl Pts',(17.4876523366178,15.0413655884993,12.));
#211891=CARTESIAN_POINT('Ctrl Pts',(17.4786973441417,15.029598928488,0.));
#211892=CARTESIAN_POINT('Ctrl Pts',(17.4786973441417,15.029598928488,12.));
#211893=CARTESIAN_POINT('Ctrl Pts',(17.4698002829357,15.0179828635087,0.));
#211894=CARTESIAN_POINT('Ctrl Pts',(17.4698002829357,15.0179828635087,12.));
#211895=CARTESIAN_POINT('Ctrl Pts',(17.4609628621419,15.0065183456923,0.));
#211896=CARTESIAN_POINT('Ctrl Pts',(17.4609628621419,15.0065183456923,12.));
#211897=CARTESIAN_POINT('Ctrl Pts',(17.4521868291005,14.9952063457779,0.));
#211898=CARTESIAN_POINT('Ctrl Pts',(17.4521868291005,14.9952063457779,12.));
#211899=CARTESIAN_POINT('Ctrl Pts',(17.4434739707773,14.9840478538357,0.));
#211900=CARTESIAN_POINT('Ctrl Pts',(17.4434739707773,14.9840478538357,12.));
#211901=CARTESIAN_POINT('Ctrl Pts',(17.4348261151395,14.973043879945,0.));
#211902=CARTESIAN_POINT('Ctrl Pts',(17.4348261151395,14.973043879945,12.));
#211903=CARTESIAN_POINT('Ctrl Pts',(17.4262451327088,14.9621954549825,0.));
#211904=CARTESIAN_POINT('Ctrl Pts',(17.4262451327088,14.9621954549825,12.));
#211905=CARTESIAN_POINT('Ctrl Pts',(17.4177329382827,14.9515036315142,0.));
#211906=CARTESIAN_POINT('Ctrl Pts',(17.4177329382827,14.9515036315142,12.));
#211907=CARTESIAN_POINT('Ctrl Pts',(17.4092914926071,14.940969484645,0.));
#211908=CARTESIAN_POINT('Ctrl Pts',(17.4092914926071,14.940969484645,12.));
#211909=CARTESIAN_POINT('Ctrl Pts',(17.400922804075,14.9305941128758,0.));
#211910=CARTESIAN_POINT('Ctrl Pts',(17.400922804075,14.9305941128758,12.));
#211911=CARTESIAN_POINT('Ctrl Pts',(17.3926289303987,14.9203786389343,0.));
#211912=CARTESIAN_POINT('Ctrl Pts',(17.3926289303987,14.9203786389343,12.));
#211913=CARTESIAN_POINT('Ctrl Pts',(17.3844119809823,14.9103242110057,0.));
#211914=CARTESIAN_POINT('Ctrl Pts',(17.3844119809823,14.9103242110057,12.));
#211915=CARTESIAN_POINT('Ctrl Pts',(17.3762741193075,14.9004320039609,0.));
#211916=CARTESIAN_POINT('Ctrl Pts',(17.3762741193075,14.9004320039609,12.));
#211917=CARTESIAN_POINT('Ctrl Pts',(17.3682175653236,14.8907032205789,0.));
#211918=CARTESIAN_POINT('Ctrl Pts',(17.3682175653236,14.8907032205789,12.));
#211919=CARTESIAN_POINT('Ctrl Pts',(17.3602445978163,14.8811390927424,0.));
#211920=CARTESIAN_POINT('Ctrl Pts',(17.3602445978163,14.8811390927424,12.));
#211921=CARTESIAN_POINT('Ctrl Pts',(17.3523575568648,14.8717408826958,0.));
#211922=CARTESIAN_POINT('Ctrl Pts',(17.3523575568648,14.8717408826958,12.));
#211923=CARTESIAN_POINT('Ctrl Pts',(17.3445588463477,14.8625098843419,0.));
#211924=CARTESIAN_POINT('Ctrl Pts',(17.3445588463477,14.8625098843419,12.));
#211925=CARTESIAN_POINT('Ctrl Pts',(17.336850936485,14.8534474245433,0.));
#211926=CARTESIAN_POINT('Ctrl Pts',(17.336850936485,14.8534474245433,12.));
#211927=CARTESIAN_POINT('Ctrl Pts',(17.3292363662601,14.8445548643505,0.));
#211928=CARTESIAN_POINT('Ctrl Pts',(17.3292363662601,14.8445548643505,12.));
#211929=CARTESIAN_POINT('Ctrl Pts',(17.3217177462096,14.8358336004193,0.));
#211930=CARTESIAN_POINT('Ctrl Pts',(17.3217177462096,14.8358336004193,12.));
#211931=CARTESIAN_POINT('Ctrl Pts',(17.3142977632656,14.8272850675375,0.));
#211932=CARTESIAN_POINT('Ctrl Pts',(17.3142977632656,14.8272850675375,12.));
#211933=CARTESIAN_POINT('Ctrl Pts',(17.3069791853705,14.8189107410161,0.));
#211934=CARTESIAN_POINT('Ctrl Pts',(17.3069791853705,14.8189107410161,12.));
#211935=CARTESIAN_POINT('Ctrl Pts',(17.2997648661483,14.8107121391038,0.));
#211936=CARTESIAN_POINT('Ctrl Pts',(17.2997648661483,14.8107121391038,12.));
#211937=CARTESIAN_POINT('Ctrl Pts',(17.2926577496519,14.8026908254281,0.));
#211938=CARTESIAN_POINT('Ctrl Pts',(17.2926577496519,14.8026908254281,12.));
#211939=CARTESIAN_POINT('Ctrl Pts',(17.28566087332,14.7948484105253,0.));
#211940=CARTESIAN_POINT('Ctrl Pts',(17.28566087332,14.7948484105253,12.));
#211941=CARTESIAN_POINT('Ctrl Pts',(17.278777370485,14.787186553128,0.));
#211942=CARTESIAN_POINT('Ctrl Pts',(17.278777370485,14.787186553128,12.));
#211943=CARTESIAN_POINT('Ctrl Pts',(17.2720104735192,14.7797069617802,0.));
#211944=CARTESIAN_POINT('Ctrl Pts',(17.2720104735192,14.7797069617802,12.));
#211945=CARTESIAN_POINT('Ctrl Pts',(17.2653635155317,14.7724113956728,0.));
#211946=CARTESIAN_POINT('Ctrl Pts',(17.2653635155317,14.7724113956728,12.));
#211947=CARTESIAN_POINT('Ctrl Pts',(17.2588399401464,14.7653016697589,0.));
#211948=CARTESIAN_POINT('Ctrl Pts',(17.2588399401464,14.7653016697589,12.));
#211949=CARTESIAN_POINT('Ctrl Pts',(17.2524433146837,14.7583796616617,0.));
#211950=CARTESIAN_POINT('Ctrl Pts',(17.2524433146837,14.7583796616617,12.));
#211951=CARTESIAN_POINT('Ctrl Pts',(17.2461773413289,14.7516473175125,0.));
#211952=CARTESIAN_POINT('Ctrl Pts',(17.2461773413289,14.7516473175125,12.));
#211953=CARTESIAN_POINT('Ctrl Pts',(17.2400458713566,14.7451066593793,0.));
#211954=CARTESIAN_POINT('Ctrl Pts',(17.2400458713566,14.7451066593793,12.));
#211955=CARTESIAN_POINT('Ctrl Pts',(17.2340529062077,14.7387597858117,0.));
#211956=CARTESIAN_POINT('Ctrl Pts',(17.2340529062077,14.7387597858117,12.));
#211957=CARTESIAN_POINT('Ctrl Pts',(17.2282025904314,14.7326088681163,0.));
#211958=CARTESIAN_POINT('Ctrl Pts',(17.2282025904314,14.7326088681163,12.));
#211959=CARTESIAN_POINT('Ctrl Pts',(17.2224992099666,14.7266561494282,0.));
#211960=CARTESIAN_POINT('Ctrl Pts',(17.2224992099666,14.7266561494282,12.));
#211961=CARTESIAN_POINT('Ctrl Pts',(17.2169471814255,14.7209039390326,0.));
#211962=CARTESIAN_POINT('Ctrl Pts',(17.2169471814255,14.7209039390326,12.));
#211963=CARTESIAN_POINT('Ctrl Pts',(17.2115510835988,14.7153546289338,0.));
#211964=CARTESIAN_POINT('Ctrl Pts',(17.2115510835988,14.7153546289338,12.));
#211965=CARTESIAN_POINT('Ctrl Pts',(17.2063157097316,14.7100107213587,0.));
#211966=CARTESIAN_POINT('Ctrl Pts',(17.2063157097316,14.7100107213587,12.));
#211967=CARTESIAN_POINT('Ctrl Pts',(17.2012461084268,14.7048748502663,0.));
#211968=CARTESIAN_POINT('Ctrl Pts',(17.2012461084268,14.7048748502663,12.));
#211969=CARTESIAN_POINT('Ctrl Pts',(17.1963476411694,14.699949811582,0.));
#211970=CARTESIAN_POINT('Ctrl Pts',(17.1963476411694,14.699949811582,12.));
#211971=CARTESIAN_POINT('Ctrl Pts',(17.1916259308415,14.6952385361706,0.));
#211972=CARTESIAN_POINT('Ctrl Pts',(17.1916259308415,14.6952385361706,12.));
#211973=CARTESIAN_POINT('Ctrl Pts',(17.1870867909918,14.6907440526958,0.));
#211974=CARTESIAN_POINT('Ctrl Pts',(17.1870867909918,14.6907440526958,12.));
#211975=CARTESIAN_POINT('Ctrl Pts',(17.182736158472,14.6864694522319,0.));
#211976=CARTESIAN_POINT('Ctrl Pts',(17.182736158472,14.6864694522319,12.));
#211977=CARTESIAN_POINT('Ctrl Pts',(17.1785800350827,14.6824178576167,0.));
#211978=CARTESIAN_POINT('Ctrl Pts',(17.1785800350827,14.6824178576167,12.));
#211979=CARTESIAN_POINT('Ctrl Pts',(17.1746247499057,14.6785925615676,0.));
#211980=CARTESIAN_POINT('Ctrl Pts',(17.1746247499057,14.6785925615676,12.));
#211981=CARTESIAN_POINT('Ctrl Pts',(17.1708771619129,14.6749971333867,0.));
#211982=CARTESIAN_POINT('Ctrl Pts',(17.1708771619129,14.6749971333867,12.));
#211983=CARTESIAN_POINT('Ctrl Pts',(17.1673449723019,14.6716355833321,0.));
#211984=CARTESIAN_POINT('Ctrl Pts',(17.1673449723019,14.6716355833321,12.));
#211985=CARTESIAN_POINT('Ctrl Pts',(17.1640366762304,14.6685123374424,0.));
#211986=CARTESIAN_POINT('Ctrl Pts',(17.1640366762304,14.6685123374424,12.));
#211987=CARTESIAN_POINT('Ctrl Pts',(17.1609609517369,14.6656319165057,0.));
#211988=CARTESIAN_POINT('Ctrl Pts',(17.1609609517369,14.6656319165057,12.));
#211989=CARTESIAN_POINT('Ctrl Pts',(17.1581262646789,14.662998728599,0.));
#211990=CARTESIAN_POINT('Ctrl Pts',(17.1581262646789,14.662998728599,12.));
#211991=CARTESIAN_POINT('Ctrl Pts',(17.1555401986403,14.660616716964,0.));
#211992=CARTESIAN_POINT('Ctrl Pts',(17.1555401986403,14.660616716964,12.));
#211993=CARTESIAN_POINT('Ctrl Pts',(17.1532107762719,14.6584900555301,0.));
#211994=CARTESIAN_POINT('Ctrl Pts',(17.1532107762719,14.6584900555301,12.));
#211995=CARTESIAN_POINT('Ctrl Pts',(17.1511476869495,14.6566237952435,0.));
#211996=CARTESIAN_POINT('Ctrl Pts',(17.1511476869495,14.6566237952435,12.));
#211997=CARTESIAN_POINT('Ctrl Pts',(17.1493641837556,14.6550248622813,0.));
#211998=CARTESIAN_POINT('Ctrl Pts',(17.1493641837556,14.6550248622813,12.));
#211999=CARTESIAN_POINT('Ctrl Pts',(17.1478763944909,14.6537016966188,0.));
#212000=CARTESIAN_POINT('Ctrl Pts',(17.1478763944909,14.6537016966188,12.));
#212001=CARTESIAN_POINT('Ctrl Pts',(17.1466998098673,14.6526624064978,0.));
#212002=CARTESIAN_POINT('Ctrl Pts',(17.1466998098673,14.6526624064978,12.));
#212003=CARTESIAN_POINT('Ctrl Pts',(17.1458462295273,14.65191316345,0.));
#212004=CARTESIAN_POINT('Ctrl Pts',(17.1458462295273,14.65191316345,12.));
#212005=CARTESIAN_POINT('Ctrl Pts',(17.1454262858045,14.6515481598057,0.));
#212006=CARTESIAN_POINT('Ctrl Pts',(17.1454262858045,14.6515481598057,12.));
#212007=CARTESIAN_POINT('Ctrl Pts',(17.1452600887039,14.6514066997188,0.));
#212008=CARTESIAN_POINT('Ctrl Pts',(17.1452600887039,14.6514066997188,12.));
#212009=CARTESIAN_POINT('Ctrl Pts',(17.1452153999142,14.651371185284,0.));
#212010=CARTESIAN_POINT('Ctrl Pts',(17.1452153999142,14.651371185284,12.));
#212011=CARTESIAN_POINT('Ctrl Pts',(17.1452095830633,14.6513681262571,0.));
#212012=CARTESIAN_POINT('Ctrl Pts',(17.1452095830633,14.6513681262571,12.));
#212013=CARTESIAN_POINT('',(18.8464468996588,17.9112098770111,0.));
#212014=CARTESIAN_POINT('Ctrl Pts',(18.8464468996588,17.9112098770111,0.));
#212015=CARTESIAN_POINT('Ctrl Pts',(18.8448126709691,17.9057348246595,0.));
#212016=CARTESIAN_POINT('Ctrl Pts',(18.8415402351786,17.8947931177807,0.));
#212017=CARTESIAN_POINT('Ctrl Pts',(18.8366196462581,17.8784057509356,0.));
#212018=CARTESIAN_POINT('Ctrl Pts',(18.8300349895974,17.8566063174771,0.));
#212019=CARTESIAN_POINT('Ctrl Pts',(18.8217643886157,17.8294410311006,0.));
#212020=CARTESIAN_POINT('Ctrl Pts',(18.8134540340417,17.8023598011057,0.));
#212021=CARTESIAN_POINT('Ctrl Pts',(18.8051039860448,17.7753627137853,0.));
#212022=CARTESIAN_POINT('Ctrl Pts',(18.7967143519419,17.7484498996905,0.));
#212023=CARTESIAN_POINT('Ctrl Pts',(18.7882852976049,17.7216215409035,0.));
#212024=CARTESIAN_POINT('Ctrl Pts',(18.7798170641374,17.6948778823014,0.));
#212025=CARTESIAN_POINT('Ctrl Pts',(18.7713099642754,17.6682192274236,0.));
#212026=CARTESIAN_POINT('Ctrl Pts',(18.762764361321,17.6416459210681,0.));
#212027=CARTESIAN_POINT('Ctrl Pts',(18.7541806530984,17.6151583357012,0.));
#212028=CARTESIAN_POINT('Ctrl Pts',(18.7455592536687,17.5887568561371,0.));
#212029=CARTESIAN_POINT('Ctrl Pts',(18.7369005764553,17.5624418653245,0.));
#212030=CARTESIAN_POINT('Ctrl Pts',(18.7282050157138,17.5362137287593,0.));
#212031=CARTESIAN_POINT('Ctrl Pts',(18.7194729318098,17.5100727820876,0.));
#212032=CARTESIAN_POINT('Ctrl Pts',(18.7107046613912,17.4840193397162,0.));
#212033=CARTESIAN_POINT('Ctrl Pts',(18.70190052503,17.4580537012753,0.));
#212034=CARTESIAN_POINT('Ctrl Pts',(18.6930608357409,17.4321761588142,0.));
#212035=CARTESIAN_POINT('Ctrl Pts',(18.6841859073471,17.4063870038562,0.));
#212036=CARTESIAN_POINT('Ctrl Pts',(18.6752760624052,17.3806865340747,0.));
#212037=CARTESIAN_POINT('Ctrl Pts',(18.6663316416582,17.3550750612443,0.));
#212038=CARTESIAN_POINT('Ctrl Pts',(18.6573530024033,17.3295529098618,0.));
#212039=CARTESIAN_POINT('Ctrl Pts',(18.6483405141865,17.3041204135074,0.));
#212040=CARTESIAN_POINT('Ctrl Pts',(18.6392945554748,17.2787779120213,0.));
#212041=CARTESIAN_POINT('Ctrl Pts',(18.6302155097943,17.2535257482187,0.));
#212042=CARTESIAN_POINT('Ctrl Pts',(18.6211037624038,17.2283642650518,0.));
#212043=CARTESIAN_POINT('Ctrl Pts',(18.6119596959949,17.2032938019284,0.));
#212044=CARTESIAN_POINT('Ctrl Pts',(18.6027836898817,17.1783146940127,0.));
#212045=CARTESIAN_POINT('Ctrl Pts',(18.5935761222825,17.1534272741643,0.));
#212046=CARTESIAN_POINT('Ctrl Pts',(18.5843373717247,17.1286318741183,0.));
#212047=CARTESIAN_POINT('Ctrl Pts',(18.5750678188542,17.1039288260001,0.));
#212048=CARTESIAN_POINT('Ctrl Pts',(18.5657678479789,17.0793184636079,0.));
#212049=CARTESIAN_POINT('Ctrl Pts',(18.556437848963,17.0548011239751,0.));
#212050=CARTESIAN_POINT('Ctrl Pts',(18.547078218209,17.0303771481738,0.));
#212051=CARTESIAN_POINT('Ctrl Pts',(18.5376893576961,17.0060468805097,0.));
#212052=CARTESIAN_POINT('Ctrl Pts',(18.5282716744197,16.981810668038,0.));
#212053=CARTESIAN_POINT('Ctrl Pts',(18.5188255796659,16.9576688599339,0.));
#212054=CARTESIAN_POINT('Ctrl Pts',(18.5093514883835,16.9336218069353,0.));
#212055=CARTESIAN_POINT('Ctrl Pts',(18.499849818462,16.9096698606943,0.));
#212056=CARTESIAN_POINT('Ctrl Pts',(18.4903209902227,16.8858133733088,0.));
#212057=CARTESIAN_POINT('Ctrl Pts',(18.4807654268771,16.8620526977171,0.));
#212058=CARTESIAN_POINT('Ctrl Pts',(18.4711835548623,16.8383881879709,0.));
#212059=CARTESIAN_POINT('Ctrl Pts',(18.4615758042305,16.8148201995472,0.));
#212060=CARTESIAN_POINT('Ctrl Pts',(18.4519426090123,16.791349089629,0.));
#212061=CARTESIAN_POINT('Ctrl Pts',(18.44228440761,16.7679752173992,0.));
#212062=CARTESIAN_POINT('Ctrl Pts',(18.4326016431392,16.7446989442882,0.));
#212063=CARTESIAN_POINT('Ctrl Pts',(18.4228947633187,16.7215206338818,0.));
#212064=CARTESIAN_POINT('Ctrl Pts',(18.413164220399,16.6984406518491,0.));
#212065=CARTESIAN_POINT('Ctrl Pts',(18.403410471079,16.6754593658513,0.));
#212066=CARTESIAN_POINT('Ctrl Pts',(18.3936339764332,16.6525771454513,0.));
#212067=CARTESIAN_POINT('Ctrl Pts',(18.3838352018327,16.6297943620056,0.));
#212068=CARTESIAN_POINT('Ctrl Pts',(18.3740146168879,16.607111388571,0.));
#212069=CARTESIAN_POINT('Ctrl Pts',(18.3641726955889,16.5845286000217,0.));
#212070=CARTESIAN_POINT('Ctrl Pts',(18.354309916433,16.5620463731413,0.));
#212071=CARTESIAN_POINT('Ctrl Pts',(18.34442676256,16.5396650867139,0.));
#212072=CARTESIAN_POINT('Ctrl Pts',(18.3345237218864,16.5173851216045,0.));
#212073=CARTESIAN_POINT('Ctrl Pts',(18.3246012872469,16.4952068608345,0.));
#212074=CARTESIAN_POINT('Ctrl Pts',(18.3146599565231,16.4731306896441,0.));
#212075=CARTESIAN_POINT('Ctrl Pts',(18.304700232686,16.4511569955233,0.));
#212076=CARTESIAN_POINT('Ctrl Pts',(18.294722623851,16.4292861682379,0.));
#212077=CARTESIAN_POINT('Ctrl Pts',(18.2847276433309,16.4075185998455,0.));
#212078=CARTESIAN_POINT('Ctrl Pts',(18.2747158096934,16.385854684708,0.));
#212079=CARTESIAN_POINT('Ctrl Pts',(18.2646876468169,16.3642948194868,0.));
#212080=CARTESIAN_POINT('Ctrl Pts',(18.2546436839608,16.3428394031589,0.));
#212081=CARTESIAN_POINT('Ctrl Pts',(18.2445844558742,16.3214888370987,0.));
#212082=CARTESIAN_POINT('Ctrl Pts',(18.2345105028982,16.3002435251378,0.));
#212083=CARTESIAN_POINT('Ctrl Pts',(18.2244223710745,16.2791038736223,0.));
#212084=CARTESIAN_POINT('Ctrl Pts',(18.2143206122529,16.2580702914615,0.));
#212085=CARTESIAN_POINT('Ctrl Pts',(18.2042057842035,16.2371431901638,0.));
#212086=CARTESIAN_POINT('Ctrl Pts',(18.1940784507229,16.2163229838875,0.));
#212087=CARTESIAN_POINT('Ctrl Pts',(18.1839391817331,16.1956100895073,0.));
#212088=CARTESIAN_POINT('Ctrl Pts',(18.1737885533849,16.1750049266671,0.));
#212089=CARTESIAN_POINT('Ctrl Pts',(18.1636271481615,16.154507917826,0.));
#212090=CARTESIAN_POINT('Ctrl Pts',(18.1534555549852,16.1341194882988,0.));
#212091=CARTESIAN_POINT('Ctrl Pts',(18.1432743693235,16.1138400662794,0.));
#212092=CARTESIAN_POINT('Ctrl Pts',(18.1330841933105,16.0936700829112,0.));
#212093=CARTESIAN_POINT('Ctrl Pts',(18.1228856358751,16.0736099723668,0.));
#212094=CARTESIAN_POINT('Ctrl Pts',(18.112679312869,16.0536601719126,0.));
#212095=CARTESIAN_POINT('Ctrl Pts',(18.1024658471966,16.0338211219693,0.));
#212096=CARTESIAN_POINT('Ctrl Pts',(18.0922458689462,16.014093266161,0.));
#212097=CARTESIAN_POINT('Ctrl Pts',(18.0820200155236,15.9944770513613,0.));
#212098=CARTESIAN_POINT('Ctrl Pts',(18.0717889317958,15.9749729277846,0.));
#212099=CARTESIAN_POINT('Ctrl Pts',(18.061553270236,15.9555813490644,0.));
#212100=CARTESIAN_POINT('Ctrl Pts',(18.0513136910691,15.9363027723244,0.));
#212101=CARTESIAN_POINT('Ctrl Pts',(18.0410708624208,15.9171376582436,0.));
#212102=CARTESIAN_POINT('Ctrl Pts',(18.0308254604636,15.8980864711042,0.));
#212103=CARTESIAN_POINT('Ctrl Pts',(18.0205781695769,15.8791496788683,0.));
#212104=CARTESIAN_POINT('Ctrl Pts',(18.0103296825205,15.8603277532831,0.));
#212105=CARTESIAN_POINT('Ctrl Pts',(18.0000807006052,15.8416211699679,0.));
#212106=CARTESIAN_POINT('Ctrl Pts',(17.9898319338664,15.8230304084962,0.));
#212107=CARTESIAN_POINT('Ctrl Pts',(17.9795841012386,15.8045559524677,0.));
#212108=CARTESIAN_POINT('Ctrl Pts',(17.9693379307303,15.7861982895724,0.));
#212109=CARTESIAN_POINT('Ctrl Pts',(17.9590941596242,15.7679579117077,0.));
#212110=CARTESIAN_POINT('Ctrl Pts',(17.9488535346781,15.749835315086,0.));
#212111=CARTESIAN_POINT('Ctrl Pts',(17.9386168123262,15.7318310003335,0.));
#212112=CARTESIAN_POINT('Ctrl Pts',(17.9283847588836,15.7139454725839,0.));
#212113=CARTESIAN_POINT('Ctrl Pts',(17.9181581507455,15.6961792415522,0.));
#212114=CARTESIAN_POINT('Ctrl Pts',(17.9079377746111,15.6785328216461,0.));
#212115=CARTESIAN_POINT('Ctrl Pts',(17.897724427724,15.661006732103,0.));
#212116=CARTESIAN_POINT('Ctrl Pts',(17.8875189181091,15.6436014971085,0.));
#212117=CARTESIAN_POINT('Ctrl Pts',(17.8773220648125,15.6263176459108,0.));
#212118=CARTESIAN_POINT('Ctrl Pts',(17.8671346981394,15.609155712921,0.));
#212119=CARTESIAN_POINT('Ctrl Pts',(17.8569576599006,15.5921162378192,0.));
#212120=CARTESIAN_POINT('Ctrl Pts',(17.8467918036987,15.5751997657163,0.));
#212121=CARTESIAN_POINT('Ctrl Pts',(17.8366379952085,15.5584068472982,0.));
#212122=CARTESIAN_POINT('Ctrl Pts',(17.8264971124606,15.541738038964,0.));
#212123=CARTESIAN_POINT('Ctrl Pts',(17.8163700461256,15.5251939029552,0.));
#212124=CARTESIAN_POINT('Ctrl Pts',(17.8062576997952,15.5087750074718,0.));
#212125=CARTESIAN_POINT('Ctrl Pts',(17.7961609903148,15.4924819268517,0.));
#212126=CARTESIAN_POINT('Ctrl Pts',(17.7860808481219,15.4763152417497,0.));
#212127=CARTESIAN_POINT('Ctrl Pts',(17.7760182175815,15.4602755393018,0.));
#212128=CARTESIAN_POINT('Ctrl Pts',(17.7659740573265,15.4443634132869,0.));
#212129=CARTESIAN_POINT('Ctrl Pts',(17.7559493405881,15.4285794642668,0.));
#212130=CARTESIAN_POINT('Ctrl Pts',(17.7459450555812,15.4129242997837,0.));
#212131=CARTESIAN_POINT('Ctrl Pts',(17.7359622059149,15.3973985345802,0.));
#212132=CARTESIAN_POINT('Ctrl Pts',(17.7260018109924,15.3820027907967,0.));
#212133=CARTESIAN_POINT('Ctrl Pts',(17.7160649064206,15.3667376981699,0.));
#212134=CARTESIAN_POINT('Ctrl Pts',(17.7061525444042,15.351603894206,0.));
#212135=CARTESIAN_POINT('Ctrl Pts',(17.6962657941983,15.3366020244066,0.));
#212136=CARTESIAN_POINT('Ctrl Pts',(17.6864057426052,15.3217327425338,0.));
#212137=CARTESIAN_POINT('Ctrl Pts',(17.676573494456,15.3069967108501,0.));
#212138=CARTESIAN_POINT('Ctrl Pts',(17.6667701731041,15.2923946003598,0.));
#212139=CARTESIAN_POINT('Ctrl Pts',(17.6569969209,15.2779270910239,0.));
#212140=CARTESIAN_POINT('Ctrl Pts',(17.6472548997328,15.2635948720292,0.));
#212141=CARTESIAN_POINT('Ctrl Pts',(17.6375452916369,15.2493986421092,0.));
#212142=CARTESIAN_POINT('Ctrl Pts',(17.6278692993764,15.2353391098367,0.));
#212143=CARTESIAN_POINT('Ctrl Pts',(17.6182281470468,15.22141699392,0.));
#212144=CARTESIAN_POINT('Ctrl Pts',(17.60862308065,15.2076330234686,0.));
#212145=CARTESIAN_POINT('Ctrl Pts',(17.5990553687599,15.1939879383268,0.));
#212146=CARTESIAN_POINT('Ctrl Pts',(17.5895263032595,15.1804824894605,0.));
#212147=CARTESIAN_POINT('Ctrl Pts',(17.580037200054,15.1671174393137,0.));
#212148=CARTESIAN_POINT('Ctrl Pts',(17.5705893998029,15.1538935621714,0.));
#212149=CARTESIAN_POINT('Ctrl Pts',(17.5611842686192,15.1408116444876,0.));
#212150=CARTESIAN_POINT('Ctrl Pts',(17.5518231989117,15.1278724853138,0.));
#212151=CARTESIAN_POINT('Ctrl Pts',(17.5425076102963,15.1150768967728,0.));
#212152=CARTESIAN_POINT('Ctrl Pts',(17.5332389504829,15.1024257045033,0.));
#212153=CARTESIAN_POINT('Ctrl Pts',(17.524018696179,15.0899197481082,0.));
#212154=CARTESIAN_POINT('Ctrl Pts',(17.5148483539687,15.0775598815749,0.));
#212155=CARTESIAN_POINT('Ctrl Pts',(17.5057294613877,15.0653469738307,0.));
#212156=CARTESIAN_POINT('Ctrl Pts',(17.4966635880246,15.0532819093085,0.));
#212157=CARTESIAN_POINT('Ctrl Pts',(17.4876523366178,15.0413655884993,0.));
#212158=CARTESIAN_POINT('Ctrl Pts',(17.4786973441417,15.029598928488,0.));
#212159=CARTESIAN_POINT('Ctrl Pts',(17.4698002829357,15.0179828635087,0.));
#212160=CARTESIAN_POINT('Ctrl Pts',(17.4609628621419,15.0065183456923,0.));
#212161=CARTESIAN_POINT('Ctrl Pts',(17.4521868291005,14.9952063457779,0.));
#212162=CARTESIAN_POINT('Ctrl Pts',(17.4434739707773,14.9840478538357,0.));
#212163=CARTESIAN_POINT('Ctrl Pts',(17.4348261151395,14.973043879945,0.));
#212164=CARTESIAN_POINT('Ctrl Pts',(17.4262451327088,14.9621954549825,0.));
#212165=CARTESIAN_POINT('Ctrl Pts',(17.4177329382827,14.9515036315142,0.));
#212166=CARTESIAN_POINT('Ctrl Pts',(17.4092914926071,14.940969484645,0.));
#212167=CARTESIAN_POINT('Ctrl Pts',(17.400922804075,14.9305941128758,0.));
#212168=CARTESIAN_POINT('Ctrl Pts',(17.3926289303987,14.9203786389343,0.));
#212169=CARTESIAN_POINT('Ctrl Pts',(17.3844119809823,14.9103242110057,0.));
#212170=CARTESIAN_POINT('Ctrl Pts',(17.3762741193075,14.9004320039609,0.));
#212171=CARTESIAN_POINT('Ctrl Pts',(17.3682175653236,14.8907032205789,0.));
#212172=CARTESIAN_POINT('Ctrl Pts',(17.3602445978163,14.8811390927424,0.));
#212173=CARTESIAN_POINT('Ctrl Pts',(17.3523575568648,14.8717408826958,0.));
#212174=CARTESIAN_POINT('Ctrl Pts',(17.3445588463477,14.8625098843419,0.));
#212175=CARTESIAN_POINT('Ctrl Pts',(17.336850936485,14.8534474245433,0.));
#212176=CARTESIAN_POINT('Ctrl Pts',(17.3292363662601,14.8445548643505,0.));
#212177=CARTESIAN_POINT('Ctrl Pts',(17.3217177462096,14.8358336004193,0.));
#212178=CARTESIAN_POINT('Ctrl Pts',(17.3142977632656,14.8272850675375,0.));
#212179=CARTESIAN_POINT('Ctrl Pts',(17.3069791853705,14.8189107410161,0.));
#212180=CARTESIAN_POINT('Ctrl Pts',(17.2997648661483,14.8107121391038,0.));
#212181=CARTESIAN_POINT('Ctrl Pts',(17.2926577496519,14.8026908254281,0.));
#212182=CARTESIAN_POINT('Ctrl Pts',(17.28566087332,14.7948484105253,0.));
#212183=CARTESIAN_POINT('Ctrl Pts',(17.278777370485,14.787186553128,0.));
#212184=CARTESIAN_POINT('Ctrl Pts',(17.2720104735192,14.7797069617802,0.));
#212185=CARTESIAN_POINT('Ctrl Pts',(17.2653635155317,14.7724113956728,0.));
#212186=CARTESIAN_POINT('Ctrl Pts',(17.2588399401464,14.7653016697589,0.));
#212187=CARTESIAN_POINT('Ctrl Pts',(17.2524433146837,14.7583796616617,0.));
#212188=CARTESIAN_POINT('Ctrl Pts',(17.2461773413289,14.7516473175125,0.));
#212189=CARTESIAN_POINT('Ctrl Pts',(17.2400458713566,14.7451066593793,0.));
#212190=CARTESIAN_POINT('Ctrl Pts',(17.2340529062077,14.7387597858117,0.));
#212191=CARTESIAN_POINT('Ctrl Pts',(17.2282025904314,14.7326088681163,0.));
#212192=CARTESIAN_POINT('Ctrl Pts',(17.2224992099666,14.7266561494282,0.));
#212193=CARTESIAN_POINT('Ctrl Pts',(17.2169471814255,14.7209039390326,0.));
#212194=CARTESIAN_POINT('Ctrl Pts',(17.2115510835988,14.7153546289338,0.));
#212195=CARTESIAN_POINT('Ctrl Pts',(17.2063157097316,14.7100107213587,0.));
#212196=CARTESIAN_POINT('Ctrl Pts',(17.2012461084268,14.7048748502663,0.));
#212197=CARTESIAN_POINT('Ctrl Pts',(17.1963476411694,14.699949811582,0.));
#212198=CARTESIAN_POINT('Ctrl Pts',(17.1916259308415,14.6952385361706,0.));
#212199=CARTESIAN_POINT('Ctrl Pts',(17.1870867909918,14.6907440526958,0.));
#212200=CARTESIAN_POINT('Ctrl Pts',(17.182736158472,14.6864694522319,0.));
#212201=CARTESIAN_POINT('Ctrl Pts',(17.1785800350827,14.6824178576167,0.));
#212202=CARTESIAN_POINT('Ctrl Pts',(17.1746247499057,14.6785925615676,0.));
#212203=CARTESIAN_POINT('Ctrl Pts',(17.1708771619129,14.6749971333867,0.));
#212204=CARTESIAN_POINT('Ctrl Pts',(17.1673449723019,14.6716355833321,0.));
#212205=CARTESIAN_POINT('Ctrl Pts',(17.1640366762304,14.6685123374424,0.));
#212206=CARTESIAN_POINT('Ctrl Pts',(17.1609609517369,14.6656319165057,0.));
#212207=CARTESIAN_POINT('Ctrl Pts',(17.1581262646789,14.662998728599,0.));
#212208=CARTESIAN_POINT('Ctrl Pts',(17.1555401986403,14.660616716964,0.));
#212209=CARTESIAN_POINT('Ctrl Pts',(17.1532107762719,14.6584900555301,0.));
#212210=CARTESIAN_POINT('Ctrl Pts',(17.1511476869495,14.6566237952435,0.));
#212211=CARTESIAN_POINT('Ctrl Pts',(17.1493641837556,14.6550248622813,0.));
#212212=CARTESIAN_POINT('Ctrl Pts',(17.1478763944909,14.6537016966188,0.));
#212213=CARTESIAN_POINT('Ctrl Pts',(17.1466998098673,14.6526624064978,0.));
#212214=CARTESIAN_POINT('Ctrl Pts',(17.1458462295273,14.65191316345,0.));
#212215=CARTESIAN_POINT('Ctrl Pts',(17.1454262858045,14.6515481598057,0.));
#212216=CARTESIAN_POINT('Ctrl Pts',(17.1452600887039,14.6514066997188,0.));
#212217=CARTESIAN_POINT('Ctrl Pts',(17.1452153999142,14.651371185284,0.));
#212218=CARTESIAN_POINT('Ctrl Pts',(17.1452095830633,14.6513681262571,0.));
#212219=CARTESIAN_POINT('',(18.8464468996588,17.9112098770111,0.));
#212220=CARTESIAN_POINT('Ctrl Pts',(18.5896416359912,12.7689476255363,0.));
#212221=CARTESIAN_POINT('Ctrl Pts',(18.5896416359912,12.7689476255363,12.));
#212222=CARTESIAN_POINT('Ctrl Pts',(18.5896460962964,12.7689524524483,0.));
#212223=CARTESIAN_POINT('Ctrl Pts',(18.5896460962964,12.7689524524483,12.));
#212224=CARTESIAN_POINT('Ctrl Pts',(18.5896919669165,12.768986426692,0.));
#212225=CARTESIAN_POINT('Ctrl Pts',(18.5896919669165,12.768986426692,12.));
#212226=CARTESIAN_POINT('Ctrl Pts',(18.589871621843,12.769110348199,0.));
#212227=CARTESIAN_POINT('Ctrl Pts',(18.589871621843,12.769110348199,12.));
#212228=CARTESIAN_POINT('Ctrl Pts',(18.5903328777227,12.7694215127919,0.));
#212229=CARTESIAN_POINT('Ctrl Pts',(18.5903328777227,12.7694215127919,12.));
#212230=CARTESIAN_POINT('Ctrl Pts',(18.5912775137806,12.7700520897173,0.));
#212231=CARTESIAN_POINT('Ctrl Pts',(18.5912775137806,12.7700520897173,12.));
#212232=CARTESIAN_POINT('Ctrl Pts',(18.5925859134579,12.7709195951156,0.));
#212233=CARTESIAN_POINT('Ctrl Pts',(18.5925859134579,12.7709195951156,12.));
#212234=CARTESIAN_POINT('Ctrl Pts',(18.5942490615407,12.7720142287172,0.));
#212235=CARTESIAN_POINT('Ctrl Pts',(18.5942490615407,12.7720142287172,12.));
#212236=CARTESIAN_POINT('Ctrl Pts',(18.5962551167772,12.7733231262108,0.));
#212237=CARTESIAN_POINT('Ctrl Pts',(18.5962551167772,12.7733231262108,12.));
#212238=CARTESIAN_POINT('Ctrl Pts',(18.598591752595,12.7748328937638,0.));
#212239=CARTESIAN_POINT('Ctrl Pts',(18.598591752595,12.7748328937638,12.));
#212240=CARTESIAN_POINT('Ctrl Pts',(18.6012488486709,12.7765325225081,0.));
#212241=CARTESIAN_POINT('Ctrl Pts',(18.6012488486709,12.7765325225081,12.));
#212242=CARTESIAN_POINT('Ctrl Pts',(18.6042190183704,12.7784139605066,0.));
#212243=CARTESIAN_POINT('Ctrl Pts',(18.6042190183704,12.7784139605066,12.));
#212244=CARTESIAN_POINT('Ctrl Pts',(18.6074961535723,12.7804705387658,0.));
#212245=CARTESIAN_POINT('Ctrl Pts',(18.6074961535723,12.7804705387658,12.));
#212246=CARTESIAN_POINT('Ctrl Pts',(18.6110744826219,12.7826959526925,0.));
#212247=CARTESIAN_POINT('Ctrl Pts',(18.6110744826219,12.7826959526925,12.));
#212248=CARTESIAN_POINT('Ctrl Pts',(18.6149475565188,12.7850831657901,0.));
#212249=CARTESIAN_POINT('Ctrl Pts',(18.6149475565188,12.7850831657901,12.));
#212250=CARTESIAN_POINT('Ctrl Pts',(18.6191087624752,12.7876249657834,0.));
#212251=CARTESIAN_POINT('Ctrl Pts',(18.6191087624752,12.7876249657834,12.));
#212252=CARTESIAN_POINT('Ctrl Pts',(18.6235516265575,12.7903142925234,0.));
#212253=CARTESIAN_POINT('Ctrl Pts',(18.6235516265575,12.7903142925234,12.));
#212254=CARTESIAN_POINT('Ctrl Pts',(18.6282702819371,12.7931447451555,0.));
#212255=CARTESIAN_POINT('Ctrl Pts',(18.6282702819371,12.7931447451555,12.));
#212256=CARTESIAN_POINT('Ctrl Pts',(18.6332595057006,12.7961106222251,0.));
#212257=CARTESIAN_POINT('Ctrl Pts',(18.6332595057006,12.7961106222251,12.));
#212258=CARTESIAN_POINT('Ctrl Pts',(18.63851447924,12.7992066625264,0.));
#212259=CARTESIAN_POINT('Ctrl Pts',(18.63851447924,12.7992066625264,12.));
#212260=CARTESIAN_POINT('Ctrl Pts',(18.6440306327456,12.8024278770153,0.));
#212261=CARTESIAN_POINT('Ctrl Pts',(18.6440306327456,12.8024278770153,12.));
#212262=CARTESIAN_POINT('Ctrl Pts',(18.6498034438987,12.805769331162,0.));
#212263=CARTESIAN_POINT('Ctrl Pts',(18.6498034438987,12.805769331162,12.));
#212264=CARTESIAN_POINT('Ctrl Pts',(18.6558284825773,12.8092261933858,0.));
#212265=CARTESIAN_POINT('Ctrl Pts',(18.6558284825773,12.8092261933858,12.));
#212266=CARTESIAN_POINT('Ctrl Pts',(18.6621014624746,12.8127937909631,0.));
#212267=CARTESIAN_POINT('Ctrl Pts',(18.6621014624746,12.8127937909631,12.));
#212268=CARTESIAN_POINT('Ctrl Pts',(18.6686182952799,12.8164676687362,0.));
#212269=CARTESIAN_POINT('Ctrl Pts',(18.6686182952799,12.8164676687362,12.));
#212270=CARTESIAN_POINT('Ctrl Pts',(18.6753751301092,12.8202436318474,0.));
#212271=CARTESIAN_POINT('Ctrl Pts',(18.6753751301092,12.8202436318474,12.));
#212272=CARTESIAN_POINT('Ctrl Pts',(18.6823683094139,12.8241176980017,0.));
#212273=CARTESIAN_POINT('Ctrl Pts',(18.6823683094139,12.8241176980017,12.));
#212274=CARTESIAN_POINT('Ctrl Pts',(18.6895943376171,12.8280860635231,0.));
#212275=CARTESIAN_POINT('Ctrl Pts',(18.6895943376171,12.8280860635231,12.));
#212276=CARTESIAN_POINT('Ctrl Pts',(18.6970498410172,12.8321450599789,0.));
#212277=CARTESIAN_POINT('Ctrl Pts',(18.6970498410172,12.8321450599789,12.));
#212278=CARTESIAN_POINT('Ctrl Pts',(18.7047315436294,12.8362911280361,0.));
#212279=CARTESIAN_POINT('Ctrl Pts',(18.7047315436294,12.8362911280361,12.));
#212280=CARTESIAN_POINT('Ctrl Pts',(18.7126362754445,12.8405208263431,0.));
#212281=CARTESIAN_POINT('Ctrl Pts',(18.7126362754445,12.8405208263431,12.));
#212282=CARTESIAN_POINT('Ctrl Pts',(18.7207609737702,12.8448308329494,0.));
#212283=CARTESIAN_POINT('Ctrl Pts',(18.7207609737702,12.8448308329494,12.));
#212284=CARTESIAN_POINT('Ctrl Pts',(18.7291026886554,12.8492179511591,0.));
#212285=CARTESIAN_POINT('Ctrl Pts',(18.7291026886554,12.8492179511591,12.));
#212286=CARTESIAN_POINT('Ctrl Pts',(18.7376585820854,12.8536791086316,0.));
#212287=CARTESIAN_POINT('Ctrl Pts',(18.7376585820854,12.8536791086316,12.));
#212288=CARTESIAN_POINT('Ctrl Pts',(18.7464259171251,12.8582113455646,0.));
#212289=CARTESIAN_POINT('Ctrl Pts',(18.7464259171251,12.8582113455646,12.));
#212290=CARTESIAN_POINT('Ctrl Pts',(18.7554020493887,12.8628118054171,0.));
#212291=CARTESIAN_POINT('Ctrl Pts',(18.7554020493887,12.8628118054171,12.));
#212292=CARTESIAN_POINT('Ctrl Pts',(18.7645844169564,12.8674777239653,0.));
#212293=CARTESIAN_POINT('Ctrl Pts',(18.7645844169564,12.8674777239653,12.));
#212294=CARTESIAN_POINT('Ctrl Pts',(18.7739705329022,12.872206421181,0.));
#212295=CARTESIAN_POINT('Ctrl Pts',(18.7739705329022,12.872206421181,12.));
#212296=CARTESIAN_POINT('Ctrl Pts',(18.7835579840477,12.8769952998095,0.));
#212297=CARTESIAN_POINT('Ctrl Pts',(18.7835579840477,12.8769952998095,12.));
#212298=CARTESIAN_POINT('Ctrl Pts',(18.7933444285868,12.8818418427475,0.));
#212299=CARTESIAN_POINT('Ctrl Pts',(18.7933444285868,12.8818418427475,12.));
#212300=CARTESIAN_POINT('Ctrl Pts',(18.8033275941943,12.8867436109546,0.));
#212301=CARTESIAN_POINT('Ctrl Pts',(18.8033275941943,12.8867436109546,12.));
#212302=CARTESIAN_POINT('Ctrl Pts',(18.813505275782,12.8916982409935,0.));
#212303=CARTESIAN_POINT('Ctrl Pts',(18.813505275782,12.8916982409935,12.));
#212304=CARTESIAN_POINT('Ctrl Pts',(18.8238753319129,12.8967034410755,0.));
#212305=CARTESIAN_POINT('Ctrl Pts',(18.8238753319129,12.8967034410755,12.));
#212306=CARTESIAN_POINT('Ctrl Pts',(18.834435681259,12.9017569871738,0.));
#212307=CARTESIAN_POINT('Ctrl Pts',(18.834435681259,12.9017569871738,12.));
#212308=CARTESIAN_POINT('Ctrl Pts',(18.8451842990984,12.9068567191854,0.));
#212309=CARTESIAN_POINT('Ctrl Pts',(18.8451842990984,12.9068567191854,12.));
#212310=CARTESIAN_POINT('Ctrl Pts',(18.8561192136198,12.9120005369063,0.));
#212311=CARTESIAN_POINT('Ctrl Pts',(18.8561192136198,12.9120005369063,12.));
#212312=CARTESIAN_POINT('Ctrl Pts',(18.8672385038326,12.9171863977045,0.));
#212313=CARTESIAN_POINT('Ctrl Pts',(18.8672385038326,12.9171863977045,12.));
#212314=CARTESIAN_POINT('Ctrl Pts',(18.8785402977527,12.9224123144982,0.));
#212315=CARTESIAN_POINT('Ctrl Pts',(18.8785402977527,12.9224123144982,12.));
#212316=CARTESIAN_POINT('Ctrl Pts',(18.8900227704889,12.9276763536373,0.));
#212317=CARTESIAN_POINT('Ctrl Pts',(18.8900227704889,12.9276763536373,12.));
#212318=CARTESIAN_POINT('Ctrl Pts',(18.9016841423403,12.9329766328185,0.));
#212319=CARTESIAN_POINT('Ctrl Pts',(18.9016841423403,12.9329766328185,12.));
#212320=CARTESIAN_POINT('Ctrl Pts',(18.9135226769465,12.9383113190375,0.));
#212321=CARTESIAN_POINT('Ctrl Pts',(18.9135226769465,12.9383113190375,12.));
#212322=CARTESIAN_POINT('Ctrl Pts',(18.9255366795195,12.9436786266105,0.));
#212323=CARTESIAN_POINT('Ctrl Pts',(18.9255366795195,12.9436786266105,12.));
#212324=CARTESIAN_POINT('Ctrl Pts',(18.9377244950435,12.9490768151821,0.));
#212325=CARTESIAN_POINT('Ctrl Pts',(18.9377244950435,12.9490768151821,12.));
#212326=CARTESIAN_POINT('Ctrl Pts',(18.9500845064715,12.9545041877377,0.));
#212327=CARTESIAN_POINT('Ctrl Pts',(18.9500845064715,12.9545041877377,12.));
#212328=CARTESIAN_POINT('Ctrl Pts',(18.9626151329229,12.9599590886319,0.));
#212329=CARTESIAN_POINT('Ctrl Pts',(18.9626151329229,12.9599590886319,12.));
#212330=CARTESIAN_POINT('Ctrl Pts',(18.9753148284475,12.9654399021869,0.));
#212331=CARTESIAN_POINT('Ctrl Pts',(18.9753148284475,12.9654399021869,12.));
#212332=CARTESIAN_POINT('Ctrl Pts',(18.9881820807585,12.9709450512747,0.));
#212333=CARTESIAN_POINT('Ctrl Pts',(18.9881820807585,12.9709450512747,12.));
#212334=CARTESIAN_POINT('Ctrl Pts',(19.0012154099791,12.9764729959205,0.));
#212335=CARTESIAN_POINT('Ctrl Pts',(19.0012154099791,12.9764729959205,12.));
#212336=CARTESIAN_POINT('Ctrl Pts',(19.0144133673348,12.9820222318716,0.));
#212337=CARTESIAN_POINT('Ctrl Pts',(19.0144133673348,12.9820222318716,12.));
#212338=CARTESIAN_POINT('Ctrl Pts',(19.0277745339908,12.9875912893003,0.));
#212339=CARTESIAN_POINT('Ctrl Pts',(19.0277745339908,12.9875912893003,12.));
#212340=CARTESIAN_POINT('Ctrl Pts',(19.0412975200398,12.9931787316515,0.));
#212341=CARTESIAN_POINT('Ctrl Pts',(19.0412975200398,12.9931787316515,12.));
#212342=CARTESIAN_POINT('Ctrl Pts',(19.0549809634355,12.9987831544502,0.));
#212343=CARTESIAN_POINT('Ctrl Pts',(19.0549809634355,12.9987831544502,12.));
#212344=CARTESIAN_POINT('Ctrl Pts',(19.0688235289437,13.0044031841381,0.));
#212345=CARTESIAN_POINT('Ctrl Pts',(19.0688235289437,13.0044031841381,12.));
#212346=CARTESIAN_POINT('Ctrl Pts',(19.0828239070482,13.0100374768786,0.));
#212347=CARTESIAN_POINT('Ctrl Pts',(19.0828239070482,13.0100374768786,12.));
#212348=CARTESIAN_POINT('Ctrl Pts',(19.0969808131226,13.0156847176094,0.));
#212349=CARTESIAN_POINT('Ctrl Pts',(19.0969808131226,13.0156847176094,12.));
#212350=CARTESIAN_POINT('Ctrl Pts',(19.1112929866308,13.0213436191326,0.));
#212351=CARTESIAN_POINT('Ctrl Pts',(19.1112929866308,13.0213436191326,12.));
#212352=CARTESIAN_POINT('Ctrl Pts',(19.1257591903099,13.0270129211976,0.));
#212353=CARTESIAN_POINT('Ctrl Pts',(19.1257591903099,13.0270129211976,12.));
#212354=CARTESIAN_POINT('Ctrl Pts',(19.1403782093389,13.0326913895841,0.));
#212355=CARTESIAN_POINT('Ctrl Pts',(19.1403782093389,13.0326913895841,12.));
#212356=CARTESIAN_POINT('Ctrl Pts',(19.1551488505233,13.0383778152072,0.));
#212357=CARTESIAN_POINT('Ctrl Pts',(19.1551488505233,13.0383778152072,12.));
#212358=CARTESIAN_POINT('Ctrl Pts',(19.1700699416625,13.0440710133775,0.));
#212359=CARTESIAN_POINT('Ctrl Pts',(19.1700699416625,13.0440710133775,12.));
#212360=CARTESIAN_POINT('Ctrl Pts',(19.1851403308825,13.0497698230442,0.));
#212361=CARTESIAN_POINT('Ctrl Pts',(19.1851403308825,13.0497698230442,12.));
#212362=CARTESIAN_POINT('Ctrl Pts',(19.2003588859771,13.0554731060537,0.));
#212363=CARTESIAN_POINT('Ctrl Pts',(19.2003588859771,13.0554731060537,12.));
#212364=CARTESIAN_POINT('Ctrl Pts',(19.2157244937141,13.0611797463913,0.));
#212365=CARTESIAN_POINT('Ctrl Pts',(19.2157244937141,13.0611797463913,12.));
#212366=CARTESIAN_POINT('Ctrl Pts',(19.2312360592031,13.0668886494791,0.));
#212367=CARTESIAN_POINT('Ctrl Pts',(19.2312360592031,13.0668886494791,12.));
#212368=CARTESIAN_POINT('Ctrl Pts',(19.2468925053988,13.0725987415856,0.));
#212369=CARTESIAN_POINT('Ctrl Pts',(19.2468925053988,13.0725987415856,12.));
#212370=CARTESIAN_POINT('Ctrl Pts',(19.2626927725596,13.0783089692118,0.));
#212371=CARTESIAN_POINT('Ctrl Pts',(19.2626927725596,13.0783089692118,12.));
#212372=CARTESIAN_POINT('Ctrl Pts',(19.2786358177198,13.0840182984949,0.));
#212373=CARTESIAN_POINT('Ctrl Pts',(19.2786358177198,13.0840182984949,12.));
#212374=CARTESIAN_POINT('Ctrl Pts',(19.2947206141246,13.089725714597,0.));
#212375=CARTESIAN_POINT('Ctrl Pts',(19.2947206141246,13.089725714597,12.));
#212376=CARTESIAN_POINT('Ctrl Pts',(19.3109461507358,13.095430221148,0.));
#212377=CARTESIAN_POINT('Ctrl Pts',(19.3109461507358,13.095430221148,12.));
#212378=CARTESIAN_POINT('Ctrl Pts',(19.3273114318268,13.1011308397592,0.));
#212379=CARTESIAN_POINT('Ctrl Pts',(19.3273114318268,13.1011308397592,12.));
#212380=CARTESIAN_POINT('Ctrl Pts',(19.3438154765395,13.1068266095186,0.));
#212381=CARTESIAN_POINT('Ctrl Pts',(19.3438154765395,13.1068266095186,12.));
#212382=CARTESIAN_POINT('Ctrl Pts',(19.3604573184516,13.1125165865021,0.));
#212383=CARTESIAN_POINT('Ctrl Pts',(19.3604573184516,13.1125165865021,12.));
#212384=CARTESIAN_POINT('Ctrl Pts',(19.3772360051093,13.118199843271,0.));
#212385=CARTESIAN_POINT('Ctrl Pts',(19.3772360051093,13.118199843271,12.));
#212386=CARTESIAN_POINT('Ctrl Pts',(19.3941505976267,13.1238754684177,0.));
#212387=CARTESIAN_POINT('Ctrl Pts',(19.3941505976267,13.1238754684177,12.));
#212388=CARTESIAN_POINT('Ctrl Pts',(19.4112001703561,13.1295425661635,0.));
#212389=CARTESIAN_POINT('Ctrl Pts',(19.4112001703561,13.1295425661635,12.));
#212390=CARTESIAN_POINT('Ctrl Pts',(19.4283838105265,13.135200255944,0.));
#212391=CARTESIAN_POINT('Ctrl Pts',(19.4283838105265,13.135200255944,12.));
#212392=CARTESIAN_POINT('Ctrl Pts',(19.4457006178875,13.140847672006,0.));
#212393=CARTESIAN_POINT('Ctrl Pts',(19.4457006178875,13.140847672006,12.));
#212394=CARTESIAN_POINT('Ctrl Pts',(19.463149704325,13.1464839629966,0.));
#212395=CARTESIAN_POINT('Ctrl Pts',(19.463149704325,13.1464839629966,12.));
#212396=CARTESIAN_POINT('Ctrl Pts',(19.4807301935256,13.1521082915846,0.));
#212397=CARTESIAN_POINT('Ctrl Pts',(19.4807301935256,13.1521082915846,12.));
#212398=CARTESIAN_POINT('Ctrl Pts',(19.498441220707,13.1577198341238,0.));
#212399=CARTESIAN_POINT('Ctrl Pts',(19.498441220707,13.1577198341238,12.));
#212400=CARTESIAN_POINT('Ctrl Pts',(19.5162819323207,13.1633177803097,0.));
#212401=CARTESIAN_POINT('Ctrl Pts',(19.5162819323207,13.1633177803097,12.));
#212402=CARTESIAN_POINT('Ctrl Pts',(19.5342514857564,13.1689013328432,0.));
#212403=CARTESIAN_POINT('Ctrl Pts',(19.5342514857564,13.1689013328432,12.));
#212404=CARTESIAN_POINT('Ctrl Pts',(19.5523490490254,13.1744697070918,0.));
#212405=CARTESIAN_POINT('Ctrl Pts',(19.5523490490254,13.1744697070918,12.));
#212406=CARTESIAN_POINT('Ctrl Pts',(19.5705738004682,13.1800221307683,0.));
#212407=CARTESIAN_POINT('Ctrl Pts',(19.5705738004682,13.1800221307683,12.));
#212408=CARTESIAN_POINT('Ctrl Pts',(19.5889249285352,13.185557843648,0.));
#212409=CARTESIAN_POINT('Ctrl Pts',(19.5889249285352,13.185557843648,12.));
#212410=CARTESIAN_POINT('Ctrl Pts',(19.6074016315421,13.1910760972818,0.));
#212411=CARTESIAN_POINT('Ctrl Pts',(19.6074016315421,13.1910760972818,12.));
#212412=CARTESIAN_POINT('Ctrl Pts',(19.6260031174244,13.196576154715,0.));
#212413=CARTESIAN_POINT('Ctrl Pts',(19.6260031174244,13.196576154715,12.));
#212414=CARTESIAN_POINT('Ctrl Pts',(19.6447286034764,13.202057290206,0.));
#212415=CARTESIAN_POINT('Ctrl Pts',(19.6447286034764,13.202057290206,12.));
#212416=CARTESIAN_POINT('Ctrl Pts',(19.6635773160924,13.2075187889522,0.));
#212417=CARTESIAN_POINT('Ctrl Pts',(19.6635773160924,13.2075187889522,12.));
#212418=CARTESIAN_POINT('Ctrl Pts',(19.6825484905812,13.2129599468478,0.));
#212419=CARTESIAN_POINT('Ctrl Pts',(19.6825484905812,13.2129599468478,12.));
#212420=CARTESIAN_POINT('Ctrl Pts',(19.7016413709678,13.2183800702431,0.));
#212421=CARTESIAN_POINT('Ctrl Pts',(19.7016413709678,13.2183800702431,12.));
#212422=CARTESIAN_POINT('Ctrl Pts',(19.7208552097867,13.2237784757065,0.));
#212423=CARTESIAN_POINT('Ctrl Pts',(19.7208552097867,13.2237784757065,12.));
#212424=CARTESIAN_POINT('Ctrl Pts',(19.7401892678701,13.2291544897902,0.));
#212425=CARTESIAN_POINT('Ctrl Pts',(19.7401892678701,13.2291544897902,12.));
#212426=CARTESIAN_POINT('Ctrl Pts',(19.7596428141176,13.2345074487968,0.));
#212427=CARTESIAN_POINT('Ctrl Pts',(19.7596428141176,13.2345074487968,12.));
#212428=CARTESIAN_POINT('Ctrl Pts',(19.7792151253297,13.239836698568,0.));
#212429=CARTESIAN_POINT('Ctrl Pts',(19.7792151253297,13.239836698568,12.));
#212430=CARTESIAN_POINT('Ctrl Pts',(19.7989054860501,13.2451415942809,0.));
#212431=CARTESIAN_POINT('Ctrl Pts',(19.7989054860501,13.2451415942809,12.));
#212432=CARTESIAN_POINT('Ctrl Pts',(19.8187131883919,13.2504215002458,0.));
#212433=CARTESIAN_POINT('Ctrl Pts',(19.8187131883919,13.2504215002458,12.));
#212434=CARTESIAN_POINT('Ctrl Pts',(19.8386375318632,13.2556757897085,0.));
#212435=CARTESIAN_POINT('Ctrl Pts',(19.8386375318632,13.2556757897085,12.));
#212436=CARTESIAN_POINT('Ctrl Pts',(19.8586778231711,13.2609038446525,0.));
#212437=CARTESIAN_POINT('Ctrl Pts',(19.8586778231711,13.2609038446525,12.));
#212438=CARTESIAN_POINT('Ctrl Pts',(19.8788333760571,13.2661050556128,0.));
#212439=CARTESIAN_POINT('Ctrl Pts',(19.8788333760571,13.2661050556128,12.));
#212440=CARTESIAN_POINT('Ctrl Pts',(19.8991035111739,13.2712788215015,0.));
#212441=CARTESIAN_POINT('Ctrl Pts',(19.8991035111739,13.2712788215015,12.));
#212442=CARTESIAN_POINT('Ctrl Pts',(19.9194875559419,13.2764245494354,0.));
#212443=CARTESIAN_POINT('Ctrl Pts',(19.9194875559419,13.2764245494354,12.));
#212444=CARTESIAN_POINT('Ctrl Pts',(19.9399848444019,13.2815416545663,0.));
#212445=CARTESIAN_POINT('Ctrl Pts',(19.9399848444019,13.2815416545663,12.));
#212446=CARTESIAN_POINT('Ctrl Pts',(19.9605947170589,13.2866295599152,0.));
#212447=CARTESIAN_POINT('Ctrl Pts',(19.9605947170589,13.2866295599152,12.));
#212448=CARTESIAN_POINT('Ctrl Pts',(19.9813165207174,13.2916876962098,0.));
#212449=CARTESIAN_POINT('Ctrl Pts',(19.9813165207174,13.2916876962098,12.));
#212450=CARTESIAN_POINT('Ctrl Pts',(20.0021496083742,13.296715501731,0.));
#212451=CARTESIAN_POINT('Ctrl Pts',(20.0021496083742,13.296715501731,12.));
#212452=CARTESIAN_POINT('Ctrl Pts',(20.0230933391039,13.3017124221639,0.));
#212453=CARTESIAN_POINT('Ctrl Pts',(20.0230933391039,13.3017124221639,12.));
#212454=CARTESIAN_POINT('Ctrl Pts',(20.0441470779345,13.3066779104515,0.));
#212455=CARTESIAN_POINT('Ctrl Pts',(20.0441470779345,13.3066779104515,12.));
#212456=CARTESIAN_POINT('Ctrl Pts',(20.0653101957188,13.3116114266514,0.));
#212457=CARTESIAN_POINT('Ctrl Pts',(20.0653101957188,13.3116114266514,12.));
#212458=CARTESIAN_POINT('Ctrl Pts',(20.0865820689883,13.3165124377963,0.));
#212459=CARTESIAN_POINT('Ctrl Pts',(20.0865820689883,13.3165124377963,12.));
#212460=CARTESIAN_POINT('Ctrl Pts',(20.1079620798377,13.3213804177588,0.));
#212461=CARTESIAN_POINT('Ctrl Pts',(20.1079620798377,13.3213804177588,12.));
#212462=CARTESIAN_POINT('Ctrl Pts',(20.1294496158405,13.3262148471228,0.));
#212463=CARTESIAN_POINT('Ctrl Pts',(20.1294496158405,13.3262148471228,12.));
#212464=CARTESIAN_POINT('Ctrl Pts',(20.1510440699477,13.3310152130565,0.));
#212465=CARTESIAN_POINT('Ctrl Pts',(20.1510440699477,13.3310152130565,12.));
#212466=CARTESIAN_POINT('Ctrl Pts',(20.1727448403818,13.3357810091903,0.));
#212467=CARTESIAN_POINT('Ctrl Pts',(20.1727448403818,13.3357810091903,12.));
#212468=CARTESIAN_POINT('Ctrl Pts',(20.1945513305233,13.3405117354969,0.));
#212469=CARTESIAN_POINT('Ctrl Pts',(20.1945513305233,13.3405117354969,12.));
#212470=CARTESIAN_POINT('Ctrl Pts',(20.2164629487855,13.3452068981763,0.));
#212471=CARTESIAN_POINT('Ctrl Pts',(20.2164629487855,13.3452068981763,12.));
#212472=CARTESIAN_POINT('Ctrl Pts',(20.2384791085354,13.3498660095382,0.));
#212473=CARTESIAN_POINT('Ctrl Pts',(20.2384791085354,13.3498660095382,12.));
#212474=CARTESIAN_POINT('Ctrl Pts',(20.2605992280117,13.3544885878886,0.));
#212475=CARTESIAN_POINT('Ctrl Pts',(20.2605992280117,13.3544885878886,12.));
#212476=CARTESIAN_POINT('Ctrl Pts',(20.2828227302337,13.3590741574194,0.));
#212477=CARTESIAN_POINT('Ctrl Pts',(20.2828227302337,13.3590741574194,12.));
#212478=CARTESIAN_POINT('Ctrl Pts',(20.3051490429049,13.3636222481017,0.));
#212479=CARTESIAN_POINT('Ctrl Pts',(20.3051490429049,13.3636222481017,12.));
#212480=CARTESIAN_POINT('Ctrl Pts',(20.3275775983032,13.3681323955828,0.));
#212481=CARTESIAN_POINT('Ctrl Pts',(20.3275775983032,13.3681323955828,12.));
#212482=CARTESIAN_POINT('Ctrl Pts',(20.3501078331818,13.372604141087,0.));
#212483=CARTESIAN_POINT('Ctrl Pts',(20.3501078331818,13.372604141087,12.));
#212484=CARTESIAN_POINT('Ctrl Pts',(20.3727391887187,13.377037031319,0.));
#212485=CARTESIAN_POINT('Ctrl Pts',(20.3727391887187,13.377037031319,12.));
#212486=CARTESIAN_POINT('Ctrl Pts',(20.3954711104504,13.3814306183721,0.));
#212487=CARTESIAN_POINT('Ctrl Pts',(20.3954711104504,13.3814306183721,12.));
#212488=CARTESIAN_POINT('Ctrl Pts',(20.4183030482002,13.3857844596387,0.));
#212489=CARTESIAN_POINT('Ctrl Pts',(20.4183030482002,13.3857844596387,12.));
#212490=CARTESIAN_POINT('Ctrl Pts',(20.4412344560007,13.3900981177254,0.));
#212491=CARTESIAN_POINT('Ctrl Pts',(20.4412344560007,13.3900981177254,12.));
#212492=CARTESIAN_POINT('Ctrl Pts',(20.4642647920038,13.3943711603739,0.));
#212493=CARTESIAN_POINT('Ctrl Pts',(20.4642647920038,13.3943711603739,12.));
#212494=CARTESIAN_POINT('Ctrl Pts',(20.4873935184041,13.3986031603716,0.));
#212495=CARTESIAN_POINT('Ctrl Pts',(20.4873935184041,13.3986031603716,12.));
#212496=CARTESIAN_POINT('Ctrl Pts',(20.5106201013755,13.4027936954529,0.));
#212497=CARTESIAN_POINT('Ctrl Pts',(20.5106201013755,13.4027936954529,12.));
#212498=CARTESIAN_POINT('Ctrl Pts',(20.5339440109957,13.4069423482077,0.));
#212499=CARTESIAN_POINT('Ctrl Pts',(20.5339440109957,13.4069423482077,12.));
#212500=CARTESIAN_POINT('Ctrl Pts',(20.557364721164,13.4110487059912,0.));
#212501=CARTESIAN_POINT('Ctrl Pts',(20.557364721164,13.4110487059912,12.));
#212502=CARTESIAN_POINT('Ctrl Pts',(20.5808817095155,13.4151123608411,0.));
#212503=CARTESIAN_POINT('Ctrl Pts',(20.5808817095155,13.4151123608411,12.));
#212504=CARTESIAN_POINT('Ctrl Pts',(20.6044944573151,13.4191329093932,0.));
#212505=CARTESIAN_POINT('Ctrl Pts',(20.6044944573151,13.4191329093932,12.));
#212506=CARTESIAN_POINT('Ctrl Pts',(20.6282024494234,13.4231099528178,0.));
#212507=CARTESIAN_POINT('Ctrl Pts',(20.6282024494234,13.4231099528178,12.));
#212508=CARTESIAN_POINT('Ctrl Pts',(20.6520051742867,13.4270430967651,0.));
#212509=CARTESIAN_POINT('Ctrl Pts',(20.6520051742867,13.4270430967651,12.));
#212510=CARTESIAN_POINT('Ctrl Pts',(20.6759021239102,13.4309319513119,0.));
#212511=CARTESIAN_POINT('Ctrl Pts',(20.6759021239102,13.4309319513119,12.));
#212512=CARTESIAN_POINT('Ctrl Pts',(20.6998927938288,13.4347761309154,0.));
#212513=CARTESIAN_POINT('Ctrl Pts',(20.6998927938288,13.4347761309154,12.));
#212514=CARTESIAN_POINT('Ctrl Pts',(20.7239766830675,13.4385752543663,0.));
#212515=CARTESIAN_POINT('Ctrl Pts',(20.7239766830675,13.4385752543663,12.));
#212516=CARTESIAN_POINT('Ctrl Pts',(20.7481532941014,13.4423289447561,0.));
#212517=CARTESIAN_POINT('Ctrl Pts',(20.7481532941014,13.4423289447561,12.));
#212518=CARTESIAN_POINT('Ctrl Pts',(20.7724221327609,13.4460368293689,0.));
#212519=CARTESIAN_POINT('Ctrl Pts',(20.7724221327609,13.4460368293689,12.));
#212520=CARTESIAN_POINT('Ctrl Pts',(20.7967827081228,13.4496985395637,0.));
#212521=CARTESIAN_POINT('Ctrl Pts',(20.7967827081228,13.4496985395637,12.));
#212522=CARTESIAN_POINT('Ctrl Pts',(20.821234532398,13.4533137106667,0.));
#212523=CARTESIAN_POINT('Ctrl Pts',(20.821234532398,13.4533137106667,12.));
#212524=CARTESIAN_POINT('Ctrl Pts',(20.8457771208083,13.4568819818631,0.));
#212525=CARTESIAN_POINT('Ctrl Pts',(20.8457771208083,13.4568819818631,12.));
#212526=CARTESIAN_POINT('Ctrl Pts',(20.8704099914641,13.4604029960983,0.));
#212527=CARTESIAN_POINT('Ctrl Pts',(20.8704099914641,13.4604029960983,12.));
#212528=CARTESIAN_POINT('Ctrl Pts',(20.8951326652158,13.4638763999725,0.));
#212529=CARTESIAN_POINT('Ctrl Pts',(20.8951326652158,13.4638763999725,12.));
#212530=CARTESIAN_POINT('Ctrl Pts',(20.9199446657583,13.4673018437717,0.));
#212531=CARTESIAN_POINT('Ctrl Pts',(20.9199446657583,13.4673018437717,12.));
#212532=CARTESIAN_POINT('Ctrl Pts',(20.9448455197557,13.4706789815166,0.));
#212533=CARTESIAN_POINT('Ctrl Pts',(20.9448455197557,13.4706789815166,12.));
#212534=CARTESIAN_POINT('Ctrl Pts',(20.9698347569477,13.4740074710086,0.));
#212535=CARTESIAN_POINT('Ctrl Pts',(20.9698347569477,13.4740074710086,12.));
#212536=CARTESIAN_POINT('Ctrl Pts',(20.9949119102592,13.4772869738879,0.));
#212537=CARTESIAN_POINT('Ctrl Pts',(20.9949119102592,13.4772869738879,12.));
#212538=CARTESIAN_POINT('Ctrl Pts',(21.0200765158884,13.4805171556822,0.));
#212539=CARTESIAN_POINT('Ctrl Pts',(21.0200765158884,13.4805171556822,12.));
#212540=CARTESIAN_POINT('Ctrl Pts',(21.0453281134245,13.4836976858912,0.));
#212541=CARTESIAN_POINT('Ctrl Pts',(21.0453281134245,13.4836976858912,12.));
#212542=CARTESIAN_POINT('Ctrl Pts',(21.0706662455199,13.4868282377191,0.));
#212543=CARTESIAN_POINT('Ctrl Pts',(21.0706662455199,13.4868282377191,12.));
#212544=CARTESIAN_POINT('Ctrl Pts',(21.0960904575046,13.4899084877717,0.));
#212545=CARTESIAN_POINT('Ctrl Pts',(21.0960904575046,13.4899084877717,12.));
#212546=CARTESIAN_POINT('Ctrl Pts',(21.1216002970207,13.4929381157778,0.));
#212547=CARTESIAN_POINT('Ctrl Pts',(21.1216002970207,13.4929381157778,12.));
#212548=CARTESIAN_POINT('Ctrl Pts',(21.1471953136209,13.4959168042934,0.));
#212549=CARTESIAN_POINT('Ctrl Pts',(21.1471953136209,13.4959168042934,12.));
#212550=CARTESIAN_POINT('Ctrl Pts',(21.1728750584175,13.4988442384491,0.));
#212551=CARTESIAN_POINT('Ctrl Pts',(21.1728750584175,13.4988442384491,12.));
#212552=CARTESIAN_POINT('Ctrl Pts',(21.1986390835828,13.5017201056088,0.));
#212553=CARTESIAN_POINT('Ctrl Pts',(21.1986390835828,13.5017201056088,12.));
#212554=CARTESIAN_POINT('Ctrl Pts',(21.2244869429332,13.5045440957404,0.));
#212555=CARTESIAN_POINT('Ctrl Pts',(21.2244869429332,13.5045440957404,12.));
#212556=CARTESIAN_POINT('Ctrl Pts',(21.250418192743,13.5073159019452,0.));
#212557=CARTESIAN_POINT('Ctrl Pts',(21.250418192743,13.5073159019452,12.));
#212558=CARTESIAN_POINT('Ctrl Pts',(21.2764323924442,13.5100352209205,0.));
#212559=CARTESIAN_POINT('Ctrl Pts',(21.2764323924442,13.5100352209205,12.));
#212560=CARTESIAN_POINT('Ctrl Pts',(21.3025291054235,13.5127017534971,0.));
#212561=CARTESIAN_POINT('Ctrl Pts',(21.3025291054235,13.5127017534971,12.));
#212562=CARTESIAN_POINT('Ctrl Pts',(21.3287078996341,13.5153152050555,0.));
#212563=CARTESIAN_POINT('Ctrl Pts',(21.3287078996341,13.5153152050555,12.));
#212564=CARTESIAN_POINT('Ctrl Pts',(21.3549683486222,13.5178752862466,0.));
#212565=CARTESIAN_POINT('Ctrl Pts',(21.3549683486222,13.5178752862466,12.));
#212566=CARTESIAN_POINT('Ctrl Pts',(21.3813100304973,13.5203817122504,0.));
#212567=CARTESIAN_POINT('Ctrl Pts',(21.3813100304973,13.5203817122504,12.));
#212568=CARTESIAN_POINT('Ctrl Pts',(21.4077325259324,13.5228342013516,0.));
#212569=CARTESIAN_POINT('Ctrl Pts',(21.4077325259324,13.5228342013516,12.));
#212570=CARTESIAN_POINT('Ctrl Pts',(21.4342354165259,13.5252324737802,0.));
#212571=CARTESIAN_POINT('Ctrl Pts',(21.4342354165259,13.5252324737802,12.));
#212572=CARTESIAN_POINT('Ctrl Pts',(21.4608182828697,13.5275762503555,0.));
#212573=CARTESIAN_POINT('Ctrl Pts',(21.4608182828697,13.5275762503555,12.));
#212574=CARTESIAN_POINT('Ctrl Pts',(21.4874807030468,13.5298652514355,0.));
#212575=CARTESIAN_POINT('Ctrl Pts',(21.4874807030468,13.5298652514355,12.));
#212576=CARTESIAN_POINT('Ctrl Pts',(21.5142222501666,13.5320991952138,0.));
#212577=CARTESIAN_POINT('Ctrl Pts',(21.5142222501666,13.5320991952138,12.));
#212578=CARTESIAN_POINT('Ctrl Pts',(21.5410424932503,13.5342777983215,0.));
#212579=CARTESIAN_POINT('Ctrl Pts',(21.5410424932503,13.5342777983215,12.));
#212580=CARTESIAN_POINT('Ctrl Pts',(21.5679410019001,13.536400779028,0.));
#212581=CARTESIAN_POINT('Ctrl Pts',(21.5679410019001,13.536400779028,12.));
#212582=CARTESIAN_POINT('Ctrl Pts',(21.5949173499013,13.5384678597195,0.));
#212583=CARTESIAN_POINT('Ctrl Pts',(21.5949173499013,13.5384678597195,12.));
#212584=CARTESIAN_POINT('Ctrl Pts',(21.6219711193946,13.5404787697792,0.));
#212585=CARTESIAN_POINT('Ctrl Pts',(21.6219711193946,13.5404787697792,12.));
#212586=CARTESIAN_POINT('Ctrl Pts',(21.6491019044648,13.5424332480699,0.));
#212587=CARTESIAN_POINT('Ctrl Pts',(21.6491019044648,13.5424332480699,12.));
#212588=CARTESIAN_POINT('Ctrl Pts',(21.6763093157699,13.5443310461526,0.));
#212589=CARTESIAN_POINT('Ctrl Pts',(21.6763093157699,13.5443310461526,12.));
#212590=CARTESIAN_POINT('Ctrl Pts',(21.7035929822955,13.5461719295048,0.));
#212591=CARTESIAN_POINT('Ctrl Pts',(21.7035929822955,13.5461719295048,12.));
#212592=CARTESIAN_POINT('Ctrl Pts',(21.7309525412281,13.5479556704481,0.));
#212593=CARTESIAN_POINT('Ctrl Pts',(21.7309525412281,13.5479556704481,12.));
#212594=CARTESIAN_POINT('Ctrl Pts',(21.7583876294554,13.5496820422211,0.));
#212595=CARTESIAN_POINT('Ctrl Pts',(21.7583876294554,13.5496820422211,12.));
#212596=CARTESIAN_POINT('Ctrl Pts',(21.7858978745865,13.551350812725,0.));
#212597=CARTESIAN_POINT('Ctrl Pts',(21.7858978745865,13.551350812725,12.));
#212598=CARTESIAN_POINT('Ctrl Pts',(21.8134828857967,13.5529617381573,0.));
#212599=CARTESIAN_POINT('Ctrl Pts',(21.8134828857967,13.5529617381573,12.));
#212600=CARTESIAN_POINT('Ctrl Pts',(21.8411422456075,13.5545145573031,0.));
#212601=CARTESIAN_POINT('Ctrl Pts',(21.8411422456075,13.5545145573031,12.));
#212602=CARTESIAN_POINT('Ctrl Pts',(21.8688754989365,13.5560089839385,0.));
#212603=CARTESIAN_POINT('Ctrl Pts',(21.8688754989365,13.5560089839385,12.));
#212604=CARTESIAN_POINT('Ctrl Pts',(21.8966821688824,13.5574447178425,0.));
#212605=CARTESIAN_POINT('Ctrl Pts',(21.8966821688824,13.5574447178425,12.));
#212606=CARTESIAN_POINT('Ctrl Pts',(21.9245617765769,13.5588214586604,0.));
#212607=CARTESIAN_POINT('Ctrl Pts',(21.9245617765769,13.5588214586604,12.));
#212608=CARTESIAN_POINT('Ctrl Pts',(21.9525138592813,13.5601389185257,0.));
#212609=CARTESIAN_POINT('Ctrl Pts',(21.9525138592813,13.5601389185257,12.));
#212610=CARTESIAN_POINT('Ctrl Pts',(21.9805379899168,13.5613968357561,0.));
#212611=CARTESIAN_POINT('Ctrl Pts',(21.9805379899168,13.5613968357561,12.));
#212612=CARTESIAN_POINT('Ctrl Pts',(22.0086337943449,13.5625949868333,0.));
#212613=CARTESIAN_POINT('Ctrl Pts',(22.0086337943449,13.5625949868333,12.));
#212614=CARTESIAN_POINT('Ctrl Pts',(22.0368009736295,13.5637332022473,0.));
#212615=CARTESIAN_POINT('Ctrl Pts',(22.0368009736295,13.5637332022473,12.));
#212616=CARTESIAN_POINT('Ctrl Pts',(22.0650393089609,13.5648113689033,0.));
#212617=CARTESIAN_POINT('Ctrl Pts',(22.0650393089609,13.5648113689033,12.));
#212618=CARTESIAN_POINT('Ctrl Pts',(22.0933486464593,13.5658294169284,0.));
#212619=CARTESIAN_POINT('Ctrl Pts',(22.0933486464593,13.5658294169284,12.));
#212620=CARTESIAN_POINT('Ctrl Pts',(22.1217288871975,13.5667873105359,0.));
#212621=CARTESIAN_POINT('Ctrl Pts',(22.1217288871975,13.5667873105359,12.));
#212622=CARTESIAN_POINT('Ctrl Pts',(22.1444897575194,13.5675054919061,0.));
#212623=CARTESIAN_POINT('Ctrl Pts',(22.1444897575194,13.5675054919061,12.));
#212624=CARTESIAN_POINT('Ctrl Pts',(22.1615922805008,13.5680170531805,0.));
#212625=CARTESIAN_POINT('Ctrl Pts',(22.1615922805008,13.5680170531805,12.));
#212626=CARTESIAN_POINT('Ctrl Pts',(22.1730081264608,13.5683460612942,0.));
#212627=CARTESIAN_POINT('Ctrl Pts',(22.1730081264608,13.5683460612942,12.));
#212628=CARTESIAN_POINT('Ctrl Pts',(22.1787195904339,13.5685075571671,0.));
#212629=CARTESIAN_POINT('Ctrl Pts',(22.1787195904339,13.5685075571671,12.));
#212630=CARTESIAN_POINT('',(22.1787195904339,13.5685075571671,0.));
#212631=CARTESIAN_POINT('Ctrl Pts',(18.5896416359912,12.7689476255363,0.));
#212632=CARTESIAN_POINT('Ctrl Pts',(18.5896460962964,12.7689524524483,0.));
#212633=CARTESIAN_POINT('Ctrl Pts',(18.5896919669165,12.768986426692,0.));
#212634=CARTESIAN_POINT('Ctrl Pts',(18.589871621843,12.769110348199,0.));
#212635=CARTESIAN_POINT('Ctrl Pts',(18.5903328777227,12.7694215127919,0.));
#212636=CARTESIAN_POINT('Ctrl Pts',(18.5912775137806,12.7700520897173,0.));
#212637=CARTESIAN_POINT('Ctrl Pts',(18.5925859134579,12.7709195951156,0.));
#212638=CARTESIAN_POINT('Ctrl Pts',(18.5942490615407,12.7720142287172,0.));
#212639=CARTESIAN_POINT('Ctrl Pts',(18.5962551167772,12.7733231262108,0.));
#212640=CARTESIAN_POINT('Ctrl Pts',(18.598591752595,12.7748328937638,0.));
#212641=CARTESIAN_POINT('Ctrl Pts',(18.6012488486709,12.7765325225081,0.));
#212642=CARTESIAN_POINT('Ctrl Pts',(18.6042190183704,12.7784139605066,0.));
#212643=CARTESIAN_POINT('Ctrl Pts',(18.6074961535723,12.7804705387658,0.));
#212644=CARTESIAN_POINT('Ctrl Pts',(18.6110744826219,12.7826959526925,0.));
#212645=CARTESIAN_POINT('Ctrl Pts',(18.6149475565188,12.7850831657901,0.));
#212646=CARTESIAN_POINT('Ctrl Pts',(18.6191087624752,12.7876249657834,0.));
#212647=CARTESIAN_POINT('Ctrl Pts',(18.6235516265575,12.7903142925234,0.));
#212648=CARTESIAN_POINT('Ctrl Pts',(18.6282702819371,12.7931447451555,0.));
#212649=CARTESIAN_POINT('Ctrl Pts',(18.6332595057006,12.7961106222251,0.));
#212650=CARTESIAN_POINT('Ctrl Pts',(18.63851447924,12.7992066625264,0.));
#212651=CARTESIAN_POINT('Ctrl Pts',(18.6440306327456,12.8024278770153,0.));
#212652=CARTESIAN_POINT('Ctrl Pts',(18.6498034438987,12.805769331162,0.));
#212653=CARTESIAN_POINT('Ctrl Pts',(18.6558284825773,12.8092261933858,0.));
#212654=CARTESIAN_POINT('Ctrl Pts',(18.6621014624746,12.8127937909631,0.));
#212655=CARTESIAN_POINT('Ctrl Pts',(18.6686182952799,12.8164676687362,0.));
#212656=CARTESIAN_POINT('Ctrl Pts',(18.6753751301092,12.8202436318474,0.));
#212657=CARTESIAN_POINT('Ctrl Pts',(18.6823683094139,12.8241176980017,0.));
#212658=CARTESIAN_POINT('Ctrl Pts',(18.6895943376171,12.8280860635231,0.));
#212659=CARTESIAN_POINT('Ctrl Pts',(18.6970498410172,12.8321450599789,0.));
#212660=CARTESIAN_POINT('Ctrl Pts',(18.7047315436294,12.8362911280361,0.));
#212661=CARTESIAN_POINT('Ctrl Pts',(18.7126362754445,12.8405208263431,0.));
#212662=CARTESIAN_POINT('Ctrl Pts',(18.7207609737702,12.8448308329494,0.));
#212663=CARTESIAN_POINT('Ctrl Pts',(18.7291026886554,12.8492179511591,0.));
#212664=CARTESIAN_POINT('Ctrl Pts',(18.7376585820854,12.8536791086316,0.));
#212665=CARTESIAN_POINT('Ctrl Pts',(18.7464259171251,12.8582113455646,0.));
#212666=CARTESIAN_POINT('Ctrl Pts',(18.7554020493887,12.8628118054171,0.));
#212667=CARTESIAN_POINT('Ctrl Pts',(18.7645844169564,12.8674777239653,0.));
#212668=CARTESIAN_POINT('Ctrl Pts',(18.7739705329022,12.872206421181,0.));
#212669=CARTESIAN_POINT('Ctrl Pts',(18.7835579840477,12.8769952998095,0.));
#212670=CARTESIAN_POINT('Ctrl Pts',(18.7933444285868,12.8818418427475,0.));
#212671=CARTESIAN_POINT('Ctrl Pts',(18.8033275941943,12.8867436109546,0.));
#212672=CARTESIAN_POINT('Ctrl Pts',(18.813505275782,12.8916982409935,0.));
#212673=CARTESIAN_POINT('Ctrl Pts',(18.8238753319129,12.8967034410755,0.));
#212674=CARTESIAN_POINT('Ctrl Pts',(18.834435681259,12.9017569871738,0.));
#212675=CARTESIAN_POINT('Ctrl Pts',(18.8451842990984,12.9068567191854,0.));
#212676=CARTESIAN_POINT('Ctrl Pts',(18.8561192136198,12.9120005369063,0.));
#212677=CARTESIAN_POINT('Ctrl Pts',(18.8672385038326,12.9171863977045,0.));
#212678=CARTESIAN_POINT('Ctrl Pts',(18.8785402977527,12.9224123144982,0.));
#212679=CARTESIAN_POINT('Ctrl Pts',(18.8900227704889,12.9276763536373,0.));
#212680=CARTESIAN_POINT('Ctrl Pts',(18.9016841423403,12.9329766328185,0.));
#212681=CARTESIAN_POINT('Ctrl Pts',(18.9135226769465,12.9383113190375,0.));
#212682=CARTESIAN_POINT('Ctrl Pts',(18.9255366795195,12.9436786266105,0.));
#212683=CARTESIAN_POINT('Ctrl Pts',(18.9377244950435,12.9490768151821,0.));
#212684=CARTESIAN_POINT('Ctrl Pts',(18.9500845064715,12.9545041877377,0.));
#212685=CARTESIAN_POINT('Ctrl Pts',(18.9626151329229,12.9599590886319,0.));
#212686=CARTESIAN_POINT('Ctrl Pts',(18.9753148284475,12.9654399021869,0.));
#212687=CARTESIAN_POINT('Ctrl Pts',(18.9881820807585,12.9709450512747,0.));
#212688=CARTESIAN_POINT('Ctrl Pts',(19.0012154099791,12.9764729959205,0.));
#212689=CARTESIAN_POINT('Ctrl Pts',(19.0144133673348,12.9820222318716,0.));
#212690=CARTESIAN_POINT('Ctrl Pts',(19.0277745339908,12.9875912893003,0.));
#212691=CARTESIAN_POINT('Ctrl Pts',(19.0412975200398,12.9931787316515,0.));
#212692=CARTESIAN_POINT('Ctrl Pts',(19.0549809634355,12.9987831544502,0.));
#212693=CARTESIAN_POINT('Ctrl Pts',(19.0688235289437,13.0044031841381,0.));
#212694=CARTESIAN_POINT('Ctrl Pts',(19.0828239070482,13.0100374768786,0.));
#212695=CARTESIAN_POINT('Ctrl Pts',(19.0969808131226,13.0156847176094,0.));
#212696=CARTESIAN_POINT('Ctrl Pts',(19.1112929866308,13.0213436191326,0.));
#212697=CARTESIAN_POINT('Ctrl Pts',(19.1257591903099,13.0270129211976,0.));
#212698=CARTESIAN_POINT('Ctrl Pts',(19.1403782093389,13.0326913895841,0.));
#212699=CARTESIAN_POINT('Ctrl Pts',(19.1551488505233,13.0383778152072,0.));
#212700=CARTESIAN_POINT('Ctrl Pts',(19.1700699416625,13.0440710133775,0.));
#212701=CARTESIAN_POINT('Ctrl Pts',(19.1851403308825,13.0497698230442,0.));
#212702=CARTESIAN_POINT('Ctrl Pts',(19.2003588859771,13.0554731060537,0.));
#212703=CARTESIAN_POINT('Ctrl Pts',(19.2157244937141,13.0611797463913,0.));
#212704=CARTESIAN_POINT('Ctrl Pts',(19.2312360592031,13.0668886494791,0.));
#212705=CARTESIAN_POINT('Ctrl Pts',(19.2468925053988,13.0725987415856,0.));
#212706=CARTESIAN_POINT('Ctrl Pts',(19.2626927725596,13.0783089692118,0.));
#212707=CARTESIAN_POINT('Ctrl Pts',(19.2786358177198,13.0840182984949,0.));
#212708=CARTESIAN_POINT('Ctrl Pts',(19.2947206141246,13.089725714597,0.));
#212709=CARTESIAN_POINT('Ctrl Pts',(19.3109461507358,13.095430221148,0.));
#212710=CARTESIAN_POINT('Ctrl Pts',(19.3273114318268,13.1011308397592,0.));
#212711=CARTESIAN_POINT('Ctrl Pts',(19.3438154765395,13.1068266095186,0.));
#212712=CARTESIAN_POINT('Ctrl Pts',(19.3604573184516,13.1125165865021,0.));
#212713=CARTESIAN_POINT('Ctrl Pts',(19.3772360051093,13.118199843271,0.));
#212714=CARTESIAN_POINT('Ctrl Pts',(19.3941505976267,13.1238754684177,0.));
#212715=CARTESIAN_POINT('Ctrl Pts',(19.4112001703561,13.1295425661635,0.));
#212716=CARTESIAN_POINT('Ctrl Pts',(19.4283838105265,13.135200255944,0.));
#212717=CARTESIAN_POINT('Ctrl Pts',(19.4457006178875,13.140847672006,0.));
#212718=CARTESIAN_POINT('Ctrl Pts',(19.463149704325,13.1464839629966,0.));
#212719=CARTESIAN_POINT('Ctrl Pts',(19.4807301935256,13.1521082915846,0.));
#212720=CARTESIAN_POINT('Ctrl Pts',(19.498441220707,13.1577198341238,0.));
#212721=CARTESIAN_POINT('Ctrl Pts',(19.5162819323207,13.1633177803097,0.));
#212722=CARTESIAN_POINT('Ctrl Pts',(19.5342514857564,13.1689013328432,0.));
#212723=CARTESIAN_POINT('Ctrl Pts',(19.5523490490254,13.1744697070918,0.));
#212724=CARTESIAN_POINT('Ctrl Pts',(19.5705738004682,13.1800221307683,0.));
#212725=CARTESIAN_POINT('Ctrl Pts',(19.5889249285352,13.185557843648,0.));
#212726=CARTESIAN_POINT('Ctrl Pts',(19.6074016315421,13.1910760972818,0.));
#212727=CARTESIAN_POINT('Ctrl Pts',(19.6260031174244,13.196576154715,0.));
#212728=CARTESIAN_POINT('Ctrl Pts',(19.6447286034764,13.202057290206,0.));
#212729=CARTESIAN_POINT('Ctrl Pts',(19.6635773160924,13.2075187889522,0.));
#212730=CARTESIAN_POINT('Ctrl Pts',(19.6825484905812,13.2129599468478,0.));
#212731=CARTESIAN_POINT('Ctrl Pts',(19.7016413709678,13.2183800702431,0.));
#212732=CARTESIAN_POINT('Ctrl Pts',(19.7208552097867,13.2237784757065,0.));
#212733=CARTESIAN_POINT('Ctrl Pts',(19.7401892678701,13.2291544897902,0.));
#212734=CARTESIAN_POINT('Ctrl Pts',(19.7596428141176,13.2345074487968,0.));
#212735=CARTESIAN_POINT('Ctrl Pts',(19.7792151253297,13.239836698568,0.));
#212736=CARTESIAN_POINT('Ctrl Pts',(19.7989054860501,13.2451415942809,0.));
#212737=CARTESIAN_POINT('Ctrl Pts',(19.8187131883919,13.2504215002458,0.));
#212738=CARTESIAN_POINT('Ctrl Pts',(19.8386375318632,13.2556757897085,0.));
#212739=CARTESIAN_POINT('Ctrl Pts',(19.8586778231711,13.2609038446525,0.));
#212740=CARTESIAN_POINT('Ctrl Pts',(19.8788333760571,13.2661050556128,0.));
#212741=CARTESIAN_POINT('Ctrl Pts',(19.8991035111739,13.2712788215015,0.));
#212742=CARTESIAN_POINT('Ctrl Pts',(19.9194875559419,13.2764245494354,0.));
#212743=CARTESIAN_POINT('Ctrl Pts',(19.9399848444019,13.2815416545663,0.));
#212744=CARTESIAN_POINT('Ctrl Pts',(19.9605947170589,13.2866295599152,0.));
#212745=CARTESIAN_POINT('Ctrl Pts',(19.9813165207174,13.2916876962098,0.));
#212746=CARTESIAN_POINT('Ctrl Pts',(20.0021496083742,13.296715501731,0.));
#212747=CARTESIAN_POINT('Ctrl Pts',(20.0230933391039,13.3017124221639,0.));
#212748=CARTESIAN_POINT('Ctrl Pts',(20.0441470779345,13.3066779104515,0.));
#212749=CARTESIAN_POINT('Ctrl Pts',(20.0653101957188,13.3116114266514,0.));
#212750=CARTESIAN_POINT('Ctrl Pts',(20.0865820689883,13.3165124377963,0.));
#212751=CARTESIAN_POINT('Ctrl Pts',(20.1079620798377,13.3213804177588,0.));
#212752=CARTESIAN_POINT('Ctrl Pts',(20.1294496158405,13.3262148471228,0.));
#212753=CARTESIAN_POINT('Ctrl Pts',(20.1510440699477,13.3310152130565,0.));
#212754=CARTESIAN_POINT('Ctrl Pts',(20.1727448403818,13.3357810091903,0.));
#212755=CARTESIAN_POINT('Ctrl Pts',(20.1945513305233,13.3405117354969,0.));
#212756=CARTESIAN_POINT('Ctrl Pts',(20.2164629487855,13.3452068981763,0.));
#212757=CARTESIAN_POINT('Ctrl Pts',(20.2384791085354,13.3498660095382,0.));
#212758=CARTESIAN_POINT('Ctrl Pts',(20.2605992280117,13.3544885878886,0.));
#212759=CARTESIAN_POINT('Ctrl Pts',(20.2828227302337,13.3590741574194,0.));
#212760=CARTESIAN_POINT('Ctrl Pts',(20.3051490429049,13.3636222481017,0.));
#212761=CARTESIAN_POINT('Ctrl Pts',(20.3275775983032,13.3681323955828,0.));
#212762=CARTESIAN_POINT('Ctrl Pts',(20.3501078331818,13.372604141087,0.));
#212763=CARTESIAN_POINT('Ctrl Pts',(20.3727391887187,13.377037031319,0.));
#212764=CARTESIAN_POINT('Ctrl Pts',(20.3954711104504,13.3814306183721,0.));
#212765=CARTESIAN_POINT('Ctrl Pts',(20.4183030482002,13.3857844596387,0.));
#212766=CARTESIAN_POINT('Ctrl Pts',(20.4412344560007,13.3900981177254,0.));
#212767=CARTESIAN_POINT('Ctrl Pts',(20.4642647920038,13.3943711603739,0.));
#212768=CARTESIAN_POINT('Ctrl Pts',(20.4873935184041,13.3986031603716,0.));
#212769=CARTESIAN_POINT('Ctrl Pts',(20.5106201013755,13.4027936954529,0.));
#212770=CARTESIAN_POINT('Ctrl Pts',(20.5339440109957,13.4069423482077,0.));
#212771=CARTESIAN_POINT('Ctrl Pts',(20.557364721164,13.4110487059912,0.));
#212772=CARTESIAN_POINT('Ctrl Pts',(20.5808817095155,13.4151123608411,0.));
#212773=CARTESIAN_POINT('Ctrl Pts',(20.6044944573151,13.4191329093932,0.));
#212774=CARTESIAN_POINT('Ctrl Pts',(20.6282024494234,13.4231099528178,0.));
#212775=CARTESIAN_POINT('Ctrl Pts',(20.6520051742867,13.4270430967651,0.));
#212776=CARTESIAN_POINT('Ctrl Pts',(20.6759021239102,13.4309319513119,0.));
#212777=CARTESIAN_POINT('Ctrl Pts',(20.6998927938288,13.4347761309154,0.));
#212778=CARTESIAN_POINT('Ctrl Pts',(20.7239766830675,13.4385752543663,0.));
#212779=CARTESIAN_POINT('Ctrl Pts',(20.7481532941014,13.4423289447561,0.));
#212780=CARTESIAN_POINT('Ctrl Pts',(20.7724221327609,13.4460368293689,0.));
#212781=CARTESIAN_POINT('Ctrl Pts',(20.7967827081228,13.4496985395637,0.));
#212782=CARTESIAN_POINT('Ctrl Pts',(20.821234532398,13.4533137106667,0.));
#212783=CARTESIAN_POINT('Ctrl Pts',(20.8457771208083,13.4568819818631,0.));
#212784=CARTESIAN_POINT('Ctrl Pts',(20.8704099914641,13.4604029960983,0.));
#212785=CARTESIAN_POINT('Ctrl Pts',(20.8951326652158,13.4638763999725,0.));
#212786=CARTESIAN_POINT('Ctrl Pts',(20.9199446657583,13.4673018437717,0.));
#212787=CARTESIAN_POINT('Ctrl Pts',(20.9448455197557,13.4706789815166,0.));
#212788=CARTESIAN_POINT('Ctrl Pts',(20.9698347569477,13.4740074710086,0.));
#212789=CARTESIAN_POINT('Ctrl Pts',(20.9949119102592,13.4772869738879,0.));
#212790=CARTESIAN_POINT('Ctrl Pts',(21.0200765158884,13.4805171556822,0.));
#212791=CARTESIAN_POINT('Ctrl Pts',(21.0453281134245,13.4836976858912,0.));
#212792=CARTESIAN_POINT('Ctrl Pts',(21.0706662455199,13.4868282377191,0.));
#212793=CARTESIAN_POINT('Ctrl Pts',(21.0960904575046,13.4899084877717,0.));
#212794=CARTESIAN_POINT('Ctrl Pts',(21.1216002970207,13.4929381157778,0.));
#212795=CARTESIAN_POINT('Ctrl Pts',(21.1471953136209,13.4959168042934,0.));
#212796=CARTESIAN_POINT('Ctrl Pts',(21.1728750584175,13.4988442384491,0.));
#212797=CARTESIAN_POINT('Ctrl Pts',(21.1986390835828,13.5017201056088,0.));
#212798=CARTESIAN_POINT('Ctrl Pts',(21.2244869429332,13.5045440957404,0.));
#212799=CARTESIAN_POINT('Ctrl Pts',(21.250418192743,13.5073159019452,0.));
#212800=CARTESIAN_POINT('Ctrl Pts',(21.2764323924442,13.5100352209205,0.));
#212801=CARTESIAN_POINT('Ctrl Pts',(21.3025291054235,13.5127017534971,0.));
#212802=CARTESIAN_POINT('Ctrl Pts',(21.3287078996341,13.5153152050555,0.));
#212803=CARTESIAN_POINT('Ctrl Pts',(21.3549683486222,13.5178752862466,0.));
#212804=CARTESIAN_POINT('Ctrl Pts',(21.3813100304973,13.5203817122504,0.));
#212805=CARTESIAN_POINT('Ctrl Pts',(21.4077325259324,13.5228342013516,0.));
#212806=CARTESIAN_POINT('Ctrl Pts',(21.4342354165259,13.5252324737802,0.));
#212807=CARTESIAN_POINT('Ctrl Pts',(21.4608182828697,13.5275762503555,0.));
#212808=CARTESIAN_POINT('Ctrl Pts',(21.4874807030468,13.5298652514355,0.));
#212809=CARTESIAN_POINT('Ctrl Pts',(21.5142222501666,13.5320991952138,0.));
#212810=CARTESIAN_POINT('Ctrl Pts',(21.5410424932503,13.5342777983215,0.));
#212811=CARTESIAN_POINT('Ctrl Pts',(21.5679410019001,13.536400779028,0.));
#212812=CARTESIAN_POINT('Ctrl Pts',(21.5949173499013,13.5384678597195,0.));
#212813=CARTESIAN_POINT('Ctrl Pts',(21.6219711193946,13.5404787697792,0.));
#212814=CARTESIAN_POINT('Ctrl Pts',(21.6491019044648,13.5424332480699,0.));
#212815=CARTESIAN_POINT('Ctrl Pts',(21.6763093157699,13.5443310461526,0.));
#212816=CARTESIAN_POINT('Ctrl Pts',(21.7035929822955,13.5461719295048,0.));
#212817=CARTESIAN_POINT('Ctrl Pts',(21.7309525412281,13.5479556704481,0.));
#212818=CARTESIAN_POINT('Ctrl Pts',(21.7583876294554,13.5496820422211,0.));
#212819=CARTESIAN_POINT('Ctrl Pts',(21.7858978745865,13.551350812725,0.));
#212820=CARTESIAN_POINT('Ctrl Pts',(21.8134828857967,13.5529617381573,0.));
#212821=CARTESIAN_POINT('Ctrl Pts',(21.8411422456075,13.5545145573031,0.));
#212822=CARTESIAN_POINT('Ctrl Pts',(21.8688754989365,13.5560089839385,0.));
#212823=CARTESIAN_POINT('Ctrl Pts',(21.8966821688824,13.5574447178425,0.));
#212824=CARTESIAN_POINT('Ctrl Pts',(21.9245617765769,13.5588214586604,0.));
#212825=CARTESIAN_POINT('Ctrl Pts',(21.9525138592813,13.5601389185257,0.));
#212826=CARTESIAN_POINT('Ctrl Pts',(21.9805379899168,13.5613968357561,0.));
#212827=CARTESIAN_POINT('Ctrl Pts',(22.0086337943449,13.5625949868333,0.));
#212828=CARTESIAN_POINT('Ctrl Pts',(22.0368009736295,13.5637332022473,0.));
#212829=CARTESIAN_POINT('Ctrl Pts',(22.0650393089609,13.5648113689033,0.));
#212830=CARTESIAN_POINT('Ctrl Pts',(22.0933486464593,13.5658294169284,0.));
#212831=CARTESIAN_POINT('Ctrl Pts',(22.1217288871975,13.5667873105359,0.));
#212832=CARTESIAN_POINT('Ctrl Pts',(22.1444897575194,13.5675054919061,0.));
#212833=CARTESIAN_POINT('Ctrl Pts',(22.1615922805008,13.5680170531805,0.));
#212834=CARTESIAN_POINT('Ctrl Pts',(22.1730081264608,13.5683460612942,0.));
#212835=CARTESIAN_POINT('Ctrl Pts',(22.1787195904339,13.5685075571671,0.));
#212836=CARTESIAN_POINT('',(22.1787195904339,13.5685075571671,0.));
#212837=CARTESIAN_POINT('Origin',(20.2687213152502,7.17139709155223,0.));
#212838=CARTESIAN_POINT('',(21.2610617890679,7.52250298901264,0.));
#212839=CARTESIAN_POINT('',(21.2610617890679,7.52250298901264,0.));
#212840=CARTESIAN_POINT('',(10.1343606576251,3.58569854577611,0.));
#212841=CARTESIAN_POINT('Ctrl Pts',(22.8400320311648,12.4230808101438,0.));
#212842=CARTESIAN_POINT('Ctrl Pts',(22.8400320311648,12.4230808101438,12.));
#212843=CARTESIAN_POINT('Ctrl Pts',(22.8370364396459,12.418215285186,0.));
#212844=CARTESIAN_POINT('Ctrl Pts',(22.8370364396459,12.418215285186,12.));
#212845=CARTESIAN_POINT('Ctrl Pts',(22.8310435872747,12.4084933766347,0.));
#212846=CARTESIAN_POINT('Ctrl Pts',(22.8310435872747,12.4084933766347,12.));
#212847=CARTESIAN_POINT('Ctrl Pts',(22.8220493007173,12.3939379378998,0.));
#212848=CARTESIAN_POINT('Ctrl Pts',(22.8220493007173,12.3939379378998,12.));
#212849=CARTESIAN_POINT('Ctrl Pts',(22.81004690224,12.374585536673,0.));
#212850=CARTESIAN_POINT('Ctrl Pts',(22.81004690224,12.374585536673,12.));
#212851=CARTESIAN_POINT('Ctrl Pts',(22.795027221673,12.3504864740319,0.));
#212852=CARTESIAN_POINT('Ctrl Pts',(22.795027221673,12.3504864740319,12.));
#212853=CARTESIAN_POINT('Ctrl Pts',(22.7799908974768,12.3264788926075,0.));
#212854=CARTESIAN_POINT('Ctrl Pts',(22.7799908974768,12.3264788926075,12.));
#212855=CARTESIAN_POINT('Ctrl Pts',(22.764938010105,12.3025628601792,0.));
#212856=CARTESIAN_POINT('Ctrl Pts',(22.764938010105,12.3025628601792,12.));
#212857=CARTESIAN_POINT('Ctrl Pts',(22.7498686970069,12.2787384750742,0.));
#212858=CARTESIAN_POINT('Ctrl Pts',(22.7498686970069,12.2787384750742,12.));
#212859=CARTESIAN_POINT('Ctrl Pts',(22.7347831655287,12.2550058702395,0.));
#212860=CARTESIAN_POINT('Ctrl Pts',(22.7347831655287,12.2550058702395,12.));
#212861=CARTESIAN_POINT('Ctrl Pts',(22.7196817119374,12.2313652198061,0.));
#212862=CARTESIAN_POINT('Ctrl Pts',(22.7196817119374,12.2313652198061,12.));
#212863=CARTESIAN_POINT('Ctrl Pts',(22.7045647168747,12.2078167360284,0.));
#212864=CARTESIAN_POINT('Ctrl Pts',(22.7045647168747,12.2078167360284,12.));
#212865=CARTESIAN_POINT('Ctrl Pts',(22.6894326205037,12.1843606579262,0.));
#212866=CARTESIAN_POINT('Ctrl Pts',(22.6894326205037,12.1843606579262,12.));
#212867=CARTESIAN_POINT('Ctrl Pts',(22.6742859034944,12.1609972423099,0.));
#212868=CARTESIAN_POINT('Ctrl Pts',(22.6742859034944,12.1609972423099,12.));
#212869=CARTESIAN_POINT('Ctrl Pts',(22.6591250653965,12.1377267537145,0.));
#212870=CARTESIAN_POINT('Ctrl Pts',(22.6591250653965,12.1377267537145,12.));
#212871=CARTESIAN_POINT('Ctrl Pts',(22.6439506046605,12.1145494550383,0.));
#212872=CARTESIAN_POINT('Ctrl Pts',(22.6439506046605,12.1145494550383,12.));
#212873=CARTESIAN_POINT('Ctrl Pts',(22.6287629967056,12.0914655972823,0.));
#212874=CARTESIAN_POINT('Ctrl Pts',(22.6287629967056,12.0914655972823,12.));
#212875=CARTESIAN_POINT('Ctrl Pts',(22.6135626764898,12.0684754113862,0.));
#212876=CARTESIAN_POINT('Ctrl Pts',(22.6135626764898,12.0684754113862,12.));
#212877=CARTESIAN_POINT('Ctrl Pts',(22.5983500505644,12.0455791139128,0.));
#212878=CARTESIAN_POINT('Ctrl Pts',(22.5983500505644,12.0455791139128,12.));
#212879=CARTESIAN_POINT('Ctrl Pts',(22.5831255061282,12.0227769113127,0.));
#212880=CARTESIAN_POINT('Ctrl Pts',(22.5831255061282,12.0227769113127,12.));
#212881=CARTESIAN_POINT('Ctrl Pts',(22.5678894211181,12.0000690046695,0.));
#212882=CARTESIAN_POINT('Ctrl Pts',(22.5678894211181,12.0000690046695,12.));
#212883=CARTESIAN_POINT('Ctrl Pts',(22.5526421741158,11.9774555943496,0.));
#212884=CARTESIAN_POINT('Ctrl Pts',(22.5526421741158,11.9774555943496,12.));
#212885=CARTESIAN_POINT('Ctrl Pts',(22.5373841537307,11.9549368843997,0.));
#212886=CARTESIAN_POINT('Ctrl Pts',(22.5373841537307,11.9549368843997,12.));
#212887=CARTESIAN_POINT('Ctrl Pts',(22.5221157697883,11.9325130877803,0.));
#212888=CARTESIAN_POINT('Ctrl Pts',(22.5221157697883,11.9325130877803,12.));
#212889=CARTESIAN_POINT('Ctrl Pts',(22.5068374513973,11.9101844254557,0.));
#212890=CARTESIAN_POINT('Ctrl Pts',(22.5068374513973,11.9101844254557,12.));
#212891=CARTESIAN_POINT('Ctrl Pts',(22.4915496418485,11.8879511239943,0.));
#212892=CARTESIAN_POINT('Ctrl Pts',(22.4915496418485,11.8879511239943,12.));
#212893=CARTESIAN_POINT('Ctrl Pts',(22.4762527946702,11.8658134137019,0.));
#212894=CARTESIAN_POINT('Ctrl Pts',(22.4762527946702,11.8658134137019,12.));
#212895=CARTESIAN_POINT('Ctrl Pts',(22.4609473690471,11.8437715264487,0.));
#212896=CARTESIAN_POINT('Ctrl Pts',(22.4609473690471,11.8437715264487,12.));
#212897=CARTESIAN_POINT('Ctrl Pts',(22.4456338258735,11.8218256937889,0.));
#212898=CARTESIAN_POINT('Ctrl Pts',(22.4456338258735,11.8218256937889,12.));
#212899=CARTESIAN_POINT('Ctrl Pts',(22.430312622646,11.7999761445173,0.));
#212900=CARTESIAN_POINT('Ctrl Pts',(22.430312622646,11.7999761445173,12.));
#212901=CARTESIAN_POINT('Ctrl Pts',(22.4149842125008,11.7782231042039,0.));
#212902=CARTESIAN_POINT('Ctrl Pts',(22.4149842125008,11.7782231042039,12.));
#212903=CARTESIAN_POINT('Ctrl Pts',(22.3996490469191,11.7565667964764,0.));
#212904=CARTESIAN_POINT('Ctrl Pts',(22.3996490469191,11.7565667964764,12.));
#212905=CARTESIAN_POINT('Ctrl Pts',(22.3843075773899,11.7350074437961,0.));
#212906=CARTESIAN_POINT('Ctrl Pts',(22.3843075773899,11.7350074437961,12.));
#212907=CARTESIAN_POINT('Ctrl Pts',(22.3689602575491,11.7135452684532,0.));
#212908=CARTESIAN_POINT('Ctrl Pts',(22.3689602575491,11.7135452684532,12.));
#212909=CARTESIAN_POINT('Ctrl Pts',(22.3536075450029,11.6921804934056,0.));
#212910=CARTESIAN_POINT('Ctrl Pts',(22.3536075450029,11.6921804934056,12.));
#212911=CARTESIAN_POINT('Ctrl Pts',(22.3382499035619,11.6709133432985,0.));
#212912=CARTESIAN_POINT('Ctrl Pts',(22.3382499035619,11.6709133432985,12.));
#212913=CARTESIAN_POINT('Ctrl Pts',(22.3228878043976,11.6497440449857,0.));
#212914=CARTESIAN_POINT('Ctrl Pts',(22.3228878043976,11.6497440449857,12.));
#212915=CARTESIAN_POINT('Ctrl Pts',(22.3075217249049,11.6286728270009,0.));
#212916=CARTESIAN_POINT('Ctrl Pts',(22.3075217249049,11.6286728270009,12.));
#212917=CARTESIAN_POINT('Ctrl Pts',(22.2921521480356,11.6076999192357,0.));
#212918=CARTESIAN_POINT('Ctrl Pts',(22.2921521480356,11.6076999192357,12.));
#212919=CARTESIAN_POINT('Ctrl Pts',(22.2767795614348,11.5868255525188,0.));
#212920=CARTESIAN_POINT('Ctrl Pts',(22.2767795614348,11.5868255525188,12.));
#212921=CARTESIAN_POINT('Ctrl Pts',(22.2614044566898,11.5660499582403,0.));
#212922=CARTESIAN_POINT('Ctrl Pts',(22.2614044566898,11.5660499582403,12.));
#212923=CARTESIAN_POINT('Ctrl Pts',(22.2460273284654,11.5453733679121,0.));
#212924=CARTESIAN_POINT('Ctrl Pts',(22.2460273284654,11.5453733679121,12.));
#212925=CARTESIAN_POINT('Ctrl Pts',(22.2306486738901,11.5247960128477,0.));
#212926=CARTESIAN_POINT('Ctrl Pts',(22.2306486738901,11.5247960128477,12.));
#212927=CARTESIAN_POINT('Ctrl Pts',(22.2152689931022,11.5043181244242,0.));
#212928=CARTESIAN_POINT('Ctrl Pts',(22.2152689931022,11.5043181244242,12.));
#212929=CARTESIAN_POINT('Ctrl Pts',(22.1998887896436,11.483939934259,0.));
#212930=CARTESIAN_POINT('Ctrl Pts',(22.1998887896436,11.483939934259,12.));
#212931=CARTESIAN_POINT('Ctrl Pts',(22.184508570917,11.463661674411,0.));
#212932=CARTESIAN_POINT('Ctrl Pts',(22.184508570917,11.463661674411,12.));
#212933=CARTESIAN_POINT('Ctrl Pts',(22.1691288486096,11.443483577557,0.));
#212934=CARTESIAN_POINT('Ctrl Pts',(22.1691288486096,11.443483577557,12.));
#212935=CARTESIAN_POINT('Ctrl Pts',(22.1537501391487,11.4234058771742,0.));
#212936=CARTESIAN_POINT('Ctrl Pts',(22.1537501391487,11.4234058771742,12.));
#212937=CARTESIAN_POINT('Ctrl Pts',(22.1383729640964,11.4034288076908,0.));
#212938=CARTESIAN_POINT('Ctrl Pts',(22.1383729640964,11.4034288076908,12.));
#212939=CARTESIAN_POINT('Ctrl Pts',(22.1229978500186,11.3835526044256,0.));
#212940=CARTESIAN_POINT('Ctrl Pts',(22.1229978500186,11.3835526044256,12.));
#212941=CARTESIAN_POINT('Ctrl Pts',(22.1076253283979,11.3637775035367,0.));
#212942=CARTESIAN_POINT('Ctrl Pts',(22.1076253283979,11.3637775035367,12.));
#212943=CARTESIAN_POINT('Ctrl Pts',(22.0922559355294,11.3441037419553,0.));
#212944=CARTESIAN_POINT('Ctrl Pts',(22.0922559355294,11.3441037419553,12.));
#212945=CARTESIAN_POINT('Ctrl Pts',(22.0768902124267,11.3245315573168,0.));
#212946=CARTESIAN_POINT('Ctrl Pts',(22.0768902124267,11.3245315573168,12.));
#212947=CARTESIAN_POINT('Ctrl Pts',(22.0615287047179,11.3050611878771,0.));
#212948=CARTESIAN_POINT('Ctrl Pts',(22.0615287047179,11.3050611878771,12.));
#212949=CARTESIAN_POINT('Ctrl Pts',(22.046171962566,11.2856928724374,0.));
#212950=CARTESIAN_POINT('Ctrl Pts',(22.046171962566,11.2856928724374,12.));
#212951=CARTESIAN_POINT('Ctrl Pts',(22.030820540835,11.2664268504206,0.));
#212952=CARTESIAN_POINT('Ctrl Pts',(22.030820540835,11.2664268504206,12.));
#212953=CARTESIAN_POINT('Ctrl Pts',(22.0154749992363,11.2472633619275,0.));
#212954=CARTESIAN_POINT('Ctrl Pts',(22.0154749992363,11.2472633619275,12.));
#212955=CARTESIAN_POINT('Ctrl Pts',(22.0001359024839,11.2282026477896,0.));
#212956=CARTESIAN_POINT('Ctrl Pts',(22.0001359024839,11.2282026477896,12.));
#212957=CARTESIAN_POINT('Ctrl Pts',(21.9848038204439,11.2092449496125,0.));
#212958=CARTESIAN_POINT('Ctrl Pts',(21.9848038204439,11.2092449496125,12.));
#212959=CARTESIAN_POINT('Ctrl Pts',(21.9694793282914,11.190390509811,0.));
#212960=CARTESIAN_POINT('Ctrl Pts',(21.9694793282914,11.190390509811,12.));
#212961=CARTESIAN_POINT('Ctrl Pts',(21.9541630066506,11.1716395716376,0.));
#212962=CARTESIAN_POINT('Ctrl Pts',(21.9541630066506,11.1716395716376,12.));
#212963=CARTESIAN_POINT('Ctrl Pts',(21.9388554416439,11.1529923792003,0.));
#212964=CARTESIAN_POINT('Ctrl Pts',(21.9388554416439,11.1529923792003,12.));
#212965=CARTESIAN_POINT('Ctrl Pts',(21.923557224952,11.1344491774741,0.));
#212966=CARTESIAN_POINT('Ctrl Pts',(21.923557224952,11.1344491774741,12.));
#212967=CARTESIAN_POINT('Ctrl Pts',(21.9082689538688,11.1160102123024,0.));
#212968=CARTESIAN_POINT('Ctrl Pts',(21.9082689538688,11.1160102123024,12.));
#212969=CARTESIAN_POINT('Ctrl Pts',(21.8929912313608,11.0976757303944,0.));
#212970=CARTESIAN_POINT('Ctrl Pts',(21.8929912313608,11.0976757303944,12.));
#212971=CARTESIAN_POINT('Ctrl Pts',(21.877724666119,11.0794459793057,0.));
#212972=CARTESIAN_POINT('Ctrl Pts',(21.877724666119,11.0794459793057,12.));
#212973=CARTESIAN_POINT('Ctrl Pts',(21.8624698726318,11.0613212074363,0.));
#212974=CARTESIAN_POINT('Ctrl Pts',(21.8624698726318,11.0613212074363,12.));
#212975=CARTESIAN_POINT('Ctrl Pts',(21.8472274713103,11.0433016640807,0.));
#212976=CARTESIAN_POINT('Ctrl Pts',(21.8472274713103,11.0433016640807,12.));
#212977=CARTESIAN_POINT('Ctrl Pts',(21.8319980886033,11.0253875994598,0.));
#212978=CARTESIAN_POINT('Ctrl Pts',(21.8319980886033,11.0253875994598,12.));
#212979=CARTESIAN_POINT('Ctrl Pts',(21.8167823571168,11.0075792647477,0.));
#212980=CARTESIAN_POINT('Ctrl Pts',(21.8167823571168,11.0075792647477,12.));
#212981=CARTESIAN_POINT('Ctrl Pts',(21.8015809157301,10.9898769120912,0.));
#212982=CARTESIAN_POINT('Ctrl Pts',(21.8015809157301,10.9898769120912,12.));
#212983=CARTESIAN_POINT('Ctrl Pts',(21.7863944097141,10.9722807946156,0.));
#212984=CARTESIAN_POINT('Ctrl Pts',(21.7863944097141,10.9722807946156,12.));
#212985=CARTESIAN_POINT('Ctrl Pts',(21.7712234908464,10.9547911664455,0.));
#212986=CARTESIAN_POINT('Ctrl Pts',(21.7712234908464,10.9547911664455,12.));
#212987=CARTESIAN_POINT('Ctrl Pts',(21.7560688175247,10.9374082827444,0.));
#212988=CARTESIAN_POINT('Ctrl Pts',(21.7560688175247,10.9374082827444,12.));
#212989=CARTESIAN_POINT('Ctrl Pts',(21.7409310548797,10.9201323997384,0.));
#212990=CARTESIAN_POINT('Ctrl Pts',(21.7409310548797,10.9201323997384,12.));
#212991=CARTESIAN_POINT('Ctrl Pts',(21.7258108748873,10.902963774734,0.));
#212992=CARTESIAN_POINT('Ctrl Pts',(21.7258108748873,10.902963774734,12.));
#212993=CARTESIAN_POINT('Ctrl Pts',(21.7107089564825,10.8859026661293,0.));
#212994=CARTESIAN_POINT('Ctrl Pts',(21.7107089564825,10.8859026661293,12.));
#212995=CARTESIAN_POINT('Ctrl Pts',(21.6956259856672,10.8689493334095,0.));
#212996=CARTESIAN_POINT('Ctrl Pts',(21.6956259856672,10.8689493334095,12.));
#212997=CARTESIAN_POINT('Ctrl Pts',(21.6805626556467,10.8521040371835,0.));
#212998=CARTESIAN_POINT('Ctrl Pts',(21.6805626556467,10.8521040371835,12.));
#212999=CARTESIAN_POINT('Ctrl Pts',(21.6655196669732,10.8353670392272,0.));
#213000=CARTESIAN_POINT('Ctrl Pts',(21.6655196669732,10.8353670392272,12.));
#213001=CARTESIAN_POINT('Ctrl Pts',(21.6504977276866,10.8187386025136,0.));
#213002=CARTESIAN_POINT('Ctrl Pts',(21.6504977276866,10.8187386025136,12.));
#213003=CARTESIAN_POINT('Ctrl Pts',(21.6354975534557,10.8022189912369,0.));
#213004=CARTESIAN_POINT('Ctrl Pts',(21.6354975534557,10.8022189912369,12.));
#213005=CARTESIAN_POINT('Ctrl Pts',(21.6205198677173,10.7858084708261,0.));
#213006=CARTESIAN_POINT('Ctrl Pts',(21.6205198677173,10.7858084708261,12.));
#213007=CARTESIAN_POINT('Ctrl Pts',(21.6055654018176,10.7695073079552,0.));
#213008=CARTESIAN_POINT('Ctrl Pts',(21.6055654018176,10.7695073079552,12.));
#213009=CARTESIAN_POINT('Ctrl Pts',(21.5906348951743,10.7533157705941,0.));
#213010=CARTESIAN_POINT('Ctrl Pts',(21.5906348951743,10.7533157705941,12.));
#213011=CARTESIAN_POINT('Ctrl Pts',(21.5757290954371,10.7372341280467,0.));
#213012=CARTESIAN_POINT('Ctrl Pts',(21.5757290954371,10.7372341280467,12.));
#213013=CARTESIAN_POINT('Ctrl Pts',(21.5608487586468,10.7212626509816,0.));
#213014=CARTESIAN_POINT('Ctrl Pts',(21.5608487586468,10.7212626509816,12.));
#213015=CARTESIAN_POINT('Ctrl Pts',(21.5459946493955,10.7054016114571,0.));
#213016=CARTESIAN_POINT('Ctrl Pts',(21.5459946493955,10.7054016114571,12.));
#213017=CARTESIAN_POINT('Ctrl Pts',(21.5311675409807,10.689651282929,0.));
#213018=CARTESIAN_POINT('Ctrl Pts',(21.5311675409807,10.689651282929,12.));
#213019=CARTESIAN_POINT('Ctrl Pts',(21.51636821558,10.6740119402834,0.));
#213020=CARTESIAN_POINT('Ctrl Pts',(21.51636821558,10.6740119402834,12.));
#213021=CARTESIAN_POINT('Ctrl Pts',(21.5015974644449,10.6584838598939,0.));
#213022=CARTESIAN_POINT('Ctrl Pts',(21.5015974644449,10.6584838598939,12.));
#213023=CARTESIAN_POINT('Ctrl Pts',(21.4868560880889,10.6430673196607,0.));
#213024=CARTESIAN_POINT('Ctrl Pts',(21.4868560880889,10.6430673196607,12.));
#213025=CARTESIAN_POINT('Ctrl Pts',(21.4721448964766,10.6277625990456,0.));
#213026=CARTESIAN_POINT('Ctrl Pts',(21.4721448964766,10.6277625990456,12.));
#213027=CARTESIAN_POINT('Ctrl Pts',(21.4574647092097,10.6125699790961,0.));
#213028=CARTESIAN_POINT('Ctrl Pts',(21.4574647092097,10.6125699790961,12.));
#213029=CARTESIAN_POINT('Ctrl Pts',(21.4428163557144,10.5974897424622,0.));
#213030=CARTESIAN_POINT('Ctrl Pts',(21.4428163557144,10.5974897424622,12.));
#213031=CARTESIAN_POINT('Ctrl Pts',(21.4282006754631,10.5825221734573,0.));
#213032=CARTESIAN_POINT('Ctrl Pts',(21.4282006754631,10.5825221734573,12.));
#213033=CARTESIAN_POINT('Ctrl Pts',(21.4136185181979,10.5676675581108,0.));
#213034=CARTESIAN_POINT('Ctrl Pts',(21.4136185181979,10.5676675581108,12.));
#213035=CARTESIAN_POINT('Ctrl Pts',(21.3990707441497,10.5529261842108,0.));
#213036=CARTESIAN_POINT('Ctrl Pts',(21.3990707441497,10.5529261842108,12.));
#213037=CARTESIAN_POINT('Ctrl Pts',(21.3845582242602,10.5382983413421,0.));
#213038=CARTESIAN_POINT('Ctrl Pts',(21.3845582242602,10.5382983413421,12.));
#213039=CARTESIAN_POINT('Ctrl Pts',(21.3700818403936,10.5237843209057,0.));
#213040=CARTESIAN_POINT('Ctrl Pts',(21.3700818403936,10.5237843209057,12.));
#213041=CARTESIAN_POINT('Ctrl Pts',(21.3556424855814,10.5093844161685,0.));
#213042=CARTESIAN_POINT('Ctrl Pts',(21.3556424855814,10.5093844161685,12.));
#213043=CARTESIAN_POINT('Ctrl Pts',(21.3412410642904,10.4950989223337,0.));
#213044=CARTESIAN_POINT('Ctrl Pts',(21.3412410642904,10.4950989223337,12.));
#213045=CARTESIAN_POINT('Ctrl Pts',(21.3268784926819,10.4809281365931,0.));
#213046=CARTESIAN_POINT('Ctrl Pts',(21.3268784926819,10.4809281365931,12.));
#213047=CARTESIAN_POINT('Ctrl Pts',(21.3125556988731,10.4668723581768,0.));
#213048=CARTESIAN_POINT('Ctrl Pts',(21.3125556988731,10.4668723581768,12.));
#213049=CARTESIAN_POINT('Ctrl Pts',(21.2982736231931,10.4529318883874,0.));
#213050=CARTESIAN_POINT('Ctrl Pts',(21.2982736231931,10.4529318883874,12.));
#213051=CARTESIAN_POINT('Ctrl Pts',(21.2840332184483,10.4391070306391,0.));
#213052=CARTESIAN_POINT('Ctrl Pts',(21.2840332184483,10.4391070306391,12.));
#213053=CARTESIAN_POINT('Ctrl Pts',(21.2698354502403,10.42539809054,0.));
#213054=CARTESIAN_POINT('Ctrl Pts',(21.2698354502403,10.42539809054,12.));
#213055=CARTESIAN_POINT('Ctrl Pts',(21.255681297275,10.4118053759588,0.));
#213056=CARTESIAN_POINT('Ctrl Pts',(21.255681297275,10.4118053759588,12.));
#213057=CARTESIAN_POINT('Ctrl Pts',(21.2415717516714,10.3983291970846,0.));
#213058=CARTESIAN_POINT('Ctrl Pts',(21.2415717516714,10.3983291970846,12.));
#213059=CARTESIAN_POINT('Ctrl Pts',(21.22750781927,10.3849698664786,0.));
#213060=CARTESIAN_POINT('Ctrl Pts',(21.22750781927,10.3849698664786,12.));
#213061=CARTESIAN_POINT('Ctrl Pts',(21.2134905199345,10.371727699113,0.));
#213062=CARTESIAN_POINT('Ctrl Pts',(21.2134905199345,10.371727699113,12.));
#213063=CARTESIAN_POINT('Ctrl Pts',(21.199520887919,10.3586030124587,0.));
#213064=CARTESIAN_POINT('Ctrl Pts',(21.199520887919,10.3586030124587,12.));
#213065=CARTESIAN_POINT('Ctrl Pts',(21.1855999722416,10.3455961265701,0.));
#213066=CARTESIAN_POINT('Ctrl Pts',(21.1855999722416,10.3455961265701,12.));
#213067=CARTESIAN_POINT('Ctrl Pts',(21.1717288370509,10.3327073641572,0.));
#213068=CARTESIAN_POINT('Ctrl Pts',(21.1717288370509,10.3327073641572,12.));
#213069=CARTESIAN_POINT('Ctrl Pts',(21.1579085619965,10.3199370506544,0.));
#213070=CARTESIAN_POINT('Ctrl Pts',(21.1579085619965,10.3199370506544,12.));
#213071=CARTESIAN_POINT('Ctrl Pts',(21.1441402425843,10.3072855142687,0.));
#213072=CARTESIAN_POINT('Ctrl Pts',(21.1441402425843,10.3072855142687,12.));
#213073=CARTESIAN_POINT('Ctrl Pts',(21.1304249906002,10.2947530860721,0.));
#213074=CARTESIAN_POINT('Ctrl Pts',(21.1304249906002,10.2947530860721,12.));
#213075=CARTESIAN_POINT('Ctrl Pts',(21.1167639345631,10.2823401001072,0.));
#213076=CARTESIAN_POINT('Ctrl Pts',(21.1167639345631,10.2823401001072,12.));
#213077=CARTESIAN_POINT('Ctrl Pts',(21.1031582201627,10.2700468934744,0.));
#213078=CARTESIAN_POINT('Ctrl Pts',(21.1031582201627,10.2700468934744,12.));
#213079=CARTESIAN_POINT('Ctrl Pts',(21.0896090107063,10.2578738064181,0.));
#213080=CARTESIAN_POINT('Ctrl Pts',(21.0896090107063,10.2578738064181,12.));
#213081=CARTESIAN_POINT('Ctrl Pts',(21.0761174875444,10.2458211823912,0.));
#213082=CARTESIAN_POINT('Ctrl Pts',(21.0761174875444,10.2458211823912,12.));
#213083=CARTESIAN_POINT('Ctrl Pts',(21.0626848505663,10.2338893681567,0.));
#213084=CARTESIAN_POINT('Ctrl Pts',(21.0626848505663,10.2338893681567,12.));
#213085=CARTESIAN_POINT('Ctrl Pts',(21.0493123187483,10.2220787139155,0.));
#213086=CARTESIAN_POINT('Ctrl Pts',(21.0493123187483,10.2220787139155,12.));
#213087=CARTESIAN_POINT('Ctrl Pts',(21.0360011306815,10.2103895734123,0.));
#213088=CARTESIAN_POINT('Ctrl Pts',(21.0360011306815,10.2103895734123,12.));
#213089=CARTESIAN_POINT('Ctrl Pts',(21.0227525451107,10.1988223040425,0.));
#213090=CARTESIAN_POINT('Ctrl Pts',(21.0227525451107,10.1988223040425,12.));
#213091=CARTESIAN_POINT('Ctrl Pts',(21.0095678414486,10.187377266936,0.));
#213092=CARTESIAN_POINT('Ctrl Pts',(21.0095678414486,10.187377266936,12.));
#213093=CARTESIAN_POINT('Ctrl Pts',(20.9964483203686,10.1760548270767,0.));
#213094=CARTESIAN_POINT('Ctrl Pts',(20.9964483203686,10.1760548270767,12.));
#213095=CARTESIAN_POINT('Ctrl Pts',(20.9833953044736,10.1648553534568,0.));
#213096=CARTESIAN_POINT('Ctrl Pts',(20.9833953044736,10.1648553534568,12.));
#213097=CARTESIAN_POINT('Ctrl Pts',(20.9704101389369,10.1537792192065,0.));
#213098=CARTESIAN_POINT('Ctrl Pts',(20.9704101389369,10.1537792192065,12.));
#213099=CARTESIAN_POINT('Ctrl Pts',(20.9574941921591,10.1428268017256,0.));
#213100=CARTESIAN_POINT('Ctrl Pts',(20.9574941921591,10.1428268017256,12.));
#213101=CARTESIAN_POINT('Ctrl Pts',(20.9446488563933,10.1319984827908,0.));
#213102=CARTESIAN_POINT('Ctrl Pts',(20.9446488563933,10.1319984827908,12.));
#213103=CARTESIAN_POINT('Ctrl Pts',(20.9318755484734,10.1212946487057,0.));
#213104=CARTESIAN_POINT('Ctrl Pts',(20.9318755484734,10.1212946487057,12.));
#213105=CARTESIAN_POINT('Ctrl Pts',(20.919175710627,10.1107156904836,0.));
#213106=CARTESIAN_POINT('Ctrl Pts',(20.919175710627,10.1107156904836,12.));
#213107=CARTESIAN_POINT('Ctrl Pts',(20.9065508112557,10.1002620040076,0.));
#213108=CARTESIAN_POINT('Ctrl Pts',(20.9065508112557,10.1002620040076,12.));
#213109=CARTESIAN_POINT('Ctrl Pts',(20.894002345737,10.0899339901916,0.));
#213110=CARTESIAN_POINT('Ctrl Pts',(20.894002345737,10.0899339901916,12.));
#213111=CARTESIAN_POINT('Ctrl Pts',(20.881531837184,10.0797320551154,0.));
#213112=CARTESIAN_POINT('Ctrl Pts',(20.881531837184,10.0797320551154,12.));
#213113=CARTESIAN_POINT('Ctrl Pts',(20.86914083737,10.0696566102218,0.));
#213114=CARTESIAN_POINT('Ctrl Pts',(20.86914083737,10.0696566102218,12.));
#213115=CARTESIAN_POINT('Ctrl Pts',(20.8568309277316,10.0597080725375,0.));
#213116=CARTESIAN_POINT('Ctrl Pts',(20.8568309277316,10.0597080725375,12.));
#213117=CARTESIAN_POINT('Ctrl Pts',(20.8446037203402,10.0498868648733,0.));
#213118=CARTESIAN_POINT('Ctrl Pts',(20.8446037203402,10.0498868648733,12.));
#213119=CARTESIAN_POINT('Ctrl Pts',(20.8324608588909,10.0401934160234,0.));
#213120=CARTESIAN_POINT('Ctrl Pts',(20.8324608588909,10.0401934160234,12.));
#213121=CARTESIAN_POINT('Ctrl Pts',(20.8204040196602,10.0306281609435,0.));
#213122=CARTESIAN_POINT('Ctrl Pts',(20.8204040196602,10.0306281609435,12.));
#213123=CARTESIAN_POINT('Ctrl Pts',(20.8084349126888,10.0211915410095,0.));
#213124=CARTESIAN_POINT('Ctrl Pts',(20.8084349126888,10.0211915410095,12.));
#213125=CARTESIAN_POINT('Ctrl Pts',(20.7965552829908,10.0118840042786,0.));
#213126=CARTESIAN_POINT('Ctrl Pts',(20.7965552829908,10.0118840042786,12.));
#213127=CARTESIAN_POINT('Ctrl Pts',(20.7847669117568,10.0027060057389,0.));
#213128=CARTESIAN_POINT('Ctrl Pts',(20.7847669117568,10.0027060057389,12.));
#213129=CARTESIAN_POINT('Ctrl Pts',(20.7730716175417,9.9936580075464,0.));
#213130=CARTESIAN_POINT('Ctrl Pts',(20.7730716175417,9.9936580075464,12.));
#213131=CARTESIAN_POINT('Ctrl Pts',(20.761471257499,9.98474047926853,0.));
#213132=CARTESIAN_POINT('Ctrl Pts',(20.761471257499,9.98474047926853,12.));
#213133=CARTESIAN_POINT('Ctrl Pts',(20.7499677289627,9.9759538982347,0.));
#213134=CARTESIAN_POINT('Ctrl Pts',(20.7499677289627,9.9759538982347,12.));
#213135=CARTESIAN_POINT('Ctrl Pts',(20.7385629709795,9.96729874986202,0.));
#213136=CARTESIAN_POINT('Ctrl Pts',(20.7385629709795,9.96729874986202,12.));
#213137=CARTESIAN_POINT('Ctrl Pts',(20.7272589658751,9.95877552798398,0.));
#213138=CARTESIAN_POINT('Ctrl Pts',(20.7272589658751,9.95877552798398,12.));
#213139=CARTESIAN_POINT('Ctrl Pts',(20.7160577407579,9.95038473514949,0.));
#213140=CARTESIAN_POINT('Ctrl Pts',(20.7160577407579,9.95038473514949,12.));
#213141=CARTESIAN_POINT('Ctrl Pts',(20.7049613692234,9.94212688298236,0.));
#213142=CARTESIAN_POINT('Ctrl Pts',(20.7049613692234,9.94212688298236,12.));
#213143=CARTESIAN_POINT('Ctrl Pts',(20.6939719732484,9.9340024925973,0.));
#213144=CARTESIAN_POINT('Ctrl Pts',(20.6939719732484,9.9340024925973,12.));
#213145=CARTESIAN_POINT('Ctrl Pts',(20.6830917250255,9.92601209498749,0.));
#213146=CARTESIAN_POINT('Ctrl Pts',(20.6830917250255,9.92601209498749,12.));
#213147=CARTESIAN_POINT('Ctrl Pts',(20.6723228488263,9.91815623141289,0.));
#213148=CARTESIAN_POINT('Ctrl Pts',(20.6723228488263,9.91815623141289,12.));
#213149=CARTESIAN_POINT('Ctrl Pts',(20.6616676228315,9.91043545377008,0.));
#213150=CARTESIAN_POINT('Ctrl Pts',(20.6616676228315,9.91043545377008,12.));
#213151=CARTESIAN_POINT('Ctrl Pts',(20.6511283817414,9.90285032516693,0.));
#213152=CARTESIAN_POINT('Ctrl Pts',(20.6511283817414,9.90285032516693,12.));
#213153=CARTESIAN_POINT('Ctrl Pts',(20.6407075193976,9.8954014204912,0.));
#213154=CARTESIAN_POINT('Ctrl Pts',(20.6407075193976,9.8954014204912,12.));
#213155=CARTESIAN_POINT('Ctrl Pts',(20.6304074914087,9.88808932697306,0.));
#213156=CARTESIAN_POINT('Ctrl Pts',(20.6304074914087,9.88808932697306,12.));
#213157=CARTESIAN_POINT('Ctrl Pts',(20.6202308177474,9.88091464472676,0.));
#213158=CARTESIAN_POINT('Ctrl Pts',(20.6202308177474,9.88091464472676,12.));
#213159=CARTESIAN_POINT('Ctrl Pts',(20.6101800854494,9.87387798732956,0.));
#213160=CARTESIAN_POINT('Ctrl Pts',(20.6101800854494,9.87387798732956,12.));
#213161=CARTESIAN_POINT('Ctrl Pts',(20.6002579513699,9.86697998242623,0.));
#213162=CARTESIAN_POINT('Ctrl Pts',(20.6002579513699,9.86697998242623,12.));
#213163=CARTESIAN_POINT('Ctrl Pts',(20.5904671449754,9.86022127232748,0.));
#213164=CARTESIAN_POINT('Ctrl Pts',(20.5904671449754,9.86022127232748,12.));
#213165=CARTESIAN_POINT('Ctrl Pts',(20.5808104710015,9.85360251456981,0.));
#213166=CARTESIAN_POINT('Ctrl Pts',(20.5808104710015,9.85360251456981,12.));
#213167=CARTESIAN_POINT('Ctrl Pts',(20.5712908125139,9.84712438256278,0.));
#213168=CARTESIAN_POINT('Ctrl Pts',(20.5712908125139,9.84712438256278,12.));
#213169=CARTESIAN_POINT('Ctrl Pts',(20.5619111362402,9.84078756677565,0.));
#213170=CARTESIAN_POINT('Ctrl Pts',(20.5619111362402,9.84078756677565,12.));
#213171=CARTESIAN_POINT('Ctrl Pts',(20.552674497646,9.83459277585315,0.));
#213172=CARTESIAN_POINT('Ctrl Pts',(20.552674497646,9.83459277585315,12.));
#213173=CARTESIAN_POINT('Ctrl Pts',(20.5435840460721,9.82854073773878,0.));
#213174=CARTESIAN_POINT('Ctrl Pts',(20.5435840460721,9.82854073773878,12.));
#213175=CARTESIAN_POINT('Ctrl Pts',(20.5346430299517,9.82263220080363,0.));
#213176=CARTESIAN_POINT('Ctrl Pts',(20.5346430299517,9.82263220080363,12.));
#213177=CARTESIAN_POINT('Ctrl Pts',(20.5258548000629,9.81686793455943,0.));
#213178=CARTESIAN_POINT('Ctrl Pts',(20.5258548000629,9.81686793455943,12.));
#213179=CARTESIAN_POINT('Ctrl Pts',(20.517222812284,9.81124873025282,0.));
#213180=CARTESIAN_POINT('Ctrl Pts',(20.517222812284,9.81124873025282,12.));
#213181=CARTESIAN_POINT('Ctrl Pts',(20.5087506310505,9.80577540161088,0.));
#213182=CARTESIAN_POINT('Ctrl Pts',(20.5087506310505,9.80577540161088,12.));
#213183=CARTESIAN_POINT('Ctrl Pts',(20.5004419312107,9.80044878520949,0.));
#213184=CARTESIAN_POINT('Ctrl Pts',(20.5004419312107,9.80044878520949,12.));
#213185=CARTESIAN_POINT('Ctrl Pts',(20.4923005087943,9.79526974288331,0.));
#213186=CARTESIAN_POINT('Ctrl Pts',(20.4923005087943,9.79526974288331,12.));
#213187=CARTESIAN_POINT('Ctrl Pts',(20.4843302955329,9.79023916498656,0.));
#213188=CARTESIAN_POINT('Ctrl Pts',(20.4843302955329,9.79023916498656,12.));
#213189=CARTESIAN_POINT('Ctrl Pts',(20.4765353711586,9.78535797314167,0.));
#213190=CARTESIAN_POINT('Ctrl Pts',(20.4765353711586,9.78535797314167,12.));
#213191=CARTESIAN_POINT('Ctrl Pts',(20.4689199790669,9.78062712373321,0.));
#213192=CARTESIAN_POINT('Ctrl Pts',(20.4689199790669,9.78062712373321,12.));
#213193=CARTESIAN_POINT('Ctrl Pts',(20.4614885274975,9.77604760815529,0.));
#213194=CARTESIAN_POINT('Ctrl Pts',(20.4614885274975,9.77604760815529,12.));
#213195=CARTESIAN_POINT('Ctrl Pts',(20.4542455817527,9.7716204510407,0.));
#213196=CARTESIAN_POINT('Ctrl Pts',(20.4542455817527,9.7716204510407,12.));
#213197=CARTESIAN_POINT('Ctrl Pts',(20.447195862298,9.76734670980892,0.));
#213198=CARTESIAN_POINT('Ctrl Pts',(20.447195862298,9.76734670980892,12.));
#213199=CARTESIAN_POINT('Ctrl Pts',(20.44034423294,9.76322747195495,0.));
#213200=CARTESIAN_POINT('Ctrl Pts',(20.44034423294,9.76322747195495,12.));
#213201=CARTESIAN_POINT('Ctrl Pts',(20.4336957355473,9.75926386289923,0.));
#213202=CARTESIAN_POINT('Ctrl Pts',(20.4336957355473,9.75926386289923,12.));
#213203=CARTESIAN_POINT('Ctrl Pts',(20.4272556476629,9.75545705902418,0.));
#213204=CARTESIAN_POINT('Ctrl Pts',(20.4272556476629,9.75545705902418,12.));
#213205=CARTESIAN_POINT('Ctrl Pts',(20.4210295275817,9.7518082978643,0.));
#213206=CARTESIAN_POINT('Ctrl Pts',(20.4210295275817,9.7518082978643,12.));
#213207=CARTESIAN_POINT('Ctrl Pts',(20.4150232777393,9.74831889242174,0.));
#213208=CARTESIAN_POINT('Ctrl Pts',(20.4150232777393,9.74831889242174,12.));
#213209=CARTESIAN_POINT('Ctrl Pts',(20.4092430879861,9.74499021838538,0.));
#213210=CARTESIAN_POINT('Ctrl Pts',(20.4092430879861,9.74499021838538,12.));
#213211=CARTESIAN_POINT('Ctrl Pts',(20.4036953576549,9.74182369656272,0.));
#213212=CARTESIAN_POINT('Ctrl Pts',(20.4036953576549,9.74182369656272,12.));
#213213=CARTESIAN_POINT('Ctrl Pts',(20.3983866213331,9.73882077613201,0.));
#213214=CARTESIAN_POINT('Ctrl Pts',(20.3983866213331,9.73882077613201,12.));
#213215=CARTESIAN_POINT('Ctrl Pts',(20.3933234845647,9.73598292014243,0.));
#213216=CARTESIAN_POINT('Ctrl Pts',(20.3933234845647,9.73598292014243,12.));
#213217=CARTESIAN_POINT('Ctrl Pts',(20.3885129129912,9.73331167102808,0.));
#213218=CARTESIAN_POINT('Ctrl Pts',(20.3885129129912,9.73331167102808,12.));
#213219=CARTESIAN_POINT('Ctrl Pts',(20.3839624556742,9.73080870123727,0.));
#213220=CARTESIAN_POINT('Ctrl Pts',(20.3839624556742,9.73080870123727,12.));
#213221=CARTESIAN_POINT('Ctrl Pts',(20.3796805893304,9.72847589116542,0.));
#213222=CARTESIAN_POINT('Ctrl Pts',(20.3796805893304,9.72847589116542,12.));
#213223=CARTESIAN_POINT('Ctrl Pts',(20.3756766651951,9.72631531732881,0.));
#213224=CARTESIAN_POINT('Ctrl Pts',(20.3756766651951,9.72631531732881,12.));
#213225=CARTESIAN_POINT('Ctrl Pts',(20.371960235676,9.72432910043194,0.));
#213226=CARTESIAN_POINT('Ctrl Pts',(20.371960235676,9.72432910043194,12.));
#213227=CARTESIAN_POINT('Ctrl Pts',(20.3685406190576,9.7225193072249,0.));
#213228=CARTESIAN_POINT('Ctrl Pts',(20.3685406190576,9.7225193072249,12.));
#213229=CARTESIAN_POINT('Ctrl Pts',(20.3654261611056,9.72088778381081,0.));
#213230=CARTESIAN_POINT('Ctrl Pts',(20.3654261611056,9.72088778381081,12.));
#213231=CARTESIAN_POINT('Ctrl Pts',(20.3626256913981,9.71943648548099,0.));
#213232=CARTESIAN_POINT('Ctrl Pts',(20.3626256913981,9.71943648548099,12.));
#213233=CARTESIAN_POINT('Ctrl Pts',(20.3601498764344,9.71816778328007,0.));
#213234=CARTESIAN_POINT('Ctrl Pts',(20.3601498764344,9.71816778328007,12.));
#213235=CARTESIAN_POINT('Ctrl Pts',(20.3580133103356,9.71708493723096,0.));
#213236=CARTESIAN_POINT('Ctrl Pts',(20.3580133103356,9.71708493723096,12.));
#213237=CARTESIAN_POINT('Ctrl Pts',(20.3562337557875,9.71619192554186,0.));
#213238=CARTESIAN_POINT('Ctrl Pts',(20.3562337557875,9.71619192554186,12.));
#213239=CARTESIAN_POINT('Ctrl Pts',(20.3548282742361,9.71549257088173,0.));
#213240=CARTESIAN_POINT('Ctrl Pts',(20.3548282742361,9.71549257088173,12.));
#213241=CARTESIAN_POINT('Ctrl Pts',(20.3538098605706,9.71498978052021,0.));
#213242=CARTESIAN_POINT('Ctrl Pts',(20.3538098605706,9.71498978052021,12.));
#213243=CARTESIAN_POINT('Ctrl Pts',(20.3533097561886,9.71474590350681,0.));
#213244=CARTESIAN_POINT('Ctrl Pts',(20.3533097561886,9.71474590350681,12.));
#213245=CARTESIAN_POINT('Ctrl Pts',(20.3531126095522,9.71465227853042,0.));
#213246=CARTESIAN_POINT('Ctrl Pts',(20.3531126095522,9.71465227853042,12.));
#213247=CARTESIAN_POINT('Ctrl Pts',(20.353060251684,9.71462954053042,0.));
#213248=CARTESIAN_POINT('Ctrl Pts',(20.353060251684,9.71462954053042,12.));
#213249=CARTESIAN_POINT('Ctrl Pts',(20.353053841303,9.71462809124916,0.));
#213250=CARTESIAN_POINT('Ctrl Pts',(20.353053841303,9.71462809124916,12.));
#213251=CARTESIAN_POINT('',(22.8400320311648,12.4230808101438,0.));
#213252=CARTESIAN_POINT('Ctrl Pts',(22.8400320311648,12.4230808101438,0.));
#213253=CARTESIAN_POINT('Ctrl Pts',(22.8370364396459,12.418215285186,0.));
#213254=CARTESIAN_POINT('Ctrl Pts',(22.8310435872747,12.4084933766347,0.));
#213255=CARTESIAN_POINT('Ctrl Pts',(22.8220493007173,12.3939379378998,0.));
#213256=CARTESIAN_POINT('Ctrl Pts',(22.81004690224,12.374585536673,0.));
#213257=CARTESIAN_POINT('Ctrl Pts',(22.795027221673,12.3504864740319,0.));
#213258=CARTESIAN_POINT('Ctrl Pts',(22.7799908974768,12.3264788926075,0.));
#213259=CARTESIAN_POINT('Ctrl Pts',(22.764938010105,12.3025628601792,0.));
#213260=CARTESIAN_POINT('Ctrl Pts',(22.7498686970069,12.2787384750742,0.));
#213261=CARTESIAN_POINT('Ctrl Pts',(22.7347831655287,12.2550058702395,0.));
#213262=CARTESIAN_POINT('Ctrl Pts',(22.7196817119374,12.2313652198061,0.));
#213263=CARTESIAN_POINT('Ctrl Pts',(22.7045647168747,12.2078167360284,0.));
#213264=CARTESIAN_POINT('Ctrl Pts',(22.6894326205037,12.1843606579262,0.));
#213265=CARTESIAN_POINT('Ctrl Pts',(22.6742859034944,12.1609972423099,0.));
#213266=CARTESIAN_POINT('Ctrl Pts',(22.6591250653965,12.1377267537145,0.));
#213267=CARTESIAN_POINT('Ctrl Pts',(22.6439506046605,12.1145494550383,0.));
#213268=CARTESIAN_POINT('Ctrl Pts',(22.6287629967056,12.0914655972823,0.));
#213269=CARTESIAN_POINT('Ctrl Pts',(22.6135626764898,12.0684754113862,0.));
#213270=CARTESIAN_POINT('Ctrl Pts',(22.5983500505644,12.0455791139128,0.));
#213271=CARTESIAN_POINT('Ctrl Pts',(22.5831255061282,12.0227769113127,0.));
#213272=CARTESIAN_POINT('Ctrl Pts',(22.5678894211181,12.0000690046695,0.));
#213273=CARTESIAN_POINT('Ctrl Pts',(22.5526421741158,11.9774555943496,0.));
#213274=CARTESIAN_POINT('Ctrl Pts',(22.5373841537307,11.9549368843997,0.));
#213275=CARTESIAN_POINT('Ctrl Pts',(22.5221157697883,11.9325130877803,0.));
#213276=CARTESIAN_POINT('Ctrl Pts',(22.5068374513973,11.9101844254557,0.));
#213277=CARTESIAN_POINT('Ctrl Pts',(22.4915496418485,11.8879511239943,0.));
#213278=CARTESIAN_POINT('Ctrl Pts',(22.4762527946702,11.8658134137019,0.));
#213279=CARTESIAN_POINT('Ctrl Pts',(22.4609473690471,11.8437715264487,0.));
#213280=CARTESIAN_POINT('Ctrl Pts',(22.4456338258735,11.8218256937889,0.));
#213281=CARTESIAN_POINT('Ctrl Pts',(22.430312622646,11.7999761445173,0.));
#213282=CARTESIAN_POINT('Ctrl Pts',(22.4149842125008,11.7782231042039,0.));
#213283=CARTESIAN_POINT('Ctrl Pts',(22.3996490469191,11.7565667964764,0.));
#213284=CARTESIAN_POINT('Ctrl Pts',(22.3843075773899,11.7350074437961,0.));
#213285=CARTESIAN_POINT('Ctrl Pts',(22.3689602575491,11.7135452684532,0.));
#213286=CARTESIAN_POINT('Ctrl Pts',(22.3536075450029,11.6921804934056,0.));
#213287=CARTESIAN_POINT('Ctrl Pts',(22.3382499035619,11.6709133432985,0.));
#213288=CARTESIAN_POINT('Ctrl Pts',(22.3228878043976,11.6497440449857,0.));
#213289=CARTESIAN_POINT('Ctrl Pts',(22.3075217249049,11.6286728270009,0.));
#213290=CARTESIAN_POINT('Ctrl Pts',(22.2921521480356,11.6076999192357,0.));
#213291=CARTESIAN_POINT('Ctrl Pts',(22.2767795614348,11.5868255525188,0.));
#213292=CARTESIAN_POINT('Ctrl Pts',(22.2614044566898,11.5660499582403,0.));
#213293=CARTESIAN_POINT('Ctrl Pts',(22.2460273284654,11.5453733679121,0.));
#213294=CARTESIAN_POINT('Ctrl Pts',(22.2306486738901,11.5247960128477,0.));
#213295=CARTESIAN_POINT('Ctrl Pts',(22.2152689931022,11.5043181244242,0.));
#213296=CARTESIAN_POINT('Ctrl Pts',(22.1998887896436,11.483939934259,0.));
#213297=CARTESIAN_POINT('Ctrl Pts',(22.184508570917,11.463661674411,0.));
#213298=CARTESIAN_POINT('Ctrl Pts',(22.1691288486096,11.443483577557,0.));
#213299=CARTESIAN_POINT('Ctrl Pts',(22.1537501391487,11.4234058771742,0.));
#213300=CARTESIAN_POINT('Ctrl Pts',(22.1383729640964,11.4034288076908,0.));
#213301=CARTESIAN_POINT('Ctrl Pts',(22.1229978500186,11.3835526044256,0.));
#213302=CARTESIAN_POINT('Ctrl Pts',(22.1076253283979,11.3637775035367,0.));
#213303=CARTESIAN_POINT('Ctrl Pts',(22.0922559355294,11.3441037419553,0.));
#213304=CARTESIAN_POINT('Ctrl Pts',(22.0768902124267,11.3245315573168,0.));
#213305=CARTESIAN_POINT('Ctrl Pts',(22.0615287047179,11.3050611878771,0.));
#213306=CARTESIAN_POINT('Ctrl Pts',(22.046171962566,11.2856928724374,0.));
#213307=CARTESIAN_POINT('Ctrl Pts',(22.030820540835,11.2664268504206,0.));
#213308=CARTESIAN_POINT('Ctrl Pts',(22.0154749992363,11.2472633619275,0.));
#213309=CARTESIAN_POINT('Ctrl Pts',(22.0001359024839,11.2282026477896,0.));
#213310=CARTESIAN_POINT('Ctrl Pts',(21.9848038204439,11.2092449496125,0.));
#213311=CARTESIAN_POINT('Ctrl Pts',(21.9694793282914,11.190390509811,0.));
#213312=CARTESIAN_POINT('Ctrl Pts',(21.9541630066506,11.1716395716376,0.));
#213313=CARTESIAN_POINT('Ctrl Pts',(21.9388554416439,11.1529923792003,0.));
#213314=CARTESIAN_POINT('Ctrl Pts',(21.923557224952,11.1344491774741,0.));
#213315=CARTESIAN_POINT('Ctrl Pts',(21.9082689538688,11.1160102123024,0.));
#213316=CARTESIAN_POINT('Ctrl Pts',(21.8929912313608,11.0976757303944,0.));
#213317=CARTESIAN_POINT('Ctrl Pts',(21.877724666119,11.0794459793057,0.));
#213318=CARTESIAN_POINT('Ctrl Pts',(21.8624698726318,11.0613212074363,0.));
#213319=CARTESIAN_POINT('Ctrl Pts',(21.8472274713103,11.0433016640807,0.));
#213320=CARTESIAN_POINT('Ctrl Pts',(21.8319980886033,11.0253875994598,0.));
#213321=CARTESIAN_POINT('Ctrl Pts',(21.8167823571168,11.0075792647477,0.));
#213322=CARTESIAN_POINT('Ctrl Pts',(21.8015809157301,10.9898769120912,0.));
#213323=CARTESIAN_POINT('Ctrl Pts',(21.7863944097141,10.9722807946156,0.));
#213324=CARTESIAN_POINT('Ctrl Pts',(21.7712234908464,10.9547911664455,0.));
#213325=CARTESIAN_POINT('Ctrl Pts',(21.7560688175247,10.9374082827444,0.));
#213326=CARTESIAN_POINT('Ctrl Pts',(21.7409310548797,10.9201323997384,0.));
#213327=CARTESIAN_POINT('Ctrl Pts',(21.7258108748873,10.902963774734,0.));
#213328=CARTESIAN_POINT('Ctrl Pts',(21.7107089564825,10.8859026661293,0.));
#213329=CARTESIAN_POINT('Ctrl Pts',(21.6956259856672,10.8689493334095,0.));
#213330=CARTESIAN_POINT('Ctrl Pts',(21.6805626556467,10.8521040371835,0.));
#213331=CARTESIAN_POINT('Ctrl Pts',(21.6655196669732,10.8353670392272,0.));
#213332=CARTESIAN_POINT('Ctrl Pts',(21.6504977276866,10.8187386025136,0.));
#213333=CARTESIAN_POINT('Ctrl Pts',(21.6354975534557,10.8022189912369,0.));
#213334=CARTESIAN_POINT('Ctrl Pts',(21.6205198677173,10.7858084708261,0.));
#213335=CARTESIAN_POINT('Ctrl Pts',(21.6055654018176,10.7695073079552,0.));
#213336=CARTESIAN_POINT('Ctrl Pts',(21.5906348951743,10.7533157705941,0.));
#213337=CARTESIAN_POINT('Ctrl Pts',(21.5757290954371,10.7372341280467,0.));
#213338=CARTESIAN_POINT('Ctrl Pts',(21.5608487586468,10.7212626509816,0.));
#213339=CARTESIAN_POINT('Ctrl Pts',(21.5459946493955,10.7054016114571,0.));
#213340=CARTESIAN_POINT('Ctrl Pts',(21.5311675409807,10.689651282929,0.));
#213341=CARTESIAN_POINT('Ctrl Pts',(21.51636821558,10.6740119402834,0.));
#213342=CARTESIAN_POINT('Ctrl Pts',(21.5015974644449,10.6584838598939,0.));
#213343=CARTESIAN_POINT('Ctrl Pts',(21.4868560880889,10.6430673196607,0.));
#213344=CARTESIAN_POINT('Ctrl Pts',(21.4721448964766,10.6277625990456,0.));
#213345=CARTESIAN_POINT('Ctrl Pts',(21.4574647092097,10.6125699790961,0.));
#213346=CARTESIAN_POINT('Ctrl Pts',(21.4428163557144,10.5974897424622,0.));
#213347=CARTESIAN_POINT('Ctrl Pts',(21.4282006754631,10.5825221734573,0.));
#213348=CARTESIAN_POINT('Ctrl Pts',(21.4136185181979,10.5676675581108,0.));
#213349=CARTESIAN_POINT('Ctrl Pts',(21.3990707441497,10.5529261842108,0.));
#213350=CARTESIAN_POINT('Ctrl Pts',(21.3845582242602,10.5382983413421,0.));
#213351=CARTESIAN_POINT('Ctrl Pts',(21.3700818403936,10.5237843209057,0.));
#213352=CARTESIAN_POINT('Ctrl Pts',(21.3556424855814,10.5093844161685,0.));
#213353=CARTESIAN_POINT('Ctrl Pts',(21.3412410642904,10.4950989223337,0.));
#213354=CARTESIAN_POINT('Ctrl Pts',(21.3268784926819,10.4809281365931,0.));
#213355=CARTESIAN_POINT('Ctrl Pts',(21.3125556988731,10.4668723581768,0.));
#213356=CARTESIAN_POINT('Ctrl Pts',(21.2982736231931,10.4529318883874,0.));
#213357=CARTESIAN_POINT('Ctrl Pts',(21.2840332184483,10.4391070306391,0.));
#213358=CARTESIAN_POINT('Ctrl Pts',(21.2698354502403,10.42539809054,0.));
#213359=CARTESIAN_POINT('Ctrl Pts',(21.255681297275,10.4118053759588,0.));
#213360=CARTESIAN_POINT('Ctrl Pts',(21.2415717516714,10.3983291970846,0.));
#213361=CARTESIAN_POINT('Ctrl Pts',(21.22750781927,10.3849698664786,0.));
#213362=CARTESIAN_POINT('Ctrl Pts',(21.2134905199345,10.371727699113,0.));
#213363=CARTESIAN_POINT('Ctrl Pts',(21.199520887919,10.3586030124587,0.));
#213364=CARTESIAN_POINT('Ctrl Pts',(21.1855999722416,10.3455961265701,0.));
#213365=CARTESIAN_POINT('Ctrl Pts',(21.1717288370509,10.3327073641572,0.));
#213366=CARTESIAN_POINT('Ctrl Pts',(21.1579085619965,10.3199370506544,0.));
#213367=CARTESIAN_POINT('Ctrl Pts',(21.1441402425843,10.3072855142687,0.));
#213368=CARTESIAN_POINT('Ctrl Pts',(21.1304249906002,10.2947530860721,0.));
#213369=CARTESIAN_POINT('Ctrl Pts',(21.1167639345631,10.2823401001072,0.));
#213370=CARTESIAN_POINT('Ctrl Pts',(21.1031582201627,10.2700468934744,0.));
#213371=CARTESIAN_POINT('Ctrl Pts',(21.0896090107063,10.2578738064181,0.));
#213372=CARTESIAN_POINT('Ctrl Pts',(21.0761174875444,10.2458211823912,0.));
#213373=CARTESIAN_POINT('Ctrl Pts',(21.0626848505663,10.2338893681567,0.));
#213374=CARTESIAN_POINT('Ctrl Pts',(21.0493123187483,10.2220787139155,0.));
#213375=CARTESIAN_POINT('Ctrl Pts',(21.0360011306815,10.2103895734123,0.));
#213376=CARTESIAN_POINT('Ctrl Pts',(21.0227525451107,10.1988223040425,0.));
#213377=CARTESIAN_POINT('Ctrl Pts',(21.0095678414486,10.187377266936,0.));
#213378=CARTESIAN_POINT('Ctrl Pts',(20.9964483203686,10.1760548270767,0.));
#213379=CARTESIAN_POINT('Ctrl Pts',(20.9833953044736,10.1648553534568,0.));
#213380=CARTESIAN_POINT('Ctrl Pts',(20.9704101389369,10.1537792192065,0.));
#213381=CARTESIAN_POINT('Ctrl Pts',(20.9574941921591,10.1428268017256,0.));
#213382=CARTESIAN_POINT('Ctrl Pts',(20.9446488563933,10.1319984827908,0.));
#213383=CARTESIAN_POINT('Ctrl Pts',(20.9318755484734,10.1212946487057,0.));
#213384=CARTESIAN_POINT('Ctrl Pts',(20.919175710627,10.1107156904836,0.));
#213385=CARTESIAN_POINT('Ctrl Pts',(20.9065508112557,10.1002620040076,0.));
#213386=CARTESIAN_POINT('Ctrl Pts',(20.894002345737,10.0899339901916,0.));
#213387=CARTESIAN_POINT('Ctrl Pts',(20.881531837184,10.0797320551154,0.));
#213388=CARTESIAN_POINT('Ctrl Pts',(20.86914083737,10.0696566102218,0.));
#213389=CARTESIAN_POINT('Ctrl Pts',(20.8568309277316,10.0597080725375,0.));
#213390=CARTESIAN_POINT('Ctrl Pts',(20.8446037203402,10.0498868648733,0.));
#213391=CARTESIAN_POINT('Ctrl Pts',(20.8324608588909,10.0401934160234,0.));
#213392=CARTESIAN_POINT('Ctrl Pts',(20.8204040196602,10.0306281609435,0.));
#213393=CARTESIAN_POINT('Ctrl Pts',(20.8084349126888,10.0211915410095,0.));
#213394=CARTESIAN_POINT('Ctrl Pts',(20.7965552829908,10.0118840042786,0.));
#213395=CARTESIAN_POINT('Ctrl Pts',(20.7847669117568,10.0027060057389,0.));
#213396=CARTESIAN_POINT('Ctrl Pts',(20.7730716175417,9.9936580075464,0.));
#213397=CARTESIAN_POINT('Ctrl Pts',(20.761471257499,9.98474047926853,0.));
#213398=CARTESIAN_POINT('Ctrl Pts',(20.7499677289627,9.9759538982347,0.));
#213399=CARTESIAN_POINT('Ctrl Pts',(20.7385629709795,9.96729874986202,0.));
#213400=CARTESIAN_POINT('Ctrl Pts',(20.7272589658751,9.95877552798398,0.));
#213401=CARTESIAN_POINT('Ctrl Pts',(20.7160577407579,9.95038473514949,0.));
#213402=CARTESIAN_POINT('Ctrl Pts',(20.7049613692234,9.94212688298236,0.));
#213403=CARTESIAN_POINT('Ctrl Pts',(20.6939719732484,9.9340024925973,0.));
#213404=CARTESIAN_POINT('Ctrl Pts',(20.6830917250255,9.92601209498749,0.));
#213405=CARTESIAN_POINT('Ctrl Pts',(20.6723228488263,9.91815623141289,0.));
#213406=CARTESIAN_POINT('Ctrl Pts',(20.6616676228315,9.91043545377008,0.));
#213407=CARTESIAN_POINT('Ctrl Pts',(20.6511283817414,9.90285032516693,0.));
#213408=CARTESIAN_POINT('Ctrl Pts',(20.6407075193976,9.8954014204912,0.));
#213409=CARTESIAN_POINT('Ctrl Pts',(20.6304074914087,9.88808932697306,0.));
#213410=CARTESIAN_POINT('Ctrl Pts',(20.6202308177474,9.88091464472676,0.));
#213411=CARTESIAN_POINT('Ctrl Pts',(20.6101800854494,9.87387798732956,0.));
#213412=CARTESIAN_POINT('Ctrl Pts',(20.6002579513699,9.86697998242623,0.));
#213413=CARTESIAN_POINT('Ctrl Pts',(20.5904671449754,9.86022127232748,0.));
#213414=CARTESIAN_POINT('Ctrl Pts',(20.5808104710015,9.85360251456981,0.));
#213415=CARTESIAN_POINT('Ctrl Pts',(20.5712908125139,9.84712438256278,0.));
#213416=CARTESIAN_POINT('Ctrl Pts',(20.5619111362402,9.84078756677565,0.));
#213417=CARTESIAN_POINT('Ctrl Pts',(20.552674497646,9.83459277585315,0.));
#213418=CARTESIAN_POINT('Ctrl Pts',(20.5435840460721,9.82854073773878,0.));
#213419=CARTESIAN_POINT('Ctrl Pts',(20.5346430299517,9.82263220080363,0.));
#213420=CARTESIAN_POINT('Ctrl Pts',(20.5258548000629,9.81686793455943,0.));
#213421=CARTESIAN_POINT('Ctrl Pts',(20.517222812284,9.81124873025282,0.));
#213422=CARTESIAN_POINT('Ctrl Pts',(20.5087506310505,9.80577540161088,0.));
#213423=CARTESIAN_POINT('Ctrl Pts',(20.5004419312107,9.80044878520949,0.));
#213424=CARTESIAN_POINT('Ctrl Pts',(20.4923005087943,9.79526974288331,0.));
#213425=CARTESIAN_POINT('Ctrl Pts',(20.4843302955329,9.79023916498656,0.));
#213426=CARTESIAN_POINT('Ctrl Pts',(20.4765353711586,9.78535797314167,0.));
#213427=CARTESIAN_POINT('Ctrl Pts',(20.4689199790669,9.78062712373321,0.));
#213428=CARTESIAN_POINT('Ctrl Pts',(20.4614885274975,9.77604760815529,0.));
#213429=CARTESIAN_POINT('Ctrl Pts',(20.4542455817527,9.7716204510407,0.));
#213430=CARTESIAN_POINT('Ctrl Pts',(20.447195862298,9.76734670980892,0.));
#213431=CARTESIAN_POINT('Ctrl Pts',(20.44034423294,9.76322747195495,0.));
#213432=CARTESIAN_POINT('Ctrl Pts',(20.4336957355473,9.75926386289923,0.));
#213433=CARTESIAN_POINT('Ctrl Pts',(20.4272556476629,9.75545705902418,0.));
#213434=CARTESIAN_POINT('Ctrl Pts',(20.4210295275817,9.7518082978643,0.));
#213435=CARTESIAN_POINT('Ctrl Pts',(20.4150232777393,9.74831889242174,0.));
#213436=CARTESIAN_POINT('Ctrl Pts',(20.4092430879861,9.74499021838538,0.));
#213437=CARTESIAN_POINT('Ctrl Pts',(20.4036953576549,9.74182369656272,0.));
#213438=CARTESIAN_POINT('Ctrl Pts',(20.3983866213331,9.73882077613201,0.));
#213439=CARTESIAN_POINT('Ctrl Pts',(20.3933234845647,9.73598292014243,0.));
#213440=CARTESIAN_POINT('Ctrl Pts',(20.3885129129912,9.73331167102808,0.));
#213441=CARTESIAN_POINT('Ctrl Pts',(20.3839624556742,9.73080870123727,0.));
#213442=CARTESIAN_POINT('Ctrl Pts',(20.3796805893304,9.72847589116542,0.));
#213443=CARTESIAN_POINT('Ctrl Pts',(20.3756766651951,9.72631531732881,0.));
#213444=CARTESIAN_POINT('Ctrl Pts',(20.371960235676,9.72432910043194,0.));
#213445=CARTESIAN_POINT('Ctrl Pts',(20.3685406190576,9.7225193072249,0.));
#213446=CARTESIAN_POINT('Ctrl Pts',(20.3654261611056,9.72088778381081,0.));
#213447=CARTESIAN_POINT('Ctrl Pts',(20.3626256913981,9.71943648548099,0.));
#213448=CARTESIAN_POINT('Ctrl Pts',(20.3601498764344,9.71816778328007,0.));
#213449=CARTESIAN_POINT('Ctrl Pts',(20.3580133103356,9.71708493723096,0.));
#213450=CARTESIAN_POINT('Ctrl Pts',(20.3562337557875,9.71619192554186,0.));
#213451=CARTESIAN_POINT('Ctrl Pts',(20.3548282742361,9.71549257088173,0.));
#213452=CARTESIAN_POINT('Ctrl Pts',(20.3538098605706,9.71498978052021,0.));
#213453=CARTESIAN_POINT('Ctrl Pts',(20.3533097561886,9.71474590350681,0.));
#213454=CARTESIAN_POINT('Ctrl Pts',(20.3531126095522,9.71465227853042,0.));
#213455=CARTESIAN_POINT('Ctrl Pts',(20.353060251684,9.71462954053042,0.));
#213456=CARTESIAN_POINT('Ctrl Pts',(20.353053841303,9.71462809124916,0.));
#213457=CARTESIAN_POINT('',(22.8400320311648,12.4230808101438,0.));
#213458=CARTESIAN_POINT('Ctrl Pts',(21.2610617890679,7.52250298901264,0.));
#213459=CARTESIAN_POINT('Ctrl Pts',(21.2610617890679,7.52250298901264,12.));
#213460=CARTESIAN_POINT('Ctrl Pts',(21.2610673466886,7.5225064970397,0.));
#213461=CARTESIAN_POINT('Ctrl Pts',(21.2610673466886,7.5225064970397,12.));
#213462=CARTESIAN_POINT('Ctrl Pts',(21.2611204474866,7.52252744144904,0.));
#213463=CARTESIAN_POINT('Ctrl Pts',(21.2611204474866,7.52252744144904,12.));
#213464=CARTESIAN_POINT('Ctrl Pts',(21.261326054066,7.52260064231661,0.));
#213465=CARTESIAN_POINT('Ctrl Pts',(21.261326054066,7.52260064231661,12.));
#213466=CARTESIAN_POINT('Ctrl Pts',(21.2618521283555,7.5227818224267,0.));
#213467=CARTESIAN_POINT('Ctrl Pts',(21.2618521283555,7.5227818224267,12.));
#213468=CARTESIAN_POINT('Ctrl Pts',(21.262927782038,7.52314642316199,0.));
#213469=CARTESIAN_POINT('Ctrl Pts',(21.262927782038,7.52314642316199,12.));
#213470=CARTESIAN_POINT('Ctrl Pts',(21.2644161259962,7.52364573027553,0.));
#213471=CARTESIAN_POINT('Ctrl Pts',(21.2644161259962,7.52364573027553,12.));
#213472=CARTESIAN_POINT('Ctrl Pts',(21.2663059157058,7.52427261074298,0.));
#213473=CARTESIAN_POINT('Ctrl Pts',(21.2663059157058,7.52427261074298,12.));
#213474=CARTESIAN_POINT('Ctrl Pts',(21.2685823838671,7.52501770333531,0.));
#213475=CARTESIAN_POINT('Ctrl Pts',(21.2685823838671,7.52501770333531,12.));
#213476=CARTESIAN_POINT('Ctrl Pts',(21.2712301573466,7.5258712609553,0.));
#213477=CARTESIAN_POINT('Ctrl Pts',(21.2712301573466,7.5258712609553,12.));
#213478=CARTESIAN_POINT('Ctrl Pts',(21.2742366113579,7.52682526918541,0.));
#213479=CARTESIAN_POINT('Ctrl Pts',(21.2742366113579,7.52682526918541,12.));
#213480=CARTESIAN_POINT('Ctrl Pts',(21.2775925269652,7.52787386225333,0.));
#213481=CARTESIAN_POINT('Ctrl Pts',(21.2775925269652,7.52787386225333,12.));
#213482=CARTESIAN_POINT('Ctrl Pts',(21.2812902781143,7.52901217930408,0.));
#213483=CARTESIAN_POINT('Ctrl Pts',(21.2812902781143,7.52901217930408,12.));
#213484=CARTESIAN_POINT('Ctrl Pts',(21.2853226580657,7.5302356243823,0.));
#213485=CARTESIAN_POINT('Ctrl Pts',(21.2853226580657,7.5302356243823,12.));
#213486=CARTESIAN_POINT('Ctrl Pts',(21.2896816163842,7.53153906987856,0.));
#213487=CARTESIAN_POINT('Ctrl Pts',(21.2896816163842,7.53153906987856,12.));
#213488=CARTESIAN_POINT('Ctrl Pts',(21.2943588989331,7.53291726078527,0.));
#213489=CARTESIAN_POINT('Ctrl Pts',(21.2943588989331,7.53291726078527,12.));
#213490=CARTESIAN_POINT('Ctrl Pts',(21.2993464250717,7.53436505309943,0.));
#213491=CARTESIAN_POINT('Ctrl Pts',(21.2993464250717,7.53436505309943,12.));
#213492=CARTESIAN_POINT('Ctrl Pts',(21.3046368712157,7.53587778251736,0.));
#213493=CARTESIAN_POINT('Ctrl Pts',(21.3046368712157,7.53587778251736,12.));
#213494=CARTESIAN_POINT('Ctrl Pts',(21.310223716773,7.53745129364616,0.));
#213495=CARTESIAN_POINT('Ctrl Pts',(21.310223716773,7.53745129364616,12.));
#213496=CARTESIAN_POINT('Ctrl Pts',(21.3161009456256,7.53908175169899,0.));
#213497=CARTESIAN_POINT('Ctrl Pts',(21.3161009456256,7.53908175169899,12.));
#213498=CARTESIAN_POINT('Ctrl Pts',(21.3222628524165,7.54076552038279,0.));
#213499=CARTESIAN_POINT('Ctrl Pts',(21.3222628524165,7.54076552038279,12.));
#213500=CARTESIAN_POINT('Ctrl Pts',(21.328703791771,7.54249900377031,0.));
#213501=CARTESIAN_POINT('Ctrl Pts',(21.328703791771,7.54249900377031,12.));
#213502=CARTESIAN_POINT('Ctrl Pts',(21.3354182340149,7.54427868151268,0.));
#213503=CARTESIAN_POINT('Ctrl Pts',(21.3354182340149,7.54427868151268,12.));
#213504=CARTESIAN_POINT('Ctrl Pts',(21.3424008295038,7.54610114948347,0.));
#213505=CARTESIAN_POINT('Ctrl Pts',(21.3424008295038,7.54610114948347,12.));
#213506=CARTESIAN_POINT('Ctrl Pts',(21.3496464761531,7.54796316246331,0.));
#213507=CARTESIAN_POINT('Ctrl Pts',(21.3496464761531,7.54796316246331,12.));
#213508=CARTESIAN_POINT('Ctrl Pts',(21.3571503685855,7.5498616652131,0.));
#213509=CARTESIAN_POINT('Ctrl Pts',(21.3571503685855,7.5498616652131,12.));
#213510=CARTESIAN_POINT('Ctrl Pts',(21.3649079431865,7.55179375777444,0.));
#213511=CARTESIAN_POINT('Ctrl Pts',(21.3649079431865,7.55179375777444,12.));
#213512=CARTESIAN_POINT('Ctrl Pts',(21.3729148390243,7.55375667080029,0.));
#213513=CARTESIAN_POINT('Ctrl Pts',(21.3729148390243,7.55375667080029,12.));
#213514=CARTESIAN_POINT('Ctrl Pts',(21.3811668478932,7.55574773403503,0.));
#213515=CARTESIAN_POINT('Ctrl Pts',(21.3811668478932,7.55574773403503,12.));
#213516=CARTESIAN_POINT('Ctrl Pts',(21.3896598842117,7.55776435731417,0.));
#213517=CARTESIAN_POINT('Ctrl Pts',(21.3896598842117,7.55776435731417,12.));
#213518=CARTESIAN_POINT('Ctrl Pts',(21.3983899952987,7.55980403700611,0.));
#213519=CARTESIAN_POINT('Ctrl Pts',(21.3983899952987,7.55980403700611,12.));
#213520=CARTESIAN_POINT('Ctrl Pts',(21.4073533630365,7.56186435703622,0.));
#213521=CARTESIAN_POINT('Ctrl Pts',(21.4073533630365,7.56186435703622,12.));
#213522=CARTESIAN_POINT('Ctrl Pts',(21.4165463106254,7.56394299313685,0.));
#213523=CARTESIAN_POINT('Ctrl Pts',(21.4165463106254,7.56394299313685,12.));
#213524=CARTESIAN_POINT('Ctrl Pts',(21.4259653015736,7.56603771218712,0.));
#213525=CARTESIAN_POINT('Ctrl Pts',(21.4259653015736,7.56603771218712,12.));
#213526=CARTESIAN_POINT('Ctrl Pts',(21.4356069261513,7.56814636360848,0.));
#213527=CARTESIAN_POINT('Ctrl Pts',(21.4356069261513,7.56814636360848,12.));
#213528=CARTESIAN_POINT('Ctrl Pts',(21.4454678907509,7.57026687261166,0.));
#213529=CARTESIAN_POINT('Ctrl Pts',(21.4454678907509,7.57026687261166,12.));
#213530=CARTESIAN_POINT('Ctrl Pts',(21.4555450053142,7.57239723223506,0.));
#213531=CARTESIAN_POINT('Ctrl Pts',(21.4555450053142,7.57239723223506,12.));
#213532=CARTESIAN_POINT('Ctrl Pts',(21.4658351740128,7.57453549743412,0.));
#213533=CARTESIAN_POINT('Ctrl Pts',(21.4658351740128,7.57453549743412,12.));
#213534=CARTESIAN_POINT('Ctrl Pts',(21.4763353936762,7.57667978402987,0.));
#213535=CARTESIAN_POINT('Ctrl Pts',(21.4763353936762,7.57667978402987,12.));
#213536=CARTESIAN_POINT('Ctrl Pts',(21.4870427508194,7.57882826679132,0.));
#213537=CARTESIAN_POINT('Ctrl Pts',(21.4870427508194,7.57882826679132,12.));
#213538=CARTESIAN_POINT('Ctrl Pts',(21.4979544192744,7.58097917790744,0.));
#213539=CARTESIAN_POINT('Ctrl Pts',(21.4979544192744,7.58097917790744,12.));
#213540=CARTESIAN_POINT('Ctrl Pts',(21.5090676573873,7.5831308051918,0.));
#213541=CARTESIAN_POINT('Ctrl Pts',(21.5090676573873,7.5831308051918,12.));
#213542=CARTESIAN_POINT('Ctrl Pts',(21.5203798035299,7.5852814891913,0.));
#213543=CARTESIAN_POINT('Ctrl Pts',(21.5203798035299,7.5852814891913,12.));
#213544=CARTESIAN_POINT('Ctrl Pts',(21.5318882716736,7.58742962034834,0.));
#213545=CARTESIAN_POINT('Ctrl Pts',(21.5318882716736,7.58742962034834,12.));
#213546=CARTESIAN_POINT('Ctrl Pts',(21.543590547011,7.58957363620014,0.));
#213547=CARTESIAN_POINT('Ctrl Pts',(21.543590547011,7.58957363620014,12.));
#213548=CARTESIAN_POINT('Ctrl Pts',(21.5554841813462,7.59171201844777,0.));
#213549=CARTESIAN_POINT('Ctrl Pts',(21.5554841813462,7.59171201844777,12.));
#213550=CARTESIAN_POINT('Ctrl Pts',(21.5675667904726,7.59384329124918,0.));
#213551=CARTESIAN_POINT('Ctrl Pts',(21.5675667904726,7.59384329124918,12.));
#213552=CARTESIAN_POINT('Ctrl Pts',(21.5798360518978,7.59596601973584,0.));
#213553=CARTESIAN_POINT('Ctrl Pts',(21.5798360518978,7.59596601973584,12.));
#213554=CARTESIAN_POINT('Ctrl Pts',(21.5922897024466,7.59807880846195,0.));
#213555=CARTESIAN_POINT('Ctrl Pts',(21.5922897024466,7.59807880846195,12.));
#213556=CARTESIAN_POINT('Ctrl Pts',(21.6049255358843,7.60018029988241,0.));
#213557=CARTESIAN_POINT('Ctrl Pts',(21.6049255358843,7.60018029988241,12.));
#213558=CARTESIAN_POINT('Ctrl Pts',(21.617741400599,7.60226917285429,0.));
#213559=CARTESIAN_POINT('Ctrl Pts',(21.617741400599,7.60226917285429,12.));
#213560=CARTESIAN_POINT('Ctrl Pts',(21.6307351973822,7.60434414118296,0.));
#213561=CARTESIAN_POINT('Ctrl Pts',(21.6307351973822,7.60434414118296,12.));
#213562=CARTESIAN_POINT('Ctrl Pts',(21.6439048771743,7.60640395216357,0.));
#213563=CARTESIAN_POINT('Ctrl Pts',(21.6439048771743,7.60640395216357,12.));
#213564=CARTESIAN_POINT('Ctrl Pts',(21.6572484388081,7.60844738512874,0.));
#213565=CARTESIAN_POINT('Ctrl Pts',(21.6572484388081,7.60844738512874,12.));
#213566=CARTESIAN_POINT('Ctrl Pts',(21.6707639267576,7.61047325000956,0.));
#213567=CARTESIAN_POINT('Ctrl Pts',(21.6707639267576,7.61047325000956,12.));
#213568=CARTESIAN_POINT('Ctrl Pts',(21.6844494295815,7.61248038630269,0.));
#213569=CARTESIAN_POINT('Ctrl Pts',(21.6844494295815,7.61248038630269,12.));
#213570=CARTESIAN_POINT('Ctrl Pts',(21.6983030783322,7.61446766202787,0.));
#213571=CARTESIAN_POINT('Ctrl Pts',(21.6983030783322,7.61446766202787,12.));
#213572=CARTESIAN_POINT('Ctrl Pts',(21.7123230449834,7.61643397270421,0.));
#213573=CARTESIAN_POINT('Ctrl Pts',(21.7123230449834,7.61643397270421,12.));
#213574=CARTESIAN_POINT('Ctrl Pts',(21.7265075407975,7.61837824030538,0.));
#213575=CARTESIAN_POINT('Ctrl Pts',(21.7265075407975,7.61837824030538,12.));
#213576=CARTESIAN_POINT('Ctrl Pts',(21.7408548148656,7.62029941230855,0.));
#213577=CARTESIAN_POINT('Ctrl Pts',(21.7408548148656,7.62029941230855,12.));
#213578=CARTESIAN_POINT('Ctrl Pts',(21.7553631528328,7.62219646084229,0.));
#213579=CARTESIAN_POINT('Ctrl Pts',(21.7553631528328,7.62219646084229,12.));
#213580=CARTESIAN_POINT('Ctrl Pts',(21.7700308755584,7.62406838181166,0.));
#213581=CARTESIAN_POINT('Ctrl Pts',(21.7700308755584,7.62406838181166,12.));
#213582=CARTESIAN_POINT('Ctrl Pts',(21.7848563378021,7.62591419404513,0.));
#213583=CARTESIAN_POINT('Ctrl Pts',(21.7848563378021,7.62591419404513,12.));
#213584=CARTESIAN_POINT('Ctrl Pts',(21.799837926858,7.62773293842389,0.));
#213585=CARTESIAN_POINT('Ctrl Pts',(21.799837926858,7.62773293842389,12.));
#213586=CARTESIAN_POINT('Ctrl Pts',(21.814974061509,7.62952367718127,0.));
#213587=CARTESIAN_POINT('Ctrl Pts',(21.814974061509,7.62952367718127,12.));
#213588=CARTESIAN_POINT('Ctrl Pts',(21.8302631910195,7.63128549323023,0.));
#213589=CARTESIAN_POINT('Ctrl Pts',(21.8302631910195,7.63128549323023,12.));
#213590=CARTESIAN_POINT('Ctrl Pts',(21.8457037941084,7.63301748948936,0.));
#213591=CARTESIAN_POINT('Ctrl Pts',(21.8457037941084,7.63301748948936,12.));
#213592=CARTESIAN_POINT('Ctrl Pts',(21.8612943779089,7.63471878821226,0.));
#213593=CARTESIAN_POINT('Ctrl Pts',(21.8612943779089,7.63471878821226,12.));
#213594=CARTESIAN_POINT('Ctrl Pts',(21.8770334769496,7.636388530334,0.));
#213595=CARTESIAN_POINT('Ctrl Pts',(21.8770334769496,7.636388530334,12.));
#213596=CARTESIAN_POINT('Ctrl Pts',(21.8929196523514,7.63802587492035,0.));
#213597=CARTESIAN_POINT('Ctrl Pts',(21.8929196523514,7.63802587492035,12.));
#213598=CARTESIAN_POINT('Ctrl Pts',(21.9089514909874,7.63962999860927,0.));
#213599=CARTESIAN_POINT('Ctrl Pts',(21.9089514909874,7.63962999860927,12.));
#213600=CARTESIAN_POINT('Ctrl Pts',(21.9251276046545,7.64120009506532,0.));
#213601=CARTESIAN_POINT('Ctrl Pts',(21.9251276046545,7.64120009506532,12.));
#213602=CARTESIAN_POINT('Ctrl Pts',(21.9414466292072,7.64273537442682,0.));
#213603=CARTESIAN_POINT('Ctrl Pts',(21.9414466292072,7.64273537442682,12.));
#213604=CARTESIAN_POINT('Ctrl Pts',(21.9579072237651,7.64423506279123,0.));
#213605=CARTESIAN_POINT('Ctrl Pts',(21.9579072237651,7.64423506279123,12.));
#213606=CARTESIAN_POINT('Ctrl Pts',(21.9745080700798,7.64569840177336,0.));
#213607=CARTESIAN_POINT('Ctrl Pts',(21.9745080700798,7.64569840177336,12.));
#213608=CARTESIAN_POINT('Ctrl Pts',(21.9912478718542,7.6471246480525,0.));
#213609=CARTESIAN_POINT('Ctrl Pts',(21.9912478718542,7.6471246480525,12.));
#213610=CARTESIAN_POINT('Ctrl Pts',(22.0081253540774,7.64851307293352,0.));
#213611=CARTESIAN_POINT('Ctrl Pts',(22.0081253540774,7.64851307293352,12.));
#213612=CARTESIAN_POINT('Ctrl Pts',(22.0251392623209,7.64986296190169,0.));
#213613=CARTESIAN_POINT('Ctrl Pts',(22.0251392623209,7.64986296190169,12.));
#213614=CARTESIAN_POINT('Ctrl Pts',(22.0422883621174,7.65117361421359,0.));
#213615=CARTESIAN_POINT('Ctrl Pts',(22.0422883621174,7.65117361421359,12.));
#213616=CARTESIAN_POINT('Ctrl Pts',(22.0595714384431,7.65244434253113,0.));
#213617=CARTESIAN_POINT('Ctrl Pts',(22.0595714384431,7.65244434253113,12.));
#213618=CARTESIAN_POINT('Ctrl Pts',(22.0769872951596,7.65367447254949,0.));
#213619=CARTESIAN_POINT('Ctrl Pts',(22.0769872951596,7.65367447254949,12.));
#213620=CARTESIAN_POINT('Ctrl Pts',(22.094534754469,7.65486334263644,0.));
#213621=CARTESIAN_POINT('Ctrl Pts',(22.094534754469,7.65486334263644,12.));
#213622=CARTESIAN_POINT('Ctrl Pts',(22.1122126563329,7.65601030346807,0.));
#213623=CARTESIAN_POINT('Ctrl Pts',(22.1122126563329,7.65601030346807,12.));
#213624=CARTESIAN_POINT('Ctrl Pts',(22.1300198579675,7.65711471769397,0.));
#213625=CARTESIAN_POINT('Ctrl Pts',(22.1300198579675,7.65711471769397,12.));
#213626=CARTESIAN_POINT('Ctrl Pts',(22.1479552334211,7.65817595963349,0.));
#213627=CARTESIAN_POINT('Ctrl Pts',(22.1479552334211,7.65817595963349,12.));
#213628=CARTESIAN_POINT('Ctrl Pts',(22.1660176731178,7.65919341496931,0.));
#213629=CARTESIAN_POINT('Ctrl Pts',(22.1660176731178,7.65919341496931,12.));
#213630=CARTESIAN_POINT('Ctrl Pts',(22.1842060834091,7.66016648045005,0.));
#213631=CARTESIAN_POINT('Ctrl Pts',(22.1842060834091,7.66016648045005,12.));
#213632=CARTESIAN_POINT('Ctrl Pts',(22.2025193860964,7.66109456359271,0.));
#213633=CARTESIAN_POINT('Ctrl Pts',(22.2025193860964,7.66109456359271,12.));
#213634=CARTESIAN_POINT('Ctrl Pts',(22.2209565180085,7.661977082404,0.));
#213635=CARTESIAN_POINT('Ctrl Pts',(22.2209565180085,7.661977082404,12.));
#213636=CARTESIAN_POINT('Ctrl Pts',(22.2395164306547,7.66281346512509,0.));
#213637=CARTESIAN_POINT('Ctrl Pts',(22.2395164306547,7.66281346512509,12.));
#213638=CARTESIAN_POINT('Ctrl Pts',(22.258198089848,7.66360314997641,0.));
#213639=CARTESIAN_POINT('Ctrl Pts',(22.258198089848,7.66360314997641,12.));
#213640=CARTESIAN_POINT('Ctrl Pts',(22.2770004753335,7.66434558490979,0.));
#213641=CARTESIAN_POINT('Ctrl Pts',(22.2770004753335,7.66434558490979,12.));
#213642=CARTESIAN_POINT('Ctrl Pts',(22.2959225803937,7.66504022736299,0.));
#213643=CARTESIAN_POINT('Ctrl Pts',(22.2959225803937,7.66504022736299,12.));
#213644=CARTESIAN_POINT('Ctrl Pts',(22.314963411484,7.66568654402494,0.));
#213645=CARTESIAN_POINT('Ctrl Pts',(22.314963411484,7.66568654402494,12.));
#213646=CARTESIAN_POINT('Ctrl Pts',(22.3341219879469,7.66628401061952,0.));
#213647=CARTESIAN_POINT('Ctrl Pts',(22.3341219879469,7.66628401061952,12.));
#213648=CARTESIAN_POINT('Ctrl Pts',(22.3533973417021,7.66683211169159,0.));
#213649=CARTESIAN_POINT('Ctrl Pts',(22.3533973417021,7.66683211169159,12.));
#213650=CARTESIAN_POINT('Ctrl Pts',(22.372788516936,7.66733034039883,0.));
#213651=CARTESIAN_POINT('Ctrl Pts',(22.372788516936,7.66733034039883,12.));
#213652=CARTESIAN_POINT('Ctrl Pts',(22.3922945697773,7.6677781983079,0.));
#213653=CARTESIAN_POINT('Ctrl Pts',(22.3922945697773,7.6677781983079,12.));
#213654=CARTESIAN_POINT('Ctrl Pts',(22.4119145679758,7.6681751951964,0.));
#213655=CARTESIAN_POINT('Ctrl Pts',(22.4119145679758,7.6681751951964,12.));
#213656=CARTESIAN_POINT('Ctrl Pts',(22.4316475906603,7.66852084886704,0.));
#213657=CARTESIAN_POINT('Ctrl Pts',(22.4316475906603,7.66852084886704,12.));
#213658=CARTESIAN_POINT('Ctrl Pts',(22.4514927280855,7.66881468496635,0.));
#213659=CARTESIAN_POINT('Ctrl Pts',(22.4514927280855,7.66881468496635,12.));
#213660=CARTESIAN_POINT('Ctrl Pts',(22.4714490813699,7.66905623680831,0.));
#213661=CARTESIAN_POINT('Ctrl Pts',(22.4714490813699,7.66905623680831,12.));
#213662=CARTESIAN_POINT('Ctrl Pts',(22.4915157622312,7.66924504520315,0.));
#213663=CARTESIAN_POINT('Ctrl Pts',(22.4915157622312,7.66924504520315,12.));
#213664=CARTESIAN_POINT('Ctrl Pts',(22.5116918927031,7.66938065829108,0.));
#213665=CARTESIAN_POINT('Ctrl Pts',(22.5116918927031,7.66938065829108,12.));
#213666=CARTESIAN_POINT('Ctrl Pts',(22.53197660492,7.66946263138144,0.));
#213667=CARTESIAN_POINT('Ctrl Pts',(22.53197660492,7.66946263138144,12.));
#213668=CARTESIAN_POINT('Ctrl Pts',(22.5523690409116,7.66949052679693,0.));
#213669=CARTESIAN_POINT('Ctrl Pts',(22.5523690409116,7.66949052679693,12.));
#213670=CARTESIAN_POINT('Ctrl Pts',(22.5728683523831,7.66946391372306,0.));
#213671=CARTESIAN_POINT('Ctrl Pts',(22.5728683523831,7.66946391372306,12.));
#213672=CARTESIAN_POINT('Ctrl Pts',(22.5934737004953,7.66938236806233,0.));
#213673=CARTESIAN_POINT('Ctrl Pts',(22.5934737004953,7.66938236806233,12.));
#213674=CARTESIAN_POINT('Ctrl Pts',(22.6141842556243,7.66924547229414,0.));
#213675=CARTESIAN_POINT('Ctrl Pts',(22.6141842556243,7.66924547229414,12.));
#213676=CARTESIAN_POINT('Ctrl Pts',(22.6349991971541,7.66905281533715,0.));
#213677=CARTESIAN_POINT('Ctrl Pts',(22.6349991971541,7.66905281533715,12.));
#213678=CARTESIAN_POINT('Ctrl Pts',(22.6559177133127,7.66880399241323,0.));
#213679=CARTESIAN_POINT('Ctrl Pts',(22.6559177133127,7.66880399241323,12.));
#213680=CARTESIAN_POINT('Ctrl Pts',(22.6769390009885,7.66849860491743,0.));
#213681=CARTESIAN_POINT('Ctrl Pts',(22.6769390009885,7.66849860491743,12.));
#213682=CARTESIAN_POINT('Ctrl Pts',(22.6980622655446,7.66813626029275,0.));
#213683=CARTESIAN_POINT('Ctrl Pts',(22.6980622655446,7.66813626029275,12.));
#213684=CARTESIAN_POINT('Ctrl Pts',(22.7192867206245,7.66771657191028,0.));
#213685=CARTESIAN_POINT('Ctrl Pts',(22.7192867206245,7.66771657191028,12.));
#213686=CARTESIAN_POINT('Ctrl Pts',(22.7406115879513,7.6672391589544,0.));
#213687=CARTESIAN_POINT('Ctrl Pts',(22.7406115879513,7.6672391589544,12.));
#213688=CARTESIAN_POINT('Ctrl Pts',(22.7620360971843,7.66670364630299,0.));
#213689=CARTESIAN_POINT('Ctrl Pts',(22.7620360971843,7.66670364630299,12.));
#213690=CARTESIAN_POINT('Ctrl Pts',(22.7835594857699,7.66610966441273,0.));
#213691=CARTESIAN_POINT('Ctrl Pts',(22.7835594857699,7.66610966441273,12.));
#213692=CARTESIAN_POINT('Ctrl Pts',(22.8051809987833,7.66545684920987,0.));
#213693=CARTESIAN_POINT('Ctrl Pts',(22.8051809987833,7.66545684920987,12.));
#213694=CARTESIAN_POINT('Ctrl Pts',(22.8268998887678,7.66474484198549,0.));
#213695=CARTESIAN_POINT('Ctrl Pts',(22.8268998887678,7.66474484198549,12.));
#213696=CARTESIAN_POINT('Ctrl Pts',(22.848715415557,7.66397328929803,0.));
#213697=CARTESIAN_POINT('Ctrl Pts',(22.848715415557,7.66397328929803,12.));
#213698=CARTESIAN_POINT('Ctrl Pts',(22.8706268461283,7.66314184287337,0.));
#213699=CARTESIAN_POINT('Ctrl Pts',(22.8706268461283,7.66314184287337,12.));
#213700=CARTESIAN_POINT('Ctrl Pts',(22.8926334544883,7.66225015950156,0.));
#213701=CARTESIAN_POINT('Ctrl Pts',(22.8926334544883,7.66225015950156,12.));
#213702=CARTESIAN_POINT('Ctrl Pts',(22.9147345215421,7.66129790094108,0.));
#213703=CARTESIAN_POINT('Ctrl Pts',(22.9147345215421,7.66129790094108,12.));
#213704=CARTESIAN_POINT('Ctrl Pts',(22.9369293349593,7.66028473382778,0.));
#213705=CARTESIAN_POINT('Ctrl Pts',(22.9369293349593,7.66028473382778,12.));
#213706=CARTESIAN_POINT('Ctrl Pts',(22.959217189033,7.65921032958902,0.));
#213707=CARTESIAN_POINT('Ctrl Pts',(22.959217189033,7.65921032958902,12.));
#213708=CARTESIAN_POINT('Ctrl Pts',(22.9815973845296,7.65807436436432,0.));
#213709=CARTESIAN_POINT('Ctrl Pts',(22.9815973845296,7.65807436436432,12.));
#213710=CARTESIAN_POINT('Ctrl Pts',(23.0040692285814,7.65687651891305,0.));
#213711=CARTESIAN_POINT('Ctrl Pts',(23.0040692285814,7.65687651891305,12.));
#213712=CARTESIAN_POINT('Ctrl Pts',(23.0266320345787,7.65561647852534,0.));
#213713=CARTESIAN_POINT('Ctrl Pts',(23.0266320345787,7.65561647852534,12.));
#213714=CARTESIAN_POINT('Ctrl Pts',(23.0492851220528,7.65429393293946,0.));
#213715=CARTESIAN_POINT('Ctrl Pts',(23.0492851220528,7.65429393293946,12.));
#213716=CARTESIAN_POINT('Ctrl Pts',(23.072027816555,7.65290857626358,0.));
#213717=CARTESIAN_POINT('Ctrl Pts',(23.072027816555,7.65290857626358,12.));
#213718=CARTESIAN_POINT('Ctrl Pts',(23.094859449525,7.65146010690476,0.));
#213719=CARTESIAN_POINT('Ctrl Pts',(23.094859449525,7.65146010690476,12.));
#213720=CARTESIAN_POINT('Ctrl Pts',(23.1177793581679,7.6499482274986,0.));
#213721=CARTESIAN_POINT('Ctrl Pts',(23.1177793581679,7.6499482274986,12.));
#213722=CARTESIAN_POINT('Ctrl Pts',(23.1407868853819,7.64837264482943,0.));
#213723=CARTESIAN_POINT('Ctrl Pts',(23.1407868853819,7.64837264482943,12.));
#213724=CARTESIAN_POINT('Ctrl Pts',(23.1638813796694,7.64673306975805,0.));
#213725=CARTESIAN_POINT('Ctrl Pts',(23.1638813796694,7.64673306975805,12.));
#213726=CARTESIAN_POINT('Ctrl Pts',(23.1870621950452,7.64502921715483,0.));
#213727=CARTESIAN_POINT('Ctrl Pts',(23.1870621950452,7.64502921715483,12.));
#213728=CARTESIAN_POINT('Ctrl Pts',(23.2103286909398,7.6432608058368,0.));
#213729=CARTESIAN_POINT('Ctrl Pts',(23.2103286909398,7.6432608058368,12.));
#213730=CARTESIAN_POINT('Ctrl Pts',(23.2336802320912,7.64142755851505,0.));
#213731=CARTESIAN_POINT('Ctrl Pts',(23.2336802320912,7.64142755851505,12.));
#213732=CARTESIAN_POINT('Ctrl Pts',(23.2571161884488,7.63952920172835,0.));
#213733=CARTESIAN_POINT('Ctrl Pts',(23.2571161884488,7.63952920172835,12.));
#213734=CARTESIAN_POINT('Ctrl Pts',(23.2806359350855,7.63756546576374,0.));
#213735=CARTESIAN_POINT('Ctrl Pts',(23.2806359350855,7.63756546576374,12.));
#213736=CARTESIAN_POINT('Ctrl Pts',(23.3042388521022,7.63553608458783,0.));
#213737=CARTESIAN_POINT('Ctrl Pts',(23.3042388521022,7.63553608458783,12.));
#213738=CARTESIAN_POINT('Ctrl Pts',(23.3279243245241,7.63344079578162,0.));
#213739=CARTESIAN_POINT('Ctrl Pts',(23.3279243245241,7.63344079578162,12.));
#213740=CARTESIAN_POINT('Ctrl Pts',(23.3516917421972,7.63127934048137,0.));
#213741=CARTESIAN_POINT('Ctrl Pts',(23.3516917421972,7.63127934048137,12.));
#213742=CARTESIAN_POINT('Ctrl Pts',(23.3755404996636,7.62905146332593,0.));
#213743=CARTESIAN_POINT('Ctrl Pts',(23.3755404996636,7.62905146332593,12.));
#213744=CARTESIAN_POINT('Ctrl Pts',(23.399469996112,7.62675691240329,0.));
#213745=CARTESIAN_POINT('Ctrl Pts',(23.399469996112,7.62675691240329,12.));
#213746=CARTESIAN_POINT('Ctrl Pts',(23.4234796353542,7.6243954392005,0.));
#213747=CARTESIAN_POINT('Ctrl Pts',(23.4234796353542,7.6243954392005,12.));
#213748=CARTESIAN_POINT('Ctrl Pts',(23.4475688257854,7.62196679855955,0.));
#213749=CARTESIAN_POINT('Ctrl Pts',(23.4475688257854,7.62196679855955,12.));
#213750=CARTESIAN_POINT('Ctrl Pts',(23.4717369803438,7.61947074863977,0.));
#213751=CARTESIAN_POINT('Ctrl Pts',(23.4717369803438,7.61947074863977,12.));
#213752=CARTESIAN_POINT('Ctrl Pts',(23.4959835164609,7.61690705088319,0.));
#213753=CARTESIAN_POINT('Ctrl Pts',(23.4959835164609,7.61690705088319,12.));
#213754=CARTESIAN_POINT('Ctrl Pts',(23.5203078560129,7.61427546999298,0.));
#213755=CARTESIAN_POINT('Ctrl Pts',(23.5203078560129,7.61427546999298,12.));
#213756=CARTESIAN_POINT('Ctrl Pts',(23.544709425203,7.61157577385372,0.));
#213757=CARTESIAN_POINT('Ctrl Pts',(23.544709425203,7.61157577385372,12.));
#213758=CARTESIAN_POINT('Ctrl Pts',(23.5691876544244,7.608807733446,0.));
#213759=CARTESIAN_POINT('Ctrl Pts',(23.5691876544244,7.608807733446,12.));
#213760=CARTESIAN_POINT('Ctrl Pts',(23.5937419781245,7.60597112277094,0.));
#213761=CARTESIAN_POINT('Ctrl Pts',(23.5937419781245,7.60597112277094,12.));
#213762=CARTESIAN_POINT('Ctrl Pts',(23.6183718346576,7.60306571877806,0.));
#213763=CARTESIAN_POINT('Ctrl Pts',(23.6183718346576,7.60306571877806,12.));
#213764=CARTESIAN_POINT('Ctrl Pts',(23.6430766661418,7.60009130130126,0.));
#213765=CARTESIAN_POINT('Ctrl Pts',(23.6430766661418,7.60009130130126,12.));
#213766=CARTESIAN_POINT('Ctrl Pts',(23.6678559182875,7.59704765299567,0.));
#213767=CARTESIAN_POINT('Ctrl Pts',(23.6678559182875,7.59704765299567,12.));
#213768=CARTESIAN_POINT('Ctrl Pts',(23.6927090405066,7.59393455934035,0.));
#213769=CARTESIAN_POINT('Ctrl Pts',(23.6927090405066,7.59393455934035,12.));
#213770=CARTESIAN_POINT('Ctrl Pts',(23.7176354860456,7.59075180865321,0.));
#213771=CARTESIAN_POINT('Ctrl Pts',(23.7176354860456,7.59075180865321,12.));
#213772=CARTESIAN_POINT('Ctrl Pts',(23.7426347121006,7.58749919210826,0.));
#213773=CARTESIAN_POINT('Ctrl Pts',(23.7426347121006,7.58749919210826,12.));
#213774=CARTESIAN_POINT('Ctrl Pts',(23.7677061799376,7.58417650376271,0.));
#213775=CARTESIAN_POINT('Ctrl Pts',(23.7677061799376,7.58417650376271,12.));
#213776=CARTESIAN_POINT('Ctrl Pts',(23.7928493549908,7.58078354058213,0.));
#213777=CARTESIAN_POINT('Ctrl Pts',(23.7928493549908,7.58078354058213,12.));
#213778=CARTESIAN_POINT('Ctrl Pts',(23.8180637069976,7.57732010249066,0.));
#213779=CARTESIAN_POINT('Ctrl Pts',(23.8180637069976,7.57732010249066,12.));
#213780=CARTESIAN_POINT('Ctrl Pts',(23.8433487096132,7.57378599219814,0.));
#213781=CARTESIAN_POINT('Ctrl Pts',(23.8433487096132,7.57378599219814,12.));
#213782=CARTESIAN_POINT('Ctrl Pts',(23.8687038399595,7.57018101500709,0.));
#213783=CARTESIAN_POINT('Ctrl Pts',(23.8687038399595,7.57018101500709,12.));
#213784=CARTESIAN_POINT('Ctrl Pts',(23.8941285782002,7.56650497863791,0.));
#213785=CARTESIAN_POINT('Ctrl Pts',(23.8941285782002,7.56650497863791,12.));
#213786=CARTESIAN_POINT('Ctrl Pts',(23.9196224070759,7.56275769304773,0.));
#213787=CARTESIAN_POINT('Ctrl Pts',(23.9196224070759,7.56275769304773,12.));
#213788=CARTESIAN_POINT('Ctrl Pts',(23.9451848115002,7.5589389702768,0.));
#213789=CARTESIAN_POINT('Ctrl Pts',(23.9451848115002,7.5589389702768,12.));
#213790=CARTESIAN_POINT('Ctrl Pts',(23.9708152779886,7.55504862424808,0.));
#213791=CARTESIAN_POINT('Ctrl Pts',(23.9708152779886,7.55504862424808,12.));
#213792=CARTESIAN_POINT('Ctrl Pts',(23.9965132953187,7.55108647097432,0.));
#213793=CARTESIAN_POINT('Ctrl Pts',(23.9965132953187,7.55108647097432,12.));
#213794=CARTESIAN_POINT('Ctrl Pts',(24.0222783554531,7.54705232885895,0.));
#213795=CARTESIAN_POINT('Ctrl Pts',(24.0222783554531,7.54705232885895,12.));
#213796=CARTESIAN_POINT('Ctrl Pts',(24.0481099543353,7.54294601896128,0.));
#213797=CARTESIAN_POINT('Ctrl Pts',(24.0481099543353,7.54294601896128,12.));
#213798=CARTESIAN_POINT('Ctrl Pts',(24.0740075927984,7.53876736531005,0.));
#213799=CARTESIAN_POINT('Ctrl Pts',(24.0740075927984,7.53876736531005,12.));
#213800=CARTESIAN_POINT('Ctrl Pts',(24.0999707772642,7.53451619514659,0.));
#213801=CARTESIAN_POINT('Ctrl Pts',(24.0999707772642,7.53451619514659,12.));
#213802=CARTESIAN_POINT('Ctrl Pts',(24.1259990209211,7.53019233935537,0.));
#213803=CARTESIAN_POINT('Ctrl Pts',(24.1259990209211,7.53019233935537,12.));
#213804=CARTESIAN_POINT('Ctrl Pts',(24.152091842537,7.52579563201479,0.));
#213805=CARTESIAN_POINT('Ctrl Pts',(24.152091842537,7.52579563201479,12.));
#213806=CARTESIAN_POINT('Ctrl Pts',(24.1782487641602,7.52132590953863,0.));
#213807=CARTESIAN_POINT('Ctrl Pts',(24.1782487641602,7.52132590953863,12.));
#213808=CARTESIAN_POINT('Ctrl Pts',(24.2044693092356,7.51678300997998,0.));
#213809=CARTESIAN_POINT('Ctrl Pts',(24.2044693092356,7.51678300997998,12.));
#213810=CARTESIAN_POINT('Ctrl Pts',(24.230753000389,7.51216677222199,0.));
#213811=CARTESIAN_POINT('Ctrl Pts',(24.230753000389,7.51216677222199,12.));
#213812=CARTESIAN_POINT('Ctrl Pts',(24.2570993577032,7.50747703535115,0.));
#213813=CARTESIAN_POINT('Ctrl Pts',(24.2570993577032,7.50747703535115,12.));
#213814=CARTESIAN_POINT('Ctrl Pts',(24.2835078958966,7.50271363765099,0.));
#213815=CARTESIAN_POINT('Ctrl Pts',(24.2835078958966,7.50271363765099,12.));
#213816=CARTESIAN_POINT('Ctrl Pts',(24.3099781253345,7.49787641695359,0.));
#213817=CARTESIAN_POINT('Ctrl Pts',(24.3099781253345,7.49787641695359,12.));
#213818=CARTESIAN_POINT('Ctrl Pts',(24.3365095573673,7.4929652125233,0.));
#213819=CARTESIAN_POINT('Ctrl Pts',(24.3365095573673,7.4929652125233,12.));
#213820=CARTESIAN_POINT('Ctrl Pts',(24.3631017084513,7.48797986651828,0.));
#213821=CARTESIAN_POINT('Ctrl Pts',(24.3631017084513,7.48797986651828,12.));
#213822=CARTESIAN_POINT('Ctrl Pts',(24.3897541049248,7.48292022569254,0.));
#213823=CARTESIAN_POINT('Ctrl Pts',(24.3897541049248,7.48292022569254,12.));
#213824=CARTESIAN_POINT('Ctrl Pts',(24.4164662871165,7.47778614286574,0.));
#213825=CARTESIAN_POINT('Ctrl Pts',(24.4164662871165,7.47778614286574,12.));
#213826=CARTESIAN_POINT('Ctrl Pts',(24.4432378146501,7.47257747883319,0.));
#213827=CARTESIAN_POINT('Ctrl Pts',(24.4432378146501,7.47257747883319,12.));
#213828=CARTESIAN_POINT('Ctrl Pts',(24.4700682684544,7.46729410308923,0.));
#213829=CARTESIAN_POINT('Ctrl Pts',(24.4700682684544,7.46729410308923,12.));
#213830=CARTESIAN_POINT('Ctrl Pts',(24.4969572391509,7.46193588961642,0.));
#213831=CARTESIAN_POINT('Ctrl Pts',(24.4969572391509,7.46193588961642,12.));
#213832=CARTESIAN_POINT('Ctrl Pts',(24.52390431731,7.45650271336046,0.));
#213833=CARTESIAN_POINT('Ctrl Pts',(24.52390431731,7.45650271336046,12.));
#213834=CARTESIAN_POINT('Ctrl Pts',(24.5509090831579,7.45099444651296,0.));
#213835=CARTESIAN_POINT('Ctrl Pts',(24.5509090831579,7.45099444651296,12.));
#213836=CARTESIAN_POINT('Ctrl Pts',(24.5779710960865,7.44541095473163,0.));
#213837=CARTESIAN_POINT('Ctrl Pts',(24.5779710960865,7.44541095473163,12.));
#213838=CARTESIAN_POINT('Ctrl Pts',(24.6050898852349,7.43975209375375,0.));
#213839=CARTESIAN_POINT('Ctrl Pts',(24.6050898852349,7.43975209375375,12.));
#213840=CARTESIAN_POINT('Ctrl Pts',(24.6322649369472,7.43401770489221,0.));
#213841=CARTESIAN_POINT('Ctrl Pts',(24.6322649369472,7.43401770489221,12.));
#213842=CARTESIAN_POINT('Ctrl Pts',(24.659495712869,7.42820762158681,0.));
#213843=CARTESIAN_POINT('Ctrl Pts',(24.659495712869,7.42820762158681,12.));
#213844=CARTESIAN_POINT('Ctrl Pts',(24.6867816727118,7.42232167765763,0.));
#213845=CARTESIAN_POINT('Ctrl Pts',(24.6867816727118,7.42232167765763,12.));
#213846=CARTESIAN_POINT('Ctrl Pts',(24.7141222949988,7.41635971481243,0.));
#213847=CARTESIAN_POINT('Ctrl Pts',(24.7141222949988,7.41635971481243,12.));
#213848=CARTESIAN_POINT('Ctrl Pts',(24.7415170994754,7.41032159082173,0.));
#213849=CARTESIAN_POINT('Ctrl Pts',(24.7415170994754,7.41032159082173,12.));
#213850=CARTESIAN_POINT('Ctrl Pts',(24.7689656669005,7.40420718661755,0.));
#213851=CARTESIAN_POINT('Ctrl Pts',(24.7689656669005,7.40420718661755,12.));
#213852=CARTESIAN_POINT('Ctrl Pts',(24.7964676646518,7.39801641583613,0.));
#213853=CARTESIAN_POINT('Ctrl Pts',(24.7964676646518,7.39801641583613,12.));
#213854=CARTESIAN_POINT('Ctrl Pts',(24.8240228521042,7.39174922586841,0.));
#213855=CARTESIAN_POINT('Ctrl Pts',(24.8240228521042,7.39174922586841,12.));
#213856=CARTESIAN_POINT('Ctrl Pts',(24.8516310625367,7.38540558904946,0.));
#213857=CARTESIAN_POINT('Ctrl Pts',(24.8516310625367,7.38540558904946,12.));
#213858=CARTESIAN_POINT('Ctrl Pts',(24.8792921911309,7.3789854964161,0.));
#213859=CARTESIAN_POINT('Ctrl Pts',(24.8792921911309,7.3789854964161,12.));
#213860=CARTESIAN_POINT('Ctrl Pts',(24.9014633826201,7.37378825962718,0.));
#213861=CARTESIAN_POINT('Ctrl Pts',(24.9014633826201,7.37378825962718,12.));
#213862=CARTESIAN_POINT('Ctrl Pts',(24.9181155530631,7.36985593120697,0.));
#213863=CARTESIAN_POINT('Ctrl Pts',(24.9181155530631,7.36985593120697,12.));
#213864=CARTESIAN_POINT('Ctrl Pts',(24.9292275670705,7.3672190902906,0.));
#213865=CARTESIAN_POINT('Ctrl Pts',(24.9292275670705,7.3672190902906,12.));
#213866=CARTESIAN_POINT('Ctrl Pts',(24.9347862158358,7.36589684767344,0.));
#213867=CARTESIAN_POINT('Ctrl Pts',(24.9347862158358,7.36589684767344,12.));
#213868=CARTESIAN_POINT('',(24.9347862158358,7.36589684767344,0.));
#213869=CARTESIAN_POINT('Ctrl Pts',(21.2610617890679,7.52250298901264,0.));
#213870=CARTESIAN_POINT('Ctrl Pts',(21.2610673466886,7.5225064970397,0.));
#213871=CARTESIAN_POINT('Ctrl Pts',(21.2611204474866,7.52252744144904,0.));
#213872=CARTESIAN_POINT('Ctrl Pts',(21.261326054066,7.52260064231661,0.));
#213873=CARTESIAN_POINT('Ctrl Pts',(21.2618521283555,7.5227818224267,0.));
#213874=CARTESIAN_POINT('Ctrl Pts',(21.262927782038,7.52314642316199,0.));
#213875=CARTESIAN_POINT('Ctrl Pts',(21.2644161259962,7.52364573027553,0.));
#213876=CARTESIAN_POINT('Ctrl Pts',(21.2663059157058,7.52427261074298,0.));
#213877=CARTESIAN_POINT('Ctrl Pts',(21.2685823838671,7.52501770333531,0.));
#213878=CARTESIAN_POINT('Ctrl Pts',(21.2712301573466,7.5258712609553,0.));
#213879=CARTESIAN_POINT('Ctrl Pts',(21.2742366113579,7.52682526918541,0.));
#213880=CARTESIAN_POINT('Ctrl Pts',(21.2775925269652,7.52787386225333,0.));
#213881=CARTESIAN_POINT('Ctrl Pts',(21.2812902781143,7.52901217930408,0.));
#213882=CARTESIAN_POINT('Ctrl Pts',(21.2853226580657,7.5302356243823,0.));
#213883=CARTESIAN_POINT('Ctrl Pts',(21.2896816163842,7.53153906987856,0.));
#213884=CARTESIAN_POINT('Ctrl Pts',(21.2943588989331,7.53291726078527,0.));
#213885=CARTESIAN_POINT('Ctrl Pts',(21.2993464250717,7.53436505309943,0.));
#213886=CARTESIAN_POINT('Ctrl Pts',(21.3046368712157,7.53587778251736,0.));
#213887=CARTESIAN_POINT('Ctrl Pts',(21.310223716773,7.53745129364616,0.));
#213888=CARTESIAN_POINT('Ctrl Pts',(21.3161009456256,7.53908175169899,0.));
#213889=CARTESIAN_POINT('Ctrl Pts',(21.3222628524165,7.54076552038279,0.));
#213890=CARTESIAN_POINT('Ctrl Pts',(21.328703791771,7.54249900377031,0.));
#213891=CARTESIAN_POINT('Ctrl Pts',(21.3354182340149,7.54427868151268,0.));
#213892=CARTESIAN_POINT('Ctrl Pts',(21.3424008295038,7.54610114948347,0.));
#213893=CARTESIAN_POINT('Ctrl Pts',(21.3496464761531,7.54796316246331,0.));
#213894=CARTESIAN_POINT('Ctrl Pts',(21.3571503685855,7.5498616652131,0.));
#213895=CARTESIAN_POINT('Ctrl Pts',(21.3649079431865,7.55179375777444,0.));
#213896=CARTESIAN_POINT('Ctrl Pts',(21.3729148390243,7.55375667080029,0.));
#213897=CARTESIAN_POINT('Ctrl Pts',(21.3811668478932,7.55574773403503,0.));
#213898=CARTESIAN_POINT('Ctrl Pts',(21.3896598842117,7.55776435731417,0.));
#213899=CARTESIAN_POINT('Ctrl Pts',(21.3983899952987,7.55980403700611,0.));
#213900=CARTESIAN_POINT('Ctrl Pts',(21.4073533630365,7.56186435703622,0.));
#213901=CARTESIAN_POINT('Ctrl Pts',(21.4165463106254,7.56394299313685,0.));
#213902=CARTESIAN_POINT('Ctrl Pts',(21.4259653015736,7.56603771218712,0.));
#213903=CARTESIAN_POINT('Ctrl Pts',(21.4356069261513,7.56814636360848,0.));
#213904=CARTESIAN_POINT('Ctrl Pts',(21.4454678907509,7.57026687261166,0.));
#213905=CARTESIAN_POINT('Ctrl Pts',(21.4555450053142,7.57239723223506,0.));
#213906=CARTESIAN_POINT('Ctrl Pts',(21.4658351740128,7.57453549743412,0.));
#213907=CARTESIAN_POINT('Ctrl Pts',(21.4763353936762,7.57667978402987,0.));
#213908=CARTESIAN_POINT('Ctrl Pts',(21.4870427508194,7.57882826679132,0.));
#213909=CARTESIAN_POINT('Ctrl Pts',(21.4979544192744,7.58097917790744,0.));
#213910=CARTESIAN_POINT('Ctrl Pts',(21.5090676573873,7.5831308051918,0.));
#213911=CARTESIAN_POINT('Ctrl Pts',(21.5203798035299,7.5852814891913,0.));
#213912=CARTESIAN_POINT('Ctrl Pts',(21.5318882716736,7.58742962034834,0.));
#213913=CARTESIAN_POINT('Ctrl Pts',(21.543590547011,7.58957363620014,0.));
#213914=CARTESIAN_POINT('Ctrl Pts',(21.5554841813462,7.59171201844777,0.));
#213915=CARTESIAN_POINT('Ctrl Pts',(21.5675667904726,7.59384329124918,0.));
#213916=CARTESIAN_POINT('Ctrl Pts',(21.5798360518978,7.59596601973584,0.));
#213917=CARTESIAN_POINT('Ctrl Pts',(21.5922897024466,7.59807880846195,0.));
#213918=CARTESIAN_POINT('Ctrl Pts',(21.6049255358843,7.60018029988241,0.));
#213919=CARTESIAN_POINT('Ctrl Pts',(21.617741400599,7.60226917285429,0.));
#213920=CARTESIAN_POINT('Ctrl Pts',(21.6307351973822,7.60434414118296,0.));
#213921=CARTESIAN_POINT('Ctrl Pts',(21.6439048771743,7.60640395216357,0.));
#213922=CARTESIAN_POINT('Ctrl Pts',(21.6572484388081,7.60844738512874,0.));
#213923=CARTESIAN_POINT('Ctrl Pts',(21.6707639267576,7.61047325000956,0.));
#213924=CARTESIAN_POINT('Ctrl Pts',(21.6844494295815,7.61248038630269,0.));
#213925=CARTESIAN_POINT('Ctrl Pts',(21.6983030783322,7.61446766202787,0.));
#213926=CARTESIAN_POINT('Ctrl Pts',(21.7123230449834,7.61643397270421,0.));
#213927=CARTESIAN_POINT('Ctrl Pts',(21.7265075407975,7.61837824030538,0.));
#213928=CARTESIAN_POINT('Ctrl Pts',(21.7408548148656,7.62029941230855,0.));
#213929=CARTESIAN_POINT('Ctrl Pts',(21.7553631528328,7.62219646084229,0.));
#213930=CARTESIAN_POINT('Ctrl Pts',(21.7700308755584,7.62406838181166,0.));
#213931=CARTESIAN_POINT('Ctrl Pts',(21.7848563378021,7.62591419404513,0.));
#213932=CARTESIAN_POINT('Ctrl Pts',(21.799837926858,7.62773293842389,0.));
#213933=CARTESIAN_POINT('Ctrl Pts',(21.814974061509,7.62952367718127,0.));
#213934=CARTESIAN_POINT('Ctrl Pts',(21.8302631910195,7.63128549323023,0.));
#213935=CARTESIAN_POINT('Ctrl Pts',(21.8457037941084,7.63301748948936,0.));
#213936=CARTESIAN_POINT('Ctrl Pts',(21.8612943779089,7.63471878821226,0.));
#213937=CARTESIAN_POINT('Ctrl Pts',(21.8770334769496,7.636388530334,0.));
#213938=CARTESIAN_POINT('Ctrl Pts',(21.8929196523514,7.63802587492035,0.));
#213939=CARTESIAN_POINT('Ctrl Pts',(21.9089514909874,7.63962999860927,0.));
#213940=CARTESIAN_POINT('Ctrl Pts',(21.9251276046545,7.64120009506532,0.));
#213941=CARTESIAN_POINT('Ctrl Pts',(21.9414466292072,7.64273537442682,0.));
#213942=CARTESIAN_POINT('Ctrl Pts',(21.9579072237651,7.64423506279123,0.));
#213943=CARTESIAN_POINT('Ctrl Pts',(21.9745080700798,7.64569840177336,0.));
#213944=CARTESIAN_POINT('Ctrl Pts',(21.9912478718542,7.6471246480525,0.));
#213945=CARTESIAN_POINT('Ctrl Pts',(22.0081253540774,7.64851307293352,0.));
#213946=CARTESIAN_POINT('Ctrl Pts',(22.0251392623209,7.64986296190169,0.));
#213947=CARTESIAN_POINT('Ctrl Pts',(22.0422883621174,7.65117361421359,0.));
#213948=CARTESIAN_POINT('Ctrl Pts',(22.0595714384431,7.65244434253113,0.));
#213949=CARTESIAN_POINT('Ctrl Pts',(22.0769872951596,7.65367447254949,0.));
#213950=CARTESIAN_POINT('Ctrl Pts',(22.094534754469,7.65486334263644,0.));
#213951=CARTESIAN_POINT('Ctrl Pts',(22.1122126563329,7.65601030346807,0.));
#213952=CARTESIAN_POINT('Ctrl Pts',(22.1300198579675,7.65711471769397,0.));
#213953=CARTESIAN_POINT('Ctrl Pts',(22.1479552334211,7.65817595963349,0.));
#213954=CARTESIAN_POINT('Ctrl Pts',(22.1660176731178,7.65919341496931,0.));
#213955=CARTESIAN_POINT('Ctrl Pts',(22.1842060834091,7.66016648045005,0.));
#213956=CARTESIAN_POINT('Ctrl Pts',(22.2025193860964,7.66109456359271,0.));
#213957=CARTESIAN_POINT('Ctrl Pts',(22.2209565180085,7.661977082404,0.));
#213958=CARTESIAN_POINT('Ctrl Pts',(22.2395164306547,7.66281346512509,0.));
#213959=CARTESIAN_POINT('Ctrl Pts',(22.258198089848,7.66360314997641,0.));
#213960=CARTESIAN_POINT('Ctrl Pts',(22.2770004753335,7.66434558490979,0.));
#213961=CARTESIAN_POINT('Ctrl Pts',(22.2959225803937,7.66504022736299,0.));
#213962=CARTESIAN_POINT('Ctrl Pts',(22.314963411484,7.66568654402494,0.));
#213963=CARTESIAN_POINT('Ctrl Pts',(22.3341219879469,7.66628401061952,0.));
#213964=CARTESIAN_POINT('Ctrl Pts',(22.3533973417021,7.66683211169159,0.));
#213965=CARTESIAN_POINT('Ctrl Pts',(22.372788516936,7.66733034039883,0.));
#213966=CARTESIAN_POINT('Ctrl Pts',(22.3922945697773,7.6677781983079,0.));
#213967=CARTESIAN_POINT('Ctrl Pts',(22.4119145679758,7.6681751951964,0.));
#213968=CARTESIAN_POINT('Ctrl Pts',(22.4316475906603,7.66852084886704,0.));
#213969=CARTESIAN_POINT('Ctrl Pts',(22.4514927280855,7.66881468496635,0.));
#213970=CARTESIAN_POINT('Ctrl Pts',(22.4714490813699,7.66905623680831,0.));
#213971=CARTESIAN_POINT('Ctrl Pts',(22.4915157622312,7.66924504520315,0.));
#213972=CARTESIAN_POINT('Ctrl Pts',(22.5116918927031,7.66938065829108,0.));
#213973=CARTESIAN_POINT('Ctrl Pts',(22.53197660492,7.66946263138144,0.));
#213974=CARTESIAN_POINT('Ctrl Pts',(22.5523690409116,7.66949052679693,0.));
#213975=CARTESIAN_POINT('Ctrl Pts',(22.5728683523831,7.66946391372306,0.));
#213976=CARTESIAN_POINT('Ctrl Pts',(22.5934737004953,7.66938236806233,0.));
#213977=CARTESIAN_POINT('Ctrl Pts',(22.6141842556243,7.66924547229414,0.));
#213978=CARTESIAN_POINT('Ctrl Pts',(22.6349991971541,7.66905281533715,0.));
#213979=CARTESIAN_POINT('Ctrl Pts',(22.6559177133127,7.66880399241323,0.));
#213980=CARTESIAN_POINT('Ctrl Pts',(22.6769390009885,7.66849860491743,0.));
#213981=CARTESIAN_POINT('Ctrl Pts',(22.6980622655446,7.66813626029275,0.));
#213982=CARTESIAN_POINT('Ctrl Pts',(22.7192867206245,7.66771657191028,0.));
#213983=CARTESIAN_POINT('Ctrl Pts',(22.7406115879513,7.6672391589544,0.));
#213984=CARTESIAN_POINT('Ctrl Pts',(22.7620360971843,7.66670364630299,0.));
#213985=CARTESIAN_POINT('Ctrl Pts',(22.7835594857699,7.66610966441273,0.));
#213986=CARTESIAN_POINT('Ctrl Pts',(22.8051809987833,7.66545684920987,0.));
#213987=CARTESIAN_POINT('Ctrl Pts',(22.8268998887678,7.66474484198549,0.));
#213988=CARTESIAN_POINT('Ctrl Pts',(22.848715415557,7.66397328929803,0.));
#213989=CARTESIAN_POINT('Ctrl Pts',(22.8706268461283,7.66314184287337,0.));
#213990=CARTESIAN_POINT('Ctrl Pts',(22.8926334544883,7.66225015950156,0.));
#213991=CARTESIAN_POINT('Ctrl Pts',(22.9147345215421,7.66129790094108,0.));
#213992=CARTESIAN_POINT('Ctrl Pts',(22.9369293349593,7.66028473382778,0.));
#213993=CARTESIAN_POINT('Ctrl Pts',(22.959217189033,7.65921032958902,0.));
#213994=CARTESIAN_POINT('Ctrl Pts',(22.9815973845296,7.65807436436432,0.));
#213995=CARTESIAN_POINT('Ctrl Pts',(23.0040692285814,7.65687651891305,0.));
#213996=CARTESIAN_POINT('Ctrl Pts',(23.0266320345787,7.65561647852534,0.));
#213997=CARTESIAN_POINT('Ctrl Pts',(23.0492851220528,7.65429393293946,0.));
#213998=CARTESIAN_POINT('Ctrl Pts',(23.072027816555,7.65290857626358,0.));
#213999=CARTESIAN_POINT('Ctrl Pts',(23.094859449525,7.65146010690476,0.));
#214000=CARTESIAN_POINT('Ctrl Pts',(23.1177793581679,7.6499482274986,0.));
#214001=CARTESIAN_POINT('Ctrl Pts',(23.1407868853819,7.64837264482943,0.));
#214002=CARTESIAN_POINT('Ctrl Pts',(23.1638813796694,7.64673306975805,0.));
#214003=CARTESIAN_POINT('Ctrl Pts',(23.1870621950452,7.64502921715483,0.));
#214004=CARTESIAN_POINT('Ctrl Pts',(23.2103286909398,7.6432608058368,0.));
#214005=CARTESIAN_POINT('Ctrl Pts',(23.2336802320912,7.64142755851505,0.));
#214006=CARTESIAN_POINT('Ctrl Pts',(23.2571161884488,7.63952920172835,0.));
#214007=CARTESIAN_POINT('Ctrl Pts',(23.2806359350855,7.63756546576374,0.));
#214008=CARTESIAN_POINT('Ctrl Pts',(23.3042388521022,7.63553608458783,0.));
#214009=CARTESIAN_POINT('Ctrl Pts',(23.3279243245241,7.63344079578162,0.));
#214010=CARTESIAN_POINT('Ctrl Pts',(23.3516917421972,7.63127934048137,0.));
#214011=CARTESIAN_POINT('Ctrl Pts',(23.3755404996636,7.62905146332593,0.));
#214012=CARTESIAN_POINT('Ctrl Pts',(23.399469996112,7.62675691240329,0.));
#214013=CARTESIAN_POINT('Ctrl Pts',(23.4234796353542,7.6243954392005,0.));
#214014=CARTESIAN_POINT('Ctrl Pts',(23.4475688257854,7.62196679855955,0.));
#214015=CARTESIAN_POINT('Ctrl Pts',(23.4717369803438,7.61947074863977,0.));
#214016=CARTESIAN_POINT('Ctrl Pts',(23.4959835164609,7.61690705088319,0.));
#214017=CARTESIAN_POINT('Ctrl Pts',(23.5203078560129,7.61427546999298,0.));
#214018=CARTESIAN_POINT('Ctrl Pts',(23.544709425203,7.61157577385372,0.));
#214019=CARTESIAN_POINT('Ctrl Pts',(23.5691876544244,7.608807733446,0.));
#214020=CARTESIAN_POINT('Ctrl Pts',(23.5937419781245,7.60597112277094,0.));
#214021=CARTESIAN_POINT('Ctrl Pts',(23.6183718346576,7.60306571877806,0.));
#214022=CARTESIAN_POINT('Ctrl Pts',(23.6430766661418,7.60009130130126,0.));
#214023=CARTESIAN_POINT('Ctrl Pts',(23.6678559182875,7.59704765299567,0.));
#214024=CARTESIAN_POINT('Ctrl Pts',(23.6927090405066,7.59393455934035,0.));
#214025=CARTESIAN_POINT('Ctrl Pts',(23.7176354860456,7.59075180865321,0.));
#214026=CARTESIAN_POINT('Ctrl Pts',(23.7426347121006,7.58749919210826,0.));
#214027=CARTESIAN_POINT('Ctrl Pts',(23.7677061799376,7.58417650376271,0.));
#214028=CARTESIAN_POINT('Ctrl Pts',(23.7928493549908,7.58078354058213,0.));
#214029=CARTESIAN_POINT('Ctrl Pts',(23.8180637069976,7.57732010249066,0.));
#214030=CARTESIAN_POINT('Ctrl Pts',(23.8433487096132,7.57378599219814,0.));
#214031=CARTESIAN_POINT('Ctrl Pts',(23.8687038399595,7.57018101500709,0.));
#214032=CARTESIAN_POINT('Ctrl Pts',(23.8941285782002,7.56650497863791,0.));
#214033=CARTESIAN_POINT('Ctrl Pts',(23.9196224070759,7.56275769304773,0.));
#214034=CARTESIAN_POINT('Ctrl Pts',(23.9451848115002,7.5589389702768,0.));
#214035=CARTESIAN_POINT('Ctrl Pts',(23.9708152779886,7.55504862424808,0.));
#214036=CARTESIAN_POINT('Ctrl Pts',(23.9965132953187,7.55108647097432,0.));
#214037=CARTESIAN_POINT('Ctrl Pts',(24.0222783554531,7.54705232885895,0.));
#214038=CARTESIAN_POINT('Ctrl Pts',(24.0481099543353,7.54294601896128,0.));
#214039=CARTESIAN_POINT('Ctrl Pts',(24.0740075927984,7.53876736531005,0.));
#214040=CARTESIAN_POINT('Ctrl Pts',(24.0999707772642,7.53451619514659,0.));
#214041=CARTESIAN_POINT('Ctrl Pts',(24.1259990209211,7.53019233935537,0.));
#214042=CARTESIAN_POINT('Ctrl Pts',(24.152091842537,7.52579563201479,0.));
#214043=CARTESIAN_POINT('Ctrl Pts',(24.1782487641602,7.52132590953863,0.));
#214044=CARTESIAN_POINT('Ctrl Pts',(24.2044693092356,7.51678300997998,0.));
#214045=CARTESIAN_POINT('Ctrl Pts',(24.230753000389,7.51216677222199,0.));
#214046=CARTESIAN_POINT('Ctrl Pts',(24.2570993577032,7.50747703535115,0.));
#214047=CARTESIAN_POINT('Ctrl Pts',(24.2835078958966,7.50271363765099,0.));
#214048=CARTESIAN_POINT('Ctrl Pts',(24.3099781253345,7.49787641695359,0.));
#214049=CARTESIAN_POINT('Ctrl Pts',(24.3365095573673,7.4929652125233,0.));
#214050=CARTESIAN_POINT('Ctrl Pts',(24.3631017084513,7.48797986651828,0.));
#214051=CARTESIAN_POINT('Ctrl Pts',(24.3897541049248,7.48292022569254,0.));
#214052=CARTESIAN_POINT('Ctrl Pts',(24.4164662871165,7.47778614286574,0.));
#214053=CARTESIAN_POINT('Ctrl Pts',(24.4432378146501,7.47257747883319,0.));
#214054=CARTESIAN_POINT('Ctrl Pts',(24.4700682684544,7.46729410308923,0.));
#214055=CARTESIAN_POINT('Ctrl Pts',(24.4969572391509,7.46193588961642,0.));
#214056=CARTESIAN_POINT('Ctrl Pts',(24.52390431731,7.45650271336046,0.));
#214057=CARTESIAN_POINT('Ctrl Pts',(24.5509090831579,7.45099444651296,0.));
#214058=CARTESIAN_POINT('Ctrl Pts',(24.5779710960865,7.44541095473163,0.));
#214059=CARTESIAN_POINT('Ctrl Pts',(24.6050898852349,7.43975209375375,0.));
#214060=CARTESIAN_POINT('Ctrl Pts',(24.6322649369472,7.43401770489221,0.));
#214061=CARTESIAN_POINT('Ctrl Pts',(24.659495712869,7.42820762158681,0.));
#214062=CARTESIAN_POINT('Ctrl Pts',(24.6867816727118,7.42232167765763,0.));
#214063=CARTESIAN_POINT('Ctrl Pts',(24.7141222949988,7.41635971481243,0.));
#214064=CARTESIAN_POINT('Ctrl Pts',(24.7415170994754,7.41032159082173,0.));
#214065=CARTESIAN_POINT('Ctrl Pts',(24.7689656669005,7.40420718661755,0.));
#214066=CARTESIAN_POINT('Ctrl Pts',(24.7964676646518,7.39801641583613,0.));
#214067=CARTESIAN_POINT('Ctrl Pts',(24.8240228521042,7.39174922586841,0.));
#214068=CARTESIAN_POINT('Ctrl Pts',(24.8516310625367,7.38540558904946,0.));
#214069=CARTESIAN_POINT('Ctrl Pts',(24.8792921911309,7.3789854964161,0.));
#214070=CARTESIAN_POINT('Ctrl Pts',(24.9014633826201,7.37378825962718,0.));
#214071=CARTESIAN_POINT('Ctrl Pts',(24.9181155530631,7.36985593120697,0.));
#214072=CARTESIAN_POINT('Ctrl Pts',(24.9292275670705,7.3672190902906,0.));
#214073=CARTESIAN_POINT('Ctrl Pts',(24.9347862158358,7.36589684767344,0.));
#214074=CARTESIAN_POINT('',(24.9347862158358,7.36589684767344,0.));
#214075=CARTESIAN_POINT('Origin',(0.,0.,0.));
#214076=CARTESIAN_POINT('Origin',(0.,0.,0.));
#214077=CARTESIAN_POINT('Origin',(0.,0.,0.));
#214078=CARTESIAN_POINT('Origin',(0.,0.,0.));
#214079=CARTESIAN_POINT('Origin',(0.,0.,0.));
#214080=CARTESIAN_POINT('Origin',(0.,0.,0.));
#214081=CARTESIAN_POINT('Origin',(0.,0.,0.));
#214082=CARTESIAN_POINT('Origin',(0.,0.,0.));
#214083=CARTESIAN_POINT('Origin',(0.,0.,0.));
#214084=CARTESIAN_POINT('Origin',(0.,0.,0.));
#214085=CARTESIAN_POINT('Origin',(0.,0.,0.));
#214086=CARTESIAN_POINT('Origin',(0.,0.,0.));
#214087=CARTESIAN_POINT('Origin',(0.,0.,0.));
#214088=CARTESIAN_POINT('Origin',(0.,0.,0.));
#214089=CARTESIAN_POINT('Origin',(0.,0.,0.));
#214090=CARTESIAN_POINT('Origin',(0.,0.,0.));
#214091=CARTESIAN_POINT('Origin',(0.,0.,0.));
#214092=CARTESIAN_POINT('Origin',(0.,0.,0.));
#214093=CARTESIAN_POINT('Origin',(0.,0.,0.));
#214094=CARTESIAN_POINT('Origin',(0.,0.,0.));
#214095=CARTESIAN_POINT('Origin',(0.,0.,0.));
#214096=CARTESIAN_POINT('Origin',(0.,0.,0.));
#214097=CARTESIAN_POINT('Origin',(0.,0.,0.));
#214098=CARTESIAN_POINT('',(25.2771067246846,6.08833931617698,0.));
#214099=CARTESIAN_POINT('Origin',(0.,0.,0.));
#214100=CARTESIAN_POINT('',(22.1738711152697,4.11585220600461,0.));
#214101=CARTESIAN_POINT('Ctrl Pts',(25.2771067246846,6.08833931617698,0.));
#214102=CARTESIAN_POINT('Ctrl Pts',(25.2729539149479,6.08441489609824,0.));
#214103=CARTESIAN_POINT('Ctrl Pts',(25.2646490489816,6.07657531787578,0.));
#214104=CARTESIAN_POINT('Ctrl Pts',(25.2521940105523,6.06484373634697,0.));
#214105=CARTESIAN_POINT('Ctrl Pts',(25.2355918138798,6.04925720151412,0.));
#214106=CARTESIAN_POINT('Ctrl Pts',(25.2148466201368,6.02986667390187,0.));
#214107=CARTESIAN_POINT('Ctrl Pts',(25.1941090269638,6.0105688180476,0.));
#214108=CARTESIAN_POINT('Ctrl Pts',(25.1733791296154,5.99136367859839,0.));
#214109=CARTESIAN_POINT('Ctrl Pts',(25.1526570863065,5.97225131495636,0.));
#214110=CARTESIAN_POINT('Ctrl Pts',(25.1319431317273,5.95323180187348,0.));
#214111=CARTESIAN_POINT('Ctrl Pts',(25.1112375971182,5.93430523086776,0.));
#214112=CARTESIAN_POINT('Ctrl Pts',(25.0905409050863,5.91547170844382,0.));
#214113=CARTESIAN_POINT('Ctrl Pts',(25.0698535426593,5.89673135155459,0.));
#214114=CARTESIAN_POINT('Ctrl Pts',(25.0491760405965,5.87808428385329,0.));
#214115=CARTESIAN_POINT('Ctrl Pts',(25.0285089498922,5.8595306315681,0.));
#214116=CARTESIAN_POINT('Ctrl Pts',(25.0078528200558,5.84107051963074,0.));
#214117=CARTESIAN_POINT('Ctrl Pts',(24.9872081752709,5.82270406744214,0.));
#214118=CARTESIAN_POINT('Ctrl Pts',(24.9665754954462,5.80443138549747,0.));
#214119=CARTESIAN_POINT('Ctrl Pts',(24.9459552293308,5.78625257775703,0.));
#214120=CARTESIAN_POINT('Ctrl Pts',(24.9253478043632,5.76816774342236,0.));
#214121=CARTESIAN_POINT('Ctrl Pts',(24.9047536376467,5.75017697890813,0.));
#214122=CARTESIAN_POINT('Ctrl Pts',(24.8841731467219,5.73228037976927,0.));
#214123=CARTESIAN_POINT('Ctrl Pts',(24.8636067597677,5.71447804252019,0.));
#214124=CARTESIAN_POINT('Ctrl Pts',(24.8430549277634,5.6967700667943,0.));
#214125=CARTESIAN_POINT('Ctrl Pts',(24.822518122386,5.67915655496524,0.));
#214126=CARTESIAN_POINT('Ctrl Pts',(24.8019968304618,5.66163761114903,0.));
#214127=CARTESIAN_POINT('Ctrl Pts',(24.7814915496728,5.64421334042248,0.));
#214128=CARTESIAN_POINT('Ctrl Pts',(24.76100278357,5.62688384790919,0.));
#214129=CARTESIAN_POINT('Ctrl Pts',(24.7405310372736,5.60964923798495,0.));
#214130=CARTESIAN_POINT('Ctrl Pts',(24.7200768119079,5.59250961323995,0.));
#214131=CARTESIAN_POINT('Ctrl Pts',(24.6996406035507,5.57546507427767,0.));
#214132=CARTESIAN_POINT('Ctrl Pts',(24.6792229061785,5.55851572025389,0.));
#214133=CARTESIAN_POINT('Ctrl Pts',(24.6588242134733,5.54166164919593,0.));
#214134=CARTESIAN_POINT('Ctrl Pts',(24.6384450211466,5.52490295840996,0.));
#214135=CARTESIAN_POINT('Ctrl Pts',(24.618085828918,5.50823974481959,0.));
#214136=CARTESIAN_POINT('Ctrl Pts',(24.5977471429365,5.49167210537235,0.));
#214137=CARTESIAN_POINT('Ctrl Pts',(24.5774294770329,5.47520013724403,0.));
#214138=CARTESIAN_POINT('Ctrl Pts',(24.5571333514841,5.45882393762244,0.));
#214139=CARTESIAN_POINT('Ctrl Pts',(24.5368592922861,5.44254360356866,0.));
#214140=CARTESIAN_POINT('Ctrl Pts',(24.5166078302107,5.42635923183411,0.));
#214141=CARTESIAN_POINT('Ctrl Pts',(24.4963794999831,5.41027091869242,0.));
#214142=CARTESIAN_POINT('Ctrl Pts',(24.4761748393322,5.39427875973831,0.));
#214143=CARTESIAN_POINT('Ctrl Pts',(24.4559943883159,5.37838284973706,0.));
#214144=CARTESIAN_POINT('Ctrl Pts',(24.4358386899152,5.36258328273639,0.));
#214145=CARTESIAN_POINT('Ctrl Pts',(24.4157082904615,5.34688015213546,0.));
#214146=CARTESIAN_POINT('Ctrl Pts',(24.3956037401293,5.33127355076037,0.));
#214147=CARTESIAN_POINT('Ctrl Pts',(24.3755255933917,5.31576357092525,0.));
#214148=CARTESIAN_POINT('Ctrl Pts',(24.3554744095075,5.30035030449059,0.));
#214149=CARTESIAN_POINT('Ctrl Pts',(24.3354507529415,5.28503384290644,0.));
#214150=CARTESIAN_POINT('Ctrl Pts',(24.3154551932222,5.26981427718796,0.));
#214151=CARTESIAN_POINT('Ctrl Pts',(24.2954883048448,5.25469169788856,0.));
#214152=CARTESIAN_POINT('Ctrl Pts',(24.2755506671526,5.23966619506289,0.));
#214153=CARTESIAN_POINT('Ctrl Pts',(24.2556428642294,5.22473785822441,0.));
#214154=CARTESIAN_POINT('Ctrl Pts',(24.2357654847765,5.20990677629173,0.));
#214155=CARTESIAN_POINT('Ctrl Pts',(24.215919122017,5.19517303753643,0.));
#214156=CARTESIAN_POINT('Ctrl Pts',(24.1961043738754,5.18053672961392,0.));
#214157=CARTESIAN_POINT('Ctrl Pts',(24.1763218431343,5.16599793957979,0.));
#214158=CARTESIAN_POINT('Ctrl Pts',(24.156572137597,5.15155675390075,0.));
#214159=CARTESIAN_POINT('Ctrl Pts',(24.1368558702443,5.13721325845745,0.));
#214160=CARTESIAN_POINT('Ctrl Pts',(24.117173659394,5.1229675385386,0.));
#214161=CARTESIAN_POINT('Ctrl Pts',(24.0975261288446,5.10881967883132,0.));
#214162=CARTESIAN_POINT('Ctrl Pts',(24.0779139079266,5.09476976342625,0.));
#214163=CARTESIAN_POINT('Ctrl Pts',(24.0583376315638,5.08081787581277,0.));
#214164=CARTESIAN_POINT('Ctrl Pts',(24.0387979403268,5.06696409886641,0.));
#214165=CARTESIAN_POINT('Ctrl Pts',(24.0192954804896,5.05320851483065,0.));
#214166=CARTESIAN_POINT('Ctrl Pts',(23.9998309040746,5.03955120528521,0.));
#214167=CARTESIAN_POINT('Ctrl Pts',(23.9804048689227,5.02599225112454,0.));
#214168=CARTESIAN_POINT('Ctrl Pts',(23.961018038827,5.01253173257453,0.));
#214169=CARTESIAN_POINT('Ctrl Pts',(23.9416710836529,4.99916972919307,0.));
#214170=CARTESIAN_POINT('Ctrl Pts',(23.9223646794592,4.98590631986533,0.));
#214171=CARTESIAN_POINT('Ctrl Pts',(23.9030995086163,4.97274158279227,0.));
#214172=CARTESIAN_POINT('Ctrl Pts',(23.8838762599218,4.95967559546561,0.));
#214173=CARTESIAN_POINT('Ctrl Pts',(23.8646956287168,4.9467084346586,0.));
#214174=CARTESIAN_POINT('Ctrl Pts',(23.8455583170057,4.93384017643432,0.));
#214175=CARTESIAN_POINT('Ctrl Pts',(23.8264650335717,4.92107089613969,0.));
#214176=CARTESIAN_POINT('Ctrl Pts',(23.8074164940896,4.90840066839344,0.));
#214177=CARTESIAN_POINT('Ctrl Pts',(23.7884134212384,4.89582956706775,0.));
#214178=CARTESIAN_POINT('Ctrl Pts',(23.7694565448049,4.88335766525573,0.));
#214179=CARTESIAN_POINT('Ctrl Pts',(23.7505466018245,4.87098503527152,0.));
#214180=CARTESIAN_POINT('Ctrl Pts',(23.7316843367313,4.85871174865499,0.));
#214181=CARTESIAN_POINT('Ctrl Pts',(23.7128705015017,4.84653787616426,0.));
#214182=CARTESIAN_POINT('Ctrl Pts',(23.6941058557971,4.83446348776266,0.));
#214183=CARTESIAN_POINT('Ctrl Pts',(23.675391167102,4.82248865259562,0.));
#214184=CARTESIAN_POINT('Ctrl Pts',(23.6567272108628,4.81061343896432,0.));
#214185=CARTESIAN_POINT('Ctrl Pts',(23.6381147706579,4.7988379143322,0.));
#214186=CARTESIAN_POINT('Ctrl Pts',(23.6195546383624,4.78716214532098,0.));
#214187=CARTESIAN_POINT('Ctrl Pts',(23.6010476143099,4.77558619769872,0.));
#214188=CARTESIAN_POINT('Ctrl Pts',(23.5825945074535,4.76411013636251,0.));
#214189=CARTESIAN_POINT('Ctrl Pts',(23.5641961355168,4.75273402530617,0.));
#214190=CARTESIAN_POINT('Ctrl Pts',(23.545853325171,4.74145792760699,0.));
#214191=CARTESIAN_POINT('Ctrl Pts',(23.5275669122372,4.7302819054303,0.));
#214192=CARTESIAN_POINT('Ctrl Pts',(23.509337741878,4.71920602001902,0.));
#214193=CARTESIAN_POINT('Ctrl Pts',(23.491166668789,4.70823033167819,0.));
#214194=CARTESIAN_POINT('Ctrl Pts',(23.4730545573853,4.69735489975024,0.));
#214195=CARTESIAN_POINT('Ctrl Pts',(23.455002281986,4.68657978258303,0.));
#214196=CARTESIAN_POINT('Ctrl Pts',(23.4370107270451,4.67590503753059,0.));
#214197=CARTESIAN_POINT('Ctrl Pts',(23.4190807873803,4.6653307209467,0.));
#214198=CARTESIAN_POINT('Ctrl Pts',(23.4012133683959,4.65485688816924,0.));
#214199=CARTESIAN_POINT('Ctrl Pts',(23.3834093863068,4.6444835934993,0.));
#214200=CARTESIAN_POINT('Ctrl Pts',(23.3656697683489,4.63421089016541,0.));
#214201=CARTESIAN_POINT('Ctrl Pts',(23.3479954530272,4.62403883030805,0.));
#214202=CARTESIAN_POINT('Ctrl Pts',(23.3303873903938,4.6139674649783,0.));
#214203=CARTESIAN_POINT('Ctrl Pts',(23.3128465423115,4.60399684412163,0.));
#214204=CARTESIAN_POINT('Ctrl Pts',(23.2953738827191,4.5941270165575,0.));
#214205=CARTESIAN_POINT('Ctrl Pts',(23.2779703978876,4.5843580299469,0.));
#214206=CARTESIAN_POINT('Ctrl Pts',(23.2606370866866,4.57468993076097,0.));
#214207=CARTESIAN_POINT('Ctrl Pts',(23.2433749609131,4.56512276427839,0.));
#214208=CARTESIAN_POINT('Ctrl Pts',(23.2261850456064,4.55565657456975,0.));
#214209=CARTESIAN_POINT('Ctrl Pts',(23.2090683793629,4.54629140447544,0.));
#214210=CARTESIAN_POINT('Ctrl Pts',(23.1920260146465,4.53702729557566,0.));
#214211=CARTESIAN_POINT('Ctrl Pts',(23.1750590180908,4.52786428815015,0.));
#214212=CARTESIAN_POINT('Ctrl Pts',(23.1581684708761,4.51880242116748,0.));
#214213=CARTESIAN_POINT('Ctrl Pts',(23.1413554691123,4.5098417322706,0.));
#214214=CARTESIAN_POINT('Ctrl Pts',(23.1246211242115,4.50098225775171,0.));
#214215=CARTESIAN_POINT('Ctrl Pts',(23.1079665632636,4.49222403252216,0.));
#214216=CARTESIAN_POINT('Ctrl Pts',(23.0913929293922,4.48356709006788,0.));
#214217=CARTESIAN_POINT('Ctrl Pts',(23.0749013821881,4.47501146242856,0.));
#214218=CARTESIAN_POINT('Ctrl Pts',(23.0584930981732,4.46655718018231,0.));
#214219=CARTESIAN_POINT('Ctrl Pts',(23.0421692712467,4.45820427241683,0.));
#214220=CARTESIAN_POINT('Ctrl Pts',(23.0259311131392,4.44995276669687,0.));
#214221=CARTESIAN_POINT('Ctrl Pts',(23.0097798538395,4.44180268901643,0.));
#214222=CARTESIAN_POINT('Ctrl Pts',(22.9937167421006,4.43375406376879,0.));
#214223=CARTESIAN_POINT('Ctrl Pts',(22.977743046002,4.42580691372752,0.));
#214224=CARTESIAN_POINT('Ctrl Pts',(22.9618600534866,4.41796126001302,0.));
#214225=CARTESIAN_POINT('Ctrl Pts',(22.9460690729093,4.41021712205554,0.));
#214226=CARTESIAN_POINT('Ctrl Pts',(22.930371433555,4.40257451754324,0.));
#214227=CARTESIAN_POINT('Ctrl Pts',(22.9147684862426,4.39503346238473,0.));
#214228=CARTESIAN_POINT('Ctrl Pts',(22.8992616040108,4.38759397068406,0.));
#214229=CARTESIAN_POINT('Ctrl Pts',(22.8838521827701,4.38025605470093,0.));
#214230=CARTESIAN_POINT('Ctrl Pts',(22.8685416419725,4.37301972480746,0.));
#214231=CARTESIAN_POINT('Ctrl Pts',(22.8533314252422,4.36588498942997,0.));
#214232=CARTESIAN_POINT('Ctrl Pts',(22.8382230011184,4.35885185500546,0.));
#214233=CARTESIAN_POINT('Ctrl Pts',(22.8232178638876,4.35192032594791,0.));
#214234=CARTESIAN_POINT('Ctrl Pts',(22.8083175343791,4.34509040460062,0.));
#214235=CARTESIAN_POINT('Ctrl Pts',(22.7935235607806,4.33836209118446,0.));
#214236=CARTESIAN_POINT('Ctrl Pts',(22.7788375194076,4.3317353837319,0.));
#214237=CARTESIAN_POINT('Ctrl Pts',(22.7642610156475,4.32521027803754,0.));
#214238=CARTESIAN_POINT('Ctrl Pts',(22.7497956849848,4.31878676761235,0.));
#214239=CARTESIAN_POINT('Ctrl Pts',(22.7354431939926,4.31246484362549,0.));
#214240=CARTESIAN_POINT('Ctrl Pts',(22.7212052413386,4.30624449484069,0.));
#214241=CARTESIAN_POINT('Ctrl Pts',(22.7070835587564,4.3001257075406,0.));
#214242=CARTESIAN_POINT('Ctrl Pts',(22.6930799122548,4.29410846547056,0.));
#214243=CARTESIAN_POINT('Ctrl Pts',(22.6791961033537,4.28819274977763,0.));
#214244=CARTESIAN_POINT('Ctrl Pts',(22.6654339703109,4.28237853894059,0.));
#214245=CARTESIAN_POINT('Ctrl Pts',(22.6517953893303,4.2766658086912,0.));
#214246=CARTESIAN_POINT('Ctrl Pts',(22.6382822758172,4.27105453193004,0.));
#214247=CARTESIAN_POINT('Ctrl Pts',(22.6248965859977,4.26554467865576,0.));
#214248=CARTESIAN_POINT('Ctrl Pts',(22.6116403184821,4.26013621588305,0.));
#214249=CARTESIAN_POINT('Ctrl Pts',(22.5985155158636,4.25482910755481,0.));
#214250=CARTESIAN_POINT('Ctrl Pts',(22.5855242662477,4.24962331444177,0.));
#214251=CARTESIAN_POINT('Ctrl Pts',(22.572668704992,4.24451879404851,0.));
#214252=CARTESIAN_POINT('Ctrl Pts',(22.5599510166429,4.23951550052523,0.));
#214253=CARTESIAN_POINT('Ctrl Pts',(22.5473734368086,4.23461338456712,0.));
#214254=CARTESIAN_POINT('Ctrl Pts',(22.5349382540588,4.22981239330733,0.));
#214255=CARTESIAN_POINT('Ctrl Pts',(22.5226478117886,4.22511247020041,0.));
#214256=CARTESIAN_POINT('Ctrl Pts',(22.5105045108881,4.22051355490196,0.));
#214257=CARTESIAN_POINT('Ctrl Pts',(22.4985108124228,4.21601558313906,0.));
#214258=CARTESIAN_POINT('Ctrl Pts',(22.4866692403147,4.21161848657428,0.));
#214259=CARTESIAN_POINT('Ctrl Pts',(22.4749823839917,4.20732219265649,0.));
#214260=CARTESIAN_POINT('Ctrl Pts',(22.4634529011437,4.20312662448174,0.));
#214261=CARTESIAN_POINT('Ctrl Pts',(22.4520835205422,4.19903170066358,0.));
#214262=CARTESIAN_POINT('Ctrl Pts',(22.4408770448917,4.1950373351886,0.));
#214263=CARTESIAN_POINT('Ctrl Pts',(22.4298363535416,4.19114343726932,0.));
#214264=CARTESIAN_POINT('Ctrl Pts',(22.4189644056109,4.18734991117707,0.));
#214265=CARTESIAN_POINT('Ctrl Pts',(22.4082642454448,4.18365665600839,0.));
#214266=CARTESIAN_POINT('Ctrl Pts',(22.3977390078074,4.18006356544879,0.));
#214267=CARTESIAN_POINT('Ctrl Pts',(22.3873919231339,4.17657052752834,0.));
#214268=CARTESIAN_POINT('Ctrl Pts',(22.3772263228624,4.17317742436162,0.));
#214269=CARTESIAN_POINT('Ctrl Pts',(22.3672456427605,4.1698841319947,0.));
#214270=CARTESIAN_POINT('Ctrl Pts',(22.3574534257397,4.16669052026602,0.));
#214271=CARTESIAN_POINT('Ctrl Pts',(22.3478533253886,4.1635964526318,0.));
#214272=CARTESIAN_POINT('Ctrl Pts',(22.3384491078599,4.16060178604154,0.));
#214273=CARTESIAN_POINT('Ctrl Pts',(22.3292446628957,4.15770637047882,0.));
#214274=CARTESIAN_POINT('Ctrl Pts',(22.3202440186979,4.15491004835278,0.));
#214275=CARTESIAN_POINT('Ctrl Pts',(22.3114513545186,4.15221265396993,0.));
#214276=CARTESIAN_POINT('Ctrl Pts',(22.3028710166935,4.14961401285526,0.));
#214277=CARTESIAN_POINT('Ctrl Pts',(22.2945075198468,4.14711394168559,0.));
#214278=CARTESIAN_POINT('Ctrl Pts',(22.2863655389167,4.14471224859295,0.));
#214279=CARTESIAN_POINT('Ctrl Pts',(22.2784499072026,4.14240873321982,0.));
#214280=CARTESIAN_POINT('Ctrl Pts',(22.2707656042456,4.14020318715988,0.));
#214281=CARTESIAN_POINT('Ctrl Pts',(22.263317791397,4.13809539255419,0.));
#214282=CARTESIAN_POINT('Ctrl Pts',(22.2561118708422,4.13608511977226,0.));
#214283=CARTESIAN_POINT('Ctrl Pts',(22.2491535317789,4.13417212558809,0.));
#214284=CARTESIAN_POINT('Ctrl Pts',(22.2424488153523,4.1323561506016,0.));
#214285=CARTESIAN_POINT('Ctrl Pts',(22.2360040565534,4.13063692157499,0.));
#214286=CARTESIAN_POINT('Ctrl Pts',(22.2298258043947,4.12901415463379,0.));
#214287=CARTESIAN_POINT('Ctrl Pts',(22.2239207458781,4.127487558301,0.));
#214288=CARTESIAN_POINT('Ctrl Pts',(22.2182956401341,4.126056836133,0.));
#214289=CARTESIAN_POINT('Ctrl Pts',(22.2129576146671,4.12472167516602,0.));
#214290=CARTESIAN_POINT('Ctrl Pts',(22.2079143941719,4.12348173702025,0.));
#214291=CARTESIAN_POINT('Ctrl Pts',(22.2031746532106,4.12233664408237,0.));
#214292=CARTESIAN_POINT('Ctrl Pts',(22.1987479618246,4.12128598183533,0.));
#214293=CARTESIAN_POINT('Ctrl Pts',(22.1946440958098,4.12032932637738,0.));
#214294=CARTESIAN_POINT('Ctrl Pts',(22.1908725908525,4.11946626228623,0.));
#214295=CARTESIAN_POINT('Ctrl Pts',(22.1874419861496,4.11869641271752,0.));
#214296=CARTESIAN_POINT('Ctrl Pts',(22.1843613164855,4.11801938107464,0.));
#214297=CARTESIAN_POINT('Ctrl Pts',(22.1816414985788,4.11743469691765,0.));
#214298=CARTESIAN_POINT('Ctrl Pts',(22.179297473024,4.11694173195041,0.));
#214299=CARTESIAN_POINT('Ctrl Pts',(22.177347426894,4.11653973150558,0.));
#214300=CARTESIAN_POINT('Ctrl Pts',(22.1758088296598,4.11622797217066,0.));
#214301=CARTESIAN_POINT('Ctrl Pts',(22.1746949858773,4.11600589882768,0.));
#214302=CARTESIAN_POINT('Ctrl Pts',(22.174148802123,4.11589976826061,0.));
#214303=CARTESIAN_POINT('Ctrl Pts',(22.1739341411684,4.1158603587821,0.));
#214304=CARTESIAN_POINT('Ctrl Pts',(22.1738776823239,4.11585194677412,0.));
#214305=CARTESIAN_POINT('Ctrl Pts',(22.1738711152697,4.11585220600461,0.));
#214306=CARTESIAN_POINT('',(21.624941921198,4.01396149767428,0.));
#214307=CARTESIAN_POINT('',(11.0869355576349,2.05792610300232,0.));
#214308=CARTESIAN_POINT('',(21.2226420728916,3.44230496120419,0.));
#214309=CARTESIAN_POINT('Origin',(21.7161918885402,3.52235856495312,0.));
#214310=CARTESIAN_POINT('',(21.3904321633055,2.16781269186828,0.));
#214311=CARTESIAN_POINT('Origin',(7.7715611723761E-13,7.16093850883226E-14,
0.));
#214312=CARTESIAN_POINT('',(21.9269795755927,1.71975774210841,0.));
#214313=CARTESIAN_POINT('Origin',(21.8878840740801,2.21822694051638,0.));
#214314=CARTESIAN_POINT('',(22.4835757167854,1.76341220531179,0.));
#214315=CARTESIAN_POINT('',(10.7170877657712,0.840553282521227,0.));
#214316=CARTESIAN_POINT('',(25.991588367311,0.661312440730894,0.));
#214317=CARTESIAN_POINT('Ctrl Pts',(22.4835757167854,1.76341220531179,0.));
#214318=CARTESIAN_POINT('Ctrl Pts',(22.483581992979,1.76341415538764,0.));
#214319=CARTESIAN_POINT('Ctrl Pts',(22.4836387052232,1.7634206426357,0.));
#214320=CARTESIAN_POINT('Ctrl Pts',(22.4838562517069,1.76343813434565,0.));
#214321=CARTESIAN_POINT('Ctrl Pts',(22.4844112933129,1.76347698284792,0.));
#214322=CARTESIAN_POINT('Ctrl Pts',(22.4855446605991,1.76355076045546,0.));
#214323=CARTESIAN_POINT('Ctrl Pts',(22.4871115206571,1.76364784232963,0.));
#214324=CARTESIAN_POINT('Ctrl Pts',(22.4890991659478,1.76376424879505,0.));
#214325=CARTESIAN_POINT('Ctrl Pts',(22.4914909094908,1.76389475965724,0.));
#214326=CARTESIAN_POINT('Ctrl Pts',(22.4942693792449,1.76403393880301,0.));
#214327=CARTESIAN_POINT('Ctrl Pts',(22.4974203063191,1.76417731243462,0.));
#214328=CARTESIAN_POINT('Ctrl Pts',(22.5009332677316,1.76432160068726,0.));
#214329=CARTESIAN_POINT('Ctrl Pts',(22.5047996391978,1.76446408210366,0.));
#214330=CARTESIAN_POINT('Ctrl Pts',(22.5090112700212,1.76460218257323,0.));
#214331=CARTESIAN_POINT('Ctrl Pts',(22.5135590569554,1.76473303281159,0.));
#214332=CARTESIAN_POINT('Ctrl Pts',(22.5184336670207,1.76485369319896,0.));
#214333=CARTESIAN_POINT('Ctrl Pts',(22.5236259635515,1.76496128643369,0.));
#214334=CARTESIAN_POINT('Ctrl Pts',(22.529127665298,1.76505320262752,0.));
#214335=CARTESIAN_POINT('Ctrl Pts',(22.5349313983571,1.7651271156325,0.));
#214336=CARTESIAN_POINT('Ctrl Pts',(22.5410303590891,1.76518087841493,0.));
#214337=CARTESIAN_POINT('Ctrl Pts',(22.5474180954006,1.76521245524047,0.));
#214338=CARTESIAN_POINT('Ctrl Pts',(22.5540882235837,1.76521983384063,0.));
#214339=CARTESIAN_POINT('Ctrl Pts',(22.5610344912501,1.7652010450045,0.));
#214340=CARTESIAN_POINT('Ctrl Pts',(22.5682508499873,1.76515418518829,0.));
#214341=CARTESIAN_POINT('Ctrl Pts',(22.5757315316355,1.76507744026747,0.));
#214342=CARTESIAN_POINT('Ctrl Pts',(22.5834711038024,1.76496910283089,0.));
#214343=CARTESIAN_POINT('Ctrl Pts',(22.5914644078106,1.76482755288411,0.));
#214344=CARTESIAN_POINT('Ctrl Pts',(22.5997065145638,1.76465124413556,0.));
#214345=CARTESIAN_POINT('Ctrl Pts',(22.6081926681342,1.76443868648015,0.));
#214346=CARTESIAN_POINT('Ctrl Pts',(22.6169182517693,1.76418843543739,0.));
#214347=CARTESIAN_POINT('Ctrl Pts',(22.6258787994847,1.76389909571402,0.));
#214348=CARTESIAN_POINT('Ctrl Pts',(22.635069997936,1.76356932176272,0.));
#214349=CARTESIAN_POINT('Ctrl Pts',(22.6444876940425,1.76319782013914,0.));
#214350=CARTESIAN_POINT('Ctrl Pts',(22.6541278938413,1.76278334912559,0.));
#214351=CARTESIAN_POINT('Ctrl Pts',(22.6639867471756,1.76232471392568,0.));
#214352=CARTESIAN_POINT('Ctrl Pts',(22.6740605356699,1.76182076289525,0.));
#214353=CARTESIAN_POINT('Ctrl Pts',(22.6843456585245,1.76127038310613,0.));
#214354=CARTESIAN_POINT('Ctrl Pts',(22.6948386219843,1.76067249704884,0.));
#214355=CARTESIAN_POINT('Ctrl Pts',(22.7055360375481,1.76002606202399,0.));
#214356=CARTESIAN_POINT('Ctrl Pts',(22.7164346186007,1.75933006905924,0.));
#214357=CARTESIAN_POINT('Ctrl Pts',(22.7275311777305,1.75858354204635,0.));
#214358=CARTESIAN_POINT('Ctrl Pts',(22.7388226235565,1.75778553673249,0.));
#214359=CARTESIAN_POINT('Ctrl Pts',(22.7503059556455,1.75693513908911,0.));
#214360=CARTESIAN_POINT('Ctrl Pts',(22.7619782595013,1.75603146371641,0.));
#214361=CARTESIAN_POINT('Ctrl Pts',(22.7738367016115,1.75507365227127,0.));
#214362=CARTESIAN_POINT('Ctrl Pts',(22.7858785242358,1.7540608718293,0.));
#214363=CARTESIAN_POINT('Ctrl Pts',(22.7981010424312,1.75299231391461,0.));
#214364=CARTESIAN_POINT('Ctrl Pts',(22.8105016414712,1.7518671936559,0.));
#214365=CARTESIAN_POINT('Ctrl Pts',(22.8230777741285,1.75068474890884,0.));
#214366=CARTESIAN_POINT('Ctrl Pts',(22.8358269579854,1.74944423940117,0.));
#214367=CARTESIAN_POINT('Ctrl Pts',(22.8487467728075,1.74814494588492,0.));
#214368=CARTESIAN_POINT('Ctrl Pts',(22.8618348580234,1.74678616930663,0.));
#214369=CARTESIAN_POINT('Ctrl Pts',(22.8750889101696,1.745367229982,0.));
#214370=CARTESIAN_POINT('Ctrl Pts',(22.8885066803351,1.74388746677702,0.));
#214371=CARTESIAN_POINT('Ctrl Pts',(22.9020859716144,1.74234623630079,0.));
#214372=CARTESIAN_POINT('Ctrl Pts',(22.9158246373365,1.74074291231057,0.));
#214373=CARTESIAN_POINT('Ctrl Pts',(22.9297205792587,1.73907688511665,0.));
#214374=CARTESIAN_POINT('Ctrl Pts',(22.9437717457825,1.73734756100038,0.));
#214375=CARTESIAN_POINT('Ctrl Pts',(22.9579761301062,1.73555436162771,0.));
#214376=CARTESIAN_POINT('Ctrl Pts',(22.9723317685688,1.73369672350818,0.));
#214377=CARTESIAN_POINT('Ctrl Pts',(22.9868367391978,1.73177409750194,0.));
#214378=CARTESIAN_POINT('Ctrl Pts',(23.0014891601891,1.72978594832137,0.));
#214379=CARTESIAN_POINT('Ctrl Pts',(23.0162871884167,1.72773175404703,0.));
#214380=CARTESIAN_POINT('Ctrl Pts',(23.031229017888,1.72561100564033,0.));
#214381=CARTESIAN_POINT('Ctrl Pts',(23.0463128785528,1.72342320653731,0.));
#214382=CARTESIAN_POINT('Ctrl Pts',(23.0615370351559,1.72116787225981,0.));
#214383=CARTESIAN_POINT('Ctrl Pts',(23.0768997860709,1.71884453003027,0.));
#214384=CARTESIAN_POINT('Ctrl Pts',(23.0923994621216,1.71645271839311,0.));
#214385=CARTESIAN_POINT('Ctrl Pts',(23.1080344254291,1.71399198684725,0.));
#214386=CARTESIAN_POINT('Ctrl Pts',(23.1238030684929,1.71146189552192,0.));
#214387=CARTESIAN_POINT('Ctrl Pts',(23.1397038132358,1.7088620148546,0.));
#214388=CARTESIAN_POINT('Ctrl Pts',(23.1557351100613,1.70619192527847,0.));
#214389=CARTESIAN_POINT('Ctrl Pts',(23.1718954368749,1.70345121691259,0.));
#214390=CARTESIAN_POINT('Ctrl Pts',(23.1881832981848,1.70063948926988,0.));
#214391=CARTESIAN_POINT('Ctrl Pts',(23.2045972243765,1.69775635099425,0.));
#214392=CARTESIAN_POINT('Ctrl Pts',(23.2211357709374,1.69480141959946,0.));
#214393=CARTESIAN_POINT('Ctrl Pts',(23.2377975177014,1.69177432121716,0.));
#214394=CARTESIAN_POINT('Ctrl Pts',(23.2545810680536,1.6886746903491,0.));
#214395=CARTESIAN_POINT('Ctrl Pts',(23.2714850482245,1.68550216963275,0.));
#214396=CARTESIAN_POINT('Ctrl Pts',(23.2885081066949,1.68225640962181,0.));
#214397=CARTESIAN_POINT('Ctrl Pts',(23.3056489135611,1.67893706857123,0.));
#214398=CARTESIAN_POINT('Ctrl Pts',(23.3229061599145,1.67554381222988,0.));
#214399=CARTESIAN_POINT('Ctrl Pts',(23.3402785571866,1.67207631363905,0.));
#214400=CARTESIAN_POINT('Ctrl Pts',(23.3577648365747,1.66853425293978,0.));
#214401=CARTESIAN_POINT('Ctrl Pts',(23.375363748555,1.66491731718864,0.));
#214402=CARTESIAN_POINT('Ctrl Pts',(23.3930740623622,1.66122520018008,0.));
#214403=CARTESIAN_POINT('Ctrl Pts',(23.4108945654803,1.65745760227507,0.));
#214404=CARTESIAN_POINT('Ctrl Pts',(23.4288240631034,1.6536142302373,0.));
#214405=CARTESIAN_POINT('Ctrl Pts',(23.446861377656,1.6496947970734,0.));
#214406=CARTESIAN_POINT('Ctrl Pts',(23.4650053483919,1.64569902187608,0.));
#214407=CARTESIAN_POINT('Ctrl Pts',(23.4832548309638,1.64162662967525,0.));
#214408=CARTESIAN_POINT('Ctrl Pts',(23.5016086970006,1.63747735129474,0.));
#214409=CARTESIAN_POINT('Ctrl Pts',(23.5200658336624,1.63325092321731,0.));
#214410=CARTESIAN_POINT('Ctrl Pts',(23.5386251432278,1.62894708745231,0.));
#214411=CARTESIAN_POINT('Ctrl Pts',(23.5572855427617,1.62456559140072,0.));
#214412=CARTESIAN_POINT('Ctrl Pts',(23.5760459637608,1.62010618772869,0.));
#214413=CARTESIAN_POINT('Ctrl Pts',(23.5949053517996,1.61556863424697,0.));
#214414=CARTESIAN_POINT('Ctrl Pts',(23.6138626661644,1.61095269379773,0.));
#214415=CARTESIAN_POINT('Ctrl Pts',(23.6329168794916,1.60625813414666,0.));
#214416=CARTESIAN_POINT('Ctrl Pts',(23.6520669774863,1.60148472786588,0.));
#214417=CARTESIAN_POINT('Ctrl Pts',(23.6713119586302,1.59663225222459,0.));
#214418=CARTESIAN_POINT('Ctrl Pts',(23.6906508338832,1.59170048908631,0.));
#214419=CARTESIAN_POINT('Ctrl Pts',(23.7100826263835,1.58668922481222,0.));
#214420=CARTESIAN_POINT('Ctrl Pts',(23.7296063711308,1.58159825017362,0.));
#214421=CARTESIAN_POINT('Ctrl Pts',(23.7492211147369,1.57642736025251,0.));
#214422=CARTESIAN_POINT('Ctrl Pts',(23.7689259151869,1.57117635434412,0.));
#214423=CARTESIAN_POINT('Ctrl Pts',(23.788719841588,1.56584503586844,0.));
#214424=CARTESIAN_POINT('Ctrl Pts',(23.8086019739192,1.56043321228631,0.));
#214425=CARTESIAN_POINT('Ctrl Pts',(23.8285714027631,1.55494069502628,0.));
#214426=CARTESIAN_POINT('Ctrl Pts',(23.8486272290698,1.5493672994053,0.));
#214427=CARTESIAN_POINT('Ctrl Pts',(23.8687685639635,1.54371284453978,0.));
#214428=CARTESIAN_POINT('Ctrl Pts',(23.8889945285313,1.53797715326748,0.));
#214429=CARTESIAN_POINT('Ctrl Pts',(23.9093042536119,1.53216005207462,0.));
#214430=CARTESIAN_POINT('Ctrl Pts',(23.9296968795761,1.5262613710304,0.));
#214431=CARTESIAN_POINT('Ctrl Pts',(23.9501715561038,1.52028094372806,0.));
#214432=CARTESIAN_POINT('Ctrl Pts',(23.9707274420145,1.51421860720628,0.));
#214433=CARTESIAN_POINT('Ctrl Pts',(23.991363705093,1.50807420187703,0.));
#214434=CARTESIAN_POINT('Ctrl Pts',(24.0120795219086,1.50184757146099,0.));
#214435=CARTESIAN_POINT('Ctrl Pts',(24.0328740776331,1.49553856292798,0.));
#214436=CARTESIAN_POINT('Ctrl Pts',(24.053746565843,1.48914702644883,0.));
#214437=CARTESIAN_POINT('Ctrl Pts',(24.074696188353,1.4826728153368,0.));
#214438=CARTESIAN_POINT('Ctrl Pts',(24.0957221550782,1.47611578597742,0.));
#214439=CARTESIAN_POINT('Ctrl Pts',(24.1168236838827,1.46947579776992,0.));
#214440=CARTESIAN_POINT('Ctrl Pts',(24.1380000004272,1.46275271307398,0.));
#214441=CARTESIAN_POINT('Ctrl Pts',(24.1592503380105,1.45594639716314,0.));
#214442=CARTESIAN_POINT('Ctrl Pts',(24.1805739374033,1.44905671818721,0.));
#214443=CARTESIAN_POINT('Ctrl Pts',(24.2019700467214,1.44208354711074,0.));
#214444=CARTESIAN_POINT('Ctrl Pts',(24.2234379212978,1.43502675765502,0.));
#214445=CARTESIAN_POINT('Ctrl Pts',(24.2449768235485,1.42788622624851,0.));
#214446=CARTESIAN_POINT('Ctrl Pts',(24.2665860228357,1.42066183198252,0.));
#214447=CARTESIAN_POINT('Ctrl Pts',(24.2882647953214,1.41335345657685,0.));
#214448=CARTESIAN_POINT('Ctrl Pts',(24.3100124238316,1.40596098434341,0.));
#214449=CARTESIAN_POINT('Ctrl Pts',(24.3318281977647,1.3984843021281,0.));
#214450=CARTESIAN_POINT('Ctrl Pts',(24.3537114129877,1.3909232992639,0.));
#214451=CARTESIAN_POINT('Ctrl Pts',(24.37566137173,1.38327786752998,0.));
#214452=CARTESIAN_POINT('Ctrl Pts',(24.3976773824731,1.37554790111608,0.));
#214453=CARTESIAN_POINT('Ctrl Pts',(24.4197587598337,1.36773329659954,0.));
#214454=CARTESIAN_POINT('Ctrl Pts',(24.4419048244524,1.35983395290624,0.));
#214455=CARTESIAN_POINT('Ctrl Pts',(24.4641149028894,1.35184977125645,0.));
#214456=CARTESIAN_POINT('Ctrl Pts',(24.4863883275135,1.34378065512335,0.));
#214457=CARTESIAN_POINT('Ctrl Pts',(24.5087244363856,1.33562651019684,0.));
#214458=CARTESIAN_POINT('Ctrl Pts',(24.5311225731434,1.32738724435326,0.));
#214459=CARTESIAN_POINT('Ctrl Pts',(24.5535820868671,1.31906276763669,0.));
#214460=CARTESIAN_POINT('Ctrl Pts',(24.576102332018,1.31065299222023,0.));
#214461=CARTESIAN_POINT('Ctrl Pts',(24.5986826684025,1.30215783236364,0.));
#214462=CARTESIAN_POINT('Ctrl Pts',(24.6213224611228,1.29357720438108,0.));
#214463=CARTESIAN_POINT('Ctrl Pts',(24.6440210805278,1.28491102661514,0.));
#214464=CARTESIAN_POINT('Ctrl Pts',(24.666777902156,1.2761592194164,0.));
#214465=CARTESIAN_POINT('Ctrl Pts',(24.6895923066837,1.26732170513497,0.));
#214466=CARTESIAN_POINT('Ctrl Pts',(24.7124636797895,1.25839840807415,0.));
#214467=CARTESIAN_POINT('Ctrl Pts',(24.7353914120012,1.24938925444324,0.));
#214468=CARTESIAN_POINT('Ctrl Pts',(24.7583748985439,1.24029417231988,0.));
#214469=CARTESIAN_POINT('Ctrl Pts',(24.78141353918,1.23111309161843,0.));
#214470=CARTESIAN_POINT('Ctrl Pts',(24.8045067380536,1.22184594406527,0.));
#214471=CARTESIAN_POINT('Ctrl Pts',(24.8276539035092,1.21249266318205,0.));
#214472=CARTESIAN_POINT('Ctrl Pts',(24.8508544481973,1.20305318426016,0.));
#214473=CARTESIAN_POINT('Ctrl Pts',(24.8741077892074,1.19352744434059,0.));
#214474=CARTESIAN_POINT('Ctrl Pts',(24.8974133481829,1.18391538220098,0.));
#214475=CARTESIAN_POINT('Ctrl Pts',(24.9207705514449,1.1742169383504,0.));
#214476=CARTESIAN_POINT('Ctrl Pts',(24.9441788300932,1.16443205502852,0.));
#214477=CARTESIAN_POINT('Ctrl Pts',(24.9676376201501,1.15456067621894,0.));
#214478=CARTESIAN_POINT('Ctrl Pts',(24.9911463621431,1.14460274758206,0.));
#214479=CARTESIAN_POINT('Ctrl Pts',(25.0147045006193,1.13455821638536,0.));
#214480=CARTESIAN_POINT('Ctrl Pts',(25.0383114836898,1.12442703144455,0.));
#214481=CARTESIAN_POINT('Ctrl Pts',(25.0619667625336,1.1142091430689,0.));
#214482=CARTESIAN_POINT('Ctrl Pts',(25.085669790968,1.10390450301741,0.));
#214483=CARTESIAN_POINT('Ctrl Pts',(25.1094200248448,1.09351306445299,0.));
#214484=CARTESIAN_POINT('Ctrl Pts',(25.1332169227415,1.08303478197174,0.));
#214485=CARTESIAN_POINT('Ctrl Pts',(25.1570599469311,1.0724696116546,0.));
#214486=CARTESIAN_POINT('Ctrl Pts',(25.1809485642191,1.06181751111754,0.));
#214487=CARTESIAN_POINT('Ctrl Pts',(25.2048822469027,1.05107843957926,0.));
#214488=CARTESIAN_POINT('Ctrl Pts',(25.2288604735087,1.04025235791515,0.));
#214489=CARTESIAN_POINT('Ctrl Pts',(25.2528827300427,1.0293392287683,0.));
#214490=CARTESIAN_POINT('Ctrl Pts',(25.2769485087268,1.01833901642273,0.));
#214491=CARTESIAN_POINT('Ctrl Pts',(25.3010573055557,1.00725168656934,0.));
#214492=CARTESIAN_POINT('Ctrl Pts',(25.3252086182976,0.996077206120921,
0.));
#214493=CARTESIAN_POINT('Ctrl Pts',(25.3494019441444,0.984815543004091,
0.));
#214494=CARTESIAN_POINT('Ctrl Pts',(25.3736367778842,0.97346666600005,0.));
#214495=CARTESIAN_POINT('Ctrl Pts',(25.3979126089155,0.962030544502806,
0.));
#214496=CARTESIAN_POINT('Ctrl Pts',(25.4222289223155,0.950507148596971,
0.));
#214497=CARTESIAN_POINT('Ctrl Pts',(25.4465852044835,0.938896449495636,
0.));
#214498=CARTESIAN_POINT('Ctrl Pts',(25.4709809474996,0.927198419885607,
0.));
#214499=CARTESIAN_POINT('Ctrl Pts',(25.4954156541787,0.915413034335334,
0.));
#214500=CARTESIAN_POINT('Ctrl Pts',(25.5198888424195,0.903540269651155,
0.));
#214501=CARTESIAN_POINT('Ctrl Pts',(25.5444000508223,0.891580105349469,
0.));
#214502=CARTESIAN_POINT('Ctrl Pts',(25.568948840818,0.879532523835094,0.));
#214503=CARTESIAN_POINT('Ctrl Pts',(25.5935347843616,0.867397509339473,
0.));
#214504=CARTESIAN_POINT('Ctrl Pts',(25.618157453608,0.855175047037618,0.));
#214505=CARTESIAN_POINT('Ctrl Pts',(25.6428164100078,0.842865122121547,
0.));
#214506=CARTESIAN_POINT('Ctrl Pts',(25.6675111931957,0.83046771886437,0.));
#214507=CARTESIAN_POINT('Ctrl Pts',(25.6922413110172,0.817982819786722,
0.));
#214508=CARTESIAN_POINT('Ctrl Pts',(25.7170062262474,0.805410404552597,
0.));
#214509=CARTESIAN_POINT('Ctrl Pts',(25.7418053757671,0.792750451613538,
0.));
#214510=CARTESIAN_POINT('Ctrl Pts',(25.7666381946871,0.780002940289028,
0.));
#214511=CARTESIAN_POINT('Ctrl Pts',(25.7915041383304,0.767167852648643,
0.));
#214512=CARTESIAN_POINT('Ctrl Pts',(25.816402705995,0.754245175608291,0.));
#214513=CARTESIAN_POINT('Ctrl Pts',(25.841333461908,0.741234902664698,0.));
#214514=CARTESIAN_POINT('Ctrl Pts',(25.8662960624285,0.728137036485881,
0.));
#214515=CARTESIAN_POINT('Ctrl Pts',(25.8912902615141,0.714951588533756,
0.));
#214516=CARTESIAN_POINT('Ctrl Pts',(25.9163158909645,0.701678575236605,
0.));
#214517=CARTESIAN_POINT('Ctrl Pts',(25.941372847213,0.68831801506568,0.));
#214518=CARTESIAN_POINT('Ctrl Pts',(25.9614434298092,0.677559543215907,
0.));
#214519=CARTESIAN_POINT('Ctrl Pts',(25.9765104298171,0.669451306784419,
0.));
#214520=CARTESIAN_POINT('Ctrl Pts',(25.9865613464809,0.664028313188916,
0.));
#214521=CARTESIAN_POINT('Ctrl Pts',(25.991588367311,0.661312440730894,0.));
#214522=CARTESIAN_POINT('Origin',(0.,0.,0.));
#214523=CARTESIAN_POINT('Origin',(0.,0.,0.));
#214524=CARTESIAN_POINT('',(25.2771067246846,6.08833931617698,0.));
#214525=CARTESIAN_POINT('Origin',(0.,0.,0.));
#214526=CARTESIAN_POINT('Origin',(0.,0.,0.));
#214527=CARTESIAN_POINT('Origin',(0.,0.,0.));
#214528=CARTESIAN_POINT('Origin',(0.,0.,0.));
#214529=CARTESIAN_POINT('Origin',(0.,0.,0.));
#214530=CARTESIAN_POINT('Origin',(0.,0.,0.));
#214531=CARTESIAN_POINT('Origin',(0.,0.,0.));
#214532=CARTESIAN_POINT('Origin',(0.,0.,0.));
#214533=CARTESIAN_POINT('Origin',(0.,0.,0.));
#214534=CARTESIAN_POINT('Origin',(0.,0.,0.));
#214535=CARTESIAN_POINT('Origin',(0.,0.,0.));
#214536=CARTESIAN_POINT('Origin',(0.,0.,0.));
#214537=CARTESIAN_POINT('Origin',(0.,0.,0.));
#214538=CARTESIAN_POINT('Origin',(0.,0.,0.));
#214539=CARTESIAN_POINT('Origin',(0.,0.,0.));
#214540=CARTESIAN_POINT('Origin',(0.,0.,0.));
#214541=CARTESIAN_POINT('Origin',(0.,0.,0.));
#214542=CARTESIAN_POINT('Origin',(0.,0.,0.));
#214543=CARTESIAN_POINT('Origin',(0.,0.,0.));
#214544=CARTESIAN_POINT('Origin',(0.,0.,0.));
#214545=CARTESIAN_POINT('Origin',(0.,0.,0.));
#214546=CARTESIAN_POINT('Origin',(0.,0.,0.));
#214547=CARTESIAN_POINT('Origin',(21.7161918885402,3.52235856495312,0.));
#214548=CARTESIAN_POINT('',(21.624941921198,4.01396149767428,0.));
#214549=CARTESIAN_POINT('',(21.2226420728916,3.44230496120418,0.));
#214550=CARTESIAN_POINT('Origin',(22.1738711152697,4.11585220600461,0.));
#214551=CARTESIAN_POINT('',(22.1738711152697,4.11585220600461,0.));
#214552=CARTESIAN_POINT('Origin',(21.8878840740801,2.21822694051638,0.));
#214553=CARTESIAN_POINT('',(21.3904321633055,2.16781269186828,0.));
#214554=CARTESIAN_POINT('',(21.9269795755927,1.71975774210841,0.));
#214555=CARTESIAN_POINT('Origin',(7.7715611723761E-13,7.16093850883226E-14,
0.));
#214556=CARTESIAN_POINT('Origin',(21.4341755315424,1.68110656504246,0.));
#214557=CARTESIAN_POINT('',(22.4835757167854,1.76341220531179,0.));
#214558=CARTESIAN_POINT('Ctrl Pts',(25.2771067246846,6.08833931617698,0.));
#214559=CARTESIAN_POINT('Ctrl Pts',(25.2771067246846,6.08833931617698,12.));
#214560=CARTESIAN_POINT('Ctrl Pts',(25.2729539149479,6.08441489609824,0.));
#214561=CARTESIAN_POINT('Ctrl Pts',(25.2729539149479,6.08441489609824,12.));
#214562=CARTESIAN_POINT('Ctrl Pts',(25.2646490489816,6.07657531787578,0.));
#214563=CARTESIAN_POINT('Ctrl Pts',(25.2646490489816,6.07657531787578,12.));
#214564=CARTESIAN_POINT('Ctrl Pts',(25.2521940105523,6.06484373634697,0.));
#214565=CARTESIAN_POINT('Ctrl Pts',(25.2521940105523,6.06484373634697,12.));
#214566=CARTESIAN_POINT('Ctrl Pts',(25.2355918138798,6.04925720151412,0.));
#214567=CARTESIAN_POINT('Ctrl Pts',(25.2355918138798,6.04925720151412,12.));
#214568=CARTESIAN_POINT('Ctrl Pts',(25.2148466201368,6.02986667390187,0.));
#214569=CARTESIAN_POINT('Ctrl Pts',(25.2148466201368,6.02986667390187,12.));
#214570=CARTESIAN_POINT('Ctrl Pts',(25.1941090269638,6.0105688180476,0.));
#214571=CARTESIAN_POINT('Ctrl Pts',(25.1941090269638,6.0105688180476,12.));
#214572=CARTESIAN_POINT('Ctrl Pts',(25.1733791296154,5.99136367859839,0.));
#214573=CARTESIAN_POINT('Ctrl Pts',(25.1733791296154,5.99136367859839,12.));
#214574=CARTESIAN_POINT('Ctrl Pts',(25.1526570863065,5.97225131495636,0.));
#214575=CARTESIAN_POINT('Ctrl Pts',(25.1526570863065,5.97225131495636,12.));
#214576=CARTESIAN_POINT('Ctrl Pts',(25.1319431317273,5.95323180187348,0.));
#214577=CARTESIAN_POINT('Ctrl Pts',(25.1319431317273,5.95323180187348,12.));
#214578=CARTESIAN_POINT('Ctrl Pts',(25.1112375971182,5.93430523086776,0.));
#214579=CARTESIAN_POINT('Ctrl Pts',(25.1112375971182,5.93430523086776,12.));
#214580=CARTESIAN_POINT('Ctrl Pts',(25.0905409050863,5.91547170844382,0.));
#214581=CARTESIAN_POINT('Ctrl Pts',(25.0905409050863,5.91547170844382,12.));
#214582=CARTESIAN_POINT('Ctrl Pts',(25.0698535426593,5.89673135155459,0.));
#214583=CARTESIAN_POINT('Ctrl Pts',(25.0698535426593,5.89673135155459,12.));
#214584=CARTESIAN_POINT('Ctrl Pts',(25.0491760405965,5.87808428385329,0.));
#214585=CARTESIAN_POINT('Ctrl Pts',(25.0491760405965,5.87808428385329,12.));
#214586=CARTESIAN_POINT('Ctrl Pts',(25.0285089498922,5.8595306315681,0.));
#214587=CARTESIAN_POINT('Ctrl Pts',(25.0285089498922,5.8595306315681,12.));
#214588=CARTESIAN_POINT('Ctrl Pts',(25.0078528200558,5.84107051963074,0.));
#214589=CARTESIAN_POINT('Ctrl Pts',(25.0078528200558,5.84107051963074,12.));
#214590=CARTESIAN_POINT('Ctrl Pts',(24.9872081752709,5.82270406744214,0.));
#214591=CARTESIAN_POINT('Ctrl Pts',(24.9872081752709,5.82270406744214,12.));
#214592=CARTESIAN_POINT('Ctrl Pts',(24.9665754954462,5.80443138549747,0.));
#214593=CARTESIAN_POINT('Ctrl Pts',(24.9665754954462,5.80443138549747,12.));
#214594=CARTESIAN_POINT('Ctrl Pts',(24.9459552293308,5.78625257775703,0.));
#214595=CARTESIAN_POINT('Ctrl Pts',(24.9459552293308,5.78625257775703,12.));
#214596=CARTESIAN_POINT('Ctrl Pts',(24.9253478043632,5.76816774342236,0.));
#214597=CARTESIAN_POINT('Ctrl Pts',(24.9253478043632,5.76816774342236,12.));
#214598=CARTESIAN_POINT('Ctrl Pts',(24.9047536376467,5.75017697890813,0.));
#214599=CARTESIAN_POINT('Ctrl Pts',(24.9047536376467,5.75017697890813,12.));
#214600=CARTESIAN_POINT('Ctrl Pts',(24.8841731467219,5.73228037976927,0.));
#214601=CARTESIAN_POINT('Ctrl Pts',(24.8841731467219,5.73228037976927,12.));
#214602=CARTESIAN_POINT('Ctrl Pts',(24.8636067597677,5.71447804252019,0.));
#214603=CARTESIAN_POINT('Ctrl Pts',(24.8636067597677,5.71447804252019,12.));
#214604=CARTESIAN_POINT('Ctrl Pts',(24.8430549277634,5.6967700667943,0.));
#214605=CARTESIAN_POINT('Ctrl Pts',(24.8430549277634,5.6967700667943,12.));
#214606=CARTESIAN_POINT('Ctrl Pts',(24.822518122386,5.67915655496524,0.));
#214607=CARTESIAN_POINT('Ctrl Pts',(24.822518122386,5.67915655496524,12.));
#214608=CARTESIAN_POINT('Ctrl Pts',(24.8019968304618,5.66163761114903,0.));
#214609=CARTESIAN_POINT('Ctrl Pts',(24.8019968304618,5.66163761114903,12.));
#214610=CARTESIAN_POINT('Ctrl Pts',(24.7814915496728,5.64421334042248,0.));
#214611=CARTESIAN_POINT('Ctrl Pts',(24.7814915496728,5.64421334042248,12.));
#214612=CARTESIAN_POINT('Ctrl Pts',(24.76100278357,5.62688384790919,0.));
#214613=CARTESIAN_POINT('Ctrl Pts',(24.76100278357,5.62688384790919,12.));
#214614=CARTESIAN_POINT('Ctrl Pts',(24.7405310372736,5.60964923798495,0.));
#214615=CARTESIAN_POINT('Ctrl Pts',(24.7405310372736,5.60964923798495,12.));
#214616=CARTESIAN_POINT('Ctrl Pts',(24.7200768119079,5.59250961323995,0.));
#214617=CARTESIAN_POINT('Ctrl Pts',(24.7200768119079,5.59250961323995,12.));
#214618=CARTESIAN_POINT('Ctrl Pts',(24.6996406035507,5.57546507427767,0.));
#214619=CARTESIAN_POINT('Ctrl Pts',(24.6996406035507,5.57546507427767,12.));
#214620=CARTESIAN_POINT('Ctrl Pts',(24.6792229061785,5.55851572025389,0.));
#214621=CARTESIAN_POINT('Ctrl Pts',(24.6792229061785,5.55851572025389,12.));
#214622=CARTESIAN_POINT('Ctrl Pts',(24.6588242134733,5.54166164919593,0.));
#214623=CARTESIAN_POINT('Ctrl Pts',(24.6588242134733,5.54166164919593,12.));
#214624=CARTESIAN_POINT('Ctrl Pts',(24.6384450211466,5.52490295840996,0.));
#214625=CARTESIAN_POINT('Ctrl Pts',(24.6384450211466,5.52490295840996,12.));
#214626=CARTESIAN_POINT('Ctrl Pts',(24.618085828918,5.50823974481959,0.));
#214627=CARTESIAN_POINT('Ctrl Pts',(24.618085828918,5.50823974481959,12.));
#214628=CARTESIAN_POINT('Ctrl Pts',(24.5977471429365,5.49167210537235,0.));
#214629=CARTESIAN_POINT('Ctrl Pts',(24.5977471429365,5.49167210537235,12.));
#214630=CARTESIAN_POINT('Ctrl Pts',(24.5774294770329,5.47520013724403,0.));
#214631=CARTESIAN_POINT('Ctrl Pts',(24.5774294770329,5.47520013724403,12.));
#214632=CARTESIAN_POINT('Ctrl Pts',(24.5571333514841,5.45882393762244,0.));
#214633=CARTESIAN_POINT('Ctrl Pts',(24.5571333514841,5.45882393762244,12.));
#214634=CARTESIAN_POINT('Ctrl Pts',(24.5368592922861,5.44254360356866,0.));
#214635=CARTESIAN_POINT('Ctrl Pts',(24.5368592922861,5.44254360356866,12.));
#214636=CARTESIAN_POINT('Ctrl Pts',(24.5166078302107,5.42635923183411,0.));
#214637=CARTESIAN_POINT('Ctrl Pts',(24.5166078302107,5.42635923183411,12.));
#214638=CARTESIAN_POINT('Ctrl Pts',(24.4963794999831,5.41027091869242,0.));
#214639=CARTESIAN_POINT('Ctrl Pts',(24.4963794999831,5.41027091869242,12.));
#214640=CARTESIAN_POINT('Ctrl Pts',(24.4761748393322,5.39427875973831,0.));
#214641=CARTESIAN_POINT('Ctrl Pts',(24.4761748393322,5.39427875973831,12.));
#214642=CARTESIAN_POINT('Ctrl Pts',(24.4559943883159,5.37838284973706,0.));
#214643=CARTESIAN_POINT('Ctrl Pts',(24.4559943883159,5.37838284973706,12.));
#214644=CARTESIAN_POINT('Ctrl Pts',(24.4358386899152,5.36258328273639,0.));
#214645=CARTESIAN_POINT('Ctrl Pts',(24.4358386899152,5.36258328273639,12.));
#214646=CARTESIAN_POINT('Ctrl Pts',(24.4157082904615,5.34688015213546,0.));
#214647=CARTESIAN_POINT('Ctrl Pts',(24.4157082904615,5.34688015213546,12.));
#214648=CARTESIAN_POINT('Ctrl Pts',(24.3956037401293,5.33127355076037,0.));
#214649=CARTESIAN_POINT('Ctrl Pts',(24.3956037401293,5.33127355076037,12.));
#214650=CARTESIAN_POINT('Ctrl Pts',(24.3755255933917,5.31576357092525,0.));
#214651=CARTESIAN_POINT('Ctrl Pts',(24.3755255933917,5.31576357092525,12.));
#214652=CARTESIAN_POINT('Ctrl Pts',(24.3554744095075,5.30035030449059,0.));
#214653=CARTESIAN_POINT('Ctrl Pts',(24.3554744095075,5.30035030449059,12.));
#214654=CARTESIAN_POINT('Ctrl Pts',(24.3354507529415,5.28503384290644,0.));
#214655=CARTESIAN_POINT('Ctrl Pts',(24.3354507529415,5.28503384290644,12.));
#214656=CARTESIAN_POINT('Ctrl Pts',(24.3154551932222,5.26981427718796,0.));
#214657=CARTESIAN_POINT('Ctrl Pts',(24.3154551932222,5.26981427718796,12.));
#214658=CARTESIAN_POINT('Ctrl Pts',(24.2954883048448,5.25469169788856,0.));
#214659=CARTESIAN_POINT('Ctrl Pts',(24.2954883048448,5.25469169788856,12.));
#214660=CARTESIAN_POINT('Ctrl Pts',(24.2755506671526,5.23966619506289,0.));
#214661=CARTESIAN_POINT('Ctrl Pts',(24.2755506671526,5.23966619506289,12.));
#214662=CARTESIAN_POINT('Ctrl Pts',(24.2556428642294,5.22473785822441,0.));
#214663=CARTESIAN_POINT('Ctrl Pts',(24.2556428642294,5.22473785822441,12.));
#214664=CARTESIAN_POINT('Ctrl Pts',(24.2357654847765,5.20990677629173,0.));
#214665=CARTESIAN_POINT('Ctrl Pts',(24.2357654847765,5.20990677629173,12.));
#214666=CARTESIAN_POINT('Ctrl Pts',(24.215919122017,5.19517303753643,0.));
#214667=CARTESIAN_POINT('Ctrl Pts',(24.215919122017,5.19517303753643,12.));
#214668=CARTESIAN_POINT('Ctrl Pts',(24.1961043738754,5.18053672961392,0.));
#214669=CARTESIAN_POINT('Ctrl Pts',(24.1961043738754,5.18053672961392,12.));
#214670=CARTESIAN_POINT('Ctrl Pts',(24.1763218431343,5.16599793957979,0.));
#214671=CARTESIAN_POINT('Ctrl Pts',(24.1763218431343,5.16599793957979,12.));
#214672=CARTESIAN_POINT('Ctrl Pts',(24.156572137597,5.15155675390075,0.));
#214673=CARTESIAN_POINT('Ctrl Pts',(24.156572137597,5.15155675390075,12.));
#214674=CARTESIAN_POINT('Ctrl Pts',(24.1368558702443,5.13721325845745,0.));
#214675=CARTESIAN_POINT('Ctrl Pts',(24.1368558702443,5.13721325845745,12.));
#214676=CARTESIAN_POINT('Ctrl Pts',(24.117173659394,5.1229675385386,0.));
#214677=CARTESIAN_POINT('Ctrl Pts',(24.117173659394,5.1229675385386,12.));
#214678=CARTESIAN_POINT('Ctrl Pts',(24.0975261288446,5.10881967883132,0.));
#214679=CARTESIAN_POINT('Ctrl Pts',(24.0975261288446,5.10881967883132,12.));
#214680=CARTESIAN_POINT('Ctrl Pts',(24.0779139079266,5.09476976342625,0.));
#214681=CARTESIAN_POINT('Ctrl Pts',(24.0779139079266,5.09476976342625,12.));
#214682=CARTESIAN_POINT('Ctrl Pts',(24.0583376315638,5.08081787581277,0.));
#214683=CARTESIAN_POINT('Ctrl Pts',(24.0583376315638,5.08081787581277,12.));
#214684=CARTESIAN_POINT('Ctrl Pts',(24.0387979403268,5.06696409886641,0.));
#214685=CARTESIAN_POINT('Ctrl Pts',(24.0387979403268,5.06696409886641,12.));
#214686=CARTESIAN_POINT('Ctrl Pts',(24.0192954804896,5.05320851483065,0.));
#214687=CARTESIAN_POINT('Ctrl Pts',(24.0192954804896,5.05320851483065,12.));
#214688=CARTESIAN_POINT('Ctrl Pts',(23.9998309040746,5.03955120528521,0.));
#214689=CARTESIAN_POINT('Ctrl Pts',(23.9998309040746,5.03955120528521,12.));
#214690=CARTESIAN_POINT('Ctrl Pts',(23.9804048689227,5.02599225112454,0.));
#214691=CARTESIAN_POINT('Ctrl Pts',(23.9804048689227,5.02599225112454,12.));
#214692=CARTESIAN_POINT('Ctrl Pts',(23.961018038827,5.01253173257453,0.));
#214693=CARTESIAN_POINT('Ctrl Pts',(23.961018038827,5.01253173257453,12.));
#214694=CARTESIAN_POINT('Ctrl Pts',(23.9416710836529,4.99916972919307,0.));
#214695=CARTESIAN_POINT('Ctrl Pts',(23.9416710836529,4.99916972919307,12.));
#214696=CARTESIAN_POINT('Ctrl Pts',(23.9223646794592,4.98590631986533,0.));
#214697=CARTESIAN_POINT('Ctrl Pts',(23.9223646794592,4.98590631986533,12.));
#214698=CARTESIAN_POINT('Ctrl Pts',(23.9030995086163,4.97274158279227,0.));
#214699=CARTESIAN_POINT('Ctrl Pts',(23.9030995086163,4.97274158279227,12.));
#214700=CARTESIAN_POINT('Ctrl Pts',(23.8838762599218,4.95967559546561,0.));
#214701=CARTESIAN_POINT('Ctrl Pts',(23.8838762599218,4.95967559546561,12.));
#214702=CARTESIAN_POINT('Ctrl Pts',(23.8646956287168,4.9467084346586,0.));
#214703=CARTESIAN_POINT('Ctrl Pts',(23.8646956287168,4.9467084346586,12.));
#214704=CARTESIAN_POINT('Ctrl Pts',(23.8455583170057,4.93384017643432,0.));
#214705=CARTESIAN_POINT('Ctrl Pts',(23.8455583170057,4.93384017643432,12.));
#214706=CARTESIAN_POINT('Ctrl Pts',(23.8264650335717,4.92107089613969,0.));
#214707=CARTESIAN_POINT('Ctrl Pts',(23.8264650335717,4.92107089613969,12.));
#214708=CARTESIAN_POINT('Ctrl Pts',(23.8074164940896,4.90840066839344,0.));
#214709=CARTESIAN_POINT('Ctrl Pts',(23.8074164940896,4.90840066839344,12.));
#214710=CARTESIAN_POINT('Ctrl Pts',(23.7884134212384,4.89582956706775,0.));
#214711=CARTESIAN_POINT('Ctrl Pts',(23.7884134212384,4.89582956706775,12.));
#214712=CARTESIAN_POINT('Ctrl Pts',(23.7694565448049,4.88335766525573,0.));
#214713=CARTESIAN_POINT('Ctrl Pts',(23.7694565448049,4.88335766525573,12.));
#214714=CARTESIAN_POINT('Ctrl Pts',(23.7505466018245,4.87098503527152,0.));
#214715=CARTESIAN_POINT('Ctrl Pts',(23.7505466018245,4.87098503527152,12.));
#214716=CARTESIAN_POINT('Ctrl Pts',(23.7316843367313,4.85871174865499,0.));
#214717=CARTESIAN_POINT('Ctrl Pts',(23.7316843367313,4.85871174865499,12.));
#214718=CARTESIAN_POINT('Ctrl Pts',(23.7128705015017,4.84653787616426,0.));
#214719=CARTESIAN_POINT('Ctrl Pts',(23.7128705015017,4.84653787616426,12.));
#214720=CARTESIAN_POINT('Ctrl Pts',(23.6941058557971,4.83446348776266,0.));
#214721=CARTESIAN_POINT('Ctrl Pts',(23.6941058557971,4.83446348776266,12.));
#214722=CARTESIAN_POINT('Ctrl Pts',(23.675391167102,4.82248865259562,0.));
#214723=CARTESIAN_POINT('Ctrl Pts',(23.675391167102,4.82248865259562,12.));
#214724=CARTESIAN_POINT('Ctrl Pts',(23.6567272108628,4.81061343896432,0.));
#214725=CARTESIAN_POINT('Ctrl Pts',(23.6567272108628,4.81061343896432,12.));
#214726=CARTESIAN_POINT('Ctrl Pts',(23.6381147706579,4.7988379143322,0.));
#214727=CARTESIAN_POINT('Ctrl Pts',(23.6381147706579,4.7988379143322,12.));
#214728=CARTESIAN_POINT('Ctrl Pts',(23.6195546383624,4.78716214532098,0.));
#214729=CARTESIAN_POINT('Ctrl Pts',(23.6195546383624,4.78716214532098,12.));
#214730=CARTESIAN_POINT('Ctrl Pts',(23.6010476143099,4.77558619769872,0.));
#214731=CARTESIAN_POINT('Ctrl Pts',(23.6010476143099,4.77558619769872,12.));
#214732=CARTESIAN_POINT('Ctrl Pts',(23.5825945074535,4.76411013636251,0.));
#214733=CARTESIAN_POINT('Ctrl Pts',(23.5825945074535,4.76411013636251,12.));
#214734=CARTESIAN_POINT('Ctrl Pts',(23.5641961355168,4.75273402530617,0.));
#214735=CARTESIAN_POINT('Ctrl Pts',(23.5641961355168,4.75273402530617,12.));
#214736=CARTESIAN_POINT('Ctrl Pts',(23.545853325171,4.74145792760699,0.));
#214737=CARTESIAN_POINT('Ctrl Pts',(23.545853325171,4.74145792760699,12.));
#214738=CARTESIAN_POINT('Ctrl Pts',(23.5275669122372,4.7302819054303,0.));
#214739=CARTESIAN_POINT('Ctrl Pts',(23.5275669122372,4.7302819054303,12.));
#214740=CARTESIAN_POINT('Ctrl Pts',(23.509337741878,4.71920602001902,0.));
#214741=CARTESIAN_POINT('Ctrl Pts',(23.509337741878,4.71920602001902,12.));
#214742=CARTESIAN_POINT('Ctrl Pts',(23.491166668789,4.70823033167819,0.));
#214743=CARTESIAN_POINT('Ctrl Pts',(23.491166668789,4.70823033167819,12.));
#214744=CARTESIAN_POINT('Ctrl Pts',(23.4730545573853,4.69735489975024,0.));
#214745=CARTESIAN_POINT('Ctrl Pts',(23.4730545573853,4.69735489975024,12.));
#214746=CARTESIAN_POINT('Ctrl Pts',(23.455002281986,4.68657978258303,0.));
#214747=CARTESIAN_POINT('Ctrl Pts',(23.455002281986,4.68657978258303,12.));
#214748=CARTESIAN_POINT('Ctrl Pts',(23.4370107270451,4.67590503753059,0.));
#214749=CARTESIAN_POINT('Ctrl Pts',(23.4370107270451,4.67590503753059,12.));
#214750=CARTESIAN_POINT('Ctrl Pts',(23.4190807873803,4.6653307209467,0.));
#214751=CARTESIAN_POINT('Ctrl Pts',(23.4190807873803,4.6653307209467,12.));
#214752=CARTESIAN_POINT('Ctrl Pts',(23.4012133683959,4.65485688816924,0.));
#214753=CARTESIAN_POINT('Ctrl Pts',(23.4012133683959,4.65485688816924,12.));
#214754=CARTESIAN_POINT('Ctrl Pts',(23.3834093863068,4.6444835934993,0.));
#214755=CARTESIAN_POINT('Ctrl Pts',(23.3834093863068,4.6444835934993,12.));
#214756=CARTESIAN_POINT('Ctrl Pts',(23.3656697683489,4.63421089016541,0.));
#214757=CARTESIAN_POINT('Ctrl Pts',(23.3656697683489,4.63421089016541,12.));
#214758=CARTESIAN_POINT('Ctrl Pts',(23.3479954530272,4.62403883030805,0.));
#214759=CARTESIAN_POINT('Ctrl Pts',(23.3479954530272,4.62403883030805,12.));
#214760=CARTESIAN_POINT('Ctrl Pts',(23.3303873903938,4.6139674649783,0.));
#214761=CARTESIAN_POINT('Ctrl Pts',(23.3303873903938,4.6139674649783,12.));
#214762=CARTESIAN_POINT('Ctrl Pts',(23.3128465423115,4.60399684412163,0.));
#214763=CARTESIAN_POINT('Ctrl Pts',(23.3128465423115,4.60399684412163,12.));
#214764=CARTESIAN_POINT('Ctrl Pts',(23.2953738827191,4.5941270165575,0.));
#214765=CARTESIAN_POINT('Ctrl Pts',(23.2953738827191,4.5941270165575,12.));
#214766=CARTESIAN_POINT('Ctrl Pts',(23.2779703978876,4.5843580299469,0.));
#214767=CARTESIAN_POINT('Ctrl Pts',(23.2779703978876,4.5843580299469,12.));
#214768=CARTESIAN_POINT('Ctrl Pts',(23.2606370866866,4.57468993076097,0.));
#214769=CARTESIAN_POINT('Ctrl Pts',(23.2606370866866,4.57468993076097,12.));
#214770=CARTESIAN_POINT('Ctrl Pts',(23.2433749609131,4.56512276427839,0.));
#214771=CARTESIAN_POINT('Ctrl Pts',(23.2433749609131,4.56512276427839,12.));
#214772=CARTESIAN_POINT('Ctrl Pts',(23.2261850456064,4.55565657456975,0.));
#214773=CARTESIAN_POINT('Ctrl Pts',(23.2261850456064,4.55565657456975,12.));
#214774=CARTESIAN_POINT('Ctrl Pts',(23.2090683793629,4.54629140447544,0.));
#214775=CARTESIAN_POINT('Ctrl Pts',(23.2090683793629,4.54629140447544,12.));
#214776=CARTESIAN_POINT('Ctrl Pts',(23.1920260146465,4.53702729557566,0.));
#214777=CARTESIAN_POINT('Ctrl Pts',(23.1920260146465,4.53702729557566,12.));
#214778=CARTESIAN_POINT('Ctrl Pts',(23.1750590180908,4.52786428815015,0.));
#214779=CARTESIAN_POINT('Ctrl Pts',(23.1750590180908,4.52786428815015,12.));
#214780=CARTESIAN_POINT('Ctrl Pts',(23.1581684708761,4.51880242116748,0.));
#214781=CARTESIAN_POINT('Ctrl Pts',(23.1581684708761,4.51880242116748,12.));
#214782=CARTESIAN_POINT('Ctrl Pts',(23.1413554691123,4.5098417322706,0.));
#214783=CARTESIAN_POINT('Ctrl Pts',(23.1413554691123,4.5098417322706,12.));
#214784=CARTESIAN_POINT('Ctrl Pts',(23.1246211242115,4.50098225775171,0.));
#214785=CARTESIAN_POINT('Ctrl Pts',(23.1246211242115,4.50098225775171,12.));
#214786=CARTESIAN_POINT('Ctrl Pts',(23.1079665632636,4.49222403252216,0.));
#214787=CARTESIAN_POINT('Ctrl Pts',(23.1079665632636,4.49222403252216,12.));
#214788=CARTESIAN_POINT('Ctrl Pts',(23.0913929293922,4.48356709006788,0.));
#214789=CARTESIAN_POINT('Ctrl Pts',(23.0913929293922,4.48356709006788,12.));
#214790=CARTESIAN_POINT('Ctrl Pts',(23.0749013821881,4.47501146242856,0.));
#214791=CARTESIAN_POINT('Ctrl Pts',(23.0749013821881,4.47501146242856,12.));
#214792=CARTESIAN_POINT('Ctrl Pts',(23.0584930981732,4.46655718018231,0.));
#214793=CARTESIAN_POINT('Ctrl Pts',(23.0584930981732,4.46655718018231,12.));
#214794=CARTESIAN_POINT('Ctrl Pts',(23.0421692712467,4.45820427241683,0.));
#214795=CARTESIAN_POINT('Ctrl Pts',(23.0421692712467,4.45820427241683,12.));
#214796=CARTESIAN_POINT('Ctrl Pts',(23.0259311131392,4.44995276669687,0.));
#214797=CARTESIAN_POINT('Ctrl Pts',(23.0259311131392,4.44995276669687,12.));
#214798=CARTESIAN_POINT('Ctrl Pts',(23.0097798538395,4.44180268901643,0.));
#214799=CARTESIAN_POINT('Ctrl Pts',(23.0097798538395,4.44180268901643,12.));
#214800=CARTESIAN_POINT('Ctrl Pts',(22.9937167421006,4.43375406376879,0.));
#214801=CARTESIAN_POINT('Ctrl Pts',(22.9937167421006,4.43375406376879,12.));
#214802=CARTESIAN_POINT('Ctrl Pts',(22.977743046002,4.42580691372752,0.));
#214803=CARTESIAN_POINT('Ctrl Pts',(22.977743046002,4.42580691372752,12.));
#214804=CARTESIAN_POINT('Ctrl Pts',(22.9618600534866,4.41796126001302,0.));
#214805=CARTESIAN_POINT('Ctrl Pts',(22.9618600534866,4.41796126001302,12.));
#214806=CARTESIAN_POINT('Ctrl Pts',(22.9460690729093,4.41021712205554,0.));
#214807=CARTESIAN_POINT('Ctrl Pts',(22.9460690729093,4.41021712205554,12.));
#214808=CARTESIAN_POINT('Ctrl Pts',(22.930371433555,4.40257451754324,0.));
#214809=CARTESIAN_POINT('Ctrl Pts',(22.930371433555,4.40257451754324,12.));
#214810=CARTESIAN_POINT('Ctrl Pts',(22.9147684862426,4.39503346238473,0.));
#214811=CARTESIAN_POINT('Ctrl Pts',(22.9147684862426,4.39503346238473,12.));
#214812=CARTESIAN_POINT('Ctrl Pts',(22.8992616040108,4.38759397068406,0.));
#214813=CARTESIAN_POINT('Ctrl Pts',(22.8992616040108,4.38759397068406,12.));
#214814=CARTESIAN_POINT('Ctrl Pts',(22.8838521827701,4.38025605470093,0.));
#214815=CARTESIAN_POINT('Ctrl Pts',(22.8838521827701,4.38025605470093,12.));
#214816=CARTESIAN_POINT('Ctrl Pts',(22.8685416419725,4.37301972480746,0.));
#214817=CARTESIAN_POINT('Ctrl Pts',(22.8685416419725,4.37301972480746,12.));
#214818=CARTESIAN_POINT('Ctrl Pts',(22.8533314252422,4.36588498942997,0.));
#214819=CARTESIAN_POINT('Ctrl Pts',(22.8533314252422,4.36588498942997,12.));
#214820=CARTESIAN_POINT('Ctrl Pts',(22.8382230011184,4.35885185500546,0.));
#214821=CARTESIAN_POINT('Ctrl Pts',(22.8382230011184,4.35885185500546,12.));
#214822=CARTESIAN_POINT('Ctrl Pts',(22.8232178638876,4.35192032594791,0.));
#214823=CARTESIAN_POINT('Ctrl Pts',(22.8232178638876,4.35192032594791,12.));
#214824=CARTESIAN_POINT('Ctrl Pts',(22.8083175343791,4.34509040460062,0.));
#214825=CARTESIAN_POINT('Ctrl Pts',(22.8083175343791,4.34509040460062,12.));
#214826=CARTESIAN_POINT('Ctrl Pts',(22.7935235607806,4.33836209118446,0.));
#214827=CARTESIAN_POINT('Ctrl Pts',(22.7935235607806,4.33836209118446,12.));
#214828=CARTESIAN_POINT('Ctrl Pts',(22.7788375194076,4.3317353837319,0.));
#214829=CARTESIAN_POINT('Ctrl Pts',(22.7788375194076,4.3317353837319,12.));
#214830=CARTESIAN_POINT('Ctrl Pts',(22.7642610156475,4.32521027803754,0.));
#214831=CARTESIAN_POINT('Ctrl Pts',(22.7642610156475,4.32521027803754,12.));
#214832=CARTESIAN_POINT('Ctrl Pts',(22.7497956849848,4.31878676761235,0.));
#214833=CARTESIAN_POINT('Ctrl Pts',(22.7497956849848,4.31878676761235,12.));
#214834=CARTESIAN_POINT('Ctrl Pts',(22.7354431939926,4.31246484362549,0.));
#214835=CARTESIAN_POINT('Ctrl Pts',(22.7354431939926,4.31246484362549,12.));
#214836=CARTESIAN_POINT('Ctrl Pts',(22.7212052413386,4.30624449484069,0.));
#214837=CARTESIAN_POINT('Ctrl Pts',(22.7212052413386,4.30624449484069,12.));
#214838=CARTESIAN_POINT('Ctrl Pts',(22.7070835587564,4.3001257075406,0.));
#214839=CARTESIAN_POINT('Ctrl Pts',(22.7070835587564,4.3001257075406,12.));
#214840=CARTESIAN_POINT('Ctrl Pts',(22.6930799122548,4.29410846547056,0.));
#214841=CARTESIAN_POINT('Ctrl Pts',(22.6930799122548,4.29410846547056,12.));
#214842=CARTESIAN_POINT('Ctrl Pts',(22.6791961033537,4.28819274977763,0.));
#214843=CARTESIAN_POINT('Ctrl Pts',(22.6791961033537,4.28819274977763,12.));
#214844=CARTESIAN_POINT('Ctrl Pts',(22.6654339703109,4.28237853894059,0.));
#214845=CARTESIAN_POINT('Ctrl Pts',(22.6654339703109,4.28237853894059,12.));
#214846=CARTESIAN_POINT('Ctrl Pts',(22.6517953893303,4.2766658086912,0.));
#214847=CARTESIAN_POINT('Ctrl Pts',(22.6517953893303,4.2766658086912,12.));
#214848=CARTESIAN_POINT('Ctrl Pts',(22.6382822758172,4.27105453193004,0.));
#214849=CARTESIAN_POINT('Ctrl Pts',(22.6382822758172,4.27105453193004,12.));
#214850=CARTESIAN_POINT('Ctrl Pts',(22.6248965859977,4.26554467865576,0.));
#214851=CARTESIAN_POINT('Ctrl Pts',(22.6248965859977,4.26554467865576,12.));
#214852=CARTESIAN_POINT('Ctrl Pts',(22.6116403184821,4.26013621588305,0.));
#214853=CARTESIAN_POINT('Ctrl Pts',(22.6116403184821,4.26013621588305,12.));
#214854=CARTESIAN_POINT('Ctrl Pts',(22.5985155158636,4.25482910755481,0.));
#214855=CARTESIAN_POINT('Ctrl Pts',(22.5985155158636,4.25482910755481,12.));
#214856=CARTESIAN_POINT('Ctrl Pts',(22.5855242662477,4.24962331444177,0.));
#214857=CARTESIAN_POINT('Ctrl Pts',(22.5855242662477,4.24962331444177,12.));
#214858=CARTESIAN_POINT('Ctrl Pts',(22.572668704992,4.24451879404851,0.));
#214859=CARTESIAN_POINT('Ctrl Pts',(22.572668704992,4.24451879404851,12.));
#214860=CARTESIAN_POINT('Ctrl Pts',(22.5599510166429,4.23951550052523,0.));
#214861=CARTESIAN_POINT('Ctrl Pts',(22.5599510166429,4.23951550052523,12.));
#214862=CARTESIAN_POINT('Ctrl Pts',(22.5473734368086,4.23461338456712,0.));
#214863=CARTESIAN_POINT('Ctrl Pts',(22.5473734368086,4.23461338456712,12.));
#214864=CARTESIAN_POINT('Ctrl Pts',(22.5349382540588,4.22981239330733,0.));
#214865=CARTESIAN_POINT('Ctrl Pts',(22.5349382540588,4.22981239330733,12.));
#214866=CARTESIAN_POINT('Ctrl Pts',(22.5226478117886,4.22511247020041,0.));
#214867=CARTESIAN_POINT('Ctrl Pts',(22.5226478117886,4.22511247020041,12.));
#214868=CARTESIAN_POINT('Ctrl Pts',(22.5105045108881,4.22051355490196,0.));
#214869=CARTESIAN_POINT('Ctrl Pts',(22.5105045108881,4.22051355490196,12.));
#214870=CARTESIAN_POINT('Ctrl Pts',(22.4985108124228,4.21601558313906,0.));
#214871=CARTESIAN_POINT('Ctrl Pts',(22.4985108124228,4.21601558313906,12.));
#214872=CARTESIAN_POINT('Ctrl Pts',(22.4866692403147,4.21161848657428,0.));
#214873=CARTESIAN_POINT('Ctrl Pts',(22.4866692403147,4.21161848657428,12.));
#214874=CARTESIAN_POINT('Ctrl Pts',(22.4749823839917,4.20732219265649,0.));
#214875=CARTESIAN_POINT('Ctrl Pts',(22.4749823839917,4.20732219265649,12.));
#214876=CARTESIAN_POINT('Ctrl Pts',(22.4634529011437,4.20312662448174,0.));
#214877=CARTESIAN_POINT('Ctrl Pts',(22.4634529011437,4.20312662448174,12.));
#214878=CARTESIAN_POINT('Ctrl Pts',(22.4520835205422,4.19903170066358,0.));
#214879=CARTESIAN_POINT('Ctrl Pts',(22.4520835205422,4.19903170066358,12.));
#214880=CARTESIAN_POINT('Ctrl Pts',(22.4408770448917,4.1950373351886,0.));
#214881=CARTESIAN_POINT('Ctrl Pts',(22.4408770448917,4.1950373351886,12.));
#214882=CARTESIAN_POINT('Ctrl Pts',(22.4298363535416,4.19114343726932,0.));
#214883=CARTESIAN_POINT('Ctrl Pts',(22.4298363535416,4.19114343726932,12.));
#214884=CARTESIAN_POINT('Ctrl Pts',(22.4189644056109,4.18734991117707,0.));
#214885=CARTESIAN_POINT('Ctrl Pts',(22.4189644056109,4.18734991117707,12.));
#214886=CARTESIAN_POINT('Ctrl Pts',(22.4082642454448,4.18365665600839,0.));
#214887=CARTESIAN_POINT('Ctrl Pts',(22.4082642454448,4.18365665600839,12.));
#214888=CARTESIAN_POINT('Ctrl Pts',(22.3977390078074,4.18006356544879,0.));
#214889=CARTESIAN_POINT('Ctrl Pts',(22.3977390078074,4.18006356544879,12.));
#214890=CARTESIAN_POINT('Ctrl Pts',(22.3873919231339,4.17657052752834,0.));
#214891=CARTESIAN_POINT('Ctrl Pts',(22.3873919231339,4.17657052752834,12.));
#214892=CARTESIAN_POINT('Ctrl Pts',(22.3772263228624,4.17317742436162,0.));
#214893=CARTESIAN_POINT('Ctrl Pts',(22.3772263228624,4.17317742436162,12.));
#214894=CARTESIAN_POINT('Ctrl Pts',(22.3672456427605,4.1698841319947,0.));
#214895=CARTESIAN_POINT('Ctrl Pts',(22.3672456427605,4.1698841319947,12.));
#214896=CARTESIAN_POINT('Ctrl Pts',(22.3574534257397,4.16669052026602,0.));
#214897=CARTESIAN_POINT('Ctrl Pts',(22.3574534257397,4.16669052026602,12.));
#214898=CARTESIAN_POINT('Ctrl Pts',(22.3478533253886,4.1635964526318,0.));
#214899=CARTESIAN_POINT('Ctrl Pts',(22.3478533253886,4.1635964526318,12.));
#214900=CARTESIAN_POINT('Ctrl Pts',(22.3384491078599,4.16060178604154,0.));
#214901=CARTESIAN_POINT('Ctrl Pts',(22.3384491078599,4.16060178604154,12.));
#214902=CARTESIAN_POINT('Ctrl Pts',(22.3292446628957,4.15770637047882,0.));
#214903=CARTESIAN_POINT('Ctrl Pts',(22.3292446628957,4.15770637047882,12.));
#214904=CARTESIAN_POINT('Ctrl Pts',(22.3202440186979,4.15491004835278,0.));
#214905=CARTESIAN_POINT('Ctrl Pts',(22.3202440186979,4.15491004835278,12.));
#214906=CARTESIAN_POINT('Ctrl Pts',(22.3114513545186,4.15221265396993,0.));
#214907=CARTESIAN_POINT('Ctrl Pts',(22.3114513545186,4.15221265396993,12.));
#214908=CARTESIAN_POINT('Ctrl Pts',(22.3028710166935,4.14961401285526,0.));
#214909=CARTESIAN_POINT('Ctrl Pts',(22.3028710166935,4.14961401285526,12.));
#214910=CARTESIAN_POINT('Ctrl Pts',(22.2945075198468,4.14711394168559,0.));
#214911=CARTESIAN_POINT('Ctrl Pts',(22.2945075198468,4.14711394168559,12.));
#214912=CARTESIAN_POINT('Ctrl Pts',(22.2863655389167,4.14471224859295,0.));
#214913=CARTESIAN_POINT('Ctrl Pts',(22.2863655389167,4.14471224859295,12.));
#214914=CARTESIAN_POINT('Ctrl Pts',(22.2784499072026,4.14240873321982,0.));
#214915=CARTESIAN_POINT('Ctrl Pts',(22.2784499072026,4.14240873321982,12.));
#214916=CARTESIAN_POINT('Ctrl Pts',(22.2707656042456,4.14020318715988,0.));
#214917=CARTESIAN_POINT('Ctrl Pts',(22.2707656042456,4.14020318715988,12.));
#214918=CARTESIAN_POINT('Ctrl Pts',(22.263317791397,4.13809539255419,0.));
#214919=CARTESIAN_POINT('Ctrl Pts',(22.263317791397,4.13809539255419,12.));
#214920=CARTESIAN_POINT('Ctrl Pts',(22.2561118708422,4.13608511977226,0.));
#214921=CARTESIAN_POINT('Ctrl Pts',(22.2561118708422,4.13608511977226,12.));
#214922=CARTESIAN_POINT('Ctrl Pts',(22.2491535317789,4.13417212558809,0.));
#214923=CARTESIAN_POINT('Ctrl Pts',(22.2491535317789,4.13417212558809,12.));
#214924=CARTESIAN_POINT('Ctrl Pts',(22.2424488153523,4.1323561506016,0.));
#214925=CARTESIAN_POINT('Ctrl Pts',(22.2424488153523,4.1323561506016,12.));
#214926=CARTESIAN_POINT('Ctrl Pts',(22.2360040565534,4.13063692157499,0.));
#214927=CARTESIAN_POINT('Ctrl Pts',(22.2360040565534,4.13063692157499,12.));
#214928=CARTESIAN_POINT('Ctrl Pts',(22.2298258043947,4.12901415463379,0.));
#214929=CARTESIAN_POINT('Ctrl Pts',(22.2298258043947,4.12901415463379,12.));
#214930=CARTESIAN_POINT('Ctrl Pts',(22.2239207458781,4.127487558301,0.));
#214931=CARTESIAN_POINT('Ctrl Pts',(22.2239207458781,4.127487558301,12.));
#214932=CARTESIAN_POINT('Ctrl Pts',(22.2182956401341,4.126056836133,0.));
#214933=CARTESIAN_POINT('Ctrl Pts',(22.2182956401341,4.126056836133,12.));
#214934=CARTESIAN_POINT('Ctrl Pts',(22.2129576146671,4.12472167516602,0.));
#214935=CARTESIAN_POINT('Ctrl Pts',(22.2129576146671,4.12472167516602,12.));
#214936=CARTESIAN_POINT('Ctrl Pts',(22.2079143941719,4.12348173702025,0.));
#214937=CARTESIAN_POINT('Ctrl Pts',(22.2079143941719,4.12348173702025,12.));
#214938=CARTESIAN_POINT('Ctrl Pts',(22.2031746532106,4.12233664408237,0.));
#214939=CARTESIAN_POINT('Ctrl Pts',(22.2031746532106,4.12233664408237,12.));
#214940=CARTESIAN_POINT('Ctrl Pts',(22.1987479618246,4.12128598183533,0.));
#214941=CARTESIAN_POINT('Ctrl Pts',(22.1987479618246,4.12128598183533,12.));
#214942=CARTESIAN_POINT('Ctrl Pts',(22.1946440958098,4.12032932637738,0.));
#214943=CARTESIAN_POINT('Ctrl Pts',(22.1946440958098,4.12032932637738,12.));
#214944=CARTESIAN_POINT('Ctrl Pts',(22.1908725908525,4.11946626228623,0.));
#214945=CARTESIAN_POINT('Ctrl Pts',(22.1908725908525,4.11946626228623,12.));
#214946=CARTESIAN_POINT('Ctrl Pts',(22.1874419861496,4.11869641271752,0.));
#214947=CARTESIAN_POINT('Ctrl Pts',(22.1874419861496,4.11869641271752,12.));
#214948=CARTESIAN_POINT('Ctrl Pts',(22.1843613164855,4.11801938107464,0.));
#214949=CARTESIAN_POINT('Ctrl Pts',(22.1843613164855,4.11801938107464,12.));
#214950=CARTESIAN_POINT('Ctrl Pts',(22.1816414985788,4.11743469691765,0.));
#214951=CARTESIAN_POINT('Ctrl Pts',(22.1816414985788,4.11743469691765,12.));
#214952=CARTESIAN_POINT('Ctrl Pts',(22.179297473024,4.11694173195041,0.));
#214953=CARTESIAN_POINT('Ctrl Pts',(22.179297473024,4.11694173195041,12.));
#214954=CARTESIAN_POINT('Ctrl Pts',(22.177347426894,4.11653973150558,0.));
#214955=CARTESIAN_POINT('Ctrl Pts',(22.177347426894,4.11653973150558,12.));
#214956=CARTESIAN_POINT('Ctrl Pts',(22.1758088296598,4.11622797217066,0.));
#214957=CARTESIAN_POINT('Ctrl Pts',(22.1758088296598,4.11622797217066,12.));
#214958=CARTESIAN_POINT('Ctrl Pts',(22.1746949858773,4.11600589882768,0.));
#214959=CARTESIAN_POINT('Ctrl Pts',(22.1746949858773,4.11600589882768,12.));
#214960=CARTESIAN_POINT('Ctrl Pts',(22.174148802123,4.11589976826061,0.));
#214961=CARTESIAN_POINT('Ctrl Pts',(22.174148802123,4.11589976826061,12.));
#214962=CARTESIAN_POINT('Ctrl Pts',(22.1739341411684,4.1158603587821,0.));
#214963=CARTESIAN_POINT('Ctrl Pts',(22.1739341411684,4.1158603587821,12.));
#214964=CARTESIAN_POINT('Ctrl Pts',(22.1738776823239,4.11585194677412,0.));
#214965=CARTESIAN_POINT('Ctrl Pts',(22.1738776823239,4.11585194677412,12.));
#214966=CARTESIAN_POINT('Ctrl Pts',(22.1738711152697,4.11585220600461,0.));
#214967=CARTESIAN_POINT('Ctrl Pts',(22.1738711152697,4.11585220600461,12.));
#214968=CARTESIAN_POINT('Ctrl Pts',(22.4835757167854,1.76341220531179,0.));
#214969=CARTESIAN_POINT('Ctrl Pts',(22.4835757167854,1.76341220531179,12.));
#214970=CARTESIAN_POINT('Ctrl Pts',(22.483581992979,1.76341415538764,0.));
#214971=CARTESIAN_POINT('Ctrl Pts',(22.483581992979,1.76341415538764,12.));
#214972=CARTESIAN_POINT('Ctrl Pts',(22.4836387052232,1.7634206426357,0.));
#214973=CARTESIAN_POINT('Ctrl Pts',(22.4836387052232,1.7634206426357,12.));
#214974=CARTESIAN_POINT('Ctrl Pts',(22.4838562517069,1.76343813434565,0.));
#214975=CARTESIAN_POINT('Ctrl Pts',(22.4838562517069,1.76343813434565,12.));
#214976=CARTESIAN_POINT('Ctrl Pts',(22.4844112933129,1.76347698284792,0.));
#214977=CARTESIAN_POINT('Ctrl Pts',(22.4844112933129,1.76347698284792,12.));
#214978=CARTESIAN_POINT('Ctrl Pts',(22.4855446605991,1.76355076045546,0.));
#214979=CARTESIAN_POINT('Ctrl Pts',(22.4855446605991,1.76355076045546,12.));
#214980=CARTESIAN_POINT('Ctrl Pts',(22.4871115206571,1.76364784232963,0.));
#214981=CARTESIAN_POINT('Ctrl Pts',(22.4871115206571,1.76364784232963,12.));
#214982=CARTESIAN_POINT('Ctrl Pts',(22.4890991659478,1.76376424879505,0.));
#214983=CARTESIAN_POINT('Ctrl Pts',(22.4890991659478,1.76376424879505,12.));
#214984=CARTESIAN_POINT('Ctrl Pts',(22.4914909094908,1.76389475965724,0.));
#214985=CARTESIAN_POINT('Ctrl Pts',(22.4914909094908,1.76389475965724,12.));
#214986=CARTESIAN_POINT('Ctrl Pts',(22.4942693792449,1.76403393880301,0.));
#214987=CARTESIAN_POINT('Ctrl Pts',(22.4942693792449,1.76403393880301,12.));
#214988=CARTESIAN_POINT('Ctrl Pts',(22.4974203063191,1.76417731243462,0.));
#214989=CARTESIAN_POINT('Ctrl Pts',(22.4974203063191,1.76417731243462,12.));
#214990=CARTESIAN_POINT('Ctrl Pts',(22.5009332677316,1.76432160068726,0.));
#214991=CARTESIAN_POINT('Ctrl Pts',(22.5009332677316,1.76432160068726,12.));
#214992=CARTESIAN_POINT('Ctrl Pts',(22.5047996391978,1.76446408210366,0.));
#214993=CARTESIAN_POINT('Ctrl Pts',(22.5047996391978,1.76446408210366,12.));
#214994=CARTESIAN_POINT('Ctrl Pts',(22.5090112700212,1.76460218257323,0.));
#214995=CARTESIAN_POINT('Ctrl Pts',(22.5090112700212,1.76460218257323,12.));
#214996=CARTESIAN_POINT('Ctrl Pts',(22.5135590569554,1.76473303281159,0.));
#214997=CARTESIAN_POINT('Ctrl Pts',(22.5135590569554,1.76473303281159,12.));
#214998=CARTESIAN_POINT('Ctrl Pts',(22.5184336670207,1.76485369319896,0.));
#214999=CARTESIAN_POINT('Ctrl Pts',(22.5184336670207,1.76485369319896,12.));
#215000=CARTESIAN_POINT('Ctrl Pts',(22.5236259635515,1.76496128643369,0.));
#215001=CARTESIAN_POINT('Ctrl Pts',(22.5236259635515,1.76496128643369,12.));
#215002=CARTESIAN_POINT('Ctrl Pts',(22.529127665298,1.76505320262752,0.));
#215003=CARTESIAN_POINT('Ctrl Pts',(22.529127665298,1.76505320262752,12.));
#215004=CARTESIAN_POINT('Ctrl Pts',(22.5349313983571,1.7651271156325,0.));
#215005=CARTESIAN_POINT('Ctrl Pts',(22.5349313983571,1.7651271156325,12.));
#215006=CARTESIAN_POINT('Ctrl Pts',(22.5410303590891,1.76518087841493,0.));
#215007=CARTESIAN_POINT('Ctrl Pts',(22.5410303590891,1.76518087841493,12.));
#215008=CARTESIAN_POINT('Ctrl Pts',(22.5474180954006,1.76521245524047,0.));
#215009=CARTESIAN_POINT('Ctrl Pts',(22.5474180954006,1.76521245524047,12.));
#215010=CARTESIAN_POINT('Ctrl Pts',(22.5540882235837,1.76521983384063,0.));
#215011=CARTESIAN_POINT('Ctrl Pts',(22.5540882235837,1.76521983384063,12.));
#215012=CARTESIAN_POINT('Ctrl Pts',(22.5610344912501,1.7652010450045,0.));
#215013=CARTESIAN_POINT('Ctrl Pts',(22.5610344912501,1.7652010450045,12.));
#215014=CARTESIAN_POINT('Ctrl Pts',(22.5682508499873,1.76515418518829,0.));
#215015=CARTESIAN_POINT('Ctrl Pts',(22.5682508499873,1.76515418518829,12.));
#215016=CARTESIAN_POINT('Ctrl Pts',(22.5757315316355,1.76507744026747,0.));
#215017=CARTESIAN_POINT('Ctrl Pts',(22.5757315316355,1.76507744026747,12.));
#215018=CARTESIAN_POINT('Ctrl Pts',(22.5834711038024,1.76496910283089,0.));
#215019=CARTESIAN_POINT('Ctrl Pts',(22.5834711038024,1.76496910283089,12.));
#215020=CARTESIAN_POINT('Ctrl Pts',(22.5914644078106,1.76482755288411,0.));
#215021=CARTESIAN_POINT('Ctrl Pts',(22.5914644078106,1.76482755288411,12.));
#215022=CARTESIAN_POINT('Ctrl Pts',(22.5997065145638,1.76465124413556,0.));
#215023=CARTESIAN_POINT('Ctrl Pts',(22.5997065145638,1.76465124413556,12.));
#215024=CARTESIAN_POINT('Ctrl Pts',(22.6081926681342,1.76443868648015,0.));
#215025=CARTESIAN_POINT('Ctrl Pts',(22.6081926681342,1.76443868648015,12.));
#215026=CARTESIAN_POINT('Ctrl Pts',(22.6169182517693,1.76418843543739,0.));
#215027=CARTESIAN_POINT('Ctrl Pts',(22.6169182517693,1.76418843543739,12.));
#215028=CARTESIAN_POINT('Ctrl Pts',(22.6258787994847,1.76389909571402,0.));
#215029=CARTESIAN_POINT('Ctrl Pts',(22.6258787994847,1.76389909571402,12.));
#215030=CARTESIAN_POINT('Ctrl Pts',(22.635069997936,1.76356932176272,0.));
#215031=CARTESIAN_POINT('Ctrl Pts',(22.635069997936,1.76356932176272,12.));
#215032=CARTESIAN_POINT('Ctrl Pts',(22.6444876940425,1.76319782013914,0.));
#215033=CARTESIAN_POINT('Ctrl Pts',(22.6444876940425,1.76319782013914,12.));
#215034=CARTESIAN_POINT('Ctrl Pts',(22.6541278938413,1.76278334912559,0.));
#215035=CARTESIAN_POINT('Ctrl Pts',(22.6541278938413,1.76278334912559,12.));
#215036=CARTESIAN_POINT('Ctrl Pts',(22.6639867471756,1.76232471392568,0.));
#215037=CARTESIAN_POINT('Ctrl Pts',(22.6639867471756,1.76232471392568,12.));
#215038=CARTESIAN_POINT('Ctrl Pts',(22.6740605356699,1.76182076289525,0.));
#215039=CARTESIAN_POINT('Ctrl Pts',(22.6740605356699,1.76182076289525,12.));
#215040=CARTESIAN_POINT('Ctrl Pts',(22.6843456585245,1.76127038310613,0.));
#215041=CARTESIAN_POINT('Ctrl Pts',(22.6843456585245,1.76127038310613,12.));
#215042=CARTESIAN_POINT('Ctrl Pts',(22.6948386219843,1.76067249704884,0.));
#215043=CARTESIAN_POINT('Ctrl Pts',(22.6948386219843,1.76067249704884,12.));
#215044=CARTESIAN_POINT('Ctrl Pts',(22.7055360375481,1.76002606202399,0.));
#215045=CARTESIAN_POINT('Ctrl Pts',(22.7055360375481,1.76002606202399,12.));
#215046=CARTESIAN_POINT('Ctrl Pts',(22.7164346186007,1.75933006905924,0.));
#215047=CARTESIAN_POINT('Ctrl Pts',(22.7164346186007,1.75933006905924,12.));
#215048=CARTESIAN_POINT('Ctrl Pts',(22.7275311777305,1.75858354204635,0.));
#215049=CARTESIAN_POINT('Ctrl Pts',(22.7275311777305,1.75858354204635,12.));
#215050=CARTESIAN_POINT('Ctrl Pts',(22.7388226235565,1.75778553673249,0.));
#215051=CARTESIAN_POINT('Ctrl Pts',(22.7388226235565,1.75778553673249,12.));
#215052=CARTESIAN_POINT('Ctrl Pts',(22.7503059556455,1.75693513908911,0.));
#215053=CARTESIAN_POINT('Ctrl Pts',(22.7503059556455,1.75693513908911,12.));
#215054=CARTESIAN_POINT('Ctrl Pts',(22.7619782595013,1.75603146371641,0.));
#215055=CARTESIAN_POINT('Ctrl Pts',(22.7619782595013,1.75603146371641,12.));
#215056=CARTESIAN_POINT('Ctrl Pts',(22.7738367016115,1.75507365227127,0.));
#215057=CARTESIAN_POINT('Ctrl Pts',(22.7738367016115,1.75507365227127,12.));
#215058=CARTESIAN_POINT('Ctrl Pts',(22.7858785242358,1.7540608718293,0.));
#215059=CARTESIAN_POINT('Ctrl Pts',(22.7858785242358,1.7540608718293,12.));
#215060=CARTESIAN_POINT('Ctrl Pts',(22.7981010424312,1.75299231391461,0.));
#215061=CARTESIAN_POINT('Ctrl Pts',(22.7981010424312,1.75299231391461,12.));
#215062=CARTESIAN_POINT('Ctrl Pts',(22.8105016414712,1.7518671936559,0.));
#215063=CARTESIAN_POINT('Ctrl Pts',(22.8105016414712,1.7518671936559,12.));
#215064=CARTESIAN_POINT('Ctrl Pts',(22.8230777741285,1.75068474890884,0.));
#215065=CARTESIAN_POINT('Ctrl Pts',(22.8230777741285,1.75068474890884,12.));
#215066=CARTESIAN_POINT('Ctrl Pts',(22.8358269579854,1.74944423940117,0.));
#215067=CARTESIAN_POINT('Ctrl Pts',(22.8358269579854,1.74944423940117,12.));
#215068=CARTESIAN_POINT('Ctrl Pts',(22.8487467728075,1.74814494588492,0.));
#215069=CARTESIAN_POINT('Ctrl Pts',(22.8487467728075,1.74814494588492,12.));
#215070=CARTESIAN_POINT('Ctrl Pts',(22.8618348580234,1.74678616930663,0.));
#215071=CARTESIAN_POINT('Ctrl Pts',(22.8618348580234,1.74678616930663,12.));
#215072=CARTESIAN_POINT('Ctrl Pts',(22.8750889101696,1.745367229982,0.));
#215073=CARTESIAN_POINT('Ctrl Pts',(22.8750889101696,1.745367229982,12.));
#215074=CARTESIAN_POINT('Ctrl Pts',(22.8885066803351,1.74388746677702,0.));
#215075=CARTESIAN_POINT('Ctrl Pts',(22.8885066803351,1.74388746677702,12.));
#215076=CARTESIAN_POINT('Ctrl Pts',(22.9020859716144,1.74234623630079,0.));
#215077=CARTESIAN_POINT('Ctrl Pts',(22.9020859716144,1.74234623630079,12.));
#215078=CARTESIAN_POINT('Ctrl Pts',(22.9158246373365,1.74074291231057,0.));
#215079=CARTESIAN_POINT('Ctrl Pts',(22.9158246373365,1.74074291231057,12.));
#215080=CARTESIAN_POINT('Ctrl Pts',(22.9297205792587,1.73907688511665,0.));
#215081=CARTESIAN_POINT('Ctrl Pts',(22.9297205792587,1.73907688511665,12.));
#215082=CARTESIAN_POINT('Ctrl Pts',(22.9437717457825,1.73734756100038,0.));
#215083=CARTESIAN_POINT('Ctrl Pts',(22.9437717457825,1.73734756100038,12.));
#215084=CARTESIAN_POINT('Ctrl Pts',(22.9579761301062,1.73555436162771,0.));
#215085=CARTESIAN_POINT('Ctrl Pts',(22.9579761301062,1.73555436162771,12.));
#215086=CARTESIAN_POINT('Ctrl Pts',(22.9723317685688,1.73369672350818,0.));
#215087=CARTESIAN_POINT('Ctrl Pts',(22.9723317685688,1.73369672350818,12.));
#215088=CARTESIAN_POINT('Ctrl Pts',(22.9868367391978,1.73177409750194,0.));
#215089=CARTESIAN_POINT('Ctrl Pts',(22.9868367391978,1.73177409750194,12.));
#215090=CARTESIAN_POINT('Ctrl Pts',(23.0014891601891,1.72978594832137,0.));
#215091=CARTESIAN_POINT('Ctrl Pts',(23.0014891601891,1.72978594832137,12.));
#215092=CARTESIAN_POINT('Ctrl Pts',(23.0162871884167,1.72773175404703,0.));
#215093=CARTESIAN_POINT('Ctrl Pts',(23.0162871884167,1.72773175404703,12.));
#215094=CARTESIAN_POINT('Ctrl Pts',(23.031229017888,1.72561100564033,0.));
#215095=CARTESIAN_POINT('Ctrl Pts',(23.031229017888,1.72561100564033,12.));
#215096=CARTESIAN_POINT('Ctrl Pts',(23.0463128785528,1.72342320653731,0.));
#215097=CARTESIAN_POINT('Ctrl Pts',(23.0463128785528,1.72342320653731,12.));
#215098=CARTESIAN_POINT('Ctrl Pts',(23.0615370351559,1.72116787225981,0.));
#215099=CARTESIAN_POINT('Ctrl Pts',(23.0615370351559,1.72116787225981,12.));
#215100=CARTESIAN_POINT('Ctrl Pts',(23.0768997860709,1.71884453003027,0.));
#215101=CARTESIAN_POINT('Ctrl Pts',(23.0768997860709,1.71884453003027,12.));
#215102=CARTESIAN_POINT('Ctrl Pts',(23.0923994621216,1.71645271839311,0.));
#215103=CARTESIAN_POINT('Ctrl Pts',(23.0923994621216,1.71645271839311,12.));
#215104=CARTESIAN_POINT('Ctrl Pts',(23.1080344254291,1.71399198684725,0.));
#215105=CARTESIAN_POINT('Ctrl Pts',(23.1080344254291,1.71399198684725,12.));
#215106=CARTESIAN_POINT('Ctrl Pts',(23.1238030684929,1.71146189552192,0.));
#215107=CARTESIAN_POINT('Ctrl Pts',(23.1238030684929,1.71146189552192,12.));
#215108=CARTESIAN_POINT('Ctrl Pts',(23.1397038132358,1.7088620148546,0.));
#215109=CARTESIAN_POINT('Ctrl Pts',(23.1397038132358,1.7088620148546,12.));
#215110=CARTESIAN_POINT('Ctrl Pts',(23.1557351100613,1.70619192527847,0.));
#215111=CARTESIAN_POINT('Ctrl Pts',(23.1557351100613,1.70619192527847,12.));
#215112=CARTESIAN_POINT('Ctrl Pts',(23.1718954368749,1.70345121691259,0.));
#215113=CARTESIAN_POINT('Ctrl Pts',(23.1718954368749,1.70345121691259,12.));
#215114=CARTESIAN_POINT('Ctrl Pts',(23.1881832981848,1.70063948926988,0.));
#215115=CARTESIAN_POINT('Ctrl Pts',(23.1881832981848,1.70063948926988,12.));
#215116=CARTESIAN_POINT('Ctrl Pts',(23.2045972243765,1.69775635099425,0.));
#215117=CARTESIAN_POINT('Ctrl Pts',(23.2045972243765,1.69775635099425,12.));
#215118=CARTESIAN_POINT('Ctrl Pts',(23.2211357709374,1.69480141959946,0.));
#215119=CARTESIAN_POINT('Ctrl Pts',(23.2211357709374,1.69480141959946,12.));
#215120=CARTESIAN_POINT('Ctrl Pts',(23.2377975177014,1.69177432121716,0.));
#215121=CARTESIAN_POINT('Ctrl Pts',(23.2377975177014,1.69177432121716,12.));
#215122=CARTESIAN_POINT('Ctrl Pts',(23.2545810680536,1.6886746903491,0.));
#215123=CARTESIAN_POINT('Ctrl Pts',(23.2545810680536,1.6886746903491,12.));
#215124=CARTESIAN_POINT('Ctrl Pts',(23.2714850482245,1.68550216963275,0.));
#215125=CARTESIAN_POINT('Ctrl Pts',(23.2714850482245,1.68550216963275,12.));
#215126=CARTESIAN_POINT('Ctrl Pts',(23.2885081066949,1.68225640962181,0.));
#215127=CARTESIAN_POINT('Ctrl Pts',(23.2885081066949,1.68225640962181,12.));
#215128=CARTESIAN_POINT('Ctrl Pts',(23.3056489135611,1.67893706857123,0.));
#215129=CARTESIAN_POINT('Ctrl Pts',(23.3056489135611,1.67893706857123,12.));
#215130=CARTESIAN_POINT('Ctrl Pts',(23.3229061599145,1.67554381222988,0.));
#215131=CARTESIAN_POINT('Ctrl Pts',(23.3229061599145,1.67554381222988,12.));
#215132=CARTESIAN_POINT('Ctrl Pts',(23.3402785571866,1.67207631363905,0.));
#215133=CARTESIAN_POINT('Ctrl Pts',(23.3402785571866,1.67207631363905,12.));
#215134=CARTESIAN_POINT('Ctrl Pts',(23.3577648365747,1.66853425293978,0.));
#215135=CARTESIAN_POINT('Ctrl Pts',(23.3577648365747,1.66853425293978,12.));
#215136=CARTESIAN_POINT('Ctrl Pts',(23.375363748555,1.66491731718864,0.));
#215137=CARTESIAN_POINT('Ctrl Pts',(23.375363748555,1.66491731718864,12.));
#215138=CARTESIAN_POINT('Ctrl Pts',(23.3930740623622,1.66122520018008,0.));
#215139=CARTESIAN_POINT('Ctrl Pts',(23.3930740623622,1.66122520018008,12.));
#215140=CARTESIAN_POINT('Ctrl Pts',(23.4108945654803,1.65745760227507,0.));
#215141=CARTESIAN_POINT('Ctrl Pts',(23.4108945654803,1.65745760227507,12.));
#215142=CARTESIAN_POINT('Ctrl Pts',(23.4288240631034,1.6536142302373,0.));
#215143=CARTESIAN_POINT('Ctrl Pts',(23.4288240631034,1.6536142302373,12.));
#215144=CARTESIAN_POINT('Ctrl Pts',(23.446861377656,1.6496947970734,0.));
#215145=CARTESIAN_POINT('Ctrl Pts',(23.446861377656,1.6496947970734,12.));
#215146=CARTESIAN_POINT('Ctrl Pts',(23.4650053483919,1.64569902187608,0.));
#215147=CARTESIAN_POINT('Ctrl Pts',(23.4650053483919,1.64569902187608,12.));
#215148=CARTESIAN_POINT('Ctrl Pts',(23.4832548309638,1.64162662967525,0.));
#215149=CARTESIAN_POINT('Ctrl Pts',(23.4832548309638,1.64162662967525,12.));
#215150=CARTESIAN_POINT('Ctrl Pts',(23.5016086970006,1.63747735129474,0.));
#215151=CARTESIAN_POINT('Ctrl Pts',(23.5016086970006,1.63747735129474,12.));
#215152=CARTESIAN_POINT('Ctrl Pts',(23.5200658336624,1.63325092321731,0.));
#215153=CARTESIAN_POINT('Ctrl Pts',(23.5200658336624,1.63325092321731,12.));
#215154=CARTESIAN_POINT('Ctrl Pts',(23.5386251432278,1.62894708745231,0.));
#215155=CARTESIAN_POINT('Ctrl Pts',(23.5386251432278,1.62894708745231,12.));
#215156=CARTESIAN_POINT('Ctrl Pts',(23.5572855427617,1.62456559140072,0.));
#215157=CARTESIAN_POINT('Ctrl Pts',(23.5572855427617,1.62456559140072,12.));
#215158=CARTESIAN_POINT('Ctrl Pts',(23.5760459637608,1.62010618772869,0.));
#215159=CARTESIAN_POINT('Ctrl Pts',(23.5760459637608,1.62010618772869,12.));
#215160=CARTESIAN_POINT('Ctrl Pts',(23.5949053517996,1.61556863424697,0.));
#215161=CARTESIAN_POINT('Ctrl Pts',(23.5949053517996,1.61556863424697,12.));
#215162=CARTESIAN_POINT('Ctrl Pts',(23.6138626661644,1.61095269379773,0.));
#215163=CARTESIAN_POINT('Ctrl Pts',(23.6138626661644,1.61095269379773,12.));
#215164=CARTESIAN_POINT('Ctrl Pts',(23.6329168794916,1.60625813414666,0.));
#215165=CARTESIAN_POINT('Ctrl Pts',(23.6329168794916,1.60625813414666,12.));
#215166=CARTESIAN_POINT('Ctrl Pts',(23.6520669774863,1.60148472786588,0.));
#215167=CARTESIAN_POINT('Ctrl Pts',(23.6520669774863,1.60148472786588,12.));
#215168=CARTESIAN_POINT('Ctrl Pts',(23.6713119586302,1.59663225222459,0.));
#215169=CARTESIAN_POINT('Ctrl Pts',(23.6713119586302,1.59663225222459,12.));
#215170=CARTESIAN_POINT('Ctrl Pts',(23.6906508338832,1.59170048908631,0.));
#215171=CARTESIAN_POINT('Ctrl Pts',(23.6906508338832,1.59170048908631,12.));
#215172=CARTESIAN_POINT('Ctrl Pts',(23.7100826263835,1.58668922481222,0.));
#215173=CARTESIAN_POINT('Ctrl Pts',(23.7100826263835,1.58668922481222,12.));
#215174=CARTESIAN_POINT('Ctrl Pts',(23.7296063711308,1.58159825017362,0.));
#215175=CARTESIAN_POINT('Ctrl Pts',(23.7296063711308,1.58159825017362,12.));
#215176=CARTESIAN_POINT('Ctrl Pts',(23.7492211147369,1.57642736025251,0.));
#215177=CARTESIAN_POINT('Ctrl Pts',(23.7492211147369,1.57642736025251,12.));
#215178=CARTESIAN_POINT('Ctrl Pts',(23.7689259151869,1.57117635434412,0.));
#215179=CARTESIAN_POINT('Ctrl Pts',(23.7689259151869,1.57117635434412,12.));
#215180=CARTESIAN_POINT('Ctrl Pts',(23.788719841588,1.56584503586844,0.));
#215181=CARTESIAN_POINT('Ctrl Pts',(23.788719841588,1.56584503586844,12.));
#215182=CARTESIAN_POINT('Ctrl Pts',(23.8086019739192,1.56043321228631,0.));
#215183=CARTESIAN_POINT('Ctrl Pts',(23.8086019739192,1.56043321228631,12.));
#215184=CARTESIAN_POINT('Ctrl Pts',(23.8285714027631,1.55494069502628,0.));
#215185=CARTESIAN_POINT('Ctrl Pts',(23.8285714027631,1.55494069502628,12.));
#215186=CARTESIAN_POINT('Ctrl Pts',(23.8486272290698,1.5493672994053,0.));
#215187=CARTESIAN_POINT('Ctrl Pts',(23.8486272290698,1.5493672994053,12.));
#215188=CARTESIAN_POINT('Ctrl Pts',(23.8687685639635,1.54371284453978,0.));
#215189=CARTESIAN_POINT('Ctrl Pts',(23.8687685639635,1.54371284453978,12.));
#215190=CARTESIAN_POINT('Ctrl Pts',(23.8889945285313,1.53797715326748,0.));
#215191=CARTESIAN_POINT('Ctrl Pts',(23.8889945285313,1.53797715326748,12.));
#215192=CARTESIAN_POINT('Ctrl Pts',(23.9093042536119,1.53216005207462,0.));
#215193=CARTESIAN_POINT('Ctrl Pts',(23.9093042536119,1.53216005207462,12.));
#215194=CARTESIAN_POINT('Ctrl Pts',(23.9296968795761,1.5262613710304,0.));
#215195=CARTESIAN_POINT('Ctrl Pts',(23.9296968795761,1.5262613710304,12.));
#215196=CARTESIAN_POINT('Ctrl Pts',(23.9501715561038,1.52028094372806,0.));
#215197=CARTESIAN_POINT('Ctrl Pts',(23.9501715561038,1.52028094372806,12.));
#215198=CARTESIAN_POINT('Ctrl Pts',(23.9707274420145,1.51421860720628,0.));
#215199=CARTESIAN_POINT('Ctrl Pts',(23.9707274420145,1.51421860720628,12.));
#215200=CARTESIAN_POINT('Ctrl Pts',(23.991363705093,1.50807420187703,0.));
#215201=CARTESIAN_POINT('Ctrl Pts',(23.991363705093,1.50807420187703,12.));
#215202=CARTESIAN_POINT('Ctrl Pts',(24.0120795219086,1.50184757146099,0.));
#215203=CARTESIAN_POINT('Ctrl Pts',(24.0120795219086,1.50184757146099,12.));
#215204=CARTESIAN_POINT('Ctrl Pts',(24.0328740776331,1.49553856292798,0.));
#215205=CARTESIAN_POINT('Ctrl Pts',(24.0328740776331,1.49553856292798,12.));
#215206=CARTESIAN_POINT('Ctrl Pts',(24.053746565843,1.48914702644883,0.));
#215207=CARTESIAN_POINT('Ctrl Pts',(24.053746565843,1.48914702644883,12.));
#215208=CARTESIAN_POINT('Ctrl Pts',(24.074696188353,1.4826728153368,0.));
#215209=CARTESIAN_POINT('Ctrl Pts',(24.074696188353,1.4826728153368,12.));
#215210=CARTESIAN_POINT('Ctrl Pts',(24.0957221550782,1.47611578597742,0.));
#215211=CARTESIAN_POINT('Ctrl Pts',(24.0957221550782,1.47611578597742,12.));
#215212=CARTESIAN_POINT('Ctrl Pts',(24.1168236838827,1.46947579776992,0.));
#215213=CARTESIAN_POINT('Ctrl Pts',(24.1168236838827,1.46947579776992,12.));
#215214=CARTESIAN_POINT('Ctrl Pts',(24.1380000004272,1.46275271307398,0.));
#215215=CARTESIAN_POINT('Ctrl Pts',(24.1380000004272,1.46275271307398,12.));
#215216=CARTESIAN_POINT('Ctrl Pts',(24.1592503380105,1.45594639716314,0.));
#215217=CARTESIAN_POINT('Ctrl Pts',(24.1592503380105,1.45594639716314,12.));
#215218=CARTESIAN_POINT('Ctrl Pts',(24.1805739374033,1.44905671818721,0.));
#215219=CARTESIAN_POINT('Ctrl Pts',(24.1805739374033,1.44905671818721,12.));
#215220=CARTESIAN_POINT('Ctrl Pts',(24.2019700467214,1.44208354711074,0.));
#215221=CARTESIAN_POINT('Ctrl Pts',(24.2019700467214,1.44208354711074,12.));
#215222=CARTESIAN_POINT('Ctrl Pts',(24.2234379212978,1.43502675765502,0.));
#215223=CARTESIAN_POINT('Ctrl Pts',(24.2234379212978,1.43502675765502,12.));
#215224=CARTESIAN_POINT('Ctrl Pts',(24.2449768235485,1.42788622624851,0.));
#215225=CARTESIAN_POINT('Ctrl Pts',(24.2449768235485,1.42788622624851,12.));
#215226=CARTESIAN_POINT('Ctrl Pts',(24.2665860228357,1.42066183198252,0.));
#215227=CARTESIAN_POINT('Ctrl Pts',(24.2665860228357,1.42066183198252,12.));
#215228=CARTESIAN_POINT('Ctrl Pts',(24.2882647953214,1.41335345657685,0.));
#215229=CARTESIAN_POINT('Ctrl Pts',(24.2882647953214,1.41335345657685,12.));
#215230=CARTESIAN_POINT('Ctrl Pts',(24.3100124238316,1.40596098434341,0.));
#215231=CARTESIAN_POINT('Ctrl Pts',(24.3100124238316,1.40596098434341,12.));
#215232=CARTESIAN_POINT('Ctrl Pts',(24.3318281977647,1.3984843021281,0.));
#215233=CARTESIAN_POINT('Ctrl Pts',(24.3318281977647,1.3984843021281,12.));
#215234=CARTESIAN_POINT('Ctrl Pts',(24.3537114129877,1.3909232992639,0.));
#215235=CARTESIAN_POINT('Ctrl Pts',(24.3537114129877,1.3909232992639,12.));
#215236=CARTESIAN_POINT('Ctrl Pts',(24.37566137173,1.38327786752998,0.));
#215237=CARTESIAN_POINT('Ctrl Pts',(24.37566137173,1.38327786752998,12.));
#215238=CARTESIAN_POINT('Ctrl Pts',(24.3976773824731,1.37554790111608,0.));
#215239=CARTESIAN_POINT('Ctrl Pts',(24.3976773824731,1.37554790111608,12.));
#215240=CARTESIAN_POINT('Ctrl Pts',(24.4197587598337,1.36773329659954,0.));
#215241=CARTESIAN_POINT('Ctrl Pts',(24.4197587598337,1.36773329659954,12.));
#215242=CARTESIAN_POINT('Ctrl Pts',(24.4419048244524,1.35983395290624,0.));
#215243=CARTESIAN_POINT('Ctrl Pts',(24.4419048244524,1.35983395290624,12.));
#215244=CARTESIAN_POINT('Ctrl Pts',(24.4641149028894,1.35184977125645,0.));
#215245=CARTESIAN_POINT('Ctrl Pts',(24.4641149028894,1.35184977125645,12.));
#215246=CARTESIAN_POINT('Ctrl Pts',(24.4863883275135,1.34378065512335,0.));
#215247=CARTESIAN_POINT('Ctrl Pts',(24.4863883275135,1.34378065512335,12.));
#215248=CARTESIAN_POINT('Ctrl Pts',(24.5087244363856,1.33562651019684,0.));
#215249=CARTESIAN_POINT('Ctrl Pts',(24.5087244363856,1.33562651019684,12.));
#215250=CARTESIAN_POINT('Ctrl Pts',(24.5311225731434,1.32738724435326,0.));
#215251=CARTESIAN_POINT('Ctrl Pts',(24.5311225731434,1.32738724435326,12.));
#215252=CARTESIAN_POINT('Ctrl Pts',(24.5535820868671,1.31906276763669,0.));
#215253=CARTESIAN_POINT('Ctrl Pts',(24.5535820868671,1.31906276763669,12.));
#215254=CARTESIAN_POINT('Ctrl Pts',(24.576102332018,1.31065299222023,0.));
#215255=CARTESIAN_POINT('Ctrl Pts',(24.576102332018,1.31065299222023,12.));
#215256=CARTESIAN_POINT('Ctrl Pts',(24.5986826684025,1.30215783236364,0.));
#215257=CARTESIAN_POINT('Ctrl Pts',(24.5986826684025,1.30215783236364,12.));
#215258=CARTESIAN_POINT('Ctrl Pts',(24.6213224611228,1.29357720438108,0.));
#215259=CARTESIAN_POINT('Ctrl Pts',(24.6213224611228,1.29357720438108,12.));
#215260=CARTESIAN_POINT('Ctrl Pts',(24.6440210805278,1.28491102661514,0.));
#215261=CARTESIAN_POINT('Ctrl Pts',(24.6440210805278,1.28491102661514,12.));
#215262=CARTESIAN_POINT('Ctrl Pts',(24.666777902156,1.2761592194164,0.));
#215263=CARTESIAN_POINT('Ctrl Pts',(24.666777902156,1.2761592194164,12.));
#215264=CARTESIAN_POINT('Ctrl Pts',(24.6895923066837,1.26732170513497,0.));
#215265=CARTESIAN_POINT('Ctrl Pts',(24.6895923066837,1.26732170513497,12.));
#215266=CARTESIAN_POINT('Ctrl Pts',(24.7124636797895,1.25839840807415,0.));
#215267=CARTESIAN_POINT('Ctrl Pts',(24.7124636797895,1.25839840807415,12.));
#215268=CARTESIAN_POINT('Ctrl Pts',(24.7353914120012,1.24938925444324,0.));
#215269=CARTESIAN_POINT('Ctrl Pts',(24.7353914120012,1.24938925444324,12.));
#215270=CARTESIAN_POINT('Ctrl Pts',(24.7583748985439,1.24029417231988,0.));
#215271=CARTESIAN_POINT('Ctrl Pts',(24.7583748985439,1.24029417231988,12.));
#215272=CARTESIAN_POINT('Ctrl Pts',(24.78141353918,1.23111309161843,0.));
#215273=CARTESIAN_POINT('Ctrl Pts',(24.78141353918,1.23111309161843,12.));
#215274=CARTESIAN_POINT('Ctrl Pts',(24.8045067380536,1.22184594406527,0.));
#215275=CARTESIAN_POINT('Ctrl Pts',(24.8045067380536,1.22184594406527,12.));
#215276=CARTESIAN_POINT('Ctrl Pts',(24.8276539035092,1.21249266318205,0.));
#215277=CARTESIAN_POINT('Ctrl Pts',(24.8276539035092,1.21249266318205,12.));
#215278=CARTESIAN_POINT('Ctrl Pts',(24.8508544481973,1.20305318426016,0.));
#215279=CARTESIAN_POINT('Ctrl Pts',(24.8508544481973,1.20305318426016,12.));
#215280=CARTESIAN_POINT('Ctrl Pts',(24.8741077892074,1.19352744434059,0.));
#215281=CARTESIAN_POINT('Ctrl Pts',(24.8741077892074,1.19352744434059,12.));
#215282=CARTESIAN_POINT('Ctrl Pts',(24.8974133481829,1.18391538220098,0.));
#215283=CARTESIAN_POINT('Ctrl Pts',(24.8974133481829,1.18391538220098,12.));
#215284=CARTESIAN_POINT('Ctrl Pts',(24.9207705514449,1.1742169383504,0.));
#215285=CARTESIAN_POINT('Ctrl Pts',(24.9207705514449,1.1742169383504,12.));
#215286=CARTESIAN_POINT('Ctrl Pts',(24.9441788300932,1.16443205502852,0.));
#215287=CARTESIAN_POINT('Ctrl Pts',(24.9441788300932,1.16443205502852,12.));
#215288=CARTESIAN_POINT('Ctrl Pts',(24.9676376201501,1.15456067621894,0.));
#215289=CARTESIAN_POINT('Ctrl Pts',(24.9676376201501,1.15456067621894,12.));
#215290=CARTESIAN_POINT('Ctrl Pts',(24.9911463621431,1.14460274758206,0.));
#215291=CARTESIAN_POINT('Ctrl Pts',(24.9911463621431,1.14460274758206,12.));
#215292=CARTESIAN_POINT('Ctrl Pts',(25.0147045006193,1.13455821638536,0.));
#215293=CARTESIAN_POINT('Ctrl Pts',(25.0147045006193,1.13455821638536,12.));
#215294=CARTESIAN_POINT('Ctrl Pts',(25.0383114836898,1.12442703144455,0.));
#215295=CARTESIAN_POINT('Ctrl Pts',(25.0383114836898,1.12442703144455,12.));
#215296=CARTESIAN_POINT('Ctrl Pts',(25.0619667625336,1.1142091430689,0.));
#215297=CARTESIAN_POINT('Ctrl Pts',(25.0619667625336,1.1142091430689,12.));
#215298=CARTESIAN_POINT('Ctrl Pts',(25.085669790968,1.10390450301741,0.));
#215299=CARTESIAN_POINT('Ctrl Pts',(25.085669790968,1.10390450301741,12.));
#215300=CARTESIAN_POINT('Ctrl Pts',(25.1094200248448,1.09351306445299,0.));
#215301=CARTESIAN_POINT('Ctrl Pts',(25.1094200248448,1.09351306445299,12.));
#215302=CARTESIAN_POINT('Ctrl Pts',(25.1332169227415,1.08303478197174,0.));
#215303=CARTESIAN_POINT('Ctrl Pts',(25.1332169227415,1.08303478197174,12.));
#215304=CARTESIAN_POINT('Ctrl Pts',(25.1570599469311,1.0724696116546,0.));
#215305=CARTESIAN_POINT('Ctrl Pts',(25.1570599469311,1.0724696116546,12.));
#215306=CARTESIAN_POINT('Ctrl Pts',(25.1809485642191,1.06181751111754,0.));
#215307=CARTESIAN_POINT('Ctrl Pts',(25.1809485642191,1.06181751111754,12.));
#215308=CARTESIAN_POINT('Ctrl Pts',(25.2048822469027,1.05107843957926,0.));
#215309=CARTESIAN_POINT('Ctrl Pts',(25.2048822469027,1.05107843957926,12.));
#215310=CARTESIAN_POINT('Ctrl Pts',(25.2288604735087,1.04025235791515,0.));
#215311=CARTESIAN_POINT('Ctrl Pts',(25.2288604735087,1.04025235791515,12.));
#215312=CARTESIAN_POINT('Ctrl Pts',(25.2528827300427,1.0293392287683,0.));
#215313=CARTESIAN_POINT('Ctrl Pts',(25.2528827300427,1.0293392287683,12.));
#215314=CARTESIAN_POINT('Ctrl Pts',(25.2769485087268,1.01833901642273,0.));
#215315=CARTESIAN_POINT('Ctrl Pts',(25.2769485087268,1.01833901642273,12.));
#215316=CARTESIAN_POINT('Ctrl Pts',(25.3010573055557,1.00725168656934,0.));
#215317=CARTESIAN_POINT('Ctrl Pts',(25.3010573055557,1.00725168656934,12.));
#215318=CARTESIAN_POINT('Ctrl Pts',(25.3252086182976,0.996077206120921,
0.));
#215319=CARTESIAN_POINT('Ctrl Pts',(25.3252086182976,0.996077206120921,
12.));
#215320=CARTESIAN_POINT('Ctrl Pts',(25.3494019441444,0.984815543004091,
0.));
#215321=CARTESIAN_POINT('Ctrl Pts',(25.3494019441444,0.984815543004091,
12.));
#215322=CARTESIAN_POINT('Ctrl Pts',(25.3736367778842,0.97346666600005,0.));
#215323=CARTESIAN_POINT('Ctrl Pts',(25.3736367778842,0.97346666600005,12.));
#215324=CARTESIAN_POINT('Ctrl Pts',(25.3979126089155,0.962030544502806,
0.));
#215325=CARTESIAN_POINT('Ctrl Pts',(25.3979126089155,0.962030544502806,
12.));
#215326=CARTESIAN_POINT('Ctrl Pts',(25.4222289223155,0.950507148596971,
0.));
#215327=CARTESIAN_POINT('Ctrl Pts',(25.4222289223155,0.950507148596971,
12.));
#215328=CARTESIAN_POINT('Ctrl Pts',(25.4465852044835,0.938896449495636,
0.));
#215329=CARTESIAN_POINT('Ctrl Pts',(25.4465852044835,0.938896449495636,
12.));
#215330=CARTESIAN_POINT('Ctrl Pts',(25.4709809474996,0.927198419885607,
0.));
#215331=CARTESIAN_POINT('Ctrl Pts',(25.4709809474996,0.927198419885607,
12.));
#215332=CARTESIAN_POINT('Ctrl Pts',(25.4954156541787,0.915413034335334,
0.));
#215333=CARTESIAN_POINT('Ctrl Pts',(25.4954156541787,0.915413034335334,
12.));
#215334=CARTESIAN_POINT('Ctrl Pts',(25.5198888424195,0.903540269651155,
0.));
#215335=CARTESIAN_POINT('Ctrl Pts',(25.5198888424195,0.903540269651155,
12.));
#215336=CARTESIAN_POINT('Ctrl Pts',(25.5444000508223,0.891580105349469,
0.));
#215337=CARTESIAN_POINT('Ctrl Pts',(25.5444000508223,0.891580105349469,
12.));
#215338=CARTESIAN_POINT('Ctrl Pts',(25.568948840818,0.879532523835094,0.));
#215339=CARTESIAN_POINT('Ctrl Pts',(25.568948840818,0.879532523835094,12.));
#215340=CARTESIAN_POINT('Ctrl Pts',(25.5935347843616,0.867397509339473,
0.));
#215341=CARTESIAN_POINT('Ctrl Pts',(25.5935347843616,0.867397509339473,
12.));
#215342=CARTESIAN_POINT('Ctrl Pts',(25.618157453608,0.855175047037618,0.));
#215343=CARTESIAN_POINT('Ctrl Pts',(25.618157453608,0.855175047037618,12.));
#215344=CARTESIAN_POINT('Ctrl Pts',(25.6428164100078,0.842865122121547,
0.));
#215345=CARTESIAN_POINT('Ctrl Pts',(25.6428164100078,0.842865122121547,
12.));
#215346=CARTESIAN_POINT('Ctrl Pts',(25.6675111931957,0.83046771886437,0.));
#215347=CARTESIAN_POINT('Ctrl Pts',(25.6675111931957,0.83046771886437,12.));
#215348=CARTESIAN_POINT('Ctrl Pts',(25.6922413110172,0.817982819786722,
0.));
#215349=CARTESIAN_POINT('Ctrl Pts',(25.6922413110172,0.817982819786722,
12.));
#215350=CARTESIAN_POINT('Ctrl Pts',(25.7170062262474,0.805410404552597,
0.));
#215351=CARTESIAN_POINT('Ctrl Pts',(25.7170062262474,0.805410404552597,
12.));
#215352=CARTESIAN_POINT('Ctrl Pts',(25.7418053757671,0.792750451613538,
0.));
#215353=CARTESIAN_POINT('Ctrl Pts',(25.7418053757671,0.792750451613538,
12.));
#215354=CARTESIAN_POINT('Ctrl Pts',(25.7666381946871,0.780002940289028,
0.));
#215355=CARTESIAN_POINT('Ctrl Pts',(25.7666381946871,0.780002940289028,
12.));
#215356=CARTESIAN_POINT('Ctrl Pts',(25.7915041383304,0.767167852648643,
0.));
#215357=CARTESIAN_POINT('Ctrl Pts',(25.7915041383304,0.767167852648643,
12.));
#215358=CARTESIAN_POINT('Ctrl Pts',(25.816402705995,0.754245175608291,0.));
#215359=CARTESIAN_POINT('Ctrl Pts',(25.816402705995,0.754245175608291,12.));
#215360=CARTESIAN_POINT('Ctrl Pts',(25.841333461908,0.741234902664698,0.));
#215361=CARTESIAN_POINT('Ctrl Pts',(25.841333461908,0.741234902664698,12.));
#215362=CARTESIAN_POINT('Ctrl Pts',(25.8662960624285,0.728137036485881,
0.));
#215363=CARTESIAN_POINT('Ctrl Pts',(25.8662960624285,0.728137036485881,
12.));
#215364=CARTESIAN_POINT('Ctrl Pts',(25.8912902615141,0.714951588533756,
0.));
#215365=CARTESIAN_POINT('Ctrl Pts',(25.8912902615141,0.714951588533756,
12.));
#215366=CARTESIAN_POINT('Ctrl Pts',(25.9163158909645,0.701678575236605,
0.));
#215367=CARTESIAN_POINT('Ctrl Pts',(25.9163158909645,0.701678575236605,
12.));
#215368=CARTESIAN_POINT('Ctrl Pts',(25.941372847213,0.68831801506568,0.));
#215369=CARTESIAN_POINT('Ctrl Pts',(25.941372847213,0.68831801506568,12.));
#215370=CARTESIAN_POINT('Ctrl Pts',(25.9614434298092,0.677559543215907,
0.));
#215371=CARTESIAN_POINT('Ctrl Pts',(25.9614434298092,0.677559543215907,
12.));
#215372=CARTESIAN_POINT('Ctrl Pts',(25.9765104298171,0.669451306784419,
0.));
#215373=CARTESIAN_POINT('Ctrl Pts',(25.9765104298171,0.669451306784419,
12.));
#215374=CARTESIAN_POINT('Ctrl Pts',(25.9865613464809,0.664028313188916,
0.));
#215375=CARTESIAN_POINT('Ctrl Pts',(25.9865613464809,0.664028313188916,
12.));
#215376=CARTESIAN_POINT('Ctrl Pts',(25.991588367311,0.661312440730894,0.));
#215377=CARTESIAN_POINT('Ctrl Pts',(25.991588367311,0.661312440730894,12.));
#215378=CARTESIAN_POINT('',(25.991588367311,0.661312440730894,0.));
#215379=CARTESIAN_POINT('Origin',(0.,0.,0.));
#259187=UNCERTAINTY_MEASURE_WITH_UNIT(LENGTH_MEASURE(0.01),#259225,
'DISTANCE_ACCURACY_VALUE',
'Maximum model space distance between geometric entities at asserted c
onnectivities');
#259202=UNCERTAINTY_MEASURE_WITH_UNIT(LENGTH_MEASURE(0.01),#259225,
'DISTANCE_ACCURACY_VALUE',
'Maximum model space distance between geometric entities at asserted c
onnectivities');
#259209=(
GEOMETRIC_REPRESENTATION_CONTEXT(3)
GLOBAL_UNCERTAINTY_ASSIGNED_CONTEXT((#259187))
GLOBAL_UNIT_ASSIGNED_CONTEXT((#259225,#259227,#259228))
REPRESENTATION_CONTEXT('','3D')
);
#259224=(
GEOMETRIC_REPRESENTATION_CONTEXT(3)
GLOBAL_UNCERTAINTY_ASSIGNED_CONTEXT((#259202))
GLOBAL_UNIT_ASSIGNED_CONTEXT((#259225,#259227,#259228))
REPRESENTATION_CONTEXT('','3D')
);
#259225=(
LENGTH_UNIT()
NAMED_UNIT(*)
SI_UNIT(.MILLI.,.METRE.)
);
#259227=(
NAMED_UNIT(*)
PLANE_ANGLE_UNIT()
SI_UNIT($,.RADIAN.)
);
#259228=(
NAMED_UNIT(*)
SI_UNIT($,.STERADIAN.)
SOLID_ANGLE_UNIT()
);
#259235=SHAPE_DEFINITION_REPRESENTATION(#259256,#259375);
#259256=PRODUCT_DEFINITION_SHAPE('',$,#259397);
#259375=SHAPE_REPRESENTATION('',(#26314),#259209);
#259390=PRODUCT_DEFINITION_CONTEXT('part definition',#259455,'design');
#259397=PRODUCT_DEFINITION('Sun gear','Sun gear',#259418,#259390);
#259418=PRODUCT_DEFINITION_FORMATION('',$,#259463);
#259455=APPLICATION_CONTEXT(
'Core Data for Automotive Mechanical Design Process');
#259456=PRODUCT_CONTEXT('part definition',#259455,'mechanical');
#259463=PRODUCT('Sun gear','Sun gear',
'{"standard_geometry": "Unshifted20degree involute", "teeth": 24, "mod
ule_mm": 2, "pitch_diameter_mm": 48.0, "root_diameter_mm": 43.0, "tip_
diameter_mm": 52.0, "face_mm": 12, "per_gear_circular_tooth_thinning_m
m": 0.1, "derived_root_fillet_mm": 0.5, "involute_fit_points_per_flank
": 41, "internal": false, "source_stock": "Native reusable Gear blank;
 assembly-specific machining", "manufacturing_scope": "Standard profil
e reference; grade, cutter/root transition validation, tolerances, bac
klash and load rating require production selection."}',(#259456));
#259484=PRESENTATION_STYLE_ASSIGNMENT((#259499));
#259499=SURFACE_STYLE_USAGE(.BOTH.,#259514);
#259514=SURFACE_SIDE_STYLE('',(#259529));
#259529=SURFACE_STYLE_FILL_AREA(#259544);
#259544=FILL_AREA_STYLE('Gear light blue',(#259559));
#259559=FILL_AREA_STYLE_COLOUR('Gear light blue',#259574);
#259574=COLOUR_RGB('Gear light blue',0.662745098039216,0.831372549019608,
0.949019607843137);
ENDSEC;
END-ISO-10303-21;
